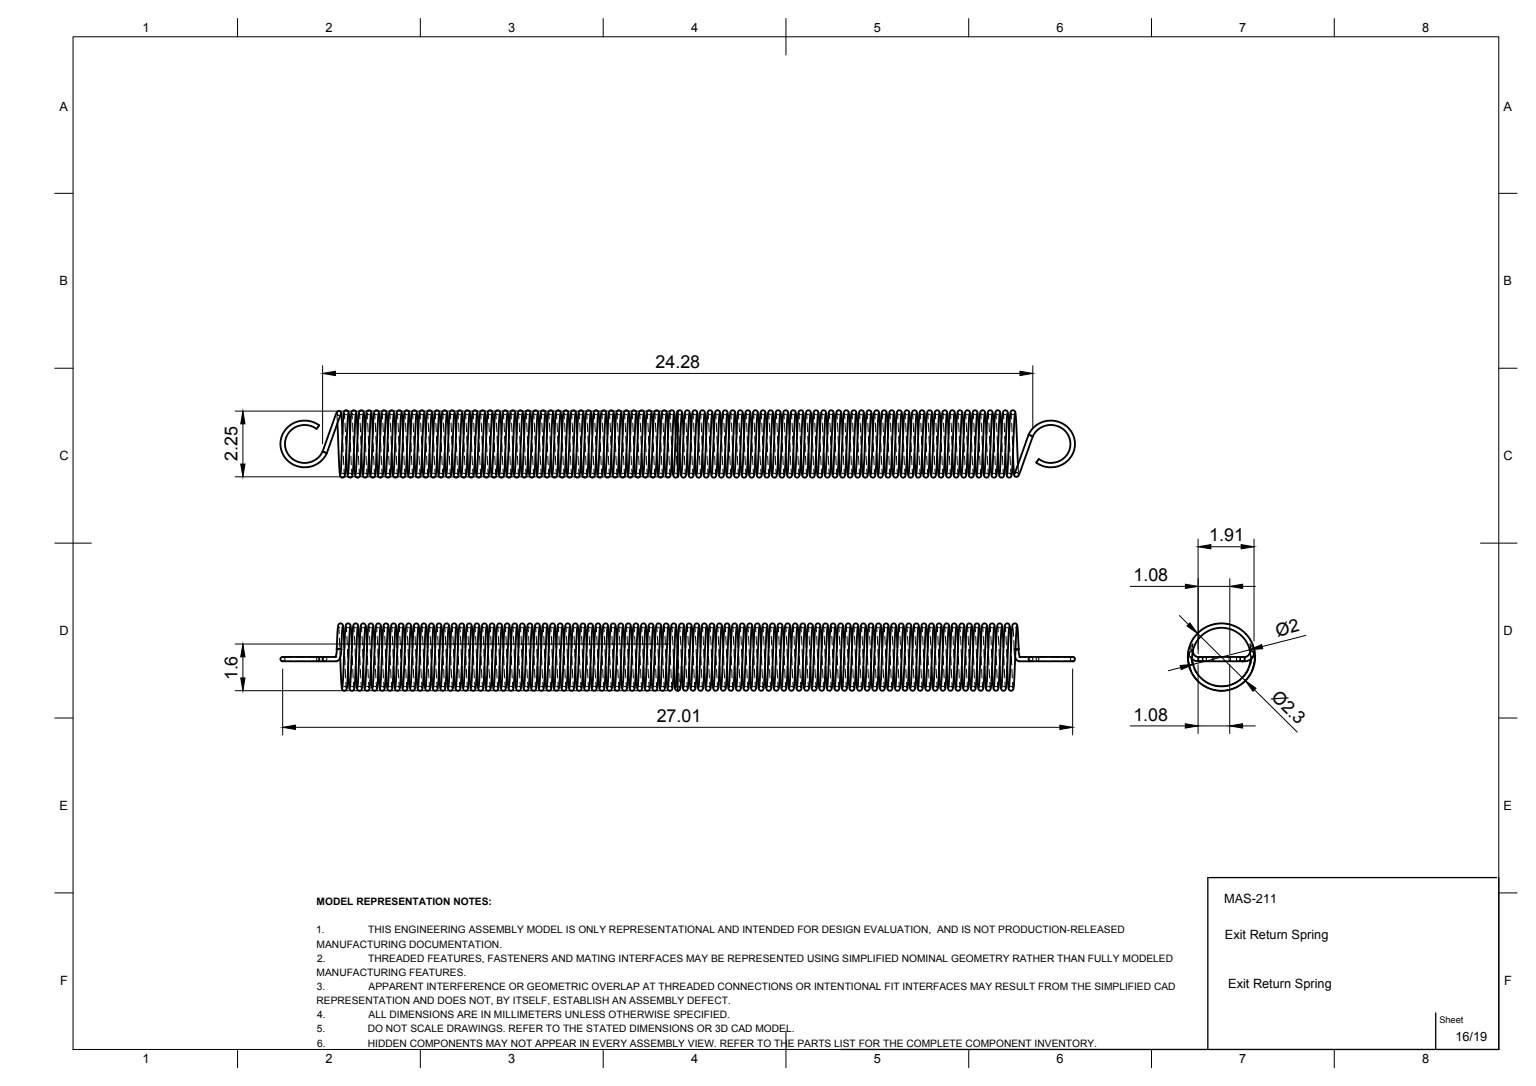
ISO-10303-21;
HEADER;
FILE_DESCRIPTION(
 (''),
 '2;1');
FILE_NAME ( 'Exit Return Spring.step', '2026-10-05T20:07:59+06:00', ( '' ), ( '' ), 'STEP AP214', 'Unspecified', '' );
FILE_SCHEMA (('AUTOMOTIVE_DESIGN { 1 0 10303 214 3 1 1 }'));
ENDSEC;
DATA;
#10=MECHANICAL_DESIGN_GEOMETRIC_PRESENTATION_REPRESENTATION('',(#334),#196741);
#27=(
BOUNDED_CURVE()
B_SPLINE_CURVE(3,(#173354,#173355,#173356,#173357,#173358,#173359,#173360,
#173361,#173362,#173363,#173364,#173365,#173366,#173367,#173368,#173369,
#173370,#173371,#173372,#173373,#173374,#173375,#173376,#173377,#173378,
#173379,#173380,#173381,#173382,#173383,#173384,#173385,#173386,#173387,
#173388,#173389,#173390,#173391,#173392,#173393,#173394,#173395,#173396,
#173397,#173398,#173399,#173400,#173401,#173402,#173403,#173404,#173405,
#173406,#173407,#173408,#173409,#173410,#173411,#173412,#173413,#173414,
#173415,#173416,#173417,#173418,#173419,#173420,#173421,#173422,#173423,
#173424,#173425,#173426,#173427,#173428,#173429,#173430,#173431,#173432,
#173433,#173434,#173435,#173436,#173437,#173438,#173439,#173440,#173441,
#173442,#173443,#173444,#173445,#173446,#173447,#173448,#173449,#173450,
#173451,#173452,#173453,#173454,#173455,#173456,#173457,#173458,#173459,
#173460,#173461,#173462,#173463,#173464,#173465,#173466,#173467,#173468,
#173469,#173470,#173471,#173472,#173473,#173474,#173475,#173476,#173477,
#173478,#173479,#173480,#173481,#173482,#173483,#173484,#173485,#173486,
#173487,#173488,#173489,#173490,#173491,#173492,#173493,#173494,#173495,
#173496,#173497,#173498,#173499,#173500,#173501,#173502,#173503,#173504,
#173505,#173506,#173507,#173508,#173509,#173510,#173511,#173512,#173513,
#173514,#173515,#173516,#173517,#173518,#173519,#173520,#173521,#173522,
#173523,#173524,#173525,#173526,#173527,#173528,#173529,#173530,#173531,
#173532,#173533,#173534,#173535,#173536,#173537,#173538,#173539,#173540,
#173541,#173542,#173543,#173544,#173545,#173546,#173547,#173548,#173549,
#173550,#173551,#173552,#173553,#173554,#173555,#173556,#173557,#173558,
#173559,#173560,#173561,#173562,#173563,#173564,#173565,#173566,#173567,
#173568,#173569,#173570,#173571,#173572,#173573,#173574,#173575,#173576,
#173577,#173578,#173579,#173580,#173581,#173582,#173583,#173584,#173585,
#173586,#173587,#173588,#173589,#173590,#173591,#173592,#173593,#173594,
#173595,#173596,#173597,#173598,#173599,#173600,#173601,#173602,#173603,
#173604,#173605,#173606,#173607,#173608,#173609,#173610,#173611,#173612,
#173613,#173614,#173615,#173616,#173617,#173618,#173619,#173620,#173621,
#173622,#173623,#173624,#173625,#173626,#173627,#173628,#173629,#173630,
#173631,#173632,#173633,#173634,#173635,#173636,#173637,#173638,#173639,
#173640,#173641,#173642,#173643,#173644,#173645,#173646,#173647,#173648,
#173649,#173650,#173651,#173652,#173653,#173654,#173655,#173656,#173657,
#173658,#173659,#173660,#173661,#173662,#173663,#173664,#173665,#173666,
#173667,#173668,#173669,#173670,#173671,#173672,#173673,#173674,#173675,
#173676,#173677,#173678,#173679,#173680,#173681,#173682,#173683,#173684,
#173685,#173686,#173687,#173688,#173689,#173690,#173691,#173692,#173693,
#173694,#173695,#173696,#173697,#173698,#173699,#173700,#173701,#173702,
#173703,#173704,#173705,#173706,#173707,#173708,#173709,#173710,#173711,
#173712,#173713,#173714,#173715,#173716,#173717,#173718,#173719,#173720,
#173721,#173722,#173723,#173724,#173725,#173726,#173727,#173728,#173729,
#173730,#173731,#173732,#173733,#173734,#173735,#173736,#173737,#173738,
#173739,#173740,#173741,#173742,#173743,#173744,#173745,#173746,#173747,
#173748,#173749,#173750,#173751,#173752,#173753,#173754,#173755,#173756,
#173757,#173758,#173759,#173760,#173761,#173762,#173763,#173764,#173765,
#173766,#173767,#173768,#173769,#173770,#173771,#173772,#173773,#173774,
#173775,#173776,#173777,#173778,#173779,#173780,#173781,#173782,#173783,
#173784,#173785,#173786,#173787,#173788,#173789,#173790,#173791,#173792,
#173793,#173794,#173795,#173796,#173797,#173798,#173799,#173800,#173801,
#173802,#173803,#173804,#173805,#173806,#173807,#173808,#173809,#173810,
#173811,#173812,#173813,#173814,#173815,#173816,#173817,#173818,#173819,
#173820,#173821,#173822,#173823,#173824,#173825,#173826,#173827,#173828,
#173829,#173830,#173831,#173832,#173833,#173834,#173835,#173836,#173837,
#173838,#173839,#173840,#173841,#173842,#173843,#173844,#173845,#173846,
#173847,#173848,#173849,#173850,#173851,#173852,#173853,#173854,#173855,
#173856,#173857,#173858,#173859,#173860,#173861,#173862,#173863,#173864,
#173865,#173866,#173867,#173868,#173869,#173870,#173871,#173872,#173873,
#173874,#173875,#173876,#173877,#173878,#173879,#173880,#173881,#173882,
#173883,#173884,#173885,#173886,#173887,#173888,#173889,#173890,#173891,
#173892,#173893,#173894,#173895,#173896,#173897,#173898,#173899,#173900,
#173901,#173902,#173903,#173904,#173905,#173906,#173907,#173908,#173909,
#173910,#173911,#173912,#173913,#173914,#173915,#173916,#173917,#173918,
#173919,#173920,#173921,#173922,#173923,#173924,#173925,#173926,#173927,
#173928,#173929,#173930,#173931,#173932,#173933,#173934,#173935,#173936,
#173937,#173938,#173939,#173940,#173941,#173942,#173943,#173944,#173945,
#173946,#173947,#173948,#173949,#173950,#173951,#173952,#173953,#173954,
#173955,#173956,#173957,#173958,#173959,#173960,#173961,#173962,#173963,
#173964,#173965,#173966,#173967,#173968,#173969,#173970,#173971,#173972,
#173973,#173974,#173975,#173976,#173977,#173978,#173979,#173980,#173981,
#173982,#173983,#173984,#173985,#173986,#173987,#173988,#173989,#173990,
#173991,#173992,#173993,#173994,#173995,#173996,#173997,#173998,#173999,
#174000,#174001,#174002,#174003,#174004,#174005,#174006,#174007,#174008,
#174009,#174010,#174011,#174012,#174013,#174014,#174015,#174016,#174017,
#174018,#174019,#174020,#174021,#174022,#174023,#174024,#174025,#174026,
#174027,#174028,#174029,#174030,#174031,#174032,#174033,#174034,#174035,
#174036,#174037,#174038,#174039,#174040,#174041,#174042,#174043,#174044,
#174045,#174046,#174047,#174048,#174049,#174050,#174051,#174052,#174053,
#174054,#174055,#174056,#174057,#174058,#174059,#174060,#174061,#174062,
#174063,#174064,#174065,#174066,#174067,#174068,#174069,#174070,#174071,
#174072,#174073,#174074,#174075,#174076,#174077,#174078,#174079,#174080,
#174081,#174082,#174083,#174084,#174085,#174086,#174087,#174088,#174089,
#174090,#174091,#174092,#174093,#174094,#174095,#174096,#174097,#174098,
#174099,#174100,#174101,#174102,#174103,#174104,#174105,#174106,#174107,
#174108,#174109,#174110,#174111,#174112,#174113,#174114,#174115,#174116,
#174117,#174118,#174119,#174120,#174121,#174122,#174123,#174124,#174125,
#174126,#174127,#174128,#174129,#174130,#174131,#174132,#174133,#174134,
#174135,#174136,#174137,#174138,#174139,#174140,#174141,#174142,#174143,
#174144,#174145,#174146,#174147,#174148,#174149,#174150,#174151,#174152,
#174153,#174154,#174155,#174156,#174157,#174158,#174159,#174160,#174161,
#174162,#174163,#174164,#174165,#174166,#174167,#174168,#174169,#174170,
#174171,#174172,#174173,#174174,#174175,#174176,#174177,#174178,#174179,
#174180,#174181,#174182,#174183,#174184,#174185,#174186,#174187,#174188,
#174189,#174190,#174191,#174192,#174193,#174194,#174195,#174196,#174197,
#174198,#174199,#174200,#174201,#174202,#174203,#174204,#174205,#174206,
#174207,#174208,#174209,#174210,#174211,#174212,#174213,#174214,#174215,
#174216,#174217,#174218,#174219,#174220,#174221,#174222,#174223,#174224,
#174225,#174226,#174227,#174228,#174229,#174230,#174231,#174232,#174233,
#174234,#174235,#174236,#174237,#174238,#174239,#174240,#174241,#174242,
#174243,#174244,#174245,#174246,#174247,#174248,#174249,#174250,#174251,
#174252,#174253,#174254,#174255,#174256,#174257,#174258,#174259,#174260,
#174261,#174262,#174263,#174264,#174265,#174266,#174267,#174268,#174269,
#174270,#174271,#174272,#174273,#174274,#174275,#174276,#174277,#174278,
#174279,#174280,#174281,#174282,#174283,#174284,#174285,#174286,#174287,
#174288,#174289,#174290,#174291,#174292,#174293,#174294,#174295,#174296,
#174297,#174298,#174299,#174300,#174301,#174302,#174303,#174304,#174305,
#174306,#174307,#174308,#174309,#174310,#174311,#174312,#174313,#174314,
#174315,#174316,#174317,#174318,#174319,#174320,#174321,#174322,#174323,
#174324,#174325,#174326,#174327,#174328,#174329,#174330,#174331,#174332,
#174333,#174334,#174335,#174336,#174337,#174338,#174339,#174340,#174341,
#174342,#174343,#174344,#174345,#174346,#174347,#174348,#174349,#174350,
#174351,#174352,#174353,#174354,#174355,#174356,#174357,#174358,#174359,
#174360,#174361,#174362,#174363,#174364,#174365,#174366,#174367,#174368,
#174369,#174370,#174371,#174372,#174373,#174374,#174375,#174376,#174377,
#174378,#174379,#174380,#174381,#174382,#174383,#174384,#174385,#174386,
#174387,#174388,#174389,#174390,#174391,#174392,#174393,#174394,#174395,
#174396,#174397,#174398,#174399,#174400,#174401,#174402,#174403,#174404,
#174405,#174406,#174407,#174408,#174409,#174410,#174411),.UNSPECIFIED.,
 .F.,.F.)
B_SPLINE_CURVE_WITH_KNOTS((4,1,1,1,1,1,1,1,1,1,1,1,1,1,1,1,1,1,1,1,1,1,
1,1,1,1,1,1,1,1,1,1,1,1,1,1,1,1,1,1,1,1,1,1,1,1,1,1,1,1,1,1,1,1,1,1,1,1,
1,1,1,1,1,1,1,1,1,1,1,1,1,1,1,1,1,1,1,1,1,1,1,1,1,1,1,1,1,1,1,1,1,1,1,1,
1,1,1,1,1,1,1,1,1,1,1,1,1,1,1,1,1,1,1,1,1,1,1,1,1,1,1,1,1,1,1,1,1,1,1,1,
1,1,1,1,1,1,1,1,1,1,1,1,1,1,1,1,1,1,1,1,1,1,1,1,1,1,1,1,1,1,1,1,1,1,1,1,
1,1,1,1,1,1,1,1,1,1,1,1,1,1,1,1,1,1,1,1,1,1,1,1,1,1,1,1,1,1,1,1,1,1,1,1,
1,1,1,1,1,1,1,1,1,1,1,1,1,1,1,1,1,1,1,1,1,1,1,1,1,1,1,1,1,1,1,1,1,1,1,1,
1,1,1,1,1,1,1,1,1,1,1,1,1,1,1,1,1,1,1,1,1,1,1,1,1,1,1,1,1,1,1,1,1,1,1,1,
1,1,1,1,1,1,1,1,1,1,1,1,1,1,1,1,1,1,1,1,1,1,1,1,1,1,1,1,1,1,1,1,1,1,1,1,
1,1,1,1,1,1,1,1,1,1,1,1,1,1,1,1,1,1,1,1,1,1,1,1,1,1,1,1,1,1,1,1,1,1,1,1,
1,1,1,1,1,1,1,1,1,1,1,1,1,1,1,1,1,1,1,1,1,1,1,1,1,1,1,1,1,1,1,1,1,1,1,1,
1,1,1,1,1,1,1,1,1,1,1,1,1,1,1,1,1,1,1,1,1,1,1,1,1,1,1,1,1,1,1,1,1,1,1,1,
1,1,1,1,1,1,1,1,1,1,1,1,1,1,1,1,1,1,1,1,1,1,1,1,1,1,1,1,1,1,1,1,1,1,1,1,
1,1,1,1,1,1,1,1,1,1,1,1,1,1,1,1,1,1,1,1,1,1,1,1,1,1,1,1,1,1,1,1,1,1,1,1,
1,1,1,1,1,1,1,1,1,1,1,1,1,1,1,1,1,1,1,1,1,1,1,1,1,1,1,1,1,1,1,1,1,1,1,1,
1,1,1,1,1,1,1,1,1,1,1,1,1,1,1,1,1,1,1,1,1,1,1,1,1,1,1,1,1,1,1,1,1,1,1,1,
1,1,1,1,1,1,1,1,1,1,1,1,1,1,1,1,1,1,1,1,1,1,1,1,1,1,1,1,1,1,1,1,1,1,1,1,
1,1,1,1,1,1,1,1,1,1,1,1,1,1,1,1,1,1,1,1,1,1,1,1,1,1,1,1,1,1,1,1,1,1,1,1,
1,1,1,1,1,1,1,1,1,1,1,1,1,1,1,1,1,1,1,1,1,1,1,1,1,1,1,1,1,1,1,1,1,1,1,1,
1,1,1,1,1,1,1,1,1,1,1,1,1,1,1,1,1,1,1,1,1,1,1,1,1,1,1,1,1,1,1,1,1,1,1,1,
1,1,1,1,1,1,1,1,1,1,1,1,1,1,1,1,1,1,1,1,1,1,1,1,1,1,1,1,1,1,1,1,1,1,1,1,
1,1,1,1,1,1,1,1,1,1,1,1,1,1,1,1,1,1,1,1,1,1,1,1,1,1,1,1,1,1,1,1,1,1,1,1,
1,1,1,1,1,1,1,1,1,1,1,1,1,1,1,1,1,1,1,1,1,1,1,1,1,1,1,1,1,1,1,1,1,1,1,1,
1,1,1,1,1,1,1,1,1,1,1,1,1,1,1,1,1,1,1,1,1,1,1,1,1,1,1,1,1,1,1,1,1,1,1,1,
1,1,1,1,1,1,1,1,1,1,1,1,1,1,1,1,1,1,1,1,1,1,1,1,1,1,1,1,1,1,1,1,1,1,1,1,
1,1,1,1,1,1,1,1,1,1,1,1,1,1,1,1,1,1,1,1,1,1,1,1,1,1,1,1,1,1,1,1,1,1,1,1,
1,1,1,1,1,1,1,1,1,1,1,1,1,1,1,1,1,1,1,1,1,1,1,1,1,1,1,1,1,1,1,1,1,1,1,1,
1,1,1,1,1,1,1,1,1,1,1,1,1,1,1,1,1,1,1,1,1,1,1,1,1,1,1,1,1,1,1,1,1,1,1,1,
1,1,1,1,1,1,1,1,1,1,1,1,1,1,1,1,1,1,1,1,1,1,1,1,1,1,1,1,1,1,1,1,1,1,1,1,
1,1,1,1,1,1,1,1,1,1,1,1,1,1,1,1,1,1,1,1,1,1,1,1,1,4),(0.,0.01797683372391,
0.286633051710584,0.555289278308216,0.823945516665782,1.09260176953922,
1.36125803873948,1.62991432588463,1.89857063164012,2.16722695661301,2.43588330050525,
2.70453966304674,2.9731960431531,3.24185243981471,3.51050885133453,3.77916527610465,
4.04782171198515,4.31647815691489,4.58513460847725,4.85379106430677,5.12244752187208,
5.39110397865606,5.65976043217153,5.92841687990537,6.19707331956994,6.46572974881596,
6.73438616570634,7.00304256821933,7.2716989549161,7.5403553242696,7.809011675483,
8.07766800769526,8.34632432089157,8.61498061505147,8.8836368910788,9.15229314997201,
9.4209493936865,9.68960562442157,9.95826184531348,10.226918059948,10.4955742727586,
10.7642304884925,11.0328867113173,11.3015429448574,11.5701991918227,11.8388554546081,
12.1075117346518,12.3761680332469,12.6448243507434,12.9134806874637,13.1821370428496,
13.450793416388,13.7194498067883,13.9881062128412,14.2567626326955,14.5254190645885,
14.7940755062772,15.0627319555912,15.3313884100611,15.6000448672586,15.8687013246492,
16.1373577797,16.4060142299691,16.6746706729765,16.9433271065265,17.2119835283531,
17.4806399366567,17.7492963295502,18.0179527057767,18.286609063996,18.555265403637,
18.8239217240786,19.0925780255742,19.3612343083975,19.6298905737625,19.898546823017,
20.1672030584666,20.4358592827168,20.7045154992928,20.973171712245,21.2418279262962,
21.5104841459723,21.7791403749736,22.0477966165324,22.316452872948,22.585109146262,
22.8537654375589,23.1224217478187,23.3910780770929,23.6597344254327,23.9283907920352,
24.197047176159,24.4657035763222,24.7343599911301,25.0030164185931,25.2716728568073,
25.5403293034427,25.8089857562333,26.0776422126729,26.3462986702843,26.6149551265448,
26.8836115789212,27.1522680250308,27.4209244624423,27.6895808890659,27.9582373027346,
28.2268937018004,28.4955500845261,28.7642064498512,29.0328627966379,29.3015191245544,
29.5701754332357,29.838831723217,30.1074879950829,30.3761442503694,30.6448004907916,
30.9134567190168,31.1821129380756,31.450769151893,31.7194253649682,31.9880815819663,
32.2567378070174,32.5253940433706,32.7940502938785,33.0627065604467,33.3313628447765,
33.6000191476151,33.8686754696427,34.1373318106287,34.405988170366,34.6746445478242,
34.9433009420458,35.2119573513747,35.480613774244,35.7492702085419,36.0179266522368,
36.2865831029275,36.5552395582669,36.8238960157264,37.0925524727952,37.3612089269773,
37.6298653757534,37.8985218168153,38.1671782477952,38.4358346667239,38.7044910715485,
38.9731474607866,39.2418038328672,39.5104601869391,39.7791165220837,40.0477728382212,
40.3164291352602,40.5850854140292,40.8537416754418,41.1223979213679,41.3910541539077,
41.6597103761025,41.9283665914244,42.1970228042084,42.4656790192,42.7343352406829,
43.0029914723808,43.2716477171096,43.540303977354,43.8089602546436,44.0776165503516,
44.3462728649052,44.614929198697,44.883585551232,45.1522419220568,45.4208983099307,
45.6895547136931,45.9582111315299,46.2268675617156,46.4955240020317,46.7641804503338,
47.0328369041642,47.3014933611089,47.5701498186329,47.8388062742058,48.107462725373,
48.3761191696448,48.6447756048012,48.9134320285537,49.1820884390673,49.4507448344197,
49.7194012133072,49.9880575743413,50.2567139168934,50.5253702402807,50.7940265446884,
51.0626828303152,51.3313390982961,51.5999953498901,51.8686515873141,52.1373078130706,
52.4059640305862,52.6746202437936,52.9432764573682,53.211932675918,53.480588903259,
53.7492451427202,54.0179013967021,54.2865576673334,54.5552139557853,54.823870263115,
55.0925265894471,55.3611829348992,55.6298392987282,55.8984956802486,56.1671520780245,
56.4358084907065,56.7044649163381,56.9731213530494,57.2417777985307,57.5104342505384,
57.7790907065743,58.0477471641719,58.3164036208043,58.5850600739368,58.8537165211707,
59.1223729600609,59.39102938849,59.6596858042645,59.9283422056975,60.1969985910129,
60.4656549590995,60.7343113087676,61.0029676396243,61.2716239512389,61.540280244075,
61.808936518638,62.0775927763821,62.3462490189291,62.6149052488546,62.8835614690812,
63.1522176834332,63.4208738963055,63.6895301124163,63.9581863359981,64.2268425704115,
64.4954988186027,64.7641550825741,65.0328113641112,65.3014676640435,65.5701239831253,
65.8387803211949,66.1074366781083,66.3760930528907,66.6447494446373,66.9134058517341,
67.1820622726558,67.4507187053199,67.7193751477252,67.988031597487,68.256688052277,
68.5253445095709,68.7940009668648,69.0626574216546,69.3313138714164,69.5999703138218,
69.8686267464858,70.1372831674076,70.4059395745042,70.6745959662509,70.9432523410334,
71.2119086979469,71.4805650360164,71.7492213550982,72.0178776550306,72.2865339365675,
72.5551902005389,72.8238464487301,73.0925026831433,73.3611589067251,73.6298151228357,
73.8984713357081,74.1671275500599,74.4357837702864,74.7044400002118,74.9730962427587,
75.2417525005027,75.5104087750655,75.7790650679015,76.047721379516,76.3163777103726,
76.5850340600405,76.853690428127,77.1223468134422,77.391003214875,77.6596596306495,
77.9283160590784,78.1969724979684,78.4656289452021,78.7342853983344,79.0029418549666,
79.2715983125641,79.5402547685998,79.8089112206075,80.0775676660886,80.3462241027997,
80.6148805284312,80.8835369411131,81.1521933388889,81.4208497204091,81.689506084238,
81.9581624296899,82.2268187560219,82.4954750633515,82.7641313518033,83.0327876224345,
83.3014438764161,83.5701001158772,83.838756343218,84.1074125617677,84.3760687753422,
84.6447249885494,84.913381206065,85.1820374318212,85.4506936692451,85.719349920839,
85.9880061888197,86.2566624744465,86.5253187788541,86.7939751022413,87.0626314447932,
87.3312878058273,87.5999441847146,87.8686005800667,88.1372569905802,88.4059134143327,
88.6745698494889,88.9432262937606,89.2118827449277,89.4805392005005,89.7491956580243,
90.0178521149689,90.2865085687992,90.5551650171012,90.8238214574172,91.0924778876028,
91.3611343054394,91.6297907092016,91.8984470970753,92.1671034679,92.4357598204347,
92.7044161542264,92.9730724687798,93.2417287644878,93.5103850417773,93.7790413020216,
94.0476975467502,94.3163537784479,94.5850099999307,94.8536662149221,95.1223224277061,
95.390978643028,95.6596348652226,95.9282910977624,96.1969473436883,96.4656036051009,
96.7342598838697,97.0029161809086,97.2715724970461,97.5402288321905,97.8088851862623,
98.0775415583427,98.3461979475807,98.6148543524051,98.8835107713336,99.1521672023136,
99.4208236433754,99.6894800921513,99.9581365463333,100.226793003402,100.495449460861,
100.7641059162,101.032762366891,101.301418810586,101.570075244884,101.838731667753,
102.107388077082,102.376044471303,102.644700848761,102.913357208498,103.182013549484,
103.450669871511,103.71932617435,103.98798245868,104.256638725248,104.525294975755,
104.793951212108,105.062607437159,105.331263654157,105.599919867233,105.86857608105,
106.137232300108,106.405888528334,106.674544768756,106.943201024042,107.211857295908,
107.480513585889,107.74916989457,108.017826222487,108.286482569273,108.555138934598,
108.823795317324,109.09245171639,109.361108130058,109.629764556682,109.898420994093,
110.167077440202,110.435733892579,110.704390348839,110.97304680645,111.24170326289,
111.51035971568,111.779016162316,112.04767260053,112.316329027993,112.5849854428,
112.853641842963,113.122298227087,113.39095459369,113.659610942029,113.928267271303,
114.196923581563,114.46557987286,114.734236146174,115.002892402589,115.271548644148,
115.540204873149,115.808861092825,116.077517306876,116.346173519828,116.614829736404,
116.883485960654,117.152142196103,117.420798445358,117.689454710722,117.958110993546,
118.226767295041,118.495423615483,118.764079955123,119.032736313343,119.301392689569,
119.570049082462,119.838705490766,120.107361912592,120.376018346142,120.644674789149,
120.913331239418,121.181987694469,121.45064415186,121.719300609057,121.987957063527,
122.256613512841,122.525269954529,122.793926386422,123.062582806276,123.331239212329,
123.599895602729,123.868551976268,124.137208331653,124.405864668374,124.67452098587,
124.943177284465,125.211833564508,125.480489827294,125.749146074259,126.017802307799,
126.286458530624,126.555114746357,126.823770959168,127.092427173802,127.361083394694,
127.629739625429,127.898395869143,128.167052128037,128.435708404064,128.704364698224,
128.97302101142,129.241677343633,129.510333694846,129.7789900642,130.047646450897,
130.31630285341,130.5849592703,130.853615699547,131.122272139211,131.390928586945,
131.659585040461,131.928241497245,132.19689795481,132.46555441064,132.734210862202,
133.002867307132,133.271523743013,133.540180167783,133.808836579303,134.077492975965,
134.346149356071,134.614805718613,134.883462062505,135.152118387478,135.420774693234,
135.689430980379,135.958087249579,136.226743502453,136.49539974081,136.76405596741,
137.032712185392,137.301368398783,137.570024612174,137.838680830155,138.107337056755,
138.375993295112,138.644649547986,138.913305817186,139.181962104332,139.450618410087,
139.71927473506,139.987931078952,140.256587441494,140.525243821601,140.793900218262,
141.062556629782,141.331213054552,141.599869490433,141.868525935363,142.137182386925,
142.405838842755,142.67449530032,142.943151757104,143.21180821062,143.480464658354,
143.749121098019,144.017777527265,144.286433944155,144.555090346668,144.823746733365,
145.092403102719,145.361059453932,145.629715786145,145.898372099341,146.167028393501,
146.435684669529,146.704340928422,146.972997172137,147.241653402872,147.510309623764,
147.778965838398,148.047622051209,148.316278266943,148.584934489768,148.853590723308,
149.122246970274,149.390903233059,149.659559513103,149.928215811698,150.196872129195,
150.465528465915,150.734184821301,151.00284119484,151.27149758524,151.540153991293,
151.808810411148,152.077466843041,152.34612328473,152.614779734044,152.883436188514,
153.152092645711,153.420749103102,153.689405558153,153.958062008422,154.22671845143,
154.49537488498,154.764031306806,155.03268771511,155.301344108004,155.57000048423,
155.838656842449,156.107313182091,156.375969502532,156.644625804028,156.913282086851,
157.181938352216,157.450594601471,157.719250836921,157.987907061171,158.256563277747,
158.525219490699,158.793875704751,159.062531924427,159.331188153428,159.599844394987,
159.868500651403,160.137156924717,160.405813216014,160.674469526274,160.943125855548,
161.211782203888,161.480438570491,161.749094954615,162.017751354778,162.286407769586,
162.555064197049,162.823720635263,163.092377081899,163.361033534689,163.629689991129,
163.898346448741,164.167002905001,164.435659357378,164.704315803488,164.972972240899,
165.241628667523,165.510285081192,165.778941480257,166.047597862983,166.316254228308,
166.584910575095,166.853566903012,167.122223211693,167.390879501675,167.659535773541,
167.928192028827,168.19684826925,168.465504497475,168.734160716534,169.002816930351,
169.271473143427,169.540129360425,169.808785585476,170.077441821829,170.346098072337,
170.614754338905,170.883410623235,171.152066926074,171.420723248102,171.689379589088,
171.958035948825,172.226692326284,172.495348720505,172.764005129834,173.032661552704,
173.301317987002,173.569974430697,173.838630881388,174.107287336727,174.375943794187,
174.644600251255,174.913256705437,175.181913154214,175.450569595276,175.719226026256,
175.987882445184,176.256538850009,176.525195239247,176.793851611328,177.0625079654,
177.331164300545,177.599820616682,177.868476913721,178.137133192491,178.405789453903,
178.674445699829,178.943101932369,179.211758154564,179.480414369886,179.74907058267,
180.017726797662,180.286383019145,180.555039250843,180.823695495572,181.092351755816,
181.361008033106,181.629664328814,181.898320643368,182.16697697716,182.435633329695,
182.70428970052,182.972946088394,183.241602492156,183.510258909993,183.778915340179,
184.047571780495,184.316228228797,184.584884682628,184.853541139572,185.122197597096,
185.39085405267,185.659510503837,185.928166948109,186.196823383265,186.465479807018,
186.734136217531,187.002792612884,187.271448991771,187.540105352806,187.808761695358,
188.077418018745,188.346074323153,188.61473060878,188.883386876761,189.152043128355,
189.420699365779,189.689355591536,189.958011809051,190.226668022259,190.495324235834,
190.763980454383,191.032636681725,191.301292921186,191.569949175168,191.838605445799,
192.107261734251,192.375918041581,192.644574367913,192.913230713365,193.181887077194,
193.450543458715,193.719199856491,193.987856269173,194.256512694805,194.525169131516,
194.793825576997,195.062482029005,195.331138485041,195.599794942639,195.868451399271,
196.137107852404,196.405764299638,196.674420738528,196.943077166957,197.211733582732,
197.480389984165,197.749046369481,198.017702737567,198.286359087236,198.555015418092,
198.823671729707,199.092328022543,199.360984297106,199.62964055485,199.898296797397,
200.166953027323,200.43560924755,200.704265461902,200.972921674774,201.241577890885,
201.510234114467,201.77889034888,202.047546597072,202.316202861043,202.584859142581,
202.853515442513,203.122171761595,203.390828099665,203.659484456579,203.928140831361,
204.196797223108,204.465453630205,204.734110051127,205.002766483791,205.271422926197,
205.540079375959,205.808735830749,206.077392288043,206.346048745337,206.614705200127,
206.883361649889,207.152018092295,207.420674524959,207.689330945881,207.957987352978,
208.226643744725,208.495300119508,208.763956476421,209.032612814491,209.301269133573,
209.569925433505,209.838581715043,210.107237979014,210.375894227206,210.644550461619,
210.913206685201,211.181862901312,211.450519114184,211.719175328536,211.987831548763,
212.256487778689,212.525144021236,212.79380027898,213.062456553543,213.331112846379,
213.599769157994,213.868425488851,214.137081838519,214.405738206606,214.674394591921,
214.943050993354,215.211707409129,215.480363837558,215.749020276448,216.017676723682,
216.286333176815,216.554989633447,216.823646091045,217.092302547081,217.360958999089,
217.62961544457,217.898271881281,218.166928306913,218.435584719595,218.704241117371,
218.972897498892,219.241553862721,219.510210208173,219.778866534505,220.047522841835,
220.316179130287,220.584835400918,220.8534916549,221.122147894361,221.390804121702,
221.659460340252,221.928116553827,222.196772767034,222.46542898455,222.734085210306,
223.00274144773,223.271397699324,223.540053967305,223.808710252932,224.07736655734,
224.346022880728,224.61467922328,224.883335584314,225.151991963201,225.420648358554,
225.689304769068,225.95796119282,226.226617627977,226.495274072249,226.763930523416,
227.032586978989,227.301243436513,227.569899893458,227.838556347288,228.10721279559,
228.375869235907,228.644525666093,228.913182083929,229.181838487692,229.450494875566,
229.719151246391,229.987807598926,230.256463932718,230.525120247271,230.79377654298,
231.062432820269,231.331089080514,231.599745325243,231.868401556941,232.137057778424,
232.405713993415,232.674370206199,232.943026421521,233.211682643716,233.480338876256,
233.748995122182,234.017651383595,234.286307662364,234.554963959403,234.823620275541,
235.092276610685,235.360932964757,235.629589336838,235.898245726076,236.166902130901,
236.43555854983,236.70421498081,236.972871421872,237.241527870648,237.51018432483,
237.778840781899,238.047497239359,238.316153694698,238.584810145389,238.853466589084,
239.122123023382,239.390779446251,239.65943585558,239.928092249802,240.19674862726,
240.465404986998,240.734061327984,241.002717650011,241.27137395285,241.54003023718,
241.808686503748,242.077342754256,242.345998990609,242.614655215661,242.883311432659,
243.151967645734,243.420623859552,243.68928007861,243.957936306836,244.226592547258,
244.495248802545,244.763905074411,245.032561364392,245.301217673074,245.56987400099,
245.838530347777,246.107186713102,246.375843095828,246.644499494894,246.913155908563,
247.181812335186,247.450468772598,247.719125218708,247.987781671084,248.256438127345,
248.525094584956,248.793751041396,249.062407494187,249.331063940822,249.599720379036,
249.8683768065,250.137033221308,250.405689621471,250.674346005595,250.943002372197,
251.211658720537,251.480315049812,251.748971360071,252.017627651368,252.286283924683,
252.554940181098,252.823596422657,253.092252651658,253.360908871335,253.629565085386,
253.898221298338,254.166877514914,254.435533739165,254.704189974614,254.972846223869,
255.241502489234,255.510158772057,255.778815073553,256.047471393995,256.316127733635,
256.584784091854,256.85344046808,257.122096860973,257.390753269276,257.659409691102,
257.928066124652,258.196722567659,258.465379017928,258.734035472978,259.002691930368,
259.271348387566,259.540004842035,259.808661291349,260.077317733037,260.345974164929,
260.614630584783,260.883286990836,261.151943381235,261.420599754774,261.689256110159,
261.957912446879,262.226568764375,262.49522506297,262.763881343014,263.032537605798,
263.301193852763,263.569850086303,263.838506309127,264.107162524861,264.375818737671,
264.644474952305,264.913131173196,265.181787403931,265.450443647645,265.719099906538,
265.987756182565,266.256412476724,266.52506878992,266.793725122132,267.062381473345,
267.331037842698,267.599694229394,267.868350631907,268.137007048797,268.405663478042,
268.674319917706,268.94297636544,269.211632818955,269.480289275739,269.748945733304,
270.017602189133,270.286258640695,270.554915085624,270.823571521504,271.092227946274,
271.360884357793,271.629540754454,271.89819713456,272.166853497101,272.435509840993,
272.704166165965,272.97282247172,273.241478758865,273.510135028065,273.778791280938,
274.047447519295,274.316103745894,274.584759963875,274.853416177266,275.122072390656,
275.390728608637,275.659384835237,275.928041073593,276.196697326466,276.465353595666,
276.734009882811,277.002666188566,277.271322513539,277.53997885743,277.808635219972,
278.077291600077,278.345947996739,278.614604408258,278.883260833028,279.151917268908,
279.420573713837,279.689230165399,279.957886621228,280.226543078793,280.495199535576,
280.763855989092,281.032512436825,281.301168876489,281.569825305735,281.838481722625,
282.107138125138,282.375794511834,282.644450881187,282.9131072324,283.140531716307),
 .UNSPECIFIED.)
CURVE()
GEOMETRIC_REPRESENTATION_ITEM()
RATIONAL_B_SPLINE_CURVE((1.,1.,1.,1.,1.,1.,1.,1.,1.,1.,1.,1.,1.,1.,1.,1.,
1.,1.,1.,1.,1.,1.,1.,1.,1.,1.,1.,1.,1.,1.,1.,1.,1.,1.,1.,1.,1.,1.,1.,1.,
1.,1.,1.,1.,1.,1.,1.,1.,1.,1.,1.,1.,1.,1.,1.,1.,1.,1.,1.,1.,1.,1.,1.,1.,
1.,1.,1.,1.,1.,1.,1.,1.,1.,1.,1.,1.,1.,1.,1.,1.,1.,1.,1.,1.,1.,1.,1.,1.,
1.,1.,1.,1.,1.,1.,1.,1.,1.,1.,1.,1.,1.,1.,1.,1.,1.,1.,1.,1.,1.,1.,1.,1.,
1.,1.,1.,1.,1.,1.,1.,1.,1.,1.,1.,1.,1.,1.,1.,1.,1.,1.,1.,1.,1.,1.,1.,1.,
1.,1.,1.,1.,1.,1.,1.,1.,1.,1.,1.,1.,1.,1.,1.,1.,1.,1.,1.,1.,1.,1.,1.,1.,
1.,1.,1.,1.,1.,1.,1.,1.,1.,1.,1.,1.,1.,1.,1.,1.,1.,1.,1.,1.,1.,1.,1.,1.,
1.,1.,1.,1.,1.,1.,1.,1.,1.,1.,1.,1.,1.,1.,1.,1.,1.,1.,1.,1.,1.,1.,1.,1.,
1.,1.,1.,1.,1.,1.,1.,1.,1.,1.,1.,1.,1.,1.,1.,1.,1.,1.,1.,1.,1.,1.,1.,1.,
1.,1.,1.,1.,1.,1.,1.,1.,1.,1.,1.,1.,1.,1.,1.,1.,1.,1.,1.,1.,1.,1.,1.,1.,
1.,1.,1.,1.,1.,1.,1.,1.,1.,1.,1.,1.,1.,1.,1.,1.,1.,1.,1.,1.,1.,1.,1.,1.,
1.,1.,1.,1.,1.,1.,1.,1.,1.,1.,1.,1.,1.,1.,1.,1.,1.,1.,1.,1.,1.,1.,1.,1.,
1.,1.,1.,1.,1.,1.,1.,1.,1.,1.,1.,1.,1.,1.,1.,1.,1.,1.,1.,1.,1.,1.,1.,1.,
1.,1.,1.,1.,1.,1.,1.,1.,1.,1.,1.,1.,1.,1.,1.,1.,1.,1.,1.,1.,1.,1.,1.,1.,
1.,1.,1.,1.,1.,1.,1.,1.,1.,1.,1.,1.,1.,1.,1.,1.,1.,1.,1.,1.,1.,1.,1.,1.,
1.,1.,1.,1.,1.,1.,1.,1.,1.,1.,1.,1.,1.,1.,1.,1.,1.,1.,1.,1.,1.,1.,1.,1.,
1.,1.,1.,1.,1.,1.,1.,1.,1.,1.,1.,1.,1.,1.,1.,1.,1.,1.,1.,1.,1.,1.,1.,1.,
1.,1.,1.,1.,1.,1.,1.,1.,1.,1.,1.,1.,1.,1.,1.,1.,1.,1.,1.,1.,1.,1.,1.,1.,
1.,1.,1.,1.,1.,1.,1.,1.,1.,1.,1.,1.,1.,1.,1.,1.,1.,1.,1.,1.,1.,1.,1.,1.,
1.,1.,1.,1.,1.,1.,1.,1.,1.,1.,1.,1.,1.,1.,1.,1.,1.,1.,1.,1.,1.,1.,1.,1.,
1.,1.,1.,1.,1.,1.,1.,1.,1.,1.,1.,1.,1.,1.,1.,1.,1.,1.,1.,1.,1.,1.,1.,1.,
1.,1.,1.,1.,1.,1.,1.,1.,1.,1.,1.,1.,1.,1.,1.,1.,1.,1.,1.,1.,1.,1.,1.,1.,
1.,1.,1.,1.,1.,1.,1.,1.,1.,1.,1.,1.,1.,1.,1.,1.,1.,1.,1.,1.,1.,1.,1.,1.,
1.,1.,1.,1.,1.,1.,1.,1.,1.,1.,1.,1.,1.,1.,1.,1.,1.,1.,1.,1.,1.,1.,1.,1.,
1.,1.,1.,1.,1.,1.,1.,1.,1.,1.,1.,1.,1.,1.,1.,1.,1.,1.,1.,1.,1.,1.,1.,1.,
1.,1.,1.,1.,1.,1.,1.,1.,1.,1.,1.,1.,1.,1.,1.,1.,1.,1.,1.,1.,1.,1.,1.,1.,
1.,1.,1.,1.,1.,1.,1.,1.,1.,1.,1.,1.,1.,1.,1.,1.,1.,1.,1.,1.,1.,1.,1.,1.,
1.,1.,1.,1.,1.,1.,1.,1.,1.,1.,1.,1.,1.,1.,1.,1.,1.,1.,1.,1.,1.,1.,1.,1.,
1.,1.,1.,1.,1.,1.,1.,1.,1.,1.,1.,1.,1.,1.,1.,1.,1.,1.,1.,1.,1.,1.,1.,1.,
1.,1.,1.,1.,1.,1.,1.,1.,1.,1.,1.,1.,1.,1.,1.,1.,1.,1.,1.,1.,1.,1.,1.,1.,
1.,1.,1.,1.,1.,1.,1.,1.,1.,1.,1.,1.,1.,1.,1.,1.,1.,1.,1.,1.,1.,1.,1.,1.,
1.,1.,1.,1.,1.,1.,1.,1.,1.,1.,1.,1.,1.,1.,1.,1.,1.,1.,1.,1.,1.,1.,1.,1.,
1.,1.,1.,1.,1.,1.,1.,1.,1.,1.,1.,1.,1.,1.,1.,1.,1.,1.,1.,1.,1.,1.,1.,1.,
1.,1.,1.,1.,1.,1.,1.,1.,1.,1.,1.,1.,1.,1.,1.,1.,1.,1.,1.,1.,1.,1.,1.,1.,
1.,1.,1.,1.,1.,1.,1.,1.,1.,1.,1.,1.,1.,1.,1.,1.,1.,1.,1.,1.,1.,1.,1.,1.,
1.,1.,1.,1.,1.,1.,1.,1.,1.,1.,1.,1.,1.,1.,1.,1.,1.,1.,1.,1.,1.,1.,1.,1.,
1.,1.,1.,1.,1.,1.,1.,1.,1.,1.,1.,1.,1.,1.,1.,1.,1.,1.,1.,1.,1.,1.,1.,1.,
1.,1.,1.,1.,1.,1.,1.,1.,1.,1.,1.,1.,1.,1.,1.,1.,1.,1.,1.,1.,1.,1.,1.,1.,
1.,1.,1.,1.,1.,1.,1.,1.,1.,1.,1.,1.,1.,1.,1.,1.,1.,1.,1.,1.,1.,1.,1.,1.,
1.,1.,1.,1.,1.,1.,1.,1.,1.,1.,1.,1.,1.,1.,1.,1.,1.,1.,1.,1.,1.,1.,1.,1.,
1.,1.,1.,1.,1.,1.,1.,1.,1.,1.,1.,1.,1.,1.,1.,1.,1.,1.,1.,1.,1.,1.,1.,1.,
1.,1.,1.,1.,1.,1.,1.,1.,1.,1.,1.,1.,1.,1.,1.,1.,1.,1.,1.,1.,1.,1.,1.,1.,
1.,1.,1.,1.,1.,1.,1.,1.,1.,1.,1.,1.,1.,1.,1.,1.,1.,1.,1.,1.,1.,1.,1.,1.,
1.,1.,1.,1.,1.,1.,1.,1.,1.,1.))
REPRESENTATION_ITEM('')
) ;
#28=(
BOUNDED_CURVE()
B_SPLINE_CURVE(3,(#174481,#174482,#174483,#174484,#174485,#174486,#174487),
 .UNSPECIFIED.,.F.,.F.)
B_SPLINE_CURVE_WITH_KNOTS((4,1,1,1,4),(0.,0.0911446219616379,0.182289243923276,
0.273433865884915,0.364578487846551),.UNSPECIFIED.)
CURVE()
GEOMETRIC_REPRESENTATION_ITEM()
RATIONAL_B_SPLINE_CURVE((1.,1.,1.,1.,1.,1.,1.))
REPRESENTATION_ITEM('')
) ;
#29=(
BOUNDED_CURVE()
B_SPLINE_CURVE(3,(#174703,#174704,#174705,#174706,#174707,#174708,#174709,
#174710,#174711,#174712,#174713,#174714,#174715,#174716,#174717,#174718,
#174719,#174720,#174721),.UNSPECIFIED.,.F.,.F.)
B_SPLINE_CURVE_WITH_KNOTS((4,1,1,1,1,1,1,1,1,1,1,1,1,1,1,1,4),(0.,0.226732296973331,
0.464902013928651,0.70307173088397,0.9298040278573,1.15653632483063,1.39470604178595,
1.63287575874127,1.8596080557146,2.08634035268793,2.32451006964325,2.56267978659857,
2.7894120835719,3.01614438054523,3.25431409750055,3.49248381445586,3.7192161114292),
 .UNSPECIFIED.)
CURVE()
GEOMETRIC_REPRESENTATION_ITEM()
RATIONAL_B_SPLINE_CURVE((1.,1.,1.,1.,1.,1.,1.,1.,1.,1.,1.,1.,1.,1.,1.,1.,
1.,1.,1.))
REPRESENTATION_ITEM('')
) ;
#30=(
BOUNDED_CURVE()
B_SPLINE_CURVE(3,(#193341,#193342,#193343,#193344,#193345,#193346,#193347,
#193348,#193349,#193350,#193351,#193352,#193353,#193354,#193355,#193356,
#193357,#193358,#193359,#193360,#193361,#193362,#193363,#193364,#193365,
#193366,#193367,#193368,#193369,#193370,#193371,#193372,#193373,#193374,
#193375,#193376,#193377,#193378,#193379,#193380,#193381,#193382,#193383,
#193384,#193385,#193386,#193387,#193388,#193389,#193390,#193391,#193392,
#193393,#193394,#193395,#193396,#193397,#193398,#193399,#193400,#193401,
#193402,#193403,#193404,#193405,#193406,#193407,#193408,#193409,#193410,
#193411,#193412,#193413,#193414,#193415,#193416,#193417,#193418,#193419,
#193420,#193421,#193422,#193423,#193424,#193425,#193426,#193427,#193428,
#193429,#193430,#193431,#193432,#193433,#193434,#193435,#193436,#193437,
#193438,#193439,#193440,#193441,#193442,#193443,#193444,#193445,#193446,
#193447,#193448,#193449,#193450,#193451,#193452,#193453,#193454,#193455,
#193456,#193457,#193458,#193459,#193460,#193461,#193462,#193463,#193464,
#193465,#193466,#193467,#193468,#193469,#193470,#193471,#193472,#193473,
#193474,#193475,#193476,#193477,#193478,#193479,#193480,#193481,#193482,
#193483,#193484,#193485,#193486,#193487,#193488,#193489,#193490,#193491,
#193492,#193493,#193494,#193495,#193496,#193497,#193498,#193499,#193500,
#193501,#193502,#193503,#193504,#193505,#193506,#193507,#193508,#193509,
#193510,#193511,#193512,#193513,#193514,#193515,#193516,#193517,#193518,
#193519,#193520,#193521,#193522,#193523,#193524,#193525,#193526,#193527,
#193528,#193529,#193530,#193531,#193532,#193533,#193534,#193535,#193536,
#193537,#193538,#193539,#193540,#193541,#193542,#193543,#193544,#193545,
#193546,#193547,#193548,#193549,#193550,#193551,#193552,#193553,#193554,
#193555,#193556,#193557,#193558,#193559,#193560,#193561,#193562,#193563,
#193564,#193565,#193566,#193567,#193568,#193569,#193570,#193571,#193572,
#193573,#193574,#193575,#193576,#193577,#193578,#193579,#193580,#193581,
#193582,#193583,#193584,#193585,#193586,#193587,#193588,#193589,#193590,
#193591,#193592,#193593,#193594,#193595,#193596,#193597,#193598,#193599,
#193600,#193601,#193602,#193603,#193604,#193605,#193606,#193607,#193608,
#193609,#193610,#193611,#193612,#193613,#193614,#193615,#193616,#193617,
#193618,#193619,#193620,#193621,#193622,#193623,#193624,#193625,#193626,
#193627,#193628,#193629,#193630,#193631,#193632,#193633,#193634,#193635,
#193636,#193637,#193638,#193639,#193640,#193641,#193642,#193643,#193644,
#193645,#193646,#193647,#193648,#193649,#193650,#193651,#193652,#193653,
#193654,#193655,#193656,#193657,#193658,#193659,#193660,#193661,#193662,
#193663,#193664,#193665,#193666,#193667,#193668,#193669,#193670,#193671,
#193672,#193673,#193674,#193675,#193676,#193677,#193678,#193679,#193680,
#193681,#193682,#193683,#193684,#193685,#193686,#193687,#193688,#193689,
#193690,#193691,#193692,#193693,#193694,#193695,#193696,#193697,#193698,
#193699,#193700,#193701,#193702,#193703,#193704,#193705,#193706,#193707,
#193708,#193709,#193710,#193711,#193712,#193713,#193714,#193715,#193716,
#193717,#193718,#193719,#193720,#193721,#193722,#193723,#193724,#193725,
#193726,#193727,#193728,#193729,#193730,#193731,#193732,#193733,#193734,
#193735,#193736,#193737,#193738,#193739,#193740,#193741,#193742,#193743,
#193744,#193745,#193746,#193747,#193748,#193749,#193750,#193751,#193752,
#193753,#193754,#193755,#193756,#193757,#193758,#193759,#193760,#193761,
#193762,#193763,#193764,#193765,#193766,#193767,#193768,#193769,#193770,
#193771,#193772,#193773,#193774,#193775,#193776,#193777,#193778,#193779,
#193780,#193781,#193782,#193783,#193784,#193785,#193786,#193787,#193788,
#193789,#193790,#193791,#193792,#193793,#193794,#193795,#193796,#193797,
#193798,#193799,#193800,#193801,#193802,#193803,#193804,#193805,#193806,
#193807,#193808,#193809,#193810,#193811,#193812,#193813,#193814,#193815,
#193816,#193817,#193818,#193819,#193820,#193821,#193822,#193823,#193824,
#193825,#193826,#193827,#193828,#193829,#193830,#193831,#193832,#193833,
#193834,#193835,#193836,#193837,#193838,#193839,#193840,#193841,#193842,
#193843,#193844,#193845,#193846,#193847,#193848,#193849,#193850,#193851,
#193852,#193853,#193854,#193855,#193856,#193857,#193858,#193859,#193860,
#193861,#193862,#193863,#193864,#193865,#193866,#193867,#193868,#193869,
#193870,#193871,#193872,#193873,#193874,#193875,#193876,#193877,#193878,
#193879,#193880,#193881,#193882,#193883,#193884,#193885,#193886,#193887,
#193888,#193889,#193890,#193891,#193892,#193893,#193894,#193895,#193896,
#193897,#193898,#193899,#193900,#193901,#193902,#193903,#193904,#193905,
#193906,#193907,#193908,#193909,#193910,#193911,#193912,#193913,#193914,
#193915,#193916,#193917,#193918,#193919,#193920,#193921,#193922,#193923,
#193924,#193925,#193926,#193927,#193928,#193929,#193930,#193931,#193932,
#193933,#193934,#193935,#193936,#193937,#193938,#193939,#193940,#193941,
#193942,#193943,#193944,#193945,#193946,#193947,#193948,#193949,#193950,
#193951,#193952,#193953,#193954,#193955,#193956,#193957,#193958,#193959,
#193960,#193961,#193962,#193963,#193964,#193965,#193966,#193967,#193968,
#193969,#193970,#193971,#193972,#193973,#193974,#193975,#193976,#193977,
#193978,#193979,#193980,#193981,#193982,#193983,#193984,#193985,#193986,
#193987,#193988,#193989,#193990,#193991,#193992,#193993,#193994,#193995,
#193996,#193997,#193998,#193999,#194000,#194001,#194002,#194003,#194004,
#194005,#194006,#194007,#194008,#194009,#194010,#194011,#194012,#194013,
#194014,#194015,#194016,#194017,#194018,#194019,#194020,#194021,#194022,
#194023,#194024,#194025,#194026,#194027,#194028,#194029,#194030,#194031,
#194032,#194033,#194034,#194035,#194036,#194037,#194038,#194039,#194040,
#194041,#194042,#194043,#194044,#194045,#194046,#194047,#194048,#194049,
#194050,#194051,#194052,#194053,#194054,#194055,#194056,#194057,#194058,
#194059,#194060,#194061,#194062,#194063,#194064,#194065,#194066,#194067,
#194068,#194069,#194070,#194071,#194072,#194073,#194074,#194075,#194076,
#194077,#194078,#194079,#194080,#194081,#194082,#194083,#194084,#194085,
#194086,#194087,#194088,#194089,#194090,#194091,#194092,#194093,#194094,
#194095,#194096,#194097,#194098,#194099,#194100,#194101,#194102,#194103,
#194104,#194105,#194106,#194107,#194108,#194109,#194110,#194111,#194112,
#194113,#194114,#194115,#194116,#194117,#194118,#194119,#194120,#194121,
#194122,#194123,#194124,#194125,#194126,#194127,#194128,#194129,#194130,
#194131,#194132,#194133,#194134,#194135,#194136,#194137,#194138,#194139,
#194140,#194141,#194142,#194143,#194144,#194145,#194146,#194147,#194148,
#194149,#194150,#194151,#194152,#194153,#194154,#194155,#194156,#194157,
#194158,#194159,#194160,#194161,#194162,#194163,#194164,#194165,#194166,
#194167,#194168,#194169,#194170,#194171,#194172,#194173,#194174,#194175,
#194176,#194177,#194178,#194179,#194180,#194181,#194182,#194183,#194184,
#194185,#194186,#194187,#194188,#194189,#194190,#194191,#194192,#194193,
#194194,#194195,#194196,#194197,#194198,#194199,#194200,#194201,#194202,
#194203,#194204,#194205,#194206,#194207,#194208,#194209,#194210,#194211,
#194212,#194213,#194214,#194215,#194216,#194217,#194218,#194219,#194220,
#194221,#194222,#194223,#194224,#194225,#194226,#194227,#194228,#194229,
#194230,#194231,#194232,#194233,#194234,#194235,#194236,#194237,#194238,
#194239,#194240,#194241,#194242,#194243,#194244,#194245,#194246,#194247,
#194248,#194249,#194250,#194251,#194252,#194253,#194254,#194255,#194256,
#194257,#194258,#194259,#194260,#194261,#194262,#194263,#194264,#194265,
#194266,#194267,#194268,#194269,#194270,#194271,#194272,#194273,#194274,
#194275,#194276,#194277,#194278,#194279,#194280,#194281,#194282,#194283,
#194284,#194285,#194286,#194287,#194288,#194289,#194290,#194291,#194292,
#194293,#194294,#194295,#194296,#194297,#194298,#194299,#194300,#194301,
#194302,#194303,#194304,#194305,#194306,#194307,#194308,#194309,#194310,
#194311,#194312,#194313,#194314,#194315,#194316,#194317,#194318,#194319,
#194320,#194321,#194322,#194323,#194324,#194325,#194326,#194327,#194328,
#194329,#194330,#194331,#194332,#194333,#194334,#194335,#194336,#194337,
#194338,#194339,#194340,#194341,#194342,#194343,#194344,#194345,#194346,
#194347,#194348,#194349,#194350,#194351,#194352,#194353,#194354,#194355,
#194356,#194357,#194358,#194359,#194360,#194361,#194362,#194363,#194364,
#194365,#194366,#194367,#194368,#194369,#194370,#194371,#194372,#194373,
#194374,#194375,#194376,#194377,#194378,#194379,#194380,#194381,#194382,
#194383,#194384,#194385,#194386,#194387,#194388,#194389,#194390,#194391,
#194392,#194393,#194394,#194395,#194396,#194397,#194398),.UNSPECIFIED.,
 .F.,.F.)
B_SPLINE_CURVE_WITH_KNOTS((4,1,1,1,1,1,1,1,1,1,1,1,1,1,1,1,1,1,1,1,1,1,
1,1,1,1,1,1,1,1,1,1,1,1,1,1,1,1,1,1,1,1,1,1,1,1,1,1,1,1,1,1,1,1,1,1,1,1,
1,1,1,1,1,1,1,1,1,1,1,1,1,1,1,1,1,1,1,1,1,1,1,1,1,1,1,1,1,1,1,1,1,1,1,1,
1,1,1,1,1,1,1,1,1,1,1,1,1,1,1,1,1,1,1,1,1,1,1,1,1,1,1,1,1,1,1,1,1,1,1,1,
1,1,1,1,1,1,1,1,1,1,1,1,1,1,1,1,1,1,1,1,1,1,1,1,1,1,1,1,1,1,1,1,1,1,1,1,
1,1,1,1,1,1,1,1,1,1,1,1,1,1,1,1,1,1,1,1,1,1,1,1,1,1,1,1,1,1,1,1,1,1,1,1,
1,1,1,1,1,1,1,1,1,1,1,1,1,1,1,1,1,1,1,1,1,1,1,1,1,1,1,1,1,1,1,1,1,1,1,1,
1,1,1,1,1,1,1,1,1,1,1,1,1,1,1,1,1,1,1,1,1,1,1,1,1,1,1,1,1,1,1,1,1,1,1,1,
1,1,1,1,1,1,1,1,1,1,1,1,1,1,1,1,1,1,1,1,1,1,1,1,1,1,1,1,1,1,1,1,1,1,1,1,
1,1,1,1,1,1,1,1,1,1,1,1,1,1,1,1,1,1,1,1,1,1,1,1,1,1,1,1,1,1,1,1,1,1,1,1,
1,1,1,1,1,1,1,1,1,1,1,1,1,1,1,1,1,1,1,1,1,1,1,1,1,1,1,1,1,1,1,1,1,1,1,1,
1,1,1,1,1,1,1,1,1,1,1,1,1,1,1,1,1,1,1,1,1,1,1,1,1,1,1,1,1,1,1,1,1,1,1,1,
1,1,1,1,1,1,1,1,1,1,1,1,1,1,1,1,1,1,1,1,1,1,1,1,1,1,1,1,1,1,1,1,1,1,1,1,
1,1,1,1,1,1,1,1,1,1,1,1,1,1,1,1,1,1,1,1,1,1,1,1,1,1,1,1,1,1,1,1,1,1,1,1,
1,1,1,1,1,1,1,1,1,1,1,1,1,1,1,1,1,1,1,1,1,1,1,1,1,1,1,1,1,1,1,1,1,1,1,1,
1,1,1,1,1,1,1,1,1,1,1,1,1,1,1,1,1,1,1,1,1,1,1,1,1,1,1,1,1,1,1,1,1,1,1,1,
1,1,1,1,1,1,1,1,1,1,1,1,1,1,1,1,1,1,1,1,1,1,1,1,1,1,1,1,1,1,1,1,1,1,1,1,
1,1,1,1,1,1,1,1,1,1,1,1,1,1,1,1,1,1,1,1,1,1,1,1,1,1,1,1,1,1,1,1,1,1,1,1,
1,1,1,1,1,1,1,1,1,1,1,1,1,1,1,1,1,1,1,1,1,1,1,1,1,1,1,1,1,1,1,1,1,1,1,1,
1,1,1,1,1,1,1,1,1,1,1,1,1,1,1,1,1,1,1,1,1,1,1,1,1,1,1,1,1,1,1,1,1,1,1,1,
1,1,1,1,1,1,1,1,1,1,1,1,1,1,1,1,1,1,1,1,1,1,1,1,1,1,1,1,1,1,1,1,1,1,1,1,
1,1,1,1,1,1,1,1,1,1,1,1,1,1,1,1,1,1,1,1,1,1,1,1,1,1,1,1,1,1,1,1,1,1,1,1,
1,1,1,1,1,1,1,1,1,1,1,1,1,1,1,1,1,1,1,1,1,1,1,1,1,1,1,1,1,1,1,1,1,1,1,1,
1,1,1,1,1,1,1,1,1,1,1,1,1,1,1,1,1,1,1,1,1,1,1,1,1,1,1,1,1,1,1,1,1,1,1,1,
1,1,1,1,1,1,1,1,1,1,1,1,1,1,1,1,1,1,1,1,1,1,1,1,1,1,1,1,1,1,1,1,1,1,1,1,
1,1,1,1,1,1,1,1,1,1,1,1,1,1,1,1,1,1,1,1,1,1,1,1,1,1,1,1,1,1,1,1,1,1,1,1,
1,1,1,1,1,1,1,1,1,1,1,1,1,1,1,1,1,1,1,1,1,1,1,1,1,1,1,1,1,1,1,1,1,1,1,1,
1,1,1,1,1,1,1,1,1,1,1,1,1,1,1,1,1,1,1,1,1,1,1,1,1,1,1,1,1,1,1,1,1,1,1,1,
1,1,1,1,1,1,1,1,1,1,1,1,1,1,1,1,1,1,1,1,1,1,1,1,1,1,1,1,1,1,1,1,1,1,1,1,
1,1,1,1,1,1,1,1,1,1,1,1,1,1,1,1,1,1,1,1,1,1,1,1,1,4),(0.,0.01797683372391,
0.286633051710584,0.555289278308216,0.823945516665782,1.09260176953922,
1.36125803873948,1.62991432588463,1.89857063164012,2.16722695661301,2.43588330050525,
2.70453966304674,2.9731960431531,3.24185243981471,3.51050885133453,3.77916527610465,
4.04782171198515,4.31647815691489,4.58513460847725,4.85379106430677,5.12244752187208,
5.39110397865606,5.65976043217153,5.92841687990537,6.19707331956994,6.46572974881596,
6.73438616570634,7.00304256821933,7.2716989549161,7.5403553242696,7.809011675483,
8.07766800769526,8.34632432089157,8.61498061505147,8.8836368910788,9.15229314997201,
9.4209493936865,9.68960562442157,9.95826184531348,10.226918059948,10.4955742727586,
10.7642304884925,11.0328867113173,11.3015429448574,11.5701991918227,11.8388554546081,
12.1075117346518,12.3761680332469,12.6448243507434,12.9134806874637,13.1821370428496,
13.450793416388,13.7194498067883,13.9881062128412,14.2567626326955,14.5254190645885,
14.7940755062772,15.0627319555912,15.3313884100611,15.6000448672586,15.8687013246492,
16.1373577797,16.4060142299691,16.6746706729765,16.9433271065265,17.2119835283531,
17.4806399366567,17.7492963295502,18.0179527057767,18.286609063996,18.555265403637,
18.8239217240786,19.0925780255742,19.3612343083975,19.6298905737625,19.898546823017,
20.1672030584666,20.4358592827168,20.7045154992928,20.973171712245,21.2418279262962,
21.5104841459723,21.7791403749736,22.0477966165324,22.316452872948,22.585109146262,
22.8537654375589,23.1224217478187,23.3910780770929,23.6597344254327,23.9283907920352,
24.197047176159,24.4657035763222,24.7343599911301,25.0030164185931,25.2716728568073,
25.5403293034427,25.8089857562333,26.0776422126729,26.3462986702843,26.6149551265448,
26.8836115789212,27.1522680250308,27.4209244624423,27.6895808890659,27.9582373027346,
28.2268937018004,28.4955500845261,28.7642064498512,29.0328627966379,29.3015191245544,
29.5701754332357,29.838831723217,30.1074879950829,30.3761442503694,30.6448004907916,
30.9134567190168,31.1821129380756,31.450769151893,31.7194253649682,31.9880815819663,
32.2567378070174,32.5253940433706,32.7940502938785,33.0627065604467,33.3313628447765,
33.6000191476151,33.8686754696427,34.1373318106287,34.405988170366,34.6746445478242,
34.9433009420458,35.2119573513747,35.480613774244,35.7492702085419,36.0179266522368,
36.2865831029275,36.5552395582669,36.8238960157264,37.0925524727952,37.3612089269773,
37.6298653757534,37.8985218168153,38.1671782477952,38.4358346667239,38.7044910715485,
38.9731474607866,39.2418038328672,39.5104601869391,39.7791165220837,40.0477728382212,
40.3164291352602,40.5850854140292,40.8537416754418,41.1223979213679,41.3910541539077,
41.6597103761025,41.9283665914244,42.1970228042084,42.4656790192,42.7343352406829,
43.0029914723808,43.2716477171096,43.540303977354,43.8089602546436,44.0776165503516,
44.3462728649052,44.614929198697,44.883585551232,45.1522419220568,45.4208983099307,
45.6895547136931,45.9582111315299,46.2268675617156,46.4955240020317,46.7641804503338,
47.0328369041642,47.3014933611089,47.5701498186329,47.8388062742058,48.107462725373,
48.3761191696448,48.6447756048012,48.9134320285537,49.1820884390673,49.4507448344197,
49.7194012133072,49.9880575743413,50.2567139168934,50.5253702402807,50.7940265446884,
51.0626828303152,51.3313390982961,51.5999953498901,51.8686515873141,52.1373078130706,
52.4059640305862,52.6746202437936,52.9432764573682,53.211932675918,53.480588903259,
53.7492451427202,54.0179013967021,54.2865576673334,54.5552139557853,54.823870263115,
55.0925265894471,55.3611829348992,55.6298392987282,55.8984956802486,56.1671520780245,
56.4358084907065,56.7044649163381,56.9731213530494,57.2417777985307,57.5104342505384,
57.7790907065743,58.0477471641719,58.3164036208043,58.5850600739368,58.8537165211707,
59.1223729600609,59.39102938849,59.6596858042645,59.9283422056975,60.1969985910129,
60.4656549590995,60.7343113087676,61.0029676396243,61.2716239512389,61.540280244075,
61.808936518638,62.0775927763821,62.3462490189291,62.6149052488546,62.8835614690812,
63.1522176834332,63.4208738963055,63.6895301124163,63.9581863359981,64.2268425704115,
64.4954988186027,64.7641550825741,65.0328113641112,65.3014676640435,65.5701239831253,
65.8387803211949,66.1074366781083,66.3760930528907,66.6447494446373,66.9134058517341,
67.1820622726558,67.4507187053199,67.7193751477252,67.988031597487,68.256688052277,
68.5253445095709,68.7940009668648,69.0626574216546,69.3313138714164,69.5999703138218,
69.8686267464858,70.1372831674076,70.4059395745042,70.6745959662509,70.9432523410334,
71.2119086979469,71.4805650360164,71.7492213550982,72.0178776550306,72.2865339365675,
72.5551902005389,72.8238464487301,73.0925026831433,73.3611589067251,73.6298151228357,
73.8984713357081,74.1671275500599,74.4357837702864,74.7044400002118,74.9730962427587,
75.2417525005027,75.5104087750655,75.7790650679015,76.047721379516,76.3163777103726,
76.5850340600405,76.853690428127,77.1223468134422,77.391003214875,77.6596596306495,
77.9283160590784,78.1969724979684,78.4656289452021,78.7342853983344,79.0029418549666,
79.2715983125641,79.5402547685998,79.8089112206075,80.0775676660886,80.3462241027997,
80.6148805284312,80.8835369411131,81.1521933388889,81.4208497204091,81.689506084238,
81.9581624296899,82.2268187560219,82.4954750633515,82.7641313518033,83.0327876224345,
83.3014438764161,83.5701001158772,83.838756343218,84.1074125617677,84.3760687753422,
84.6447249885494,84.913381206065,85.1820374318212,85.4506936692451,85.719349920839,
85.9880061888197,86.2566624744465,86.5253187788541,86.7939751022413,87.0626314447932,
87.3312878058273,87.5999441847146,87.8686005800667,88.1372569905802,88.4059134143327,
88.6745698494889,88.9432262937606,89.2118827449277,89.4805392005005,89.7491956580243,
90.0178521149689,90.2865085687992,90.5551650171012,90.8238214574172,91.0924778876028,
91.3611343054394,91.6297907092016,91.8984470970753,92.1671034679,92.4357598204347,
92.7044161542264,92.9730724687798,93.2417287644878,93.5103850417773,93.7790413020216,
94.0476975467502,94.3163537784479,94.5850099999307,94.8536662149221,95.1223224277061,
95.390978643028,95.6596348652226,95.9282910977624,96.1969473436883,96.4656036051009,
96.7342598838697,97.0029161809086,97.2715724970461,97.5402288321905,97.8088851862623,
98.0775415583427,98.3461979475807,98.6148543524051,98.8835107713336,99.1521672023136,
99.4208236433754,99.6894800921513,99.9581365463333,100.226793003402,100.495449460861,
100.7641059162,101.032762366891,101.301418810586,101.570075244884,101.838731667753,
102.107388077082,102.376044471303,102.644700848761,102.913357208498,103.182013549484,
103.450669871511,103.71932617435,103.98798245868,104.256638725248,104.525294975755,
104.793951212108,105.062607437159,105.331263654157,105.599919867233,105.86857608105,
106.137232300108,106.405888528334,106.674544768756,106.943201024042,107.211857295908,
107.480513585889,107.74916989457,108.017826222487,108.286482569273,108.555138934598,
108.823795317324,109.09245171639,109.361108130058,109.629764556682,109.898420994093,
110.167077440202,110.435733892579,110.704390348839,110.97304680645,111.24170326289,
111.51035971568,111.779016162316,112.04767260053,112.316329027993,112.5849854428,
112.853641842963,113.122298227087,113.39095459369,113.659610942029,113.928267271303,
114.196923581563,114.46557987286,114.734236146174,115.002892402589,115.271548644148,
115.540204873149,115.808861092825,116.077517306876,116.346173519828,116.614829736404,
116.883485960654,117.152142196103,117.420798445358,117.689454710722,117.958110993546,
118.226767295041,118.495423615483,118.764079955123,119.032736313343,119.301392689569,
119.570049082462,119.838705490766,120.107361912592,120.376018346142,120.644674789149,
120.913331239418,121.181987694469,121.45064415186,121.719300609057,121.987957063527,
122.256613512841,122.525269954529,122.793926386422,123.062582806276,123.331239212329,
123.599895602729,123.868551976268,124.137208331653,124.405864668374,124.67452098587,
124.943177284465,125.211833564508,125.480489827294,125.749146074259,126.017802307799,
126.286458530624,126.555114746357,126.823770959168,127.092427173802,127.361083394694,
127.629739625429,127.898395869143,128.167052128037,128.435708404064,128.704364698224,
128.97302101142,129.241677343633,129.510333694846,129.7789900642,130.047646450897,
130.31630285341,130.5849592703,130.853615699547,131.122272139211,131.390928586945,
131.659585040461,131.928241497245,132.19689795481,132.46555441064,132.734210862202,
133.002867307132,133.271523743013,133.540180167783,133.808836579303,134.077492975965,
134.346149356071,134.614805718613,134.883462062505,135.152118387478,135.420774693234,
135.689430980379,135.958087249579,136.226743502453,136.49539974081,136.76405596741,
137.032712185392,137.301368398783,137.570024612174,137.838680830155,138.107337056755,
138.375993295112,138.644649547986,138.913305817186,139.181962104332,139.450618410087,
139.71927473506,139.987931078952,140.256587441494,140.525243821601,140.793900218262,
141.062556629782,141.331213054552,141.599869490433,141.868525935363,142.137182386925,
142.405838842755,142.67449530032,142.943151757104,143.21180821062,143.480464658354,
143.749121098019,144.017777527265,144.286433944155,144.555090346668,144.823746733365,
145.092403102719,145.361059453932,145.629715786145,145.898372099341,146.167028393501,
146.435684669529,146.704340928422,146.972997172137,147.241653402872,147.510309623764,
147.778965838398,148.047622051209,148.316278266943,148.584934489768,148.853590723308,
149.122246970274,149.390903233059,149.659559513103,149.928215811698,150.196872129195,
150.465528465915,150.734184821301,151.00284119484,151.27149758524,151.540153991293,
151.808810411148,152.077466843041,152.34612328473,152.614779734044,152.883436188514,
153.152092645711,153.420749103102,153.689405558153,153.958062008422,154.22671845143,
154.49537488498,154.764031306806,155.03268771511,155.301344108004,155.57000048423,
155.838656842449,156.107313182091,156.375969502532,156.644625804028,156.913282086851,
157.181938352216,157.450594601471,157.719250836921,157.987907061171,158.256563277747,
158.525219490699,158.793875704751,159.062531924427,159.331188153428,159.599844394987,
159.868500651403,160.137156924717,160.405813216014,160.674469526274,160.943125855548,
161.211782203888,161.480438570491,161.749094954615,162.017751354778,162.286407769586,
162.555064197049,162.823720635263,163.092377081899,163.361033534689,163.629689991129,
163.898346448741,164.167002905001,164.435659357378,164.704315803488,164.972972240899,
165.241628667523,165.510285081192,165.778941480257,166.047597862983,166.316254228308,
166.584910575095,166.853566903012,167.122223211693,167.390879501675,167.659535773541,
167.928192028827,168.19684826925,168.465504497475,168.734160716534,169.002816930351,
169.271473143427,169.540129360425,169.808785585476,170.077441821829,170.346098072337,
170.614754338905,170.883410623235,171.152066926074,171.420723248102,171.689379589088,
171.958035948825,172.226692326284,172.495348720505,172.764005129834,173.032661552704,
173.301317987002,173.569974430697,173.838630881388,174.107287336727,174.375943794187,
174.644600251255,174.913256705437,175.181913154214,175.450569595276,175.719226026256,
175.987882445184,176.256538850009,176.525195239247,176.793851611328,177.0625079654,
177.331164300545,177.599820616682,177.868476913721,178.137133192491,178.405789453903,
178.674445699829,178.943101932369,179.211758154564,179.480414369886,179.74907058267,
180.017726797662,180.286383019145,180.555039250843,180.823695495572,181.092351755816,
181.361008033106,181.629664328814,181.898320643368,182.16697697716,182.435633329695,
182.70428970052,182.972946088394,183.241602492156,183.510258909993,183.778915340179,
184.047571780495,184.316228228797,184.584884682628,184.853541139572,185.122197597096,
185.39085405267,185.659510503837,185.928166948109,186.196823383265,186.465479807018,
186.734136217531,187.002792612884,187.271448991771,187.540105352806,187.808761695358,
188.077418018745,188.346074323153,188.61473060878,188.883386876761,189.152043128355,
189.420699365779,189.689355591536,189.958011809051,190.226668022259,190.495324235834,
190.763980454383,191.032636681725,191.301292921186,191.569949175168,191.838605445799,
192.107261734251,192.375918041581,192.644574367913,192.913230713365,193.181887077194,
193.450543458715,193.719199856491,193.987856269173,194.256512694805,194.525169131516,
194.793825576997,195.062482029005,195.331138485041,195.599794942639,195.868451399271,
196.137107852404,196.405764299638,196.674420738528,196.943077166957,197.211733582732,
197.480389984165,197.749046369481,198.017702737567,198.286359087236,198.555015418092,
198.823671729707,199.092328022543,199.360984297106,199.62964055485,199.898296797397,
200.166953027323,200.43560924755,200.704265461902,200.972921674774,201.241577890885,
201.510234114467,201.77889034888,202.047546597072,202.316202861043,202.584859142581,
202.853515442513,203.122171761595,203.390828099665,203.659484456579,203.928140831361,
204.196797223108,204.465453630205,204.734110051127,205.002766483791,205.271422926197,
205.540079375959,205.808735830749,206.077392288043,206.346048745337,206.614705200127,
206.883361649889,207.152018092295,207.420674524959,207.689330945881,207.957987352978,
208.226643744725,208.495300119508,208.763956476421,209.032612814491,209.301269133573,
209.569925433505,209.838581715043,210.107237979014,210.375894227206,210.644550461619,
210.913206685201,211.181862901312,211.450519114184,211.719175328536,211.987831548763,
212.256487778689,212.525144021236,212.79380027898,213.062456553543,213.331112846379,
213.599769157994,213.868425488851,214.137081838519,214.405738206606,214.674394591921,
214.943050993354,215.211707409129,215.480363837558,215.749020276448,216.017676723682,
216.286333176815,216.554989633447,216.823646091045,217.092302547081,217.360958999089,
217.62961544457,217.898271881281,218.166928306913,218.435584719595,218.704241117371,
218.972897498892,219.241553862721,219.510210208173,219.778866534505,220.047522841835,
220.316179130287,220.584835400918,220.8534916549,221.122147894361,221.390804121702,
221.659460340252,221.928116553827,222.196772767034,222.46542898455,222.734085210306,
223.00274144773,223.271397699324,223.540053967305,223.808710252932,224.07736655734,
224.346022880728,224.61467922328,224.883335584314,225.151991963201,225.420648358554,
225.689304769068,225.95796119282,226.226617627977,226.495274072249,226.763930523416,
227.032586978989,227.301243436513,227.569899893458,227.838556347288,228.10721279559,
228.375869235907,228.644525666093,228.913182083929,229.181838487692,229.450494875566,
229.719151246391,229.987807598926,230.256463932718,230.525120247271,230.79377654298,
231.062432820269,231.331089080514,231.599745325243,231.868401556941,232.137057778424,
232.405713993415,232.674370206199,232.943026421521,233.211682643716,233.480338876256,
233.748995122182,234.017651383595,234.286307662364,234.554963959403,234.823620275541,
235.092276610685,235.360932964757,235.629589336838,235.898245726076,236.166902130901,
236.43555854983,236.70421498081,236.972871421872,237.241527870648,237.51018432483,
237.778840781899,238.047497239359,238.316153694698,238.584810145389,238.853466589084,
239.122123023382,239.390779446251,239.65943585558,239.928092249802,240.19674862726,
240.465404986998,240.734061327984,241.002717650011,241.27137395285,241.54003023718,
241.808686503748,242.077342754256,242.345998990609,242.614655215661,242.883311432659,
243.151967645734,243.420623859552,243.68928007861,243.957936306836,244.226592547258,
244.495248802545,244.763905074411,245.032561364392,245.301217673074,245.56987400099,
245.838530347777,246.107186713102,246.375843095828,246.644499494894,246.913155908563,
247.181812335186,247.450468772598,247.719125218708,247.987781671084,248.256438127345,
248.525094584956,248.793751041396,249.062407494187,249.331063940822,249.599720379036,
249.8683768065,250.137033221308,250.405689621471,250.674346005595,250.943002372197,
251.211658720537,251.480315049812,251.748971360071,252.017627651368,252.286283924683,
252.554940181098,252.823596422657,253.092252651658,253.360908871335,253.629565085386,
253.898221298338,254.166877514914,254.435533739165,254.704189974614,254.972846223869,
255.241502489234,255.510158772057,255.778815073553,256.047471393995,256.316127733635,
256.584784091854,256.85344046808,257.122096860973,257.390753269276,257.659409691102,
257.928066124652,258.196722567659,258.465379017928,258.734035472978,259.002691930368,
259.271348387566,259.540004842035,259.808661291349,260.077317733037,260.345974164929,
260.614630584783,260.883286990836,261.151943381235,261.420599754774,261.689256110159,
261.957912446879,262.226568764375,262.49522506297,262.763881343014,263.032537605798,
263.301193852763,263.569850086303,263.838506309127,264.107162524861,264.375818737671,
264.644474952305,264.913131173196,265.181787403931,265.450443647645,265.719099906538,
265.987756182565,266.256412476724,266.52506878992,266.793725122132,267.062381473345,
267.331037842698,267.599694229394,267.868350631907,268.137007048797,268.405663478042,
268.674319917706,268.94297636544,269.211632818955,269.480289275739,269.748945733304,
270.017602189133,270.286258640695,270.554915085624,270.823571521504,271.092227946274,
271.360884357793,271.629540754454,271.89819713456,272.166853497101,272.435509840993,
272.704166165965,272.97282247172,273.241478758865,273.510135028065,273.778791280938,
274.047447519295,274.316103745894,274.584759963875,274.853416177266,275.122072390656,
275.390728608637,275.659384835237,275.928041073593,276.196697326466,276.465353595666,
276.734009882811,277.002666188566,277.271322513539,277.53997885743,277.808635219972,
278.077291600077,278.345947996739,278.614604408258,278.883260833028,279.151917268908,
279.420573713837,279.689230165399,279.957886621228,280.226543078793,280.495199535576,
280.763855989092,281.032512436825,281.301168876489,281.569825305735,281.838481722625,
282.107138125138,282.375794511834,282.644450881187,282.9131072324,283.140531716307),
 .UNSPECIFIED.)
CURVE()
GEOMETRIC_REPRESENTATION_ITEM()
RATIONAL_B_SPLINE_CURVE((1.,1.,1.,1.,1.,1.,1.,1.,1.,1.,1.,1.,1.,1.,1.,1.,
1.,1.,1.,1.,1.,1.,1.,1.,1.,1.,1.,1.,1.,1.,1.,1.,1.,1.,1.,1.,1.,1.,1.,1.,
1.,1.,1.,1.,1.,1.,1.,1.,1.,1.,1.,1.,1.,1.,1.,1.,1.,1.,1.,1.,1.,1.,1.,1.,
1.,1.,1.,1.,1.,1.,1.,1.,1.,1.,1.,1.,1.,1.,1.,1.,1.,1.,1.,1.,1.,1.,1.,1.,
1.,1.,1.,1.,1.,1.,1.,1.,1.,1.,1.,1.,1.,1.,1.,1.,1.,1.,1.,1.,1.,1.,1.,1.,
1.,1.,1.,1.,1.,1.,1.,1.,1.,1.,1.,1.,1.,1.,1.,1.,1.,1.,1.,1.,1.,1.,1.,1.,
1.,1.,1.,1.,1.,1.,1.,1.,1.,1.,1.,1.,1.,1.,1.,1.,1.,1.,1.,1.,1.,1.,1.,1.,
1.,1.,1.,1.,1.,1.,1.,1.,1.,1.,1.,1.,1.,1.,1.,1.,1.,1.,1.,1.,1.,1.,1.,1.,
1.,1.,1.,1.,1.,1.,1.,1.,1.,1.,1.,1.,1.,1.,1.,1.,1.,1.,1.,1.,1.,1.,1.,1.,
1.,1.,1.,1.,1.,1.,1.,1.,1.,1.,1.,1.,1.,1.,1.,1.,1.,1.,1.,1.,1.,1.,1.,1.,
1.,1.,1.,1.,1.,1.,1.,1.,1.,1.,1.,1.,1.,1.,1.,1.,1.,1.,1.,1.,1.,1.,1.,1.,
1.,1.,1.,1.,1.,1.,1.,1.,1.,1.,1.,1.,1.,1.,1.,1.,1.,1.,1.,1.,1.,1.,1.,1.,
1.,1.,1.,1.,1.,1.,1.,1.,1.,1.,1.,1.,1.,1.,1.,1.,1.,1.,1.,1.,1.,1.,1.,1.,
1.,1.,1.,1.,1.,1.,1.,1.,1.,1.,1.,1.,1.,1.,1.,1.,1.,1.,1.,1.,1.,1.,1.,1.,
1.,1.,1.,1.,1.,1.,1.,1.,1.,1.,1.,1.,1.,1.,1.,1.,1.,1.,1.,1.,1.,1.,1.,1.,
1.,1.,1.,1.,1.,1.,1.,1.,1.,1.,1.,1.,1.,1.,1.,1.,1.,1.,1.,1.,1.,1.,1.,1.,
1.,1.,1.,1.,1.,1.,1.,1.,1.,1.,1.,1.,1.,1.,1.,1.,1.,1.,1.,1.,1.,1.,1.,1.,
1.,1.,1.,1.,1.,1.,1.,1.,1.,1.,1.,1.,1.,1.,1.,1.,1.,1.,1.,1.,1.,1.,1.,1.,
1.,1.,1.,1.,1.,1.,1.,1.,1.,1.,1.,1.,1.,1.,1.,1.,1.,1.,1.,1.,1.,1.,1.,1.,
1.,1.,1.,1.,1.,1.,1.,1.,1.,1.,1.,1.,1.,1.,1.,1.,1.,1.,1.,1.,1.,1.,1.,1.,
1.,1.,1.,1.,1.,1.,1.,1.,1.,1.,1.,1.,1.,1.,1.,1.,1.,1.,1.,1.,1.,1.,1.,1.,
1.,1.,1.,1.,1.,1.,1.,1.,1.,1.,1.,1.,1.,1.,1.,1.,1.,1.,1.,1.,1.,1.,1.,1.,
1.,1.,1.,1.,1.,1.,1.,1.,1.,1.,1.,1.,1.,1.,1.,1.,1.,1.,1.,1.,1.,1.,1.,1.,
1.,1.,1.,1.,1.,1.,1.,1.,1.,1.,1.,1.,1.,1.,1.,1.,1.,1.,1.,1.,1.,1.,1.,1.,
1.,1.,1.,1.,1.,1.,1.,1.,1.,1.,1.,1.,1.,1.,1.,1.,1.,1.,1.,1.,1.,1.,1.,1.,
1.,1.,1.,1.,1.,1.,1.,1.,1.,1.,1.,1.,1.,1.,1.,1.,1.,1.,1.,1.,1.,1.,1.,1.,
1.,1.,1.,1.,1.,1.,1.,1.,1.,1.,1.,1.,1.,1.,1.,1.,1.,1.,1.,1.,1.,1.,1.,1.,
1.,1.,1.,1.,1.,1.,1.,1.,1.,1.,1.,1.,1.,1.,1.,1.,1.,1.,1.,1.,1.,1.,1.,1.,
1.,1.,1.,1.,1.,1.,1.,1.,1.,1.,1.,1.,1.,1.,1.,1.,1.,1.,1.,1.,1.,1.,1.,1.,
1.,1.,1.,1.,1.,1.,1.,1.,1.,1.,1.,1.,1.,1.,1.,1.,1.,1.,1.,1.,1.,1.,1.,1.,
1.,1.,1.,1.,1.,1.,1.,1.,1.,1.,1.,1.,1.,1.,1.,1.,1.,1.,1.,1.,1.,1.,1.,1.,
1.,1.,1.,1.,1.,1.,1.,1.,1.,1.,1.,1.,1.,1.,1.,1.,1.,1.,1.,1.,1.,1.,1.,1.,
1.,1.,1.,1.,1.,1.,1.,1.,1.,1.,1.,1.,1.,1.,1.,1.,1.,1.,1.,1.,1.,1.,1.,1.,
1.,1.,1.,1.,1.,1.,1.,1.,1.,1.,1.,1.,1.,1.,1.,1.,1.,1.,1.,1.,1.,1.,1.,1.,
1.,1.,1.,1.,1.,1.,1.,1.,1.,1.,1.,1.,1.,1.,1.,1.,1.,1.,1.,1.,1.,1.,1.,1.,
1.,1.,1.,1.,1.,1.,1.,1.,1.,1.,1.,1.,1.,1.,1.,1.,1.,1.,1.,1.,1.,1.,1.,1.,
1.,1.,1.,1.,1.,1.,1.,1.,1.,1.,1.,1.,1.,1.,1.,1.,1.,1.,1.,1.,1.,1.,1.,1.,
1.,1.,1.,1.,1.,1.,1.,1.,1.,1.,1.,1.,1.,1.,1.,1.,1.,1.,1.,1.,1.,1.,1.,1.,
1.,1.,1.,1.,1.,1.,1.,1.,1.,1.,1.,1.,1.,1.,1.,1.,1.,1.,1.,1.,1.,1.,1.,1.,
1.,1.,1.,1.,1.,1.,1.,1.,1.,1.,1.,1.,1.,1.,1.,1.,1.,1.,1.,1.,1.,1.,1.,1.,
1.,1.,1.,1.,1.,1.,1.,1.,1.,1.,1.,1.,1.,1.,1.,1.,1.,1.,1.,1.,1.,1.,1.,1.,
1.,1.,1.,1.,1.,1.,1.,1.,1.,1.,1.,1.,1.,1.,1.,1.,1.,1.,1.,1.,1.,1.,1.,1.,
1.,1.,1.,1.,1.,1.,1.,1.,1.,1.,1.,1.,1.,1.,1.,1.,1.,1.,1.,1.,1.,1.,1.,1.,
1.,1.,1.,1.,1.,1.,1.,1.,1.,1.,1.,1.,1.,1.,1.,1.,1.,1.,1.,1.,1.,1.,1.,1.,
1.,1.,1.,1.,1.,1.,1.,1.,1.,1.))
REPRESENTATION_ITEM('')
) ;
#31=(
BOUNDED_CURVE()
B_SPLINE_CURVE(3,(#194468,#194469,#194470,#194471,#194472,#194473,#194474),
 .UNSPECIFIED.,.F.,.F.)
B_SPLINE_CURVE_WITH_KNOTS((4,1,1,1,4),(0.,0.0911446219616379,0.182289243923276,
0.273433865884915,0.364578487846551),.UNSPECIFIED.)
CURVE()
GEOMETRIC_REPRESENTATION_ITEM()
RATIONAL_B_SPLINE_CURVE((1.,1.,1.,1.,1.,1.,1.))
REPRESENTATION_ITEM('')
) ;
#32=(
BOUNDED_CURVE()
B_SPLINE_CURVE(3,(#194690,#194691,#194692,#194693,#194694,#194695,#194696,
#194697,#194698,#194699,#194700,#194701,#194702,#194703,#194704,#194705,
#194706,#194707,#194708),.UNSPECIFIED.,.F.,.F.)
B_SPLINE_CURVE_WITH_KNOTS((4,1,1,1,1,1,1,1,1,1,1,1,1,1,1,1,4),(0.,0.226732296973331,
0.464902013928651,0.70307173088397,0.9298040278573,1.15653632483063,1.39470604178595,
1.63287575874127,1.8596080557146,2.08634035268793,2.32451006964325,2.56267978659857,
2.7894120835719,3.01614438054523,3.25431409750055,3.49248381445586,3.7192161114292),
 .UNSPECIFIED.)
CURVE()
GEOMETRIC_REPRESENTATION_ITEM()
RATIONAL_B_SPLINE_CURVE((1.,1.,1.,1.,1.,1.,1.,1.,1.,1.,1.,1.,1.,1.,1.,1.,
1.,1.,1.))
REPRESENTATION_ITEM('')
) ;
#61=(
BOUNDED_SURFACE()
B_SPLINE_SURFACE(3,2,((#154736,#154737,#154738,#154739,#154740,#154741,
#154742,#154743,#154744),(#154745,#154746,#154747,#154748,#154749,#154750,
#154751,#154752,#154753),(#154754,#154755,#154756,#154757,#154758,#154759,
#154760,#154761,#154762),(#154763,#154764,#154765,#154766,#154767,#154768,
#154769,#154770,#154771),(#154772,#154773,#154774,#154775,#154776,#154777,
#154778,#154779,#154780),(#154781,#154782,#154783,#154784,#154785,#154786,
#154787,#154788,#154789),(#154790,#154791,#154792,#154793,#154794,#154795,
#154796,#154797,#154798),(#154799,#154800,#154801,#154802,#154803,#154804,
#154805,#154806,#154807),(#154808,#154809,#154810,#154811,#154812,#154813,
#154814,#154815,#154816),(#154817,#154818,#154819,#154820,#154821,#154822,
#154823,#154824,#154825),(#154826,#154827,#154828,#154829,#154830,#154831,
#154832,#154833,#154834),(#154835,#154836,#154837,#154838,#154839,#154840,
#154841,#154842,#154843),(#154844,#154845,#154846,#154847,#154848,#154849,
#154850,#154851,#154852),(#154853,#154854,#154855,#154856,#154857,#154858,
#154859,#154860,#154861),(#154862,#154863,#154864,#154865,#154866,#154867,
#154868,#154869,#154870),(#154871,#154872,#154873,#154874,#154875,#154876,
#154877,#154878,#154879),(#154880,#154881,#154882,#154883,#154884,#154885,
#154886,#154887,#154888),(#154889,#154890,#154891,#154892,#154893,#154894,
#154895,#154896,#154897),(#154898,#154899,#154900,#154901,#154902,#154903,
#154904,#154905,#154906),(#154907,#154908,#154909,#154910,#154911,#154912,
#154913,#154914,#154915),(#154916,#154917,#154918,#154919,#154920,#154921,
#154922,#154923,#154924),(#154925,#154926,#154927,#154928,#154929,#154930,
#154931,#154932,#154933),(#154934,#154935,#154936,#154937,#154938,#154939,
#154940,#154941,#154942),(#154943,#154944,#154945,#154946,#154947,#154948,
#154949,#154950,#154951),(#154952,#154953,#154954,#154955,#154956,#154957,
#154958,#154959,#154960),(#154961,#154962,#154963,#154964,#154965,#154966,
#154967,#154968,#154969),(#154970,#154971,#154972,#154973,#154974,#154975,
#154976,#154977,#154978),(#154979,#154980,#154981,#154982,#154983,#154984,
#154985,#154986,#154987),(#154988,#154989,#154990,#154991,#154992,#154993,
#154994,#154995,#154996),(#154997,#154998,#154999,#155000,#155001,#155002,
#155003,#155004,#155005),(#155006,#155007,#155008,#155009,#155010,#155011,
#155012,#155013,#155014),(#155015,#155016,#155017,#155018,#155019,#155020,
#155021,#155022,#155023),(#155024,#155025,#155026,#155027,#155028,#155029,
#155030,#155031,#155032),(#155033,#155034,#155035,#155036,#155037,#155038,
#155039,#155040,#155041),(#155042,#155043,#155044,#155045,#155046,#155047,
#155048,#155049,#155050),(#155051,#155052,#155053,#155054,#155055,#155056,
#155057,#155058,#155059),(#155060,#155061,#155062,#155063,#155064,#155065,
#155066,#155067,#155068),(#155069,#155070,#155071,#155072,#155073,#155074,
#155075,#155076,#155077),(#155078,#155079,#155080,#155081,#155082,#155083,
#155084,#155085,#155086),(#155087,#155088,#155089,#155090,#155091,#155092,
#155093,#155094,#155095),(#155096,#155097,#155098,#155099,#155100,#155101,
#155102,#155103,#155104),(#155105,#155106,#155107,#155108,#155109,#155110,
#155111,#155112,#155113),(#155114,#155115,#155116,#155117,#155118,#155119,
#155120,#155121,#155122),(#155123,#155124,#155125,#155126,#155127,#155128,
#155129,#155130,#155131),(#155132,#155133,#155134,#155135,#155136,#155137,
#155138,#155139,#155140),(#155141,#155142,#155143,#155144,#155145,#155146,
#155147,#155148,#155149),(#155150,#155151,#155152,#155153,#155154,#155155,
#155156,#155157,#155158),(#155159,#155160,#155161,#155162,#155163,#155164,
#155165,#155166,#155167),(#155168,#155169,#155170,#155171,#155172,#155173,
#155174,#155175,#155176),(#155177,#155178,#155179,#155180,#155181,#155182,
#155183,#155184,#155185),(#155186,#155187,#155188,#155189,#155190,#155191,
#155192,#155193,#155194),(#155195,#155196,#155197,#155198,#155199,#155200,
#155201,#155202,#155203),(#155204,#155205,#155206,#155207,#155208,#155209,
#155210,#155211,#155212),(#155213,#155214,#155215,#155216,#155217,#155218,
#155219,#155220,#155221),(#155222,#155223,#155224,#155225,#155226,#155227,
#155228,#155229,#155230),(#155231,#155232,#155233,#155234,#155235,#155236,
#155237,#155238,#155239),(#155240,#155241,#155242,#155243,#155244,#155245,
#155246,#155247,#155248),(#155249,#155250,#155251,#155252,#155253,#155254,
#155255,#155256,#155257),(#155258,#155259,#155260,#155261,#155262,#155263,
#155264,#155265,#155266),(#155267,#155268,#155269,#155270,#155271,#155272,
#155273,#155274,#155275),(#155276,#155277,#155278,#155279,#155280,#155281,
#155282,#155283,#155284),(#155285,#155286,#155287,#155288,#155289,#155290,
#155291,#155292,#155293),(#155294,#155295,#155296,#155297,#155298,#155299,
#155300,#155301,#155302),(#155303,#155304,#155305,#155306,#155307,#155308,
#155309,#155310,#155311),(#155312,#155313,#155314,#155315,#155316,#155317,
#155318,#155319,#155320),(#155321,#155322,#155323,#155324,#155325,#155326,
#155327,#155328,#155329),(#155330,#155331,#155332,#155333,#155334,#155335,
#155336,#155337,#155338),(#155339,#155340,#155341,#155342,#155343,#155344,
#155345,#155346,#155347),(#155348,#155349,#155350,#155351,#155352,#155353,
#155354,#155355,#155356),(#155357,#155358,#155359,#155360,#155361,#155362,
#155363,#155364,#155365),(#155366,#155367,#155368,#155369,#155370,#155371,
#155372,#155373,#155374),(#155375,#155376,#155377,#155378,#155379,#155380,
#155381,#155382,#155383),(#155384,#155385,#155386,#155387,#155388,#155389,
#155390,#155391,#155392),(#155393,#155394,#155395,#155396,#155397,#155398,
#155399,#155400,#155401),(#155402,#155403,#155404,#155405,#155406,#155407,
#155408,#155409,#155410),(#155411,#155412,#155413,#155414,#155415,#155416,
#155417,#155418,#155419),(#155420,#155421,#155422,#155423,#155424,#155425,
#155426,#155427,#155428),(#155429,#155430,#155431,#155432,#155433,#155434,
#155435,#155436,#155437),(#155438,#155439,#155440,#155441,#155442,#155443,
#155444,#155445,#155446),(#155447,#155448,#155449,#155450,#155451,#155452,
#155453,#155454,#155455),(#155456,#155457,#155458,#155459,#155460,#155461,
#155462,#155463,#155464),(#155465,#155466,#155467,#155468,#155469,#155470,
#155471,#155472,#155473),(#155474,#155475,#155476,#155477,#155478,#155479,
#155480,#155481,#155482),(#155483,#155484,#155485,#155486,#155487,#155488,
#155489,#155490,#155491),(#155492,#155493,#155494,#155495,#155496,#155497,
#155498,#155499,#155500),(#155501,#155502,#155503,#155504,#155505,#155506,
#155507,#155508,#155509),(#155510,#155511,#155512,#155513,#155514,#155515,
#155516,#155517,#155518),(#155519,#155520,#155521,#155522,#155523,#155524,
#155525,#155526,#155527),(#155528,#155529,#155530,#155531,#155532,#155533,
#155534,#155535,#155536),(#155537,#155538,#155539,#155540,#155541,#155542,
#155543,#155544,#155545),(#155546,#155547,#155548,#155549,#155550,#155551,
#155552,#155553,#155554),(#155555,#155556,#155557,#155558,#155559,#155560,
#155561,#155562,#155563),(#155564,#155565,#155566,#155567,#155568,#155569,
#155570,#155571,#155572),(#155573,#155574,#155575,#155576,#155577,#155578,
#155579,#155580,#155581),(#155582,#155583,#155584,#155585,#155586,#155587,
#155588,#155589,#155590),(#155591,#155592,#155593,#155594,#155595,#155596,
#155597,#155598,#155599),(#155600,#155601,#155602,#155603,#155604,#155605,
#155606,#155607,#155608),(#155609,#155610,#155611,#155612,#155613,#155614,
#155615,#155616,#155617),(#155618,#155619,#155620,#155621,#155622,#155623,
#155624,#155625,#155626),(#155627,#155628,#155629,#155630,#155631,#155632,
#155633,#155634,#155635),(#155636,#155637,#155638,#155639,#155640,#155641,
#155642,#155643,#155644),(#155645,#155646,#155647,#155648,#155649,#155650,
#155651,#155652,#155653),(#155654,#155655,#155656,#155657,#155658,#155659,
#155660,#155661,#155662),(#155663,#155664,#155665,#155666,#155667,#155668,
#155669,#155670,#155671),(#155672,#155673,#155674,#155675,#155676,#155677,
#155678,#155679,#155680),(#155681,#155682,#155683,#155684,#155685,#155686,
#155687,#155688,#155689),(#155690,#155691,#155692,#155693,#155694,#155695,
#155696,#155697,#155698),(#155699,#155700,#155701,#155702,#155703,#155704,
#155705,#155706,#155707),(#155708,#155709,#155710,#155711,#155712,#155713,
#155714,#155715,#155716),(#155717,#155718,#155719,#155720,#155721,#155722,
#155723,#155724,#155725),(#155726,#155727,#155728,#155729,#155730,#155731,
#155732,#155733,#155734),(#155735,#155736,#155737,#155738,#155739,#155740,
#155741,#155742,#155743),(#155744,#155745,#155746,#155747,#155748,#155749,
#155750,#155751,#155752),(#155753,#155754,#155755,#155756,#155757,#155758,
#155759,#155760,#155761),(#155762,#155763,#155764,#155765,#155766,#155767,
#155768,#155769,#155770),(#155771,#155772,#155773,#155774,#155775,#155776,
#155777,#155778,#155779),(#155780,#155781,#155782,#155783,#155784,#155785,
#155786,#155787,#155788),(#155789,#155790,#155791,#155792,#155793,#155794,
#155795,#155796,#155797),(#155798,#155799,#155800,#155801,#155802,#155803,
#155804,#155805,#155806),(#155807,#155808,#155809,#155810,#155811,#155812,
#155813,#155814,#155815),(#155816,#155817,#155818,#155819,#155820,#155821,
#155822,#155823,#155824),(#155825,#155826,#155827,#155828,#155829,#155830,
#155831,#155832,#155833),(#155834,#155835,#155836,#155837,#155838,#155839,
#155840,#155841,#155842),(#155843,#155844,#155845,#155846,#155847,#155848,
#155849,#155850,#155851),(#155852,#155853,#155854,#155855,#155856,#155857,
#155858,#155859,#155860),(#155861,#155862,#155863,#155864,#155865,#155866,
#155867,#155868,#155869),(#155870,#155871,#155872,#155873,#155874,#155875,
#155876,#155877,#155878),(#155879,#155880,#155881,#155882,#155883,#155884,
#155885,#155886,#155887),(#155888,#155889,#155890,#155891,#155892,#155893,
#155894,#155895,#155896),(#155897,#155898,#155899,#155900,#155901,#155902,
#155903,#155904,#155905),(#155906,#155907,#155908,#155909,#155910,#155911,
#155912,#155913,#155914),(#155915,#155916,#155917,#155918,#155919,#155920,
#155921,#155922,#155923),(#155924,#155925,#155926,#155927,#155928,#155929,
#155930,#155931,#155932),(#155933,#155934,#155935,#155936,#155937,#155938,
#155939,#155940,#155941),(#155942,#155943,#155944,#155945,#155946,#155947,
#155948,#155949,#155950),(#155951,#155952,#155953,#155954,#155955,#155956,
#155957,#155958,#155959),(#155960,#155961,#155962,#155963,#155964,#155965,
#155966,#155967,#155968),(#155969,#155970,#155971,#155972,#155973,#155974,
#155975,#155976,#155977),(#155978,#155979,#155980,#155981,#155982,#155983,
#155984,#155985,#155986),(#155987,#155988,#155989,#155990,#155991,#155992,
#155993,#155994,#155995),(#155996,#155997,#155998,#155999,#156000,#156001,
#156002,#156003,#156004),(#156005,#156006,#156007,#156008,#156009,#156010,
#156011,#156012,#156013),(#156014,#156015,#156016,#156017,#156018,#156019,
#156020,#156021,#156022),(#156023,#156024,#156025,#156026,#156027,#156028,
#156029,#156030,#156031),(#156032,#156033,#156034,#156035,#156036,#156037,
#156038,#156039,#156040),(#156041,#156042,#156043,#156044,#156045,#156046,
#156047,#156048,#156049),(#156050,#156051,#156052,#156053,#156054,#156055,
#156056,#156057,#156058),(#156059,#156060,#156061,#156062,#156063,#156064,
#156065,#156066,#156067),(#156068,#156069,#156070,#156071,#156072,#156073,
#156074,#156075,#156076),(#156077,#156078,#156079,#156080,#156081,#156082,
#156083,#156084,#156085),(#156086,#156087,#156088,#156089,#156090,#156091,
#156092,#156093,#156094),(#156095,#156096,#156097,#156098,#156099,#156100,
#156101,#156102,#156103),(#156104,#156105,#156106,#156107,#156108,#156109,
#156110,#156111,#156112),(#156113,#156114,#156115,#156116,#156117,#156118,
#156119,#156120,#156121),(#156122,#156123,#156124,#156125,#156126,#156127,
#156128,#156129,#156130),(#156131,#156132,#156133,#156134,#156135,#156136,
#156137,#156138,#156139),(#156140,#156141,#156142,#156143,#156144,#156145,
#156146,#156147,#156148),(#156149,#156150,#156151,#156152,#156153,#156154,
#156155,#156156,#156157),(#156158,#156159,#156160,#156161,#156162,#156163,
#156164,#156165,#156166),(#156167,#156168,#156169,#156170,#156171,#156172,
#156173,#156174,#156175),(#156176,#156177,#156178,#156179,#156180,#156181,
#156182,#156183,#156184),(#156185,#156186,#156187,#156188,#156189,#156190,
#156191,#156192,#156193),(#156194,#156195,#156196,#156197,#156198,#156199,
#156200,#156201,#156202),(#156203,#156204,#156205,#156206,#156207,#156208,
#156209,#156210,#156211),(#156212,#156213,#156214,#156215,#156216,#156217,
#156218,#156219,#156220),(#156221,#156222,#156223,#156224,#156225,#156226,
#156227,#156228,#156229),(#156230,#156231,#156232,#156233,#156234,#156235,
#156236,#156237,#156238),(#156239,#156240,#156241,#156242,#156243,#156244,
#156245,#156246,#156247),(#156248,#156249,#156250,#156251,#156252,#156253,
#156254,#156255,#156256),(#156257,#156258,#156259,#156260,#156261,#156262,
#156263,#156264,#156265),(#156266,#156267,#156268,#156269,#156270,#156271,
#156272,#156273,#156274),(#156275,#156276,#156277,#156278,#156279,#156280,
#156281,#156282,#156283),(#156284,#156285,#156286,#156287,#156288,#156289,
#156290,#156291,#156292),(#156293,#156294,#156295,#156296,#156297,#156298,
#156299,#156300,#156301),(#156302,#156303,#156304,#156305,#156306,#156307,
#156308,#156309,#156310),(#156311,#156312,#156313,#156314,#156315,#156316,
#156317,#156318,#156319),(#156320,#156321,#156322,#156323,#156324,#156325,
#156326,#156327,#156328),(#156329,#156330,#156331,#156332,#156333,#156334,
#156335,#156336,#156337),(#156338,#156339,#156340,#156341,#156342,#156343,
#156344,#156345,#156346),(#156347,#156348,#156349,#156350,#156351,#156352,
#156353,#156354,#156355),(#156356,#156357,#156358,#156359,#156360,#156361,
#156362,#156363,#156364),(#156365,#156366,#156367,#156368,#156369,#156370,
#156371,#156372,#156373),(#156374,#156375,#156376,#156377,#156378,#156379,
#156380,#156381,#156382),(#156383,#156384,#156385,#156386,#156387,#156388,
#156389,#156390,#156391),(#156392,#156393,#156394,#156395,#156396,#156397,
#156398,#156399,#156400),(#156401,#156402,#156403,#156404,#156405,#156406,
#156407,#156408,#156409),(#156410,#156411,#156412,#156413,#156414,#156415,
#156416,#156417,#156418),(#156419,#156420,#156421,#156422,#156423,#156424,
#156425,#156426,#156427),(#156428,#156429,#156430,#156431,#156432,#156433,
#156434,#156435,#156436),(#156437,#156438,#156439,#156440,#156441,#156442,
#156443,#156444,#156445),(#156446,#156447,#156448,#156449,#156450,#156451,
#156452,#156453,#156454),(#156455,#156456,#156457,#156458,#156459,#156460,
#156461,#156462,#156463),(#156464,#156465,#156466,#156467,#156468,#156469,
#156470,#156471,#156472),(#156473,#156474,#156475,#156476,#156477,#156478,
#156479,#156480,#156481),(#156482,#156483,#156484,#156485,#156486,#156487,
#156488,#156489,#156490),(#156491,#156492,#156493,#156494,#156495,#156496,
#156497,#156498,#156499),(#156500,#156501,#156502,#156503,#156504,#156505,
#156506,#156507,#156508),(#156509,#156510,#156511,#156512,#156513,#156514,
#156515,#156516,#156517),(#156518,#156519,#156520,#156521,#156522,#156523,
#156524,#156525,#156526),(#156527,#156528,#156529,#156530,#156531,#156532,
#156533,#156534,#156535),(#156536,#156537,#156538,#156539,#156540,#156541,
#156542,#156543,#156544),(#156545,#156546,#156547,#156548,#156549,#156550,
#156551,#156552,#156553),(#156554,#156555,#156556,#156557,#156558,#156559,
#156560,#156561,#156562),(#156563,#156564,#156565,#156566,#156567,#156568,
#156569,#156570,#156571),(#156572,#156573,#156574,#156575,#156576,#156577,
#156578,#156579,#156580),(#156581,#156582,#156583,#156584,#156585,#156586,
#156587,#156588,#156589),(#156590,#156591,#156592,#156593,#156594,#156595,
#156596,#156597,#156598),(#156599,#156600,#156601,#156602,#156603,#156604,
#156605,#156606,#156607),(#156608,#156609,#156610,#156611,#156612,#156613,
#156614,#156615,#156616),(#156617,#156618,#156619,#156620,#156621,#156622,
#156623,#156624,#156625),(#156626,#156627,#156628,#156629,#156630,#156631,
#156632,#156633,#156634),(#156635,#156636,#156637,#156638,#156639,#156640,
#156641,#156642,#156643),(#156644,#156645,#156646,#156647,#156648,#156649,
#156650,#156651,#156652),(#156653,#156654,#156655,#156656,#156657,#156658,
#156659,#156660,#156661),(#156662,#156663,#156664,#156665,#156666,#156667,
#156668,#156669,#156670),(#156671,#156672,#156673,#156674,#156675,#156676,
#156677,#156678,#156679),(#156680,#156681,#156682,#156683,#156684,#156685,
#156686,#156687,#156688),(#156689,#156690,#156691,#156692,#156693,#156694,
#156695,#156696,#156697),(#156698,#156699,#156700,#156701,#156702,#156703,
#156704,#156705,#156706),(#156707,#156708,#156709,#156710,#156711,#156712,
#156713,#156714,#156715),(#156716,#156717,#156718,#156719,#156720,#156721,
#156722,#156723,#156724),(#156725,#156726,#156727,#156728,#156729,#156730,
#156731,#156732,#156733),(#156734,#156735,#156736,#156737,#156738,#156739,
#156740,#156741,#156742),(#156743,#156744,#156745,#156746,#156747,#156748,
#156749,#156750,#156751),(#156752,#156753,#156754,#156755,#156756,#156757,
#156758,#156759,#156760),(#156761,#156762,#156763,#156764,#156765,#156766,
#156767,#156768,#156769),(#156770,#156771,#156772,#156773,#156774,#156775,
#156776,#156777,#156778),(#156779,#156780,#156781,#156782,#156783,#156784,
#156785,#156786,#156787),(#156788,#156789,#156790,#156791,#156792,#156793,
#156794,#156795,#156796),(#156797,#156798,#156799,#156800,#156801,#156802,
#156803,#156804,#156805),(#156806,#156807,#156808,#156809,#156810,#156811,
#156812,#156813,#156814),(#156815,#156816,#156817,#156818,#156819,#156820,
#156821,#156822,#156823),(#156824,#156825,#156826,#156827,#156828,#156829,
#156830,#156831,#156832),(#156833,#156834,#156835,#156836,#156837,#156838,
#156839,#156840,#156841),(#156842,#156843,#156844,#156845,#156846,#156847,
#156848,#156849,#156850),(#156851,#156852,#156853,#156854,#156855,#156856,
#156857,#156858,#156859),(#156860,#156861,#156862,#156863,#156864,#156865,
#156866,#156867,#156868),(#156869,#156870,#156871,#156872,#156873,#156874,
#156875,#156876,#156877),(#156878,#156879,#156880,#156881,#156882,#156883,
#156884,#156885,#156886),(#156887,#156888,#156889,#156890,#156891,#156892,
#156893,#156894,#156895),(#156896,#156897,#156898,#156899,#156900,#156901,
#156902,#156903,#156904),(#156905,#156906,#156907,#156908,#156909,#156910,
#156911,#156912,#156913),(#156914,#156915,#156916,#156917,#156918,#156919,
#156920,#156921,#156922),(#156923,#156924,#156925,#156926,#156927,#156928,
#156929,#156930,#156931),(#156932,#156933,#156934,#156935,#156936,#156937,
#156938,#156939,#156940),(#156941,#156942,#156943,#156944,#156945,#156946,
#156947,#156948,#156949),(#156950,#156951,#156952,#156953,#156954,#156955,
#156956,#156957,#156958),(#156959,#156960,#156961,#156962,#156963,#156964,
#156965,#156966,#156967),(#156968,#156969,#156970,#156971,#156972,#156973,
#156974,#156975,#156976),(#156977,#156978,#156979,#156980,#156981,#156982,
#156983,#156984,#156985),(#156986,#156987,#156988,#156989,#156990,#156991,
#156992,#156993,#156994),(#156995,#156996,#156997,#156998,#156999,#157000,
#157001,#157002,#157003),(#157004,#157005,#157006,#157007,#157008,#157009,
#157010,#157011,#157012),(#157013,#157014,#157015,#157016,#157017,#157018,
#157019,#157020,#157021),(#157022,#157023,#157024,#157025,#157026,#157027,
#157028,#157029,#157030),(#157031,#157032,#157033,#157034,#157035,#157036,
#157037,#157038,#157039),(#157040,#157041,#157042,#157043,#157044,#157045,
#157046,#157047,#157048),(#157049,#157050,#157051,#157052,#157053,#157054,
#157055,#157056,#157057),(#157058,#157059,#157060,#157061,#157062,#157063,
#157064,#157065,#157066),(#157067,#157068,#157069,#157070,#157071,#157072,
#157073,#157074,#157075),(#157076,#157077,#157078,#157079,#157080,#157081,
#157082,#157083,#157084),(#157085,#157086,#157087,#157088,#157089,#157090,
#157091,#157092,#157093),(#157094,#157095,#157096,#157097,#157098,#157099,
#157100,#157101,#157102),(#157103,#157104,#157105,#157106,#157107,#157108,
#157109,#157110,#157111),(#157112,#157113,#157114,#157115,#157116,#157117,
#157118,#157119,#157120),(#157121,#157122,#157123,#157124,#157125,#157126,
#157127,#157128,#157129),(#157130,#157131,#157132,#157133,#157134,#157135,
#157136,#157137,#157138),(#157139,#157140,#157141,#157142,#157143,#157144,
#157145,#157146,#157147),(#157148,#157149,#157150,#157151,#157152,#157153,
#157154,#157155,#157156),(#157157,#157158,#157159,#157160,#157161,#157162,
#157163,#157164,#157165),(#157166,#157167,#157168,#157169,#157170,#157171,
#157172,#157173,#157174),(#157175,#157176,#157177,#157178,#157179,#157180,
#157181,#157182,#157183),(#157184,#157185,#157186,#157187,#157188,#157189,
#157190,#157191,#157192),(#157193,#157194,#157195,#157196,#157197,#157198,
#157199,#157200,#157201),(#157202,#157203,#157204,#157205,#157206,#157207,
#157208,#157209,#157210),(#157211,#157212,#157213,#157214,#157215,#157216,
#157217,#157218,#157219),(#157220,#157221,#157222,#157223,#157224,#157225,
#157226,#157227,#157228),(#157229,#157230,#157231,#157232,#157233,#157234,
#157235,#157236,#157237),(#157238,#157239,#157240,#157241,#157242,#157243,
#157244,#157245,#157246),(#157247,#157248,#157249,#157250,#157251,#157252,
#157253,#157254,#157255),(#157256,#157257,#157258,#157259,#157260,#157261,
#157262,#157263,#157264),(#157265,#157266,#157267,#157268,#157269,#157270,
#157271,#157272,#157273),(#157274,#157275,#157276,#157277,#157278,#157279,
#157280,#157281,#157282),(#157283,#157284,#157285,#157286,#157287,#157288,
#157289,#157290,#157291),(#157292,#157293,#157294,#157295,#157296,#157297,
#157298,#157299,#157300),(#157301,#157302,#157303,#157304,#157305,#157306,
#157307,#157308,#157309),(#157310,#157311,#157312,#157313,#157314,#157315,
#157316,#157317,#157318),(#157319,#157320,#157321,#157322,#157323,#157324,
#157325,#157326,#157327),(#157328,#157329,#157330,#157331,#157332,#157333,
#157334,#157335,#157336),(#157337,#157338,#157339,#157340,#157341,#157342,
#157343,#157344,#157345),(#157346,#157347,#157348,#157349,#157350,#157351,
#157352,#157353,#157354),(#157355,#157356,#157357,#157358,#157359,#157360,
#157361,#157362,#157363),(#157364,#157365,#157366,#157367,#157368,#157369,
#157370,#157371,#157372),(#157373,#157374,#157375,#157376,#157377,#157378,
#157379,#157380,#157381),(#157382,#157383,#157384,#157385,#157386,#157387,
#157388,#157389,#157390),(#157391,#157392,#157393,#157394,#157395,#157396,
#157397,#157398,#157399),(#157400,#157401,#157402,#157403,#157404,#157405,
#157406,#157407,#157408),(#157409,#157410,#157411,#157412,#157413,#157414,
#157415,#157416,#157417),(#157418,#157419,#157420,#157421,#157422,#157423,
#157424,#157425,#157426),(#157427,#157428,#157429,#157430,#157431,#157432,
#157433,#157434,#157435),(#157436,#157437,#157438,#157439,#157440,#157441,
#157442,#157443,#157444),(#157445,#157446,#157447,#157448,#157449,#157450,
#157451,#157452,#157453),(#157454,#157455,#157456,#157457,#157458,#157459,
#157460,#157461,#157462),(#157463,#157464,#157465,#157466,#157467,#157468,
#157469,#157470,#157471),(#157472,#157473,#157474,#157475,#157476,#157477,
#157478,#157479,#157480),(#157481,#157482,#157483,#157484,#157485,#157486,
#157487,#157488,#157489),(#157490,#157491,#157492,#157493,#157494,#157495,
#157496,#157497,#157498),(#157499,#157500,#157501,#157502,#157503,#157504,
#157505,#157506,#157507),(#157508,#157509,#157510,#157511,#157512,#157513,
#157514,#157515,#157516),(#157517,#157518,#157519,#157520,#157521,#157522,
#157523,#157524,#157525),(#157526,#157527,#157528,#157529,#157530,#157531,
#157532,#157533,#157534),(#157535,#157536,#157537,#157538,#157539,#157540,
#157541,#157542,#157543),(#157544,#157545,#157546,#157547,#157548,#157549,
#157550,#157551,#157552),(#157553,#157554,#157555,#157556,#157557,#157558,
#157559,#157560,#157561),(#157562,#157563,#157564,#157565,#157566,#157567,
#157568,#157569,#157570),(#157571,#157572,#157573,#157574,#157575,#157576,
#157577,#157578,#157579),(#157580,#157581,#157582,#157583,#157584,#157585,
#157586,#157587,#157588),(#157589,#157590,#157591,#157592,#157593,#157594,
#157595,#157596,#157597),(#157598,#157599,#157600,#157601,#157602,#157603,
#157604,#157605,#157606),(#157607,#157608,#157609,#157610,#157611,#157612,
#157613,#157614,#157615),(#157616,#157617,#157618,#157619,#157620,#157621,
#157622,#157623,#157624),(#157625,#157626,#157627,#157628,#157629,#157630,
#157631,#157632,#157633),(#157634,#157635,#157636,#157637,#157638,#157639,
#157640,#157641,#157642),(#157643,#157644,#157645,#157646,#157647,#157648,
#157649,#157650,#157651),(#157652,#157653,#157654,#157655,#157656,#157657,
#157658,#157659,#157660),(#157661,#157662,#157663,#157664,#157665,#157666,
#157667,#157668,#157669),(#157670,#157671,#157672,#157673,#157674,#157675,
#157676,#157677,#157678),(#157679,#157680,#157681,#157682,#157683,#157684,
#157685,#157686,#157687),(#157688,#157689,#157690,#157691,#157692,#157693,
#157694,#157695,#157696),(#157697,#157698,#157699,#157700,#157701,#157702,
#157703,#157704,#157705),(#157706,#157707,#157708,#157709,#157710,#157711,
#157712,#157713,#157714),(#157715,#157716,#157717,#157718,#157719,#157720,
#157721,#157722,#157723),(#157724,#157725,#157726,#157727,#157728,#157729,
#157730,#157731,#157732),(#157733,#157734,#157735,#157736,#157737,#157738,
#157739,#157740,#157741),(#157742,#157743,#157744,#157745,#157746,#157747,
#157748,#157749,#157750),(#157751,#157752,#157753,#157754,#157755,#157756,
#157757,#157758,#157759),(#157760,#157761,#157762,#157763,#157764,#157765,
#157766,#157767,#157768),(#157769,#157770,#157771,#157772,#157773,#157774,
#157775,#157776,#157777),(#157778,#157779,#157780,#157781,#157782,#157783,
#157784,#157785,#157786),(#157787,#157788,#157789,#157790,#157791,#157792,
#157793,#157794,#157795),(#157796,#157797,#157798,#157799,#157800,#157801,
#157802,#157803,#157804),(#157805,#157806,#157807,#157808,#157809,#157810,
#157811,#157812,#157813),(#157814,#157815,#157816,#157817,#157818,#157819,
#157820,#157821,#157822),(#157823,#157824,#157825,#157826,#157827,#157828,
#157829,#157830,#157831),(#157832,#157833,#157834,#157835,#157836,#157837,
#157838,#157839,#157840),(#157841,#157842,#157843,#157844,#157845,#157846,
#157847,#157848,#157849),(#157850,#157851,#157852,#157853,#157854,#157855,
#157856,#157857,#157858),(#157859,#157860,#157861,#157862,#157863,#157864,
#157865,#157866,#157867),(#157868,#157869,#157870,#157871,#157872,#157873,
#157874,#157875,#157876),(#157877,#157878,#157879,#157880,#157881,#157882,
#157883,#157884,#157885),(#157886,#157887,#157888,#157889,#157890,#157891,
#157892,#157893,#157894),(#157895,#157896,#157897,#157898,#157899,#157900,
#157901,#157902,#157903),(#157904,#157905,#157906,#157907,#157908,#157909,
#157910,#157911,#157912),(#157913,#157914,#157915,#157916,#157917,#157918,
#157919,#157920,#157921),(#157922,#157923,#157924,#157925,#157926,#157927,
#157928,#157929,#157930),(#157931,#157932,#157933,#157934,#157935,#157936,
#157937,#157938,#157939),(#157940,#157941,#157942,#157943,#157944,#157945,
#157946,#157947,#157948),(#157949,#157950,#157951,#157952,#157953,#157954,
#157955,#157956,#157957),(#157958,#157959,#157960,#157961,#157962,#157963,
#157964,#157965,#157966),(#157967,#157968,#157969,#157970,#157971,#157972,
#157973,#157974,#157975),(#157976,#157977,#157978,#157979,#157980,#157981,
#157982,#157983,#157984),(#157985,#157986,#157987,#157988,#157989,#157990,
#157991,#157992,#157993),(#157994,#157995,#157996,#157997,#157998,#157999,
#158000,#158001,#158002),(#158003,#158004,#158005,#158006,#158007,#158008,
#158009,#158010,#158011),(#158012,#158013,#158014,#158015,#158016,#158017,
#158018,#158019,#158020),(#158021,#158022,#158023,#158024,#158025,#158026,
#158027,#158028,#158029),(#158030,#158031,#158032,#158033,#158034,#158035,
#158036,#158037,#158038),(#158039,#158040,#158041,#158042,#158043,#158044,
#158045,#158046,#158047),(#158048,#158049,#158050,#158051,#158052,#158053,
#158054,#158055,#158056),(#158057,#158058,#158059,#158060,#158061,#158062,
#158063,#158064,#158065),(#158066,#158067,#158068,#158069,#158070,#158071,
#158072,#158073,#158074),(#158075,#158076,#158077,#158078,#158079,#158080,
#158081,#158082,#158083),(#158084,#158085,#158086,#158087,#158088,#158089,
#158090,#158091,#158092),(#158093,#158094,#158095,#158096,#158097,#158098,
#158099,#158100,#158101),(#158102,#158103,#158104,#158105,#158106,#158107,
#158108,#158109,#158110),(#158111,#158112,#158113,#158114,#158115,#158116,
#158117,#158118,#158119),(#158120,#158121,#158122,#158123,#158124,#158125,
#158126,#158127,#158128),(#158129,#158130,#158131,#158132,#158133,#158134,
#158135,#158136,#158137),(#158138,#158139,#158140,#158141,#158142,#158143,
#158144,#158145,#158146),(#158147,#158148,#158149,#158150,#158151,#158152,
#158153,#158154,#158155),(#158156,#158157,#158158,#158159,#158160,#158161,
#158162,#158163,#158164),(#158165,#158166,#158167,#158168,#158169,#158170,
#158171,#158172,#158173),(#158174,#158175,#158176,#158177,#158178,#158179,
#158180,#158181,#158182),(#158183,#158184,#158185,#158186,#158187,#158188,
#158189,#158190,#158191),(#158192,#158193,#158194,#158195,#158196,#158197,
#158198,#158199,#158200),(#158201,#158202,#158203,#158204,#158205,#158206,
#158207,#158208,#158209),(#158210,#158211,#158212,#158213,#158214,#158215,
#158216,#158217,#158218),(#158219,#158220,#158221,#158222,#158223,#158224,
#158225,#158226,#158227),(#158228,#158229,#158230,#158231,#158232,#158233,
#158234,#158235,#158236),(#158237,#158238,#158239,#158240,#158241,#158242,
#158243,#158244,#158245),(#158246,#158247,#158248,#158249,#158250,#158251,
#158252,#158253,#158254),(#158255,#158256,#158257,#158258,#158259,#158260,
#158261,#158262,#158263),(#158264,#158265,#158266,#158267,#158268,#158269,
#158270,#158271,#158272),(#158273,#158274,#158275,#158276,#158277,#158278,
#158279,#158280,#158281),(#158282,#158283,#158284,#158285,#158286,#158287,
#158288,#158289,#158290),(#158291,#158292,#158293,#158294,#158295,#158296,
#158297,#158298,#158299),(#158300,#158301,#158302,#158303,#158304,#158305,
#158306,#158307,#158308),(#158309,#158310,#158311,#158312,#158313,#158314,
#158315,#158316,#158317),(#158318,#158319,#158320,#158321,#158322,#158323,
#158324,#158325,#158326),(#158327,#158328,#158329,#158330,#158331,#158332,
#158333,#158334,#158335),(#158336,#158337,#158338,#158339,#158340,#158341,
#158342,#158343,#158344),(#158345,#158346,#158347,#158348,#158349,#158350,
#158351,#158352,#158353),(#158354,#158355,#158356,#158357,#158358,#158359,
#158360,#158361,#158362),(#158363,#158364,#158365,#158366,#158367,#158368,
#158369,#158370,#158371),(#158372,#158373,#158374,#158375,#158376,#158377,
#158378,#158379,#158380),(#158381,#158382,#158383,#158384,#158385,#158386,
#158387,#158388,#158389),(#158390,#158391,#158392,#158393,#158394,#158395,
#158396,#158397,#158398),(#158399,#158400,#158401,#158402,#158403,#158404,
#158405,#158406,#158407),(#158408,#158409,#158410,#158411,#158412,#158413,
#158414,#158415,#158416),(#158417,#158418,#158419,#158420,#158421,#158422,
#158423,#158424,#158425),(#158426,#158427,#158428,#158429,#158430,#158431,
#158432,#158433,#158434),(#158435,#158436,#158437,#158438,#158439,#158440,
#158441,#158442,#158443),(#158444,#158445,#158446,#158447,#158448,#158449,
#158450,#158451,#158452),(#158453,#158454,#158455,#158456,#158457,#158458,
#158459,#158460,#158461),(#158462,#158463,#158464,#158465,#158466,#158467,
#158468,#158469,#158470),(#158471,#158472,#158473,#158474,#158475,#158476,
#158477,#158478,#158479),(#158480,#158481,#158482,#158483,#158484,#158485,
#158486,#158487,#158488),(#158489,#158490,#158491,#158492,#158493,#158494,
#158495,#158496,#158497),(#158498,#158499,#158500,#158501,#158502,#158503,
#158504,#158505,#158506),(#158507,#158508,#158509,#158510,#158511,#158512,
#158513,#158514,#158515),(#158516,#158517,#158518,#158519,#158520,#158521,
#158522,#158523,#158524),(#158525,#158526,#158527,#158528,#158529,#158530,
#158531,#158532,#158533),(#158534,#158535,#158536,#158537,#158538,#158539,
#158540,#158541,#158542),(#158543,#158544,#158545,#158546,#158547,#158548,
#158549,#158550,#158551),(#158552,#158553,#158554,#158555,#158556,#158557,
#158558,#158559,#158560),(#158561,#158562,#158563,#158564,#158565,#158566,
#158567,#158568,#158569),(#158570,#158571,#158572,#158573,#158574,#158575,
#158576,#158577,#158578),(#158579,#158580,#158581,#158582,#158583,#158584,
#158585,#158586,#158587),(#158588,#158589,#158590,#158591,#158592,#158593,
#158594,#158595,#158596),(#158597,#158598,#158599,#158600,#158601,#158602,
#158603,#158604,#158605),(#158606,#158607,#158608,#158609,#158610,#158611,
#158612,#158613,#158614),(#158615,#158616,#158617,#158618,#158619,#158620,
#158621,#158622,#158623),(#158624,#158625,#158626,#158627,#158628,#158629,
#158630,#158631,#158632),(#158633,#158634,#158635,#158636,#158637,#158638,
#158639,#158640,#158641),(#158642,#158643,#158644,#158645,#158646,#158647,
#158648,#158649,#158650),(#158651,#158652,#158653,#158654,#158655,#158656,
#158657,#158658,#158659),(#158660,#158661,#158662,#158663,#158664,#158665,
#158666,#158667,#158668),(#158669,#158670,#158671,#158672,#158673,#158674,
#158675,#158676,#158677),(#158678,#158679,#158680,#158681,#158682,#158683,
#158684,#158685,#158686),(#158687,#158688,#158689,#158690,#158691,#158692,
#158693,#158694,#158695),(#158696,#158697,#158698,#158699,#158700,#158701,
#158702,#158703,#158704),(#158705,#158706,#158707,#158708,#158709,#158710,
#158711,#158712,#158713),(#158714,#158715,#158716,#158717,#158718,#158719,
#158720,#158721,#158722),(#158723,#158724,#158725,#158726,#158727,#158728,
#158729,#158730,#158731),(#158732,#158733,#158734,#158735,#158736,#158737,
#158738,#158739,#158740),(#158741,#158742,#158743,#158744,#158745,#158746,
#158747,#158748,#158749),(#158750,#158751,#158752,#158753,#158754,#158755,
#158756,#158757,#158758),(#158759,#158760,#158761,#158762,#158763,#158764,
#158765,#158766,#158767),(#158768,#158769,#158770,#158771,#158772,#158773,
#158774,#158775,#158776),(#158777,#158778,#158779,#158780,#158781,#158782,
#158783,#158784,#158785),(#158786,#158787,#158788,#158789,#158790,#158791,
#158792,#158793,#158794),(#158795,#158796,#158797,#158798,#158799,#158800,
#158801,#158802,#158803),(#158804,#158805,#158806,#158807,#158808,#158809,
#158810,#158811,#158812),(#158813,#158814,#158815,#158816,#158817,#158818,
#158819,#158820,#158821),(#158822,#158823,#158824,#158825,#158826,#158827,
#158828,#158829,#158830),(#158831,#158832,#158833,#158834,#158835,#158836,
#158837,#158838,#158839),(#158840,#158841,#158842,#158843,#158844,#158845,
#158846,#158847,#158848),(#158849,#158850,#158851,#158852,#158853,#158854,
#158855,#158856,#158857),(#158858,#158859,#158860,#158861,#158862,#158863,
#158864,#158865,#158866),(#158867,#158868,#158869,#158870,#158871,#158872,
#158873,#158874,#158875),(#158876,#158877,#158878,#158879,#158880,#158881,
#158882,#158883,#158884),(#158885,#158886,#158887,#158888,#158889,#158890,
#158891,#158892,#158893),(#158894,#158895,#158896,#158897,#158898,#158899,
#158900,#158901,#158902),(#158903,#158904,#158905,#158906,#158907,#158908,
#158909,#158910,#158911),(#158912,#158913,#158914,#158915,#158916,#158917,
#158918,#158919,#158920),(#158921,#158922,#158923,#158924,#158925,#158926,
#158927,#158928,#158929),(#158930,#158931,#158932,#158933,#158934,#158935,
#158936,#158937,#158938),(#158939,#158940,#158941,#158942,#158943,#158944,
#158945,#158946,#158947),(#158948,#158949,#158950,#158951,#158952,#158953,
#158954,#158955,#158956),(#158957,#158958,#158959,#158960,#158961,#158962,
#158963,#158964,#158965),(#158966,#158967,#158968,#158969,#158970,#158971,
#158972,#158973,#158974),(#158975,#158976,#158977,#158978,#158979,#158980,
#158981,#158982,#158983),(#158984,#158985,#158986,#158987,#158988,#158989,
#158990,#158991,#158992),(#158993,#158994,#158995,#158996,#158997,#158998,
#158999,#159000,#159001),(#159002,#159003,#159004,#159005,#159006,#159007,
#159008,#159009,#159010),(#159011,#159012,#159013,#159014,#159015,#159016,
#159017,#159018,#159019),(#159020,#159021,#159022,#159023,#159024,#159025,
#159026,#159027,#159028),(#159029,#159030,#159031,#159032,#159033,#159034,
#159035,#159036,#159037),(#159038,#159039,#159040,#159041,#159042,#159043,
#159044,#159045,#159046),(#159047,#159048,#159049,#159050,#159051,#159052,
#159053,#159054,#159055),(#159056,#159057,#159058,#159059,#159060,#159061,
#159062,#159063,#159064),(#159065,#159066,#159067,#159068,#159069,#159070,
#159071,#159072,#159073),(#159074,#159075,#159076,#159077,#159078,#159079,
#159080,#159081,#159082),(#159083,#159084,#159085,#159086,#159087,#159088,
#159089,#159090,#159091),(#159092,#159093,#159094,#159095,#159096,#159097,
#159098,#159099,#159100),(#159101,#159102,#159103,#159104,#159105,#159106,
#159107,#159108,#159109),(#159110,#159111,#159112,#159113,#159114,#159115,
#159116,#159117,#159118),(#159119,#159120,#159121,#159122,#159123,#159124,
#159125,#159126,#159127),(#159128,#159129,#159130,#159131,#159132,#159133,
#159134,#159135,#159136),(#159137,#159138,#159139,#159140,#159141,#159142,
#159143,#159144,#159145),(#159146,#159147,#159148,#159149,#159150,#159151,
#159152,#159153,#159154),(#159155,#159156,#159157,#159158,#159159,#159160,
#159161,#159162,#159163),(#159164,#159165,#159166,#159167,#159168,#159169,
#159170,#159171,#159172),(#159173,#159174,#159175,#159176,#159177,#159178,
#159179,#159180,#159181),(#159182,#159183,#159184,#159185,#159186,#159187,
#159188,#159189,#159190),(#159191,#159192,#159193,#159194,#159195,#159196,
#159197,#159198,#159199),(#159200,#159201,#159202,#159203,#159204,#159205,
#159206,#159207,#159208),(#159209,#159210,#159211,#159212,#159213,#159214,
#159215,#159216,#159217),(#159218,#159219,#159220,#159221,#159222,#159223,
#159224,#159225,#159226),(#159227,#159228,#159229,#159230,#159231,#159232,
#159233,#159234,#159235),(#159236,#159237,#159238,#159239,#159240,#159241,
#159242,#159243,#159244),(#159245,#159246,#159247,#159248,#159249,#159250,
#159251,#159252,#159253),(#159254,#159255,#159256,#159257,#159258,#159259,
#159260,#159261,#159262),(#159263,#159264,#159265,#159266,#159267,#159268,
#159269,#159270,#159271),(#159272,#159273,#159274,#159275,#159276,#159277,
#159278,#159279,#159280),(#159281,#159282,#159283,#159284,#159285,#159286,
#159287,#159288,#159289),(#159290,#159291,#159292,#159293,#159294,#159295,
#159296,#159297,#159298),(#159299,#159300,#159301,#159302,#159303,#159304,
#159305,#159306,#159307),(#159308,#159309,#159310,#159311,#159312,#159313,
#159314,#159315,#159316),(#159317,#159318,#159319,#159320,#159321,#159322,
#159323,#159324,#159325),(#159326,#159327,#159328,#159329,#159330,#159331,
#159332,#159333,#159334),(#159335,#159336,#159337,#159338,#159339,#159340,
#159341,#159342,#159343),(#159344,#159345,#159346,#159347,#159348,#159349,
#159350,#159351,#159352),(#159353,#159354,#159355,#159356,#159357,#159358,
#159359,#159360,#159361),(#159362,#159363,#159364,#159365,#159366,#159367,
#159368,#159369,#159370),(#159371,#159372,#159373,#159374,#159375,#159376,
#159377,#159378,#159379),(#159380,#159381,#159382,#159383,#159384,#159385,
#159386,#159387,#159388),(#159389,#159390,#159391,#159392,#159393,#159394,
#159395,#159396,#159397),(#159398,#159399,#159400,#159401,#159402,#159403,
#159404,#159405,#159406),(#159407,#159408,#159409,#159410,#159411,#159412,
#159413,#159414,#159415),(#159416,#159417,#159418,#159419,#159420,#159421,
#159422,#159423,#159424),(#159425,#159426,#159427,#159428,#159429,#159430,
#159431,#159432,#159433),(#159434,#159435,#159436,#159437,#159438,#159439,
#159440,#159441,#159442),(#159443,#159444,#159445,#159446,#159447,#159448,
#159449,#159450,#159451),(#159452,#159453,#159454,#159455,#159456,#159457,
#159458,#159459,#159460),(#159461,#159462,#159463,#159464,#159465,#159466,
#159467,#159468,#159469),(#159470,#159471,#159472,#159473,#159474,#159475,
#159476,#159477,#159478),(#159479,#159480,#159481,#159482,#159483,#159484,
#159485,#159486,#159487),(#159488,#159489,#159490,#159491,#159492,#159493,
#159494,#159495,#159496),(#159497,#159498,#159499,#159500,#159501,#159502,
#159503,#159504,#159505),(#159506,#159507,#159508,#159509,#159510,#159511,
#159512,#159513,#159514),(#159515,#159516,#159517,#159518,#159519,#159520,
#159521,#159522,#159523),(#159524,#159525,#159526,#159527,#159528,#159529,
#159530,#159531,#159532),(#159533,#159534,#159535,#159536,#159537,#159538,
#159539,#159540,#159541),(#159542,#159543,#159544,#159545,#159546,#159547,
#159548,#159549,#159550),(#159551,#159552,#159553,#159554,#159555,#159556,
#159557,#159558,#159559),(#159560,#159561,#159562,#159563,#159564,#159565,
#159566,#159567,#159568),(#159569,#159570,#159571,#159572,#159573,#159574,
#159575,#159576,#159577),(#159578,#159579,#159580,#159581,#159582,#159583,
#159584,#159585,#159586),(#159587,#159588,#159589,#159590,#159591,#159592,
#159593,#159594,#159595),(#159596,#159597,#159598,#159599,#159600,#159601,
#159602,#159603,#159604),(#159605,#159606,#159607,#159608,#159609,#159610,
#159611,#159612,#159613),(#159614,#159615,#159616,#159617,#159618,#159619,
#159620,#159621,#159622),(#159623,#159624,#159625,#159626,#159627,#159628,
#159629,#159630,#159631),(#159632,#159633,#159634,#159635,#159636,#159637,
#159638,#159639,#159640),(#159641,#159642,#159643,#159644,#159645,#159646,
#159647,#159648,#159649),(#159650,#159651,#159652,#159653,#159654,#159655,
#159656,#159657,#159658),(#159659,#159660,#159661,#159662,#159663,#159664,
#159665,#159666,#159667),(#159668,#159669,#159670,#159671,#159672,#159673,
#159674,#159675,#159676),(#159677,#159678,#159679,#159680,#159681,#159682,
#159683,#159684,#159685),(#159686,#159687,#159688,#159689,#159690,#159691,
#159692,#159693,#159694),(#159695,#159696,#159697,#159698,#159699,#159700,
#159701,#159702,#159703),(#159704,#159705,#159706,#159707,#159708,#159709,
#159710,#159711,#159712),(#159713,#159714,#159715,#159716,#159717,#159718,
#159719,#159720,#159721),(#159722,#159723,#159724,#159725,#159726,#159727,
#159728,#159729,#159730),(#159731,#159732,#159733,#159734,#159735,#159736,
#159737,#159738,#159739),(#159740,#159741,#159742,#159743,#159744,#159745,
#159746,#159747,#159748),(#159749,#159750,#159751,#159752,#159753,#159754,
#159755,#159756,#159757),(#159758,#159759,#159760,#159761,#159762,#159763,
#159764,#159765,#159766),(#159767,#159768,#159769,#159770,#159771,#159772,
#159773,#159774,#159775),(#159776,#159777,#159778,#159779,#159780,#159781,
#159782,#159783,#159784),(#159785,#159786,#159787,#159788,#159789,#159790,
#159791,#159792,#159793),(#159794,#159795,#159796,#159797,#159798,#159799,
#159800,#159801,#159802),(#159803,#159804,#159805,#159806,#159807,#159808,
#159809,#159810,#159811),(#159812,#159813,#159814,#159815,#159816,#159817,
#159818,#159819,#159820),(#159821,#159822,#159823,#159824,#159825,#159826,
#159827,#159828,#159829),(#159830,#159831,#159832,#159833,#159834,#159835,
#159836,#159837,#159838),(#159839,#159840,#159841,#159842,#159843,#159844,
#159845,#159846,#159847),(#159848,#159849,#159850,#159851,#159852,#159853,
#159854,#159855,#159856),(#159857,#159858,#159859,#159860,#159861,#159862,
#159863,#159864,#159865),(#159866,#159867,#159868,#159869,#159870,#159871,
#159872,#159873,#159874),(#159875,#159876,#159877,#159878,#159879,#159880,
#159881,#159882,#159883),(#159884,#159885,#159886,#159887,#159888,#159889,
#159890,#159891,#159892),(#159893,#159894,#159895,#159896,#159897,#159898,
#159899,#159900,#159901),(#159902,#159903,#159904,#159905,#159906,#159907,
#159908,#159909,#159910),(#159911,#159912,#159913,#159914,#159915,#159916,
#159917,#159918,#159919),(#159920,#159921,#159922,#159923,#159924,#159925,
#159926,#159927,#159928),(#159929,#159930,#159931,#159932,#159933,#159934,
#159935,#159936,#159937),(#159938,#159939,#159940,#159941,#159942,#159943,
#159944,#159945,#159946),(#159947,#159948,#159949,#159950,#159951,#159952,
#159953,#159954,#159955),(#159956,#159957,#159958,#159959,#159960,#159961,
#159962,#159963,#159964),(#159965,#159966,#159967,#159968,#159969,#159970,
#159971,#159972,#159973),(#159974,#159975,#159976,#159977,#159978,#159979,
#159980,#159981,#159982),(#159983,#159984,#159985,#159986,#159987,#159988,
#159989,#159990,#159991),(#159992,#159993,#159994,#159995,#159996,#159997,
#159998,#159999,#160000),(#160001,#160002,#160003,#160004,#160005,#160006,
#160007,#160008,#160009),(#160010,#160011,#160012,#160013,#160014,#160015,
#160016,#160017,#160018),(#160019,#160020,#160021,#160022,#160023,#160024,
#160025,#160026,#160027),(#160028,#160029,#160030,#160031,#160032,#160033,
#160034,#160035,#160036),(#160037,#160038,#160039,#160040,#160041,#160042,
#160043,#160044,#160045),(#160046,#160047,#160048,#160049,#160050,#160051,
#160052,#160053,#160054),(#160055,#160056,#160057,#160058,#160059,#160060,
#160061,#160062,#160063),(#160064,#160065,#160066,#160067,#160068,#160069,
#160070,#160071,#160072),(#160073,#160074,#160075,#160076,#160077,#160078,
#160079,#160080,#160081),(#160082,#160083,#160084,#160085,#160086,#160087,
#160088,#160089,#160090),(#160091,#160092,#160093,#160094,#160095,#160096,
#160097,#160098,#160099),(#160100,#160101,#160102,#160103,#160104,#160105,
#160106,#160107,#160108),(#160109,#160110,#160111,#160112,#160113,#160114,
#160115,#160116,#160117),(#160118,#160119,#160120,#160121,#160122,#160123,
#160124,#160125,#160126),(#160127,#160128,#160129,#160130,#160131,#160132,
#160133,#160134,#160135),(#160136,#160137,#160138,#160139,#160140,#160141,
#160142,#160143,#160144),(#160145,#160146,#160147,#160148,#160149,#160150,
#160151,#160152,#160153),(#160154,#160155,#160156,#160157,#160158,#160159,
#160160,#160161,#160162),(#160163,#160164,#160165,#160166,#160167,#160168,
#160169,#160170,#160171),(#160172,#160173,#160174,#160175,#160176,#160177,
#160178,#160179,#160180),(#160181,#160182,#160183,#160184,#160185,#160186,
#160187,#160188,#160189),(#160190,#160191,#160192,#160193,#160194,#160195,
#160196,#160197,#160198),(#160199,#160200,#160201,#160202,#160203,#160204,
#160205,#160206,#160207),(#160208,#160209,#160210,#160211,#160212,#160213,
#160214,#160215,#160216),(#160217,#160218,#160219,#160220,#160221,#160222,
#160223,#160224,#160225),(#160226,#160227,#160228,#160229,#160230,#160231,
#160232,#160233,#160234),(#160235,#160236,#160237,#160238,#160239,#160240,
#160241,#160242,#160243),(#160244,#160245,#160246,#160247,#160248,#160249,
#160250,#160251,#160252),(#160253,#160254,#160255,#160256,#160257,#160258,
#160259,#160260,#160261),(#160262,#160263,#160264,#160265,#160266,#160267,
#160268,#160269,#160270),(#160271,#160272,#160273,#160274,#160275,#160276,
#160277,#160278,#160279),(#160280,#160281,#160282,#160283,#160284,#160285,
#160286,#160287,#160288),(#160289,#160290,#160291,#160292,#160293,#160294,
#160295,#160296,#160297),(#160298,#160299,#160300,#160301,#160302,#160303,
#160304,#160305,#160306),(#160307,#160308,#160309,#160310,#160311,#160312,
#160313,#160314,#160315),(#160316,#160317,#160318,#160319,#160320,#160321,
#160322,#160323,#160324),(#160325,#160326,#160327,#160328,#160329,#160330,
#160331,#160332,#160333),(#160334,#160335,#160336,#160337,#160338,#160339,
#160340,#160341,#160342),(#160343,#160344,#160345,#160346,#160347,#160348,
#160349,#160350,#160351),(#160352,#160353,#160354,#160355,#160356,#160357,
#160358,#160359,#160360),(#160361,#160362,#160363,#160364,#160365,#160366,
#160367,#160368,#160369),(#160370,#160371,#160372,#160373,#160374,#160375,
#160376,#160377,#160378),(#160379,#160380,#160381,#160382,#160383,#160384,
#160385,#160386,#160387),(#160388,#160389,#160390,#160391,#160392,#160393,
#160394,#160395,#160396),(#160397,#160398,#160399,#160400,#160401,#160402,
#160403,#160404,#160405),(#160406,#160407,#160408,#160409,#160410,#160411,
#160412,#160413,#160414),(#160415,#160416,#160417,#160418,#160419,#160420,
#160421,#160422,#160423),(#160424,#160425,#160426,#160427,#160428,#160429,
#160430,#160431,#160432),(#160433,#160434,#160435,#160436,#160437,#160438,
#160439,#160440,#160441),(#160442,#160443,#160444,#160445,#160446,#160447,
#160448,#160449,#160450),(#160451,#160452,#160453,#160454,#160455,#160456,
#160457,#160458,#160459),(#160460,#160461,#160462,#160463,#160464,#160465,
#160466,#160467,#160468),(#160469,#160470,#160471,#160472,#160473,#160474,
#160475,#160476,#160477),(#160478,#160479,#160480,#160481,#160482,#160483,
#160484,#160485,#160486),(#160487,#160488,#160489,#160490,#160491,#160492,
#160493,#160494,#160495),(#160496,#160497,#160498,#160499,#160500,#160501,
#160502,#160503,#160504),(#160505,#160506,#160507,#160508,#160509,#160510,
#160511,#160512,#160513),(#160514,#160515,#160516,#160517,#160518,#160519,
#160520,#160521,#160522),(#160523,#160524,#160525,#160526,#160527,#160528,
#160529,#160530,#160531),(#160532,#160533,#160534,#160535,#160536,#160537,
#160538,#160539,#160540),(#160541,#160542,#160543,#160544,#160545,#160546,
#160547,#160548,#160549),(#160550,#160551,#160552,#160553,#160554,#160555,
#160556,#160557,#160558),(#160559,#160560,#160561,#160562,#160563,#160564,
#160565,#160566,#160567),(#160568,#160569,#160570,#160571,#160572,#160573,
#160574,#160575,#160576),(#160577,#160578,#160579,#160580,#160581,#160582,
#160583,#160584,#160585),(#160586,#160587,#160588,#160589,#160590,#160591,
#160592,#160593,#160594),(#160595,#160596,#160597,#160598,#160599,#160600,
#160601,#160602,#160603),(#160604,#160605,#160606,#160607,#160608,#160609,
#160610,#160611,#160612),(#160613,#160614,#160615,#160616,#160617,#160618,
#160619,#160620,#160621),(#160622,#160623,#160624,#160625,#160626,#160627,
#160628,#160629,#160630),(#160631,#160632,#160633,#160634,#160635,#160636,
#160637,#160638,#160639),(#160640,#160641,#160642,#160643,#160644,#160645,
#160646,#160647,#160648),(#160649,#160650,#160651,#160652,#160653,#160654,
#160655,#160656,#160657),(#160658,#160659,#160660,#160661,#160662,#160663,
#160664,#160665,#160666),(#160667,#160668,#160669,#160670,#160671,#160672,
#160673,#160674,#160675),(#160676,#160677,#160678,#160679,#160680,#160681,
#160682,#160683,#160684),(#160685,#160686,#160687,#160688,#160689,#160690,
#160691,#160692,#160693),(#160694,#160695,#160696,#160697,#160698,#160699,
#160700,#160701,#160702),(#160703,#160704,#160705,#160706,#160707,#160708,
#160709,#160710,#160711),(#160712,#160713,#160714,#160715,#160716,#160717,
#160718,#160719,#160720),(#160721,#160722,#160723,#160724,#160725,#160726,
#160727,#160728,#160729),(#160730,#160731,#160732,#160733,#160734,#160735,
#160736,#160737,#160738),(#160739,#160740,#160741,#160742,#160743,#160744,
#160745,#160746,#160747),(#160748,#160749,#160750,#160751,#160752,#160753,
#160754,#160755,#160756),(#160757,#160758,#160759,#160760,#160761,#160762,
#160763,#160764,#160765),(#160766,#160767,#160768,#160769,#160770,#160771,
#160772,#160773,#160774),(#160775,#160776,#160777,#160778,#160779,#160780,
#160781,#160782,#160783),(#160784,#160785,#160786,#160787,#160788,#160789,
#160790,#160791,#160792),(#160793,#160794,#160795,#160796,#160797,#160798,
#160799,#160800,#160801),(#160802,#160803,#160804,#160805,#160806,#160807,
#160808,#160809,#160810),(#160811,#160812,#160813,#160814,#160815,#160816,
#160817,#160818,#160819),(#160820,#160821,#160822,#160823,#160824,#160825,
#160826,#160827,#160828),(#160829,#160830,#160831,#160832,#160833,#160834,
#160835,#160836,#160837),(#160838,#160839,#160840,#160841,#160842,#160843,
#160844,#160845,#160846),(#160847,#160848,#160849,#160850,#160851,#160852,
#160853,#160854,#160855),(#160856,#160857,#160858,#160859,#160860,#160861,
#160862,#160863,#160864),(#160865,#160866,#160867,#160868,#160869,#160870,
#160871,#160872,#160873),(#160874,#160875,#160876,#160877,#160878,#160879,
#160880,#160881,#160882),(#160883,#160884,#160885,#160886,#160887,#160888,
#160889,#160890,#160891),(#160892,#160893,#160894,#160895,#160896,#160897,
#160898,#160899,#160900),(#160901,#160902,#160903,#160904,#160905,#160906,
#160907,#160908,#160909),(#160910,#160911,#160912,#160913,#160914,#160915,
#160916,#160917,#160918),(#160919,#160920,#160921,#160922,#160923,#160924,
#160925,#160926,#160927),(#160928,#160929,#160930,#160931,#160932,#160933,
#160934,#160935,#160936),(#160937,#160938,#160939,#160940,#160941,#160942,
#160943,#160944,#160945),(#160946,#160947,#160948,#160949,#160950,#160951,
#160952,#160953,#160954),(#160955,#160956,#160957,#160958,#160959,#160960,
#160961,#160962,#160963),(#160964,#160965,#160966,#160967,#160968,#160969,
#160970,#160971,#160972),(#160973,#160974,#160975,#160976,#160977,#160978,
#160979,#160980,#160981),(#160982,#160983,#160984,#160985,#160986,#160987,
#160988,#160989,#160990),(#160991,#160992,#160993,#160994,#160995,#160996,
#160997,#160998,#160999),(#161000,#161001,#161002,#161003,#161004,#161005,
#161006,#161007,#161008),(#161009,#161010,#161011,#161012,#161013,#161014,
#161015,#161016,#161017),(#161018,#161019,#161020,#161021,#161022,#161023,
#161024,#161025,#161026),(#161027,#161028,#161029,#161030,#161031,#161032,
#161033,#161034,#161035),(#161036,#161037,#161038,#161039,#161040,#161041,
#161042,#161043,#161044),(#161045,#161046,#161047,#161048,#161049,#161050,
#161051,#161052,#161053),(#161054,#161055,#161056,#161057,#161058,#161059,
#161060,#161061,#161062),(#161063,#161064,#161065,#161066,#161067,#161068,
#161069,#161070,#161071),(#161072,#161073,#161074,#161075,#161076,#161077,
#161078,#161079,#161080),(#161081,#161082,#161083,#161084,#161085,#161086,
#161087,#161088,#161089),(#161090,#161091,#161092,#161093,#161094,#161095,
#161096,#161097,#161098),(#161099,#161100,#161101,#161102,#161103,#161104,
#161105,#161106,#161107),(#161108,#161109,#161110,#161111,#161112,#161113,
#161114,#161115,#161116),(#161117,#161118,#161119,#161120,#161121,#161122,
#161123,#161124,#161125),(#161126,#161127,#161128,#161129,#161130,#161131,
#161132,#161133,#161134),(#161135,#161136,#161137,#161138,#161139,#161140,
#161141,#161142,#161143),(#161144,#161145,#161146,#161147,#161148,#161149,
#161150,#161151,#161152),(#161153,#161154,#161155,#161156,#161157,#161158,
#161159,#161160,#161161),(#161162,#161163,#161164,#161165,#161166,#161167,
#161168,#161169,#161170),(#161171,#161172,#161173,#161174,#161175,#161176,
#161177,#161178,#161179),(#161180,#161181,#161182,#161183,#161184,#161185,
#161186,#161187,#161188),(#161189,#161190,#161191,#161192,#161193,#161194,
#161195,#161196,#161197),(#161198,#161199,#161200,#161201,#161202,#161203,
#161204,#161205,#161206),(#161207,#161208,#161209,#161210,#161211,#161212,
#161213,#161214,#161215),(#161216,#161217,#161218,#161219,#161220,#161221,
#161222,#161223,#161224),(#161225,#161226,#161227,#161228,#161229,#161230,
#161231,#161232,#161233),(#161234,#161235,#161236,#161237,#161238,#161239,
#161240,#161241,#161242),(#161243,#161244,#161245,#161246,#161247,#161248,
#161249,#161250,#161251),(#161252,#161253,#161254,#161255,#161256,#161257,
#161258,#161259,#161260),(#161261,#161262,#161263,#161264,#161265,#161266,
#161267,#161268,#161269),(#161270,#161271,#161272,#161273,#161274,#161275,
#161276,#161277,#161278),(#161279,#161280,#161281,#161282,#161283,#161284,
#161285,#161286,#161287),(#161288,#161289,#161290,#161291,#161292,#161293,
#161294,#161295,#161296),(#161297,#161298,#161299,#161300,#161301,#161302,
#161303,#161304,#161305),(#161306,#161307,#161308,#161309,#161310,#161311,
#161312,#161313,#161314),(#161315,#161316,#161317,#161318,#161319,#161320,
#161321,#161322,#161323),(#161324,#161325,#161326,#161327,#161328,#161329,
#161330,#161331,#161332),(#161333,#161334,#161335,#161336,#161337,#161338,
#161339,#161340,#161341),(#161342,#161343,#161344,#161345,#161346,#161347,
#161348,#161349,#161350),(#161351,#161352,#161353,#161354,#161355,#161356,
#161357,#161358,#161359),(#161360,#161361,#161362,#161363,#161364,#161365,
#161366,#161367,#161368),(#161369,#161370,#161371,#161372,#161373,#161374,
#161375,#161376,#161377),(#161378,#161379,#161380,#161381,#161382,#161383,
#161384,#161385,#161386),(#161387,#161388,#161389,#161390,#161391,#161392,
#161393,#161394,#161395),(#161396,#161397,#161398,#161399,#161400,#161401,
#161402,#161403,#161404),(#161405,#161406,#161407,#161408,#161409,#161410,
#161411,#161412,#161413),(#161414,#161415,#161416,#161417,#161418,#161419,
#161420,#161421,#161422),(#161423,#161424,#161425,#161426,#161427,#161428,
#161429,#161430,#161431),(#161432,#161433,#161434,#161435,#161436,#161437,
#161438,#161439,#161440),(#161441,#161442,#161443,#161444,#161445,#161446,
#161447,#161448,#161449),(#161450,#161451,#161452,#161453,#161454,#161455,
#161456,#161457,#161458),(#161459,#161460,#161461,#161462,#161463,#161464,
#161465,#161466,#161467),(#161468,#161469,#161470,#161471,#161472,#161473,
#161474,#161475,#161476),(#161477,#161478,#161479,#161480,#161481,#161482,
#161483,#161484,#161485),(#161486,#161487,#161488,#161489,#161490,#161491,
#161492,#161493,#161494),(#161495,#161496,#161497,#161498,#161499,#161500,
#161501,#161502,#161503),(#161504,#161505,#161506,#161507,#161508,#161509,
#161510,#161511,#161512),(#161513,#161514,#161515,#161516,#161517,#161518,
#161519,#161520,#161521),(#161522,#161523,#161524,#161525,#161526,#161527,
#161528,#161529,#161530),(#161531,#161532,#161533,#161534,#161535,#161536,
#161537,#161538,#161539),(#161540,#161541,#161542,#161543,#161544,#161545,
#161546,#161547,#161548),(#161549,#161550,#161551,#161552,#161553,#161554,
#161555,#161556,#161557),(#161558,#161559,#161560,#161561,#161562,#161563,
#161564,#161565,#161566),(#161567,#161568,#161569,#161570,#161571,#161572,
#161573,#161574,#161575),(#161576,#161577,#161578,#161579,#161580,#161581,
#161582,#161583,#161584),(#161585,#161586,#161587,#161588,#161589,#161590,
#161591,#161592,#161593),(#161594,#161595,#161596,#161597,#161598,#161599,
#161600,#161601,#161602),(#161603,#161604,#161605,#161606,#161607,#161608,
#161609,#161610,#161611),(#161612,#161613,#161614,#161615,#161616,#161617,
#161618,#161619,#161620),(#161621,#161622,#161623,#161624,#161625,#161626,
#161627,#161628,#161629),(#161630,#161631,#161632,#161633,#161634,#161635,
#161636,#161637,#161638),(#161639,#161640,#161641,#161642,#161643,#161644,
#161645,#161646,#161647),(#161648,#161649,#161650,#161651,#161652,#161653,
#161654,#161655,#161656),(#161657,#161658,#161659,#161660,#161661,#161662,
#161663,#161664,#161665),(#161666,#161667,#161668,#161669,#161670,#161671,
#161672,#161673,#161674),(#161675,#161676,#161677,#161678,#161679,#161680,
#161681,#161682,#161683),(#161684,#161685,#161686,#161687,#161688,#161689,
#161690,#161691,#161692),(#161693,#161694,#161695,#161696,#161697,#161698,
#161699,#161700,#161701),(#161702,#161703,#161704,#161705,#161706,#161707,
#161708,#161709,#161710),(#161711,#161712,#161713,#161714,#161715,#161716,
#161717,#161718,#161719),(#161720,#161721,#161722,#161723,#161724,#161725,
#161726,#161727,#161728),(#161729,#161730,#161731,#161732,#161733,#161734,
#161735,#161736,#161737),(#161738,#161739,#161740,#161741,#161742,#161743,
#161744,#161745,#161746),(#161747,#161748,#161749,#161750,#161751,#161752,
#161753,#161754,#161755),(#161756,#161757,#161758,#161759,#161760,#161761,
#161762,#161763,#161764),(#161765,#161766,#161767,#161768,#161769,#161770,
#161771,#161772,#161773),(#161774,#161775,#161776,#161777,#161778,#161779,
#161780,#161781,#161782),(#161783,#161784,#161785,#161786,#161787,#161788,
#161789,#161790,#161791),(#161792,#161793,#161794,#161795,#161796,#161797,
#161798,#161799,#161800),(#161801,#161802,#161803,#161804,#161805,#161806,
#161807,#161808,#161809),(#161810,#161811,#161812,#161813,#161814,#161815,
#161816,#161817,#161818),(#161819,#161820,#161821,#161822,#161823,#161824,
#161825,#161826,#161827),(#161828,#161829,#161830,#161831,#161832,#161833,
#161834,#161835,#161836),(#161837,#161838,#161839,#161840,#161841,#161842,
#161843,#161844,#161845),(#161846,#161847,#161848,#161849,#161850,#161851,
#161852,#161853,#161854),(#161855,#161856,#161857,#161858,#161859,#161860,
#161861,#161862,#161863),(#161864,#161865,#161866,#161867,#161868,#161869,
#161870,#161871,#161872),(#161873,#161874,#161875,#161876,#161877,#161878,
#161879,#161880,#161881),(#161882,#161883,#161884,#161885,#161886,#161887,
#161888,#161889,#161890),(#161891,#161892,#161893,#161894,#161895,#161896,
#161897,#161898,#161899),(#161900,#161901,#161902,#161903,#161904,#161905,
#161906,#161907,#161908),(#161909,#161910,#161911,#161912,#161913,#161914,
#161915,#161916,#161917),(#161918,#161919,#161920,#161921,#161922,#161923,
#161924,#161925,#161926),(#161927,#161928,#161929,#161930,#161931,#161932,
#161933,#161934,#161935),(#161936,#161937,#161938,#161939,#161940,#161941,
#161942,#161943,#161944),(#161945,#161946,#161947,#161948,#161949,#161950,
#161951,#161952,#161953),(#161954,#161955,#161956,#161957,#161958,#161959,
#161960,#161961,#161962),(#161963,#161964,#161965,#161966,#161967,#161968,
#161969,#161970,#161971),(#161972,#161973,#161974,#161975,#161976,#161977,
#161978,#161979,#161980),(#161981,#161982,#161983,#161984,#161985,#161986,
#161987,#161988,#161989),(#161990,#161991,#161992,#161993,#161994,#161995,
#161996,#161997,#161998),(#161999,#162000,#162001,#162002,#162003,#162004,
#162005,#162006,#162007),(#162008,#162009,#162010,#162011,#162012,#162013,
#162014,#162015,#162016),(#162017,#162018,#162019,#162020,#162021,#162022,
#162023,#162024,#162025),(#162026,#162027,#162028,#162029,#162030,#162031,
#162032,#162033,#162034),(#162035,#162036,#162037,#162038,#162039,#162040,
#162041,#162042,#162043),(#162044,#162045,#162046,#162047,#162048,#162049,
#162050,#162051,#162052),(#162053,#162054,#162055,#162056,#162057,#162058,
#162059,#162060,#162061),(#162062,#162063,#162064,#162065,#162066,#162067,
#162068,#162069,#162070),(#162071,#162072,#162073,#162074,#162075,#162076,
#162077,#162078,#162079),(#162080,#162081,#162082,#162083,#162084,#162085,
#162086,#162087,#162088),(#162089,#162090,#162091,#162092,#162093,#162094,
#162095,#162096,#162097),(#162098,#162099,#162100,#162101,#162102,#162103,
#162104,#162105,#162106),(#162107,#162108,#162109,#162110,#162111,#162112,
#162113,#162114,#162115),(#162116,#162117,#162118,#162119,#162120,#162121,
#162122,#162123,#162124),(#162125,#162126,#162127,#162128,#162129,#162130,
#162131,#162132,#162133),(#162134,#162135,#162136,#162137,#162138,#162139,
#162140,#162141,#162142),(#162143,#162144,#162145,#162146,#162147,#162148,
#162149,#162150,#162151),(#162152,#162153,#162154,#162155,#162156,#162157,
#162158,#162159,#162160),(#162161,#162162,#162163,#162164,#162165,#162166,
#162167,#162168,#162169),(#162170,#162171,#162172,#162173,#162174,#162175,
#162176,#162177,#162178),(#162179,#162180,#162181,#162182,#162183,#162184,
#162185,#162186,#162187),(#162188,#162189,#162190,#162191,#162192,#162193,
#162194,#162195,#162196),(#162197,#162198,#162199,#162200,#162201,#162202,
#162203,#162204,#162205),(#162206,#162207,#162208,#162209,#162210,#162211,
#162212,#162213,#162214),(#162215,#162216,#162217,#162218,#162219,#162220,
#162221,#162222,#162223),(#162224,#162225,#162226,#162227,#162228,#162229,
#162230,#162231,#162232),(#162233,#162234,#162235,#162236,#162237,#162238,
#162239,#162240,#162241),(#162242,#162243,#162244,#162245,#162246,#162247,
#162248,#162249,#162250),(#162251,#162252,#162253,#162254,#162255,#162256,
#162257,#162258,#162259),(#162260,#162261,#162262,#162263,#162264,#162265,
#162266,#162267,#162268),(#162269,#162270,#162271,#162272,#162273,#162274,
#162275,#162276,#162277),(#162278,#162279,#162280,#162281,#162282,#162283,
#162284,#162285,#162286),(#162287,#162288,#162289,#162290,#162291,#162292,
#162293,#162294,#162295),(#162296,#162297,#162298,#162299,#162300,#162301,
#162302,#162303,#162304),(#162305,#162306,#162307,#162308,#162309,#162310,
#162311,#162312,#162313),(#162314,#162315,#162316,#162317,#162318,#162319,
#162320,#162321,#162322),(#162323,#162324,#162325,#162326,#162327,#162328,
#162329,#162330,#162331),(#162332,#162333,#162334,#162335,#162336,#162337,
#162338,#162339,#162340),(#162341,#162342,#162343,#162344,#162345,#162346,
#162347,#162348,#162349),(#162350,#162351,#162352,#162353,#162354,#162355,
#162356,#162357,#162358),(#162359,#162360,#162361,#162362,#162363,#162364,
#162365,#162366,#162367),(#162368,#162369,#162370,#162371,#162372,#162373,
#162374,#162375,#162376),(#162377,#162378,#162379,#162380,#162381,#162382,
#162383,#162384,#162385),(#162386,#162387,#162388,#162389,#162390,#162391,
#162392,#162393,#162394),(#162395,#162396,#162397,#162398,#162399,#162400,
#162401,#162402,#162403),(#162404,#162405,#162406,#162407,#162408,#162409,
#162410,#162411,#162412),(#162413,#162414,#162415,#162416,#162417,#162418,
#162419,#162420,#162421),(#162422,#162423,#162424,#162425,#162426,#162427,
#162428,#162429,#162430),(#162431,#162432,#162433,#162434,#162435,#162436,
#162437,#162438,#162439),(#162440,#162441,#162442,#162443,#162444,#162445,
#162446,#162447,#162448),(#162449,#162450,#162451,#162452,#162453,#162454,
#162455,#162456,#162457),(#162458,#162459,#162460,#162461,#162462,#162463,
#162464,#162465,#162466),(#162467,#162468,#162469,#162470,#162471,#162472,
#162473,#162474,#162475),(#162476,#162477,#162478,#162479,#162480,#162481,
#162482,#162483,#162484),(#162485,#162486,#162487,#162488,#162489,#162490,
#162491,#162492,#162493),(#162494,#162495,#162496,#162497,#162498,#162499,
#162500,#162501,#162502),(#162503,#162504,#162505,#162506,#162507,#162508,
#162509,#162510,#162511),(#162512,#162513,#162514,#162515,#162516,#162517,
#162518,#162519,#162520),(#162521,#162522,#162523,#162524,#162525,#162526,
#162527,#162528,#162529),(#162530,#162531,#162532,#162533,#162534,#162535,
#162536,#162537,#162538),(#162539,#162540,#162541,#162542,#162543,#162544,
#162545,#162546,#162547),(#162548,#162549,#162550,#162551,#162552,#162553,
#162554,#162555,#162556),(#162557,#162558,#162559,#162560,#162561,#162562,
#162563,#162564,#162565),(#162566,#162567,#162568,#162569,#162570,#162571,
#162572,#162573,#162574),(#162575,#162576,#162577,#162578,#162579,#162580,
#162581,#162582,#162583),(#162584,#162585,#162586,#162587,#162588,#162589,
#162590,#162591,#162592),(#162593,#162594,#162595,#162596,#162597,#162598,
#162599,#162600,#162601),(#162602,#162603,#162604,#162605,#162606,#162607,
#162608,#162609,#162610),(#162611,#162612,#162613,#162614,#162615,#162616,
#162617,#162618,#162619),(#162620,#162621,#162622,#162623,#162624,#162625,
#162626,#162627,#162628),(#162629,#162630,#162631,#162632,#162633,#162634,
#162635,#162636,#162637),(#162638,#162639,#162640,#162641,#162642,#162643,
#162644,#162645,#162646),(#162647,#162648,#162649,#162650,#162651,#162652,
#162653,#162654,#162655),(#162656,#162657,#162658,#162659,#162660,#162661,
#162662,#162663,#162664),(#162665,#162666,#162667,#162668,#162669,#162670,
#162671,#162672,#162673),(#162674,#162675,#162676,#162677,#162678,#162679,
#162680,#162681,#162682),(#162683,#162684,#162685,#162686,#162687,#162688,
#162689,#162690,#162691),(#162692,#162693,#162694,#162695,#162696,#162697,
#162698,#162699,#162700),(#162701,#162702,#162703,#162704,#162705,#162706,
#162707,#162708,#162709),(#162710,#162711,#162712,#162713,#162714,#162715,
#162716,#162717,#162718),(#162719,#162720,#162721,#162722,#162723,#162724,
#162725,#162726,#162727),(#162728,#162729,#162730,#162731,#162732,#162733,
#162734,#162735,#162736),(#162737,#162738,#162739,#162740,#162741,#162742,
#162743,#162744,#162745),(#162746,#162747,#162748,#162749,#162750,#162751,
#162752,#162753,#162754),(#162755,#162756,#162757,#162758,#162759,#162760,
#162761,#162762,#162763),(#162764,#162765,#162766,#162767,#162768,#162769,
#162770,#162771,#162772),(#162773,#162774,#162775,#162776,#162777,#162778,
#162779,#162780,#162781),(#162782,#162783,#162784,#162785,#162786,#162787,
#162788,#162789,#162790),(#162791,#162792,#162793,#162794,#162795,#162796,
#162797,#162798,#162799),(#162800,#162801,#162802,#162803,#162804,#162805,
#162806,#162807,#162808),(#162809,#162810,#162811,#162812,#162813,#162814,
#162815,#162816,#162817),(#162818,#162819,#162820,#162821,#162822,#162823,
#162824,#162825,#162826),(#162827,#162828,#162829,#162830,#162831,#162832,
#162833,#162834,#162835),(#162836,#162837,#162838,#162839,#162840,#162841,
#162842,#162843,#162844),(#162845,#162846,#162847,#162848,#162849,#162850,
#162851,#162852,#162853),(#162854,#162855,#162856,#162857,#162858,#162859,
#162860,#162861,#162862),(#162863,#162864,#162865,#162866,#162867,#162868,
#162869,#162870,#162871),(#162872,#162873,#162874,#162875,#162876,#162877,
#162878,#162879,#162880),(#162881,#162882,#162883,#162884,#162885,#162886,
#162887,#162888,#162889),(#162890,#162891,#162892,#162893,#162894,#162895,
#162896,#162897,#162898),(#162899,#162900,#162901,#162902,#162903,#162904,
#162905,#162906,#162907),(#162908,#162909,#162910,#162911,#162912,#162913,
#162914,#162915,#162916),(#162917,#162918,#162919,#162920,#162921,#162922,
#162923,#162924,#162925),(#162926,#162927,#162928,#162929,#162930,#162931,
#162932,#162933,#162934),(#162935,#162936,#162937,#162938,#162939,#162940,
#162941,#162942,#162943),(#162944,#162945,#162946,#162947,#162948,#162949,
#162950,#162951,#162952),(#162953,#162954,#162955,#162956,#162957,#162958,
#162959,#162960,#162961),(#162962,#162963,#162964,#162965,#162966,#162967,
#162968,#162969,#162970),(#162971,#162972,#162973,#162974,#162975,#162976,
#162977,#162978,#162979),(#162980,#162981,#162982,#162983,#162984,#162985,
#162986,#162987,#162988),(#162989,#162990,#162991,#162992,#162993,#162994,
#162995,#162996,#162997),(#162998,#162999,#163000,#163001,#163002,#163003,
#163004,#163005,#163006),(#163007,#163008,#163009,#163010,#163011,#163012,
#163013,#163014,#163015),(#163016,#163017,#163018,#163019,#163020,#163021,
#163022,#163023,#163024),(#163025,#163026,#163027,#163028,#163029,#163030,
#163031,#163032,#163033),(#163034,#163035,#163036,#163037,#163038,#163039,
#163040,#163041,#163042),(#163043,#163044,#163045,#163046,#163047,#163048,
#163049,#163050,#163051),(#163052,#163053,#163054,#163055,#163056,#163057,
#163058,#163059,#163060),(#163061,#163062,#163063,#163064,#163065,#163066,
#163067,#163068,#163069),(#163070,#163071,#163072,#163073,#163074,#163075,
#163076,#163077,#163078),(#163079,#163080,#163081,#163082,#163083,#163084,
#163085,#163086,#163087),(#163088,#163089,#163090,#163091,#163092,#163093,
#163094,#163095,#163096),(#163097,#163098,#163099,#163100,#163101,#163102,
#163103,#163104,#163105),(#163106,#163107,#163108,#163109,#163110,#163111,
#163112,#163113,#163114),(#163115,#163116,#163117,#163118,#163119,#163120,
#163121,#163122,#163123),(#163124,#163125,#163126,#163127,#163128,#163129,
#163130,#163131,#163132),(#163133,#163134,#163135,#163136,#163137,#163138,
#163139,#163140,#163141),(#163142,#163143,#163144,#163145,#163146,#163147,
#163148,#163149,#163150),(#163151,#163152,#163153,#163154,#163155,#163156,
#163157,#163158,#163159),(#163160,#163161,#163162,#163163,#163164,#163165,
#163166,#163167,#163168),(#163169,#163170,#163171,#163172,#163173,#163174,
#163175,#163176,#163177),(#163178,#163179,#163180,#163181,#163182,#163183,
#163184,#163185,#163186),(#163187,#163188,#163189,#163190,#163191,#163192,
#163193,#163194,#163195),(#163196,#163197,#163198,#163199,#163200,#163201,
#163202,#163203,#163204),(#163205,#163206,#163207,#163208,#163209,#163210,
#163211,#163212,#163213),(#163214,#163215,#163216,#163217,#163218,#163219,
#163220,#163221,#163222),(#163223,#163224,#163225,#163226,#163227,#163228,
#163229,#163230,#163231),(#163232,#163233,#163234,#163235,#163236,#163237,
#163238,#163239,#163240),(#163241,#163242,#163243,#163244,#163245,#163246,
#163247,#163248,#163249),(#163250,#163251,#163252,#163253,#163254,#163255,
#163256,#163257,#163258),(#163259,#163260,#163261,#163262,#163263,#163264,
#163265,#163266,#163267),(#163268,#163269,#163270,#163271,#163272,#163273,
#163274,#163275,#163276),(#163277,#163278,#163279,#163280,#163281,#163282,
#163283,#163284,#163285),(#163286,#163287,#163288,#163289,#163290,#163291,
#163292,#163293,#163294),(#163295,#163296,#163297,#163298,#163299,#163300,
#163301,#163302,#163303),(#163304,#163305,#163306,#163307,#163308,#163309,
#163310,#163311,#163312),(#163313,#163314,#163315,#163316,#163317,#163318,
#163319,#163320,#163321),(#163322,#163323,#163324,#163325,#163326,#163327,
#163328,#163329,#163330),(#163331,#163332,#163333,#163334,#163335,#163336,
#163337,#163338,#163339),(#163340,#163341,#163342,#163343,#163344,#163345,
#163346,#163347,#163348),(#163349,#163350,#163351,#163352,#163353,#163354,
#163355,#163356,#163357),(#163358,#163359,#163360,#163361,#163362,#163363,
#163364,#163365,#163366),(#163367,#163368,#163369,#163370,#163371,#163372,
#163373,#163374,#163375),(#163376,#163377,#163378,#163379,#163380,#163381,
#163382,#163383,#163384),(#163385,#163386,#163387,#163388,#163389,#163390,
#163391,#163392,#163393),(#163394,#163395,#163396,#163397,#163398,#163399,
#163400,#163401,#163402),(#163403,#163404,#163405,#163406,#163407,#163408,
#163409,#163410,#163411),(#163412,#163413,#163414,#163415,#163416,#163417,
#163418,#163419,#163420),(#163421,#163422,#163423,#163424,#163425,#163426,
#163427,#163428,#163429),(#163430,#163431,#163432,#163433,#163434,#163435,
#163436,#163437,#163438),(#163439,#163440,#163441,#163442,#163443,#163444,
#163445,#163446,#163447),(#163448,#163449,#163450,#163451,#163452,#163453,
#163454,#163455,#163456),(#163457,#163458,#163459,#163460,#163461,#163462,
#163463,#163464,#163465),(#163466,#163467,#163468,#163469,#163470,#163471,
#163472,#163473,#163474),(#163475,#163476,#163477,#163478,#163479,#163480,
#163481,#163482,#163483),(#163484,#163485,#163486,#163487,#163488,#163489,
#163490,#163491,#163492),(#163493,#163494,#163495,#163496,#163497,#163498,
#163499,#163500,#163501),(#163502,#163503,#163504,#163505,#163506,#163507,
#163508,#163509,#163510),(#163511,#163512,#163513,#163514,#163515,#163516,
#163517,#163518,#163519),(#163520,#163521,#163522,#163523,#163524,#163525,
#163526,#163527,#163528),(#163529,#163530,#163531,#163532,#163533,#163534,
#163535,#163536,#163537),(#163538,#163539,#163540,#163541,#163542,#163543,
#163544,#163545,#163546),(#163547,#163548,#163549,#163550,#163551,#163552,
#163553,#163554,#163555),(#163556,#163557,#163558,#163559,#163560,#163561,
#163562,#163563,#163564),(#163565,#163566,#163567,#163568,#163569,#163570,
#163571,#163572,#163573),(#163574,#163575,#163576,#163577,#163578,#163579,
#163580,#163581,#163582),(#163583,#163584,#163585,#163586,#163587,#163588,
#163589,#163590,#163591),(#163592,#163593,#163594,#163595,#163596,#163597,
#163598,#163599,#163600),(#163601,#163602,#163603,#163604,#163605,#163606,
#163607,#163608,#163609),(#163610,#163611,#163612,#163613,#163614,#163615,
#163616,#163617,#163618),(#163619,#163620,#163621,#163622,#163623,#163624,
#163625,#163626,#163627),(#163628,#163629,#163630,#163631,#163632,#163633,
#163634,#163635,#163636),(#163637,#163638,#163639,#163640,#163641,#163642,
#163643,#163644,#163645),(#163646,#163647,#163648,#163649,#163650,#163651,
#163652,#163653,#163654),(#163655,#163656,#163657,#163658,#163659,#163660,
#163661,#163662,#163663),(#163664,#163665,#163666,#163667,#163668,#163669,
#163670,#163671,#163672),(#163673,#163674,#163675,#163676,#163677,#163678,
#163679,#163680,#163681),(#163682,#163683,#163684,#163685,#163686,#163687,
#163688,#163689,#163690),(#163691,#163692,#163693,#163694,#163695,#163696,
#163697,#163698,#163699),(#163700,#163701,#163702,#163703,#163704,#163705,
#163706,#163707,#163708),(#163709,#163710,#163711,#163712,#163713,#163714,
#163715,#163716,#163717),(#163718,#163719,#163720,#163721,#163722,#163723,
#163724,#163725,#163726),(#163727,#163728,#163729,#163730,#163731,#163732,
#163733,#163734,#163735),(#163736,#163737,#163738,#163739,#163740,#163741,
#163742,#163743,#163744),(#163745,#163746,#163747,#163748,#163749,#163750,
#163751,#163752,#163753),(#163754,#163755,#163756,#163757,#163758,#163759,
#163760,#163761,#163762),(#163763,#163764,#163765,#163766,#163767,#163768,
#163769,#163770,#163771),(#163772,#163773,#163774,#163775,#163776,#163777,
#163778,#163779,#163780),(#163781,#163782,#163783,#163784,#163785,#163786,
#163787,#163788,#163789),(#163790,#163791,#163792,#163793,#163794,#163795,
#163796,#163797,#163798),(#163799,#163800,#163801,#163802,#163803,#163804,
#163805,#163806,#163807),(#163808,#163809,#163810,#163811,#163812,#163813,
#163814,#163815,#163816),(#163817,#163818,#163819,#163820,#163821,#163822,
#163823,#163824,#163825),(#163826,#163827,#163828,#163829,#163830,#163831,
#163832,#163833,#163834),(#163835,#163836,#163837,#163838,#163839,#163840,
#163841,#163842,#163843),(#163844,#163845,#163846,#163847,#163848,#163849,
#163850,#163851,#163852),(#163853,#163854,#163855,#163856,#163857,#163858,
#163859,#163860,#163861),(#163862,#163863,#163864,#163865,#163866,#163867,
#163868,#163869,#163870),(#163871,#163872,#163873,#163874,#163875,#163876,
#163877,#163878,#163879),(#163880,#163881,#163882,#163883,#163884,#163885,
#163886,#163887,#163888),(#163889,#163890,#163891,#163892,#163893,#163894,
#163895,#163896,#163897),(#163898,#163899,#163900,#163901,#163902,#163903,
#163904,#163905,#163906),(#163907,#163908,#163909,#163910,#163911,#163912,
#163913,#163914,#163915),(#163916,#163917,#163918,#163919,#163920,#163921,
#163922,#163923,#163924),(#163925,#163926,#163927,#163928,#163929,#163930,
#163931,#163932,#163933),(#163934,#163935,#163936,#163937,#163938,#163939,
#163940,#163941,#163942),(#163943,#163944,#163945,#163946,#163947,#163948,
#163949,#163950,#163951),(#163952,#163953,#163954,#163955,#163956,#163957,
#163958,#163959,#163960),(#163961,#163962,#163963,#163964,#163965,#163966,
#163967,#163968,#163969),(#163970,#163971,#163972,#163973,#163974,#163975,
#163976,#163977,#163978),(#163979,#163980,#163981,#163982,#163983,#163984,
#163985,#163986,#163987),(#163988,#163989,#163990,#163991,#163992,#163993,
#163994,#163995,#163996),(#163997,#163998,#163999,#164000,#164001,#164002,
#164003,#164004,#164005),(#164006,#164007,#164008,#164009,#164010,#164011,
#164012,#164013,#164014),(#164015,#164016,#164017,#164018,#164019,#164020,
#164021,#164022,#164023),(#164024,#164025,#164026,#164027,#164028,#164029,
#164030,#164031,#164032),(#164033,#164034,#164035,#164036,#164037,#164038,
#164039,#164040,#164041),(#164042,#164043,#164044,#164045,#164046,#164047,
#164048,#164049,#164050),(#164051,#164052,#164053,#164054,#164055,#164056,
#164057,#164058,#164059),(#164060,#164061,#164062,#164063,#164064,#164065,
#164066,#164067,#164068),(#164069,#164070,#164071,#164072,#164073,#164074,
#164075,#164076,#164077),(#164078,#164079,#164080,#164081,#164082,#164083,
#164084,#164085,#164086),(#164087,#164088,#164089,#164090,#164091,#164092,
#164093,#164094,#164095),(#164096,#164097,#164098,#164099,#164100,#164101,
#164102,#164103,#164104),(#164105,#164106,#164107,#164108,#164109,#164110,
#164111,#164112,#164113),(#164114,#164115,#164116,#164117,#164118,#164119,
#164120,#164121,#164122),(#164123,#164124,#164125,#164126,#164127,#164128,
#164129,#164130,#164131),(#164132,#164133,#164134,#164135,#164136,#164137,
#164138,#164139,#164140),(#164141,#164142,#164143,#164144,#164145,#164146,
#164147,#164148,#164149),(#164150,#164151,#164152,#164153,#164154,#164155,
#164156,#164157,#164158),(#164159,#164160,#164161,#164162,#164163,#164164,
#164165,#164166,#164167),(#164168,#164169,#164170,#164171,#164172,#164173,
#164174,#164175,#164176),(#164177,#164178,#164179,#164180,#164181,#164182,
#164183,#164184,#164185),(#164186,#164187,#164188,#164189,#164190,#164191,
#164192,#164193,#164194),(#164195,#164196,#164197,#164198,#164199,#164200,
#164201,#164202,#164203),(#164204,#164205,#164206,#164207,#164208,#164209,
#164210,#164211,#164212),(#164213,#164214,#164215,#164216,#164217,#164218,
#164219,#164220,#164221),(#164222,#164223,#164224,#164225,#164226,#164227,
#164228,#164229,#164230),(#164231,#164232,#164233,#164234,#164235,#164236,
#164237,#164238,#164239),(#164240,#164241,#164242,#164243,#164244,#164245,
#164246,#164247,#164248),(#164249,#164250,#164251,#164252,#164253,#164254,
#164255,#164256,#164257),(#164258,#164259,#164260,#164261,#164262,#164263,
#164264,#164265,#164266),(#164267,#164268,#164269,#164270,#164271,#164272,
#164273,#164274,#164275),(#164276,#164277,#164278,#164279,#164280,#164281,
#164282,#164283,#164284),(#164285,#164286,#164287,#164288,#164289,#164290,
#164291,#164292,#164293),(#164294,#164295,#164296,#164297,#164298,#164299,
#164300,#164301,#164302),(#164303,#164304,#164305,#164306,#164307,#164308,
#164309,#164310,#164311),(#164312,#164313,#164314,#164315,#164316,#164317,
#164318,#164319,#164320),(#164321,#164322,#164323,#164324,#164325,#164326,
#164327,#164328,#164329),(#164330,#164331,#164332,#164333,#164334,#164335,
#164336,#164337,#164338),(#164339,#164340,#164341,#164342,#164343,#164344,
#164345,#164346,#164347),(#164348,#164349,#164350,#164351,#164352,#164353,
#164354,#164355,#164356),(#164357,#164358,#164359,#164360,#164361,#164362,
#164363,#164364,#164365),(#164366,#164367,#164368,#164369,#164370,#164371,
#164372,#164373,#164374),(#164375,#164376,#164377,#164378,#164379,#164380,
#164381,#164382,#164383),(#164384,#164385,#164386,#164387,#164388,#164389,
#164390,#164391,#164392),(#164393,#164394,#164395,#164396,#164397,#164398,
#164399,#164400,#164401),(#164402,#164403,#164404,#164405,#164406,#164407,
#164408,#164409,#164410),(#164411,#164412,#164413,#164414,#164415,#164416,
#164417,#164418,#164419),(#164420,#164421,#164422,#164423,#164424,#164425,
#164426,#164427,#164428),(#164429,#164430,#164431,#164432,#164433,#164434,
#164435,#164436,#164437),(#164438,#164439,#164440,#164441,#164442,#164443,
#164444,#164445,#164446),(#164447,#164448,#164449,#164450,#164451,#164452,
#164453,#164454,#164455),(#164456,#164457,#164458,#164459,#164460,#164461,
#164462,#164463,#164464),(#164465,#164466,#164467,#164468,#164469,#164470,
#164471,#164472,#164473),(#164474,#164475,#164476,#164477,#164478,#164479,
#164480,#164481,#164482),(#164483,#164484,#164485,#164486,#164487,#164488,
#164489,#164490,#164491),(#164492,#164493,#164494,#164495,#164496,#164497,
#164498,#164499,#164500),(#164501,#164502,#164503,#164504,#164505,#164506,
#164507,#164508,#164509),(#164510,#164511,#164512,#164513,#164514,#164515,
#164516,#164517,#164518),(#164519,#164520,#164521,#164522,#164523,#164524,
#164525,#164526,#164527),(#164528,#164529,#164530,#164531,#164532,#164533,
#164534,#164535,#164536),(#164537,#164538,#164539,#164540,#164541,#164542,
#164543,#164544,#164545),(#164546,#164547,#164548,#164549,#164550,#164551,
#164552,#164553,#164554),(#164555,#164556,#164557,#164558,#164559,#164560,
#164561,#164562,#164563),(#164564,#164565,#164566,#164567,#164568,#164569,
#164570,#164571,#164572),(#164573,#164574,#164575,#164576,#164577,#164578,
#164579,#164580,#164581),(#164582,#164583,#164584,#164585,#164586,#164587,
#164588,#164589,#164590),(#164591,#164592,#164593,#164594,#164595,#164596,
#164597,#164598,#164599),(#164600,#164601,#164602,#164603,#164604,#164605,
#164606,#164607,#164608),(#164609,#164610,#164611,#164612,#164613,#164614,
#164615,#164616,#164617),(#164618,#164619,#164620,#164621,#164622,#164623,
#164624,#164625,#164626),(#164627,#164628,#164629,#164630,#164631,#164632,
#164633,#164634,#164635),(#164636,#164637,#164638,#164639,#164640,#164641,
#164642,#164643,#164644),(#164645,#164646,#164647,#164648,#164649,#164650,
#164651,#164652,#164653),(#164654,#164655,#164656,#164657,#164658,#164659,
#164660,#164661,#164662),(#164663,#164664,#164665,#164666,#164667,#164668,
#164669,#164670,#164671),(#164672,#164673,#164674,#164675,#164676,#164677,
#164678,#164679,#164680),(#164681,#164682,#164683,#164684,#164685,#164686,
#164687,#164688,#164689),(#164690,#164691,#164692,#164693,#164694,#164695,
#164696,#164697,#164698),(#164699,#164700,#164701,#164702,#164703,#164704,
#164705,#164706,#164707),(#164708,#164709,#164710,#164711,#164712,#164713,
#164714,#164715,#164716),(#164717,#164718,#164719,#164720,#164721,#164722,
#164723,#164724,#164725),(#164726,#164727,#164728,#164729,#164730,#164731,
#164732,#164733,#164734),(#164735,#164736,#164737,#164738,#164739,#164740,
#164741,#164742,#164743),(#164744,#164745,#164746,#164747,#164748,#164749,
#164750,#164751,#164752),(#164753,#164754,#164755,#164756,#164757,#164758,
#164759,#164760,#164761),(#164762,#164763,#164764,#164765,#164766,#164767,
#164768,#164769,#164770),(#164771,#164772,#164773,#164774,#164775,#164776,
#164777,#164778,#164779),(#164780,#164781,#164782,#164783,#164784,#164785,
#164786,#164787,#164788),(#164789,#164790,#164791,#164792,#164793,#164794,
#164795,#164796,#164797),(#164798,#164799,#164800,#164801,#164802,#164803,
#164804,#164805,#164806),(#164807,#164808,#164809,#164810,#164811,#164812,
#164813,#164814,#164815),(#164816,#164817,#164818,#164819,#164820,#164821,
#164822,#164823,#164824),(#164825,#164826,#164827,#164828,#164829,#164830,
#164831,#164832,#164833),(#164834,#164835,#164836,#164837,#164838,#164839,
#164840,#164841,#164842),(#164843,#164844,#164845,#164846,#164847,#164848,
#164849,#164850,#164851),(#164852,#164853,#164854,#164855,#164856,#164857,
#164858,#164859,#164860),(#164861,#164862,#164863,#164864,#164865,#164866,
#164867,#164868,#164869),(#164870,#164871,#164872,#164873,#164874,#164875,
#164876,#164877,#164878),(#164879,#164880,#164881,#164882,#164883,#164884,
#164885,#164886,#164887),(#164888,#164889,#164890,#164891,#164892,#164893,
#164894,#164895,#164896),(#164897,#164898,#164899,#164900,#164901,#164902,
#164903,#164904,#164905),(#164906,#164907,#164908,#164909,#164910,#164911,
#164912,#164913,#164914),(#164915,#164916,#164917,#164918,#164919,#164920,
#164921,#164922,#164923),(#164924,#164925,#164926,#164927,#164928,#164929,
#164930,#164931,#164932),(#164933,#164934,#164935,#164936,#164937,#164938,
#164939,#164940,#164941),(#164942,#164943,#164944,#164945,#164946,#164947,
#164948,#164949,#164950),(#164951,#164952,#164953,#164954,#164955,#164956,
#164957,#164958,#164959),(#164960,#164961,#164962,#164963,#164964,#164965,
#164966,#164967,#164968),(#164969,#164970,#164971,#164972,#164973,#164974,
#164975,#164976,#164977),(#164978,#164979,#164980,#164981,#164982,#164983,
#164984,#164985,#164986),(#164987,#164988,#164989,#164990,#164991,#164992,
#164993,#164994,#164995),(#164996,#164997,#164998,#164999,#165000,#165001,
#165002,#165003,#165004),(#165005,#165006,#165007,#165008,#165009,#165010,
#165011,#165012,#165013),(#165014,#165015,#165016,#165017,#165018,#165019,
#165020,#165021,#165022),(#165023,#165024,#165025,#165026,#165027,#165028,
#165029,#165030,#165031),(#165032,#165033,#165034,#165035,#165036,#165037,
#165038,#165039,#165040),(#165041,#165042,#165043,#165044,#165045,#165046,
#165047,#165048,#165049),(#165050,#165051,#165052,#165053,#165054,#165055,
#165056,#165057,#165058),(#165059,#165060,#165061,#165062,#165063,#165064,
#165065,#165066,#165067),(#165068,#165069,#165070,#165071,#165072,#165073,
#165074,#165075,#165076),(#165077,#165078,#165079,#165080,#165081,#165082,
#165083,#165084,#165085),(#165086,#165087,#165088,#165089,#165090,#165091,
#165092,#165093,#165094),(#165095,#165096,#165097,#165098,#165099,#165100,
#165101,#165102,#165103),(#165104,#165105,#165106,#165107,#165108,#165109,
#165110,#165111,#165112),(#165113,#165114,#165115,#165116,#165117,#165118,
#165119,#165120,#165121),(#165122,#165123,#165124,#165125,#165126,#165127,
#165128,#165129,#165130),(#165131,#165132,#165133,#165134,#165135,#165136,
#165137,#165138,#165139),(#165140,#165141,#165142,#165143,#165144,#165145,
#165146,#165147,#165148),(#165149,#165150,#165151,#165152,#165153,#165154,
#165155,#165156,#165157),(#165158,#165159,#165160,#165161,#165162,#165163,
#165164,#165165,#165166),(#165167,#165168,#165169,#165170,#165171,#165172,
#165173,#165174,#165175),(#165176,#165177,#165178,#165179,#165180,#165181,
#165182,#165183,#165184),(#165185,#165186,#165187,#165188,#165189,#165190,
#165191,#165192,#165193),(#165194,#165195,#165196,#165197,#165198,#165199,
#165200,#165201,#165202),(#165203,#165204,#165205,#165206,#165207,#165208,
#165209,#165210,#165211),(#165212,#165213,#165214,#165215,#165216,#165217,
#165218,#165219,#165220),(#165221,#165222,#165223,#165224,#165225,#165226,
#165227,#165228,#165229),(#165230,#165231,#165232,#165233,#165234,#165235,
#165236,#165237,#165238),(#165239,#165240,#165241,#165242,#165243,#165244,
#165245,#165246,#165247),(#165248,#165249,#165250,#165251,#165252,#165253,
#165254,#165255,#165256),(#165257,#165258,#165259,#165260,#165261,#165262,
#165263,#165264,#165265),(#165266,#165267,#165268,#165269,#165270,#165271,
#165272,#165273,#165274),(#165275,#165276,#165277,#165278,#165279,#165280,
#165281,#165282,#165283),(#165284,#165285,#165286,#165287,#165288,#165289,
#165290,#165291,#165292),(#165293,#165294,#165295,#165296,#165297,#165298,
#165299,#165300,#165301),(#165302,#165303,#165304,#165305,#165306,#165307,
#165308,#165309,#165310),(#165311,#165312,#165313,#165314,#165315,#165316,
#165317,#165318,#165319),(#165320,#165321,#165322,#165323,#165324,#165325,
#165326,#165327,#165328),(#165329,#165330,#165331,#165332,#165333,#165334,
#165335,#165336,#165337),(#165338,#165339,#165340,#165341,#165342,#165343,
#165344,#165345,#165346),(#165347,#165348,#165349,#165350,#165351,#165352,
#165353,#165354,#165355),(#165356,#165357,#165358,#165359,#165360,#165361,
#165362,#165363,#165364),(#165365,#165366,#165367,#165368,#165369,#165370,
#165371,#165372,#165373),(#165374,#165375,#165376,#165377,#165378,#165379,
#165380,#165381,#165382),(#165383,#165384,#165385,#165386,#165387,#165388,
#165389,#165390,#165391),(#165392,#165393,#165394,#165395,#165396,#165397,
#165398,#165399,#165400),(#165401,#165402,#165403,#165404,#165405,#165406,
#165407,#165408,#165409),(#165410,#165411,#165412,#165413,#165414,#165415,
#165416,#165417,#165418),(#165419,#165420,#165421,#165422,#165423,#165424,
#165425,#165426,#165427),(#165428,#165429,#165430,#165431,#165432,#165433,
#165434,#165435,#165436),(#165437,#165438,#165439,#165440,#165441,#165442,
#165443,#165444,#165445),(#165446,#165447,#165448,#165449,#165450,#165451,
#165452,#165453,#165454),(#165455,#165456,#165457,#165458,#165459,#165460,
#165461,#165462,#165463),(#165464,#165465,#165466,#165467,#165468,#165469,
#165470,#165471,#165472),(#165473,#165474,#165475,#165476,#165477,#165478,
#165479,#165480,#165481),(#165482,#165483,#165484,#165485,#165486,#165487,
#165488,#165489,#165490),(#165491,#165492,#165493,#165494,#165495,#165496,
#165497,#165498,#165499),(#165500,#165501,#165502,#165503,#165504,#165505,
#165506,#165507,#165508),(#165509,#165510,#165511,#165512,#165513,#165514,
#165515,#165516,#165517),(#165518,#165519,#165520,#165521,#165522,#165523,
#165524,#165525,#165526),(#165527,#165528,#165529,#165530,#165531,#165532,
#165533,#165534,#165535),(#165536,#165537,#165538,#165539,#165540,#165541,
#165542,#165543,#165544),(#165545,#165546,#165547,#165548,#165549,#165550,
#165551,#165552,#165553),(#165554,#165555,#165556,#165557,#165558,#165559,
#165560,#165561,#165562),(#165563,#165564,#165565,#165566,#165567,#165568,
#165569,#165570,#165571),(#165572,#165573,#165574,#165575,#165576,#165577,
#165578,#165579,#165580),(#165581,#165582,#165583,#165584,#165585,#165586,
#165587,#165588,#165589),(#165590,#165591,#165592,#165593,#165594,#165595,
#165596,#165597,#165598),(#165599,#165600,#165601,#165602,#165603,#165604,
#165605,#165606,#165607),(#165608,#165609,#165610,#165611,#165612,#165613,
#165614,#165615,#165616),(#165617,#165618,#165619,#165620,#165621,#165622,
#165623,#165624,#165625),(#165626,#165627,#165628,#165629,#165630,#165631,
#165632,#165633,#165634),(#165635,#165636,#165637,#165638,#165639,#165640,
#165641,#165642,#165643),(#165644,#165645,#165646,#165647,#165648,#165649,
#165650,#165651,#165652),(#165653,#165654,#165655,#165656,#165657,#165658,
#165659,#165660,#165661),(#165662,#165663,#165664,#165665,#165666,#165667,
#165668,#165669,#165670),(#165671,#165672,#165673,#165674,#165675,#165676,
#165677,#165678,#165679),(#165680,#165681,#165682,#165683,#165684,#165685,
#165686,#165687,#165688),(#165689,#165690,#165691,#165692,#165693,#165694,
#165695,#165696,#165697),(#165698,#165699,#165700,#165701,#165702,#165703,
#165704,#165705,#165706),(#165707,#165708,#165709,#165710,#165711,#165712,
#165713,#165714,#165715),(#165716,#165717,#165718,#165719,#165720,#165721,
#165722,#165723,#165724),(#165725,#165726,#165727,#165728,#165729,#165730,
#165731,#165732,#165733),(#165734,#165735,#165736,#165737,#165738,#165739,
#165740,#165741,#165742),(#165743,#165744,#165745,#165746,#165747,#165748,
#165749,#165750,#165751),(#165752,#165753,#165754,#165755,#165756,#165757,
#165758,#165759,#165760),(#165761,#165762,#165763,#165764,#165765,#165766,
#165767,#165768,#165769),(#165770,#165771,#165772,#165773,#165774,#165775,
#165776,#165777,#165778),(#165779,#165780,#165781,#165782,#165783,#165784,
#165785,#165786,#165787),(#165788,#165789,#165790,#165791,#165792,#165793,
#165794,#165795,#165796),(#165797,#165798,#165799,#165800,#165801,#165802,
#165803,#165804,#165805),(#165806,#165807,#165808,#165809,#165810,#165811,
#165812,#165813,#165814),(#165815,#165816,#165817,#165818,#165819,#165820,
#165821,#165822,#165823),(#165824,#165825,#165826,#165827,#165828,#165829,
#165830,#165831,#165832),(#165833,#165834,#165835,#165836,#165837,#165838,
#165839,#165840,#165841),(#165842,#165843,#165844,#165845,#165846,#165847,
#165848,#165849,#165850),(#165851,#165852,#165853,#165854,#165855,#165856,
#165857,#165858,#165859),(#165860,#165861,#165862,#165863,#165864,#165865,
#165866,#165867,#165868),(#165869,#165870,#165871,#165872,#165873,#165874,
#165875,#165876,#165877),(#165878,#165879,#165880,#165881,#165882,#165883,
#165884,#165885,#165886),(#165887,#165888,#165889,#165890,#165891,#165892,
#165893,#165894,#165895),(#165896,#165897,#165898,#165899,#165900,#165901,
#165902,#165903,#165904),(#165905,#165906,#165907,#165908,#165909,#165910,
#165911,#165912,#165913),(#165914,#165915,#165916,#165917,#165918,#165919,
#165920,#165921,#165922),(#165923,#165924,#165925,#165926,#165927,#165928,
#165929,#165930,#165931),(#165932,#165933,#165934,#165935,#165936,#165937,
#165938,#165939,#165940),(#165941,#165942,#165943,#165944,#165945,#165946,
#165947,#165948,#165949),(#165950,#165951,#165952,#165953,#165954,#165955,
#165956,#165957,#165958),(#165959,#165960,#165961,#165962,#165963,#165964,
#165965,#165966,#165967),(#165968,#165969,#165970,#165971,#165972,#165973,
#165974,#165975,#165976),(#165977,#165978,#165979,#165980,#165981,#165982,
#165983,#165984,#165985),(#165986,#165987,#165988,#165989,#165990,#165991,
#165992,#165993,#165994),(#165995,#165996,#165997,#165998,#165999,#166000,
#166001,#166002,#166003),(#166004,#166005,#166006,#166007,#166008,#166009,
#166010,#166011,#166012),(#166013,#166014,#166015,#166016,#166017,#166018,
#166019,#166020,#166021),(#166022,#166023,#166024,#166025,#166026,#166027,
#166028,#166029,#166030),(#166031,#166032,#166033,#166034,#166035,#166036,
#166037,#166038,#166039),(#166040,#166041,#166042,#166043,#166044,#166045,
#166046,#166047,#166048),(#166049,#166050,#166051,#166052,#166053,#166054,
#166055,#166056,#166057),(#166058,#166059,#166060,#166061,#166062,#166063,
#166064,#166065,#166066),(#166067,#166068,#166069,#166070,#166071,#166072,
#166073,#166074,#166075),(#166076,#166077,#166078,#166079,#166080,#166081,
#166082,#166083,#166084),(#166085,#166086,#166087,#166088,#166089,#166090,
#166091,#166092,#166093),(#166094,#166095,#166096,#166097,#166098,#166099,
#166100,#166101,#166102),(#166103,#166104,#166105,#166106,#166107,#166108,
#166109,#166110,#166111),(#166112,#166113,#166114,#166115,#166116,#166117,
#166118,#166119,#166120),(#166121,#166122,#166123,#166124,#166125,#166126,
#166127,#166128,#166129),(#166130,#166131,#166132,#166133,#166134,#166135,
#166136,#166137,#166138),(#166139,#166140,#166141,#166142,#166143,#166144,
#166145,#166146,#166147),(#166148,#166149,#166150,#166151,#166152,#166153,
#166154,#166155,#166156),(#166157,#166158,#166159,#166160,#166161,#166162,
#166163,#166164,#166165),(#166166,#166167,#166168,#166169,#166170,#166171,
#166172,#166173,#166174),(#166175,#166176,#166177,#166178,#166179,#166180,
#166181,#166182,#166183),(#166184,#166185,#166186,#166187,#166188,#166189,
#166190,#166191,#166192),(#166193,#166194,#166195,#166196,#166197,#166198,
#166199,#166200,#166201),(#166202,#166203,#166204,#166205,#166206,#166207,
#166208,#166209,#166210),(#166211,#166212,#166213,#166214,#166215,#166216,
#166217,#166218,#166219),(#166220,#166221,#166222,#166223,#166224,#166225,
#166226,#166227,#166228),(#166229,#166230,#166231,#166232,#166233,#166234,
#166235,#166236,#166237),(#166238,#166239,#166240,#166241,#166242,#166243,
#166244,#166245,#166246),(#166247,#166248,#166249,#166250,#166251,#166252,
#166253,#166254,#166255),(#166256,#166257,#166258,#166259,#166260,#166261,
#166262,#166263,#166264),(#166265,#166266,#166267,#166268,#166269,#166270,
#166271,#166272,#166273),(#166274,#166275,#166276,#166277,#166278,#166279,
#166280,#166281,#166282),(#166283,#166284,#166285,#166286,#166287,#166288,
#166289,#166290,#166291),(#166292,#166293,#166294,#166295,#166296,#166297,
#166298,#166299,#166300),(#166301,#166302,#166303,#166304,#166305,#166306,
#166307,#166308,#166309),(#166310,#166311,#166312,#166313,#166314,#166315,
#166316,#166317,#166318),(#166319,#166320,#166321,#166322,#166323,#166324,
#166325,#166326,#166327),(#166328,#166329,#166330,#166331,#166332,#166333,
#166334,#166335,#166336),(#166337,#166338,#166339,#166340,#166341,#166342,
#166343,#166344,#166345),(#166346,#166347,#166348,#166349,#166350,#166351,
#166352,#166353,#166354),(#166355,#166356,#166357,#166358,#166359,#166360,
#166361,#166362,#166363),(#166364,#166365,#166366,#166367,#166368,#166369,
#166370,#166371,#166372),(#166373,#166374,#166375,#166376,#166377,#166378,
#166379,#166380,#166381),(#166382,#166383,#166384,#166385,#166386,#166387,
#166388,#166389,#166390),(#166391,#166392,#166393,#166394,#166395,#166396,
#166397,#166398,#166399),(#166400,#166401,#166402,#166403,#166404,#166405,
#166406,#166407,#166408),(#166409,#166410,#166411,#166412,#166413,#166414,
#166415,#166416,#166417),(#166418,#166419,#166420,#166421,#166422,#166423,
#166424,#166425,#166426),(#166427,#166428,#166429,#166430,#166431,#166432,
#166433,#166434,#166435),(#166436,#166437,#166438,#166439,#166440,#166441,
#166442,#166443,#166444),(#166445,#166446,#166447,#166448,#166449,#166450,
#166451,#166452,#166453),(#166454,#166455,#166456,#166457,#166458,#166459,
#166460,#166461,#166462),(#166463,#166464,#166465,#166466,#166467,#166468,
#166469,#166470,#166471),(#166472,#166473,#166474,#166475,#166476,#166477,
#166478,#166479,#166480),(#166481,#166482,#166483,#166484,#166485,#166486,
#166487,#166488,#166489),(#166490,#166491,#166492,#166493,#166494,#166495,
#166496,#166497,#166498),(#166499,#166500,#166501,#166502,#166503,#166504,
#166505,#166506,#166507),(#166508,#166509,#166510,#166511,#166512,#166513,
#166514,#166515,#166516),(#166517,#166518,#166519,#166520,#166521,#166522,
#166523,#166524,#166525),(#166526,#166527,#166528,#166529,#166530,#166531,
#166532,#166533,#166534),(#166535,#166536,#166537,#166538,#166539,#166540,
#166541,#166542,#166543),(#166544,#166545,#166546,#166547,#166548,#166549,
#166550,#166551,#166552),(#166553,#166554,#166555,#166556,#166557,#166558,
#166559,#166560,#166561),(#166562,#166563,#166564,#166565,#166566,#166567,
#166568,#166569,#166570),(#166571,#166572,#166573,#166574,#166575,#166576,
#166577,#166578,#166579),(#166580,#166581,#166582,#166583,#166584,#166585,
#166586,#166587,#166588),(#166589,#166590,#166591,#166592,#166593,#166594,
#166595,#166596,#166597),(#166598,#166599,#166600,#166601,#166602,#166603,
#166604,#166605,#166606),(#166607,#166608,#166609,#166610,#166611,#166612,
#166613,#166614,#166615),(#166616,#166617,#166618,#166619,#166620,#166621,
#166622,#166623,#166624),(#166625,#166626,#166627,#166628,#166629,#166630,
#166631,#166632,#166633),(#166634,#166635,#166636,#166637,#166638,#166639,
#166640,#166641,#166642),(#166643,#166644,#166645,#166646,#166647,#166648,
#166649,#166650,#166651),(#166652,#166653,#166654,#166655,#166656,#166657,
#166658,#166659,#166660),(#166661,#166662,#166663,#166664,#166665,#166666,
#166667,#166668,#166669),(#166670,#166671,#166672,#166673,#166674,#166675,
#166676,#166677,#166678),(#166679,#166680,#166681,#166682,#166683,#166684,
#166685,#166686,#166687),(#166688,#166689,#166690,#166691,#166692,#166693,
#166694,#166695,#166696),(#166697,#166698,#166699,#166700,#166701,#166702,
#166703,#166704,#166705),(#166706,#166707,#166708,#166709,#166710,#166711,
#166712,#166713,#166714),(#166715,#166716,#166717,#166718,#166719,#166720,
#166721,#166722,#166723),(#166724,#166725,#166726,#166727,#166728,#166729,
#166730,#166731,#166732),(#166733,#166734,#166735,#166736,#166737,#166738,
#166739,#166740,#166741),(#166742,#166743,#166744,#166745,#166746,#166747,
#166748,#166749,#166750),(#166751,#166752,#166753,#166754,#166755,#166756,
#166757,#166758,#166759),(#166760,#166761,#166762,#166763,#166764,#166765,
#166766,#166767,#166768),(#166769,#166770,#166771,#166772,#166773,#166774,
#166775,#166776,#166777),(#166778,#166779,#166780,#166781,#166782,#166783,
#166784,#166785,#166786),(#166787,#166788,#166789,#166790,#166791,#166792,
#166793,#166794,#166795),(#166796,#166797,#166798,#166799,#166800,#166801,
#166802,#166803,#166804),(#166805,#166806,#166807,#166808,#166809,#166810,
#166811,#166812,#166813),(#166814,#166815,#166816,#166817,#166818,#166819,
#166820,#166821,#166822),(#166823,#166824,#166825,#166826,#166827,#166828,
#166829,#166830,#166831),(#166832,#166833,#166834,#166835,#166836,#166837,
#166838,#166839,#166840),(#166841,#166842,#166843,#166844,#166845,#166846,
#166847,#166848,#166849),(#166850,#166851,#166852,#166853,#166854,#166855,
#166856,#166857,#166858),(#166859,#166860,#166861,#166862,#166863,#166864,
#166865,#166866,#166867),(#166868,#166869,#166870,#166871,#166872,#166873,
#166874,#166875,#166876),(#166877,#166878,#166879,#166880,#166881,#166882,
#166883,#166884,#166885),(#166886,#166887,#166888,#166889,#166890,#166891,
#166892,#166893,#166894),(#166895,#166896,#166897,#166898,#166899,#166900,
#166901,#166902,#166903),(#166904,#166905,#166906,#166907,#166908,#166909,
#166910,#166911,#166912),(#166913,#166914,#166915,#166916,#166917,#166918,
#166919,#166920,#166921),(#166922,#166923,#166924,#166925,#166926,#166927,
#166928,#166929,#166930),(#166931,#166932,#166933,#166934,#166935,#166936,
#166937,#166938,#166939),(#166940,#166941,#166942,#166943,#166944,#166945,
#166946,#166947,#166948),(#166949,#166950,#166951,#166952,#166953,#166954,
#166955,#166956,#166957),(#166958,#166959,#166960,#166961,#166962,#166963,
#166964,#166965,#166966),(#166967,#166968,#166969,#166970,#166971,#166972,
#166973,#166974,#166975),(#166976,#166977,#166978,#166979,#166980,#166981,
#166982,#166983,#166984),(#166985,#166986,#166987,#166988,#166989,#166990,
#166991,#166992,#166993),(#166994,#166995,#166996,#166997,#166998,#166999,
#167000,#167001,#167002),(#167003,#167004,#167005,#167006,#167007,#167008,
#167009,#167010,#167011),(#167012,#167013,#167014,#167015,#167016,#167017,
#167018,#167019,#167020),(#167021,#167022,#167023,#167024,#167025,#167026,
#167027,#167028,#167029),(#167030,#167031,#167032,#167033,#167034,#167035,
#167036,#167037,#167038),(#167039,#167040,#167041,#167042,#167043,#167044,
#167045,#167046,#167047),(#167048,#167049,#167050,#167051,#167052,#167053,
#167054,#167055,#167056),(#167057,#167058,#167059,#167060,#167061,#167062,
#167063,#167064,#167065),(#167066,#167067,#167068,#167069,#167070,#167071,
#167072,#167073,#167074),(#167075,#167076,#167077,#167078,#167079,#167080,
#167081,#167082,#167083),(#167084,#167085,#167086,#167087,#167088,#167089,
#167090,#167091,#167092),(#167093,#167094,#167095,#167096,#167097,#167098,
#167099,#167100,#167101),(#167102,#167103,#167104,#167105,#167106,#167107,
#167108,#167109,#167110),(#167111,#167112,#167113,#167114,#167115,#167116,
#167117,#167118,#167119),(#167120,#167121,#167122,#167123,#167124,#167125,
#167126,#167127,#167128),(#167129,#167130,#167131,#167132,#167133,#167134,
#167135,#167136,#167137),(#167138,#167139,#167140,#167141,#167142,#167143,
#167144,#167145,#167146),(#167147,#167148,#167149,#167150,#167151,#167152,
#167153,#167154,#167155),(#167156,#167157,#167158,#167159,#167160,#167161,
#167162,#167163,#167164),(#167165,#167166,#167167,#167168,#167169,#167170,
#167171,#167172,#167173),(#167174,#167175,#167176,#167177,#167178,#167179,
#167180,#167181,#167182),(#167183,#167184,#167185,#167186,#167187,#167188,
#167189,#167190,#167191),(#167192,#167193,#167194,#167195,#167196,#167197,
#167198,#167199,#167200),(#167201,#167202,#167203,#167204,#167205,#167206,
#167207,#167208,#167209),(#167210,#167211,#167212,#167213,#167214,#167215,
#167216,#167217,#167218),(#167219,#167220,#167221,#167222,#167223,#167224,
#167225,#167226,#167227),(#167228,#167229,#167230,#167231,#167232,#167233,
#167234,#167235,#167236),(#167237,#167238,#167239,#167240,#167241,#167242,
#167243,#167244,#167245),(#167246,#167247,#167248,#167249,#167250,#167251,
#167252,#167253,#167254),(#167255,#167256,#167257,#167258,#167259,#167260,
#167261,#167262,#167263),(#167264,#167265,#167266,#167267,#167268,#167269,
#167270,#167271,#167272),(#167273,#167274,#167275,#167276,#167277,#167278,
#167279,#167280,#167281),(#167282,#167283,#167284,#167285,#167286,#167287,
#167288,#167289,#167290),(#167291,#167292,#167293,#167294,#167295,#167296,
#167297,#167298,#167299),(#167300,#167301,#167302,#167303,#167304,#167305,
#167306,#167307,#167308),(#167309,#167310,#167311,#167312,#167313,#167314,
#167315,#167316,#167317),(#167318,#167319,#167320,#167321,#167322,#167323,
#167324,#167325,#167326),(#167327,#167328,#167329,#167330,#167331,#167332,
#167333,#167334,#167335),(#167336,#167337,#167338,#167339,#167340,#167341,
#167342,#167343,#167344),(#167345,#167346,#167347,#167348,#167349,#167350,
#167351,#167352,#167353),(#167354,#167355,#167356,#167357,#167358,#167359,
#167360,#167361,#167362),(#167363,#167364,#167365,#167366,#167367,#167368,
#167369,#167370,#167371),(#167372,#167373,#167374,#167375,#167376,#167377,
#167378,#167379,#167380),(#167381,#167382,#167383,#167384,#167385,#167386,
#167387,#167388,#167389),(#167390,#167391,#167392,#167393,#167394,#167395,
#167396,#167397,#167398),(#167399,#167400,#167401,#167402,#167403,#167404,
#167405,#167406,#167407),(#167408,#167409,#167410,#167411,#167412,#167413,
#167414,#167415,#167416),(#167417,#167418,#167419,#167420,#167421,#167422,
#167423,#167424,#167425),(#167426,#167427,#167428,#167429,#167430,#167431,
#167432,#167433,#167434),(#167435,#167436,#167437,#167438,#167439,#167440,
#167441,#167442,#167443),(#167444,#167445,#167446,#167447,#167448,#167449,
#167450,#167451,#167452),(#167453,#167454,#167455,#167456,#167457,#167458,
#167459,#167460,#167461),(#167462,#167463,#167464,#167465,#167466,#167467,
#167468,#167469,#167470),(#167471,#167472,#167473,#167474,#167475,#167476,
#167477,#167478,#167479),(#167480,#167481,#167482,#167483,#167484,#167485,
#167486,#167487,#167488),(#167489,#167490,#167491,#167492,#167493,#167494,
#167495,#167496,#167497),(#167498,#167499,#167500,#167501,#167502,#167503,
#167504,#167505,#167506),(#167507,#167508,#167509,#167510,#167511,#167512,
#167513,#167514,#167515),(#167516,#167517,#167518,#167519,#167520,#167521,
#167522,#167523,#167524),(#167525,#167526,#167527,#167528,#167529,#167530,
#167531,#167532,#167533),(#167534,#167535,#167536,#167537,#167538,#167539,
#167540,#167541,#167542),(#167543,#167544,#167545,#167546,#167547,#167548,
#167549,#167550,#167551),(#167552,#167553,#167554,#167555,#167556,#167557,
#167558,#167559,#167560),(#167561,#167562,#167563,#167564,#167565,#167566,
#167567,#167568,#167569),(#167570,#167571,#167572,#167573,#167574,#167575,
#167576,#167577,#167578),(#167579,#167580,#167581,#167582,#167583,#167584,
#167585,#167586,#167587),(#167588,#167589,#167590,#167591,#167592,#167593,
#167594,#167595,#167596),(#167597,#167598,#167599,#167600,#167601,#167602,
#167603,#167604,#167605),(#167606,#167607,#167608,#167609,#167610,#167611,
#167612,#167613,#167614),(#167615,#167616,#167617,#167618,#167619,#167620,
#167621,#167622,#167623),(#167624,#167625,#167626,#167627,#167628,#167629,
#167630,#167631,#167632),(#167633,#167634,#167635,#167636,#167637,#167638,
#167639,#167640,#167641),(#167642,#167643,#167644,#167645,#167646,#167647,
#167648,#167649,#167650),(#167651,#167652,#167653,#167654,#167655,#167656,
#167657,#167658,#167659),(#167660,#167661,#167662,#167663,#167664,#167665,
#167666,#167667,#167668),(#167669,#167670,#167671,#167672,#167673,#167674,
#167675,#167676,#167677),(#167678,#167679,#167680,#167681,#167682,#167683,
#167684,#167685,#167686),(#167687,#167688,#167689,#167690,#167691,#167692,
#167693,#167694,#167695),(#167696,#167697,#167698,#167699,#167700,#167701,
#167702,#167703,#167704),(#167705,#167706,#167707,#167708,#167709,#167710,
#167711,#167712,#167713),(#167714,#167715,#167716,#167717,#167718,#167719,
#167720,#167721,#167722),(#167723,#167724,#167725,#167726,#167727,#167728,
#167729,#167730,#167731),(#167732,#167733,#167734,#167735,#167736,#167737,
#167738,#167739,#167740),(#167741,#167742,#167743,#167744,#167745,#167746,
#167747,#167748,#167749),(#167750,#167751,#167752,#167753,#167754,#167755,
#167756,#167757,#167758),(#167759,#167760,#167761,#167762,#167763,#167764,
#167765,#167766,#167767),(#167768,#167769,#167770,#167771,#167772,#167773,
#167774,#167775,#167776),(#167777,#167778,#167779,#167780,#167781,#167782,
#167783,#167784,#167785),(#167786,#167787,#167788,#167789,#167790,#167791,
#167792,#167793,#167794),(#167795,#167796,#167797,#167798,#167799,#167800,
#167801,#167802,#167803),(#167804,#167805,#167806,#167807,#167808,#167809,
#167810,#167811,#167812),(#167813,#167814,#167815,#167816,#167817,#167818,
#167819,#167820,#167821),(#167822,#167823,#167824,#167825,#167826,#167827,
#167828,#167829,#167830),(#167831,#167832,#167833,#167834,#167835,#167836,
#167837,#167838,#167839),(#167840,#167841,#167842,#167843,#167844,#167845,
#167846,#167847,#167848),(#167849,#167850,#167851,#167852,#167853,#167854,
#167855,#167856,#167857),(#167858,#167859,#167860,#167861,#167862,#167863,
#167864,#167865,#167866),(#167867,#167868,#167869,#167870,#167871,#167872,
#167873,#167874,#167875),(#167876,#167877,#167878,#167879,#167880,#167881,
#167882,#167883,#167884),(#167885,#167886,#167887,#167888,#167889,#167890,
#167891,#167892,#167893),(#167894,#167895,#167896,#167897,#167898,#167899,
#167900,#167901,#167902),(#167903,#167904,#167905,#167906,#167907,#167908,
#167909,#167910,#167911),(#167912,#167913,#167914,#167915,#167916,#167917,
#167918,#167919,#167920),(#167921,#167922,#167923,#167924,#167925,#167926,
#167927,#167928,#167929),(#167930,#167931,#167932,#167933,#167934,#167935,
#167936,#167937,#167938),(#167939,#167940,#167941,#167942,#167943,#167944,
#167945,#167946,#167947),(#167948,#167949,#167950,#167951,#167952,#167953,
#167954,#167955,#167956),(#167957,#167958,#167959,#167960,#167961,#167962,
#167963,#167964,#167965),(#167966,#167967,#167968,#167969,#167970,#167971,
#167972,#167973,#167974),(#167975,#167976,#167977,#167978,#167979,#167980,
#167981,#167982,#167983),(#167984,#167985,#167986,#167987,#167988,#167989,
#167990,#167991,#167992),(#167993,#167994,#167995,#167996,#167997,#167998,
#167999,#168000,#168001),(#168002,#168003,#168004,#168005,#168006,#168007,
#168008,#168009,#168010),(#168011,#168012,#168013,#168014,#168015,#168016,
#168017,#168018,#168019),(#168020,#168021,#168022,#168023,#168024,#168025,
#168026,#168027,#168028),(#168029,#168030,#168031,#168032,#168033,#168034,
#168035,#168036,#168037),(#168038,#168039,#168040,#168041,#168042,#168043,
#168044,#168045,#168046),(#168047,#168048,#168049,#168050,#168051,#168052,
#168053,#168054,#168055),(#168056,#168057,#168058,#168059,#168060,#168061,
#168062,#168063,#168064),(#168065,#168066,#168067,#168068,#168069,#168070,
#168071,#168072,#168073),(#168074,#168075,#168076,#168077,#168078,#168079,
#168080,#168081,#168082),(#168083,#168084,#168085,#168086,#168087,#168088,
#168089,#168090,#168091),(#168092,#168093,#168094,#168095,#168096,#168097,
#168098,#168099,#168100),(#168101,#168102,#168103,#168104,#168105,#168106,
#168107,#168108,#168109),(#168110,#168111,#168112,#168113,#168114,#168115,
#168116,#168117,#168118),(#168119,#168120,#168121,#168122,#168123,#168124,
#168125,#168126,#168127),(#168128,#168129,#168130,#168131,#168132,#168133,
#168134,#168135,#168136),(#168137,#168138,#168139,#168140,#168141,#168142,
#168143,#168144,#168145),(#168146,#168147,#168148,#168149,#168150,#168151,
#168152,#168153,#168154),(#168155,#168156,#168157,#168158,#168159,#168160,
#168161,#168162,#168163),(#168164,#168165,#168166,#168167,#168168,#168169,
#168170,#168171,#168172),(#168173,#168174,#168175,#168176,#168177,#168178,
#168179,#168180,#168181),(#168182,#168183,#168184,#168185,#168186,#168187,
#168188,#168189,#168190),(#168191,#168192,#168193,#168194,#168195,#168196,
#168197,#168198,#168199),(#168200,#168201,#168202,#168203,#168204,#168205,
#168206,#168207,#168208),(#168209,#168210,#168211,#168212,#168213,#168214,
#168215,#168216,#168217),(#168218,#168219,#168220,#168221,#168222,#168223,
#168224,#168225,#168226),(#168227,#168228,#168229,#168230,#168231,#168232,
#168233,#168234,#168235),(#168236,#168237,#168238,#168239,#168240,#168241,
#168242,#168243,#168244),(#168245,#168246,#168247,#168248,#168249,#168250,
#168251,#168252,#168253),(#168254,#168255,#168256,#168257,#168258,#168259,
#168260,#168261,#168262),(#168263,#168264,#168265,#168266,#168267,#168268,
#168269,#168270,#168271),(#168272,#168273,#168274,#168275,#168276,#168277,
#168278,#168279,#168280),(#168281,#168282,#168283,#168284,#168285,#168286,
#168287,#168288,#168289),(#168290,#168291,#168292,#168293,#168294,#168295,
#168296,#168297,#168298),(#168299,#168300,#168301,#168302,#168303,#168304,
#168305,#168306,#168307),(#168308,#168309,#168310,#168311,#168312,#168313,
#168314,#168315,#168316),(#168317,#168318,#168319,#168320,#168321,#168322,
#168323,#168324,#168325),(#168326,#168327,#168328,#168329,#168330,#168331,
#168332,#168333,#168334),(#168335,#168336,#168337,#168338,#168339,#168340,
#168341,#168342,#168343),(#168344,#168345,#168346,#168347,#168348,#168349,
#168350,#168351,#168352),(#168353,#168354,#168355,#168356,#168357,#168358,
#168359,#168360,#168361),(#168362,#168363,#168364,#168365,#168366,#168367,
#168368,#168369,#168370),(#168371,#168372,#168373,#168374,#168375,#168376,
#168377,#168378,#168379),(#168380,#168381,#168382,#168383,#168384,#168385,
#168386,#168387,#168388),(#168389,#168390,#168391,#168392,#168393,#168394,
#168395,#168396,#168397),(#168398,#168399,#168400,#168401,#168402,#168403,
#168404,#168405,#168406),(#168407,#168408,#168409,#168410,#168411,#168412,
#168413,#168414,#168415),(#168416,#168417,#168418,#168419,#168420,#168421,
#168422,#168423,#168424),(#168425,#168426,#168427,#168428,#168429,#168430,
#168431,#168432,#168433),(#168434,#168435,#168436,#168437,#168438,#168439,
#168440,#168441,#168442),(#168443,#168444,#168445,#168446,#168447,#168448,
#168449,#168450,#168451),(#168452,#168453,#168454,#168455,#168456,#168457,
#168458,#168459,#168460),(#168461,#168462,#168463,#168464,#168465,#168466,
#168467,#168468,#168469),(#168470,#168471,#168472,#168473,#168474,#168475,
#168476,#168477,#168478),(#168479,#168480,#168481,#168482,#168483,#168484,
#168485,#168486,#168487),(#168488,#168489,#168490,#168491,#168492,#168493,
#168494,#168495,#168496),(#168497,#168498,#168499,#168500,#168501,#168502,
#168503,#168504,#168505),(#168506,#168507,#168508,#168509,#168510,#168511,
#168512,#168513,#168514),(#168515,#168516,#168517,#168518,#168519,#168520,
#168521,#168522,#168523),(#168524,#168525,#168526,#168527,#168528,#168529,
#168530,#168531,#168532),(#168533,#168534,#168535,#168536,#168537,#168538,
#168539,#168540,#168541),(#168542,#168543,#168544,#168545,#168546,#168547,
#168548,#168549,#168550),(#168551,#168552,#168553,#168554,#168555,#168556,
#168557,#168558,#168559),(#168560,#168561,#168562,#168563,#168564,#168565,
#168566,#168567,#168568),(#168569,#168570,#168571,#168572,#168573,#168574,
#168575,#168576,#168577),(#168578,#168579,#168580,#168581,#168582,#168583,
#168584,#168585,#168586),(#168587,#168588,#168589,#168590,#168591,#168592,
#168593,#168594,#168595),(#168596,#168597,#168598,#168599,#168600,#168601,
#168602,#168603,#168604),(#168605,#168606,#168607,#168608,#168609,#168610,
#168611,#168612,#168613),(#168614,#168615,#168616,#168617,#168618,#168619,
#168620,#168621,#168622),(#168623,#168624,#168625,#168626,#168627,#168628,
#168629,#168630,#168631),(#168632,#168633,#168634,#168635,#168636,#168637,
#168638,#168639,#168640),(#168641,#168642,#168643,#168644,#168645,#168646,
#168647,#168648,#168649),(#168650,#168651,#168652,#168653,#168654,#168655,
#168656,#168657,#168658),(#168659,#168660,#168661,#168662,#168663,#168664,
#168665,#168666,#168667),(#168668,#168669,#168670,#168671,#168672,#168673,
#168674,#168675,#168676),(#168677,#168678,#168679,#168680,#168681,#168682,
#168683,#168684,#168685),(#168686,#168687,#168688,#168689,#168690,#168691,
#168692,#168693,#168694),(#168695,#168696,#168697,#168698,#168699,#168700,
#168701,#168702,#168703),(#168704,#168705,#168706,#168707,#168708,#168709,
#168710,#168711,#168712),(#168713,#168714,#168715,#168716,#168717,#168718,
#168719,#168720,#168721),(#168722,#168723,#168724,#168725,#168726,#168727,
#168728,#168729,#168730),(#168731,#168732,#168733,#168734,#168735,#168736,
#168737,#168738,#168739),(#168740,#168741,#168742,#168743,#168744,#168745,
#168746,#168747,#168748),(#168749,#168750,#168751,#168752,#168753,#168754,
#168755,#168756,#168757),(#168758,#168759,#168760,#168761,#168762,#168763,
#168764,#168765,#168766),(#168767,#168768,#168769,#168770,#168771,#168772,
#168773,#168774,#168775),(#168776,#168777,#168778,#168779,#168780,#168781,
#168782,#168783,#168784),(#168785,#168786,#168787,#168788,#168789,#168790,
#168791,#168792,#168793),(#168794,#168795,#168796,#168797,#168798,#168799,
#168800,#168801,#168802),(#168803,#168804,#168805,#168806,#168807,#168808,
#168809,#168810,#168811),(#168812,#168813,#168814,#168815,#168816,#168817,
#168818,#168819,#168820),(#168821,#168822,#168823,#168824,#168825,#168826,
#168827,#168828,#168829),(#168830,#168831,#168832,#168833,#168834,#168835,
#168836,#168837,#168838),(#168839,#168840,#168841,#168842,#168843,#168844,
#168845,#168846,#168847),(#168848,#168849,#168850,#168851,#168852,#168853,
#168854,#168855,#168856),(#168857,#168858,#168859,#168860,#168861,#168862,
#168863,#168864,#168865),(#168866,#168867,#168868,#168869,#168870,#168871,
#168872,#168873,#168874),(#168875,#168876,#168877,#168878,#168879,#168880,
#168881,#168882,#168883),(#168884,#168885,#168886,#168887,#168888,#168889,
#168890,#168891,#168892),(#168893,#168894,#168895,#168896,#168897,#168898,
#168899,#168900,#168901),(#168902,#168903,#168904,#168905,#168906,#168907,
#168908,#168909,#168910),(#168911,#168912,#168913,#168914,#168915,#168916,
#168917,#168918,#168919),(#168920,#168921,#168922,#168923,#168924,#168925,
#168926,#168927,#168928),(#168929,#168930,#168931,#168932,#168933,#168934,
#168935,#168936,#168937),(#168938,#168939,#168940,#168941,#168942,#168943,
#168944,#168945,#168946),(#168947,#168948,#168949,#168950,#168951,#168952,
#168953,#168954,#168955),(#168956,#168957,#168958,#168959,#168960,#168961,
#168962,#168963,#168964),(#168965,#168966,#168967,#168968,#168969,#168970,
#168971,#168972,#168973),(#168974,#168975,#168976,#168977,#168978,#168979,
#168980,#168981,#168982),(#168983,#168984,#168985,#168986,#168987,#168988,
#168989,#168990,#168991),(#168992,#168993,#168994,#168995,#168996,#168997,
#168998,#168999,#169000),(#169001,#169002,#169003,#169004,#169005,#169006,
#169007,#169008,#169009),(#169010,#169011,#169012,#169013,#169014,#169015,
#169016,#169017,#169018),(#169019,#169020,#169021,#169022,#169023,#169024,
#169025,#169026,#169027),(#169028,#169029,#169030,#169031,#169032,#169033,
#169034,#169035,#169036),(#169037,#169038,#169039,#169040,#169041,#169042,
#169043,#169044,#169045),(#169046,#169047,#169048,#169049,#169050,#169051,
#169052,#169053,#169054),(#169055,#169056,#169057,#169058,#169059,#169060,
#169061,#169062,#169063),(#169064,#169065,#169066,#169067,#169068,#169069,
#169070,#169071,#169072),(#169073,#169074,#169075,#169076,#169077,#169078,
#169079,#169080,#169081),(#169082,#169083,#169084,#169085,#169086,#169087,
#169088,#169089,#169090),(#169091,#169092,#169093,#169094,#169095,#169096,
#169097,#169098,#169099),(#169100,#169101,#169102,#169103,#169104,#169105,
#169106,#169107,#169108),(#169109,#169110,#169111,#169112,#169113,#169114,
#169115,#169116,#169117),(#169118,#169119,#169120,#169121,#169122,#169123,
#169124,#169125,#169126),(#169127,#169128,#169129,#169130,#169131,#169132,
#169133,#169134,#169135),(#169136,#169137,#169138,#169139,#169140,#169141,
#169142,#169143,#169144),(#169145,#169146,#169147,#169148,#169149,#169150,
#169151,#169152,#169153),(#169154,#169155,#169156,#169157,#169158,#169159,
#169160,#169161,#169162),(#169163,#169164,#169165,#169166,#169167,#169168,
#169169,#169170,#169171),(#169172,#169173,#169174,#169175,#169176,#169177,
#169178,#169179,#169180),(#169181,#169182,#169183,#169184,#169185,#169186,
#169187,#169188,#169189),(#169190,#169191,#169192,#169193,#169194,#169195,
#169196,#169197,#169198),(#169199,#169200,#169201,#169202,#169203,#169204,
#169205,#169206,#169207),(#169208,#169209,#169210,#169211,#169212,#169213,
#169214,#169215,#169216),(#169217,#169218,#169219,#169220,#169221,#169222,
#169223,#169224,#169225),(#169226,#169227,#169228,#169229,#169230,#169231,
#169232,#169233,#169234),(#169235,#169236,#169237,#169238,#169239,#169240,
#169241,#169242,#169243),(#169244,#169245,#169246,#169247,#169248,#169249,
#169250,#169251,#169252),(#169253,#169254,#169255,#169256,#169257,#169258,
#169259,#169260,#169261),(#169262,#169263,#169264,#169265,#169266,#169267,
#169268,#169269,#169270),(#169271,#169272,#169273,#169274,#169275,#169276,
#169277,#169278,#169279),(#169280,#169281,#169282,#169283,#169284,#169285,
#169286,#169287,#169288),(#169289,#169290,#169291,#169292,#169293,#169294,
#169295,#169296,#169297),(#169298,#169299,#169300,#169301,#169302,#169303,
#169304,#169305,#169306),(#169307,#169308,#169309,#169310,#169311,#169312,
#169313,#169314,#169315),(#169316,#169317,#169318,#169319,#169320,#169321,
#169322,#169323,#169324),(#169325,#169326,#169327,#169328,#169329,#169330,
#169331,#169332,#169333),(#169334,#169335,#169336,#169337,#169338,#169339,
#169340,#169341,#169342),(#169343,#169344,#169345,#169346,#169347,#169348,
#169349,#169350,#169351),(#169352,#169353,#169354,#169355,#169356,#169357,
#169358,#169359,#169360),(#169361,#169362,#169363,#169364,#169365,#169366,
#169367,#169368,#169369),(#169370,#169371,#169372,#169373,#169374,#169375,
#169376,#169377,#169378),(#169379,#169380,#169381,#169382,#169383,#169384,
#169385,#169386,#169387),(#169388,#169389,#169390,#169391,#169392,#169393,
#169394,#169395,#169396),(#169397,#169398,#169399,#169400,#169401,#169402,
#169403,#169404,#169405),(#169406,#169407,#169408,#169409,#169410,#169411,
#169412,#169413,#169414),(#169415,#169416,#169417,#169418,#169419,#169420,
#169421,#169422,#169423),(#169424,#169425,#169426,#169427,#169428,#169429,
#169430,#169431,#169432),(#169433,#169434,#169435,#169436,#169437,#169438,
#169439,#169440,#169441),(#169442,#169443,#169444,#169445,#169446,#169447,
#169448,#169449,#169450),(#169451,#169452,#169453,#169454,#169455,#169456,
#169457,#169458,#169459),(#169460,#169461,#169462,#169463,#169464,#169465,
#169466,#169467,#169468),(#169469,#169470,#169471,#169472,#169473,#169474,
#169475,#169476,#169477),(#169478,#169479,#169480,#169481,#169482,#169483,
#169484,#169485,#169486),(#169487,#169488,#169489,#169490,#169491,#169492,
#169493,#169494,#169495),(#169496,#169497,#169498,#169499,#169500,#169501,
#169502,#169503,#169504),(#169505,#169506,#169507,#169508,#169509,#169510,
#169511,#169512,#169513),(#169514,#169515,#169516,#169517,#169518,#169519,
#169520,#169521,#169522),(#169523,#169524,#169525,#169526,#169527,#169528,
#169529,#169530,#169531),(#169532,#169533,#169534,#169535,#169536,#169537,
#169538,#169539,#169540),(#169541,#169542,#169543,#169544,#169545,#169546,
#169547,#169548,#169549),(#169550,#169551,#169552,#169553,#169554,#169555,
#169556,#169557,#169558),(#169559,#169560,#169561,#169562,#169563,#169564,
#169565,#169566,#169567),(#169568,#169569,#169570,#169571,#169572,#169573,
#169574,#169575,#169576),(#169577,#169578,#169579,#169580,#169581,#169582,
#169583,#169584,#169585),(#169586,#169587,#169588,#169589,#169590,#169591,
#169592,#169593,#169594),(#169595,#169596,#169597,#169598,#169599,#169600,
#169601,#169602,#169603),(#169604,#169605,#169606,#169607,#169608,#169609,
#169610,#169611,#169612),(#169613,#169614,#169615,#169616,#169617,#169618,
#169619,#169620,#169621),(#169622,#169623,#169624,#169625,#169626,#169627,
#169628,#169629,#169630),(#169631,#169632,#169633,#169634,#169635,#169636,
#169637,#169638,#169639),(#169640,#169641,#169642,#169643,#169644,#169645,
#169646,#169647,#169648),(#169649,#169650,#169651,#169652,#169653,#169654,
#169655,#169656,#169657),(#169658,#169659,#169660,#169661,#169662,#169663,
#169664,#169665,#169666),(#169667,#169668,#169669,#169670,#169671,#169672,
#169673,#169674,#169675),(#169676,#169677,#169678,#169679,#169680,#169681,
#169682,#169683,#169684),(#169685,#169686,#169687,#169688,#169689,#169690,
#169691,#169692,#169693),(#169694,#169695,#169696,#169697,#169698,#169699,
#169700,#169701,#169702),(#169703,#169704,#169705,#169706,#169707,#169708,
#169709,#169710,#169711),(#169712,#169713,#169714,#169715,#169716,#169717,
#169718,#169719,#169720),(#169721,#169722,#169723,#169724,#169725,#169726,
#169727,#169728,#169729),(#169730,#169731,#169732,#169733,#169734,#169735,
#169736,#169737,#169738),(#169739,#169740,#169741,#169742,#169743,#169744,
#169745,#169746,#169747),(#169748,#169749,#169750,#169751,#169752,#169753,
#169754,#169755,#169756),(#169757,#169758,#169759,#169760,#169761,#169762,
#169763,#169764,#169765),(#169766,#169767,#169768,#169769,#169770,#169771,
#169772,#169773,#169774),(#169775,#169776,#169777,#169778,#169779,#169780,
#169781,#169782,#169783),(#169784,#169785,#169786,#169787,#169788,#169789,
#169790,#169791,#169792),(#169793,#169794,#169795,#169796,#169797,#169798,
#169799,#169800,#169801),(#169802,#169803,#169804,#169805,#169806,#169807,
#169808,#169809,#169810),(#169811,#169812,#169813,#169814,#169815,#169816,
#169817,#169818,#169819),(#169820,#169821,#169822,#169823,#169824,#169825,
#169826,#169827,#169828),(#169829,#169830,#169831,#169832,#169833,#169834,
#169835,#169836,#169837),(#169838,#169839,#169840,#169841,#169842,#169843,
#169844,#169845,#169846),(#169847,#169848,#169849,#169850,#169851,#169852,
#169853,#169854,#169855),(#169856,#169857,#169858,#169859,#169860,#169861,
#169862,#169863,#169864),(#169865,#169866,#169867,#169868,#169869,#169870,
#169871,#169872,#169873),(#169874,#169875,#169876,#169877,#169878,#169879,
#169880,#169881,#169882),(#169883,#169884,#169885,#169886,#169887,#169888,
#169889,#169890,#169891),(#169892,#169893,#169894,#169895,#169896,#169897,
#169898,#169899,#169900),(#169901,#169902,#169903,#169904,#169905,#169906,
#169907,#169908,#169909),(#169910,#169911,#169912,#169913,#169914,#169915,
#169916,#169917,#169918),(#169919,#169920,#169921,#169922,#169923,#169924,
#169925,#169926,#169927),(#169928,#169929,#169930,#169931,#169932,#169933,
#169934,#169935,#169936),(#169937,#169938,#169939,#169940,#169941,#169942,
#169943,#169944,#169945),(#169946,#169947,#169948,#169949,#169950,#169951,
#169952,#169953,#169954),(#169955,#169956,#169957,#169958,#169959,#169960,
#169961,#169962,#169963),(#169964,#169965,#169966,#169967,#169968,#169969,
#169970,#169971,#169972),(#169973,#169974,#169975,#169976,#169977,#169978,
#169979,#169980,#169981),(#169982,#169983,#169984,#169985,#169986,#169987,
#169988,#169989,#169990),(#169991,#169992,#169993,#169994,#169995,#169996,
#169997,#169998,#169999),(#170000,#170001,#170002,#170003,#170004,#170005,
#170006,#170007,#170008),(#170009,#170010,#170011,#170012,#170013,#170014,
#170015,#170016,#170017),(#170018,#170019,#170020,#170021,#170022,#170023,
#170024,#170025,#170026),(#170027,#170028,#170029,#170030,#170031,#170032,
#170033,#170034,#170035),(#170036,#170037,#170038,#170039,#170040,#170041,
#170042,#170043,#170044),(#170045,#170046,#170047,#170048,#170049,#170050,
#170051,#170052,#170053),(#170054,#170055,#170056,#170057,#170058,#170059,
#170060,#170061,#170062),(#170063,#170064,#170065,#170066,#170067,#170068,
#170069,#170070,#170071),(#170072,#170073,#170074,#170075,#170076,#170077,
#170078,#170079,#170080),(#170081,#170082,#170083,#170084,#170085,#170086,
#170087,#170088,#170089),(#170090,#170091,#170092,#170093,#170094,#170095,
#170096,#170097,#170098),(#170099,#170100,#170101,#170102,#170103,#170104,
#170105,#170106,#170107),(#170108,#170109,#170110,#170111,#170112,#170113,
#170114,#170115,#170116),(#170117,#170118,#170119,#170120,#170121,#170122,
#170123,#170124,#170125),(#170126,#170127,#170128,#170129,#170130,#170131,
#170132,#170133,#170134),(#170135,#170136,#170137,#170138,#170139,#170140,
#170141,#170142,#170143),(#170144,#170145,#170146,#170147,#170148,#170149,
#170150,#170151,#170152),(#170153,#170154,#170155,#170156,#170157,#170158,
#170159,#170160,#170161),(#170162,#170163,#170164,#170165,#170166,#170167,
#170168,#170169,#170170),(#170171,#170172,#170173,#170174,#170175,#170176,
#170177,#170178,#170179),(#170180,#170181,#170182,#170183,#170184,#170185,
#170186,#170187,#170188),(#170189,#170190,#170191,#170192,#170193,#170194,
#170195,#170196,#170197),(#170198,#170199,#170200,#170201,#170202,#170203,
#170204,#170205,#170206),(#170207,#170208,#170209,#170210,#170211,#170212,
#170213,#170214,#170215),(#170216,#170217,#170218,#170219,#170220,#170221,
#170222,#170223,#170224),(#170225,#170226,#170227,#170228,#170229,#170230,
#170231,#170232,#170233),(#170234,#170235,#170236,#170237,#170238,#170239,
#170240,#170241,#170242),(#170243,#170244,#170245,#170246,#170247,#170248,
#170249,#170250,#170251),(#170252,#170253,#170254,#170255,#170256,#170257,
#170258,#170259,#170260),(#170261,#170262,#170263,#170264,#170265,#170266,
#170267,#170268,#170269),(#170270,#170271,#170272,#170273,#170274,#170275,
#170276,#170277,#170278),(#170279,#170280,#170281,#170282,#170283,#170284,
#170285,#170286,#170287),(#170288,#170289,#170290,#170291,#170292,#170293,
#170294,#170295,#170296),(#170297,#170298,#170299,#170300,#170301,#170302,
#170303,#170304,#170305),(#170306,#170307,#170308,#170309,#170310,#170311,
#170312,#170313,#170314),(#170315,#170316,#170317,#170318,#170319,#170320,
#170321,#170322,#170323),(#170324,#170325,#170326,#170327,#170328,#170329,
#170330,#170331,#170332),(#170333,#170334,#170335,#170336,#170337,#170338,
#170339,#170340,#170341),(#170342,#170343,#170344,#170345,#170346,#170347,
#170348,#170349,#170350),(#170351,#170352,#170353,#170354,#170355,#170356,
#170357,#170358,#170359),(#170360,#170361,#170362,#170363,#170364,#170365,
#170366,#170367,#170368),(#170369,#170370,#170371,#170372,#170373,#170374,
#170375,#170376,#170377),(#170378,#170379,#170380,#170381,#170382,#170383,
#170384,#170385,#170386),(#170387,#170388,#170389,#170390,#170391,#170392,
#170393,#170394,#170395),(#170396,#170397,#170398,#170399,#170400,#170401,
#170402,#170403,#170404),(#170405,#170406,#170407,#170408,#170409,#170410,
#170411,#170412,#170413),(#170414,#170415,#170416,#170417,#170418,#170419,
#170420,#170421,#170422),(#170423,#170424,#170425,#170426,#170427,#170428,
#170429,#170430,#170431),(#170432,#170433,#170434,#170435,#170436,#170437,
#170438,#170439,#170440),(#170441,#170442,#170443,#170444,#170445,#170446,
#170447,#170448,#170449),(#170450,#170451,#170452,#170453,#170454,#170455,
#170456,#170457,#170458),(#170459,#170460,#170461,#170462,#170463,#170464,
#170465,#170466,#170467),(#170468,#170469,#170470,#170471,#170472,#170473,
#170474,#170475,#170476),(#170477,#170478,#170479,#170480,#170481,#170482,
#170483,#170484,#170485),(#170486,#170487,#170488,#170489,#170490,#170491,
#170492,#170493,#170494),(#170495,#170496,#170497,#170498,#170499,#170500,
#170501,#170502,#170503),(#170504,#170505,#170506,#170507,#170508,#170509,
#170510,#170511,#170512),(#170513,#170514,#170515,#170516,#170517,#170518,
#170519,#170520,#170521),(#170522,#170523,#170524,#170525,#170526,#170527,
#170528,#170529,#170530),(#170531,#170532,#170533,#170534,#170535,#170536,
#170537,#170538,#170539),(#170540,#170541,#170542,#170543,#170544,#170545,
#170546,#170547,#170548),(#170549,#170550,#170551,#170552,#170553,#170554,
#170555,#170556,#170557),(#170558,#170559,#170560,#170561,#170562,#170563,
#170564,#170565,#170566),(#170567,#170568,#170569,#170570,#170571,#170572,
#170573,#170574,#170575),(#170576,#170577,#170578,#170579,#170580,#170581,
#170582,#170583,#170584),(#170585,#170586,#170587,#170588,#170589,#170590,
#170591,#170592,#170593),(#170594,#170595,#170596,#170597,#170598,#170599,
#170600,#170601,#170602),(#170603,#170604,#170605,#170606,#170607,#170608,
#170609,#170610,#170611),(#170612,#170613,#170614,#170615,#170616,#170617,
#170618,#170619,#170620),(#170621,#170622,#170623,#170624,#170625,#170626,
#170627,#170628,#170629),(#170630,#170631,#170632,#170633,#170634,#170635,
#170636,#170637,#170638),(#170639,#170640,#170641,#170642,#170643,#170644,
#170645,#170646,#170647),(#170648,#170649,#170650,#170651,#170652,#170653,
#170654,#170655,#170656),(#170657,#170658,#170659,#170660,#170661,#170662,
#170663,#170664,#170665),(#170666,#170667,#170668,#170669,#170670,#170671,
#170672,#170673,#170674),(#170675,#170676,#170677,#170678,#170679,#170680,
#170681,#170682,#170683),(#170684,#170685,#170686,#170687,#170688,#170689,
#170690,#170691,#170692),(#170693,#170694,#170695,#170696,#170697,#170698,
#170699,#170700,#170701),(#170702,#170703,#170704,#170705,#170706,#170707,
#170708,#170709,#170710),(#170711,#170712,#170713,#170714,#170715,#170716,
#170717,#170718,#170719),(#170720,#170721,#170722,#170723,#170724,#170725,
#170726,#170727,#170728),(#170729,#170730,#170731,#170732,#170733,#170734,
#170735,#170736,#170737),(#170738,#170739,#170740,#170741,#170742,#170743,
#170744,#170745,#170746),(#170747,#170748,#170749,#170750,#170751,#170752,
#170753,#170754,#170755),(#170756,#170757,#170758,#170759,#170760,#170761,
#170762,#170763,#170764),(#170765,#170766,#170767,#170768,#170769,#170770,
#170771,#170772,#170773),(#170774,#170775,#170776,#170777,#170778,#170779,
#170780,#170781,#170782),(#170783,#170784,#170785,#170786,#170787,#170788,
#170789,#170790,#170791),(#170792,#170793,#170794,#170795,#170796,#170797,
#170798,#170799,#170800),(#170801,#170802,#170803,#170804,#170805,#170806,
#170807,#170808,#170809),(#170810,#170811,#170812,#170813,#170814,#170815,
#170816,#170817,#170818),(#170819,#170820,#170821,#170822,#170823,#170824,
#170825,#170826,#170827),(#170828,#170829,#170830,#170831,#170832,#170833,
#170834,#170835,#170836),(#170837,#170838,#170839,#170840,#170841,#170842,
#170843,#170844,#170845),(#170846,#170847,#170848,#170849,#170850,#170851,
#170852,#170853,#170854),(#170855,#170856,#170857,#170858,#170859,#170860,
#170861,#170862,#170863),(#170864,#170865,#170866,#170867,#170868,#170869,
#170870,#170871,#170872),(#170873,#170874,#170875,#170876,#170877,#170878,
#170879,#170880,#170881),(#170882,#170883,#170884,#170885,#170886,#170887,
#170888,#170889,#170890),(#170891,#170892,#170893,#170894,#170895,#170896,
#170897,#170898,#170899),(#170900,#170901,#170902,#170903,#170904,#170905,
#170906,#170907,#170908),(#170909,#170910,#170911,#170912,#170913,#170914,
#170915,#170916,#170917),(#170918,#170919,#170920,#170921,#170922,#170923,
#170924,#170925,#170926),(#170927,#170928,#170929,#170930,#170931,#170932,
#170933,#170934,#170935),(#170936,#170937,#170938,#170939,#170940,#170941,
#170942,#170943,#170944),(#170945,#170946,#170947,#170948,#170949,#170950,
#170951,#170952,#170953),(#170954,#170955,#170956,#170957,#170958,#170959,
#170960,#170961,#170962),(#170963,#170964,#170965,#170966,#170967,#170968,
#170969,#170970,#170971),(#170972,#170973,#170974,#170975,#170976,#170977,
#170978,#170979,#170980),(#170981,#170982,#170983,#170984,#170985,#170986,
#170987,#170988,#170989),(#170990,#170991,#170992,#170993,#170994,#170995,
#170996,#170997,#170998),(#170999,#171000,#171001,#171002,#171003,#171004,
#171005,#171006,#171007),(#171008,#171009,#171010,#171011,#171012,#171013,
#171014,#171015,#171016),(#171017,#171018,#171019,#171020,#171021,#171022,
#171023,#171024,#171025),(#171026,#171027,#171028,#171029,#171030,#171031,
#171032,#171033,#171034),(#171035,#171036,#171037,#171038,#171039,#171040,
#171041,#171042,#171043),(#171044,#171045,#171046,#171047,#171048,#171049,
#171050,#171051,#171052),(#171053,#171054,#171055,#171056,#171057,#171058,
#171059,#171060,#171061),(#171062,#171063,#171064,#171065,#171066,#171067,
#171068,#171069,#171070),(#171071,#171072,#171073,#171074,#171075,#171076,
#171077,#171078,#171079),(#171080,#171081,#171082,#171083,#171084,#171085,
#171086,#171087,#171088),(#171089,#171090,#171091,#171092,#171093,#171094,
#171095,#171096,#171097),(#171098,#171099,#171100,#171101,#171102,#171103,
#171104,#171105,#171106),(#171107,#171108,#171109,#171110,#171111,#171112,
#171113,#171114,#171115),(#171116,#171117,#171118,#171119,#171120,#171121,
#171122,#171123,#171124),(#171125,#171126,#171127,#171128,#171129,#171130,
#171131,#171132,#171133),(#171134,#171135,#171136,#171137,#171138,#171139,
#171140,#171141,#171142),(#171143,#171144,#171145,#171146,#171147,#171148,
#171149,#171150,#171151),(#171152,#171153,#171154,#171155,#171156,#171157,
#171158,#171159,#171160),(#171161,#171162,#171163,#171164,#171165,#171166,
#171167,#171168,#171169),(#171170,#171171,#171172,#171173,#171174,#171175,
#171176,#171177,#171178),(#171179,#171180,#171181,#171182,#171183,#171184,
#171185,#171186,#171187),(#171188,#171189,#171190,#171191,#171192,#171193,
#171194,#171195,#171196),(#171197,#171198,#171199,#171200,#171201,#171202,
#171203,#171204,#171205),(#171206,#171207,#171208,#171209,#171210,#171211,
#171212,#171213,#171214),(#171215,#171216,#171217,#171218,#171219,#171220,
#171221,#171222,#171223),(#171224,#171225,#171226,#171227,#171228,#171229,
#171230,#171231,#171232),(#171233,#171234,#171235,#171236,#171237,#171238,
#171239,#171240,#171241),(#171242,#171243,#171244,#171245,#171246,#171247,
#171248,#171249,#171250),(#171251,#171252,#171253,#171254,#171255,#171256,
#171257,#171258,#171259),(#171260,#171261,#171262,#171263,#171264,#171265,
#171266,#171267,#171268),(#171269,#171270,#171271,#171272,#171273,#171274,
#171275,#171276,#171277),(#171278,#171279,#171280,#171281,#171282,#171283,
#171284,#171285,#171286),(#171287,#171288,#171289,#171290,#171291,#171292,
#171293,#171294,#171295),(#171296,#171297,#171298,#171299,#171300,#171301,
#171302,#171303,#171304),(#171305,#171306,#171307,#171308,#171309,#171310,
#171311,#171312,#171313),(#171314,#171315,#171316,#171317,#171318,#171319,
#171320,#171321,#171322),(#171323,#171324,#171325,#171326,#171327,#171328,
#171329,#171330,#171331),(#171332,#171333,#171334,#171335,#171336,#171337,
#171338,#171339,#171340),(#171341,#171342,#171343,#171344,#171345,#171346,
#171347,#171348,#171349),(#171350,#171351,#171352,#171353,#171354,#171355,
#171356,#171357,#171358),(#171359,#171360,#171361,#171362,#171363,#171364,
#171365,#171366,#171367),(#171368,#171369,#171370,#171371,#171372,#171373,
#171374,#171375,#171376),(#171377,#171378,#171379,#171380,#171381,#171382,
#171383,#171384,#171385),(#171386,#171387,#171388,#171389,#171390,#171391,
#171392,#171393,#171394),(#171395,#171396,#171397,#171398,#171399,#171400,
#171401,#171402,#171403),(#171404,#171405,#171406,#171407,#171408,#171409,
#171410,#171411,#171412),(#171413,#171414,#171415,#171416,#171417,#171418,
#171419,#171420,#171421),(#171422,#171423,#171424,#171425,#171426,#171427,
#171428,#171429,#171430),(#171431,#171432,#171433,#171434,#171435,#171436,
#171437,#171438,#171439),(#171440,#171441,#171442,#171443,#171444,#171445,
#171446,#171447,#171448),(#171449,#171450,#171451,#171452,#171453,#171454,
#171455,#171456,#171457),(#171458,#171459,#171460,#171461,#171462,#171463,
#171464,#171465,#171466),(#171467,#171468,#171469,#171470,#171471,#171472,
#171473,#171474,#171475),(#171476,#171477,#171478,#171479,#171480,#171481,
#171482,#171483,#171484),(#171485,#171486,#171487,#171488,#171489,#171490,
#171491,#171492,#171493),(#171494,#171495,#171496,#171497,#171498,#171499,
#171500,#171501,#171502),(#171503,#171504,#171505,#171506,#171507,#171508,
#171509,#171510,#171511),(#171512,#171513,#171514,#171515,#171516,#171517,
#171518,#171519,#171520),(#171521,#171522,#171523,#171524,#171525,#171526,
#171527,#171528,#171529),(#171530,#171531,#171532,#171533,#171534,#171535,
#171536,#171537,#171538),(#171539,#171540,#171541,#171542,#171543,#171544,
#171545,#171546,#171547),(#171548,#171549,#171550,#171551,#171552,#171553,
#171554,#171555,#171556),(#171557,#171558,#171559,#171560,#171561,#171562,
#171563,#171564,#171565),(#171566,#171567,#171568,#171569,#171570,#171571,
#171572,#171573,#171574),(#171575,#171576,#171577,#171578,#171579,#171580,
#171581,#171582,#171583),(#171584,#171585,#171586,#171587,#171588,#171589,
#171590,#171591,#171592),(#171593,#171594,#171595,#171596,#171597,#171598,
#171599,#171600,#171601),(#171602,#171603,#171604,#171605,#171606,#171607,
#171608,#171609,#171610),(#171611,#171612,#171613,#171614,#171615,#171616,
#171617,#171618,#171619),(#171620,#171621,#171622,#171623,#171624,#171625,
#171626,#171627,#171628),(#171629,#171630,#171631,#171632,#171633,#171634,
#171635,#171636,#171637),(#171638,#171639,#171640,#171641,#171642,#171643,
#171644,#171645,#171646),(#171647,#171648,#171649,#171650,#171651,#171652,
#171653,#171654,#171655),(#171656,#171657,#171658,#171659,#171660,#171661,
#171662,#171663,#171664),(#171665,#171666,#171667,#171668,#171669,#171670,
#171671,#171672,#171673),(#171674,#171675,#171676,#171677,#171678,#171679,
#171680,#171681,#171682),(#171683,#171684,#171685,#171686,#171687,#171688,
#171689,#171690,#171691),(#171692,#171693,#171694,#171695,#171696,#171697,
#171698,#171699,#171700),(#171701,#171702,#171703,#171704,#171705,#171706,
#171707,#171708,#171709),(#171710,#171711,#171712,#171713,#171714,#171715,
#171716,#171717,#171718),(#171719,#171720,#171721,#171722,#171723,#171724,
#171725,#171726,#171727),(#171728,#171729,#171730,#171731,#171732,#171733,
#171734,#171735,#171736),(#171737,#171738,#171739,#171740,#171741,#171742,
#171743,#171744,#171745),(#171746,#171747,#171748,#171749,#171750,#171751,
#171752,#171753,#171754),(#171755,#171756,#171757,#171758,#171759,#171760,
#171761,#171762,#171763),(#171764,#171765,#171766,#171767,#171768,#171769,
#171770,#171771,#171772),(#171773,#171774,#171775,#171776,#171777,#171778,
#171779,#171780,#171781),(#171782,#171783,#171784,#171785,#171786,#171787,
#171788,#171789,#171790),(#171791,#171792,#171793,#171794,#171795,#171796,
#171797,#171798,#171799),(#171800,#171801,#171802,#171803,#171804,#171805,
#171806,#171807,#171808),(#171809,#171810,#171811,#171812,#171813,#171814,
#171815,#171816,#171817),(#171818,#171819,#171820,#171821,#171822,#171823,
#171824,#171825,#171826),(#171827,#171828,#171829,#171830,#171831,#171832,
#171833,#171834,#171835),(#171836,#171837,#171838,#171839,#171840,#171841,
#171842,#171843,#171844),(#171845,#171846,#171847,#171848,#171849,#171850,
#171851,#171852,#171853),(#171854,#171855,#171856,#171857,#171858,#171859,
#171860,#171861,#171862),(#171863,#171864,#171865,#171866,#171867,#171868,
#171869,#171870,#171871),(#171872,#171873,#171874,#171875,#171876,#171877,
#171878,#171879,#171880),(#171881,#171882,#171883,#171884,#171885,#171886,
#171887,#171888,#171889),(#171890,#171891,#171892,#171893,#171894,#171895,
#171896,#171897,#171898),(#171899,#171900,#171901,#171902,#171903,#171904,
#171905,#171906,#171907),(#171908,#171909,#171910,#171911,#171912,#171913,
#171914,#171915,#171916),(#171917,#171918,#171919,#171920,#171921,#171922,
#171923,#171924,#171925),(#171926,#171927,#171928,#171929,#171930,#171931,
#171932,#171933,#171934),(#171935,#171936,#171937,#171938,#171939,#171940,
#171941,#171942,#171943),(#171944,#171945,#171946,#171947,#171948,#171949,
#171950,#171951,#171952),(#171953,#171954,#171955,#171956,#171957,#171958,
#171959,#171960,#171961),(#171962,#171963,#171964,#171965,#171966,#171967,
#171968,#171969,#171970),(#171971,#171972,#171973,#171974,#171975,#171976,
#171977,#171978,#171979),(#171980,#171981,#171982,#171983,#171984,#171985,
#171986,#171987,#171988),(#171989,#171990,#171991,#171992,#171993,#171994,
#171995,#171996,#171997),(#171998,#171999,#172000,#172001,#172002,#172003,
#172004,#172005,#172006),(#172007,#172008,#172009,#172010,#172011,#172012,
#172013,#172014,#172015),(#172016,#172017,#172018,#172019,#172020,#172021,
#172022,#172023,#172024),(#172025,#172026,#172027,#172028,#172029,#172030,
#172031,#172032,#172033),(#172034,#172035,#172036,#172037,#172038,#172039,
#172040,#172041,#172042),(#172043,#172044,#172045,#172046,#172047,#172048,
#172049,#172050,#172051),(#172052,#172053,#172054,#172055,#172056,#172057,
#172058,#172059,#172060),(#172061,#172062,#172063,#172064,#172065,#172066,
#172067,#172068,#172069),(#172070,#172071,#172072,#172073,#172074,#172075,
#172076,#172077,#172078),(#172079,#172080,#172081,#172082,#172083,#172084,
#172085,#172086,#172087),(#172088,#172089,#172090,#172091,#172092,#172093,
#172094,#172095,#172096),(#172097,#172098,#172099,#172100,#172101,#172102,
#172103,#172104,#172105),(#172106,#172107,#172108,#172109,#172110,#172111,
#172112,#172113,#172114),(#172115,#172116,#172117,#172118,#172119,#172120,
#172121,#172122,#172123),(#172124,#172125,#172126,#172127,#172128,#172129,
#172130,#172131,#172132),(#172133,#172134,#172135,#172136,#172137,#172138,
#172139,#172140,#172141),(#172142,#172143,#172144,#172145,#172146,#172147,
#172148,#172149,#172150),(#172151,#172152,#172153,#172154,#172155,#172156,
#172157,#172158,#172159),(#172160,#172161,#172162,#172163,#172164,#172165,
#172166,#172167,#172168),(#172169,#172170,#172171,#172172,#172173,#172174,
#172175,#172176,#172177),(#172178,#172179,#172180,#172181,#172182,#172183,
#172184,#172185,#172186),(#172187,#172188,#172189,#172190,#172191,#172192,
#172193,#172194,#172195),(#172196,#172197,#172198,#172199,#172200,#172201,
#172202,#172203,#172204),(#172205,#172206,#172207,#172208,#172209,#172210,
#172211,#172212,#172213),(#172214,#172215,#172216,#172217,#172218,#172219,
#172220,#172221,#172222),(#172223,#172224,#172225,#172226,#172227,#172228,
#172229,#172230,#172231),(#172232,#172233,#172234,#172235,#172236,#172237,
#172238,#172239,#172240),(#172241,#172242,#172243,#172244,#172245,#172246,
#172247,#172248,#172249),(#172250,#172251,#172252,#172253,#172254,#172255,
#172256,#172257,#172258),(#172259,#172260,#172261,#172262,#172263,#172264,
#172265,#172266,#172267),(#172268,#172269,#172270,#172271,#172272,#172273,
#172274,#172275,#172276),(#172277,#172278,#172279,#172280,#172281,#172282,
#172283,#172284,#172285),(#172286,#172287,#172288,#172289,#172290,#172291,
#172292,#172293,#172294),(#172295,#172296,#172297,#172298,#172299,#172300,
#172301,#172302,#172303),(#172304,#172305,#172306,#172307,#172308,#172309,
#172310,#172311,#172312),(#172313,#172314,#172315,#172316,#172317,#172318,
#172319,#172320,#172321),(#172322,#172323,#172324,#172325,#172326,#172327,
#172328,#172329,#172330),(#172331,#172332,#172333,#172334,#172335,#172336,
#172337,#172338,#172339),(#172340,#172341,#172342,#172343,#172344,#172345,
#172346,#172347,#172348),(#172349,#172350,#172351,#172352,#172353,#172354,
#172355,#172356,#172357),(#172358,#172359,#172360,#172361,#172362,#172363,
#172364,#172365,#172366),(#172367,#172368,#172369,#172370,#172371,#172372,
#172373,#172374,#172375),(#172376,#172377,#172378,#172379,#172380,#172381,
#172382,#172383,#172384),(#172385,#172386,#172387,#172388,#172389,#172390,
#172391,#172392,#172393),(#172394,#172395,#172396,#172397,#172398,#172399,
#172400,#172401,#172402),(#172403,#172404,#172405,#172406,#172407,#172408,
#172409,#172410,#172411),(#172412,#172413,#172414,#172415,#172416,#172417,
#172418,#172419,#172420),(#172421,#172422,#172423,#172424,#172425,#172426,
#172427,#172428,#172429),(#172430,#172431,#172432,#172433,#172434,#172435,
#172436,#172437,#172438),(#172439,#172440,#172441,#172442,#172443,#172444,
#172445,#172446,#172447),(#172448,#172449,#172450,#172451,#172452,#172453,
#172454,#172455,#172456),(#172457,#172458,#172459,#172460,#172461,#172462,
#172463,#172464,#172465),(#172466,#172467,#172468,#172469,#172470,#172471,
#172472,#172473,#172474),(#172475,#172476,#172477,#172478,#172479,#172480,
#172481,#172482,#172483),(#172484,#172485,#172486,#172487,#172488,#172489,
#172490,#172491,#172492),(#172493,#172494,#172495,#172496,#172497,#172498,
#172499,#172500,#172501),(#172502,#172503,#172504,#172505,#172506,#172507,
#172508,#172509,#172510),(#172511,#172512,#172513,#172514,#172515,#172516,
#172517,#172518,#172519),(#172520,#172521,#172522,#172523,#172524,#172525,
#172526,#172527,#172528),(#172529,#172530,#172531,#172532,#172533,#172534,
#172535,#172536,#172537),(#172538,#172539,#172540,#172541,#172542,#172543,
#172544,#172545,#172546),(#172547,#172548,#172549,#172550,#172551,#172552,
#172553,#172554,#172555),(#172556,#172557,#172558,#172559,#172560,#172561,
#172562,#172563,#172564),(#172565,#172566,#172567,#172568,#172569,#172570,
#172571,#172572,#172573),(#172574,#172575,#172576,#172577,#172578,#172579,
#172580,#172581,#172582),(#172583,#172584,#172585,#172586,#172587,#172588,
#172589,#172590,#172591),(#172592,#172593,#172594,#172595,#172596,#172597,
#172598,#172599,#172600),(#172601,#172602,#172603,#172604,#172605,#172606,
#172607,#172608,#172609),(#172610,#172611,#172612,#172613,#172614,#172615,
#172616,#172617,#172618),(#172619,#172620,#172621,#172622,#172623,#172624,
#172625,#172626,#172627),(#172628,#172629,#172630,#172631,#172632,#172633,
#172634,#172635,#172636),(#172637,#172638,#172639,#172640,#172641,#172642,
#172643,#172644,#172645),(#172646,#172647,#172648,#172649,#172650,#172651,
#172652,#172653,#172654),(#172655,#172656,#172657,#172658,#172659,#172660,
#172661,#172662,#172663),(#172664,#172665,#172666,#172667,#172668,#172669,
#172670,#172671,#172672),(#172673,#172674,#172675,#172676,#172677,#172678,
#172679,#172680,#172681),(#172682,#172683,#172684,#172685,#172686,#172687,
#172688,#172689,#172690),(#172691,#172692,#172693,#172694,#172695,#172696,
#172697,#172698,#172699),(#172700,#172701,#172702,#172703,#172704,#172705,
#172706,#172707,#172708),(#172709,#172710,#172711,#172712,#172713,#172714,
#172715,#172716,#172717),(#172718,#172719,#172720,#172721,#172722,#172723,
#172724,#172725,#172726),(#172727,#172728,#172729,#172730,#172731,#172732,
#172733,#172734,#172735),(#172736,#172737,#172738,#172739,#172740,#172741,
#172742,#172743,#172744),(#172745,#172746,#172747,#172748,#172749,#172750,
#172751,#172752,#172753),(#172754,#172755,#172756,#172757,#172758,#172759,
#172760,#172761,#172762),(#172763,#172764,#172765,#172766,#172767,#172768,
#172769,#172770,#172771),(#172772,#172773,#172774,#172775,#172776,#172777,
#172778,#172779,#172780),(#172781,#172782,#172783,#172784,#172785,#172786,
#172787,#172788,#172789),(#172790,#172791,#172792,#172793,#172794,#172795,
#172796,#172797,#172798),(#172799,#172800,#172801,#172802,#172803,#172804,
#172805,#172806,#172807),(#172808,#172809,#172810,#172811,#172812,#172813,
#172814,#172815,#172816),(#172817,#172818,#172819,#172820,#172821,#172822,
#172823,#172824,#172825),(#172826,#172827,#172828,#172829,#172830,#172831,
#172832,#172833,#172834),(#172835,#172836,#172837,#172838,#172839,#172840,
#172841,#172842,#172843),(#172844,#172845,#172846,#172847,#172848,#172849,
#172850,#172851,#172852),(#172853,#172854,#172855,#172856,#172857,#172858,
#172859,#172860,#172861),(#172862,#172863,#172864,#172865,#172866,#172867,
#172868,#172869,#172870),(#172871,#172872,#172873,#172874,#172875,#172876,
#172877,#172878,#172879),(#172880,#172881,#172882,#172883,#172884,#172885,
#172886,#172887,#172888),(#172889,#172890,#172891,#172892,#172893,#172894,
#172895,#172896,#172897),(#172898,#172899,#172900,#172901,#172902,#172903,
#172904,#172905,#172906),(#172907,#172908,#172909,#172910,#172911,#172912,
#172913,#172914,#172915),(#172916,#172917,#172918,#172919,#172920,#172921,
#172922,#172923,#172924),(#172925,#172926,#172927,#172928,#172929,#172930,
#172931,#172932,#172933),(#172934,#172935,#172936,#172937,#172938,#172939,
#172940,#172941,#172942),(#172943,#172944,#172945,#172946,#172947,#172948,
#172949,#172950,#172951),(#172952,#172953,#172954,#172955,#172956,#172957,
#172958,#172959,#172960),(#172961,#172962,#172963,#172964,#172965,#172966,
#172967,#172968,#172969),(#172970,#172971,#172972,#172973,#172974,#172975,
#172976,#172977,#172978),(#172979,#172980,#172981,#172982,#172983,#172984,
#172985,#172986,#172987),(#172988,#172989,#172990,#172991,#172992,#172993,
#172994,#172995,#172996),(#172997,#172998,#172999,#173000,#173001,#173002,
#173003,#173004,#173005),(#173006,#173007,#173008,#173009,#173010,#173011,
#173012,#173013,#173014),(#173015,#173016,#173017,#173018,#173019,#173020,
#173021,#173022,#173023),(#173024,#173025,#173026,#173027,#173028,#173029,
#173030,#173031,#173032),(#173033,#173034,#173035,#173036,#173037,#173038,
#173039,#173040,#173041),(#173042,#173043,#173044,#173045,#173046,#173047,
#173048,#173049,#173050),(#173051,#173052,#173053,#173054,#173055,#173056,
#173057,#173058,#173059),(#173060,#173061,#173062,#173063,#173064,#173065,
#173066,#173067,#173068),(#173069,#173070,#173071,#173072,#173073,#173074,
#173075,#173076,#173077),(#173078,#173079,#173080,#173081,#173082,#173083,
#173084,#173085,#173086),(#173087,#173088,#173089,#173090,#173091,#173092,
#173093,#173094,#173095),(#173096,#173097,#173098,#173099,#173100,#173101,
#173102,#173103,#173104),(#173105,#173106,#173107,#173108,#173109,#173110,
#173111,#173112,#173113),(#173114,#173115,#173116,#173117,#173118,#173119,
#173120,#173121,#173122),(#173123,#173124,#173125,#173126,#173127,#173128,
#173129,#173130,#173131),(#173132,#173133,#173134,#173135,#173136,#173137,
#173138,#173139,#173140),(#173141,#173142,#173143,#173144,#173145,#173146,
#173147,#173148,#173149),(#173150,#173151,#173152,#173153,#173154,#173155,
#173156,#173157,#173158),(#173159,#173160,#173161,#173162,#173163,#173164,
#173165,#173166,#173167),(#173168,#173169,#173170,#173171,#173172,#173173,
#173174,#173175,#173176),(#173177,#173178,#173179,#173180,#173181,#173182,
#173183,#173184,#173185),(#173186,#173187,#173188,#173189,#173190,#173191,
#173192,#173193,#173194)),.UNSPECIFIED.,.F.,.T.,.F.)
B_SPLINE_SURFACE_WITH_KNOTS((4,1,1,1,1,1,1,1,1,1,1,1,1,1,1,1,1,1,1,1,1,
1,1,1,1,1,1,1,1,1,1,1,1,1,1,1,1,1,1,1,1,1,1,1,1,1,1,1,1,1,1,1,1,1,1,1,1,
1,1,1,1,1,1,1,1,1,1,1,1,1,1,1,1,1,1,1,1,1,1,1,1,1,1,1,1,1,1,1,1,1,1,1,1,
1,1,1,1,1,1,1,1,1,1,1,1,1,1,1,1,1,1,1,1,1,1,1,1,1,1,1,1,1,1,1,1,1,1,1,1,
1,1,1,1,1,1,1,1,1,1,1,1,1,1,1,1,1,1,1,1,1,1,1,1,1,1,1,1,1,1,1,1,1,1,1,1,
1,1,1,1,1,1,1,1,1,1,1,1,1,1,1,1,1,1,1,1,1,1,1,1,1,1,1,1,1,1,1,1,1,1,1,1,
1,1,1,1,1,1,1,1,1,1,1,1,1,1,1,1,1,1,1,1,1,1,1,1,1,1,1,1,1,1,1,1,1,1,1,1,
1,1,1,1,1,1,1,1,1,1,1,1,1,1,1,1,1,1,1,1,1,1,1,1,1,1,1,1,1,1,1,1,1,1,1,1,
1,1,1,1,1,1,1,1,1,1,1,1,1,1,1,1,1,1,1,1,1,1,1,1,1,1,1,1,1,1,1,1,1,1,1,1,
1,1,1,1,1,1,1,1,1,1,1,1,1,1,1,1,1,1,1,1,1,1,1,1,1,1,1,1,1,1,1,1,1,1,1,1,
1,1,1,1,1,1,1,1,1,1,1,1,1,1,1,1,1,1,1,1,1,1,1,1,1,1,1,1,1,1,1,1,1,1,1,1,
1,1,1,1,1,1,1,1,1,1,1,1,1,1,1,1,1,1,1,1,1,1,1,1,1,1,1,1,1,1,1,1,1,1,1,1,
1,1,1,1,1,1,1,1,1,1,1,1,1,1,1,1,1,1,1,1,1,1,1,1,1,1,1,1,1,1,1,1,1,1,1,1,
1,1,1,1,1,1,1,1,1,1,1,1,1,1,1,1,1,1,1,1,1,1,1,1,1,1,1,1,1,1,1,1,1,1,1,1,
1,1,1,1,1,1,1,1,1,1,1,1,1,1,1,1,1,1,1,1,1,1,1,1,1,1,1,1,1,1,1,1,1,1,1,1,
1,1,1,1,1,1,1,1,1,1,1,1,1,1,1,1,1,1,1,1,1,1,1,1,1,1,1,1,1,1,1,1,1,1,1,1,
1,1,1,1,1,1,1,1,1,1,1,1,1,1,1,1,1,1,1,1,1,1,1,1,1,1,1,1,1,1,1,1,1,1,1,1,
1,1,1,1,1,1,1,1,1,1,1,1,1,1,1,1,1,1,1,1,1,1,1,1,1,1,1,1,1,1,1,1,1,1,1,1,
1,1,1,1,1,1,1,1,1,1,1,1,1,1,1,1,1,1,1,1,1,1,1,1,1,1,1,1,1,1,1,1,1,1,1,1,
1,1,1,1,1,1,1,1,1,1,1,1,1,1,1,1,1,1,1,1,1,1,1,1,1,1,1,1,1,1,1,1,1,1,1,1,
1,1,1,1,1,1,1,1,1,1,1,1,1,1,1,1,1,1,1,1,1,1,1,1,1,1,1,1,1,1,1,1,1,1,1,1,
1,1,1,1,1,1,1,1,1,1,1,1,1,1,1,1,1,1,1,1,1,1,1,1,1,1,1,1,1,1,1,1,1,1,1,1,
1,1,1,1,1,1,1,1,1,1,1,1,1,1,1,1,1,1,1,1,1,1,1,1,1,1,1,1,1,1,1,1,1,1,1,1,
1,1,1,1,1,1,1,1,1,1,1,1,1,1,1,1,1,1,1,1,1,1,1,1,1,1,1,1,1,1,1,1,1,1,1,1,
1,1,1,1,1,1,1,1,1,1,1,1,1,1,1,1,1,1,1,1,1,1,1,1,1,1,1,1,1,1,1,1,1,1,1,1,
1,1,1,1,1,1,1,1,1,1,1,1,1,1,1,1,1,1,1,1,1,1,1,1,1,1,1,1,1,1,1,1,1,1,1,1,
1,1,1,1,1,1,1,1,1,1,1,1,1,1,1,1,1,1,1,1,1,1,1,1,1,1,1,1,1,1,1,1,1,1,1,1,
1,1,1,1,1,1,1,1,1,1,1,1,1,1,1,1,1,1,1,1,1,1,1,1,1,1,1,1,1,1,1,1,1,1,1,1,
1,1,1,1,1,1,1,1,1,1,1,1,1,1,1,1,1,1,1,1,1,1,1,1,1,1,1,1,1,1,1,1,1,1,1,1,
1,1,1,1,1,1,1,1,1,1,1,1,1,1,1,1,1,1,1,1,1,1,1,1,1,1,1,1,1,1,1,1,1,1,1,1,
1,1,1,1,1,1,1,1,1,1,1,1,1,1,1,1,1,1,1,1,1,1,1,1,1,1,1,1,1,1,1,1,1,1,1,1,
1,1,1,1,1,1,1,1,1,1,1,1,1,1,1,1,1,1,1,1,1,1,1,1,1,1,1,1,1,1,1,1,1,1,1,1,
1,1,1,1,1,1,1,1,1,1,1,1,1,1,1,1,1,1,1,1,1,1,1,1,1,1,1,1,1,1,1,1,1,1,1,1,
1,1,1,1,1,1,1,1,1,1,1,1,1,1,1,1,1,1,1,1,1,1,1,1,1,1,1,1,1,1,1,1,1,1,1,1,
1,1,1,1,1,1,1,1,1,1,1,1,1,1,1,1,1,1,1,1,1,1,1,1,1,1,1,1,1,1,1,1,1,1,1,1,
1,1,1,1,1,1,1,1,1,1,1,1,1,1,1,1,1,1,1,1,1,1,1,1,1,1,1,1,1,1,1,1,1,1,1,1,
1,1,1,1,1,1,1,1,1,1,1,1,1,1,1,1,1,1,1,1,1,1,1,1,1,1,1,1,1,1,1,1,1,1,1,1,
1,1,1,1,1,1,1,1,1,1,1,1,1,1,1,1,1,1,1,1,1,1,1,1,1,1,1,1,1,1,1,1,1,1,1,1,
1,1,1,1,1,1,1,1,1,1,1,1,1,1,1,1,1,1,1,1,1,1,1,1,1,1,1,1,1,1,1,1,1,1,1,1,
1,1,1,1,1,1,1,1,1,1,1,1,1,1,1,1,1,1,1,1,1,1,1,1,1,1,1,1,1,1,1,1,1,1,1,1,
1,1,1,1,1,1,1,1,1,1,1,1,1,1,1,1,1,1,1,1,1,1,1,1,1,1,1,1,1,1,1,1,1,1,1,1,
1,1,1,1,1,1,1,1,1,1,1,1,1,1,1,1,1,1,1,1,1,1,1,1,1,1,1,1,1,1,1,1,1,1,1,1,
1,1,1,1,1,1,1,1,1,1,1,1,1,1,1,1,1,1,1,1,1,1,1,1,1,1,1,1,1,1,1,1,1,1,1,1,
1,1,1,1,1,1,1,1,1,1,1,1,1,1,1,1,1,1,1,1,1,1,1,1,1,1,1,1,1,1,1,1,1,1,1,1,
1,1,1,1,1,1,1,1,1,1,1,1,1,1,1,1,1,1,1,1,1,1,1,1,1,1,1,1,1,1,1,1,1,1,1,1,
1,1,1,1,1,1,1,1,1,1,1,1,1,1,1,1,1,1,1,1,1,1,1,1,1,1,1,1,1,1,1,1,1,1,1,1,
1,1,1,1,1,1,1,1,1,1,1,1,1,1,1,1,1,1,1,1,1,1,1,1,1,1,1,1,1,1,1,1,1,1,1,1,
1,1,1,1,1,1,1,1,1,1,1,1,1,1,1,1,1,1,1,1,1,1,1,1,1,1,1,1,1,1,1,1,1,1,1,1,
1,1,1,1,1,1,1,1,1,1,1,1,1,1,1,1,1,1,1,1,1,1,1,1,1,1,1,1,1,1,1,1,1,1,1,1,
1,1,1,1,1,1,1,1,1,1,1,1,1,1,1,1,1,1,1,1,1,1,1,1,1,1,1,1,1,1,1,1,1,1,1,1,
1,1,1,1,1,1,1,1,1,1,1,1,1,1,1,1,1,1,1,1,1,1,1,1,1,1,1,1,1,1,1,1,1,1,1,1,
1,1,1,1,1,1,1,1,1,1,1,1,1,1,1,1,1,1,1,1,1,1,1,1,1,1,1,1,1,1,1,1,1,1,1,1,
1,1,1,1,1,1,1,1,1,1,1,1,1,1,1,1,1,1,1,1,1,1,1,1,1,1,1,1,1,1,1,1,1,1,1,1,
1,1,1,1,1,1,1,1,1,1,1,1,1,1,1,1,1,1,1,1,1,1,1,1,1,1,1,1,1,1,1,1,1,1,1,1,
1,1,1,1,1,1,1,1,1,1,1,1,1,1,1,1,1,1,1,1,1,1,1,1,1,1,1,1,1,1,1,1,1,1,1,1,
1,1,1,1,1,1,1,1,1,1,1,1,1,1,1,1,1,1,1,1,1,1,1,1,1,1,1,1,1,1,1,1,1,1,1,1,
1,1,1,1,1,1,1,1,1,1,1,1,1,1,1,1,1,1,1,1,1,1,1,1,1,1,1,1,1,1,1,1,1,1,1,1,
1,1,1,1,1,1,1,1,1,1,1,4),(3,2,2,2,3),(0.,0.01797683372391,0.286633051710584,
0.555289278308216,0.823945516665782,1.09260176953922,1.36125803873948,1.62991432588463,
1.89857063164012,2.16722695661301,2.43588330050525,2.70453966304674,2.9731960431531,
3.24185243981471,3.51050885133453,3.77916527610465,4.04782171198515,4.31647815691489,
4.58513460847725,4.85379106430677,5.12244752187208,5.39110397865606,5.65976043217153,
5.92841687990537,6.19707331956994,6.46572974881596,6.73438616570634,7.00304256821933,
7.2716989549161,7.5403553242696,7.809011675483,8.07766800769526,8.34632432089157,
8.61498061505147,8.8836368910788,9.15229314997201,9.4209493936865,9.68960562442157,
9.95826184531348,10.226918059948,10.4955742727586,10.7642304884925,11.0328867113173,
11.3015429448574,11.5701991918227,11.8388554546081,12.1075117346518,12.3761680332469,
12.6448243507434,12.9134806874637,13.1821370428496,13.450793416388,13.7194498067883,
13.9881062128412,14.2567626326955,14.5254190645885,14.7940755062772,15.0627319555912,
15.3313884100611,15.6000448672586,15.8687013246492,16.1373577797,16.4060142299691,
16.6746706729765,16.9433271065265,17.2119835283531,17.4806399366567,17.7492963295502,
18.0179527057767,18.286609063996,18.555265403637,18.8239217240786,19.0925780255742,
19.3612343083975,19.6298905737625,19.898546823017,20.1672030584666,20.4358592827168,
20.7045154992928,20.973171712245,21.2418279262962,21.5104841459723,21.7791403749736,
22.0477966165324,22.316452872948,22.585109146262,22.8537654375589,23.1224217478187,
23.3910780770929,23.6597344254327,23.9283907920352,24.197047176159,24.4657035763222,
24.7343599911301,25.0030164185931,25.2716728568073,25.5403293034427,25.8089857562333,
26.0776422126729,26.3462986702843,26.6149551265448,26.8836115789212,27.1522680250308,
27.4209244624423,27.6895808890659,27.9582373027346,28.2268937018004,28.4955500845261,
28.7642064498512,29.0328627966379,29.3015191245544,29.5701754332357,29.838831723217,
30.1074879950829,30.3761442503694,30.6448004907916,30.9134567190168,31.1821129380756,
31.450769151893,31.7194253649682,31.9880815819663,32.2567378070174,32.5253940433706,
32.7940502938785,33.0627065604467,33.3313628447765,33.6000191476151,33.8686754696427,
34.1373318106287,34.405988170366,34.6746445478242,34.9433009420458,35.2119573513747,
35.480613774244,35.7492702085419,36.0179266522368,36.2865831029275,36.5552395582669,
36.8238960157264,37.0925524727952,37.3612089269773,37.6298653757534,37.8985218168153,
38.1671782477952,38.4358346667239,38.7044910715485,38.9731474607866,39.2418038328672,
39.5104601869391,39.7791165220837,40.0477728382212,40.3164291352602,40.5850854140292,
40.8537416754418,41.1223979213679,41.3910541539077,41.6597103761025,41.9283665914244,
42.1970228042084,42.4656790192,42.7343352406829,43.0029914723808,43.2716477171096,
43.540303977354,43.8089602546436,44.0776165503516,44.3462728649052,44.614929198697,
44.883585551232,45.1522419220568,45.4208983099307,45.6895547136931,45.9582111315299,
46.2268675617156,46.4955240020317,46.7641804503338,47.0328369041642,47.3014933611089,
47.5701498186329,47.8388062742058,48.107462725373,48.3761191696448,48.6447756048012,
48.9134320285537,49.1820884390673,49.4507448344197,49.7194012133072,49.9880575743413,
50.2567139168934,50.5253702402807,50.7940265446884,51.0626828303152,51.3313390982961,
51.5999953498901,51.8686515873141,52.1373078130706,52.4059640305862,52.6746202437936,
52.9432764573682,53.211932675918,53.480588903259,53.7492451427202,54.0179013967021,
54.2865576673334,54.5552139557853,54.823870263115,55.0925265894471,55.3611829348992,
55.6298392987282,55.8984956802486,56.1671520780245,56.4358084907065,56.7044649163381,
56.9731213530494,57.2417777985307,57.5104342505384,57.7790907065743,58.0477471641719,
58.3164036208043,58.5850600739368,58.8537165211707,59.1223729600609,59.39102938849,
59.6596858042645,59.9283422056975,60.1969985910129,60.4656549590995,60.7343113087676,
61.0029676396243,61.2716239512389,61.540280244075,61.808936518638,62.0775927763821,
62.3462490189291,62.6149052488546,62.8835614690812,63.1522176834332,63.4208738963055,
63.6895301124163,63.9581863359981,64.2268425704115,64.4954988186027,64.7641550825741,
65.0328113641112,65.3014676640435,65.5701239831253,65.8387803211949,66.1074366781083,
66.3760930528907,66.6447494446373,66.9134058517341,67.1820622726558,67.4507187053199,
67.7193751477252,67.988031597487,68.256688052277,68.5253445095709,68.7940009668648,
69.0626574216546,69.3313138714164,69.5999703138218,69.8686267464858,70.1372831674076,
70.4059395745042,70.6745959662509,70.9432523410334,71.2119086979469,71.4805650360164,
71.7492213550982,72.0178776550306,72.2865339365675,72.5551902005389,72.8238464487301,
73.0925026831433,73.3611589067251,73.6298151228357,73.8984713357081,74.1671275500599,
74.4357837702864,74.7044400002118,74.9730962427587,75.2417525005027,75.5104087750655,
75.7790650679015,76.047721379516,76.3163777103726,76.5850340600405,76.853690428127,
77.1223468134422,77.391003214875,77.6596596306495,77.9283160590784,78.1969724979684,
78.4656289452021,78.7342853983344,79.0029418549666,79.2715983125641,79.5402547685998,
79.8089112206075,80.0775676660886,80.3462241027997,80.6148805284312,80.8835369411131,
81.1521933388889,81.4208497204091,81.689506084238,81.9581624296899,82.2268187560219,
82.4954750633515,82.7641313518033,83.0327876224345,83.3014438764161,83.5701001158772,
83.838756343218,84.1074125617677,84.3760687753422,84.6447249885494,84.913381206065,
85.1820374318212,85.4506936692451,85.719349920839,85.9880061888197,86.2566624744465,
86.5253187788541,86.7939751022413,87.0626314447932,87.3312878058273,87.5999441847146,
87.8686005800667,88.1372569905802,88.4059134143327,88.6745698494889,88.9432262937606,
89.2118827449277,89.4805392005005,89.7491956580243,90.0178521149689,90.2865085687992,
90.5551650171012,90.8238214574172,91.0924778876028,91.3611343054394,91.6297907092016,
91.8984470970753,92.1671034679,92.4357598204347,92.7044161542264,92.9730724687798,
93.2417287644878,93.5103850417773,93.7790413020216,94.0476975467502,94.3163537784479,
94.5850099999307,94.8536662149221,95.1223224277061,95.390978643028,95.6596348652226,
95.9282910977624,96.1969473436883,96.4656036051009,96.7342598838697,97.0029161809086,
97.2715724970461,97.5402288321905,97.8088851862623,98.0775415583427,98.3461979475807,
98.6148543524051,98.8835107713336,99.1521672023136,99.4208236433754,99.6894800921513,
99.9581365463333,100.226793003402,100.495449460861,100.7641059162,101.032762366891,
101.301418810586,101.570075244884,101.838731667753,102.107388077082,102.376044471303,
102.644700848761,102.913357208498,103.182013549484,103.450669871511,103.71932617435,
103.98798245868,104.256638725248,104.525294975755,104.793951212108,105.062607437159,
105.331263654157,105.599919867233,105.86857608105,106.137232300108,106.405888528334,
106.674544768756,106.943201024042,107.211857295908,107.480513585889,107.74916989457,
108.017826222487,108.286482569273,108.555138934598,108.823795317324,109.09245171639,
109.361108130058,109.629764556682,109.898420994093,110.167077440202,110.435733892579,
110.704390348839,110.97304680645,111.24170326289,111.51035971568,111.779016162316,
112.04767260053,112.316329027993,112.5849854428,112.853641842963,113.122298227087,
113.39095459369,113.659610942029,113.928267271303,114.196923581563,114.46557987286,
114.734236146174,115.002892402589,115.271548644148,115.540204873149,115.808861092825,
116.077517306876,116.346173519828,116.614829736404,116.883485960654,117.152142196103,
117.420798445358,117.689454710722,117.958110993546,118.226767295041,118.495423615483,
118.764079955123,119.032736313343,119.301392689569,119.570049082462,119.838705490766,
120.107361912592,120.376018346142,120.644674789149,120.913331239418,121.181987694469,
121.45064415186,121.719300609057,121.987957063527,122.256613512841,122.525269954529,
122.793926386422,123.062582806276,123.331239212329,123.599895602729,123.868551976268,
124.137208331653,124.405864668374,124.67452098587,124.943177284465,125.211833564508,
125.480489827294,125.749146074259,126.017802307799,126.286458530624,126.555114746357,
126.823770959168,127.092427173802,127.361083394694,127.629739625429,127.898395869143,
128.167052128037,128.435708404064,128.704364698224,128.97302101142,129.241677343633,
129.510333694846,129.7789900642,130.047646450897,130.31630285341,130.5849592703,
130.853615699547,131.122272139211,131.390928586945,131.659585040461,131.928241497245,
132.19689795481,132.46555441064,132.734210862202,133.002867307132,133.271523743013,
133.540180167783,133.808836579303,134.077492975965,134.346149356071,134.614805718613,
134.883462062505,135.152118387478,135.420774693234,135.689430980379,135.958087249579,
136.226743502453,136.49539974081,136.76405596741,137.032712185392,137.301368398783,
137.570024612174,137.838680830155,138.107337056755,138.375993295112,138.644649547986,
138.913305817186,139.181962104332,139.450618410087,139.71927473506,139.987931078952,
140.256587441494,140.525243821601,140.793900218262,141.062556629782,141.331213054552,
141.599869490433,141.868525935363,142.137182386925,142.405838842755,142.67449530032,
142.943151757104,143.21180821062,143.480464658354,143.749121098019,144.017777527265,
144.286433944155,144.555090346668,144.823746733365,145.092403102719,145.361059453932,
145.629715786145,145.898372099341,146.167028393501,146.435684669529,146.704340928422,
146.972997172137,147.241653402872,147.510309623764,147.778965838398,148.047622051209,
148.316278266943,148.584934489768,148.853590723308,149.122246970274,149.390903233059,
149.659559513103,149.928215811698,150.196872129195,150.465528465915,150.734184821301,
151.00284119484,151.27149758524,151.540153991293,151.808810411148,152.077466843041,
152.34612328473,152.614779734044,152.883436188514,153.152092645711,153.420749103102,
153.689405558153,153.958062008422,154.22671845143,154.49537488498,154.764031306806,
155.03268771511,155.301344108004,155.57000048423,155.838656842449,156.107313182091,
156.375969502532,156.644625804028,156.913282086851,157.181938352216,157.450594601471,
157.719250836921,157.987907061171,158.256563277747,158.525219490699,158.793875704751,
159.062531924427,159.331188153428,159.599844394987,159.868500651403,160.137156924717,
160.405813216014,160.674469526274,160.943125855548,161.211782203888,161.480438570491,
161.749094954615,162.017751354778,162.286407769586,162.555064197049,162.823720635263,
163.092377081899,163.361033534689,163.629689991129,163.898346448741,164.167002905001,
164.435659357378,164.704315803488,164.972972240899,165.241628667523,165.510285081192,
165.778941480257,166.047597862983,166.316254228308,166.584910575095,166.853566903012,
167.122223211693,167.390879501675,167.659535773541,167.928192028827,168.19684826925,
168.465504497475,168.734160716534,169.002816930351,169.271473143427,169.540129360425,
169.808785585476,170.077441821829,170.346098072337,170.614754338905,170.883410623235,
171.152066926074,171.420723248102,171.689379589088,171.958035948825,172.226692326284,
172.495348720505,172.764005129834,173.032661552704,173.301317987002,173.569974430697,
173.838630881388,174.107287336727,174.375943794187,174.644600251255,174.913256705437,
175.181913154214,175.450569595276,175.719226026256,175.987882445184,176.256538850009,
176.525195239247,176.793851611328,177.0625079654,177.331164300545,177.599820616682,
177.868476913721,178.137133192491,178.405789453903,178.674445699829,178.943101932369,
179.211758154564,179.480414369886,179.74907058267,180.017726797662,180.286383019145,
180.555039250843,180.823695495572,181.092351755816,181.361008033106,181.629664328814,
181.898320643368,182.16697697716,182.435633329695,182.70428970052,182.972946088394,
183.241602492156,183.510258909993,183.778915340179,184.047571780495,184.316228228797,
184.584884682628,184.853541139572,185.122197597096,185.39085405267,185.659510503837,
185.928166948109,186.196823383265,186.465479807018,186.734136217531,187.002792612884,
187.271448991771,187.540105352806,187.808761695358,188.077418018745,188.346074323153,
188.61473060878,188.883386876761,189.152043128355,189.420699365779,189.689355591536,
189.958011809051,190.226668022259,190.495324235834,190.763980454383,191.032636681725,
191.301292921186,191.569949175168,191.838605445799,192.107261734251,192.375918041581,
192.644574367913,192.913230713365,193.181887077194,193.450543458715,193.719199856491,
193.987856269173,194.256512694805,194.525169131516,194.793825576997,195.062482029005,
195.331138485041,195.599794942639,195.868451399271,196.137107852404,196.405764299638,
196.674420738528,196.943077166957,197.211733582732,197.480389984165,197.749046369481,
198.017702737567,198.286359087236,198.555015418092,198.823671729707,199.092328022543,
199.360984297106,199.62964055485,199.898296797397,200.166953027323,200.43560924755,
200.704265461902,200.972921674774,201.241577890885,201.510234114467,201.77889034888,
202.047546597072,202.316202861043,202.584859142581,202.853515442513,203.122171761595,
203.390828099665,203.659484456579,203.928140831361,204.196797223108,204.465453630205,
204.734110051127,205.002766483791,205.271422926197,205.540079375959,205.808735830749,
206.077392288043,206.346048745337,206.614705200127,206.883361649889,207.152018092295,
207.420674524959,207.689330945881,207.957987352978,208.226643744725,208.495300119508,
208.763956476421,209.032612814491,209.301269133573,209.569925433505,209.838581715043,
210.107237979014,210.375894227206,210.644550461619,210.913206685201,211.181862901312,
211.450519114184,211.719175328536,211.987831548763,212.256487778689,212.525144021236,
212.79380027898,213.062456553543,213.331112846379,213.599769157994,213.868425488851,
214.137081838519,214.405738206606,214.674394591921,214.943050993354,215.211707409129,
215.480363837558,215.749020276448,216.017676723682,216.286333176815,216.554989633447,
216.823646091045,217.092302547081,217.360958999089,217.62961544457,217.898271881281,
218.166928306913,218.435584719595,218.704241117371,218.972897498892,219.241553862721,
219.510210208173,219.778866534505,220.047522841835,220.316179130287,220.584835400918,
220.8534916549,221.122147894361,221.390804121702,221.659460340252,221.928116553827,
222.196772767034,222.46542898455,222.734085210306,223.00274144773,223.271397699324,
223.540053967305,223.808710252932,224.07736655734,224.346022880728,224.61467922328,
224.883335584314,225.151991963201,225.420648358554,225.689304769068,225.95796119282,
226.226617627977,226.495274072249,226.763930523416,227.032586978989,227.301243436513,
227.569899893458,227.838556347288,228.10721279559,228.375869235907,228.644525666093,
228.913182083929,229.181838487692,229.450494875566,229.719151246391,229.987807598926,
230.256463932718,230.525120247271,230.79377654298,231.062432820269,231.331089080514,
231.599745325243,231.868401556941,232.137057778424,232.405713993415,232.674370206199,
232.943026421521,233.211682643716,233.480338876256,233.748995122182,234.017651383595,
234.286307662364,234.554963959403,234.823620275541,235.092276610685,235.360932964757,
235.629589336838,235.898245726076,236.166902130901,236.43555854983,236.70421498081,
236.972871421872,237.241527870648,237.51018432483,237.778840781899,238.047497239359,
238.316153694698,238.584810145389,238.853466589084,239.122123023382,239.390779446251,
239.65943585558,239.928092249802,240.19674862726,240.465404986998,240.734061327984,
241.002717650011,241.27137395285,241.54003023718,241.808686503748,242.077342754256,
242.345998990609,242.614655215661,242.883311432659,243.151967645734,243.420623859552,
243.68928007861,243.957936306836,244.226592547258,244.495248802545,244.763905074411,
245.032561364392,245.301217673074,245.56987400099,245.838530347777,246.107186713102,
246.375843095828,246.644499494894,246.913155908563,247.181812335186,247.450468772598,
247.719125218708,247.987781671084,248.256438127345,248.525094584956,248.793751041396,
249.062407494187,249.331063940822,249.599720379036,249.8683768065,250.137033221308,
250.405689621471,250.674346005595,250.943002372197,251.211658720537,251.480315049812,
251.748971360071,252.017627651368,252.286283924683,252.554940181098,252.823596422657,
253.092252651658,253.360908871335,253.629565085386,253.898221298338,254.166877514914,
254.435533739165,254.704189974614,254.972846223869,255.241502489234,255.510158772057,
255.778815073553,256.047471393995,256.316127733635,256.584784091854,256.85344046808,
257.122096860973,257.390753269276,257.659409691102,257.928066124652,258.196722567659,
258.465379017928,258.734035472978,259.002691930368,259.271348387566,259.540004842035,
259.808661291349,260.077317733037,260.345974164929,260.614630584783,260.883286990836,
261.151943381235,261.420599754774,261.689256110159,261.957912446879,262.226568764375,
262.49522506297,262.763881343014,263.032537605798,263.301193852763,263.569850086303,
263.838506309127,264.107162524861,264.375818737671,264.644474952305,264.913131173196,
265.181787403931,265.450443647645,265.719099906538,265.987756182565,266.256412476724,
266.52506878992,266.793725122132,267.062381473345,267.331037842698,267.599694229394,
267.868350631907,268.137007048797,268.405663478042,268.674319917706,268.94297636544,
269.211632818955,269.480289275739,269.748945733304,270.017602189133,270.286258640695,
270.554915085624,270.823571521504,271.092227946274,271.360884357793,271.629540754454,
271.89819713456,272.166853497101,272.435509840993,272.704166165965,272.97282247172,
273.241478758865,273.510135028065,273.778791280938,274.047447519295,274.316103745894,
274.584759963875,274.853416177266,275.122072390656,275.390728608637,275.659384835237,
275.928041073593,276.196697326466,276.465353595666,276.734009882811,277.002666188566,
277.271322513539,277.53997885743,277.808635219972,278.077291600077,278.345947996739,
278.614604408258,278.883260833028,279.151917268908,279.420573713837,279.689230165399,
279.957886621228,280.226543078793,280.495199535576,280.763855989092,281.032512436825,
281.301168876489,281.569825305735,281.838481722625,282.107138125138,282.375794511834,
282.644450881187,282.9131072324,283.181763564612,283.450419877808,283.719076171967,
283.987732447994,284.256388706887,284.525044950601,284.793701181336,285.062357402228,
285.331013616862,285.599669829672,285.868326045405,286.136982268229,286.405638501769,
286.674294748734,286.942951011519,287.211607291562,287.480263590157,287.748919907653,
288.017576244373,288.286232599758,288.554888973296,288.823545363696,289.092201769749,
289.360858189603,289.629514621495,289.898171063183,290.166827512497,290.435483966966,
290.704140424163,290.972796881554,291.241453336604,291.510109786873,291.77876622988,
292.047422663429,292.316079085255,292.584735493559,292.853391886452,293.122048262678,
293.390704620897,293.659360960537,293.928017280978,294.196673582474,294.465329865297,
294.733986130661,295.002642379915,295.271298615364,295.539954839614,295.808611056189,
296.077267269141,296.345923483192,296.614579702867,296.883235931868,297.151892173427,
297.420548429842,297.689204703155,297.957860994452,298.226517304711,298.495173633985,
298.763829982324,299.032486348927,299.30114273305,299.569799133212,299.83845554802,
300.107111975482,300.375768413696,300.644424860331,300.913081313121,301.181737769561,
301.450394227172,301.719050683432,301.987707135808,302.256363581917,302.525020019328,
302.793676445951,303.062332859619,303.330989258684,303.59964564141,303.868302006734,
304.136958353521,304.405614681437,304.674270990118,304.942927280098,305.211583551964,
305.48023980725,305.748896047671,306.017552275896,306.286208494954,306.554864708772,
306.823520921846,307.092177138844,307.360833363895,307.629489600247,307.898145850755,
308.166802117323,308.435458401652,308.70411470449,308.972771026517,309.241427367503,
309.51008372724,309.778740104698,310.047396498919,310.316052908247,310.584709331116,
310.853365765414,311.122022209108,311.390678659798,311.659335115137,311.927991572596,
312.196648029665,312.465304483846,312.733960932622,313.002617373684,313.271273804663,
313.539930223591,313.808586628416,314.077243017653,314.345899389733,314.614555743805,
314.883212078949,315.151868395086,315.420524692125,315.689180970894,315.957837232306,
316.226493478231,316.495149710771,316.763805932965,317.032462148286,317.30111836107,
317.569774576061,317.838430797543,318.107087029241,318.375743273969,318.644399534213,
318.913055811502,319.18171210721,319.450368421763,319.719024755555,319.987681108089,
320.256337478914,320.524993866787,320.793650270549,321.062306688385,321.33096311857,
321.599619558886,321.868276007188,322.136932461018,322.405588917962,322.674245375486,
322.942901831059,323.211558282225,323.480214726497,323.748871161653,324.017527585405,
324.286183995918,324.55484039127,324.823496770157,325.09215313119,325.360809473742,
325.629465797129,325.898122101536,326.166778387163,326.435434655143,326.704090906737,
326.97274714416,327.241403369916,327.510059587432,327.778715800638,328.047372014213,
328.316028232762,328.584684460102,328.853340699563,329.121996953545,329.390653224175,
329.659309512627,329.927965819956,330.196622146288,330.46527849174,330.733934855568,
331.002591237088,331.271247634863,331.539904047545,331.808560473176,332.077216909887,
332.345873355368,332.614529807375,332.883186263411,333.151842721008,333.42049917764,
333.689155630772,333.957812078005,334.226468516895,334.495124945324,334.763781361098,
335.03243776253,335.301094147845,335.569750515931,335.838406865599,336.107063196455,
336.375719508069,336.644375800905,336.913032075468,337.181688333211,337.450344575758,
337.719000805683,337.987657025909,338.256313240261,338.524969453133,338.793625669243,
339.062281892824,339.330938127237,339.599594375428,339.868250639399,340.136906920936,
340.405563220868,340.674219539949,340.942875878019,341.211532234932,341.480188609714,
341.74884500146,342.017501408557,342.286157829478,342.554814262142,342.823470704547,
343.092127154308,343.360783609098,343.629440066391,343.898096523685,344.166752978475,
344.435409428236,344.704065870641,344.972722303305,345.241378724226,345.510035131323,
345.778691523069,346.047347897851,346.316004254764,346.584660592834,346.853316911915,
347.121973211847,347.390629493384,347.659285757355,347.927942005546,348.196598239959,
348.46525446354,348.733910679651,349.002566892523,349.271223106874,349.5398793271,
349.808535557025,350.077191799572,350.345848057315,350.614504331878,350.883160624714,
351.151816936328,351.420473267184,351.689129616852,351.957785984938,352.226442370253,
352.495098771685,352.76375518746,353.032411615888,353.301068054778,353.569724502012,
353.838380955144,354.107037411776,354.375693869373,354.644350325408,354.913006777416,
355.181663222896,355.450319659607,355.718976085238,355.98763249792,356.256288895695,
356.524945277215,356.793601641044,357.062257986496,357.330914312827,357.599570620156,
357.868226908608,358.136883179239,358.40553943322,358.674195672681,358.942851900021,
359.211508118571,359.480164332145,359.748820545352,360.017476762867,360.286132988623,
360.554789226047,360.82344547764,361.09210174562,361.360758031247,361.629414335654,
361.898070659041,362.166727001593,362.435383362626,362.704039741513,362.972696136865,
363.241352547378,363.510008971131,363.778665406287,364.047321850558,364.315978301725,
364.584634757297,364.853291214821,365.121947671765,365.390604125595,365.659260573897,
365.927917014213,366.196573444398,366.465229862234,366.733886265996,367.002542653869,
367.271199024694,367.539855377228,367.808511711019,368.077168025573,368.34582432128,
368.614480598569,368.883136858813,369.151793103542,369.420449335239,369.689105556722,
369.957761771713,370.226417984496,370.495074199818,370.763730422012,371.032386654551,
371.301042900477,371.569699161889,371.838355440658,372.107011737697,372.375668053834,
372.644324388978,372.912980743049,373.18163711513,373.450293504367,373.718949909191,
373.98760632812,374.256262759099,374.524919200161,374.793575648936,375.062232103118,
375.330888560186,375.599545017646,375.868201472985,376.136857923675,376.40551436737,
376.674170801667,376.942827224536,377.211483633864,377.480140028085,377.748796405543,
378.01745276528,378.286109106266,378.554765428293,378.823421731131,379.092078015461,
379.360734282028,379.629390532536,379.898046768888,380.166702993939,380.435359210937,
380.704015424011,380.972671637828,381.241327856887,381.509984085112,381.778640325533,
382.047296580819,382.315952852685,382.584609142666,382.853265451347,383.121921779263,
383.390578126049,383.659234491374,383.927890874099,384.196547273165,384.465203686833,
384.733860113456,385.002516550867,385.271172996977,385.539829449352,385.808485905613,
386.077142363224,386.345798819663,386.614455272453,386.883111719088,387.151768157302,
387.420424584764,387.689080999572,387.957737399735,388.226393783858,388.49505015046,
388.7637064988,389.032362828074,389.301019138333,389.56967542963,389.838331702943,
390.106987959358,390.375644200917,390.644300429918,390.912956649593,391.181612863644,
391.450269076596,391.718925293171,391.987581517421,392.25623775287,392.524894002124,
392.793550267489,393.062206550312,393.330862851807,393.599519172248,393.868175511888,
394.136831870107,394.405488246334,394.674144639227,394.94280104753,395.211457469356,
395.480113902905,395.748770345913,396.017426796181,396.286083251232,396.554739708622,
396.823396165819,397.092052620289,397.360709069602,397.629365511291,397.898021943183,
398.166678363037,398.43533476909,398.703991159489,398.972647533028,399.241303888413,
399.509960225133,399.778616542629,400.047272841224,400.315929121267,400.584585384052,
400.853241631017,401.121897864557,401.390554087381,401.659210303115,401.927866515925,
402.196522730559,402.465178951451,402.733835182185,403.002491425899,403.271147684792,
403.539803960819,403.808460254978,404.077116568174,404.345772900386,404.614429251599,
404.883085620952,405.151742007649,405.420398410161,405.689054827051,405.957711256297,
406.226367695961,406.495024143695,406.76368059721,407.032337053993,407.300993511558,
407.569649967387,407.838306418949,408.106962863879,408.375619299759,408.644275724528,
408.912932136048,409.181588532709,409.450244912815,409.718901275356,409.987557619248,
410.25621394422,410.524870249975,410.79352653712,411.06218280632,411.330839059193,
411.599495297549,411.868151524149,412.13680774213,412.40546395552,412.674120168911,
412.942776386892,413.211432613491,413.480088851848,413.748745104721,414.017401373921,
414.286057661065,414.55471396682,414.823370291793,415.092026635685,415.360682998226,
415.629339378332,415.897995774993,416.166652186512,416.435308611282,416.703965047162,
416.972621492092,417.241277943654,417.509934399483,417.778590857048,418.047247313831,
418.315903767346,418.58456021508,418.853216654744,419.121873083989,419.390529500879,
419.659185903392,419.927842290088,420.196498659441,420.465155010654,420.733811342866,
421.002467656062,421.271123950222,421.539780226249,421.808436485141,422.077092728855,
422.34574895959,422.614405180482,422.883061395116,423.151717607926,423.42037382366,
423.689030046484,423.957686280024,424.226342526988,424.494998789773,424.763655069817,
425.032311368411,425.300967685907,425.569624022627,425.838280378013,426.106936751551,
426.375593141951,426.644249548003,426.912905967857,427.18156239975,427.450218841438,
427.718875290752,427.987531745221,428.256188202418,428.524844659809,428.793501114859,
429.062157565128,429.330814008135,429.599470441684,429.868126863511,430.136783271814,
430.405439664707,430.674096040933,430.942752399152,431.211408738792,431.480065059233,
431.748721360729,432.017377643552,432.286033908916,432.554690158171,432.823346393619,
433.092002617869,433.360658834445,433.629315047397,433.897971261447,434.166627481123,
434.435283710124,434.703939951682,434.972596208097,435.241252481411,435.509908772707,
435.778565082967,436.047221412241,436.31587776058,436.584534127182,436.853190511305,
437.121846911468,437.390503326275,437.659159753738,437.927816191952,438.196472638587,
438.465129091377,438.733785547816,439.002442005427,439.271098461688,439.539754914064,
439.808411360173,440.077067797584,440.345724224207,440.614380637875,440.883037036941,
441.151693419666,441.420349784991,441.689006131777,441.957662459693,442.226318768374,
442.494975058355,442.763631330221,443.032287585506,443.300943825928,443.569600054153,
443.838256273211,444.106912487028,444.375568700103,444.644224917101,444.912881142151,
445.181537378504,445.450193629011,445.718849895579,445.987506179909,446.256162482747,
446.524818804774,446.79347514576,447.062131505496,447.330787882954,447.599444277176,
447.868100686504,448.136757109373,448.40541354367,448.674069987365,448.942726438055,
449.211382893394,449.480039350853,449.748695807921,450.017352262103,450.286008710879,
450.55466515194,450.82332158292,451.091978001848,451.360634406672,451.62929079591,
451.89794716799,452.166603522061,452.435259857205,452.703916173343,452.972572470381,
453.24122874915,453.509885010562,453.778541256488,454.047197489028,454.315853711222,
454.584509926543,454.853166139327,455.121822354318,455.3904785758,455.659134807498,
455.927791052226,456.19644731247,456.465103589759,456.733759885467,457.00241620002,
457.271072533811,457.539728886346,457.80838525717,458.077041645044,458.345698048806,
458.614354466642,458.883010896827,459.151667337143,459.420323785445,459.688980239275,
459.957636696219,460.226293153743,460.494949609316,460.763606060482,461.032262504754,
461.300918939909,461.569575363662,461.838231774175,462.106888169527,462.375544548414,
462.644200909447,462.912857251999,463.181513575386,463.450169879794,463.71882616542,
463.987482433401,464.256138684994,464.524794922418,464.793451148174,465.062107365689,
465.330763578896,465.59941979247,465.86807601102,466.13673223836,466.405388477821,
466.674044731802,466.942701002433,467.211357290885,467.480013598214,467.748669924546,
468.017326269997,468.285982633826,468.554639015346,468.823295413121,469.091951825803,
469.360608251434,469.629264688145,469.897921133626,470.166577585633,470.435234041669,
470.703890499266,470.972546955898,471.24120340903,471.509859856263,471.778516295153,
472.047172723582,472.315829139356,472.584485540789,472.853141926103,473.12179829419,
473.390454643857,473.659110974714,473.927767286328,474.196423579164,474.465079853726,
474.73373611147,475.002392354016,475.271048583941,475.539704804167,475.808361018519,
476.077017231391,476.345673447501,476.614329671083,476.882985905496,477.151642153686,
477.420298417658,477.688954699194,477.957610999126,478.226267318208,478.494923656277,
478.76358001319,479.032236387973,479.300892779719,479.569549186815,479.838205607737,
480.106862040401,480.375518482806,480.644174932567,480.912831387357,481.18148784465,
481.450144301944,481.718800756733,481.987457206495,482.2561136489,482.524770081563,
482.793426502485,483.062082909582,483.330739301328,483.59939567611,483.868052033023,
484.136708371092,484.405364690174,484.674020990106,484.942677271643,485.211333535614,
485.479989783805,485.748646018218,486.017302241799,486.28595845791,486.554614670781,
486.823270885133,487.091927105359,487.360583335284,487.629239577831,487.897895835574,
488.166552110137,488.435208402973,488.703864714587,488.972521045443,489.241177395111,
489.509833763197,489.778490148512,490.047146549945,490.315802965719,490.584459394147,
490.853115833037,491.12177228027,491.390428733402,491.659085190034,491.927741647632,
492.196398103667,492.465054555674,492.733711001155,493.002367437866,493.271023863497,
493.539680276179,493.808336673954,494.076993055474,494.345649419303,494.614305764754,
494.882962091086,495.151618398416,495.420274686867,495.688930957498,495.95758721148,
496.22624345094,496.494899678281,496.76355589683,497.032212110404,497.300868323611,
497.569524541126,497.838180766882,498.106837004306,498.3754932559,498.64414952388,
498.912805809507,499.181462113914,499.450118437301,499.718774779852,499.987431140886,
500.256087519773,500.524743915125,500.793400325638,501.06205674939,501.330713184546,
501.599369628818,501.868026079984,502.136682535557,502.40533899308,502.673995450025,
502.942651903855,503.211308352156,503.479964792472,503.748621222657,504.017277640494,
504.285934044256,504.554590432129,504.823246802954,505.091903155488,505.360559489279,
505.629215803832,505.89787209954,506.166528376829,506.435184637073,506.703840881801,
506.972497113499,507.241153334981,507.509809549972,507.778465762756,508.047121978078,
508.315778200272,508.584434432811,508.853090678737,509.121746940149,509.390403218918,
509.659059515956,509.927715832093,510.196372167238,510.465028521309,510.733684893389,
511.002341282627,511.270997687451,511.53965410638,511.808310537359,512.076966978421,
512.345623427198,512.614279881382,512.882936338452,513.151592795914,513.420249251254,
513.688905701946,513.957562145643,514.226218579942,514.494875002812,514.763531412143,
515.032187806366,515.300844183826,515.569500543564,515.838156884552,516.106813206581,
516.375469509421,516.644125793752,516.912782060321,517.181438310831,517.450094547186,
517.718750772238,517.987406989238,518.256063202315,518.524719416134,518.793375635194,
519.062031863421,519.330688103845,519.599344359133,519.868000631,520.136656920983,
520.405313229665,520.673969557583,520.942625904371,521.211282269698,521.479938652425,
521.748595051492,522.017251465163,522.285907891788,522.554564329201,522.823220775312,
523.091877227689,523.360533683951,523.629190141564,523.897846598005,524.166503050797,
524.435159497434,524.70381593565,524.972472363114,525.241128777924,525.509785178088,
525.778441562214,526.047097928818,526.315754277159,526.584410606435,526.853066916696,
527.121723207994,527.390379481309,527.659035737726,527.927691979287,528.19634820829,
528.465004427967,528.73366064202,529.002316854973,529.270973071551,529.539629295803,
529.808285531254,530.07694178051,530.345598045876,530.614254328701,530.882910630198,
531.151566950641,531.420223290284,531.688879648504,531.957536024733,532.226192417628,
532.494848825933,532.76350524776,533.032161681312,533.30081812432,533.569474574591,
533.838131029643,534.106787487035,534.375443944235,534.644100398706,534.912756848021,
535.181413289711,535.450069721605,535.718726141461,535.987382547516,536.256038937917,
536.524695311458,536.793351666845,537.062008003567,537.330664321065,537.599320619661,
537.867976899706,538.136633162493,538.40528940946,538.673945643001,538.942601865828,
539.211258081563,539.479914294375,539.748570509011,540.017226729904,540.285882960641,
540.554539204357,540.823195463252,541.09185173928,541.360508033441,541.629164346639,
541.897820678853,542.166477030068,542.435133399423,542.703789786121,542.972446188636,
543.241102605527,543.509759034775,543.778415474441,544.047071922176,544.315728375693,
544.584384832479,544.853041290046,545.121697745877,545.390354197441,545.659010642372,
545.927667078254,546.196323503025,546.464979914547,546.733636311202,547.002292691334,
547.270949053789,547.539605397955,547.808261722147,548.076918029812,548.345574313508,
548.614230583738,548.882886864851,549.151542935882,549.420199787641,549.68885445376,
549.957511414581),(0.,0.117809724509617,0.235619449019234,0.353429173528852,
0.471238898038469),.UNSPECIFIED.)
GEOMETRIC_REPRESENTATION_ITEM()
RATIONAL_B_SPLINE_SURFACE(((1.,0.707106781186548,1.,0.707106781186548,1.,
0.707106781186548,1.,0.707106781186548,1.),(1.,0.707106781186548,1.,0.707106781186548,
1.,0.707106781186548,1.,0.707106781186548,1.),(1.,0.707106781186548,1.,
0.707106781186548,1.,0.707106781186548,1.,0.707106781186548,1.),(1.,0.707106781186547,
1.,0.707106781186547,1.,0.707106781186547,1.,0.707106781186547,1.),(1.,
0.707106781186547,1.,0.707106781186547,1.,0.707106781186547,1.,0.707106781186547,
1.),(1.,0.707106781186548,1.,0.707106781186548,1.,0.707106781186548,1.,
0.707106781186548,1.),(1.,0.707106781186547,1.,0.707106781186547,1.,0.707106781186547,
1.,0.707106781186547,1.),(1.,0.707106781186547,1.,0.707106781186547,1.,
0.707106781186547,1.,0.707106781186547,1.),(1.,0.707106781186547,1.,0.707106781186547,
1.,0.707106781186547,1.,0.707106781186547,1.),(1.,0.707106781186547,1.,
0.707106781186547,1.,0.707106781186547,1.,0.707106781186547,1.),(1.,0.707106781186547,
1.,0.707106781186547,1.,0.707106781186547,1.,0.707106781186547,1.),(1.,
0.707106781186548,1.,0.707106781186548,1.,0.707106781186548,1.,0.707106781186548,
1.),(1.,0.707106781186548,1.,0.707106781186548,1.,0.707106781186548,1.,
0.707106781186548,1.),(1.,0.707106781186548,1.,0.707106781186548,1.,0.707106781186548,
1.,0.707106781186548,1.),(1.,0.707106781186547,1.,0.707106781186547,1.,
0.707106781186547,1.,0.707106781186547,1.),(1.,0.707106781186548,1.,0.707106781186548,
1.,0.707106781186548,1.,0.707106781186548,1.),(1.,0.707106781186547,1.,
0.707106781186547,1.,0.707106781186547,1.,0.707106781186547,1.),(1.,0.707106781186547,
1.,0.707106781186547,1.,0.707106781186547,1.,0.707106781186547,1.),(1.,
0.707106781186548,1.,0.707106781186548,1.,0.707106781186548,1.,0.707106781186548,
1.),(1.,0.707106781186547,1.,0.707106781186547,1.,0.707106781186547,1.,
0.707106781186547,1.),(1.,0.707106781186548,1.,0.707106781186548,1.,0.707106781186548,
1.,0.707106781186548,1.),(1.,0.707106781186547,1.,0.707106781186547,1.,
0.707106781186547,1.,0.707106781186547,1.),(1.,0.707106781186548,1.,0.707106781186548,
1.,0.707106781186548,1.,0.707106781186548,1.),(1.,0.707106781186547,1.,
0.707106781186547,1.,0.707106781186547,1.,0.707106781186547,1.),(1.,0.707106781186548,
1.,0.707106781186548,1.,0.707106781186548,1.,0.707106781186548,1.),(1.,
0.707106781186547,1.,0.707106781186547,1.,0.707106781186547,1.,0.707106781186547,
1.),(1.,0.707106781186547,1.,0.707106781186547,1.,0.707106781186547,1.,
0.707106781186547,1.),(1.,0.707106781186547,1.,0.707106781186547,1.,0.707106781186547,
1.,0.707106781186547,1.),(1.,0.707106781186547,1.,0.707106781186547,1.,
0.707106781186547,1.,0.707106781186547,1.),(1.,0.707106781186547,1.,0.707106781186547,
1.,0.707106781186547,1.,0.707106781186547,1.),(1.,0.707106781186548,1.,
0.707106781186548,1.,0.707106781186548,1.,0.707106781186548,1.),(1.,0.707106781186547,
1.,0.707106781186547,1.,0.707106781186547,1.,0.707106781186547,1.),(1.,
0.707106781186547,1.,0.707106781186547,1.,0.707106781186547,1.,0.707106781186547,
1.),(1.,0.707106781186548,1.,0.707106781186548,1.,0.707106781186548,1.,
0.707106781186548,1.),(1.,0.707106781186547,1.,0.707106781186547,1.,0.707106781186547,
1.,0.707106781186547,1.),(1.,0.707106781186547,1.,0.707106781186547,1.,
0.707106781186547,1.,0.707106781186547,1.),(1.,0.707106781186548,1.,0.707106781186548,
1.,0.707106781186548,1.,0.707106781186548,1.),(1.,0.707106781186547,1.,
0.707106781186547,1.,0.707106781186547,1.,0.707106781186547,1.),(1.,0.707106781186547,
1.,0.707106781186547,1.,0.707106781186547,1.,0.707106781186547,1.),(1.,
0.707106781186548,1.,0.707106781186548,1.,0.707106781186548,1.,0.707106781186548,
1.),(1.,0.707106781186548,1.,0.707106781186548,1.,0.707106781186548,1.,
0.707106781186548,1.),(1.,0.707106781186547,1.,0.707106781186547,1.,0.707106781186547,
1.,0.707106781186547,1.),(1.,0.707106781186548,1.,0.707106781186548,1.,
0.707106781186548,1.,0.707106781186548,1.),(1.,0.707106781186547,1.,0.707106781186547,
1.,0.707106781186547,1.,0.707106781186547,1.),(1.,0.707106781186547,1.,
0.707106781186547,1.,0.707106781186547,1.,0.707106781186547,1.),(1.,0.707106781186547,
1.,0.707106781186547,1.,0.707106781186547,1.,0.707106781186547,1.),(1.,
0.707106781186548,1.,0.707106781186548,1.,0.707106781186548,1.,0.707106781186548,
1.),(1.,0.707106781186548,1.,0.707106781186548,1.,0.707106781186548,1.,
0.707106781186548,1.),(1.,0.707106781186547,1.,0.707106781186547,1.,0.707106781186547,
1.,0.707106781186547,1.),(1.,0.707106781186547,1.,0.707106781186547,1.,
0.707106781186547,1.,0.707106781186547,1.),(1.,0.707106781186548,1.,0.707106781186548,
1.,0.707106781186548,1.,0.707106781186548,1.),(1.,0.707106781186547,1.,
0.707106781186547,1.,0.707106781186547,1.,0.707106781186547,1.),(1.,0.707106781186548,
1.,0.707106781186548,1.,0.707106781186548,1.,0.707106781186548,1.),(1.,
0.707106781186547,1.,0.707106781186547,1.,0.707106781186547,1.,0.707106781186547,
1.),(1.,0.707106781186547,1.,0.707106781186547,1.,0.707106781186547,1.,
0.707106781186547,1.),(1.,0.707106781186547,1.,0.707106781186547,1.,0.707106781186547,
1.,0.707106781186547,1.),(1.,0.707106781186547,1.,0.707106781186547,1.,
0.707106781186547,1.,0.707106781186547,1.),(1.,0.707106781186547,1.,0.707106781186547,
1.,0.707106781186547,1.,0.707106781186547,1.),(1.,0.707106781186548,1.,
0.707106781186548,1.,0.707106781186548,1.,0.707106781186548,1.),(1.,0.707106781186547,
1.,0.707106781186547,1.,0.707106781186547,1.,0.707106781186547,1.),(1.,
0.707106781186548,1.,0.707106781186548,1.,0.707106781186548,1.,0.707106781186548,
1.),(1.,0.707106781186547,1.,0.707106781186547,1.,0.707106781186547,1.,
0.707106781186547,1.),(1.,0.707106781186548,1.,0.707106781186548,1.,0.707106781186548,
1.,0.707106781186548,1.),(1.,0.707106781186547,1.,0.707106781186547,1.,
0.707106781186547,1.,0.707106781186547,1.),(1.,0.707106781186548,1.,0.707106781186548,
1.,0.707106781186548,1.,0.707106781186548,1.),(1.,0.707106781186547,1.,
0.707106781186547,1.,0.707106781186547,1.,0.707106781186547,1.),(1.,0.707106781186547,
1.,0.707106781186547,1.,0.707106781186547,1.,0.707106781186547,1.),(1.,
0.707106781186548,1.,0.707106781186548,1.,0.707106781186548,1.,0.707106781186548,
1.),(1.,0.707106781186547,1.,0.707106781186547,1.,0.707106781186547,1.,
0.707106781186547,1.),(1.,0.707106781186547,1.,0.707106781186547,1.,0.707106781186547,
1.,0.707106781186547,1.),(1.,0.707106781186548,1.,0.707106781186548,1.,
0.707106781186548,1.,0.707106781186548,1.),(1.,0.707106781186547,1.,0.707106781186547,
1.,0.707106781186547,1.,0.707106781186547,1.),(1.,0.707106781186548,1.,
0.707106781186548,1.,0.707106781186548,1.,0.707106781186548,1.),(1.,0.707106781186547,
1.,0.707106781186547,1.,0.707106781186547,1.,0.707106781186547,1.),(1.,
0.707106781186548,1.,0.707106781186548,1.,0.707106781186548,1.,0.707106781186548,
1.),(1.,0.707106781186548,1.,0.707106781186548,1.,0.707106781186548,1.,
0.707106781186548,1.),(1.,0.707106781186547,1.,0.707106781186547,1.,0.707106781186547,
1.,0.707106781186547,1.),(1.,0.707106781186548,1.,0.707106781186548,1.,
0.707106781186548,1.,0.707106781186548,1.),(1.,0.707106781186547,1.,0.707106781186547,
1.,0.707106781186547,1.,0.707106781186547,1.),(1.,0.707106781186547,1.,
0.707106781186547,1.,0.707106781186547,1.,0.707106781186547,1.),(1.,0.707106781186548,
1.,0.707106781186548,1.,0.707106781186548,1.,0.707106781186548,1.),(1.,
0.707106781186547,1.,0.707106781186547,1.,0.707106781186547,1.,0.707106781186547,
1.),(1.,0.707106781186547,1.,0.707106781186547,1.,0.707106781186547,1.,
0.707106781186547,1.),(1.,0.707106781186547,1.,0.707106781186547,1.,0.707106781186547,
1.,0.707106781186547,1.),(1.,0.707106781186548,1.,0.707106781186548,1.,
0.707106781186548,1.,0.707106781186548,1.),(1.,0.707106781186547,1.,0.707106781186547,
1.,0.707106781186547,1.,0.707106781186547,1.),(1.,0.707106781186547,1.,
0.707106781186547,1.,0.707106781186547,1.,0.707106781186547,1.),(1.,0.707106781186547,
1.,0.707106781186547,1.,0.707106781186547,1.,0.707106781186547,1.),(1.,
0.707106781186547,1.,0.707106781186547,1.,0.707106781186547,1.,0.707106781186547,
1.),(1.,0.707106781186547,1.,0.707106781186547,1.,0.707106781186547,1.,
0.707106781186547,1.),(1.,0.707106781186547,1.,0.707106781186547,1.,0.707106781186547,
1.,0.707106781186547,1.),(1.,0.707106781186548,1.,0.707106781186548,1.,
0.707106781186548,1.,0.707106781186548,1.),(1.,0.707106781186548,1.,0.707106781186548,
1.,0.707106781186548,1.,0.707106781186548,1.),(1.,0.707106781186547,1.,
0.707106781186547,1.,0.707106781186547,1.,0.707106781186547,1.),(1.,0.707106781186548,
1.,0.707106781186548,1.,0.707106781186548,1.,0.707106781186548,1.),(1.,
0.707106781186547,1.,0.707106781186547,1.,0.707106781186547,1.,0.707106781186547,
1.),(1.,0.707106781186548,1.,0.707106781186548,1.,0.707106781186548,1.,
0.707106781186548,1.),(1.,0.707106781186548,1.,0.707106781186548,1.,0.707106781186548,
1.,0.707106781186548,1.),(1.,0.707106781186547,1.,0.707106781186547,1.,
0.707106781186547,1.,0.707106781186547,1.),(1.,0.707106781186548,1.,0.707106781186548,
1.,0.707106781186548,1.,0.707106781186548,1.),(1.,0.707106781186548,1.,
0.707106781186548,1.,0.707106781186548,1.,0.707106781186548,1.),(1.,0.707106781186548,
1.,0.707106781186548,1.,0.707106781186548,1.,0.707106781186548,1.),(1.,
0.707106781186547,1.,0.707106781186547,1.,0.707106781186547,1.,0.707106781186547,
1.),(1.,0.707106781186548,1.,0.707106781186548,1.,0.707106781186548,1.,
0.707106781186548,1.),(1.,0.707106781186547,1.,0.707106781186547,1.,0.707106781186547,
1.,0.707106781186547,1.),(1.,0.707106781186548,1.,0.707106781186548,1.,
0.707106781186548,1.,0.707106781186548,1.),(1.,0.707106781186548,1.,0.707106781186548,
1.,0.707106781186548,1.,0.707106781186548,1.),(1.,0.707106781186548,1.,
0.707106781186548,1.,0.707106781186548,1.,0.707106781186548,1.),(1.,0.707106781186547,
1.,0.707106781186547,1.,0.707106781186547,1.,0.707106781186547,1.),(1.,
0.707106781186547,1.,0.707106781186547,1.,0.707106781186547,1.,0.707106781186547,
1.),(1.,0.707106781186547,1.,0.707106781186547,1.,0.707106781186547,1.,
0.707106781186547,1.),(1.,0.707106781186548,1.,0.707106781186548,1.,0.707106781186548,
1.,0.707106781186548,1.),(1.,0.707106781186548,1.,0.707106781186548,1.,
0.707106781186548,1.,0.707106781186548,1.),(1.,0.707106781186548,1.,0.707106781186548,
1.,0.707106781186548,1.,0.707106781186548,1.),(1.,0.707106781186547,1.,
0.707106781186547,1.,0.707106781186547,1.,0.707106781186547,1.),(1.,0.707106781186547,
1.,0.707106781186547,1.,0.707106781186547,1.,0.707106781186547,1.),(1.,
0.707106781186547,1.,0.707106781186547,1.,0.707106781186547,1.,0.707106781186547,
1.),(1.,0.707106781186548,1.,0.707106781186548,1.,0.707106781186548,1.,
0.707106781186548,1.),(1.,0.707106781186548,1.,0.707106781186548,1.,0.707106781186548,
1.,0.707106781186548,1.),(1.,0.707106781186547,1.,0.707106781186547,1.,
0.707106781186547,1.,0.707106781186547,1.),(1.,0.707106781186547,1.,0.707106781186547,
1.,0.707106781186547,1.,0.707106781186547,1.),(1.,0.707106781186548,1.,
0.707106781186548,1.,0.707106781186548,1.,0.707106781186548,1.),(1.,0.707106781186547,
1.,0.707106781186547,1.,0.707106781186547,1.,0.707106781186547,1.),(1.,
0.707106781186547,1.,0.707106781186547,1.,0.707106781186547,1.,0.707106781186547,
1.),(1.,0.707106781186547,1.,0.707106781186547,1.,0.707106781186547,1.,
0.707106781186547,1.),(1.,0.707106781186547,1.,0.707106781186547,1.,0.707106781186547,
1.,0.707106781186547,1.),(1.,0.707106781186548,1.,0.707106781186548,1.,
0.707106781186548,1.,0.707106781186548,1.),(1.,0.707106781186547,1.,0.707106781186547,
1.,0.707106781186547,1.,0.707106781186547,1.),(1.,0.707106781186548,1.,
0.707106781186548,1.,0.707106781186548,1.,0.707106781186548,1.),(1.,0.707106781186547,
1.,0.707106781186547,1.,0.707106781186547,1.,0.707106781186547,1.),(1.,
0.707106781186547,1.,0.707106781186547,1.,0.707106781186547,1.,0.707106781186547,
1.),(1.,0.707106781186547,1.,0.707106781186547,1.,0.707106781186547,1.,
0.707106781186547,1.),(1.,0.707106781186548,1.,0.707106781186548,1.,0.707106781186548,
1.,0.707106781186548,1.),(1.,0.707106781186548,1.,0.707106781186548,1.,
0.707106781186548,1.,0.707106781186548,1.),(1.,0.707106781186547,1.,0.707106781186547,
1.,0.707106781186547,1.,0.707106781186547,1.),(1.,0.707106781186548,1.,
0.707106781186548,1.,0.707106781186548,1.,0.707106781186548,1.),(1.,0.707106781186548,
1.,0.707106781186548,1.,0.707106781186548,1.,0.707106781186548,1.),(1.,
0.707106781186547,1.,0.707106781186547,1.,0.707106781186547,1.,0.707106781186547,
1.),(1.,0.707106781186548,1.,0.707106781186548,1.,0.707106781186548,1.,
0.707106781186548,1.),(1.,0.707106781186547,1.,0.707106781186547,1.,0.707106781186547,
1.,0.707106781186547,1.),(1.,0.707106781186548,1.,0.707106781186548,1.,
0.707106781186548,1.,0.707106781186548,1.),(1.,0.707106781186547,1.,0.707106781186547,
1.,0.707106781186547,1.,0.707106781186547,1.),(1.,0.707106781186548,1.,
0.707106781186548,1.,0.707106781186548,1.,0.707106781186548,1.),(1.,0.707106781186547,
1.,0.707106781186547,1.,0.707106781186547,1.,0.707106781186547,1.),(1.,
0.707106781186547,1.,0.707106781186547,1.,0.707106781186547,1.,0.707106781186547,
1.),(1.,0.707106781186548,1.,0.707106781186548,1.,0.707106781186548,1.,
0.707106781186548,1.),(1.,0.707106781186547,1.,0.707106781186547,1.,0.707106781186547,
1.,0.707106781186547,1.),(1.,0.707106781186547,1.,0.707106781186547,1.,
0.707106781186547,1.,0.707106781186547,1.),(1.,0.707106781186548,1.,0.707106781186548,
1.,0.707106781186548,1.,0.707106781186548,1.),(1.,0.707106781186547,1.,
0.707106781186547,1.,0.707106781186547,1.,0.707106781186547,1.),(1.,0.707106781186547,
1.,0.707106781186547,1.,0.707106781186547,1.,0.707106781186547,1.),(1.,
0.707106781186548,1.,0.707106781186548,1.,0.707106781186548,1.,0.707106781186548,
1.),(1.,0.707106781186547,1.,0.707106781186547,1.,0.707106781186547,1.,
0.707106781186547,1.),(1.,0.707106781186548,1.,0.707106781186548,1.,0.707106781186548,
1.,0.707106781186548,1.),(1.,0.707106781186547,1.,0.707106781186547,1.,
0.707106781186547,1.,0.707106781186547,1.),(1.,0.707106781186547,1.,0.707106781186547,
1.,0.707106781186547,1.,0.707106781186547,1.),(1.,0.707106781186548,1.,
0.707106781186548,1.,0.707106781186548,1.,0.707106781186548,1.),(1.,0.707106781186548,
1.,0.707106781186548,1.,0.707106781186548,1.,0.707106781186548,1.),(1.,
0.707106781186547,1.,0.707106781186547,1.,0.707106781186547,1.,0.707106781186547,
1.),(1.,0.707106781186548,1.,0.707106781186548,1.,0.707106781186548,1.,
0.707106781186548,1.),(1.,0.707106781186547,1.,0.707106781186547,1.,0.707106781186547,
1.,0.707106781186547,1.),(1.,0.707106781186548,1.,0.707106781186548,1.,
0.707106781186548,1.,0.707106781186548,1.),(1.,0.707106781186547,1.,0.707106781186547,
1.,0.707106781186547,1.,0.707106781186547,1.),(1.,0.707106781186548,1.,
0.707106781186548,1.,0.707106781186548,1.,0.707106781186548,1.),(1.,0.707106781186547,
1.,0.707106781186547,1.,0.707106781186547,1.,0.707106781186547,1.),(1.,
0.707106781186548,1.,0.707106781186548,1.,0.707106781186548,1.,0.707106781186548,
1.),(1.,0.707106781186547,1.,0.707106781186547,1.,0.707106781186547,1.,
0.707106781186547,1.),(1.,0.707106781186548,1.,0.707106781186548,1.,0.707106781186548,
1.,0.707106781186548,1.),(1.,0.707106781186547,1.,0.707106781186547,1.,
0.707106781186547,1.,0.707106781186547,1.),(1.,0.707106781186548,1.,0.707106781186548,
1.,0.707106781186548,1.,0.707106781186548,1.),(1.,0.707106781186547,1.,
0.707106781186547,1.,0.707106781186547,1.,0.707106781186547,1.),(1.,0.707106781186548,
1.,0.707106781186548,1.,0.707106781186548,1.,0.707106781186548,1.),(1.,
0.707106781186547,1.,0.707106781186547,1.,0.707106781186547,1.,0.707106781186547,
1.),(1.,0.707106781186547,1.,0.707106781186547,1.,0.707106781186547,1.,
0.707106781186547,1.),(1.,0.707106781186548,1.,0.707106781186548,1.,0.707106781186548,
1.,0.707106781186548,1.),(1.,0.707106781186547,1.,0.707106781186547,1.,
0.707106781186547,1.,0.707106781186547,1.),(1.,0.707106781186548,1.,0.707106781186548,
1.,0.707106781186548,1.,0.707106781186548,1.),(1.,0.707106781186547,1.,
0.707106781186547,1.,0.707106781186547,1.,0.707106781186547,1.),(1.,0.707106781186548,
1.,0.707106781186548,1.,0.707106781186548,1.,0.707106781186548,1.),(1.,
0.707106781186547,1.,0.707106781186547,1.,0.707106781186547,1.,0.707106781186547,
1.),(1.,0.707106781186548,1.,0.707106781186548,1.,0.707106781186548,1.,
0.707106781186548,1.),(1.,0.707106781186547,1.,0.707106781186547,1.,0.707106781186547,
1.,0.707106781186547,1.),(1.,0.707106781186547,1.,0.707106781186547,1.,
0.707106781186547,1.,0.707106781186547,1.),(1.,0.707106781186548,1.,0.707106781186548,
1.,0.707106781186548,1.,0.707106781186548,1.),(1.,0.707106781186547,1.,
0.707106781186547,1.,0.707106781186547,1.,0.707106781186547,1.),(1.,0.707106781186548,
1.,0.707106781186548,1.,0.707106781186548,1.,0.707106781186548,1.),(1.,
0.707106781186548,1.,0.707106781186548,1.,0.707106781186548,1.,0.707106781186548,
1.),(1.,0.707106781186548,1.,0.707106781186548,1.,0.707106781186548,1.,
0.707106781186548,1.),(1.,0.707106781186547,1.,0.707106781186547,1.,0.707106781186547,
1.,0.707106781186547,1.),(1.,0.707106781186547,1.,0.707106781186547,1.,
0.707106781186547,1.,0.707106781186547,1.),(1.,0.707106781186547,1.,0.707106781186547,
1.,0.707106781186547,1.,0.707106781186547,1.),(1.,0.707106781186547,1.,
0.707106781186547,1.,0.707106781186547,1.,0.707106781186547,1.),(1.,0.707106781186548,
1.,0.707106781186548,1.,0.707106781186548,1.,0.707106781186548,1.),(1.,
0.707106781186547,1.,0.707106781186547,1.,0.707106781186547,1.,0.707106781186547,
1.),(1.,0.707106781186548,1.,0.707106781186548,1.,0.707106781186548,1.,
0.707106781186548,1.),(1.,0.707106781186548,1.,0.707106781186548,1.,0.707106781186548,
1.,0.707106781186548,1.),(1.,0.707106781186547,1.,0.707106781186547,1.,
0.707106781186547,1.,0.707106781186547,1.),(1.,0.707106781186547,1.,0.707106781186547,
1.,0.707106781186547,1.,0.707106781186547,1.),(1.,0.707106781186548,1.,
0.707106781186548,1.,0.707106781186548,1.,0.707106781186548,1.),(1.,0.707106781186548,
1.,0.707106781186548,1.,0.707106781186548,1.,0.707106781186548,1.),(1.,
0.707106781186547,1.,0.707106781186547,1.,0.707106781186547,1.,0.707106781186547,
1.),(1.,0.707106781186547,1.,0.707106781186547,1.,0.707106781186547,1.,
0.707106781186547,1.),(1.,0.707106781186548,1.,0.707106781186548,1.,0.707106781186548,
1.,0.707106781186548,1.),(1.,0.707106781186547,1.,0.707106781186547,1.,
0.707106781186547,1.,0.707106781186547,1.),(1.,0.707106781186548,1.,0.707106781186548,
1.,0.707106781186548,1.,0.707106781186548,1.),(1.,0.707106781186547,1.,
0.707106781186547,1.,0.707106781186547,1.,0.707106781186547,1.),(1.,0.707106781186547,
1.,0.707106781186547,1.,0.707106781186547,1.,0.707106781186547,1.),(1.,
0.707106781186547,1.,0.707106781186547,1.,0.707106781186547,1.,0.707106781186547,
1.),(1.,0.707106781186547,1.,0.707106781186547,1.,0.707106781186547,1.,
0.707106781186547,1.),(1.,0.707106781186547,1.,0.707106781186547,1.,0.707106781186547,
1.,0.707106781186547,1.),(1.,0.707106781186547,1.,0.707106781186547,1.,
0.707106781186547,1.,0.707106781186547,1.),(1.,0.707106781186547,1.,0.707106781186547,
1.,0.707106781186547,1.,0.707106781186547,1.),(1.,0.707106781186548,1.,
0.707106781186548,1.,0.707106781186548,1.,0.707106781186548,1.),(1.,0.707106781186547,
1.,0.707106781186547,1.,0.707106781186547,1.,0.707106781186547,1.),(1.,
0.707106781186548,1.,0.707106781186548,1.,0.707106781186548,1.,0.707106781186548,
1.),(1.,0.707106781186547,1.,0.707106781186547,1.,0.707106781186547,1.,
0.707106781186547,1.),(1.,0.707106781186548,1.,0.707106781186548,1.,0.707106781186548,
1.,0.707106781186548,1.),(1.,0.707106781186548,1.,0.707106781186548,1.,
0.707106781186548,1.,0.707106781186548,1.),(1.,0.707106781186547,1.,0.707106781186547,
1.,0.707106781186547,1.,0.707106781186547,1.),(1.,0.707106781186548,1.,
0.707106781186548,1.,0.707106781186548,1.,0.707106781186548,1.),(1.,0.707106781186548,
1.,0.707106781186548,1.,0.707106781186548,1.,0.707106781186548,1.),(1.,
0.707106781186548,1.,0.707106781186548,1.,0.707106781186548,1.,0.707106781186548,
1.),(1.,0.707106781186548,1.,0.707106781186548,1.,0.707106781186548,1.,
0.707106781186548,1.),(1.,0.707106781186547,1.,0.707106781186547,1.,0.707106781186547,
1.,0.707106781186547,1.),(1.,0.707106781186548,1.,0.707106781186548,1.,
0.707106781186548,1.,0.707106781186548,1.),(1.,0.707106781186547,1.,0.707106781186547,
1.,0.707106781186547,1.,0.707106781186547,1.),(1.,0.707106781186548,1.,
0.707106781186548,1.,0.707106781186548,1.,0.707106781186548,1.),(1.,0.707106781186547,
1.,0.707106781186547,1.,0.707106781186547,1.,0.707106781186547,1.),(1.,
0.707106781186547,1.,0.707106781186547,1.,0.707106781186547,1.,0.707106781186547,
1.),(1.,0.707106781186548,1.,0.707106781186548,1.,0.707106781186548,1.,
0.707106781186548,1.),(1.,0.707106781186548,1.,0.707106781186548,1.,0.707106781186548,
1.,0.707106781186548,1.),(1.,0.707106781186547,1.,0.707106781186547,1.,
0.707106781186547,1.,0.707106781186547,1.),(1.,0.707106781186547,1.,0.707106781186547,
1.,0.707106781186547,1.,0.707106781186547,1.),(1.,0.707106781186547,1.,
0.707106781186547,1.,0.707106781186547,1.,0.707106781186547,1.),(1.,0.707106781186547,
1.,0.707106781186547,1.,0.707106781186547,1.,0.707106781186547,1.),(1.,
0.707106781186547,1.,0.707106781186547,1.,0.707106781186547,1.,0.707106781186547,
1.),(1.,0.707106781186548,1.,0.707106781186548,1.,0.707106781186548,1.,
0.707106781186548,1.),(1.,0.707106781186548,1.,0.707106781186548,1.,0.707106781186548,
1.,0.707106781186548,1.),(1.,0.707106781186547,1.,0.707106781186547,1.,
0.707106781186547,1.,0.707106781186547,1.),(1.,0.707106781186547,1.,0.707106781186547,
1.,0.707106781186547,1.,0.707106781186547,1.),(1.,0.707106781186548,1.,
0.707106781186548,1.,0.707106781186548,1.,0.707106781186548,1.),(1.,0.707106781186548,
1.,0.707106781186548,1.,0.707106781186548,1.,0.707106781186548,1.),(1.,
0.707106781186547,1.,0.707106781186547,1.,0.707106781186547,1.,0.707106781186547,
1.),(1.,0.707106781186548,1.,0.707106781186548,1.,0.707106781186548,1.,
0.707106781186548,1.),(1.,0.707106781186547,1.,0.707106781186547,1.,0.707106781186547,
1.,0.707106781186547,1.),(1.,0.707106781186548,1.,0.707106781186548,1.,
0.707106781186548,1.,0.707106781186548,1.),(1.,0.707106781186548,1.,0.707106781186548,
1.,0.707106781186548,1.,0.707106781186548,1.),(1.,0.707106781186547,1.,
0.707106781186547,1.,0.707106781186547,1.,0.707106781186547,1.),(1.,0.707106781186547,
1.,0.707106781186547,1.,0.707106781186547,1.,0.707106781186547,1.),(1.,
0.707106781186548,1.,0.707106781186548,1.,0.707106781186548,1.,0.707106781186548,
1.),(1.,0.707106781186547,1.,0.707106781186547,1.,0.707106781186547,1.,
0.707106781186547,1.),(1.,0.707106781186547,1.,0.707106781186547,1.,0.707106781186547,
1.,0.707106781186547,1.),(1.,0.707106781186548,1.,0.707106781186548,1.,
0.707106781186548,1.,0.707106781186548,1.),(1.,0.707106781186547,1.,0.707106781186547,
1.,0.707106781186547,1.,0.707106781186547,1.),(1.,0.707106781186548,1.,
0.707106781186548,1.,0.707106781186548,1.,0.707106781186548,1.),(1.,0.707106781186547,
1.,0.707106781186547,1.,0.707106781186547,1.,0.707106781186547,1.),(1.,
0.707106781186548,1.,0.707106781186548,1.,0.707106781186548,1.,0.707106781186548,
1.),(1.,0.707106781186547,1.,0.707106781186547,1.,0.707106781186547,1.,
0.707106781186547,1.),(1.,0.707106781186547,1.,0.707106781186547,1.,0.707106781186547,
1.,0.707106781186547,1.),(1.,0.707106781186548,1.,0.707106781186548,1.,
0.707106781186548,1.,0.707106781186548,1.),(1.,0.707106781186548,1.,0.707106781186548,
1.,0.707106781186548,1.,0.707106781186548,1.),(1.,0.707106781186547,1.,
0.707106781186547,1.,0.707106781186547,1.,0.707106781186547,1.),(1.,0.707106781186547,
1.,0.707106781186547,1.,0.707106781186547,1.,0.707106781186547,1.),(1.,
0.707106781186548,1.,0.707106781186548,1.,0.707106781186548,1.,0.707106781186548,
1.),(1.,0.707106781186547,1.,0.707106781186547,1.,0.707106781186547,1.,
0.707106781186547,1.),(1.,0.707106781186547,1.,0.707106781186547,1.,0.707106781186547,
1.,0.707106781186547,1.),(1.,0.707106781186548,1.,0.707106781186548,1.,
0.707106781186548,1.,0.707106781186548,1.),(1.,0.707106781186547,1.,0.707106781186547,
1.,0.707106781186547,1.,0.707106781186547,1.),(1.,0.707106781186548,1.,
0.707106781186548,1.,0.707106781186548,1.,0.707106781186548,1.),(1.,0.707106781186547,
1.,0.707106781186547,1.,0.707106781186547,1.,0.707106781186547,1.),(1.,
0.707106781186548,1.,0.707106781186548,1.,0.707106781186548,1.,0.707106781186548,
1.),(1.,0.707106781186547,1.,0.707106781186547,1.,0.707106781186547,1.,
0.707106781186547,1.),(1.,0.707106781186548,1.,0.707106781186548,1.,0.707106781186548,
1.,0.707106781186548,1.),(1.,0.707106781186547,1.,0.707106781186547,1.,
0.707106781186547,1.,0.707106781186547,1.),(1.,0.707106781186547,1.,0.707106781186547,
1.,0.707106781186547,1.,0.707106781186547,1.),(1.,0.707106781186547,1.,
0.707106781186547,1.,0.707106781186547,1.,0.707106781186547,1.),(1.,0.707106781186547,
1.,0.707106781186547,1.,0.707106781186547,1.,0.707106781186547,1.),(1.,
0.707106781186547,1.,0.707106781186547,1.,0.707106781186547,1.,0.707106781186547,
1.),(1.,0.707106781186547,1.,0.707106781186547,1.,0.707106781186547,1.,
0.707106781186547,1.),(1.,0.707106781186548,1.,0.707106781186548,1.,0.707106781186548,
1.,0.707106781186548,1.),(1.,0.707106781186547,1.,0.707106781186547,1.,
0.707106781186547,1.,0.707106781186547,1.),(1.,0.707106781186548,1.,0.707106781186548,
1.,0.707106781186548,1.,0.707106781186548,1.),(1.,0.707106781186547,1.,
0.707106781186547,1.,0.707106781186547,1.,0.707106781186547,1.),(1.,0.707106781186548,
1.,0.707106781186548,1.,0.707106781186548,1.,0.707106781186548,1.),(1.,
0.707106781186548,1.,0.707106781186548,1.,0.707106781186548,1.,0.707106781186548,
1.),(1.,0.707106781186547,1.,0.707106781186547,1.,0.707106781186547,1.,
0.707106781186547,1.),(1.,0.707106781186548,1.,0.707106781186548,1.,0.707106781186548,
1.,0.707106781186548,1.),(1.,0.707106781186548,1.,0.707106781186548,1.,
0.707106781186548,1.,0.707106781186548,1.),(1.,0.707106781186547,1.,0.707106781186547,
1.,0.707106781186547,1.,0.707106781186547,1.),(1.,0.707106781186548,1.,
0.707106781186548,1.,0.707106781186548,1.,0.707106781186548,1.),(1.,0.707106781186547,
1.,0.707106781186547,1.,0.707106781186547,1.,0.707106781186547,1.),(1.,
0.707106781186547,1.,0.707106781186547,1.,0.707106781186547,1.,0.707106781186547,
1.),(1.,0.707106781186547,1.,0.707106781186547,1.,0.707106781186547,1.,
0.707106781186547,1.),(1.,0.707106781186548,1.,0.707106781186548,1.,0.707106781186548,
1.,0.707106781186548,1.),(1.,0.707106781186547,1.,0.707106781186547,1.,
0.707106781186547,1.,0.707106781186547,1.),(1.,0.707106781186547,1.,0.707106781186547,
1.,0.707106781186547,1.,0.707106781186547,1.),(1.,0.707106781186548,1.,
0.707106781186548,1.,0.707106781186548,1.,0.707106781186548,1.),(1.,0.707106781186547,
1.,0.707106781186547,1.,0.707106781186547,1.,0.707106781186547,1.),(1.,
0.707106781186548,1.,0.707106781186548,1.,0.707106781186548,1.,0.707106781186548,
1.),(1.,0.707106781186547,1.,0.707106781186547,1.,0.707106781186547,1.,
0.707106781186547,1.),(1.,0.707106781186547,1.,0.707106781186547,1.,0.707106781186547,
1.,0.707106781186547,1.),(1.,0.707106781186547,1.,0.707106781186547,1.,
0.707106781186547,1.,0.707106781186547,1.),(1.,0.707106781186548,1.,0.707106781186548,
1.,0.707106781186548,1.,0.707106781186548,1.),(1.,0.707106781186548,1.,
0.707106781186548,1.,0.707106781186548,1.,0.707106781186548,1.),(1.,0.707106781186547,
1.,0.707106781186547,1.,0.707106781186547,1.,0.707106781186547,1.),(1.,
0.707106781186548,1.,0.707106781186548,1.,0.707106781186548,1.,0.707106781186548,
1.),(1.,0.707106781186548,1.,0.707106781186548,1.,0.707106781186548,1.,
0.707106781186548,1.),(1.,0.707106781186547,1.,0.707106781186547,1.,0.707106781186547,
1.,0.707106781186547,1.),(1.,0.707106781186548,1.,0.707106781186548,1.,
0.707106781186548,1.,0.707106781186548,1.),(1.,0.707106781186547,1.,0.707106781186547,
1.,0.707106781186547,1.,0.707106781186547,1.),(1.,0.707106781186548,1.,
0.707106781186548,1.,0.707106781186548,1.,0.707106781186548,1.),(1.,0.707106781186548,
1.,0.707106781186548,1.,0.707106781186548,1.,0.707106781186548,1.),(1.,
0.707106781186547,1.,0.707106781186547,1.,0.707106781186547,1.,0.707106781186547,
1.),(1.,0.707106781186548,1.,0.707106781186548,1.,0.707106781186548,1.,
0.707106781186548,1.),(1.,0.707106781186548,1.,0.707106781186548,1.,0.707106781186548,
1.,0.707106781186548,1.),(1.,0.707106781186548,1.,0.707106781186548,1.,
0.707106781186548,1.,0.707106781186548,1.),(1.,0.707106781186547,1.,0.707106781186547,
1.,0.707106781186547,1.,0.707106781186547,1.),(1.,0.707106781186547,1.,
0.707106781186547,1.,0.707106781186547,1.,0.707106781186547,1.),(1.,0.707106781186548,
1.,0.707106781186548,1.,0.707106781186548,1.,0.707106781186548,1.),(1.,
0.707106781186547,1.,0.707106781186547,1.,0.707106781186547,1.,0.707106781186547,
1.),(1.,0.707106781186548,1.,0.707106781186548,1.,0.707106781186548,1.,
0.707106781186548,1.),(1.,0.707106781186547,1.,0.707106781186547,1.,0.707106781186547,
1.,0.707106781186547,1.),(1.,0.707106781186547,1.,0.707106781186547,1.,
0.707106781186547,1.,0.707106781186547,1.),(1.,0.707106781186548,1.,0.707106781186548,
1.,0.707106781186548,1.,0.707106781186548,1.),(1.,0.707106781186548,1.,
0.707106781186548,1.,0.707106781186548,1.,0.707106781186548,1.),(1.,0.707106781186548,
1.,0.707106781186548,1.,0.707106781186548,1.,0.707106781186548,1.),(1.,
0.707106781186547,1.,0.707106781186547,1.,0.707106781186547,1.,0.707106781186547,
1.),(1.,0.707106781186547,1.,0.707106781186547,1.,0.707106781186547,1.,
0.707106781186547,1.),(1.,0.707106781186548,1.,0.707106781186548,1.,0.707106781186548,
1.,0.707106781186548,1.),(1.,0.707106781186548,1.,0.707106781186548,1.,
0.707106781186548,1.,0.707106781186548,1.),(1.,0.707106781186547,1.,0.707106781186547,
1.,0.707106781186547,1.,0.707106781186547,1.),(1.,0.707106781186547,1.,
0.707106781186547,1.,0.707106781186547,1.,0.707106781186547,1.),(1.,0.707106781186548,
1.,0.707106781186548,1.,0.707106781186548,1.,0.707106781186548,1.),(1.,
0.707106781186547,1.,0.707106781186547,1.,0.707106781186547,1.,0.707106781186547,
1.),(1.,0.707106781186547,1.,0.707106781186547,1.,0.707106781186547,1.,
0.707106781186547,1.),(1.,0.707106781186548,1.,0.707106781186548,1.,0.707106781186548,
1.,0.707106781186548,1.),(1.,0.707106781186548,1.,0.707106781186548,1.,
0.707106781186548,1.,0.707106781186548,1.),(1.,0.707106781186547,1.,0.707106781186547,
1.,0.707106781186547,1.,0.707106781186547,1.),(1.,0.707106781186547,1.,
0.707106781186547,1.,0.707106781186547,1.,0.707106781186547,1.),(1.,0.707106781186547,
1.,0.707106781186547,1.,0.707106781186547,1.,0.707106781186547,1.),(1.,
0.707106781186548,1.,0.707106781186548,1.,0.707106781186548,1.,0.707106781186548,
1.),(1.,0.707106781186547,1.,0.707106781186547,1.,0.707106781186547,1.,
0.707106781186547,1.),(1.,0.707106781186547,1.,0.707106781186547,1.,0.707106781186547,
1.,0.707106781186547,1.),(1.,0.707106781186547,1.,0.707106781186547,1.,
0.707106781186547,1.,0.707106781186547,1.),(1.,0.707106781186548,1.,0.707106781186548,
1.,0.707106781186548,1.,0.707106781186548,1.),(1.,0.707106781186548,1.,
0.707106781186548,1.,0.707106781186548,1.,0.707106781186548,1.),(1.,0.707106781186547,
1.,0.707106781186547,1.,0.707106781186547,1.,0.707106781186547,1.),(1.,
0.707106781186548,1.,0.707106781186548,1.,0.707106781186548,1.,0.707106781186548,
1.),(1.,0.707106781186547,1.,0.707106781186547,1.,0.707106781186547,1.,
0.707106781186547,1.),(1.,0.707106781186548,1.,0.707106781186548,1.,0.707106781186548,
1.,0.707106781186548,1.),(1.,0.707106781186547,1.,0.707106781186547,1.,
0.707106781186547,1.,0.707106781186547,1.),(1.,0.707106781186548,1.,0.707106781186548,
1.,0.707106781186548,1.,0.707106781186548,1.),(1.,0.707106781186548,1.,
0.707106781186548,1.,0.707106781186548,1.,0.707106781186548,1.),(1.,0.707106781186547,
1.,0.707106781186547,1.,0.707106781186547,1.,0.707106781186547,1.),(1.,
0.707106781186547,1.,0.707106781186547,1.,0.707106781186547,1.,0.707106781186547,
1.),(1.,0.707106781186548,1.,0.707106781186548,1.,0.707106781186548,1.,
0.707106781186548,1.),(1.,0.707106781186547,1.,0.707106781186547,1.,0.707106781186547,
1.,0.707106781186547,1.),(1.,0.707106781186547,1.,0.707106781186547,1.,
0.707106781186547,1.,0.707106781186547,1.),(1.,0.707106781186548,1.,0.707106781186548,
1.,0.707106781186548,1.,0.707106781186548,1.),(1.,0.707106781186547,1.,
0.707106781186547,1.,0.707106781186547,1.,0.707106781186547,1.),(1.,0.707106781186548,
1.,0.707106781186548,1.,0.707106781186548,1.,0.707106781186548,1.),(1.,
0.707106781186548,1.,0.707106781186548,1.,0.707106781186548,1.,0.707106781186548,
1.),(1.,0.707106781186547,1.,0.707106781186547,1.,0.707106781186547,1.,
0.707106781186547,1.),(1.,0.707106781186548,1.,0.707106781186548,1.,0.707106781186548,
1.,0.707106781186548,1.),(1.,0.707106781186547,1.,0.707106781186547,1.,
0.707106781186547,1.,0.707106781186547,1.),(1.,0.707106781186547,1.,0.707106781186547,
1.,0.707106781186547,1.,0.707106781186547,1.),(1.,0.707106781186547,1.,
0.707106781186547,1.,0.707106781186547,1.,0.707106781186547,1.),(1.,0.707106781186548,
1.,0.707106781186548,1.,0.707106781186548,1.,0.707106781186548,1.),(1.,
0.707106781186548,1.,0.707106781186548,1.,0.707106781186548,1.,0.707106781186548,
1.),(1.,0.707106781186548,1.,0.707106781186548,1.,0.707106781186548,1.,
0.707106781186548,1.),(1.,0.707106781186547,1.,0.707106781186547,1.,0.707106781186547,
1.,0.707106781186547,1.),(1.,0.707106781186548,1.,0.707106781186548,1.,
0.707106781186548,1.,0.707106781186548,1.),(1.,0.707106781186547,1.,0.707106781186547,
1.,0.707106781186547,1.,0.707106781186547,1.),(1.,0.707106781186548,1.,
0.707106781186548,1.,0.707106781186548,1.,0.707106781186548,1.),(1.,0.707106781186547,
1.,0.707106781186547,1.,0.707106781186547,1.,0.707106781186547,1.),(1.,
0.707106781186547,1.,0.707106781186547,1.,0.707106781186547,1.,0.707106781186547,
1.),(1.,0.707106781186547,1.,0.707106781186547,1.,0.707106781186547,1.,
0.707106781186547,1.),(1.,0.707106781186547,1.,0.707106781186547,1.,0.707106781186547,
1.,0.707106781186547,1.),(1.,0.707106781186548,1.,0.707106781186548,1.,
0.707106781186548,1.,0.707106781186548,1.),(1.,0.707106781186548,1.,0.707106781186548,
1.,0.707106781186548,1.,0.707106781186548,1.),(1.,0.707106781186547,1.,
0.707106781186547,1.,0.707106781186547,1.,0.707106781186547,1.),(1.,0.707106781186547,
1.,0.707106781186547,1.,0.707106781186547,1.,0.707106781186547,1.),(1.,
0.707106781186548,1.,0.707106781186548,1.,0.707106781186548,1.,0.707106781186548,
1.),(1.,0.707106781186547,1.,0.707106781186547,1.,0.707106781186547,1.,
0.707106781186547,1.),(1.,0.707106781186548,1.,0.707106781186548,1.,0.707106781186548,
1.,0.707106781186548,1.),(1.,0.707106781186547,1.,0.707106781186547,1.,
0.707106781186547,1.,0.707106781186547,1.),(1.,0.707106781186548,1.,0.707106781186548,
1.,0.707106781186548,1.,0.707106781186548,1.),(1.,0.707106781186547,1.,
0.707106781186547,1.,0.707106781186547,1.,0.707106781186547,1.),(1.,0.707106781186547,
1.,0.707106781186547,1.,0.707106781186547,1.,0.707106781186547,1.),(1.,
0.707106781186548,1.,0.707106781186548,1.,0.707106781186548,1.,0.707106781186548,
1.),(1.,0.707106781186547,1.,0.707106781186547,1.,0.707106781186547,1.,
0.707106781186547,1.),(1.,0.707106781186548,1.,0.707106781186548,1.,0.707106781186548,
1.,0.707106781186548,1.),(1.,0.707106781186547,1.,0.707106781186547,1.,
0.707106781186547,1.,0.707106781186547,1.),(1.,0.707106781186548,1.,0.707106781186548,
1.,0.707106781186548,1.,0.707106781186548,1.),(1.,0.707106781186548,1.,
0.707106781186548,1.,0.707106781186548,1.,0.707106781186548,1.),(1.,0.707106781186547,
1.,0.707106781186547,1.,0.707106781186547,1.,0.707106781186547,1.),(1.,
0.707106781186548,1.,0.707106781186548,1.,0.707106781186548,1.,0.707106781186548,
1.),(1.,0.707106781186547,1.,0.707106781186547,1.,0.707106781186547,1.,
0.707106781186547,1.),(1.,0.707106781186548,1.,0.707106781186548,1.,0.707106781186548,
1.,0.707106781186548,1.),(1.,0.707106781186548,1.,0.707106781186548,1.,
0.707106781186548,1.,0.707106781186548,1.),(1.,0.707106781186547,1.,0.707106781186547,
1.,0.707106781186547,1.,0.707106781186547,1.),(1.,0.707106781186548,1.,
0.707106781186548,1.,0.707106781186548,1.,0.707106781186548,1.),(1.,0.707106781186547,
1.,0.707106781186547,1.,0.707106781186547,1.,0.707106781186547,1.),(1.,
0.707106781186547,1.,0.707106781186547,1.,0.707106781186547,1.,0.707106781186547,
1.),(1.,0.707106781186548,1.,0.707106781186548,1.,0.707106781186548,1.,
0.707106781186548,1.),(1.,0.707106781186547,1.,0.707106781186547,1.,0.707106781186547,
1.,0.707106781186547,1.),(1.,0.707106781186548,1.,0.707106781186548,1.,
0.707106781186548,1.,0.707106781186548,1.),(1.,0.707106781186547,1.,0.707106781186547,
1.,0.707106781186547,1.,0.707106781186547,1.),(1.,0.707106781186548,1.,
0.707106781186548,1.,0.707106781186548,1.,0.707106781186548,1.),(1.,0.707106781186547,
1.,0.707106781186547,1.,0.707106781186547,1.,0.707106781186547,1.),(1.,
0.707106781186547,1.,0.707106781186547,1.,0.707106781186547,1.,0.707106781186547,
1.),(1.,0.707106781186548,1.,0.707106781186548,1.,0.707106781186548,1.,
0.707106781186548,1.),(1.,0.707106781186548,1.,0.707106781186548,1.,0.707106781186548,
1.,0.707106781186548,1.),(1.,0.707106781186548,1.,0.707106781186548,1.,
0.707106781186548,1.,0.707106781186548,1.),(1.,0.707106781186548,1.,0.707106781186548,
1.,0.707106781186548,1.,0.707106781186548,1.),(1.,0.707106781186547,1.,
0.707106781186547,1.,0.707106781186547,1.,0.707106781186547,1.),(1.,0.707106781186548,
1.,0.707106781186548,1.,0.707106781186548,1.,0.707106781186548,1.),(1.,
0.707106781186548,1.,0.707106781186548,1.,0.707106781186548,1.,0.707106781186548,
1.),(1.,0.707106781186548,1.,0.707106781186548,1.,0.707106781186548,1.,
0.707106781186548,1.),(1.,0.707106781186547,1.,0.707106781186547,1.,0.707106781186547,
1.,0.707106781186547,1.),(1.,0.707106781186548,1.,0.707106781186548,1.,
0.707106781186548,1.,0.707106781186548,1.),(1.,0.707106781186548,1.,0.707106781186548,
1.,0.707106781186548,1.,0.707106781186548,1.),(1.,0.707106781186548,1.,
0.707106781186548,1.,0.707106781186548,1.,0.707106781186548,1.),(1.,0.707106781186547,
1.,0.707106781186547,1.,0.707106781186547,1.,0.707106781186547,1.),(1.,
0.707106781186547,1.,0.707106781186547,1.,0.707106781186547,1.,0.707106781186547,
1.),(1.,0.707106781186548,1.,0.707106781186548,1.,0.707106781186548,1.,
0.707106781186548,1.),(1.,0.707106781186547,1.,0.707106781186547,1.,0.707106781186547,
1.,0.707106781186547,1.),(1.,0.707106781186548,1.,0.707106781186548,1.,
0.707106781186548,1.,0.707106781186548,1.),(1.,0.707106781186547,1.,0.707106781186547,
1.,0.707106781186547,1.,0.707106781186547,1.),(1.,0.707106781186548,1.,
0.707106781186548,1.,0.707106781186548,1.,0.707106781186548,1.),(1.,0.707106781186548,
1.,0.707106781186548,1.,0.707106781186548,1.,0.707106781186548,1.),(1.,
0.707106781186547,1.,0.707106781186547,1.,0.707106781186547,1.,0.707106781186547,
1.),(1.,0.707106781186547,1.,0.707106781186547,1.,0.707106781186547,1.,
0.707106781186547,1.),(1.,0.707106781186548,1.,0.707106781186548,1.,0.707106781186548,
1.,0.707106781186548,1.),(1.,0.707106781186547,1.,0.707106781186547,1.,
0.707106781186547,1.,0.707106781186547,1.),(1.,0.707106781186548,1.,0.707106781186548,
1.,0.707106781186548,1.,0.707106781186548,1.),(1.,0.707106781186547,1.,
0.707106781186547,1.,0.707106781186547,1.,0.707106781186547,1.),(1.,0.707106781186548,
1.,0.707106781186548,1.,0.707106781186548,1.,0.707106781186548,1.),(1.,
0.707106781186548,1.,0.707106781186548,1.,0.707106781186548,1.,0.707106781186548,
1.),(1.,0.707106781186547,1.,0.707106781186547,1.,0.707106781186547,1.,
0.707106781186547,1.),(1.,0.707106781186547,1.,0.707106781186547,1.,0.707106781186547,
1.,0.707106781186547,1.),(1.,0.707106781186547,1.,0.707106781186547,1.,
0.707106781186547,1.,0.707106781186547,1.),(1.,0.707106781186548,1.,0.707106781186548,
1.,0.707106781186548,1.,0.707106781186548,1.),(1.,0.707106781186548,1.,
0.707106781186548,1.,0.707106781186548,1.,0.707106781186548,1.),(1.,0.707106781186547,
1.,0.707106781186547,1.,0.707106781186547,1.,0.707106781186547,1.),(1.,
0.707106781186547,1.,0.707106781186547,1.,0.707106781186547,1.,0.707106781186547,
1.),(1.,0.707106781186548,1.,0.707106781186548,1.,0.707106781186548,1.,
0.707106781186548,1.),(1.,0.707106781186548,1.,0.707106781186548,1.,0.707106781186548,
1.,0.707106781186548,1.),(1.,0.707106781186548,1.,0.707106781186548,1.,
0.707106781186548,1.,0.707106781186548,1.),(1.,0.707106781186548,1.,0.707106781186548,
1.,0.707106781186548,1.,0.707106781186548,1.),(1.,0.707106781186547,1.,
0.707106781186547,1.,0.707106781186547,1.,0.707106781186547,1.),(1.,0.707106781186547,
1.,0.707106781186547,1.,0.707106781186547,1.,0.707106781186547,1.),(1.,
0.707106781186548,1.,0.707106781186548,1.,0.707106781186548,1.,0.707106781186548,
1.),(1.,0.707106781186548,1.,0.707106781186548,1.,0.707106781186548,1.,
0.707106781186548,1.),(1.,0.707106781186547,1.,0.707106781186547,1.,0.707106781186547,
1.,0.707106781186547,1.),(1.,0.707106781186548,1.,0.707106781186548,1.,
0.707106781186548,1.,0.707106781186548,1.),(1.,0.707106781186547,1.,0.707106781186547,
1.,0.707106781186547,1.,0.707106781186547,1.),(1.,0.707106781186548,1.,
0.707106781186548,1.,0.707106781186548,1.,0.707106781186548,1.),(1.,0.707106781186547,
1.,0.707106781186547,1.,0.707106781186547,1.,0.707106781186547,1.),(1.,
0.707106781186548,1.,0.707106781186548,1.,0.707106781186548,1.,0.707106781186548,
1.),(1.,0.707106781186547,1.,0.707106781186547,1.,0.707106781186547,1.,
0.707106781186547,1.),(1.,0.707106781186547,1.,0.707106781186547,1.,0.707106781186547,
1.,0.707106781186547,1.),(1.,0.707106781186548,1.,0.707106781186548,1.,
0.707106781186548,1.,0.707106781186548,1.),(1.,0.707106781186547,1.,0.707106781186547,
1.,0.707106781186547,1.,0.707106781186547,1.),(1.,0.707106781186547,1.,
0.707106781186547,1.,0.707106781186547,1.,0.707106781186547,1.),(1.,0.707106781186548,
1.,0.707106781186548,1.,0.707106781186548,1.,0.707106781186548,1.),(1.,
0.707106781186547,1.,0.707106781186547,1.,0.707106781186547,1.,0.707106781186547,
1.),(1.,0.707106781186548,1.,0.707106781186548,1.,0.707106781186548,1.,
0.707106781186548,1.),(1.,0.707106781186547,1.,0.707106781186547,1.,0.707106781186547,
1.,0.707106781186547,1.),(1.,0.707106781186548,1.,0.707106781186548,1.,
0.707106781186548,1.,0.707106781186548,1.),(1.,0.707106781186547,1.,0.707106781186547,
1.,0.707106781186547,1.,0.707106781186547,1.),(1.,0.707106781186548,1.,
0.707106781186548,1.,0.707106781186548,1.,0.707106781186548,1.),(1.,0.707106781186547,
1.,0.707106781186547,1.,0.707106781186547,1.,0.707106781186547,1.),(1.,
0.707106781186548,1.,0.707106781186548,1.,0.707106781186548,1.,0.707106781186548,
1.),(1.,0.707106781186547,1.,0.707106781186547,1.,0.707106781186547,1.,
0.707106781186547,1.),(1.,0.707106781186548,1.,0.707106781186548,1.,0.707106781186548,
1.,0.707106781186548,1.),(1.,0.707106781186547,1.,0.707106781186547,1.,
0.707106781186547,1.,0.707106781186547,1.),(1.,0.707106781186547,1.,0.707106781186547,
1.,0.707106781186547,1.,0.707106781186547,1.),(1.,0.707106781186548,1.,
0.707106781186548,1.,0.707106781186548,1.,0.707106781186548,1.),(1.,0.707106781186548,
1.,0.707106781186548,1.,0.707106781186548,1.,0.707106781186548,1.),(1.,
0.707106781186547,1.,0.707106781186547,1.,0.707106781186547,1.,0.707106781186547,
1.),(1.,0.707106781186547,1.,0.707106781186547,1.,0.707106781186547,1.,
0.707106781186547,1.),(1.,0.707106781186547,1.,0.707106781186547,1.,0.707106781186547,
1.,0.707106781186547,1.),(1.,0.707106781186548,1.,0.707106781186548,1.,
0.707106781186548,1.,0.707106781186548,1.),(1.,0.707106781186547,1.,0.707106781186547,
1.,0.707106781186547,1.,0.707106781186547,1.),(1.,0.707106781186548,1.,
0.707106781186548,1.,0.707106781186548,1.,0.707106781186548,1.),(1.,0.707106781186547,
1.,0.707106781186547,1.,0.707106781186547,1.,0.707106781186547,1.),(1.,
0.707106781186548,1.,0.707106781186548,1.,0.707106781186548,1.,0.707106781186548,
1.),(1.,0.707106781186547,1.,0.707106781186547,1.,0.707106781186547,1.,
0.707106781186547,1.),(1.,0.707106781186548,1.,0.707106781186548,1.,0.707106781186548,
1.,0.707106781186548,1.),(1.,0.707106781186547,1.,0.707106781186547,1.,
0.707106781186547,1.,0.707106781186547,1.),(1.,0.707106781186547,1.,0.707106781186547,
1.,0.707106781186547,1.,0.707106781186547,1.),(1.,0.707106781186547,1.,
0.707106781186547,1.,0.707106781186547,1.,0.707106781186547,1.),(1.,0.707106781186548,
1.,0.707106781186548,1.,0.707106781186548,1.,0.707106781186548,1.),(1.,
0.707106781186547,1.,0.707106781186547,1.,0.707106781186547,1.,0.707106781186547,
1.),(1.,0.707106781186548,1.,0.707106781186548,1.,0.707106781186548,1.,
0.707106781186548,1.),(1.,0.707106781186548,1.,0.707106781186548,1.,0.707106781186548,
1.,0.707106781186548,1.),(1.,0.707106781186547,1.,0.707106781186547,1.,
0.707106781186547,1.,0.707106781186547,1.),(1.,0.707106781186548,1.,0.707106781186548,
1.,0.707106781186548,1.,0.707106781186548,1.),(1.,0.707106781186547,1.,
0.707106781186547,1.,0.707106781186547,1.,0.707106781186547,1.),(1.,0.707106781186547,
1.,0.707106781186547,1.,0.707106781186547,1.,0.707106781186547,1.),(1.,
0.707106781186548,1.,0.707106781186548,1.,0.707106781186548,1.,0.707106781186548,
1.),(1.,0.707106781186547,1.,0.707106781186547,1.,0.707106781186547,1.,
0.707106781186547,1.),(1.,0.707106781186547,1.,0.707106781186547,1.,0.707106781186547,
1.,0.707106781186547,1.),(1.,0.707106781186548,1.,0.707106781186548,1.,
0.707106781186548,1.,0.707106781186548,1.),(1.,0.707106781186547,1.,0.707106781186547,
1.,0.707106781186547,1.,0.707106781186547,1.),(1.,0.707106781186547,1.,
0.707106781186547,1.,0.707106781186547,1.,0.707106781186547,1.),(1.,0.707106781186547,
1.,0.707106781186547,1.,0.707106781186547,1.,0.707106781186547,1.),(1.,
0.707106781186547,1.,0.707106781186547,1.,0.707106781186547,1.,0.707106781186547,
1.),(1.,0.707106781186548,1.,0.707106781186548,1.,0.707106781186548,1.,
0.707106781186548,1.),(1.,0.707106781186547,1.,0.707106781186547,1.,0.707106781186547,
1.,0.707106781186547,1.),(1.,0.707106781186547,1.,0.707106781186547,1.,
0.707106781186547,1.,0.707106781186547,1.),(1.,0.707106781186547,1.,0.707106781186547,
1.,0.707106781186547,1.,0.707106781186547,1.),(1.,0.707106781186548,1.,
0.707106781186548,1.,0.707106781186548,1.,0.707106781186548,1.),(1.,0.707106781186547,
1.,0.707106781186547,1.,0.707106781186547,1.,0.707106781186547,1.),(1.,
0.707106781186547,1.,0.707106781186547,1.,0.707106781186547,1.,0.707106781186547,
1.),(1.,0.707106781186548,1.,0.707106781186548,1.,0.707106781186548,1.,
0.707106781186548,1.),(1.,0.707106781186548,1.,0.707106781186548,1.,0.707106781186548,
1.,0.707106781186548,1.),(1.,0.707106781186547,1.,0.707106781186547,1.,
0.707106781186547,1.,0.707106781186547,1.),(1.,0.707106781186548,1.,0.707106781186548,
1.,0.707106781186548,1.,0.707106781186548,1.),(1.,0.707106781186548,1.,
0.707106781186548,1.,0.707106781186548,1.,0.707106781186548,1.),(1.,0.707106781186547,
1.,0.707106781186547,1.,0.707106781186547,1.,0.707106781186547,1.),(1.,
0.707106781186547,1.,0.707106781186547,1.,0.707106781186547,1.,0.707106781186547,
1.),(1.,0.707106781186548,1.,0.707106781186548,1.,0.707106781186548,1.,
0.707106781186548,1.),(1.,0.707106781186547,1.,0.707106781186547,1.,0.707106781186547,
1.,0.707106781186547,1.),(1.,0.707106781186547,1.,0.707106781186547,1.,
0.707106781186547,1.,0.707106781186547,1.),(1.,0.707106781186548,1.,0.707106781186548,
1.,0.707106781186548,1.,0.707106781186548,1.),(1.,0.707106781186547,1.,
0.707106781186547,1.,0.707106781186547,1.,0.707106781186547,1.),(1.,0.707106781186547,
1.,0.707106781186547,1.,0.707106781186547,1.,0.707106781186547,1.),(1.,
0.707106781186547,1.,0.707106781186547,1.,0.707106781186547,1.,0.707106781186547,
1.),(1.,0.707106781186548,1.,0.707106781186548,1.,0.707106781186548,1.,
0.707106781186548,1.),(1.,0.707106781186547,1.,0.707106781186547,1.,0.707106781186547,
1.,0.707106781186547,1.),(1.,0.707106781186548,1.,0.707106781186548,1.,
0.707106781186548,1.,0.707106781186548,1.),(1.,0.707106781186547,1.,0.707106781186547,
1.,0.707106781186547,1.,0.707106781186547,1.),(1.,0.707106781186548,1.,
0.707106781186548,1.,0.707106781186548,1.,0.707106781186548,1.),(1.,0.707106781186547,
1.,0.707106781186547,1.,0.707106781186547,1.,0.707106781186547,1.),(1.,
0.707106781186548,1.,0.707106781186548,1.,0.707106781186548,1.,0.707106781186548,
1.),(1.,0.707106781186547,1.,0.707106781186547,1.,0.707106781186547,1.,
0.707106781186547,1.),(1.,0.707106781186548,1.,0.707106781186548,1.,0.707106781186548,
1.,0.707106781186548,1.),(1.,0.707106781186547,1.,0.707106781186547,1.,
0.707106781186547,1.,0.707106781186547,1.),(1.,0.707106781186548,1.,0.707106781186548,
1.,0.707106781186548,1.,0.707106781186548,1.),(1.,0.707106781186548,1.,
0.707106781186548,1.,0.707106781186548,1.,0.707106781186548,1.),(1.,0.707106781186547,
1.,0.707106781186547,1.,0.707106781186547,1.,0.707106781186547,1.),(1.,
0.707106781186547,1.,0.707106781186547,1.,0.707106781186547,1.,0.707106781186547,
1.),(1.,0.707106781186548,1.,0.707106781186548,1.,0.707106781186548,1.,
0.707106781186548,1.),(1.,0.707106781186547,1.,0.707106781186547,1.,0.707106781186547,
1.,0.707106781186547,1.),(1.,0.707106781186548,1.,0.707106781186548,1.,
0.707106781186548,1.,0.707106781186548,1.),(1.,0.707106781186547,1.,0.707106781186547,
1.,0.707106781186547,1.,0.707106781186547,1.),(1.,0.707106781186548,1.,
0.707106781186548,1.,0.707106781186548,1.,0.707106781186548,1.),(1.,0.707106781186548,
1.,0.707106781186548,1.,0.707106781186548,1.,0.707106781186548,1.),(1.,
0.707106781186547,1.,0.707106781186547,1.,0.707106781186547,1.,0.707106781186547,
1.),(1.,0.707106781186548,1.,0.707106781186548,1.,0.707106781186548,1.,
0.707106781186548,1.),(1.,0.707106781186547,1.,0.707106781186547,1.,0.707106781186547,
1.,0.707106781186547,1.),(1.,0.707106781186548,1.,0.707106781186548,1.,
0.707106781186548,1.,0.707106781186548,1.),(1.,0.707106781186548,1.,0.707106781186548,
1.,0.707106781186548,1.,0.707106781186548,1.),(1.,0.707106781186547,1.,
0.707106781186547,1.,0.707106781186547,1.,0.707106781186547,1.),(1.,0.707106781186547,
1.,0.707106781186547,1.,0.707106781186547,1.,0.707106781186547,1.),(1.,
0.707106781186548,1.,0.707106781186548,1.,0.707106781186548,1.,0.707106781186548,
1.),(1.,0.707106781186547,1.,0.707106781186547,1.,0.707106781186547,1.,
0.707106781186547,1.),(1.,0.707106781186548,1.,0.707106781186548,1.,0.707106781186548,
1.,0.707106781186548,1.),(1.,0.707106781186547,1.,0.707106781186547,1.,
0.707106781186547,1.,0.707106781186547,1.),(1.,0.707106781186548,1.,0.707106781186548,
1.,0.707106781186548,1.,0.707106781186548,1.),(1.,0.707106781186547,1.,
0.707106781186547,1.,0.707106781186547,1.,0.707106781186547,1.),(1.,0.707106781186548,
1.,0.707106781186548,1.,0.707106781186548,1.,0.707106781186548,1.),(1.,
0.707106781186547,1.,0.707106781186547,1.,0.707106781186547,1.,0.707106781186547,
1.),(1.,0.707106781186547,1.,0.707106781186547,1.,0.707106781186547,1.,
0.707106781186547,1.),(1.,0.707106781186547,1.,0.707106781186547,1.,0.707106781186547,
1.,0.707106781186547,1.),(1.,0.707106781186547,1.,0.707106781186547,1.,
0.707106781186547,1.,0.707106781186547,1.),(1.,0.707106781186547,1.,0.707106781186547,
1.,0.707106781186547,1.,0.707106781186547,1.),(1.,0.707106781186547,1.,
0.707106781186547,1.,0.707106781186547,1.,0.707106781186547,1.),(1.,0.707106781186547,
1.,0.707106781186547,1.,0.707106781186547,1.,0.707106781186547,1.),(1.,
0.707106781186547,1.,0.707106781186547,1.,0.707106781186547,1.,0.707106781186547,
1.),(1.,0.707106781186548,1.,0.707106781186548,1.,0.707106781186548,1.,
0.707106781186548,1.),(1.,0.707106781186547,1.,0.707106781186547,1.,0.707106781186547,
1.,0.707106781186547,1.),(1.,0.707106781186548,1.,0.707106781186548,1.,
0.707106781186548,1.,0.707106781186548,1.),(1.,0.707106781186547,1.,0.707106781186547,
1.,0.707106781186547,1.,0.707106781186547,1.),(1.,0.707106781186547,1.,
0.707106781186547,1.,0.707106781186547,1.,0.707106781186547,1.),(1.,0.707106781186548,
1.,0.707106781186548,1.,0.707106781186548,1.,0.707106781186548,1.),(1.,
0.707106781186547,1.,0.707106781186547,1.,0.707106781186547,1.,0.707106781186547,
1.),(1.,0.707106781186548,1.,0.707106781186548,1.,0.707106781186548,1.,
0.707106781186548,1.),(1.,0.707106781186547,1.,0.707106781186547,1.,0.707106781186547,
1.,0.707106781186547,1.),(1.,0.707106781186547,1.,0.707106781186547,1.,
0.707106781186547,1.,0.707106781186547,1.),(1.,0.707106781186548,1.,0.707106781186548,
1.,0.707106781186548,1.,0.707106781186548,1.),(1.,0.707106781186547,1.,
0.707106781186547,1.,0.707106781186547,1.,0.707106781186547,1.),(1.,0.707106781186548,
1.,0.707106781186548,1.,0.707106781186548,1.,0.707106781186548,1.),(1.,
0.707106781186547,1.,0.707106781186547,1.,0.707106781186547,1.,0.707106781186547,
1.),(1.,0.707106781186548,1.,0.707106781186548,1.,0.707106781186548,1.,
0.707106781186548,1.),(1.,0.707106781186547,1.,0.707106781186547,1.,0.707106781186547,
1.,0.707106781186547,1.),(1.,0.707106781186548,1.,0.707106781186548,1.,
0.707106781186548,1.,0.707106781186548,1.),(1.,0.707106781186547,1.,0.707106781186547,
1.,0.707106781186547,1.,0.707106781186547,1.),(1.,0.707106781186548,1.,
0.707106781186548,1.,0.707106781186548,1.,0.707106781186548,1.),(1.,0.707106781186547,
1.,0.707106781186547,1.,0.707106781186547,1.,0.707106781186547,1.),(1.,
0.707106781186548,1.,0.707106781186548,1.,0.707106781186548,1.,0.707106781186548,
1.),(1.,0.707106781186547,1.,0.707106781186547,1.,0.707106781186547,1.,
0.707106781186547,1.),(1.,0.707106781186548,1.,0.707106781186548,1.,0.707106781186548,
1.,0.707106781186548,1.),(1.,0.707106781186548,1.,0.707106781186548,1.,
0.707106781186548,1.,0.707106781186548,1.),(1.,0.707106781186547,1.,0.707106781186547,
1.,0.707106781186547,1.,0.707106781186547,1.),(1.,0.707106781186548,1.,
0.707106781186548,1.,0.707106781186548,1.,0.707106781186548,1.),(1.,0.707106781186547,
1.,0.707106781186547,1.,0.707106781186547,1.,0.707106781186547,1.),(1.,
0.707106781186547,1.,0.707106781186547,1.,0.707106781186547,1.,0.707106781186547,
1.),(1.,0.707106781186547,1.,0.707106781186547,1.,0.707106781186547,1.,
0.707106781186547,1.),(1.,0.707106781186548,1.,0.707106781186548,1.,0.707106781186548,
1.,0.707106781186548,1.),(1.,0.707106781186547,1.,0.707106781186547,1.,
0.707106781186547,1.,0.707106781186547,1.),(1.,0.707106781186547,1.,0.707106781186547,
1.,0.707106781186547,1.,0.707106781186547,1.),(1.,0.707106781186547,1.,
0.707106781186547,1.,0.707106781186547,1.,0.707106781186547,1.),(1.,0.707106781186548,
1.,0.707106781186548,1.,0.707106781186548,1.,0.707106781186548,1.),(1.,
0.707106781186547,1.,0.707106781186547,1.,0.707106781186547,1.,0.707106781186547,
1.),(1.,0.707106781186547,1.,0.707106781186547,1.,0.707106781186547,1.,
0.707106781186547,1.),(1.,0.707106781186548,1.,0.707106781186548,1.,0.707106781186548,
1.,0.707106781186548,1.),(1.,0.707106781186547,1.,0.707106781186547,1.,
0.707106781186547,1.,0.707106781186547,1.),(1.,0.707106781186547,1.,0.707106781186547,
1.,0.707106781186547,1.,0.707106781186547,1.),(1.,0.707106781186547,1.,
0.707106781186547,1.,0.707106781186547,1.,0.707106781186547,1.),(1.,0.707106781186547,
1.,0.707106781186547,1.,0.707106781186547,1.,0.707106781186547,1.),(1.,
0.707106781186548,1.,0.707106781186548,1.,0.707106781186548,1.,0.707106781186548,
1.),(1.,0.707106781186547,1.,0.707106781186547,1.,0.707106781186547,1.,
0.707106781186547,1.),(1.,0.707106781186547,1.,0.707106781186547,1.,0.707106781186547,
1.,0.707106781186547,1.),(1.,0.707106781186547,1.,0.707106781186547,1.,
0.707106781186547,1.,0.707106781186547,1.),(1.,0.707106781186548,1.,0.707106781186548,
1.,0.707106781186548,1.,0.707106781186548,1.),(1.,0.707106781186548,1.,
0.707106781186548,1.,0.707106781186548,1.,0.707106781186548,1.),(1.,0.707106781186548,
1.,0.707106781186548,1.,0.707106781186548,1.,0.707106781186548,1.),(1.,
0.707106781186548,1.,0.707106781186548,1.,0.707106781186548,1.,0.707106781186548,
1.),(1.,0.707106781186547,1.,0.707106781186547,1.,0.707106781186547,1.,
0.707106781186547,1.),(1.,0.707106781186548,1.,0.707106781186548,1.,0.707106781186548,
1.,0.707106781186548,1.),(1.,0.707106781186547,1.,0.707106781186547,1.,
0.707106781186547,1.,0.707106781186547,1.),(1.,0.707106781186547,1.,0.707106781186547,
1.,0.707106781186547,1.,0.707106781186547,1.),(1.,0.707106781186548,1.,
0.707106781186548,1.,0.707106781186548,1.,0.707106781186548,1.),(1.,0.707106781186547,
1.,0.707106781186547,1.,0.707106781186547,1.,0.707106781186547,1.),(1.,
0.707106781186548,1.,0.707106781186548,1.,0.707106781186548,1.,0.707106781186548,
1.),(1.,0.707106781186547,1.,0.707106781186547,1.,0.707106781186547,1.,
0.707106781186547,1.),(1.,0.707106781186547,1.,0.707106781186547,1.,0.707106781186547,
1.,0.707106781186547,1.),(1.,0.707106781186548,1.,0.707106781186548,1.,
0.707106781186548,1.,0.707106781186548,1.),(1.,0.707106781186547,1.,0.707106781186547,
1.,0.707106781186547,1.,0.707106781186547,1.),(1.,0.707106781186547,1.,
0.707106781186547,1.,0.707106781186547,1.,0.707106781186547,1.),(1.,0.707106781186547,
1.,0.707106781186547,1.,0.707106781186547,1.,0.707106781186547,1.),(1.,
0.707106781186547,1.,0.707106781186547,1.,0.707106781186547,1.,0.707106781186547,
1.),(1.,0.707106781186548,1.,0.707106781186548,1.,0.707106781186548,1.,
0.707106781186548,1.),(1.,0.707106781186548,1.,0.707106781186548,1.,0.707106781186548,
1.,0.707106781186548,1.),(1.,0.707106781186547,1.,0.707106781186547,1.,
0.707106781186547,1.,0.707106781186547,1.),(1.,0.707106781186547,1.,0.707106781186547,
1.,0.707106781186547,1.,0.707106781186547,1.),(1.,0.707106781186548,1.,
0.707106781186548,1.,0.707106781186548,1.,0.707106781186548,1.),(1.,0.707106781186547,
1.,0.707106781186547,1.,0.707106781186547,1.,0.707106781186547,1.),(1.,
0.707106781186548,1.,0.707106781186548,1.,0.707106781186548,1.,0.707106781186548,
1.),(1.,0.707106781186547,1.,0.707106781186547,1.,0.707106781186547,1.,
0.707106781186547,1.),(1.,0.707106781186548,1.,0.707106781186548,1.,0.707106781186548,
1.,0.707106781186548,1.),(1.,0.707106781186548,1.,0.707106781186548,1.,
0.707106781186548,1.,0.707106781186548,1.),(1.,0.707106781186547,1.,0.707106781186547,
1.,0.707106781186547,1.,0.707106781186547,1.),(1.,0.707106781186547,1.,
0.707106781186547,1.,0.707106781186547,1.,0.707106781186547,1.),(1.,0.707106781186548,
1.,0.707106781186548,1.,0.707106781186548,1.,0.707106781186548,1.),(1.,
0.707106781186548,1.,0.707106781186548,1.,0.707106781186548,1.,0.707106781186548,
1.),(1.,0.707106781186547,1.,0.707106781186547,1.,0.707106781186547,1.,
0.707106781186547,1.),(1.,0.707106781186548,1.,0.707106781186548,1.,0.707106781186548,
1.,0.707106781186548,1.),(1.,0.707106781186548,1.,0.707106781186548,1.,
0.707106781186548,1.,0.707106781186548,1.),(1.,0.707106781186547,1.,0.707106781186547,
1.,0.707106781186547,1.,0.707106781186547,1.),(1.,0.707106781186548,1.,
0.707106781186548,1.,0.707106781186548,1.,0.707106781186548,1.),(1.,0.707106781186548,
1.,0.707106781186548,1.,0.707106781186548,1.,0.707106781186548,1.),(1.,
0.707106781186548,1.,0.707106781186548,1.,0.707106781186548,1.,0.707106781186548,
1.),(1.,0.707106781186547,1.,0.707106781186547,1.,0.707106781186547,1.,
0.707106781186547,1.),(1.,0.707106781186548,1.,0.707106781186548,1.,0.707106781186548,
1.,0.707106781186548,1.),(1.,0.707106781186547,1.,0.707106781186547,1.,
0.707106781186547,1.,0.707106781186547,1.),(1.,0.707106781186548,1.,0.707106781186548,
1.,0.707106781186548,1.,0.707106781186548,1.),(1.,0.707106781186547,1.,
0.707106781186547,1.,0.707106781186547,1.,0.707106781186547,1.),(1.,0.707106781186548,
1.,0.707106781186548,1.,0.707106781186548,1.,0.707106781186548,1.),(1.,
0.707106781186547,1.,0.707106781186547,1.,0.707106781186547,1.,0.707106781186547,
1.),(1.,0.707106781186548,1.,0.707106781186548,1.,0.707106781186548,1.,
0.707106781186548,1.),(1.,0.707106781186547,1.,0.707106781186547,1.,0.707106781186547,
1.,0.707106781186547,1.),(1.,0.707106781186548,1.,0.707106781186548,1.,
0.707106781186548,1.,0.707106781186548,1.),(1.,0.707106781186548,1.,0.707106781186548,
1.,0.707106781186548,1.,0.707106781186548,1.),(1.,0.707106781186547,1.,
0.707106781186547,1.,0.707106781186547,1.,0.707106781186547,1.),(1.,0.707106781186547,
1.,0.707106781186547,1.,0.707106781186547,1.,0.707106781186547,1.),(1.,
0.707106781186548,1.,0.707106781186548,1.,0.707106781186548,1.,0.707106781186548,
1.),(1.,0.707106781186547,1.,0.707106781186547,1.,0.707106781186547,1.,
0.707106781186547,1.),(1.,0.707106781186548,1.,0.707106781186548,1.,0.707106781186548,
1.,0.707106781186548,1.),(1.,0.707106781186547,1.,0.707106781186547,1.,
0.707106781186547,1.,0.707106781186547,1.),(1.,0.707106781186548,1.,0.707106781186548,
1.,0.707106781186548,1.,0.707106781186548,1.),(1.,0.707106781186548,1.,
0.707106781186548,1.,0.707106781186548,1.,0.707106781186548,1.),(1.,0.707106781186548,
1.,0.707106781186548,1.,0.707106781186548,1.,0.707106781186548,1.),(1.,
0.707106781186548,1.,0.707106781186548,1.,0.707106781186548,1.,0.707106781186548,
1.),(1.,0.707106781186548,1.,0.707106781186548,1.,0.707106781186548,1.,
0.707106781186548,1.),(1.,0.707106781186547,1.,0.707106781186547,1.,0.707106781186547,
1.,0.707106781186547,1.),(1.,0.707106781186547,1.,0.707106781186547,1.,
0.707106781186547,1.,0.707106781186547,1.),(1.,0.707106781186547,1.,0.707106781186547,
1.,0.707106781186547,1.,0.707106781186547,1.),(1.,0.707106781186547,1.,
0.707106781186547,1.,0.707106781186547,1.,0.707106781186547,1.),(1.,0.707106781186548,
1.,0.707106781186548,1.,0.707106781186548,1.,0.707106781186548,1.),(1.,
0.707106781186547,1.,0.707106781186547,1.,0.707106781186547,1.,0.707106781186547,
1.),(1.,0.707106781186548,1.,0.707106781186548,1.,0.707106781186548,1.,
0.707106781186548,1.),(1.,0.707106781186547,1.,0.707106781186547,1.,0.707106781186547,
1.,0.707106781186547,1.),(1.,0.707106781186547,1.,0.707106781186547,1.,
0.707106781186547,1.,0.707106781186547,1.),(1.,0.707106781186548,1.,0.707106781186548,
1.,0.707106781186548,1.,0.707106781186548,1.),(1.,0.707106781186548,1.,
0.707106781186548,1.,0.707106781186548,1.,0.707106781186548,1.),(1.,0.707106781186547,
1.,0.707106781186547,1.,0.707106781186547,1.,0.707106781186547,1.),(1.,
0.707106781186548,1.,0.707106781186548,1.,0.707106781186548,1.,0.707106781186548,
1.),(1.,0.707106781186547,1.,0.707106781186547,1.,0.707106781186547,1.,
0.707106781186547,1.),(1.,0.707106781186548,1.,0.707106781186548,1.,0.707106781186548,
1.,0.707106781186548,1.),(1.,0.707106781186548,1.,0.707106781186548,1.,
0.707106781186548,1.,0.707106781186548,1.),(1.,0.707106781186547,1.,0.707106781186547,
1.,0.707106781186547,1.,0.707106781186547,1.),(1.,0.707106781186547,1.,
0.707106781186547,1.,0.707106781186547,1.,0.707106781186547,1.),(1.,0.707106781186548,
1.,0.707106781186548,1.,0.707106781186548,1.,0.707106781186548,1.),(1.,
0.707106781186547,1.,0.707106781186547,1.,0.707106781186547,1.,0.707106781186547,
1.),(1.,0.707106781186548,1.,0.707106781186548,1.,0.707106781186548,1.,
0.707106781186548,1.),(1.,0.707106781186547,1.,0.707106781186547,1.,0.707106781186547,
1.,0.707106781186547,1.),(1.,0.707106781186548,1.,0.707106781186548,1.,
0.707106781186548,1.,0.707106781186548,1.),(1.,0.707106781186547,1.,0.707106781186547,
1.,0.707106781186547,1.,0.707106781186547,1.),(1.,0.707106781186548,1.,
0.707106781186548,1.,0.707106781186548,1.,0.707106781186548,1.),(1.,0.707106781186547,
1.,0.707106781186547,1.,0.707106781186547,1.,0.707106781186547,1.),(1.,
0.707106781186548,1.,0.707106781186548,1.,0.707106781186548,1.,0.707106781186548,
1.),(1.,0.707106781186547,1.,0.707106781186547,1.,0.707106781186547,1.,
0.707106781186547,1.),(1.,0.707106781186548,1.,0.707106781186548,1.,0.707106781186548,
1.,0.707106781186548,1.),(1.,0.707106781186547,1.,0.707106781186547,1.,
0.707106781186547,1.,0.707106781186547,1.),(1.,0.707106781186548,1.,0.707106781186548,
1.,0.707106781186548,1.,0.707106781186548,1.),(1.,0.707106781186548,1.,
0.707106781186548,1.,0.707106781186548,1.,0.707106781186548,1.),(1.,0.707106781186547,
1.,0.707106781186547,1.,0.707106781186547,1.,0.707106781186547,1.),(1.,
0.707106781186548,1.,0.707106781186548,1.,0.707106781186548,1.,0.707106781186548,
1.),(1.,0.707106781186547,1.,0.707106781186547,1.,0.707106781186547,1.,
0.707106781186547,1.),(1.,0.707106781186548,1.,0.707106781186548,1.,0.707106781186548,
1.,0.707106781186548,1.),(1.,0.707106781186547,1.,0.707106781186547,1.,
0.707106781186547,1.,0.707106781186547,1.),(1.,0.707106781186548,1.,0.707106781186548,
1.,0.707106781186548,1.,0.707106781186548,1.),(1.,0.707106781186548,1.,
0.707106781186548,1.,0.707106781186548,1.,0.707106781186548,1.),(1.,0.707106781186548,
1.,0.707106781186548,1.,0.707106781186548,1.,0.707106781186548,1.),(1.,
0.707106781186547,1.,0.707106781186547,1.,0.707106781186547,1.,0.707106781186547,
1.),(1.,0.707106781186547,1.,0.707106781186547,1.,0.707106781186547,1.,
0.707106781186547,1.),(1.,0.707106781186548,1.,0.707106781186548,1.,0.707106781186548,
1.,0.707106781186548,1.),(1.,0.707106781186548,1.,0.707106781186548,1.,
0.707106781186548,1.,0.707106781186548,1.),(1.,0.707106781186547,1.,0.707106781186547,
1.,0.707106781186547,1.,0.707106781186547,1.),(1.,0.707106781186547,1.,
0.707106781186547,1.,0.707106781186547,1.,0.707106781186547,1.),(1.,0.707106781186547,
1.,0.707106781186547,1.,0.707106781186547,1.,0.707106781186547,1.),(1.,
0.707106781186548,1.,0.707106781186548,1.,0.707106781186548,1.,0.707106781186548,
1.),(1.,0.707106781186547,1.,0.707106781186547,1.,0.707106781186547,1.,
0.707106781186547,1.),(1.,0.707106781186548,1.,0.707106781186548,1.,0.707106781186548,
1.,0.707106781186548,1.),(1.,0.707106781186547,1.,0.707106781186547,1.,
0.707106781186547,1.,0.707106781186547,1.),(1.,0.707106781186548,1.,0.707106781186548,
1.,0.707106781186548,1.,0.707106781186548,1.),(1.,0.707106781186547,1.,
0.707106781186547,1.,0.707106781186547,1.,0.707106781186547,1.),(1.,0.707106781186547,
1.,0.707106781186547,1.,0.707106781186547,1.,0.707106781186547,1.),(1.,
0.707106781186547,1.,0.707106781186547,1.,0.707106781186547,1.,0.707106781186547,
1.),(1.,0.707106781186548,1.,0.707106781186548,1.,0.707106781186548,1.,
0.707106781186548,1.),(1.,0.707106781186547,1.,0.707106781186547,1.,0.707106781186547,
1.,0.707106781186547,1.),(1.,0.707106781186548,1.,0.707106781186548,1.,
0.707106781186548,1.,0.707106781186548,1.),(1.,0.707106781186547,1.,0.707106781186547,
1.,0.707106781186547,1.,0.707106781186547,1.),(1.,0.707106781186548,1.,
0.707106781186548,1.,0.707106781186548,1.,0.707106781186548,1.),(1.,0.707106781186547,
1.,0.707106781186547,1.,0.707106781186547,1.,0.707106781186547,1.),(1.,
0.707106781186548,1.,0.707106781186548,1.,0.707106781186548,1.,0.707106781186548,
1.),(1.,0.707106781186547,1.,0.707106781186547,1.,0.707106781186547,1.,
0.707106781186547,1.),(1.,0.707106781186547,1.,0.707106781186547,1.,0.707106781186547,
1.,0.707106781186547,1.),(1.,0.707106781186548,1.,0.707106781186548,1.,
0.707106781186548,1.,0.707106781186548,1.),(1.,0.707106781186547,1.,0.707106781186547,
1.,0.707106781186547,1.,0.707106781186547,1.),(1.,0.707106781186547,1.,
0.707106781186547,1.,0.707106781186547,1.,0.707106781186547,1.),(1.,0.707106781186548,
1.,0.707106781186548,1.,0.707106781186548,1.,0.707106781186548,1.),(1.,
0.707106781186547,1.,0.707106781186547,1.,0.707106781186547,1.,0.707106781186547,
1.),(1.,0.707106781186547,1.,0.707106781186547,1.,0.707106781186547,1.,
0.707106781186547,1.),(1.,0.707106781186548,1.,0.707106781186548,1.,0.707106781186548,
1.,0.707106781186548,1.),(1.,0.707106781186547,1.,0.707106781186547,1.,
0.707106781186547,1.,0.707106781186547,1.),(1.,0.707106781186547,1.,0.707106781186547,
1.,0.707106781186547,1.,0.707106781186547,1.),(1.,0.707106781186547,1.,
0.707106781186547,1.,0.707106781186547,1.,0.707106781186547,1.),(1.,0.707106781186548,
1.,0.707106781186548,1.,0.707106781186548,1.,0.707106781186548,1.),(1.,
0.707106781186547,1.,0.707106781186547,1.,0.707106781186547,1.,0.707106781186547,
1.),(1.,0.707106781186548,1.,0.707106781186548,1.,0.707106781186548,1.,
0.707106781186548,1.),(1.,0.707106781186547,1.,0.707106781186547,1.,0.707106781186547,
1.,0.707106781186547,1.),(1.,0.707106781186547,1.,0.707106781186547,1.,
0.707106781186547,1.,0.707106781186547,1.),(1.,0.707106781186547,1.,0.707106781186547,
1.,0.707106781186547,1.,0.707106781186547,1.),(1.,0.707106781186548,1.,
0.707106781186548,1.,0.707106781186548,1.,0.707106781186548,1.),(1.,0.707106781186548,
1.,0.707106781186548,1.,0.707106781186548,1.,0.707106781186548,1.),(1.,
0.707106781186547,1.,0.707106781186547,1.,0.707106781186547,1.,0.707106781186547,
1.),(1.,0.707106781186547,1.,0.707106781186547,1.,0.707106781186547,1.,
0.707106781186547,1.),(1.,0.707106781186548,1.,0.707106781186548,1.,0.707106781186548,
1.,0.707106781186548,1.),(1.,0.707106781186548,1.,0.707106781186548,1.,
0.707106781186548,1.,0.707106781186548,1.),(1.,0.707106781186548,1.,0.707106781186548,
1.,0.707106781186548,1.,0.707106781186548,1.),(1.,0.707106781186547,1.,
0.707106781186547,1.,0.707106781186547,1.,0.707106781186547,1.),(1.,0.707106781186548,
1.,0.707106781186548,1.,0.707106781186548,1.,0.707106781186548,1.),(1.,
0.707106781186547,1.,0.707106781186547,1.,0.707106781186547,1.,0.707106781186547,
1.),(1.,0.707106781186548,1.,0.707106781186548,1.,0.707106781186548,1.,
0.707106781186548,1.),(1.,0.707106781186547,1.,0.707106781186547,1.,0.707106781186547,
1.,0.707106781186547,1.),(1.,0.707106781186548,1.,0.707106781186548,1.,
0.707106781186548,1.,0.707106781186548,1.),(1.,0.707106781186547,1.,0.707106781186547,
1.,0.707106781186547,1.,0.707106781186547,1.),(1.,0.707106781186547,1.,
0.707106781186547,1.,0.707106781186547,1.,0.707106781186547,1.),(1.,0.707106781186547,
1.,0.707106781186547,1.,0.707106781186547,1.,0.707106781186547,1.),(1.,
0.707106781186547,1.,0.707106781186547,1.,0.707106781186547,1.,0.707106781186547,
1.),(1.,0.707106781186548,1.,0.707106781186548,1.,0.707106781186548,1.,
0.707106781186548,1.),(1.,0.707106781186547,1.,0.707106781186547,1.,0.707106781186547,
1.,0.707106781186547,1.),(1.,0.707106781186548,1.,0.707106781186548,1.,
0.707106781186548,1.,0.707106781186548,1.),(1.,0.707106781186548,1.,0.707106781186548,
1.,0.707106781186548,1.,0.707106781186548,1.),(1.,0.707106781186547,1.,
0.707106781186547,1.,0.707106781186547,1.,0.707106781186547,1.),(1.,0.707106781186548,
1.,0.707106781186548,1.,0.707106781186548,1.,0.707106781186548,1.),(1.,
0.707106781186547,1.,0.707106781186547,1.,0.707106781186547,1.,0.707106781186547,
1.),(1.,0.707106781186547,1.,0.707106781186547,1.,0.707106781186547,1.,
0.707106781186547,1.),(1.,0.707106781186547,1.,0.707106781186547,1.,0.707106781186547,
1.,0.707106781186547,1.),(1.,0.707106781186547,1.,0.707106781186547,1.,
0.707106781186547,1.,0.707106781186547,1.),(1.,0.707106781186548,1.,0.707106781186548,
1.,0.707106781186548,1.,0.707106781186548,1.),(1.,0.707106781186547,1.,
0.707106781186547,1.,0.707106781186547,1.,0.707106781186547,1.),(1.,0.707106781186548,
1.,0.707106781186548,1.,0.707106781186548,1.,0.707106781186548,1.),(1.,
0.707106781186547,1.,0.707106781186547,1.,0.707106781186547,1.,0.707106781186547,
1.),(1.,0.707106781186548,1.,0.707106781186548,1.,0.707106781186548,1.,
0.707106781186548,1.),(1.,0.707106781186548,1.,0.707106781186548,1.,0.707106781186548,
1.,0.707106781186548,1.),(1.,0.707106781186547,1.,0.707106781186547,1.,
0.707106781186547,1.,0.707106781186547,1.),(1.,0.707106781186548,1.,0.707106781186548,
1.,0.707106781186548,1.,0.707106781186548,1.),(1.,0.707106781186547,1.,
0.707106781186547,1.,0.707106781186547,1.,0.707106781186547,1.),(1.,0.707106781186547,
1.,0.707106781186547,1.,0.707106781186547,1.,0.707106781186547,1.),(1.,
0.707106781186547,1.,0.707106781186547,1.,0.707106781186547,1.,0.707106781186547,
1.),(1.,0.707106781186547,1.,0.707106781186547,1.,0.707106781186547,1.,
0.707106781186547,1.),(1.,0.707106781186548,1.,0.707106781186548,1.,0.707106781186548,
1.,0.707106781186548,1.),(1.,0.707106781186547,1.,0.707106781186547,1.,
0.707106781186547,1.,0.707106781186547,1.),(1.,0.707106781186548,1.,0.707106781186548,
1.,0.707106781186548,1.,0.707106781186548,1.),(1.,0.707106781186548,1.,
0.707106781186548,1.,0.707106781186548,1.,0.707106781186548,1.),(1.,0.707106781186547,
1.,0.707106781186547,1.,0.707106781186547,1.,0.707106781186547,1.),(1.,
0.707106781186548,1.,0.707106781186548,1.,0.707106781186548,1.,0.707106781186548,
1.),(1.,0.707106781186547,1.,0.707106781186547,1.,0.707106781186547,1.,
0.707106781186547,1.),(1.,0.707106781186548,1.,0.707106781186548,1.,0.707106781186548,
1.,0.707106781186548,1.),(1.,0.707106781186547,1.,0.707106781186547,1.,
0.707106781186547,1.,0.707106781186547,1.),(1.,0.707106781186547,1.,0.707106781186547,
1.,0.707106781186547,1.,0.707106781186547,1.),(1.,0.707106781186548,1.,
0.707106781186548,1.,0.707106781186548,1.,0.707106781186548,1.),(1.,0.707106781186547,
1.,0.707106781186547,1.,0.707106781186547,1.,0.707106781186547,1.),(1.,
0.707106781186548,1.,0.707106781186548,1.,0.707106781186548,1.,0.707106781186548,
1.),(1.,0.707106781186548,1.,0.707106781186548,1.,0.707106781186548,1.,
0.707106781186548,1.),(1.,0.707106781186547,1.,0.707106781186547,1.,0.707106781186547,
1.,0.707106781186547,1.),(1.,0.707106781186547,1.,0.707106781186547,1.,
0.707106781186547,1.,0.707106781186547,1.),(1.,0.707106781186548,1.,0.707106781186548,
1.,0.707106781186548,1.,0.707106781186548,1.),(1.,0.707106781186548,1.,
0.707106781186548,1.,0.707106781186548,1.,0.707106781186548,1.),(1.,0.707106781186547,
1.,0.707106781186547,1.,0.707106781186547,1.,0.707106781186547,1.),(1.,
0.707106781186547,1.,0.707106781186547,1.,0.707106781186547,1.,0.707106781186547,
1.),(1.,0.707106781186548,1.,0.707106781186548,1.,0.707106781186548,1.,
0.707106781186548,1.),(1.,0.707106781186547,1.,0.707106781186547,1.,0.707106781186547,
1.,0.707106781186547,1.),(1.,0.707106781186547,1.,0.707106781186547,1.,
0.707106781186547,1.,0.707106781186547,1.),(1.,0.707106781186548,1.,0.707106781186548,
1.,0.707106781186548,1.,0.707106781186548,1.),(1.,0.707106781186547,1.,
0.707106781186547,1.,0.707106781186547,1.,0.707106781186547,1.),(1.,0.707106781186547,
1.,0.707106781186547,1.,0.707106781186547,1.,0.707106781186547,1.),(1.,
0.707106781186548,1.,0.707106781186548,1.,0.707106781186548,1.,0.707106781186548,
1.),(1.,0.707106781186547,1.,0.707106781186547,1.,0.707106781186547,1.,
0.707106781186547,1.),(1.,0.707106781186548,1.,0.707106781186548,1.,0.707106781186548,
1.,0.707106781186548,1.),(1.,0.707106781186547,1.,0.707106781186547,1.,
0.707106781186547,1.,0.707106781186547,1.),(1.,0.707106781186547,1.,0.707106781186547,
1.,0.707106781186547,1.,0.707106781186547,1.),(1.,0.707106781186548,1.,
0.707106781186548,1.,0.707106781186548,1.,0.707106781186548,1.),(1.,0.707106781186547,
1.,0.707106781186547,1.,0.707106781186547,1.,0.707106781186547,1.),(1.,
0.707106781186548,1.,0.707106781186548,1.,0.707106781186548,1.,0.707106781186548,
1.),(1.,0.707106781186547,1.,0.707106781186547,1.,0.707106781186547,1.,
0.707106781186547,1.),(1.,0.707106781186548,1.,0.707106781186548,1.,0.707106781186548,
1.,0.707106781186548,1.),(1.,0.707106781186547,1.,0.707106781186547,1.,
0.707106781186547,1.,0.707106781186547,1.),(1.,0.707106781186547,1.,0.707106781186547,
1.,0.707106781186547,1.,0.707106781186547,1.),(1.,0.707106781186547,1.,
0.707106781186547,1.,0.707106781186547,1.,0.707106781186547,1.),(1.,0.707106781186548,
1.,0.707106781186548,1.,0.707106781186548,1.,0.707106781186548,1.),(1.,
0.707106781186547,1.,0.707106781186547,1.,0.707106781186547,1.,0.707106781186547,
1.),(1.,0.707106781186548,1.,0.707106781186548,1.,0.707106781186548,1.,
0.707106781186548,1.),(1.,0.707106781186547,1.,0.707106781186547,1.,0.707106781186547,
1.,0.707106781186547,1.),(1.,0.707106781186548,1.,0.707106781186548,1.,
0.707106781186548,1.,0.707106781186548,1.),(1.,0.707106781186548,1.,0.707106781186548,
1.,0.707106781186548,1.,0.707106781186548,1.),(1.,0.707106781186548,1.,
0.707106781186548,1.,0.707106781186548,1.,0.707106781186548,1.),(1.,0.707106781186548,
1.,0.707106781186548,1.,0.707106781186548,1.,0.707106781186548,1.),(1.,
0.707106781186547,1.,0.707106781186547,1.,0.707106781186547,1.,0.707106781186547,
1.),(1.,0.707106781186547,1.,0.707106781186547,1.,0.707106781186547,1.,
0.707106781186547,1.),(1.,0.707106781186547,1.,0.707106781186547,1.,0.707106781186547,
1.,0.707106781186547,1.),(1.,0.707106781186548,1.,0.707106781186548,1.,
0.707106781186548,1.,0.707106781186548,1.),(1.,0.707106781186547,1.,0.707106781186547,
1.,0.707106781186547,1.,0.707106781186547,1.),(1.,0.707106781186548,1.,
0.707106781186548,1.,0.707106781186548,1.,0.707106781186548,1.),(1.,0.707106781186547,
1.,0.707106781186547,1.,0.707106781186547,1.,0.707106781186547,1.),(1.,
0.707106781186547,1.,0.707106781186547,1.,0.707106781186547,1.,0.707106781186547,
1.),(1.,0.707106781186548,1.,0.707106781186548,1.,0.707106781186548,1.,
0.707106781186548,1.),(1.,0.707106781186547,1.,0.707106781186547,1.,0.707106781186547,
1.,0.707106781186547,1.),(1.,0.707106781186547,1.,0.707106781186547,1.,
0.707106781186547,1.,0.707106781186547,1.),(1.,0.707106781186548,1.,0.707106781186548,
1.,0.707106781186548,1.,0.707106781186548,1.),(1.,0.707106781186547,1.,
0.707106781186547,1.,0.707106781186547,1.,0.707106781186547,1.),(1.,0.707106781186547,
1.,0.707106781186547,1.,0.707106781186547,1.,0.707106781186547,1.),(1.,
0.707106781186548,1.,0.707106781186548,1.,0.707106781186548,1.,0.707106781186548,
1.),(1.,0.707106781186548,1.,0.707106781186548,1.,0.707106781186548,1.,
0.707106781186548,1.),(1.,0.707106781186547,1.,0.707106781186547,1.,0.707106781186547,
1.,0.707106781186547,1.),(1.,0.707106781186548,1.,0.707106781186548,1.,
0.707106781186548,1.,0.707106781186548,1.),(1.,0.707106781186547,1.,0.707106781186547,
1.,0.707106781186547,1.,0.707106781186547,1.),(1.,0.707106781186547,1.,
0.707106781186547,1.,0.707106781186547,1.,0.707106781186547,1.),(1.,0.707106781186548,
1.,0.707106781186548,1.,0.707106781186548,1.,0.707106781186548,1.),(1.,
0.707106781186547,1.,0.707106781186547,1.,0.707106781186547,1.,0.707106781186547,
1.),(1.,0.707106781186548,1.,0.707106781186548,1.,0.707106781186548,1.,
0.707106781186548,1.),(1.,0.707106781186547,1.,0.707106781186547,1.,0.707106781186547,
1.,0.707106781186547,1.),(1.,0.707106781186548,1.,0.707106781186548,1.,
0.707106781186548,1.,0.707106781186548,1.),(1.,0.707106781186547,1.,0.707106781186547,
1.,0.707106781186547,1.,0.707106781186547,1.),(1.,0.707106781186547,1.,
0.707106781186547,1.,0.707106781186547,1.,0.707106781186547,1.),(1.,0.707106781186547,
1.,0.707106781186547,1.,0.707106781186547,1.,0.707106781186547,1.),(1.,
0.707106781186548,1.,0.707106781186548,1.,0.707106781186548,1.,0.707106781186548,
1.),(1.,0.707106781186547,1.,0.707106781186547,1.,0.707106781186547,1.,
0.707106781186547,1.),(1.,0.707106781186548,1.,0.707106781186548,1.,0.707106781186548,
1.,0.707106781186548,1.),(1.,0.707106781186547,1.,0.707106781186547,1.,
0.707106781186547,1.,0.707106781186547,1.),(1.,0.707106781186548,1.,0.707106781186548,
1.,0.707106781186548,1.,0.707106781186548,1.),(1.,0.707106781186547,1.,
0.707106781186547,1.,0.707106781186547,1.,0.707106781186547,1.),(1.,0.707106781186547,
1.,0.707106781186547,1.,0.707106781186547,1.,0.707106781186547,1.),(1.,
0.707106781186548,1.,0.707106781186548,1.,0.707106781186548,1.,0.707106781186548,
1.),(1.,0.707106781186548,1.,0.707106781186548,1.,0.707106781186548,1.,
0.707106781186548,1.),(1.,0.707106781186548,1.,0.707106781186548,1.,0.707106781186548,
1.,0.707106781186548,1.),(1.,0.707106781186547,1.,0.707106781186547,1.,
0.707106781186547,1.,0.707106781186547,1.),(1.,0.707106781186548,1.,0.707106781186548,
1.,0.707106781186548,1.,0.707106781186548,1.),(1.,0.707106781186547,1.,
0.707106781186547,1.,0.707106781186547,1.,0.707106781186547,1.),(1.,0.707106781186548,
1.,0.707106781186548,1.,0.707106781186548,1.,0.707106781186548,1.),(1.,
0.707106781186547,1.,0.707106781186547,1.,0.707106781186547,1.,0.707106781186547,
1.),(1.,0.707106781186548,1.,0.707106781186548,1.,0.707106781186548,1.,
0.707106781186548,1.),(1.,0.707106781186547,1.,0.707106781186547,1.,0.707106781186547,
1.,0.707106781186547,1.),(1.,0.707106781186548,1.,0.707106781186548,1.,
0.707106781186548,1.,0.707106781186548,1.),(1.,0.707106781186548,1.,0.707106781186548,
1.,0.707106781186548,1.,0.707106781186548,1.),(1.,0.707106781186547,1.,
0.707106781186547,1.,0.707106781186547,1.,0.707106781186547,1.),(1.,0.707106781186547,
1.,0.707106781186547,1.,0.707106781186547,1.,0.707106781186547,1.),(1.,
0.707106781186547,1.,0.707106781186547,1.,0.707106781186547,1.,0.707106781186547,
1.),(1.,0.707106781186548,1.,0.707106781186548,1.,0.707106781186548,1.,
0.707106781186548,1.),(1.,0.707106781186547,1.,0.707106781186547,1.,0.707106781186547,
1.,0.707106781186547,1.),(1.,0.707106781186547,1.,0.707106781186547,1.,
0.707106781186547,1.,0.707106781186547,1.),(1.,0.707106781186548,1.,0.707106781186548,
1.,0.707106781186548,1.,0.707106781186548,1.),(1.,0.707106781186547,1.,
0.707106781186547,1.,0.707106781186547,1.,0.707106781186547,1.),(1.,0.707106781186547,
1.,0.707106781186547,1.,0.707106781186547,1.,0.707106781186547,1.),(1.,
0.707106781186548,1.,0.707106781186548,1.,0.707106781186548,1.,0.707106781186548,
1.),(1.,0.707106781186547,1.,0.707106781186547,1.,0.707106781186547,1.,
0.707106781186547,1.),(1.,0.707106781186548,1.,0.707106781186548,1.,0.707106781186548,
1.,0.707106781186548,1.),(1.,0.707106781186548,1.,0.707106781186548,1.,
0.707106781186548,1.,0.707106781186548,1.),(1.,0.707106781186548,1.,0.707106781186548,
1.,0.707106781186548,1.,0.707106781186548,1.),(1.,0.707106781186547,1.,
0.707106781186547,1.,0.707106781186547,1.,0.707106781186547,1.),(1.,0.707106781186548,
1.,0.707106781186548,1.,0.707106781186548,1.,0.707106781186548,1.),(1.,
0.707106781186547,1.,0.707106781186547,1.,0.707106781186547,1.,0.707106781186547,
1.),(1.,0.707106781186548,1.,0.707106781186548,1.,0.707106781186548,1.,
0.707106781186548,1.),(1.,0.707106781186547,1.,0.707106781186547,1.,0.707106781186547,
1.,0.707106781186547,1.),(1.,0.707106781186548,1.,0.707106781186548,1.,
0.707106781186548,1.,0.707106781186548,1.),(1.,0.707106781186547,1.,0.707106781186547,
1.,0.707106781186547,1.,0.707106781186547,1.),(1.,0.707106781186548,1.,
0.707106781186548,1.,0.707106781186548,1.,0.707106781186548,1.),(1.,0.707106781186547,
1.,0.707106781186547,1.,0.707106781186547,1.,0.707106781186547,1.),(1.,
0.707106781186548,1.,0.707106781186548,1.,0.707106781186548,1.,0.707106781186548,
1.),(1.,0.707106781186547,1.,0.707106781186547,1.,0.707106781186547,1.,
0.707106781186547,1.),(1.,0.707106781186548,1.,0.707106781186548,1.,0.707106781186548,
1.,0.707106781186548,1.),(1.,0.707106781186548,1.,0.707106781186548,1.,
0.707106781186548,1.,0.707106781186548,1.),(1.,0.707106781186547,1.,0.707106781186547,
1.,0.707106781186547,1.,0.707106781186547,1.),(1.,0.707106781186548,1.,
0.707106781186548,1.,0.707106781186548,1.,0.707106781186548,1.),(1.,0.707106781186547,
1.,0.707106781186547,1.,0.707106781186547,1.,0.707106781186547,1.),(1.,
0.707106781186548,1.,0.707106781186548,1.,0.707106781186548,1.,0.707106781186548,
1.),(1.,0.707106781186548,1.,0.707106781186548,1.,0.707106781186548,1.,
0.707106781186548,1.),(1.,0.707106781186547,1.,0.707106781186547,1.,0.707106781186547,
1.,0.707106781186547,1.),(1.,0.707106781186547,1.,0.707106781186547,1.,
0.707106781186547,1.,0.707106781186547,1.),(1.,0.707106781186548,1.,0.707106781186548,
1.,0.707106781186548,1.,0.707106781186548,1.),(1.,0.707106781186547,1.,
0.707106781186547,1.,0.707106781186547,1.,0.707106781186547,1.),(1.,0.707106781186547,
1.,0.707106781186547,1.,0.707106781186547,1.,0.707106781186547,1.),(1.,
0.707106781186548,1.,0.707106781186548,1.,0.707106781186548,1.,0.707106781186548,
1.),(1.,0.707106781186547,1.,0.707106781186547,1.,0.707106781186547,1.,
0.707106781186547,1.),(1.,0.707106781186548,1.,0.707106781186548,1.,0.707106781186548,
1.,0.707106781186548,1.),(1.,0.707106781186548,1.,0.707106781186548,1.,
0.707106781186548,1.,0.707106781186548,1.),(1.,0.707106781186547,1.,0.707106781186547,
1.,0.707106781186547,1.,0.707106781186547,1.),(1.,0.707106781186548,1.,
0.707106781186548,1.,0.707106781186548,1.,0.707106781186548,1.),(1.,0.707106781186548,
1.,0.707106781186548,1.,0.707106781186548,1.,0.707106781186548,1.),(1.,
0.707106781186548,1.,0.707106781186548,1.,0.707106781186548,1.,0.707106781186548,
1.),(1.,0.707106781186548,1.,0.707106781186548,1.,0.707106781186548,1.,
0.707106781186548,1.),(1.,0.707106781186548,1.,0.707106781186548,1.,0.707106781186548,
1.,0.707106781186548,1.),(1.,0.707106781186547,1.,0.707106781186547,1.,
0.707106781186547,1.,0.707106781186547,1.),(1.,0.707106781186548,1.,0.707106781186548,
1.,0.707106781186548,1.,0.707106781186548,1.),(1.,0.707106781186548,1.,
0.707106781186548,1.,0.707106781186548,1.,0.707106781186548,1.),(1.,0.707106781186548,
1.,0.707106781186548,1.,0.707106781186548,1.,0.707106781186548,1.),(1.,
0.707106781186547,1.,0.707106781186547,1.,0.707106781186547,1.,0.707106781186547,
1.),(1.,0.707106781186548,1.,0.707106781186548,1.,0.707106781186548,1.,
0.707106781186548,1.),(1.,0.707106781186547,1.,0.707106781186547,1.,0.707106781186547,
1.,0.707106781186547,1.),(1.,0.707106781186548,1.,0.707106781186548,1.,
0.707106781186548,1.,0.707106781186548,1.),(1.,0.707106781186547,1.,0.707106781186547,
1.,0.707106781186547,1.,0.707106781186547,1.),(1.,0.707106781186548,1.,
0.707106781186548,1.,0.707106781186548,1.,0.707106781186548,1.),(1.,0.707106781186547,
1.,0.707106781186547,1.,0.707106781186547,1.,0.707106781186547,1.),(1.,
0.707106781186548,1.,0.707106781186548,1.,0.707106781186548,1.,0.707106781186548,
1.),(1.,0.707106781186547,1.,0.707106781186547,1.,0.707106781186547,1.,
0.707106781186547,1.),(1.,0.707106781186548,1.,0.707106781186548,1.,0.707106781186548,
1.,0.707106781186548,1.),(1.,0.707106781186547,1.,0.707106781186547,1.,
0.707106781186547,1.,0.707106781186547,1.),(1.,0.707106781186547,1.,0.707106781186547,
1.,0.707106781186547,1.,0.707106781186547,1.),(1.,0.707106781186548,1.,
0.707106781186548,1.,0.707106781186548,1.,0.707106781186548,1.),(1.,0.707106781186547,
1.,0.707106781186547,1.,0.707106781186547,1.,0.707106781186547,1.),(1.,
0.707106781186547,1.,0.707106781186547,1.,0.707106781186547,1.,0.707106781186547,
1.),(1.,0.707106781186548,1.,0.707106781186548,1.,0.707106781186548,1.,
0.707106781186548,1.),(1.,0.707106781186547,1.,0.707106781186547,1.,0.707106781186547,
1.,0.707106781186547,1.),(1.,0.707106781186548,1.,0.707106781186548,1.,
0.707106781186548,1.,0.707106781186548,1.),(1.,0.707106781186547,1.,0.707106781186547,
1.,0.707106781186547,1.,0.707106781186547,1.),(1.,0.707106781186548,1.,
0.707106781186548,1.,0.707106781186548,1.,0.707106781186548,1.),(1.,0.707106781186547,
1.,0.707106781186547,1.,0.707106781186547,1.,0.707106781186547,1.),(1.,
0.707106781186548,1.,0.707106781186548,1.,0.707106781186548,1.,0.707106781186548,
1.),(1.,0.707106781186547,1.,0.707106781186547,1.,0.707106781186547,1.,
0.707106781186547,1.),(1.,0.707106781186547,1.,0.707106781186547,1.,0.707106781186547,
1.,0.707106781186547,1.),(1.,0.707106781186548,1.,0.707106781186548,1.,
0.707106781186548,1.,0.707106781186548,1.),(1.,0.707106781186547,1.,0.707106781186547,
1.,0.707106781186547,1.,0.707106781186547,1.),(1.,0.707106781186547,1.,
0.707106781186547,1.,0.707106781186547,1.,0.707106781186547,1.),(1.,0.707106781186548,
1.,0.707106781186548,1.,0.707106781186548,1.,0.707106781186548,1.),(1.,
0.707106781186547,1.,0.707106781186547,1.,0.707106781186547,1.,0.707106781186547,
1.),(1.,0.707106781186548,1.,0.707106781186548,1.,0.707106781186548,1.,
0.707106781186548,1.),(1.,0.707106781186547,1.,0.707106781186547,1.,0.707106781186547,
1.,0.707106781186547,1.),(1.,0.707106781186547,1.,0.707106781186547,1.,
0.707106781186547,1.,0.707106781186547,1.),(1.,0.707106781186548,1.,0.707106781186548,
1.,0.707106781186548,1.,0.707106781186548,1.),(1.,0.707106781186548,1.,
0.707106781186548,1.,0.707106781186548,1.,0.707106781186548,1.),(1.,0.707106781186547,
1.,0.707106781186547,1.,0.707106781186547,1.,0.707106781186547,1.),(1.,
0.707106781186548,1.,0.707106781186548,1.,0.707106781186548,1.,0.707106781186548,
1.),(1.,0.707106781186547,1.,0.707106781186547,1.,0.707106781186547,1.,
0.707106781186547,1.),(1.,0.707106781186547,1.,0.707106781186547,1.,0.707106781186547,
1.,0.707106781186547,1.),(1.,0.707106781186547,1.,0.707106781186547,1.,
0.707106781186547,1.,0.707106781186547,1.),(1.,0.707106781186548,1.,0.707106781186548,
1.,0.707106781186548,1.,0.707106781186548,1.),(1.,0.707106781186547,1.,
0.707106781186547,1.,0.707106781186547,1.,0.707106781186547,1.),(1.,0.707106781186547,
1.,0.707106781186547,1.,0.707106781186547,1.,0.707106781186547,1.),(1.,
0.707106781186548,1.,0.707106781186548,1.,0.707106781186548,1.,0.707106781186548,
1.),(1.,0.707106781186547,1.,0.707106781186547,1.,0.707106781186547,1.,
0.707106781186547,1.),(1.,0.707106781186547,1.,0.707106781186547,1.,0.707106781186547,
1.,0.707106781186547,1.),(1.,0.707106781186547,1.,0.707106781186547,1.,
0.707106781186547,1.,0.707106781186547,1.),(1.,0.707106781186548,1.,0.707106781186548,
1.,0.707106781186548,1.,0.707106781186548,1.),(1.,0.707106781186548,1.,
0.707106781186548,1.,0.707106781186548,1.,0.707106781186548,1.),(1.,0.707106781186547,
1.,0.707106781186547,1.,0.707106781186547,1.,0.707106781186547,1.),(1.,
0.707106781186548,1.,0.707106781186548,1.,0.707106781186548,1.,0.707106781186548,
1.),(1.,0.707106781186547,1.,0.707106781186547,1.,0.707106781186547,1.,
0.707106781186547,1.),(1.,0.707106781186548,1.,0.707106781186548,1.,0.707106781186548,
1.,0.707106781186548,1.),(1.,0.707106781186547,1.,0.707106781186547,1.,
0.707106781186547,1.,0.707106781186547,1.),(1.,0.707106781186547,1.,0.707106781186547,
1.,0.707106781186547,1.,0.707106781186547,1.),(1.,0.707106781186548,1.,
0.707106781186548,1.,0.707106781186548,1.,0.707106781186548,1.),(1.,0.707106781186547,
1.,0.707106781186547,1.,0.707106781186547,1.,0.707106781186547,1.),(1.,
0.707106781186548,1.,0.707106781186548,1.,0.707106781186548,1.,0.707106781186548,
1.),(1.,0.707106781186547,1.,0.707106781186547,1.,0.707106781186547,1.,
0.707106781186547,1.),(1.,0.707106781186547,1.,0.707106781186547,1.,0.707106781186547,
1.,0.707106781186547,1.),(1.,0.707106781186547,1.,0.707106781186547,1.,
0.707106781186547,1.,0.707106781186547,1.),(1.,0.707106781186547,1.,0.707106781186547,
1.,0.707106781186547,1.,0.707106781186547,1.),(1.,0.707106781186548,1.,
0.707106781186548,1.,0.707106781186548,1.,0.707106781186548,1.),(1.,0.707106781186547,
1.,0.707106781186547,1.,0.707106781186547,1.,0.707106781186547,1.),(1.,
0.707106781186547,1.,0.707106781186547,1.,0.707106781186547,1.,0.707106781186547,
1.),(1.,0.707106781186547,1.,0.707106781186547,1.,0.707106781186547,1.,
0.707106781186547,1.),(1.,0.707106781186547,1.,0.707106781186547,1.,0.707106781186547,
1.,0.707106781186547,1.),(1.,0.707106781186547,1.,0.707106781186547,1.,
0.707106781186547,1.,0.707106781186547,1.),(1.,0.707106781186548,1.,0.707106781186548,
1.,0.707106781186548,1.,0.707106781186548,1.),(1.,0.707106781186547,1.,
0.707106781186547,1.,0.707106781186547,1.,0.707106781186547,1.),(1.,0.707106781186547,
1.,0.707106781186547,1.,0.707106781186547,1.,0.707106781186547,1.),(1.,
0.707106781186547,1.,0.707106781186547,1.,0.707106781186547,1.,0.707106781186547,
1.),(1.,0.707106781186547,1.,0.707106781186547,1.,0.707106781186547,1.,
0.707106781186547,1.),(1.,0.707106781186548,1.,0.707106781186548,1.,0.707106781186548,
1.,0.707106781186548,1.),(1.,0.707106781186547,1.,0.707106781186547,1.,
0.707106781186547,1.,0.707106781186547,1.),(1.,0.707106781186548,1.,0.707106781186548,
1.,0.707106781186548,1.,0.707106781186548,1.),(1.,0.707106781186547,1.,
0.707106781186547,1.,0.707106781186547,1.,0.707106781186547,1.),(1.,0.707106781186547,
1.,0.707106781186547,1.,0.707106781186547,1.,0.707106781186547,1.),(1.,
0.707106781186548,1.,0.707106781186548,1.,0.707106781186548,1.,0.707106781186548,
1.),(1.,0.707106781186547,1.,0.707106781186547,1.,0.707106781186547,1.,
0.707106781186547,1.),(1.,0.707106781186548,1.,0.707106781186548,1.,0.707106781186548,
1.,0.707106781186548,1.),(1.,0.707106781186547,1.,0.707106781186547,1.,
0.707106781186547,1.,0.707106781186547,1.),(1.,0.707106781186547,1.,0.707106781186547,
1.,0.707106781186547,1.,0.707106781186547,1.),(1.,0.707106781186548,1.,
0.707106781186548,1.,0.707106781186548,1.,0.707106781186548,1.),(1.,0.707106781186547,
1.,0.707106781186547,1.,0.707106781186547,1.,0.707106781186547,1.),(1.,
0.707106781186547,1.,0.707106781186547,1.,0.707106781186547,1.,0.707106781186547,
1.),(1.,0.707106781186548,1.,0.707106781186548,1.,0.707106781186548,1.,
0.707106781186548,1.),(1.,0.707106781186547,1.,0.707106781186547,1.,0.707106781186547,
1.,0.707106781186547,1.),(1.,0.707106781186547,1.,0.707106781186547,1.,
0.707106781186547,1.,0.707106781186547,1.),(1.,0.707106781186547,1.,0.707106781186547,
1.,0.707106781186547,1.,0.707106781186547,1.),(1.,0.707106781186547,1.,
0.707106781186547,1.,0.707106781186547,1.,0.707106781186547,1.),(1.,0.707106781186548,
1.,0.707106781186548,1.,0.707106781186548,1.,0.707106781186548,1.),(1.,
0.707106781186547,1.,0.707106781186547,1.,0.707106781186547,1.,0.707106781186547,
1.),(1.,0.707106781186548,1.,0.707106781186548,1.,0.707106781186548,1.,
0.707106781186548,1.),(1.,0.707106781186548,1.,0.707106781186548,1.,0.707106781186548,
1.,0.707106781186548,1.),(1.,0.707106781186547,1.,0.707106781186547,1.,
0.707106781186547,1.,0.707106781186547,1.),(1.,0.707106781186548,1.,0.707106781186548,
1.,0.707106781186548,1.,0.707106781186548,1.),(1.,0.707106781186548,1.,
0.707106781186548,1.,0.707106781186548,1.,0.707106781186548,1.),(1.,0.707106781186547,
1.,0.707106781186547,1.,0.707106781186547,1.,0.707106781186547,1.),(1.,
0.707106781186547,1.,0.707106781186547,1.,0.707106781186547,1.,0.707106781186547,
1.),(1.,0.707106781186548,1.,0.707106781186548,1.,0.707106781186548,1.,
0.707106781186548,1.),(1.,0.707106781186547,1.,0.707106781186547,1.,0.707106781186547,
1.,0.707106781186547,1.),(1.,0.707106781186547,1.,0.707106781186547,1.,
0.707106781186547,1.,0.707106781186547,1.),(1.,0.707106781186547,1.,0.707106781186547,
1.,0.707106781186547,1.,0.707106781186547,1.),(1.,0.707106781186548,1.,
0.707106781186548,1.,0.707106781186548,1.,0.707106781186548,1.),(1.,0.707106781186547,
1.,0.707106781186547,1.,0.707106781186547,1.,0.707106781186547,1.),(1.,
0.707106781186547,1.,0.707106781186547,1.,0.707106781186547,1.,0.707106781186547,
1.),(1.,0.707106781186548,1.,0.707106781186548,1.,0.707106781186548,1.,
0.707106781186548,1.),(1.,0.707106781186547,1.,0.707106781186547,1.,0.707106781186547,
1.,0.707106781186547,1.),(1.,0.707106781186548,1.,0.707106781186548,1.,
0.707106781186548,1.,0.707106781186548,1.),(1.,0.707106781186547,1.,0.707106781186547,
1.,0.707106781186547,1.,0.707106781186547,1.),(1.,0.707106781186548,1.,
0.707106781186548,1.,0.707106781186548,1.,0.707106781186548,1.),(1.,0.707106781186547,
1.,0.707106781186547,1.,0.707106781186547,1.,0.707106781186547,1.),(1.,
0.707106781186547,1.,0.707106781186547,1.,0.707106781186547,1.,0.707106781186547,
1.),(1.,0.707106781186548,1.,0.707106781186548,1.,0.707106781186548,1.,
0.707106781186548,1.),(1.,0.707106781186547,1.,0.707106781186547,1.,0.707106781186547,
1.,0.707106781186547,1.),(1.,0.707106781186548,1.,0.707106781186548,1.,
0.707106781186548,1.,0.707106781186548,1.),(1.,0.707106781186547,1.,0.707106781186547,
1.,0.707106781186547,1.,0.707106781186547,1.),(1.,0.707106781186548,1.,
0.707106781186548,1.,0.707106781186548,1.,0.707106781186548,1.),(1.,0.707106781186547,
1.,0.707106781186547,1.,0.707106781186547,1.,0.707106781186547,1.),(1.,
0.707106781186548,1.,0.707106781186548,1.,0.707106781186548,1.,0.707106781186548,
1.),(1.,0.707106781186547,1.,0.707106781186547,1.,0.707106781186547,1.,
0.707106781186547,1.),(1.,0.707106781186548,1.,0.707106781186548,1.,0.707106781186548,
1.,0.707106781186548,1.),(1.,0.707106781186547,1.,0.707106781186547,1.,
0.707106781186547,1.,0.707106781186547,1.),(1.,0.707106781186547,1.,0.707106781186547,
1.,0.707106781186547,1.,0.707106781186547,1.),(1.,0.707106781186547,1.,
0.707106781186547,1.,0.707106781186547,1.,0.707106781186547,1.),(1.,0.707106781186547,
1.,0.707106781186547,1.,0.707106781186547,1.,0.707106781186547,1.),(1.,
0.707106781186548,1.,0.707106781186548,1.,0.707106781186548,1.,0.707106781186548,
1.),(1.,0.707106781186548,1.,0.707106781186548,1.,0.707106781186548,1.,
0.707106781186548,1.),(1.,0.707106781186547,1.,0.707106781186547,1.,0.707106781186547,
1.,0.707106781186547,1.),(1.,0.707106781186548,1.,0.707106781186548,1.,
0.707106781186548,1.,0.707106781186548,1.),(1.,0.707106781186548,1.,0.707106781186548,
1.,0.707106781186548,1.,0.707106781186548,1.),(1.,0.707106781186547,1.,
0.707106781186547,1.,0.707106781186547,1.,0.707106781186547,1.),(1.,0.707106781186548,
1.,0.707106781186548,1.,0.707106781186548,1.,0.707106781186548,1.),(1.,
0.707106781186547,1.,0.707106781186547,1.,0.707106781186547,1.,0.707106781186547,
1.),(1.,0.707106781186547,1.,0.707106781186547,1.,0.707106781186547,1.,
0.707106781186547,1.),(1.,0.707106781186548,1.,0.707106781186548,1.,0.707106781186548,
1.,0.707106781186548,1.),(1.,0.707106781186547,1.,0.707106781186547,1.,
0.707106781186547,1.,0.707106781186547,1.),(1.,0.707106781186547,1.,0.707106781186547,
1.,0.707106781186547,1.,0.707106781186547,1.),(1.,0.707106781186547,1.,
0.707106781186547,1.,0.707106781186547,1.,0.707106781186547,1.),(1.,0.707106781186547,
1.,0.707106781186547,1.,0.707106781186547,1.,0.707106781186547,1.),(1.,
0.707106781186548,1.,0.707106781186548,1.,0.707106781186548,1.,0.707106781186548,
1.),(1.,0.707106781186547,1.,0.707106781186547,1.,0.707106781186547,1.,
0.707106781186547,1.),(1.,0.707106781186547,1.,0.707106781186547,1.,0.707106781186547,
1.,0.707106781186547,1.),(1.,0.707106781186547,1.,0.707106781186547,1.,
0.707106781186547,1.,0.707106781186547,1.),(1.,0.707106781186548,1.,0.707106781186548,
1.,0.707106781186548,1.,0.707106781186548,1.),(1.,0.707106781186547,1.,
0.707106781186547,1.,0.707106781186547,1.,0.707106781186547,1.),(1.,0.707106781186547,
1.,0.707106781186547,1.,0.707106781186547,1.,0.707106781186547,1.),(1.,
0.707106781186548,1.,0.707106781186548,1.,0.707106781186548,1.,0.707106781186548,
1.),(1.,0.707106781186547,1.,0.707106781186547,1.,0.707106781186547,1.,
0.707106781186547,1.),(1.,0.707106781186548,1.,0.707106781186548,1.,0.707106781186548,
1.,0.707106781186548,1.),(1.,0.707106781186548,1.,0.707106781186548,1.,
0.707106781186548,1.,0.707106781186548,1.),(1.,0.707106781186547,1.,0.707106781186547,
1.,0.707106781186547,1.,0.707106781186547,1.),(1.,0.707106781186548,1.,
0.707106781186548,1.,0.707106781186548,1.,0.707106781186548,1.),(1.,0.707106781186547,
1.,0.707106781186547,1.,0.707106781186547,1.,0.707106781186547,1.),(1.,
0.707106781186548,1.,0.707106781186548,1.,0.707106781186548,1.,0.707106781186548,
1.),(1.,0.707106781186547,1.,0.707106781186547,1.,0.707106781186547,1.,
0.707106781186547,1.),(1.,0.707106781186548,1.,0.707106781186548,1.,0.707106781186548,
1.,0.707106781186548,1.),(1.,0.707106781186547,1.,0.707106781186547,1.,
0.707106781186547,1.,0.707106781186547,1.),(1.,0.707106781186547,1.,0.707106781186547,
1.,0.707106781186547,1.,0.707106781186547,1.),(1.,0.707106781186548,1.,
0.707106781186548,1.,0.707106781186548,1.,0.707106781186548,1.),(1.,0.707106781186547,
1.,0.707106781186547,1.,0.707106781186547,1.,0.707106781186547,1.),(1.,
0.707106781186548,1.,0.707106781186548,1.,0.707106781186548,1.,0.707106781186548,
1.),(1.,0.707106781186548,1.,0.707106781186548,1.,0.707106781186548,1.,
0.707106781186548,1.),(1.,0.707106781186547,1.,0.707106781186547,1.,0.707106781186547,
1.,0.707106781186547,1.),(1.,0.707106781186547,1.,0.707106781186547,1.,
0.707106781186547,1.,0.707106781186547,1.),(1.,0.707106781186548,1.,0.707106781186548,
1.,0.707106781186548,1.,0.707106781186548,1.),(1.,0.707106781186547,1.,
0.707106781186547,1.,0.707106781186547,1.,0.707106781186547,1.),(1.,0.707106781186548,
1.,0.707106781186548,1.,0.707106781186548,1.,0.707106781186548,1.),(1.,
0.707106781186547,1.,0.707106781186547,1.,0.707106781186547,1.,0.707106781186547,
1.),(1.,0.707106781186548,1.,0.707106781186548,1.,0.707106781186548,1.,
0.707106781186548,1.),(1.,0.707106781186547,1.,0.707106781186547,1.,0.707106781186547,
1.,0.707106781186547,1.),(1.,0.707106781186547,1.,0.707106781186547,1.,
0.707106781186547,1.,0.707106781186547,1.),(1.,0.707106781186548,1.,0.707106781186548,
1.,0.707106781186548,1.,0.707106781186548,1.),(1.,0.707106781186548,1.,
0.707106781186548,1.,0.707106781186548,1.,0.707106781186548,1.),(1.,0.707106781186547,
1.,0.707106781186547,1.,0.707106781186547,1.,0.707106781186547,1.),(1.,
0.707106781186548,1.,0.707106781186548,1.,0.707106781186548,1.,0.707106781186548,
1.),(1.,0.707106781186548,1.,0.707106781186548,1.,0.707106781186548,1.,
0.707106781186548,1.),(1.,0.707106781186547,1.,0.707106781186547,1.,0.707106781186547,
1.,0.707106781186547,1.),(1.,0.707106781186548,1.,0.707106781186548,1.,
0.707106781186548,1.,0.707106781186548,1.),(1.,0.707106781186548,1.,0.707106781186548,
1.,0.707106781186548,1.,0.707106781186548,1.),(1.,0.707106781186547,1.,
0.707106781186547,1.,0.707106781186547,1.,0.707106781186547,1.),(1.,0.707106781186548,
1.,0.707106781186548,1.,0.707106781186548,1.,0.707106781186548,1.),(1.,
0.707106781186547,1.,0.707106781186547,1.,0.707106781186547,1.,0.707106781186547,
1.),(1.,0.707106781186548,1.,0.707106781186548,1.,0.707106781186548,1.,
0.707106781186548,1.),(1.,0.707106781186547,1.,0.707106781186547,1.,0.707106781186547,
1.,0.707106781186547,1.),(1.,0.707106781186548,1.,0.707106781186548,1.,
0.707106781186548,1.,0.707106781186548,1.),(1.,0.707106781186547,1.,0.707106781186547,
1.,0.707106781186547,1.,0.707106781186547,1.),(1.,0.707106781186548,1.,
0.707106781186548,1.,0.707106781186548,1.,0.707106781186548,1.),(1.,0.707106781186547,
1.,0.707106781186547,1.,0.707106781186547,1.,0.707106781186547,1.),(1.,
0.707106781186547,1.,0.707106781186547,1.,0.707106781186547,1.,0.707106781186547,
1.),(1.,0.707106781186548,1.,0.707106781186548,1.,0.707106781186548,1.,
0.707106781186548,1.),(1.,0.707106781186547,1.,0.707106781186547,1.,0.707106781186547,
1.,0.707106781186547,1.),(1.,0.707106781186547,1.,0.707106781186547,1.,
0.707106781186547,1.,0.707106781186547,1.),(1.,0.707106781186548,1.,0.707106781186548,
1.,0.707106781186548,1.,0.707106781186548,1.),(1.,0.707106781186547,1.,
0.707106781186547,1.,0.707106781186547,1.,0.707106781186547,1.),(1.,0.707106781186548,
1.,0.707106781186548,1.,0.707106781186548,1.,0.707106781186548,1.),(1.,
0.707106781186548,1.,0.707106781186548,1.,0.707106781186548,1.,0.707106781186548,
1.),(1.,0.707106781186547,1.,0.707106781186547,1.,0.707106781186547,1.,
0.707106781186547,1.),(1.,0.707106781186547,1.,0.707106781186547,1.,0.707106781186547,
1.,0.707106781186547,1.),(1.,0.707106781186547,1.,0.707106781186547,1.,
0.707106781186547,1.,0.707106781186547,1.),(1.,0.707106781186548,1.,0.707106781186548,
1.,0.707106781186548,1.,0.707106781186548,1.),(1.,0.707106781186547,1.,
0.707106781186547,1.,0.707106781186547,1.,0.707106781186547,1.),(1.,0.707106781186548,
1.,0.707106781186548,1.,0.707106781186548,1.,0.707106781186548,1.),(1.,
0.707106781186548,1.,0.707106781186548,1.,0.707106781186548,1.,0.707106781186548,
1.),(1.,0.707106781186547,1.,0.707106781186547,1.,0.707106781186547,1.,
0.707106781186547,1.),(1.,0.707106781186548,1.,0.707106781186548,1.,0.707106781186548,
1.,0.707106781186548,1.),(1.,0.707106781186547,1.,0.707106781186547,1.,
0.707106781186547,1.,0.707106781186547,1.),(1.,0.707106781186548,1.,0.707106781186548,
1.,0.707106781186548,1.,0.707106781186548,1.),(1.,0.707106781186547,1.,
0.707106781186547,1.,0.707106781186547,1.,0.707106781186547,1.),(1.,0.707106781186548,
1.,0.707106781186548,1.,0.707106781186548,1.,0.707106781186548,1.),(1.,
0.707106781186547,1.,0.707106781186547,1.,0.707106781186547,1.,0.707106781186547,
1.),(1.,0.707106781186547,1.,0.707106781186547,1.,0.707106781186547,1.,
0.707106781186547,1.),(1.,0.707106781186548,1.,0.707106781186548,1.,0.707106781186548,
1.,0.707106781186548,1.),(1.,0.707106781186548,1.,0.707106781186548,1.,
0.707106781186548,1.,0.707106781186548,1.),(1.,0.707106781186548,1.,0.707106781186548,
1.,0.707106781186548,1.,0.707106781186548,1.),(1.,0.707106781186547,1.,
0.707106781186547,1.,0.707106781186547,1.,0.707106781186547,1.),(1.,0.707106781186548,
1.,0.707106781186548,1.,0.707106781186548,1.,0.707106781186548,1.),(1.,
0.707106781186548,1.,0.707106781186548,1.,0.707106781186548,1.,0.707106781186548,
1.),(1.,0.707106781186547,1.,0.707106781186547,1.,0.707106781186547,1.,
0.707106781186547,1.),(1.,0.707106781186548,1.,0.707106781186548,1.,0.707106781186548,
1.,0.707106781186548,1.),(1.,0.707106781186547,1.,0.707106781186547,1.,
0.707106781186547,1.,0.707106781186547,1.),(1.,0.707106781186548,1.,0.707106781186548,
1.,0.707106781186548,1.,0.707106781186548,1.),(1.,0.707106781186548,1.,
0.707106781186548,1.,0.707106781186548,1.,0.707106781186548,1.),(1.,0.707106781186548,
1.,0.707106781186548,1.,0.707106781186548,1.,0.707106781186548,1.),(1.,
0.707106781186548,1.,0.707106781186548,1.,0.707106781186548,1.,0.707106781186548,
1.),(1.,0.707106781186548,1.,0.707106781186548,1.,0.707106781186548,1.,
0.707106781186548,1.),(1.,0.707106781186548,1.,0.707106781186548,1.,0.707106781186548,
1.,0.707106781186548,1.),(1.,0.707106781186547,1.,0.707106781186547,1.,
0.707106781186547,1.,0.707106781186547,1.),(1.,0.707106781186547,1.,0.707106781186547,
1.,0.707106781186547,1.,0.707106781186547,1.),(1.,0.707106781186548,1.,
0.707106781186548,1.,0.707106781186548,1.,0.707106781186548,1.),(1.,0.707106781186547,
1.,0.707106781186547,1.,0.707106781186547,1.,0.707106781186547,1.),(1.,
0.707106781186547,1.,0.707106781186547,1.,0.707106781186547,1.,0.707106781186547,
1.),(1.,0.707106781186548,1.,0.707106781186548,1.,0.707106781186548,1.,
0.707106781186548,1.),(1.,0.707106781186547,1.,0.707106781186547,1.,0.707106781186547,
1.,0.707106781186547,1.),(1.,0.707106781186547,1.,0.707106781186547,1.,
0.707106781186547,1.,0.707106781186547,1.),(1.,0.707106781186548,1.,0.707106781186548,
1.,0.707106781186548,1.,0.707106781186548,1.),(1.,0.707106781186547,1.,
0.707106781186547,1.,0.707106781186547,1.,0.707106781186547,1.),(1.,0.707106781186548,
1.,0.707106781186548,1.,0.707106781186548,1.,0.707106781186548,1.),(1.,
0.707106781186547,1.,0.707106781186547,1.,0.707106781186547,1.,0.707106781186547,
1.),(1.,0.707106781186548,1.,0.707106781186548,1.,0.707106781186548,1.,
0.707106781186548,1.),(1.,0.707106781186547,1.,0.707106781186547,1.,0.707106781186547,
1.,0.707106781186547,1.),(1.,0.707106781186547,1.,0.707106781186547,1.,
0.707106781186547,1.,0.707106781186547,1.),(1.,0.707106781186547,1.,0.707106781186547,
1.,0.707106781186547,1.,0.707106781186547,1.),(1.,0.707106781186548,1.,
0.707106781186548,1.,0.707106781186548,1.,0.707106781186548,1.),(1.,0.707106781186547,
1.,0.707106781186547,1.,0.707106781186547,1.,0.707106781186547,1.),(1.,
0.707106781186547,1.,0.707106781186547,1.,0.707106781186547,1.,0.707106781186547,
1.),(1.,0.707106781186548,1.,0.707106781186548,1.,0.707106781186548,1.,
0.707106781186548,1.),(1.,0.707106781186547,1.,0.707106781186547,1.,0.707106781186547,
1.,0.707106781186547,1.),(1.,0.707106781186548,1.,0.707106781186548,1.,
0.707106781186548,1.,0.707106781186548,1.),(1.,0.707106781186547,1.,0.707106781186547,
1.,0.707106781186547,1.,0.707106781186547,1.),(1.,0.707106781186548,1.,
0.707106781186548,1.,0.707106781186548,1.,0.707106781186548,1.),(1.,0.707106781186547,
1.,0.707106781186547,1.,0.707106781186547,1.,0.707106781186547,1.),(1.,
0.707106781186547,1.,0.707106781186547,1.,0.707106781186547,1.,0.707106781186547,
1.),(1.,0.707106781186547,1.,0.707106781186547,1.,0.707106781186547,1.,
0.707106781186547,1.),(1.,0.707106781186547,1.,0.707106781186547,1.,0.707106781186547,
1.,0.707106781186547,1.),(1.,0.707106781186548,1.,0.707106781186548,1.,
0.707106781186548,1.,0.707106781186548,1.),(1.,0.707106781186547,1.,0.707106781186547,
1.,0.707106781186547,1.,0.707106781186547,1.),(1.,0.707106781186547,1.,
0.707106781186547,1.,0.707106781186547,1.,0.707106781186547,1.),(1.,0.707106781186548,
1.,0.707106781186548,1.,0.707106781186548,1.,0.707106781186548,1.),(1.,
0.707106781186548,1.,0.707106781186548,1.,0.707106781186548,1.,0.707106781186548,
1.),(1.,0.707106781186547,1.,0.707106781186547,1.,0.707106781186547,1.,
0.707106781186547,1.),(1.,0.707106781186548,1.,0.707106781186548,1.,0.707106781186548,
1.,0.707106781186548,1.),(1.,0.707106781186547,1.,0.707106781186547,1.,
0.707106781186547,1.,0.707106781186547,1.),(1.,0.707106781186548,1.,0.707106781186548,
1.,0.707106781186548,1.,0.707106781186548,1.),(1.,0.707106781186547,1.,
0.707106781186547,1.,0.707106781186547,1.,0.707106781186547,1.),(1.,0.707106781186547,
1.,0.707106781186547,1.,0.707106781186547,1.,0.707106781186547,1.),(1.,
0.707106781186548,1.,0.707106781186548,1.,0.707106781186548,1.,0.707106781186548,
1.),(1.,0.707106781186547,1.,0.707106781186547,1.,0.707106781186547,1.,
0.707106781186547,1.),(1.,0.707106781186548,1.,0.707106781186548,1.,0.707106781186548,
1.,0.707106781186548,1.),(1.,0.707106781186547,1.,0.707106781186547,1.,
0.707106781186547,1.,0.707106781186547,1.),(1.,0.707106781186548,1.,0.707106781186548,
1.,0.707106781186548,1.,0.707106781186548,1.),(1.,0.707106781186547,1.,
0.707106781186547,1.,0.707106781186547,1.,0.707106781186547,1.),(1.,0.707106781186548,
1.,0.707106781186548,1.,0.707106781186548,1.,0.707106781186548,1.),(1.,
0.707106781186548,1.,0.707106781186548,1.,0.707106781186548,1.,0.707106781186548,
1.),(1.,0.707106781186547,1.,0.707106781186547,1.,0.707106781186547,1.,
0.707106781186547,1.),(1.,0.707106781186548,1.,0.707106781186548,1.,0.707106781186548,
1.,0.707106781186548,1.),(1.,0.707106781186547,1.,0.707106781186547,1.,
0.707106781186547,1.,0.707106781186547,1.),(1.,0.707106781186547,1.,0.707106781186547,
1.,0.707106781186547,1.,0.707106781186547,1.),(1.,0.707106781186548,1.,
0.707106781186548,1.,0.707106781186548,1.,0.707106781186548,1.),(1.,0.707106781186547,
1.,0.707106781186547,1.,0.707106781186547,1.,0.707106781186547,1.),(1.,
0.707106781186547,1.,0.707106781186547,1.,0.707106781186547,1.,0.707106781186547,
1.),(1.,0.707106781186548,1.,0.707106781186548,1.,0.707106781186548,1.,
0.707106781186548,1.),(1.,0.707106781186548,1.,0.707106781186548,1.,0.707106781186548,
1.,0.707106781186548,1.),(1.,0.707106781186548,1.,0.707106781186548,1.,
0.707106781186548,1.,0.707106781186548,1.),(1.,0.707106781186547,1.,0.707106781186547,
1.,0.707106781186547,1.,0.707106781186547,1.),(1.,0.707106781186548,1.,
0.707106781186548,1.,0.707106781186548,1.,0.707106781186548,1.),(1.,0.707106781186547,
1.,0.707106781186547,1.,0.707106781186547,1.,0.707106781186547,1.),(1.,
0.707106781186547,1.,0.707106781186547,1.,0.707106781186547,1.,0.707106781186547,
1.),(1.,0.707106781186547,1.,0.707106781186547,1.,0.707106781186547,1.,
0.707106781186547,1.),(1.,0.707106781186548,1.,0.707106781186548,1.,0.707106781186548,
1.,0.707106781186548,1.),(1.,0.707106781186547,1.,0.707106781186547,1.,
0.707106781186547,1.,0.707106781186547,1.),(1.,0.707106781186548,1.,0.707106781186548,
1.,0.707106781186548,1.,0.707106781186548,1.),(1.,0.707106781186548,1.,
0.707106781186548,1.,0.707106781186548,1.,0.707106781186548,1.),(1.,0.707106781186548,
1.,0.707106781186548,1.,0.707106781186548,1.,0.707106781186548,1.),(1.,
0.707106781186547,1.,0.707106781186547,1.,0.707106781186547,1.,0.707106781186547,
1.),(1.,0.707106781186547,1.,0.707106781186547,1.,0.707106781186547,1.,
0.707106781186547,1.),(1.,0.707106781186547,1.,0.707106781186547,1.,0.707106781186547,
1.,0.707106781186547,1.),(1.,0.707106781186547,1.,0.707106781186547,1.,
0.707106781186547,1.,0.707106781186547,1.),(1.,0.707106781186548,1.,0.707106781186548,
1.,0.707106781186548,1.,0.707106781186548,1.),(1.,0.707106781186547,1.,
0.707106781186547,1.,0.707106781186547,1.,0.707106781186547,1.),(1.,0.707106781186547,
1.,0.707106781186547,1.,0.707106781186547,1.,0.707106781186547,1.),(1.,
0.707106781186548,1.,0.707106781186548,1.,0.707106781186548,1.,0.707106781186548,
1.),(1.,0.707106781186547,1.,0.707106781186547,1.,0.707106781186547,1.,
0.707106781186547,1.),(1.,0.707106781186548,1.,0.707106781186548,1.,0.707106781186548,
1.,0.707106781186548,1.),(1.,0.707106781186547,1.,0.707106781186547,1.,
0.707106781186547,1.,0.707106781186547,1.),(1.,0.707106781186547,1.,0.707106781186547,
1.,0.707106781186547,1.,0.707106781186547,1.),(1.,0.707106781186548,1.,
0.707106781186548,1.,0.707106781186548,1.,0.707106781186548,1.),(1.,0.707106781186547,
1.,0.707106781186547,1.,0.707106781186547,1.,0.707106781186547,1.),(1.,
0.707106781186548,1.,0.707106781186548,1.,0.707106781186548,1.,0.707106781186548,
1.),(1.,0.707106781186547,1.,0.707106781186547,1.,0.707106781186547,1.,
0.707106781186547,1.),(1.,0.707106781186548,1.,0.707106781186548,1.,0.707106781186548,
1.,0.707106781186548,1.),(1.,0.707106781186547,1.,0.707106781186547,1.,
0.707106781186547,1.,0.707106781186547,1.),(1.,0.707106781186547,1.,0.707106781186547,
1.,0.707106781186547,1.,0.707106781186547,1.),(1.,0.707106781186547,1.,
0.707106781186547,1.,0.707106781186547,1.,0.707106781186547,1.),(1.,0.707106781186547,
1.,0.707106781186547,1.,0.707106781186547,1.,0.707106781186547,1.),(1.,
0.707106781186547,1.,0.707106781186547,1.,0.707106781186547,1.,0.707106781186547,
1.),(1.,0.707106781186547,1.,0.707106781186547,1.,0.707106781186547,1.,
0.707106781186547,1.),(1.,0.707106781186548,1.,0.707106781186548,1.,0.707106781186548,
1.,0.707106781186548,1.),(1.,0.707106781186547,1.,0.707106781186547,1.,
0.707106781186547,1.,0.707106781186547,1.),(1.,0.707106781186547,1.,0.707106781186547,
1.,0.707106781186547,1.,0.707106781186547,1.),(1.,0.707106781186548,1.,
0.707106781186548,1.,0.707106781186548,1.,0.707106781186548,1.),(1.,0.707106781186548,
1.,0.707106781186548,1.,0.707106781186548,1.,0.707106781186548,1.),(1.,
0.707106781186547,1.,0.707106781186547,1.,0.707106781186547,1.,0.707106781186547,
1.),(1.,0.707106781186548,1.,0.707106781186548,1.,0.707106781186548,1.,
0.707106781186548,1.),(1.,0.707106781186548,1.,0.707106781186548,1.,0.707106781186548,
1.,0.707106781186548,1.),(1.,0.707106781186547,1.,0.707106781186547,1.,
0.707106781186547,1.,0.707106781186547,1.),(1.,0.707106781186547,1.,0.707106781186547,
1.,0.707106781186547,1.,0.707106781186547,1.),(1.,0.707106781186548,1.,
0.707106781186548,1.,0.707106781186548,1.,0.707106781186548,1.),(1.,0.707106781186547,
1.,0.707106781186547,1.,0.707106781186547,1.,0.707106781186547,1.),(1.,
0.707106781186547,1.,0.707106781186547,1.,0.707106781186547,1.,0.707106781186547,
1.),(1.,0.707106781186548,1.,0.707106781186548,1.,0.707106781186548,1.,
0.707106781186548,1.),(1.,0.707106781186547,1.,0.707106781186547,1.,0.707106781186547,
1.,0.707106781186547,1.),(1.,0.707106781186548,1.,0.707106781186548,1.,
0.707106781186548,1.,0.707106781186548,1.),(1.,0.707106781186548,1.,0.707106781186548,
1.,0.707106781186548,1.,0.707106781186548,1.),(1.,0.707106781186548,1.,
0.707106781186548,1.,0.707106781186548,1.,0.707106781186548,1.),(1.,0.707106781186547,
1.,0.707106781186547,1.,0.707106781186547,1.,0.707106781186547,1.),(1.,
0.707106781186547,1.,0.707106781186547,1.,0.707106781186547,1.,0.707106781186547,
1.),(1.,0.707106781186547,1.,0.707106781186547,1.,0.707106781186547,1.,
0.707106781186547,1.),(1.,0.707106781186547,1.,0.707106781186547,1.,0.707106781186547,
1.,0.707106781186547,1.),(1.,0.707106781186548,1.,0.707106781186548,1.,
0.707106781186548,1.,0.707106781186548,1.),(1.,0.707106781186548,1.,0.707106781186548,
1.,0.707106781186548,1.,0.707106781186548,1.),(1.,0.707106781186548,1.,
0.707106781186548,1.,0.707106781186548,1.,0.707106781186548,1.),(1.,0.707106781186547,
1.,0.707106781186547,1.,0.707106781186547,1.,0.707106781186547,1.),(1.,
0.707106781186548,1.,0.707106781186548,1.,0.707106781186548,1.,0.707106781186548,
1.),(1.,0.707106781186547,1.,0.707106781186547,1.,0.707106781186547,1.,
0.707106781186547,1.),(1.,0.707106781186548,1.,0.707106781186548,1.,0.707106781186548,
1.,0.707106781186548,1.),(1.,0.707106781186548,1.,0.707106781186548,1.,
0.707106781186548,1.,0.707106781186548,1.),(1.,0.707106781186547,1.,0.707106781186547,
1.,0.707106781186547,1.,0.707106781186547,1.),(1.,0.707106781186548,1.,
0.707106781186548,1.,0.707106781186548,1.,0.707106781186548,1.),(1.,0.707106781186547,
1.,0.707106781186547,1.,0.707106781186547,1.,0.707106781186547,1.),(1.,
0.707106781186548,1.,0.707106781186548,1.,0.707106781186548,1.,0.707106781186548,
1.),(1.,0.707106781186548,1.,0.707106781186548,1.,0.707106781186548,1.,
0.707106781186548,1.),(1.,0.707106781186547,1.,0.707106781186547,1.,0.707106781186547,
1.,0.707106781186547,1.),(1.,0.707106781186547,1.,0.707106781186547,1.,
0.707106781186547,1.,0.707106781186547,1.),(1.,0.707106781186548,1.,0.707106781186548,
1.,0.707106781186548,1.,0.707106781186548,1.),(1.,0.707106781186547,1.,
0.707106781186547,1.,0.707106781186547,1.,0.707106781186547,1.),(1.,0.707106781186548,
1.,0.707106781186548,1.,0.707106781186548,1.,0.707106781186548,1.),(1.,
0.707106781186547,1.,0.707106781186547,1.,0.707106781186547,1.,0.707106781186547,
1.),(1.,0.707106781186548,1.,0.707106781186548,1.,0.707106781186548,1.,
0.707106781186548,1.),(1.,0.707106781186548,1.,0.707106781186548,1.,0.707106781186548,
1.,0.707106781186548,1.),(1.,0.707106781186548,1.,0.707106781186548,1.,
0.707106781186548,1.,0.707106781186548,1.),(1.,0.707106781186547,1.,0.707106781186547,
1.,0.707106781186547,1.,0.707106781186547,1.),(1.,0.707106781186548,1.,
0.707106781186548,1.,0.707106781186548,1.,0.707106781186548,1.),(1.,0.707106781186547,
1.,0.707106781186547,1.,0.707106781186547,1.,0.707106781186547,1.),(1.,
0.707106781186547,1.,0.707106781186547,1.,0.707106781186547,1.,0.707106781186547,
1.),(1.,0.707106781186547,1.,0.707106781186547,1.,0.707106781186547,1.,
0.707106781186547,1.),(1.,0.707106781186547,1.,0.707106781186547,1.,0.707106781186547,
1.,0.707106781186547,1.),(1.,0.707106781186548,1.,0.707106781186548,1.,
0.707106781186548,1.,0.707106781186548,1.),(1.,0.707106781186548,1.,0.707106781186548,
1.,0.707106781186548,1.,0.707106781186548,1.),(1.,0.707106781186547,1.,
0.707106781186547,1.,0.707106781186547,1.,0.707106781186547,1.),(1.,0.707106781186547,
1.,0.707106781186547,1.,0.707106781186547,1.,0.707106781186547,1.),(1.,
0.707106781186547,1.,0.707106781186547,1.,0.707106781186547,1.,0.707106781186547,
1.),(1.,0.707106781186548,1.,0.707106781186548,1.,0.707106781186548,1.,
0.707106781186548,1.),(1.,0.707106781186547,1.,0.707106781186547,1.,0.707106781186547,
1.,0.707106781186547,1.),(1.,0.707106781186547,1.,0.707106781186547,1.,
0.707106781186547,1.,0.707106781186547,1.),(1.,0.707106781186548,1.,0.707106781186548,
1.,0.707106781186548,1.,0.707106781186548,1.),(1.,0.707106781186547,1.,
0.707106781186547,1.,0.707106781186547,1.,0.707106781186547,1.),(1.,0.707106781186548,
1.,0.707106781186548,1.,0.707106781186548,1.,0.707106781186548,1.),(1.,
0.707106781186548,1.,0.707106781186548,1.,0.707106781186548,1.,0.707106781186548,
1.),(1.,0.707106781186548,1.,0.707106781186548,1.,0.707106781186548,1.,
0.707106781186548,1.),(1.,0.707106781186547,1.,0.707106781186547,1.,0.707106781186547,
1.,0.707106781186547,1.),(1.,0.707106781186547,1.,0.707106781186547,1.,
0.707106781186547,1.,0.707106781186547,1.),(1.,0.707106781186547,1.,0.707106781186547,
1.,0.707106781186547,1.,0.707106781186547,1.),(1.,0.707106781186547,1.,
0.707106781186547,1.,0.707106781186547,1.,0.707106781186547,1.),(1.,0.707106781186548,
1.,0.707106781186548,1.,0.707106781186548,1.,0.707106781186548,1.),(1.,
0.707106781186548,1.,0.707106781186548,1.,0.707106781186548,1.,0.707106781186548,
1.),(1.,0.707106781186547,1.,0.707106781186547,1.,0.707106781186547,1.,
0.707106781186547,1.),(1.,0.707106781186548,1.,0.707106781186548,1.,0.707106781186548,
1.,0.707106781186548,1.),(1.,0.707106781186547,1.,0.707106781186547,1.,
0.707106781186547,1.,0.707106781186547,1.),(1.,0.707106781186548,1.,0.707106781186548,
1.,0.707106781186548,1.,0.707106781186548,1.),(1.,0.707106781186548,1.,
0.707106781186548,1.,0.707106781186548,1.,0.707106781186548,1.),(1.,0.707106781186547,
1.,0.707106781186547,1.,0.707106781186547,1.,0.707106781186547,1.),(1.,
0.707106781186548,1.,0.707106781186548,1.,0.707106781186548,1.,0.707106781186548,
1.),(1.,0.707106781186547,1.,0.707106781186547,1.,0.707106781186547,1.,
0.707106781186547,1.),(1.,0.707106781186548,1.,0.707106781186548,1.,0.707106781186548,
1.,0.707106781186548,1.),(1.,0.707106781186547,1.,0.707106781186547,1.,
0.707106781186547,1.,0.707106781186547,1.),(1.,0.707106781186547,1.,0.707106781186547,
1.,0.707106781186547,1.,0.707106781186547,1.),(1.,0.707106781186547,1.,
0.707106781186547,1.,0.707106781186547,1.,0.707106781186547,1.),(1.,0.707106781186548,
1.,0.707106781186548,1.,0.707106781186548,1.,0.707106781186548,1.),(1.,
0.707106781186547,1.,0.707106781186547,1.,0.707106781186547,1.,0.707106781186547,
1.),(1.,0.707106781186548,1.,0.707106781186548,1.,0.707106781186548,1.,
0.707106781186548,1.),(1.,0.707106781186547,1.,0.707106781186547,1.,0.707106781186547,
1.,0.707106781186547,1.),(1.,0.707106781186548,1.,0.707106781186548,1.,
0.707106781186548,1.,0.707106781186548,1.),(1.,0.707106781186547,1.,0.707106781186547,
1.,0.707106781186547,1.,0.707106781186547,1.),(1.,0.707106781186548,1.,
0.707106781186548,1.,0.707106781186548,1.,0.707106781186548,1.),(1.,0.707106781186547,
1.,0.707106781186547,1.,0.707106781186547,1.,0.707106781186547,1.),(1.,
0.707106781186548,1.,0.707106781186548,1.,0.707106781186548,1.,0.707106781186548,
1.),(1.,0.707106781186547,1.,0.707106781186547,1.,0.707106781186547,1.,
0.707106781186547,1.),(1.,0.707106781186547,1.,0.707106781186547,1.,0.707106781186547,
1.,0.707106781186547,1.),(1.,0.707106781186548,1.,0.707106781186548,1.,
0.707106781186548,1.,0.707106781186548,1.),(1.,0.707106781186547,1.,0.707106781186547,
1.,0.707106781186547,1.,0.707106781186547,1.),(1.,0.707106781186548,1.,
0.707106781186548,1.,0.707106781186548,1.,0.707106781186548,1.),(1.,0.707106781186547,
1.,0.707106781186547,1.,0.707106781186547,1.,0.707106781186547,1.),(1.,
0.707106781186547,1.,0.707106781186547,1.,0.707106781186547,1.,0.707106781186547,
1.),(1.,0.707106781186548,1.,0.707106781186548,1.,0.707106781186548,1.,
0.707106781186548,1.),(1.,0.707106781186548,1.,0.707106781186548,1.,0.707106781186548,
1.,0.707106781186548,1.),(1.,0.707106781186547,1.,0.707106781186547,1.,
0.707106781186547,1.,0.707106781186547,1.),(1.,0.707106781186548,1.,0.707106781186548,
1.,0.707106781186548,1.,0.707106781186548,1.),(1.,0.707106781186548,1.,
0.707106781186548,1.,0.707106781186548,1.,0.707106781186548,1.),(1.,0.707106781186547,
1.,0.707106781186547,1.,0.707106781186547,1.,0.707106781186547,1.),(1.,
0.707106781186548,1.,0.707106781186548,1.,0.707106781186548,1.,0.707106781186548,
1.),(1.,0.707106781186547,1.,0.707106781186547,1.,0.707106781186547,1.,
0.707106781186547,1.),(1.,0.707106781186548,1.,0.707106781186548,1.,0.707106781186548,
1.,0.707106781186548,1.),(1.,0.707106781186547,1.,0.707106781186547,1.,
0.707106781186547,1.,0.707106781186547,1.),(1.,0.707106781186547,1.,0.707106781186547,
1.,0.707106781186547,1.,0.707106781186547,1.),(1.,0.707106781186547,1.,
0.707106781186547,1.,0.707106781186547,1.,0.707106781186547,1.),(1.,0.707106781186548,
1.,0.707106781186548,1.,0.707106781186548,1.,0.707106781186548,1.),(1.,
0.707106781186547,1.,0.707106781186547,1.,0.707106781186547,1.,0.707106781186547,
1.),(1.,0.707106781186547,1.,0.707106781186547,1.,0.707106781186547,1.,
0.707106781186547,1.),(1.,0.707106781186548,1.,0.707106781186548,1.,0.707106781186548,
1.,0.707106781186548,1.),(1.,0.707106781186547,1.,0.707106781186547,1.,
0.707106781186547,1.,0.707106781186547,1.),(1.,0.707106781186548,1.,0.707106781186548,
1.,0.707106781186548,1.,0.707106781186548,1.),(1.,0.707106781186547,1.,
0.707106781186547,1.,0.707106781186547,1.,0.707106781186547,1.),(1.,0.707106781186548,
1.,0.707106781186548,1.,0.707106781186548,1.,0.707106781186548,1.),(1.,
0.707106781186548,1.,0.707106781186548,1.,0.707106781186548,1.,0.707106781186548,
1.),(1.,0.707106781186547,1.,0.707106781186547,1.,0.707106781186547,1.,
0.707106781186547,1.),(1.,0.707106781186548,1.,0.707106781186548,1.,0.707106781186548,
1.,0.707106781186548,1.),(1.,0.707106781186547,1.,0.707106781186547,1.,
0.707106781186547,1.,0.707106781186547,1.),(1.,0.707106781186548,1.,0.707106781186548,
1.,0.707106781186548,1.,0.707106781186548,1.),(1.,0.707106781186548,1.,
0.707106781186548,1.,0.707106781186548,1.,0.707106781186548,1.),(1.,0.707106781186548,
1.,0.707106781186548,1.,0.707106781186548,1.,0.707106781186548,1.),(1.,
0.707106781186548,1.,0.707106781186548,1.,0.707106781186548,1.,0.707106781186548,
1.),(1.,0.707106781186547,1.,0.707106781186547,1.,0.707106781186547,1.,
0.707106781186547,1.),(1.,0.707106781186547,1.,0.707106781186547,1.,0.707106781186547,
1.,0.707106781186547,1.),(1.,0.707106781186548,1.,0.707106781186548,1.,
0.707106781186548,1.,0.707106781186548,1.),(1.,0.707106781186547,1.,0.707106781186547,
1.,0.707106781186547,1.,0.707106781186547,1.),(1.,0.707106781186547,1.,
0.707106781186547,1.,0.707106781186547,1.,0.707106781186547,1.),(1.,0.707106781186548,
1.,0.707106781186548,1.,0.707106781186548,1.,0.707106781186548,1.),(1.,
0.707106781186548,1.,0.707106781186548,1.,0.707106781186548,1.,0.707106781186548,
1.),(1.,0.707106781186547,1.,0.707106781186547,1.,0.707106781186547,1.,
0.707106781186547,1.),(1.,0.707106781186547,1.,0.707106781186547,1.,0.707106781186547,
1.,0.707106781186547,1.),(1.,0.707106781186548,1.,0.707106781186548,1.,
0.707106781186548,1.,0.707106781186548,1.),(1.,0.707106781186547,1.,0.707106781186547,
1.,0.707106781186547,1.,0.707106781186547,1.),(1.,0.707106781186547,1.,
0.707106781186547,1.,0.707106781186547,1.,0.707106781186547,1.),(1.,0.707106781186548,
1.,0.707106781186548,1.,0.707106781186548,1.,0.707106781186548,1.),(1.,
0.707106781186547,1.,0.707106781186547,1.,0.707106781186547,1.,0.707106781186547,
1.),(1.,0.707106781186548,1.,0.707106781186548,1.,0.707106781186548,1.,
0.707106781186548,1.),(1.,0.707106781186547,1.,0.707106781186547,1.,0.707106781186547,
1.,0.707106781186547,1.),(1.,0.707106781186548,1.,0.707106781186548,1.,
0.707106781186548,1.,0.707106781186548,1.),(1.,0.707106781186547,1.,0.707106781186547,
1.,0.707106781186547,1.,0.707106781186547,1.),(1.,0.707106781186547,1.,
0.707106781186547,1.,0.707106781186547,1.,0.707106781186547,1.),(1.,0.707106781186547,
1.,0.707106781186547,1.,0.707106781186547,1.,0.707106781186547,1.),(1.,
0.707106781186548,1.,0.707106781186548,1.,0.707106781186548,1.,0.707106781186548,
1.),(1.,0.707106781186547,1.,0.707106781186547,1.,0.707106781186547,1.,
0.707106781186547,1.),(1.,0.707106781186547,1.,0.707106781186547,1.,0.707106781186547,
1.,0.707106781186547,1.),(1.,0.707106781186548,1.,0.707106781186548,1.,
0.707106781186548,1.,0.707106781186548,1.),(1.,0.707106781186547,1.,0.707106781186547,
1.,0.707106781186547,1.,0.707106781186547,1.),(1.,0.707106781186548,1.,
0.707106781186548,1.,0.707106781186548,1.,0.707106781186548,1.),(1.,0.707106781186548,
1.,0.707106781186548,1.,0.707106781186548,1.,0.707106781186548,1.),(1.,
0.707106781186548,1.,0.707106781186548,1.,0.707106781186548,1.,0.707106781186548,
1.),(1.,0.707106781186547,1.,0.707106781186547,1.,0.707106781186547,1.,
0.707106781186547,1.),(1.,0.707106781186547,1.,0.707106781186547,1.,0.707106781186547,
1.,0.707106781186547,1.),(1.,0.707106781186547,1.,0.707106781186547,1.,
0.707106781186547,1.,0.707106781186547,1.),(1.,0.707106781186548,1.,0.707106781186548,
1.,0.707106781186548,1.,0.707106781186548,1.),(1.,0.707106781186548,1.,
0.707106781186548,1.,0.707106781186548,1.,0.707106781186548,1.),(1.,0.707106781186547,
1.,0.707106781186547,1.,0.707106781186547,1.,0.707106781186547,1.),(1.,
0.707106781186547,1.,0.707106781186547,1.,0.707106781186547,1.,0.707106781186547,
1.),(1.,0.707106781186547,1.,0.707106781186547,1.,0.707106781186547,1.,
0.707106781186547,1.),(1.,0.707106781186547,1.,0.707106781186547,1.,0.707106781186547,
1.,0.707106781186547,1.),(1.,0.707106781186548,1.,0.707106781186548,1.,
0.707106781186548,1.,0.707106781186548,1.),(1.,0.707106781186548,1.,0.707106781186548,
1.,0.707106781186548,1.,0.707106781186548,1.),(1.,0.707106781186547,1.,
0.707106781186547,1.,0.707106781186547,1.,0.707106781186547,1.),(1.,0.707106781186547,
1.,0.707106781186547,1.,0.707106781186547,1.,0.707106781186547,1.),(1.,
0.707106781186547,1.,0.707106781186547,1.,0.707106781186547,1.,0.707106781186547,
1.),(1.,0.707106781186548,1.,0.707106781186548,1.,0.707106781186548,1.,
0.707106781186548,1.),(1.,0.707106781186548,1.,0.707106781186548,1.,0.707106781186548,
1.,0.707106781186548,1.),(1.,0.707106781186547,1.,0.707106781186547,1.,
0.707106781186547,1.,0.707106781186547,1.),(1.,0.707106781186548,1.,0.707106781186548,
1.,0.707106781186548,1.,0.707106781186548,1.),(1.,0.707106781186547,1.,
0.707106781186547,1.,0.707106781186547,1.,0.707106781186547,1.),(1.,0.707106781186548,
1.,0.707106781186548,1.,0.707106781186548,1.,0.707106781186548,1.),(1.,
0.707106781186547,1.,0.707106781186547,1.,0.707106781186547,1.,0.707106781186547,
1.),(1.,0.707106781186548,1.,0.707106781186548,1.,0.707106781186548,1.,
0.707106781186548,1.),(1.,0.707106781186548,1.,0.707106781186548,1.,0.707106781186548,
1.,0.707106781186548,1.),(1.,0.707106781186547,1.,0.707106781186547,1.,
0.707106781186547,1.,0.707106781186547,1.),(1.,0.707106781186548,1.,0.707106781186548,
1.,0.707106781186548,1.,0.707106781186548,1.),(1.,0.707106781186548,1.,
0.707106781186548,1.,0.707106781186548,1.,0.707106781186548,1.),(1.,0.707106781186548,
1.,0.707106781186548,1.,0.707106781186548,1.,0.707106781186548,1.),(1.,
0.707106781186547,1.,0.707106781186547,1.,0.707106781186547,1.,0.707106781186547,
1.),(1.,0.707106781186547,1.,0.707106781186547,1.,0.707106781186547,1.,
0.707106781186547,1.),(1.,0.707106781186547,1.,0.707106781186547,1.,0.707106781186547,
1.,0.707106781186547,1.),(1.,0.707106781186548,1.,0.707106781186548,1.,
0.707106781186548,1.,0.707106781186548,1.),(1.,0.707106781186548,1.,0.707106781186548,
1.,0.707106781186548,1.,0.707106781186548,1.),(1.,0.707106781186548,1.,
0.707106781186548,1.,0.707106781186548,1.,0.707106781186548,1.),(1.,0.707106781186547,
1.,0.707106781186547,1.,0.707106781186547,1.,0.707106781186547,1.),(1.,
0.707106781186547,1.,0.707106781186547,1.,0.707106781186547,1.,0.707106781186547,
1.),(1.,0.707106781186548,1.,0.707106781186548,1.,0.707106781186548,1.,
0.707106781186548,1.),(1.,0.707106781186548,1.,0.707106781186548,1.,0.707106781186548,
1.,0.707106781186548,1.),(1.,0.707106781186547,1.,0.707106781186547,1.,
0.707106781186547,1.,0.707106781186547,1.),(1.,0.707106781186548,1.,0.707106781186548,
1.,0.707106781186548,1.,0.707106781186548,1.),(1.,0.707106781186547,1.,
0.707106781186547,1.,0.707106781186547,1.,0.707106781186547,1.),(1.,0.707106781186547,
1.,0.707106781186547,1.,0.707106781186547,1.,0.707106781186547,1.),(1.,
0.707106781186548,1.,0.707106781186548,1.,0.707106781186548,1.,0.707106781186548,
1.),(1.,0.707106781186547,1.,0.707106781186547,1.,0.707106781186547,1.,
0.707106781186547,1.),(1.,0.707106781186548,1.,0.707106781186548,1.,0.707106781186548,
1.,0.707106781186548,1.),(1.,0.707106781186547,1.,0.707106781186547,1.,
0.707106781186547,1.,0.707106781186547,1.),(1.,0.707106781186547,1.,0.707106781186547,
1.,0.707106781186547,1.,0.707106781186547,1.),(1.,0.707106781186548,1.,
0.707106781186548,1.,0.707106781186548,1.,0.707106781186548,1.),(1.,0.707106781186547,
1.,0.707106781186547,1.,0.707106781186547,1.,0.707106781186547,1.),(1.,
0.707106781186548,1.,0.707106781186548,1.,0.707106781186548,1.,0.707106781186548,
1.),(1.,0.707106781186548,1.,0.707106781186548,1.,0.707106781186548,1.,
0.707106781186548,1.),(1.,0.707106781186547,1.,0.707106781186547,1.,0.707106781186547,
1.,0.707106781186547,1.),(1.,0.707106781186547,1.,0.707106781186547,1.,
0.707106781186547,1.,0.707106781186547,1.),(1.,0.707106781186548,1.,0.707106781186548,
1.,0.707106781186548,1.,0.707106781186548,1.),(1.,0.707106781186547,1.,
0.707106781186547,1.,0.707106781186547,1.,0.707106781186547,1.),(1.,0.707106781186548,
1.,0.707106781186548,1.,0.707106781186548,1.,0.707106781186548,1.),(1.,
0.707106781186547,1.,0.707106781186547,1.,0.707106781186547,1.,0.707106781186547,
1.),(1.,0.707106781186547,1.,0.707106781186547,1.,0.707106781186547,1.,
0.707106781186547,1.),(1.,0.707106781186548,1.,0.707106781186548,1.,0.707106781186548,
1.,0.707106781186548,1.),(1.,0.707106781186547,1.,0.707106781186547,1.,
0.707106781186547,1.,0.707106781186547,1.),(1.,0.707106781186548,1.,0.707106781186548,
1.,0.707106781186548,1.,0.707106781186548,1.),(1.,0.707106781186547,1.,
0.707106781186547,1.,0.707106781186547,1.,0.707106781186547,1.),(1.,0.707106781186548,
1.,0.707106781186548,1.,0.707106781186548,1.,0.707106781186548,1.),(1.,
0.707106781186547,1.,0.707106781186547,1.,0.707106781186547,1.,0.707106781186547,
1.),(1.,0.707106781186547,1.,0.707106781186547,1.,0.707106781186547,1.,
0.707106781186547,1.),(1.,0.707106781186548,1.,0.707106781186548,1.,0.707106781186548,
1.,0.707106781186548,1.),(1.,0.707106781186547,1.,0.707106781186547,1.,
0.707106781186547,1.,0.707106781186547,1.),(1.,0.707106781186547,1.,0.707106781186547,
1.,0.707106781186547,1.,0.707106781186547,1.),(1.,0.707106781186547,1.,
0.707106781186547,1.,0.707106781186547,1.,0.707106781186547,1.),(1.,0.707106781186547,
1.,0.707106781186547,1.,0.707106781186547,1.,0.707106781186547,1.),(1.,
0.707106781186547,1.,0.707106781186547,1.,0.707106781186547,1.,0.707106781186547,
1.),(1.,0.707106781186547,1.,0.707106781186547,1.,0.707106781186547,1.,
0.707106781186547,1.),(1.,0.707106781186548,1.,0.707106781186548,1.,0.707106781186548,
1.,0.707106781186548,1.),(1.,0.707106781186547,1.,0.707106781186547,1.,
0.707106781186547,1.,0.707106781186547,1.),(1.,0.707106781186548,1.,0.707106781186548,
1.,0.707106781186548,1.,0.707106781186548,1.),(1.,0.707106781186548,1.,
0.707106781186548,1.,0.707106781186548,1.,0.707106781186548,1.),(1.,0.707106781186548,
1.,0.707106781186548,1.,0.707106781186548,1.,0.707106781186548,1.),(1.,
0.707106781186547,1.,0.707106781186547,1.,0.707106781186547,1.,0.707106781186547,
1.),(1.,0.707106781186547,1.,0.707106781186547,1.,0.707106781186547,1.,
0.707106781186547,1.),(1.,0.707106781186547,1.,0.707106781186547,1.,0.707106781186547,
1.,0.707106781186547,1.),(1.,0.707106781186548,1.,0.707106781186548,1.,
0.707106781186548,1.,0.707106781186548,1.),(1.,0.707106781186547,1.,0.707106781186547,
1.,0.707106781186547,1.,0.707106781186547,1.),(1.,0.707106781186548,1.,
0.707106781186548,1.,0.707106781186548,1.,0.707106781186548,1.),(1.,0.707106781186547,
1.,0.707106781186547,1.,0.707106781186547,1.,0.707106781186547,1.),(1.,
0.707106781186547,1.,0.707106781186547,1.,0.707106781186547,1.,0.707106781186547,
1.),(1.,0.707106781186548,1.,0.707106781186548,1.,0.707106781186548,1.,
0.707106781186548,1.),(1.,0.707106781186547,1.,0.707106781186547,1.,0.707106781186547,
1.,0.707106781186547,1.),(1.,0.707106781186547,1.,0.707106781186547,1.,
0.707106781186547,1.,0.707106781186547,1.),(1.,0.707106781186547,1.,0.707106781186547,
1.,0.707106781186547,1.,0.707106781186547,1.),(1.,0.707106781186547,1.,
0.707106781186547,1.,0.707106781186547,1.,0.707106781186547,1.),(1.,0.707106781186547,
1.,0.707106781186547,1.,0.707106781186547,1.,0.707106781186547,1.),(1.,
0.707106781186548,1.,0.707106781186548,1.,0.707106781186548,1.,0.707106781186548,
1.),(1.,0.707106781186547,1.,0.707106781186547,1.,0.707106781186547,1.,
0.707106781186547,1.),(1.,0.707106781186548,1.,0.707106781186548,1.,0.707106781186548,
1.,0.707106781186548,1.),(1.,0.707106781186547,1.,0.707106781186547,1.,
0.707106781186547,1.,0.707106781186547,1.),(1.,0.707106781186547,1.,0.707106781186547,
1.,0.707106781186547,1.,0.707106781186547,1.),(1.,0.707106781186548,1.,
0.707106781186548,1.,0.707106781186548,1.,0.707106781186548,1.),(1.,0.707106781186548,
1.,0.707106781186548,1.,0.707106781186548,1.,0.707106781186548,1.),(1.,
0.707106781186547,1.,0.707106781186547,1.,0.707106781186547,1.,0.707106781186547,
1.),(1.,0.707106781186547,1.,0.707106781186547,1.,0.707106781186547,1.,
0.707106781186547,1.),(1.,0.707106781186547,1.,0.707106781186547,1.,0.707106781186547,
1.,0.707106781186547,1.),(1.,0.707106781186548,1.,0.707106781186548,1.,
0.707106781186548,1.,0.707106781186548,1.),(1.,0.707106781186547,1.,0.707106781186547,
1.,0.707106781186547,1.,0.707106781186547,1.),(1.,0.707106781186547,1.,
0.707106781186547,1.,0.707106781186547,1.,0.707106781186547,1.),(1.,0.707106781186548,
1.,0.707106781186548,1.,0.707106781186548,1.,0.707106781186548,1.),(1.,
0.707106781186548,1.,0.707106781186548,1.,0.707106781186548,1.,0.707106781186548,
1.),(1.,0.707106781186547,1.,0.707106781186547,1.,0.707106781186547,1.,
0.707106781186547,1.),(1.,0.707106781186548,1.,0.707106781186548,1.,0.707106781186548,
1.,0.707106781186548,1.),(1.,0.707106781186547,1.,0.707106781186547,1.,
0.707106781186547,1.,0.707106781186547,1.),(1.,0.707106781186548,1.,0.707106781186548,
1.,0.707106781186548,1.,0.707106781186548,1.),(1.,0.707106781186548,1.,
0.707106781186548,1.,0.707106781186548,1.,0.707106781186548,1.),(1.,0.707106781186547,
1.,0.707106781186547,1.,0.707106781186547,1.,0.707106781186547,1.),(1.,
0.707106781186547,1.,0.707106781186547,1.,0.707106781186547,1.,0.707106781186547,
1.),(1.,0.707106781186547,1.,0.707106781186547,1.,0.707106781186547,1.,
0.707106781186547,1.),(1.,0.707106781186548,1.,0.707106781186548,1.,0.707106781186548,
1.,0.707106781186548,1.),(1.,0.707106781186548,1.,0.707106781186548,1.,
0.707106781186548,1.,0.707106781186548,1.),(1.,0.707106781186547,1.,0.707106781186547,
1.,0.707106781186547,1.,0.707106781186547,1.),(1.,0.707106781186548,1.,
0.707106781186548,1.,0.707106781186548,1.,0.707106781186548,1.),(1.,0.707106781186547,
1.,0.707106781186547,1.,0.707106781186547,1.,0.707106781186547,1.),(1.,
0.707106781186548,1.,0.707106781186548,1.,0.707106781186548,1.,0.707106781186548,
1.),(1.,0.707106781186548,1.,0.707106781186548,1.,0.707106781186548,1.,
0.707106781186548,1.),(1.,0.707106781186547,1.,0.707106781186547,1.,0.707106781186547,
1.,0.707106781186547,1.),(1.,0.707106781186548,1.,0.707106781186548,1.,
0.707106781186548,1.,0.707106781186548,1.),(1.,0.707106781186547,1.,0.707106781186547,
1.,0.707106781186547,1.,0.707106781186547,1.),(1.,0.707106781186547,1.,
0.707106781186547,1.,0.707106781186547,1.,0.707106781186547,1.),(1.,0.707106781186547,
1.,0.707106781186547,1.,0.707106781186547,1.,0.707106781186547,1.),(1.,
0.707106781186548,1.,0.707106781186548,1.,0.707106781186548,1.,0.707106781186548,
1.),(1.,0.707106781186547,1.,0.707106781186547,1.,0.707106781186547,1.,
0.707106781186547,1.),(1.,0.707106781186548,1.,0.707106781186548,1.,0.707106781186548,
1.,0.707106781186548,1.),(1.,0.707106781186547,1.,0.707106781186547,1.,
0.707106781186547,1.,0.707106781186547,1.),(1.,0.707106781186548,1.,0.707106781186548,
1.,0.707106781186548,1.,0.707106781186548,1.),(1.,0.707106781186547,1.,
0.707106781186547,1.,0.707106781186547,1.,0.707106781186547,1.),(1.,0.707106781186547,
1.,0.707106781186547,1.,0.707106781186547,1.,0.707106781186547,1.),(1.,
0.707106781186547,1.,0.707106781186547,1.,0.707106781186547,1.,0.707106781186547,
1.),(1.,0.707106781186547,1.,0.707106781186547,1.,0.707106781186547,1.,
0.707106781186547,1.),(1.,0.707106781186547,1.,0.707106781186547,1.,0.707106781186547,
1.,0.707106781186547,1.),(1.,0.707106781186548,1.,0.707106781186548,1.,
0.707106781186548,1.,0.707106781186548,1.),(1.,0.707106781186547,1.,0.707106781186547,
1.,0.707106781186547,1.,0.707106781186547,1.),(1.,0.707106781186548,1.,
0.707106781186548,1.,0.707106781186548,1.,0.707106781186548,1.),(1.,0.707106781186547,
1.,0.707106781186547,1.,0.707106781186547,1.,0.707106781186547,1.),(1.,
0.707106781186548,1.,0.707106781186548,1.,0.707106781186548,1.,0.707106781186548,
1.),(1.,0.707106781186547,1.,0.707106781186547,1.,0.707106781186547,1.,
0.707106781186547,1.),(1.,0.707106781186548,1.,0.707106781186548,1.,0.707106781186548,
1.,0.707106781186548,1.),(1.,0.707106781186547,1.,0.707106781186547,1.,
0.707106781186547,1.,0.707106781186547,1.),(1.,0.707106781186547,1.,0.707106781186547,
1.,0.707106781186547,1.,0.707106781186547,1.),(1.,0.707106781186547,1.,
0.707106781186547,1.,0.707106781186547,1.,0.707106781186547,1.),(1.,0.707106781186547,
1.,0.707106781186547,1.,0.707106781186547,1.,0.707106781186547,1.),(1.,
0.707106781186547,1.,0.707106781186547,1.,0.707106781186547,1.,0.707106781186547,
1.),(1.,0.707106781186548,1.,0.707106781186548,1.,0.707106781186548,1.,
0.707106781186548,1.),(1.,0.707106781186548,1.,0.707106781186548,1.,0.707106781186548,
1.,0.707106781186548,1.),(1.,0.707106781186548,1.,0.707106781186548,1.,
0.707106781186548,1.,0.707106781186548,1.),(1.,0.707106781186547,1.,0.707106781186547,
1.,0.707106781186547,1.,0.707106781186547,1.),(1.,0.707106781186548,1.,
0.707106781186548,1.,0.707106781186548,1.,0.707106781186548,1.),(1.,0.707106781186547,
1.,0.707106781186547,1.,0.707106781186547,1.,0.707106781186547,1.),(1.,
0.707106781186548,1.,0.707106781186548,1.,0.707106781186548,1.,0.707106781186548,
1.),(1.,0.707106781186547,1.,0.707106781186547,1.,0.707106781186547,1.,
0.707106781186547,1.),(1.,0.707106781186547,1.,0.707106781186547,1.,0.707106781186547,
1.,0.707106781186547,1.),(1.,0.707106781186548,1.,0.707106781186548,1.,
0.707106781186548,1.,0.707106781186548,1.),(1.,0.707106781186547,1.,0.707106781186547,
1.,0.707106781186547,1.,0.707106781186547,1.),(1.,0.707106781186548,1.,
0.707106781186548,1.,0.707106781186548,1.,0.707106781186548,1.),(1.,0.707106781186547,
1.,0.707106781186547,1.,0.707106781186547,1.,0.707106781186547,1.),(1.,
0.707106781186547,1.,0.707106781186547,1.,0.707106781186547,1.,0.707106781186547,
1.),(1.,0.707106781186547,1.,0.707106781186547,1.,0.707106781186547,1.,
0.707106781186547,1.),(1.,0.707106781186548,1.,0.707106781186548,1.,0.707106781186548,
1.,0.707106781186548,1.),(1.,0.707106781186548,1.,0.707106781186548,1.,
0.707106781186548,1.,0.707106781186548,1.),(1.,0.707106781186547,1.,0.707106781186547,
1.,0.707106781186547,1.,0.707106781186547,1.),(1.,0.707106781186548,1.,
0.707106781186548,1.,0.707106781186548,1.,0.707106781186548,1.),(1.,0.707106781186547,
1.,0.707106781186547,1.,0.707106781186547,1.,0.707106781186547,1.),(1.,
0.707106781186548,1.,0.707106781186548,1.,0.707106781186548,1.,0.707106781186548,
1.),(1.,0.707106781186548,1.,0.707106781186548,1.,0.707106781186548,1.,
0.707106781186548,1.),(1.,0.707106781186547,1.,0.707106781186547,1.,0.707106781186547,
1.,0.707106781186547,1.),(1.,0.707106781186548,1.,0.707106781186548,1.,
0.707106781186548,1.,0.707106781186548,1.),(1.,0.707106781186547,1.,0.707106781186547,
1.,0.707106781186547,1.,0.707106781186547,1.),(1.,0.707106781186548,1.,
0.707106781186548,1.,0.707106781186548,1.,0.707106781186548,1.),(1.,0.707106781186548,
1.,0.707106781186548,1.,0.707106781186548,1.,0.707106781186548,1.),(1.,
0.707106781186547,1.,0.707106781186547,1.,0.707106781186547,1.,0.707106781186547,
1.),(1.,0.707106781186547,1.,0.707106781186547,1.,0.707106781186547,1.,
0.707106781186547,1.),(1.,0.707106781186547,1.,0.707106781186547,1.,0.707106781186547,
1.,0.707106781186547,1.),(1.,0.707106781186547,1.,0.707106781186547,1.,
0.707106781186547,1.,0.707106781186547,1.),(1.,0.707106781186547,1.,0.707106781186547,
1.,0.707106781186547,1.,0.707106781186547,1.),(1.,0.707106781186547,1.,
0.707106781186547,1.,0.707106781186547,1.,0.707106781186547,1.),(1.,0.707106781186548,
1.,0.707106781186548,1.,0.707106781186548,1.,0.707106781186548,1.),(1.,
0.707106781186548,1.,0.707106781186548,1.,0.707106781186548,1.,0.707106781186548,
1.),(1.,0.707106781186547,1.,0.707106781186547,1.,0.707106781186547,1.,
0.707106781186547,1.),(1.,0.707106781186548,1.,0.707106781186548,1.,0.707106781186548,
1.,0.707106781186548,1.),(1.,0.707106781186547,1.,0.707106781186547,1.,
0.707106781186547,1.,0.707106781186547,1.),(1.,0.707106781186547,1.,0.707106781186547,
1.,0.707106781186547,1.,0.707106781186547,1.),(1.,0.707106781186548,1.,
0.707106781186548,1.,0.707106781186548,1.,0.707106781186548,1.),(1.,0.707106781186547,
1.,0.707106781186547,1.,0.707106781186547,1.,0.707106781186547,1.),(1.,
0.707106781186547,1.,0.707106781186547,1.,0.707106781186547,1.,0.707106781186547,
1.),(1.,0.707106781186548,1.,0.707106781186548,1.,0.707106781186548,1.,
0.707106781186548,1.),(1.,0.707106781186547,1.,0.707106781186547,1.,0.707106781186547,
1.,0.707106781186547,1.),(1.,0.707106781186547,1.,0.707106781186547,1.,
0.707106781186547,1.,0.707106781186547,1.),(1.,0.707106781186547,1.,0.707106781186547,
1.,0.707106781186547,1.,0.707106781186547,1.),(1.,0.707106781186548,1.,
0.707106781186548,1.,0.707106781186548,1.,0.707106781186548,1.),(1.,0.707106781186547,
1.,0.707106781186547,1.,0.707106781186547,1.,0.707106781186547,1.),(1.,
0.707106781186547,1.,0.707106781186547,1.,0.707106781186547,1.,0.707106781186547,
1.),(1.,0.707106781186548,1.,0.707106781186548,1.,0.707106781186548,1.,
0.707106781186548,1.),(1.,0.707106781186547,1.,0.707106781186547,1.,0.707106781186547,
1.,0.707106781186547,1.),(1.,0.707106781186548,1.,0.707106781186548,1.,
0.707106781186548,1.,0.707106781186548,1.),(1.,0.707106781186548,1.,0.707106781186548,
1.,0.707106781186548,1.,0.707106781186548,1.),(1.,0.707106781186547,1.,
0.707106781186547,1.,0.707106781186547,1.,0.707106781186547,1.),(1.,0.707106781186547,
1.,0.707106781186547,1.,0.707106781186547,1.,0.707106781186547,1.),(1.,
0.707106781186547,1.,0.707106781186547,1.,0.707106781186547,1.,0.707106781186547,
1.),(1.,0.707106781186548,1.,0.707106781186548,1.,0.707106781186548,1.,
0.707106781186548,1.),(1.,0.707106781186547,1.,0.707106781186547,1.,0.707106781186547,
1.,0.707106781186547,1.),(1.,0.707106781186547,1.,0.707106781186547,1.,
0.707106781186547,1.,0.707106781186547,1.),(1.,0.707106781186548,1.,0.707106781186548,
1.,0.707106781186548,1.,0.707106781186548,1.),(1.,0.707106781186548,1.,
0.707106781186548,1.,0.707106781186548,1.,0.707106781186548,1.),(1.,0.707106781186548,
1.,0.707106781186548,1.,0.707106781186548,1.,0.707106781186548,1.),(1.,
0.707106781186548,1.,0.707106781186548,1.,0.707106781186548,1.,0.707106781186548,
1.),(1.,0.707106781186547,1.,0.707106781186547,1.,0.707106781186547,1.,
0.707106781186547,1.),(1.,0.707106781186548,1.,0.707106781186548,1.,0.707106781186548,
1.,0.707106781186548,1.),(1.,0.707106781186548,1.,0.707106781186548,1.,
0.707106781186548,1.,0.707106781186548,1.),(1.,0.707106781186547,1.,0.707106781186547,
1.,0.707106781186547,1.,0.707106781186547,1.),(1.,0.707106781186547,1.,
0.707106781186547,1.,0.707106781186547,1.,0.707106781186547,1.),(1.,0.707106781186548,
1.,0.707106781186548,1.,0.707106781186548,1.,0.707106781186548,1.),(1.,
0.707106781186547,1.,0.707106781186547,1.,0.707106781186547,1.,0.707106781186547,
1.),(1.,0.707106781186548,1.,0.707106781186548,1.,0.707106781186548,1.,
0.707106781186548,1.),(1.,0.707106781186547,1.,0.707106781186547,1.,0.707106781186547,
1.,0.707106781186547,1.),(1.,0.707106781186547,1.,0.707106781186547,1.,
0.707106781186547,1.,0.707106781186547,1.),(1.,0.707106781186548,1.,0.707106781186548,
1.,0.707106781186548,1.,0.707106781186548,1.),(1.,0.707106781186547,1.,
0.707106781186547,1.,0.707106781186547,1.,0.707106781186547,1.),(1.,0.707106781186547,
1.,0.707106781186547,1.,0.707106781186547,1.,0.707106781186547,1.),(1.,
0.707106781186548,1.,0.707106781186548,1.,0.707106781186548,1.,0.707106781186548,
1.),(1.,0.707106781186547,1.,0.707106781186547,1.,0.707106781186547,1.,
0.707106781186547,1.),(1.,0.707106781186548,1.,0.707106781186548,1.,0.707106781186548,
1.,0.707106781186548,1.),(1.,0.707106781186547,1.,0.707106781186547,1.,
0.707106781186547,1.,0.707106781186547,1.),(1.,0.707106781186548,1.,0.707106781186548,
1.,0.707106781186548,1.,0.707106781186548,1.),(1.,0.707106781186547,1.,
0.707106781186547,1.,0.707106781186547,1.,0.707106781186547,1.),(1.,0.707106781186548,
1.,0.707106781186548,1.,0.707106781186548,1.,0.707106781186548,1.),(1.,
0.707106781186547,1.,0.707106781186547,1.,0.707106781186547,1.,0.707106781186547,
1.),(1.,0.707106781186548,1.,0.707106781186548,1.,0.707106781186548,1.,
0.707106781186548,1.),(1.,0.707106781186547,1.,0.707106781186547,1.,0.707106781186547,
1.,0.707106781186547,1.),(1.,0.707106781186548,1.,0.707106781186548,1.,
0.707106781186548,1.,0.707106781186548,1.),(1.,0.707106781186548,1.,0.707106781186548,
1.,0.707106781186548,1.,0.707106781186548,1.),(1.,0.707106781186547,1.,
0.707106781186547,1.,0.707106781186547,1.,0.707106781186547,1.),(1.,0.707106781186547,
1.,0.707106781186547,1.,0.707106781186547,1.,0.707106781186547,1.),(1.,
0.707106781186548,1.,0.707106781186548,1.,0.707106781186548,1.,0.707106781186548,
1.),(1.,0.707106781186548,1.,0.707106781186548,1.,0.707106781186548,1.,
0.707106781186548,1.),(1.,0.707106781186547,1.,0.707106781186547,1.,0.707106781186547,
1.,0.707106781186547,1.),(1.,0.707106781186547,1.,0.707106781186547,1.,
0.707106781186547,1.,0.707106781186547,1.),(1.,0.707106781186547,1.,0.707106781186547,
1.,0.707106781186547,1.,0.707106781186547,1.),(1.,0.707106781186547,1.,
0.707106781186547,1.,0.707106781186547,1.,0.707106781186547,1.),(1.,0.707106781186547,
1.,0.707106781186547,1.,0.707106781186547,1.,0.707106781186547,1.),(1.,
0.707106781186548,1.,0.707106781186548,1.,0.707106781186548,1.,0.707106781186548,
1.),(1.,0.707106781186547,1.,0.707106781186547,1.,0.707106781186547,1.,
0.707106781186547,1.),(1.,0.707106781186547,1.,0.707106781186547,1.,0.707106781186547,
1.,0.707106781186547,1.),(1.,0.707106781186548,1.,0.707106781186548,1.,
0.707106781186548,1.,0.707106781186548,1.),(1.,0.707106781186547,1.,0.707106781186547,
1.,0.707106781186547,1.,0.707106781186547,1.),(1.,0.707106781186548,1.,
0.707106781186548,1.,0.707106781186548,1.,0.707106781186548,1.),(1.,0.707106781186548,
1.,0.707106781186548,1.,0.707106781186548,1.,0.707106781186548,1.),(1.,
0.707106781186547,1.,0.707106781186547,1.,0.707106781186547,1.,0.707106781186547,
1.),(1.,0.707106781186548,1.,0.707106781186548,1.,0.707106781186548,1.,
0.707106781186548,1.),(1.,0.707106781186547,1.,0.707106781186547,1.,0.707106781186547,
1.,0.707106781186547,1.),(1.,0.707106781186548,1.,0.707106781186548,1.,
0.707106781186548,1.,0.707106781186548,1.),(1.,0.707106781186547,1.,0.707106781186547,
1.,0.707106781186547,1.,0.707106781186547,1.),(1.,0.707106781186548,1.,
0.707106781186548,1.,0.707106781186548,1.,0.707106781186548,1.),(1.,0.707106781186547,
1.,0.707106781186547,1.,0.707106781186547,1.,0.707106781186547,1.),(1.,
0.707106781186547,1.,0.707106781186547,1.,0.707106781186547,1.,0.707106781186547,
1.),(1.,0.707106781186547,1.,0.707106781186547,1.,0.707106781186547,1.,
0.707106781186547,1.),(1.,0.707106781186547,1.,0.707106781186547,1.,0.707106781186547,
1.,0.707106781186547,1.),(1.,0.707106781186547,1.,0.707106781186547,1.,
0.707106781186547,1.,0.707106781186547,1.),(1.,0.707106781186547,1.,0.707106781186547,
1.,0.707106781186547,1.,0.707106781186547,1.),(1.,0.707106781186548,1.,
0.707106781186548,1.,0.707106781186548,1.,0.707106781186548,1.),(1.,0.707106781186547,
1.,0.707106781186547,1.,0.707106781186547,1.,0.707106781186547,1.),(1.,
0.707106781186548,1.,0.707106781186548,1.,0.707106781186548,1.,0.707106781186548,
1.),(1.,0.707106781186547,1.,0.707106781186547,1.,0.707106781186547,1.,
0.707106781186547,1.),(1.,0.707106781186547,1.,0.707106781186547,1.,0.707106781186547,
1.,0.707106781186547,1.),(1.,0.707106781186547,1.,0.707106781186547,1.,
0.707106781186547,1.,0.707106781186547,1.),(1.,0.707106781186548,1.,0.707106781186548,
1.,0.707106781186548,1.,0.707106781186548,1.),(1.,0.707106781186547,1.,
0.707106781186547,1.,0.707106781186547,1.,0.707106781186547,1.),(1.,0.707106781186548,
1.,0.707106781186548,1.,0.707106781186548,1.,0.707106781186548,1.),(1.,
0.707106781186548,1.,0.707106781186548,1.,0.707106781186548,1.,0.707106781186548,
1.),(1.,0.707106781186547,1.,0.707106781186547,1.,0.707106781186547,1.,
0.707106781186547,1.),(1.,0.707106781186547,1.,0.707106781186547,1.,0.707106781186547,
1.,0.707106781186547,1.),(1.,0.707106781186548,1.,0.707106781186548,1.,
0.707106781186548,1.,0.707106781186548,1.),(1.,0.707106781186547,1.,0.707106781186547,
1.,0.707106781186547,1.,0.707106781186547,1.),(1.,0.707106781186548,1.,
0.707106781186548,1.,0.707106781186548,1.,0.707106781186548,1.),(1.,0.707106781186547,
1.,0.707106781186547,1.,0.707106781186547,1.,0.707106781186547,1.),(1.,
0.707106781186548,1.,0.707106781186548,1.,0.707106781186548,1.,0.707106781186548,
1.),(1.,0.707106781186547,1.,0.707106781186547,1.,0.707106781186547,1.,
0.707106781186547,1.),(1.,0.707106781186548,1.,0.707106781186548,1.,0.707106781186548,
1.,0.707106781186548,1.),(1.,0.707106781186547,1.,0.707106781186547,1.,
0.707106781186547,1.,0.707106781186547,1.),(1.,0.707106781186547,1.,0.707106781186547,
1.,0.707106781186547,1.,0.707106781186547,1.),(1.,0.707106781186548,1.,
0.707106781186548,1.,0.707106781186548,1.,0.707106781186548,1.),(1.,0.707106781186547,
1.,0.707106781186547,1.,0.707106781186547,1.,0.707106781186547,1.),(1.,
0.707106781186548,1.,0.707106781186548,1.,0.707106781186548,1.,0.707106781186548,
1.),(1.,0.707106781186547,1.,0.707106781186547,1.,0.707106781186547,1.,
0.707106781186547,1.),(1.,0.707106781186548,1.,0.707106781186548,1.,0.707106781186548,
1.,0.707106781186548,1.),(1.,0.707106781186548,1.,0.707106781186548,1.,
0.707106781186548,1.,0.707106781186548,1.),(1.,0.707106781186548,1.,0.707106781186548,
1.,0.707106781186548,1.,0.707106781186548,1.),(1.,0.707106781186548,1.,
0.707106781186548,1.,0.707106781186548,1.,0.707106781186548,1.),(1.,0.707106781186547,
1.,0.707106781186547,1.,0.707106781186547,1.,0.707106781186547,1.),(1.,
0.707106781186548,1.,0.707106781186548,1.,0.707106781186548,1.,0.707106781186548,
1.),(1.,0.707106781186548,1.,0.707106781186548,1.,0.707106781186548,1.,
0.707106781186548,1.),(1.,0.707106781186548,1.,0.707106781186548,1.,0.707106781186548,
1.,0.707106781186548,1.),(1.,0.707106781186547,1.,0.707106781186547,1.,
0.707106781186547,1.,0.707106781186547,1.),(1.,0.707106781186548,1.,0.707106781186548,
1.,0.707106781186548,1.,0.707106781186548,1.),(1.,0.707106781186548,1.,
0.707106781186548,1.,0.707106781186548,1.,0.707106781186548,1.),(1.,0.707106781186547,
1.,0.707106781186547,1.,0.707106781186547,1.,0.707106781186547,1.),(1.,
0.707106781186548,1.,0.707106781186548,1.,0.707106781186548,1.,0.707106781186548,
1.),(1.,0.707106781186547,1.,0.707106781186547,1.,0.707106781186547,1.,
0.707106781186547,1.),(1.,0.707106781186548,1.,0.707106781186548,1.,0.707106781186548,
1.,0.707106781186548,1.),(1.,0.707106781186547,1.,0.707106781186547,1.,
0.707106781186547,1.,0.707106781186547,1.),(1.,0.707106781186547,1.,0.707106781186547,
1.,0.707106781186547,1.,0.707106781186547,1.),(1.,0.707106781186547,1.,
0.707106781186547,1.,0.707106781186547,1.,0.707106781186547,1.),(1.,0.707106781186548,
1.,0.707106781186548,1.,0.707106781186548,1.,0.707106781186548,1.),(1.,
0.707106781186548,1.,0.707106781186548,1.,0.707106781186548,1.,0.707106781186548,
1.),(1.,0.707106781186547,1.,0.707106781186547,1.,0.707106781186547,1.,
0.707106781186547,1.),(1.,0.707106781186548,1.,0.707106781186548,1.,0.707106781186548,
1.,0.707106781186548,1.),(1.,0.707106781186547,1.,0.707106781186547,1.,
0.707106781186547,1.,0.707106781186547,1.),(1.,0.707106781186548,1.,0.707106781186548,
1.,0.707106781186548,1.,0.707106781186548,1.),(1.,0.707106781186547,1.,
0.707106781186547,1.,0.707106781186547,1.,0.707106781186547,1.),(1.,0.707106781186548,
1.,0.707106781186548,1.,0.707106781186548,1.,0.707106781186548,1.),(1.,
0.707106781186548,1.,0.707106781186548,1.,0.707106781186548,1.,0.707106781186548,
1.),(1.,0.707106781186547,1.,0.707106781186547,1.,0.707106781186547,1.,
0.707106781186547,1.),(1.,0.707106781186548,1.,0.707106781186548,1.,0.707106781186548,
1.,0.707106781186548,1.),(1.,0.707106781186547,1.,0.707106781186547,1.,
0.707106781186547,1.,0.707106781186547,1.),(1.,0.707106781186547,1.,0.707106781186547,
1.,0.707106781186547,1.,0.707106781186547,1.),(1.,0.707106781186548,1.,
0.707106781186548,1.,0.707106781186548,1.,0.707106781186548,1.),(1.,0.707106781186547,
1.,0.707106781186547,1.,0.707106781186547,1.,0.707106781186547,1.),(1.,
0.707106781186547,1.,0.707106781186547,1.,0.707106781186547,1.,0.707106781186547,
1.),(1.,0.707106781186547,1.,0.707106781186547,1.,0.707106781186547,1.,
0.707106781186547,1.),(1.,0.707106781186548,1.,0.707106781186548,1.,0.707106781186548,
1.,0.707106781186548,1.),(1.,0.707106781186547,1.,0.707106781186547,1.,
0.707106781186547,1.,0.707106781186547,1.),(1.,0.707106781186548,1.,0.707106781186548,
1.,0.707106781186548,1.,0.707106781186548,1.),(1.,0.707106781186548,1.,
0.707106781186548,1.,0.707106781186548,1.,0.707106781186548,1.),(1.,0.707106781186547,
1.,0.707106781186547,1.,0.707106781186547,1.,0.707106781186547,1.),(1.,
0.707106781186548,1.,0.707106781186548,1.,0.707106781186548,1.,0.707106781186548,
1.),(1.,0.707106781186547,1.,0.707106781186547,1.,0.707106781186547,1.,
0.707106781186547,1.),(1.,0.707106781186548,1.,0.707106781186548,1.,0.707106781186548,
1.,0.707106781186548,1.),(1.,0.707106781186548,1.,0.707106781186548,1.,
0.707106781186548,1.,0.707106781186548,1.),(1.,0.707106781186548,1.,0.707106781186548,
1.,0.707106781186548,1.,0.707106781186548,1.),(1.,0.707106781186548,1.,
0.707106781186548,1.,0.707106781186548,1.,0.707106781186548,1.),(1.,0.707106781186547,
1.,0.707106781186547,1.,0.707106781186547,1.,0.707106781186547,1.),(1.,
0.707106781186548,1.,0.707106781186548,1.,0.707106781186548,1.,0.707106781186548,
1.),(1.,0.707106781186547,1.,0.707106781186547,1.,0.707106781186547,1.,
0.707106781186547,1.),(1.,0.707106781186548,1.,0.707106781186548,1.,0.707106781186548,
1.,0.707106781186548,1.),(1.,0.707106781186547,1.,0.707106781186547,1.,
0.707106781186547,1.,0.707106781186547,1.),(1.,0.707106781186548,1.,0.707106781186548,
1.,0.707106781186548,1.,0.707106781186548,1.),(1.,0.707106781186547,1.,
0.707106781186547,1.,0.707106781186547,1.,0.707106781186547,1.),(1.,0.707106781186547,
1.,0.707106781186547,1.,0.707106781186547,1.,0.707106781186547,1.),(1.,
0.707106781186547,1.,0.707106781186547,1.,0.707106781186547,1.,0.707106781186547,
1.),(1.,0.707106781186547,1.,0.707106781186547,1.,0.707106781186547,1.,
0.707106781186547,1.),(1.,0.707106781186548,1.,0.707106781186548,1.,0.707106781186548,
1.,0.707106781186548,1.),(1.,0.707106781186547,1.,0.707106781186547,1.,
0.707106781186547,1.,0.707106781186547,1.),(1.,0.707106781186548,1.,0.707106781186548,
1.,0.707106781186548,1.,0.707106781186548,1.),(1.,0.707106781186547,1.,
0.707106781186547,1.,0.707106781186547,1.,0.707106781186547,1.),(1.,0.707106781186547,
1.,0.707106781186547,1.,0.707106781186547,1.,0.707106781186547,1.),(1.,
0.707106781186548,1.,0.707106781186548,1.,0.707106781186548,1.,0.707106781186548,
1.),(1.,0.707106781186547,1.,0.707106781186547,1.,0.707106781186547,1.,
0.707106781186547,1.),(1.,0.707106781186548,1.,0.707106781186548,1.,0.707106781186548,
1.,0.707106781186548,1.),(1.,0.707106781186547,1.,0.707106781186547,1.,
0.707106781186547,1.,0.707106781186547,1.),(1.,0.707106781186548,1.,0.707106781186548,
1.,0.707106781186548,1.,0.707106781186548,1.),(1.,0.707106781186547,1.,
0.707106781186547,1.,0.707106781186547,1.,0.707106781186547,1.),(1.,0.707106781186548,
1.,0.707106781186548,1.,0.707106781186548,1.,0.707106781186548,1.),(1.,
0.707106781186548,1.,0.707106781186548,1.,0.707106781186548,1.,0.707106781186548,
1.),(1.,0.707106781186548,1.,0.707106781186548,1.,0.707106781186548,1.,
0.707106781186548,1.),(1.,0.707106781186548,1.,0.707106781186548,1.,0.707106781186548,
1.,0.707106781186548,1.),(1.,0.707106781186547,1.,0.707106781186547,1.,
0.707106781186547,1.,0.707106781186547,1.),(1.,0.707106781186548,1.,0.707106781186548,
1.,0.707106781186548,1.,0.707106781186548,1.),(1.,0.707106781186548,1.,
0.707106781186548,1.,0.707106781186548,1.,0.707106781186548,1.),(1.,0.707106781186547,
1.,0.707106781186547,1.,0.707106781186547,1.,0.707106781186547,1.),(1.,
0.707106781186548,1.,0.707106781186548,1.,0.707106781186548,1.,0.707106781186548,
1.),(1.,0.707106781186547,1.,0.707106781186547,1.,0.707106781186547,1.,
0.707106781186547,1.),(1.,0.707106781186548,1.,0.707106781186548,1.,0.707106781186548,
1.,0.707106781186548,1.),(1.,0.707106781186547,1.,0.707106781186547,1.,
0.707106781186547,1.,0.707106781186547,1.),(1.,0.707106781186548,1.,0.707106781186548,
1.,0.707106781186548,1.,0.707106781186548,1.),(1.,0.707106781186547,1.,
0.707106781186547,1.,0.707106781186547,1.,0.707106781186547,1.),(1.,0.707106781186547,
1.,0.707106781186547,1.,0.707106781186547,1.,0.707106781186547,1.),(1.,
0.707106781186548,1.,0.707106781186548,1.,0.707106781186548,1.,0.707106781186548,
1.),(1.,0.707106781186547,1.,0.707106781186547,1.,0.707106781186547,1.,
0.707106781186547,1.),(1.,0.707106781186548,1.,0.707106781186548,1.,0.707106781186548,
1.,0.707106781186548,1.),(1.,0.707106781186547,1.,0.707106781186547,1.,
0.707106781186547,1.,0.707106781186547,1.),(1.,0.707106781186547,1.,0.707106781186547,
1.,0.707106781186547,1.,0.707106781186547,1.),(1.,0.707106781186548,1.,
0.707106781186548,1.,0.707106781186548,1.,0.707106781186548,1.),(1.,0.707106781186547,
1.,0.707106781186547,1.,0.707106781186547,1.,0.707106781186547,1.),(1.,
0.707106781186548,1.,0.707106781186548,1.,0.707106781186548,1.,0.707106781186548,
1.),(1.,0.707106781186547,1.,0.707106781186547,1.,0.707106781186547,1.,
0.707106781186547,1.),(1.,0.707106781186547,1.,0.707106781186547,1.,0.707106781186547,
1.,0.707106781186547,1.),(1.,0.707106781186548,1.,0.707106781186548,1.,
0.707106781186548,1.,0.707106781186548,1.),(1.,0.707106781186548,1.,0.707106781186548,
1.,0.707106781186548,1.,0.707106781186548,1.),(1.,0.707106781186548,1.,
0.707106781186548,1.,0.707106781186548,1.,0.707106781186548,1.),(1.,0.707106781186548,
1.,0.707106781186548,1.,0.707106781186548,1.,0.707106781186548,1.),(1.,
0.707106781186548,1.,0.707106781186548,1.,0.707106781186548,1.,0.707106781186548,
1.),(1.,0.707106781186548,1.,0.707106781186548,1.,0.707106781186548,1.,
0.707106781186548,1.),(1.,0.707106781186548,1.,0.707106781186548,1.,0.707106781186548,
1.,0.707106781186548,1.),(1.,0.707106781186548,1.,0.707106781186548,1.,
0.707106781186548,1.,0.707106781186548,1.),(1.,0.707106781186548,1.,0.707106781186548,
1.,0.707106781186548,1.,0.707106781186548,1.),(1.,0.707106781186547,1.,
0.707106781186547,1.,0.707106781186547,1.,0.707106781186547,1.),(1.,0.707106781186548,
1.,0.707106781186548,1.,0.707106781186548,1.,0.707106781186548,1.),(1.,
0.707106781186547,1.,0.707106781186547,1.,0.707106781186547,1.,0.707106781186547,
1.),(1.,0.707106781186547,1.,0.707106781186547,1.,0.707106781186547,1.,
0.707106781186547,1.),(1.,0.707106781186548,1.,0.707106781186548,1.,0.707106781186548,
1.,0.707106781186548,1.),(1.,0.707106781186547,1.,0.707106781186547,1.,
0.707106781186547,1.,0.707106781186547,1.),(1.,0.707106781186548,1.,0.707106781186548,
1.,0.707106781186548,1.,0.707106781186548,1.),(1.,0.707106781186548,1.,
0.707106781186548,1.,0.707106781186548,1.,0.707106781186548,1.),(1.,0.707106781186547,
1.,0.707106781186547,1.,0.707106781186547,1.,0.707106781186547,1.),(1.,
0.707106781186547,1.,0.707106781186547,1.,0.707106781186547,1.,0.707106781186547,
1.),(1.,0.707106781186548,1.,0.707106781186548,1.,0.707106781186548,1.,
0.707106781186548,1.),(1.,0.707106781186548,1.,0.707106781186548,1.,0.707106781186548,
1.,0.707106781186548,1.),(1.,0.707106781186547,1.,0.707106781186547,1.,
0.707106781186547,1.,0.707106781186547,1.),(1.,0.707106781186547,1.,0.707106781186547,
1.,0.707106781186547,1.,0.707106781186547,1.),(1.,0.707106781186547,1.,
0.707106781186547,1.,0.707106781186547,1.,0.707106781186547,1.),(1.,0.707106781186547,
1.,0.707106781186547,1.,0.707106781186547,1.,0.707106781186547,1.),(1.,
0.707106781186547,1.,0.707106781186547,1.,0.707106781186547,1.,0.707106781186547,
1.),(1.,0.707106781186548,1.,0.707106781186548,1.,0.707106781186548,1.,
0.707106781186548,1.),(1.,0.707106781186547,1.,0.707106781186547,1.,0.707106781186547,
1.,0.707106781186547,1.),(1.,0.707106781186548,1.,0.707106781186548,1.,
0.707106781186548,1.,0.707106781186548,1.),(1.,0.707106781186548,1.,0.707106781186548,
1.,0.707106781186548,1.,0.707106781186548,1.),(1.,0.707106781186548,1.,
0.707106781186548,1.,0.707106781186548,1.,0.707106781186548,1.),(1.,0.707106781186547,
1.,0.707106781186547,1.,0.707106781186547,1.,0.707106781186547,1.),(1.,
0.707106781186548,1.,0.707106781186548,1.,0.707106781186548,1.,0.707106781186548,
1.),(1.,0.707106781186547,1.,0.707106781186547,1.,0.707106781186547,1.,
0.707106781186547,1.),(1.,0.707106781186548,1.,0.707106781186548,1.,0.707106781186548,
1.,0.707106781186548,1.),(1.,0.707106781186547,1.,0.707106781186547,1.,
0.707106781186547,1.,0.707106781186547,1.),(1.,0.707106781186548,1.,0.707106781186548,
1.,0.707106781186548,1.,0.707106781186548,1.),(1.,0.707106781186547,1.,
0.707106781186547,1.,0.707106781186547,1.,0.707106781186547,1.),(1.,0.707106781186548,
1.,0.707106781186548,1.,0.707106781186548,1.,0.707106781186548,1.),(1.,
0.707106781186548,1.,0.707106781186548,1.,0.707106781186548,1.,0.707106781186548,
1.),(1.,0.707106781186547,1.,0.707106781186547,1.,0.707106781186547,1.,
0.707106781186547,1.),(1.,0.707106781186547,1.,0.707106781186547,1.,0.707106781186547,
1.,0.707106781186547,1.),(1.,0.707106781186548,1.,0.707106781186548,1.,
0.707106781186548,1.,0.707106781186548,1.),(1.,0.707106781186548,1.,0.707106781186548,
1.,0.707106781186548,1.,0.707106781186548,1.),(1.,0.707106781186548,1.,
0.707106781186548,1.,0.707106781186548,1.,0.707106781186548,1.),(1.,0.707106781186547,
1.,0.707106781186547,1.,0.707106781186547,1.,0.707106781186547,1.),(1.,
0.707106781186547,1.,0.707106781186547,1.,0.707106781186547,1.,0.707106781186547,
1.),(1.,0.707106781186548,1.,0.707106781186548,1.,0.707106781186548,1.,
0.707106781186548,1.),(1.,0.707106781186547,1.,0.707106781186547,1.,0.707106781186547,
1.,0.707106781186547,1.),(1.,0.707106781186547,1.,0.707106781186547,1.,
0.707106781186547,1.,0.707106781186547,1.),(1.,0.707106781186548,1.,0.707106781186548,
1.,0.707106781186548,1.,0.707106781186548,1.),(1.,0.707106781186547,1.,
0.707106781186547,1.,0.707106781186547,1.,0.707106781186547,1.),(1.,0.707106781186548,
1.,0.707106781186548,1.,0.707106781186548,1.,0.707106781186548,1.),(1.,
0.707106781186547,1.,0.707106781186547,1.,0.707106781186547,1.,0.707106781186547,
1.),(1.,0.707106781186547,1.,0.707106781186547,1.,0.707106781186547,1.,
0.707106781186547,1.),(1.,0.707106781186548,1.,0.707106781186548,1.,0.707106781186548,
1.,0.707106781186548,1.),(1.,0.707106781186548,1.,0.707106781186548,1.,
0.707106781186548,1.,0.707106781186548,1.),(1.,0.707106781186548,1.,0.707106781186548,
1.,0.707106781186548,1.,0.707106781186548,1.),(1.,0.707106781186547,1.,
0.707106781186547,1.,0.707106781186547,1.,0.707106781186547,1.),(1.,0.707106781186547,
1.,0.707106781186547,1.,0.707106781186547,1.,0.707106781186547,1.),(1.,
0.707106781186548,1.,0.707106781186548,1.,0.707106781186548,1.,0.707106781186548,
1.),(1.,0.707106781186547,1.,0.707106781186547,1.,0.707106781186547,1.,
0.707106781186547,1.),(1.,0.707106781186548,1.,0.707106781186548,1.,0.707106781186548,
1.,0.707106781186548,1.),(1.,0.707106781186547,1.,0.707106781186547,1.,
0.707106781186547,1.,0.707106781186547,1.),(1.,0.707106781186548,1.,0.707106781186548,
1.,0.707106781186548,1.,0.707106781186548,1.),(1.,0.707106781186547,1.,
0.707106781186547,1.,0.707106781186547,1.,0.707106781186547,1.),(1.,0.707106781186548,
1.,0.707106781186548,1.,0.707106781186548,1.,0.707106781186548,1.),(1.,
0.707106781186548,1.,0.707106781186548,1.,0.707106781186548,1.,0.707106781186548,
1.),(1.,0.707106781186547,1.,0.707106781186547,1.,0.707106781186547,1.,
0.707106781186547,1.),(1.,0.707106781186548,1.,0.707106781186548,1.,0.707106781186548,
1.,0.707106781186548,1.),(1.,0.707106781186547,1.,0.707106781186547,1.,
0.707106781186547,1.,0.707106781186547,1.),(1.,0.707106781186548,1.,0.707106781186548,
1.,0.707106781186548,1.,0.707106781186548,1.),(1.,0.707106781186547,1.,
0.707106781186547,1.,0.707106781186547,1.,0.707106781186547,1.),(1.,0.707106781186547,
1.,0.707106781186547,1.,0.707106781186547,1.,0.707106781186547,1.),(1.,
0.707106781186547,1.,0.707106781186547,1.,0.707106781186547,1.,0.707106781186547,
1.),(1.,0.707106781186548,1.,0.707106781186548,1.,0.707106781186548,1.,
0.707106781186548,1.),(1.,0.707106781186547,1.,0.707106781186547,1.,0.707106781186547,
1.,0.707106781186547,1.),(1.,0.707106781186548,1.,0.707106781186548,1.,
0.707106781186548,1.,0.707106781186548,1.),(1.,0.707106781186547,1.,0.707106781186547,
1.,0.707106781186547,1.,0.707106781186547,1.),(1.,0.707106781186547,1.,
0.707106781186547,1.,0.707106781186547,1.,0.707106781186547,1.),(1.,0.707106781186547,
1.,0.707106781186547,1.,0.707106781186547,1.,0.707106781186547,1.),(1.,
0.707106781186548,1.,0.707106781186548,1.,0.707106781186548,1.,0.707106781186548,
1.),(1.,0.707106781186547,1.,0.707106781186547,1.,0.707106781186547,1.,
0.707106781186547,1.),(1.,0.707106781186547,1.,0.707106781186547,1.,0.707106781186547,
1.,0.707106781186547,1.),(1.,0.707106781186548,1.,0.707106781186548,1.,
0.707106781186548,1.,0.707106781186548,1.),(1.,0.707106781186548,1.,0.707106781186548,
1.,0.707106781186548,1.,0.707106781186548,1.),(1.,0.707106781186547,1.,
0.707106781186547,1.,0.707106781186547,1.,0.707106781186547,1.),(1.,0.707106781186548,
1.,0.707106781186548,1.,0.707106781186548,1.,0.707106781186548,1.),(1.,
0.707106781186547,1.,0.707106781186547,1.,0.707106781186547,1.,0.707106781186547,
1.),(1.,0.707106781186548,1.,0.707106781186548,1.,0.707106781186548,1.,
0.707106781186548,1.),(1.,0.707106781186548,1.,0.707106781186548,1.,0.707106781186548,
1.,0.707106781186548,1.),(1.,0.707106781186547,1.,0.707106781186547,1.,
0.707106781186547,1.,0.707106781186547,1.),(1.,0.707106781186548,1.,0.707106781186548,
1.,0.707106781186548,1.,0.707106781186548,1.),(1.,0.707106781186547,1.,
0.707106781186547,1.,0.707106781186547,1.,0.707106781186547,1.),(1.,0.707106781186547,
1.,0.707106781186547,1.,0.707106781186547,1.,0.707106781186547,1.),(1.,
0.707106781186548,1.,0.707106781186548,1.,0.707106781186548,1.,0.707106781186548,
1.),(1.,0.707106781186547,1.,0.707106781186547,1.,0.707106781186547,1.,
0.707106781186547,1.),(1.,0.707106781186547,1.,0.707106781186547,1.,0.707106781186547,
1.,0.707106781186547,1.),(1.,0.707106781186547,1.,0.707106781186547,1.,
0.707106781186547,1.,0.707106781186547,1.),(1.,0.707106781186548,1.,0.707106781186548,
1.,0.707106781186548,1.,0.707106781186548,1.),(1.,0.707106781186547,1.,
0.707106781186547,1.,0.707106781186547,1.,0.707106781186547,1.),(1.,0.707106781186548,
1.,0.707106781186548,1.,0.707106781186548,1.,0.707106781186548,1.),(1.,
0.707106781186547,1.,0.707106781186547,1.,0.707106781186547,1.,0.707106781186547,
1.),(1.,0.707106781186548,1.,0.707106781186548,1.,0.707106781186548,1.,
0.707106781186548,1.),(1.,0.707106781186548,1.,0.707106781186548,1.,0.707106781186548,
1.,0.707106781186548,1.),(1.,0.707106781186548,1.,0.707106781186548,1.,
0.707106781186548,1.,0.707106781186548,1.),(1.,0.707106781186547,1.,0.707106781186547,
1.,0.707106781186547,1.,0.707106781186547,1.),(1.,0.707106781186548,1.,
0.707106781186548,1.,0.707106781186548,1.,0.707106781186548,1.),(1.,0.707106781186548,
1.,0.707106781186548,1.,0.707106781186548,1.,0.707106781186548,1.),(1.,
0.707106781186548,1.,0.707106781186548,1.,0.707106781186548,1.,0.707106781186548,
1.),(1.,0.707106781186547,1.,0.707106781186547,1.,0.707106781186547,1.,
0.707106781186547,1.),(1.,0.707106781186548,1.,0.707106781186548,1.,0.707106781186548,
1.,0.707106781186548,1.),(1.,0.707106781186547,1.,0.707106781186547,1.,
0.707106781186547,1.,0.707106781186547,1.),(1.,0.707106781186547,1.,0.707106781186547,
1.,0.707106781186547,1.,0.707106781186547,1.),(1.,0.707106781186548,1.,
0.707106781186548,1.,0.707106781186548,1.,0.707106781186548,1.),(1.,0.707106781186547,
1.,0.707106781186547,1.,0.707106781186547,1.,0.707106781186547,1.),(1.,
0.707106781186547,1.,0.707106781186547,1.,0.707106781186547,1.,0.707106781186547,
1.),(1.,0.707106781186548,1.,0.707106781186548,1.,0.707106781186548,1.,
0.707106781186548,1.),(1.,0.707106781186548,1.,0.707106781186548,1.,0.707106781186548,
1.,0.707106781186548,1.),(1.,0.707106781186547,1.,0.707106781186547,1.,
0.707106781186547,1.,0.707106781186547,1.),(1.,0.707106781186548,1.,0.707106781186548,
1.,0.707106781186548,1.,0.707106781186548,1.),(1.,0.707106781186547,1.,
0.707106781186547,1.,0.707106781186547,1.,0.707106781186547,1.),(1.,0.707106781186548,
1.,0.707106781186548,1.,0.707106781186548,1.,0.707106781186548,1.),(1.,
0.707106781186548,1.,0.707106781186548,1.,0.707106781186548,1.,0.707106781186548,
1.),(1.,0.707106781186547,1.,0.707106781186547,1.,0.707106781186547,1.,
0.707106781186547,1.),(1.,0.707106781186548,1.,0.707106781186548,1.,0.707106781186548,
1.,0.707106781186548,1.),(1.,0.707106781186547,1.,0.707106781186547,1.,
0.707106781186547,1.,0.707106781186547,1.),(1.,0.707106781186548,1.,0.707106781186548,
1.,0.707106781186548,1.,0.707106781186548,1.),(1.,0.707106781186547,1.,
0.707106781186547,1.,0.707106781186547,1.,0.707106781186547,1.),(1.,0.707106781186548,
1.,0.707106781186548,1.,0.707106781186548,1.,0.707106781186548,1.),(1.,
0.707106781186547,1.,0.707106781186547,1.,0.707106781186547,1.,0.707106781186547,
1.),(1.,0.707106781186548,1.,0.707106781186548,1.,0.707106781186548,1.,
0.707106781186548,1.),(1.,0.707106781186548,1.,0.707106781186548,1.,0.707106781186548,
1.,0.707106781186548,1.),(1.,0.707106781186548,1.,0.707106781186548,1.,
0.707106781186548,1.,0.707106781186548,1.),(1.,0.707106781186547,1.,0.707106781186547,
1.,0.707106781186547,1.,0.707106781186547,1.),(1.,0.707106781186548,1.,
0.707106781186548,1.,0.707106781186548,1.,0.707106781186548,1.),(1.,0.707106781186548,
1.,0.707106781186548,1.,0.707106781186548,1.,0.707106781186548,1.),(1.,
0.707106781186547,1.,0.707106781186547,1.,0.707106781186547,1.,0.707106781186547,
1.),(1.,0.707106781186547,1.,0.707106781186547,1.,0.707106781186547,1.,
0.707106781186547,1.),(1.,0.707106781186548,1.,0.707106781186548,1.,0.707106781186548,
1.,0.707106781186548,1.),(1.,0.707106781186547,1.,0.707106781186547,1.,
0.707106781186547,1.,0.707106781186547,1.),(1.,0.707106781186548,1.,0.707106781186548,
1.,0.707106781186548,1.,0.707106781186548,1.),(1.,0.707106781186548,1.,
0.707106781186548,1.,0.707106781186548,1.,0.707106781186548,1.),(1.,0.707106781186547,
1.,0.707106781186547,1.,0.707106781186547,1.,0.707106781186547,1.),(1.,
0.707106781186548,1.,0.707106781186548,1.,0.707106781186548,1.,0.707106781186548,
1.),(1.,0.707106781186548,1.,0.707106781186548,1.,0.707106781186548,1.,
0.707106781186548,1.),(1.,0.707106781186547,1.,0.707106781186547,1.,0.707106781186547,
1.,0.707106781186547,1.),(1.,0.707106781186548,1.,0.707106781186548,1.,
0.707106781186548,1.,0.707106781186548,1.),(1.,0.707106781186548,1.,0.707106781186548,
1.,0.707106781186548,1.,0.707106781186548,1.),(1.,0.707106781186547,1.,
0.707106781186547,1.,0.707106781186547,1.,0.707106781186547,1.),(1.,0.707106781186547,
1.,0.707106781186547,1.,0.707106781186547,1.,0.707106781186547,1.),(1.,
0.707106781186548,1.,0.707106781186548,1.,0.707106781186548,1.,0.707106781186548,
1.),(1.,0.707106781186547,1.,0.707106781186547,1.,0.707106781186547,1.,
0.707106781186547,1.),(1.,0.707106781186548,1.,0.707106781186548,1.,0.707106781186548,
1.,0.707106781186548,1.),(1.,0.707106781186547,1.,0.707106781186547,1.,
0.707106781186547,1.,0.707106781186547,1.),(1.,0.707106781186548,1.,0.707106781186548,
1.,0.707106781186548,1.,0.707106781186548,1.),(1.,0.707106781186547,1.,
0.707106781186547,1.,0.707106781186547,1.,0.707106781186547,1.),(1.,0.707106781186548,
1.,0.707106781186548,1.,0.707106781186548,1.,0.707106781186548,1.),(1.,
0.707106781186548,1.,0.707106781186548,1.,0.707106781186548,1.,0.707106781186548,
1.),(1.,0.707106781186548,1.,0.707106781186548,1.,0.707106781186548,1.,
0.707106781186548,1.),(1.,0.707106781186547,1.,0.707106781186547,1.,0.707106781186547,
1.,0.707106781186547,1.),(1.,0.707106781186548,1.,0.707106781186548,1.,
0.707106781186548,1.,0.707106781186548,1.),(1.,0.707106781186547,1.,0.707106781186547,
1.,0.707106781186547,1.,0.707106781186547,1.),(1.,0.707106781186548,1.,
0.707106781186548,1.,0.707106781186548,1.,0.707106781186548,1.),(1.,0.707106781186547,
1.,0.707106781186547,1.,0.707106781186547,1.,0.707106781186547,1.),(1.,
0.707106781186548,1.,0.707106781186548,1.,0.707106781186548,1.,0.707106781186548,
1.),(1.,0.707106781186547,1.,0.707106781186547,1.,0.707106781186547,1.,
0.707106781186547,1.),(1.,0.707106781186548,1.,0.707106781186548,1.,0.707106781186548,
1.,0.707106781186548,1.),(1.,0.707106781186547,1.,0.707106781186547,1.,
0.707106781186547,1.,0.707106781186547,1.),(1.,0.707106781186548,1.,0.707106781186548,
1.,0.707106781186548,1.,0.707106781186548,1.),(1.,0.707106781186547,1.,
0.707106781186547,1.,0.707106781186547,1.,0.707106781186547,1.),(1.,0.707106781186548,
1.,0.707106781186548,1.,0.707106781186548,1.,0.707106781186548,1.),(1.,
0.707106781186547,1.,0.707106781186547,1.,0.707106781186547,1.,0.707106781186547,
1.),(1.,0.707106781186547,1.,0.707106781186547,1.,0.707106781186547,1.,
0.707106781186547,1.),(1.,0.707106781186547,1.,0.707106781186547,1.,0.707106781186547,
1.,0.707106781186547,1.),(1.,0.707106781186548,1.,0.707106781186548,1.,
0.707106781186548,1.,0.707106781186548,1.),(1.,0.707106781186547,1.,0.707106781186547,
1.,0.707106781186547,1.,0.707106781186547,1.),(1.,0.707106781186548,1.,
0.707106781186548,1.,0.707106781186548,1.,0.707106781186548,1.),(1.,0.707106781186547,
1.,0.707106781186547,1.,0.707106781186547,1.,0.707106781186547,1.),(1.,
0.707106781186548,1.,0.707106781186548,1.,0.707106781186548,1.,0.707106781186548,
1.),(1.,0.707106781186547,1.,0.707106781186547,1.,0.707106781186547,1.,
0.707106781186547,1.),(1.,0.707106781186548,1.,0.707106781186548,1.,0.707106781186548,
1.,0.707106781186548,1.),(1.,0.707106781186547,1.,0.707106781186547,1.,
0.707106781186547,1.,0.707106781186547,1.),(1.,0.707106781186548,1.,0.707106781186548,
1.,0.707106781186548,1.,0.707106781186548,1.),(1.,0.707106781186548,1.,
0.707106781186548,1.,0.707106781186548,1.,0.707106781186548,1.),(1.,0.707106781186548,
1.,0.707106781186548,1.,0.707106781186548,1.,0.707106781186548,1.),(1.,
0.707106781186547,1.,0.707106781186547,1.,0.707106781186547,1.,0.707106781186547,
1.),(1.,0.707106781186548,1.,0.707106781186548,1.,0.707106781186548,1.,
0.707106781186548,1.),(1.,0.707106781186547,1.,0.707106781186547,1.,0.707106781186547,
1.,0.707106781186547,1.),(1.,0.707106781186548,1.,0.707106781186548,1.,
0.707106781186548,1.,0.707106781186548,1.),(1.,0.707106781186548,1.,0.707106781186548,
1.,0.707106781186548,1.,0.707106781186548,1.),(1.,0.707106781186547,1.,
0.707106781186547,1.,0.707106781186547,1.,0.707106781186547,1.),(1.,0.707106781186548,
1.,0.707106781186548,1.,0.707106781186548,1.,0.707106781186548,1.),(1.,
0.707106781186547,1.,0.707106781186547,1.,0.707106781186547,1.,0.707106781186547,
1.),(1.,0.707106781186548,1.,0.707106781186548,1.,0.707106781186548,1.,
0.707106781186548,1.),(1.,0.707106781186547,1.,0.707106781186547,1.,0.707106781186547,
1.,0.707106781186547,1.),(1.,0.707106781186548,1.,0.707106781186548,1.,
0.707106781186548,1.,0.707106781186548,1.),(1.,0.707106781186547,1.,0.707106781186547,
1.,0.707106781186547,1.,0.707106781186547,1.),(1.,0.707106781186548,1.,
0.707106781186548,1.,0.707106781186548,1.,0.707106781186548,1.),(1.,0.707106781186547,
1.,0.707106781186547,1.,0.707106781186547,1.,0.707106781186547,1.),(1.,
0.707106781186547,1.,0.707106781186547,1.,0.707106781186547,1.,0.707106781186547,
1.),(1.,0.707106781186547,1.,0.707106781186547,1.,0.707106781186547,1.,
0.707106781186547,1.),(1.,0.707106781186548,1.,0.707106781186548,1.,0.707106781186548,
1.,0.707106781186548,1.),(1.,0.707106781186547,1.,0.707106781186547,1.,
0.707106781186547,1.,0.707106781186547,1.),(1.,0.707106781186547,1.,0.707106781186547,
1.,0.707106781186547,1.,0.707106781186547,1.),(1.,0.707106781186548,1.,
0.707106781186548,1.,0.707106781186548,1.,0.707106781186548,1.),(1.,0.707106781186547,
1.,0.707106781186547,1.,0.707106781186547,1.,0.707106781186547,1.),(1.,
0.707106781186548,1.,0.707106781186548,1.,0.707106781186548,1.,0.707106781186548,
1.),(1.,0.707106781186547,1.,0.707106781186547,1.,0.707106781186547,1.,
0.707106781186547,1.),(1.,0.707106781186547,1.,0.707106781186547,1.,0.707106781186547,
1.,0.707106781186547,1.),(1.,0.707106781186548,1.,0.707106781186548,1.,
0.707106781186548,1.,0.707106781186548,1.),(1.,0.707106781186547,1.,0.707106781186547,
1.,0.707106781186547,1.,0.707106781186547,1.),(1.,0.707106781186548,1.,
0.707106781186548,1.,0.707106781186548,1.,0.707106781186548,1.),(1.,0.707106781186547,
1.,0.707106781186547,1.,0.707106781186547,1.,0.707106781186547,1.),(1.,
0.707106781186548,1.,0.707106781186548,1.,0.707106781186548,1.,0.707106781186548,
1.),(1.,0.707106781186548,1.,0.707106781186548,1.,0.707106781186548,1.,
0.707106781186548,1.),(1.,0.707106781186548,1.,0.707106781186548,1.,0.707106781186548,
1.,0.707106781186548,1.),(1.,0.707106781186547,1.,0.707106781186547,1.,
0.707106781186547,1.,0.707106781186547,1.),(1.,0.707106781186547,1.,0.707106781186547,
1.,0.707106781186547,1.,0.707106781186547,1.),(1.,0.707106781186548,1.,
0.707106781186548,1.,0.707106781186548,1.,0.707106781186548,1.),(1.,0.707106781186548,
1.,0.707106781186548,1.,0.707106781186548,1.,0.707106781186548,1.),(1.,
0.707106781186547,1.,0.707106781186547,1.,0.707106781186547,1.,0.707106781186547,
1.),(1.,0.707106781186548,1.,0.707106781186548,1.,0.707106781186548,1.,
0.707106781186548,1.),(1.,0.707106781186547,1.,0.707106781186547,1.,0.707106781186547,
1.,0.707106781186547,1.),(1.,0.707106781186547,1.,0.707106781186547,1.,
0.707106781186547,1.,0.707106781186547,1.),(1.,0.707106781186547,1.,0.707106781186547,
1.,0.707106781186547,1.,0.707106781186547,1.),(1.,0.707106781186548,1.,
0.707106781186548,1.,0.707106781186548,1.,0.707106781186548,1.),(1.,0.707106781186547,
1.,0.707106781186547,1.,0.707106781186547,1.,0.707106781186547,1.),(1.,
0.707106781186548,1.,0.707106781186548,1.,0.707106781186548,1.,0.707106781186548,
1.),(1.,0.707106781186547,1.,0.707106781186547,1.,0.707106781186547,1.,
0.707106781186547,1.),(1.,0.707106781186548,1.,0.707106781186548,1.,0.707106781186548,
1.,0.707106781186548,1.),(1.,0.707106781186548,1.,0.707106781186548,1.,
0.707106781186548,1.,0.707106781186548,1.),(1.,0.707106781186548,1.,0.707106781186548,
1.,0.707106781186548,1.,0.707106781186548,1.),(1.,0.707106781186547,1.,
0.707106781186547,1.,0.707106781186547,1.,0.707106781186547,1.),(1.,0.707106781186547,
1.,0.707106781186547,1.,0.707106781186547,1.,0.707106781186547,1.),(1.,
0.707106781186547,1.,0.707106781186547,1.,0.707106781186547,1.,0.707106781186547,
1.),(1.,0.707106781186547,1.,0.707106781186547,1.,0.707106781186547,1.,
0.707106781186547,1.),(1.,0.707106781186547,1.,0.707106781186547,1.,0.707106781186547,
1.,0.707106781186547,1.),(1.,0.707106781186547,1.,0.707106781186547,1.,
0.707106781186547,1.,0.707106781186547,1.),(1.,0.707106781186548,1.,0.707106781186548,
1.,0.707106781186548,1.,0.707106781186548,1.),(1.,0.707106781186547,1.,
0.707106781186547,1.,0.707106781186547,1.,0.707106781186547,1.),(1.,0.707106781186548,
1.,0.707106781186548,1.,0.707106781186548,1.,0.707106781186548,1.),(1.,
0.707106781186547,1.,0.707106781186547,1.,0.707106781186547,1.,0.707106781186547,
1.),(1.,0.707106781186548,1.,0.707106781186548,1.,0.707106781186548,1.,
0.707106781186548,1.),(1.,0.707106781186547,1.,0.707106781186547,1.,0.707106781186547,
1.,0.707106781186547,1.),(1.,0.707106781186547,1.,0.707106781186547,1.,
0.707106781186547,1.,0.707106781186547,1.),(1.,0.707106781186548,1.,0.707106781186548,
1.,0.707106781186548,1.,0.707106781186548,1.),(1.,0.707106781186547,1.,
0.707106781186547,1.,0.707106781186547,1.,0.707106781186547,1.),(1.,0.707106781186547,
1.,0.707106781186547,1.,0.707106781186547,1.,0.707106781186547,1.),(1.,
0.707106781186548,1.,0.707106781186548,1.,0.707106781186548,1.,0.707106781186548,
1.),(1.,0.707106781186548,1.,0.707106781186548,1.,0.707106781186548,1.,
0.707106781186548,1.),(1.,0.707106781186547,1.,0.707106781186547,1.,0.707106781186547,
1.,0.707106781186547,1.),(1.,0.707106781186547,1.,0.707106781186547,1.,
0.707106781186547,1.,0.707106781186547,1.),(1.,0.707106781186547,1.,0.707106781186547,
1.,0.707106781186547,1.,0.707106781186547,1.),(1.,0.707106781186548,1.,
0.707106781186548,1.,0.707106781186548,1.,0.707106781186548,1.),(1.,0.707106781186547,
1.,0.707106781186547,1.,0.707106781186547,1.,0.707106781186547,1.),(1.,
0.707106781186547,1.,0.707106781186547,1.,0.707106781186547,1.,0.707106781186547,
1.),(1.,0.707106781186548,1.,0.707106781186548,1.,0.707106781186548,1.,
0.707106781186548,1.),(1.,0.707106781186548,1.,0.707106781186548,1.,0.707106781186548,
1.,0.707106781186548,1.)))
REPRESENTATION_ITEM('')
SURFACE()
) ;
#62=(
BOUNDED_SURFACE()
B_SPLINE_SURFACE(2,3,((#174417,#174418,#174419,#174420,#174421,#174422,
#174423),(#174424,#174425,#174426,#174427,#174428,#174429,#174430),(#174431,
#174432,#174433,#174434,#174435,#174436,#174437),(#174438,#174439,#174440,
#174441,#174442,#174443,#174444),(#174445,#174446,#174447,#174448,#174449,
#174450,#174451),(#174452,#174453,#174454,#174455,#174456,#174457,#174458),
(#174459,#174460,#174461,#174462,#174463,#174464,#174465),(#174466,#174467,
#174468,#174469,#174470,#174471,#174472),(#174473,#174474,#174475,#174476,
#174477,#174478,#174479)),.UNSPECIFIED.,.T.,.F.,.F.)
B_SPLINE_SURFACE_WITH_KNOTS((3,2,2,2,3),(4,1,1,1,4),(0.,0.117809724509617,
0.235619449019234,0.353429173528852,0.471238898038469),(0.,0.0911446219616379,
0.182289243923276,0.273433865884915,0.364578487846551),.UNSPECIFIED.)
GEOMETRIC_REPRESENTATION_ITEM()
RATIONAL_B_SPLINE_SURFACE(((1.,1.,1.,1.,1.,1.,1.),(0.707106781186548,0.707106781186548,
0.707106781186547,0.707106781186548,0.707106781186547,0.707106781186548,
0.707106781186548),(1.,1.,1.,1.,1.,1.,1.),(0.707106781186548,0.707106781186548,
0.707106781186547,0.707106781186548,0.707106781186547,0.707106781186548,
0.707106781186548),(1.,1.,1.,1.,1.,1.,1.),(0.707106781186548,0.707106781186548,
0.707106781186547,0.707106781186548,0.707106781186547,0.707106781186548,
0.707106781186548),(1.,1.,1.,1.,1.,1.,1.),(0.707106781186548,0.707106781186548,
0.707106781186547,0.707106781186548,0.707106781186547,0.707106781186548,
0.707106781186548),(1.,1.,1.,1.,1.,1.,1.)))
REPRESENTATION_ITEM('')
SURFACE()
) ;
#63=(
BOUNDED_SURFACE()
B_SPLINE_SURFACE(2,3,((#174489,#174490,#174491,#174492),(#174493,#174494,
#174495,#174496),(#174497,#174498,#174499,#174500),(#174501,#174502,#174503,
#174504),(#174505,#174506,#174507,#174508),(#174509,#174510,#174511,#174512),
(#174513,#174514,#174515,#174516),(#174517,#174518,#174519,#174520),(#174521,
#174522,#174523,#174524)),.UNSPECIFIED.,.T.,.F.,.F.)
B_SPLINE_SURFACE_WITH_KNOTS((3,2,2,2,3),(4,4),(0.,0.117809724509617,0.235619449019234,
0.353429173528852,0.471238898038469),(0.,1.1454147408364),.UNSPECIFIED.)
GEOMETRIC_REPRESENTATION_ITEM()
RATIONAL_B_SPLINE_SURFACE(((1.,1.,1.,1.),(0.707106781186548,0.707106781186548,
0.707106781186547,0.707106781186548),(1.,1.,1.,1.),(0.707106781186548,0.707106781186548,
0.707106781186547,0.707106781186548),(1.,1.,1.,1.),(0.707106781186548,0.707106781186548,
0.707106781186547,0.707106781186548),(1.,1.,1.,1.),(0.707106781186548,0.707106781186548,
0.707106781186547,0.707106781186548),(1.,1.,1.,1.)))
REPRESENTATION_ITEM('')
SURFACE()
) ;
#64=(
BOUNDED_SURFACE()
B_SPLINE_SURFACE(2,3,((#174532,#174533,#174534,#174535,#174536,#174537,
#174538,#174539,#174540,#174541,#174542,#174543,#174544,#174545,#174546,
#174547,#174548,#174549,#174550),(#174551,#174552,#174553,#174554,#174555,
#174556,#174557,#174558,#174559,#174560,#174561,#174562,#174563,#174564,
#174565,#174566,#174567,#174568,#174569),(#174570,#174571,#174572,#174573,
#174574,#174575,#174576,#174577,#174578,#174579,#174580,#174581,#174582,
#174583,#174584,#174585,#174586,#174587,#174588),(#174589,#174590,#174591,
#174592,#174593,#174594,#174595,#174596,#174597,#174598,#174599,#174600,
#174601,#174602,#174603,#174604,#174605,#174606,#174607),(#174608,#174609,
#174610,#174611,#174612,#174613,#174614,#174615,#174616,#174617,#174618,
#174619,#174620,#174621,#174622,#174623,#174624,#174625,#174626),(#174627,
#174628,#174629,#174630,#174631,#174632,#174633,#174634,#174635,#174636,
#174637,#174638,#174639,#174640,#174641,#174642,#174643,#174644,#174645),
(#174646,#174647,#174648,#174649,#174650,#174651,#174652,#174653,#174654,
#174655,#174656,#174657,#174658,#174659,#174660,#174661,#174662,#174663,
#174664),(#174665,#174666,#174667,#174668,#174669,#174670,#174671,#174672,
#174673,#174674,#174675,#174676,#174677,#174678,#174679,#174680,#174681,
#174682,#174683),(#174684,#174685,#174686,#174687,#174688,#174689,#174690,
#174691,#174692,#174693,#174694,#174695,#174696,#174697,#174698,#174699,
#174700,#174701,#174702)),.UNSPECIFIED.,.T.,.F.,.F.)
B_SPLINE_SURFACE_WITH_KNOTS((3,2,2,2,3),(4,1,1,1,1,1,1,1,1,1,1,1,1,1,1,
1,4),(0.,0.117809724509617,0.235619449019234,0.353429173528852,0.471238898038469),
(0.,0.226732296973331,0.464902013928651,0.70307173088397,0.9298040278573,
1.15653632483063,1.39470604178595,1.63287575874127,1.8596080557146,2.08634035268793,
2.32451006964325,2.56267978659857,2.7894120835719,3.01614438054523,3.25431409750055,
3.49248381445586,3.7192161114292),.UNSPECIFIED.)
GEOMETRIC_REPRESENTATION_ITEM()
RATIONAL_B_SPLINE_SURFACE(((1.,1.,1.,1.,1.,1.,1.,1.,1.,1.,1.,1.,1.,1.,1.,
1.,1.,1.,1.),(0.707106781186548,0.707106781186547,0.707106781186548,0.707106781186547,
0.707106781186548,0.707106781186547,0.707106781186548,0.707106781186547,
0.707106781186547,0.707106781186547,0.707106781186548,0.707106781186547,
0.707106781186547,0.707106781186547,0.707106781186547,0.707106781186547,
0.707106781186548,0.707106781186547,0.707106781186548),(1.,1.,1.,1.,1.,
1.,1.,1.,1.,1.,1.,1.,1.,1.,1.,1.,1.,1.,1.),(0.707106781186548,0.707106781186547,
0.707106781186548,0.707106781186547,0.707106781186548,0.707106781186547,
0.707106781186548,0.707106781186547,0.707106781186547,0.707106781186547,
0.707106781186548,0.707106781186547,0.707106781186547,0.707106781186547,
0.707106781186547,0.707106781186547,0.707106781186548,0.707106781186547,
0.707106781186548),(1.,1.,1.,1.,1.,1.,1.,1.,1.,1.,1.,1.,1.,1.,1.,1.,1.,
1.,1.),(0.707106781186548,0.707106781186547,0.707106781186548,0.707106781186547,
0.707106781186548,0.707106781186547,0.707106781186548,0.707106781186547,
0.707106781186547,0.707106781186547,0.707106781186548,0.707106781186547,
0.707106781186547,0.707106781186547,0.707106781186547,0.707106781186547,
0.707106781186548,0.707106781186547,0.707106781186548),(1.,1.,1.,1.,1.,
1.,1.,1.,1.,1.,1.,1.,1.,1.,1.,1.,1.,1.,1.),(0.707106781186548,0.707106781186547,
0.707106781186548,0.707106781186547,0.707106781186548,0.707106781186547,
0.707106781186548,0.707106781186547,0.707106781186547,0.707106781186547,
0.707106781186548,0.707106781186547,0.707106781186547,0.707106781186547,
0.707106781186547,0.707106781186547,0.707106781186548,0.707106781186547,
0.707106781186548),(1.,1.,1.,1.,1.,1.,1.,1.,1.,1.,1.,1.,1.,1.,1.,1.,1.,
1.,1.)))
REPRESENTATION_ITEM('')
SURFACE()
) ;
#65=(
BOUNDED_SURFACE()
B_SPLINE_SURFACE(3,2,((#174725,#174726,#174727,#174728,#174729,#174730,
#174731,#174732,#174733),(#174734,#174735,#174736,#174737,#174738,#174739,
#174740,#174741,#174742),(#174743,#174744,#174745,#174746,#174747,#174748,
#174749,#174750,#174751),(#174752,#174753,#174754,#174755,#174756,#174757,
#174758,#174759,#174760),(#174761,#174762,#174763,#174764,#174765,#174766,
#174767,#174768,#174769),(#174770,#174771,#174772,#174773,#174774,#174775,
#174776,#174777,#174778),(#174779,#174780,#174781,#174782,#174783,#174784,
#174785,#174786,#174787),(#174788,#174789,#174790,#174791,#174792,#174793,
#174794,#174795,#174796),(#174797,#174798,#174799,#174800,#174801,#174802,
#174803,#174804,#174805),(#174806,#174807,#174808,#174809,#174810,#174811,
#174812,#174813,#174814),(#174815,#174816,#174817,#174818,#174819,#174820,
#174821,#174822,#174823),(#174824,#174825,#174826,#174827,#174828,#174829,
#174830,#174831,#174832),(#174833,#174834,#174835,#174836,#174837,#174838,
#174839,#174840,#174841),(#174842,#174843,#174844,#174845,#174846,#174847,
#174848,#174849,#174850),(#174851,#174852,#174853,#174854,#174855,#174856,
#174857,#174858,#174859),(#174860,#174861,#174862,#174863,#174864,#174865,
#174866,#174867,#174868),(#174869,#174870,#174871,#174872,#174873,#174874,
#174875,#174876,#174877),(#174878,#174879,#174880,#174881,#174882,#174883,
#174884,#174885,#174886),(#174887,#174888,#174889,#174890,#174891,#174892,
#174893,#174894,#174895),(#174896,#174897,#174898,#174899,#174900,#174901,
#174902,#174903,#174904),(#174905,#174906,#174907,#174908,#174909,#174910,
#174911,#174912,#174913),(#174914,#174915,#174916,#174917,#174918,#174919,
#174920,#174921,#174922),(#174923,#174924,#174925,#174926,#174927,#174928,
#174929,#174930,#174931),(#174932,#174933,#174934,#174935,#174936,#174937,
#174938,#174939,#174940),(#174941,#174942,#174943,#174944,#174945,#174946,
#174947,#174948,#174949),(#174950,#174951,#174952,#174953,#174954,#174955,
#174956,#174957,#174958),(#174959,#174960,#174961,#174962,#174963,#174964,
#174965,#174966,#174967),(#174968,#174969,#174970,#174971,#174972,#174973,
#174974,#174975,#174976),(#174977,#174978,#174979,#174980,#174981,#174982,
#174983,#174984,#174985),(#174986,#174987,#174988,#174989,#174990,#174991,
#174992,#174993,#174994),(#174995,#174996,#174997,#174998,#174999,#175000,
#175001,#175002,#175003),(#175004,#175005,#175006,#175007,#175008,#175009,
#175010,#175011,#175012),(#175013,#175014,#175015,#175016,#175017,#175018,
#175019,#175020,#175021),(#175022,#175023,#175024,#175025,#175026,#175027,
#175028,#175029,#175030),(#175031,#175032,#175033,#175034,#175035,#175036,
#175037,#175038,#175039),(#175040,#175041,#175042,#175043,#175044,#175045,
#175046,#175047,#175048),(#175049,#175050,#175051,#175052,#175053,#175054,
#175055,#175056,#175057),(#175058,#175059,#175060,#175061,#175062,#175063,
#175064,#175065,#175066),(#175067,#175068,#175069,#175070,#175071,#175072,
#175073,#175074,#175075),(#175076,#175077,#175078,#175079,#175080,#175081,
#175082,#175083,#175084),(#175085,#175086,#175087,#175088,#175089,#175090,
#175091,#175092,#175093),(#175094,#175095,#175096,#175097,#175098,#175099,
#175100,#175101,#175102),(#175103,#175104,#175105,#175106,#175107,#175108,
#175109,#175110,#175111),(#175112,#175113,#175114,#175115,#175116,#175117,
#175118,#175119,#175120),(#175121,#175122,#175123,#175124,#175125,#175126,
#175127,#175128,#175129),(#175130,#175131,#175132,#175133,#175134,#175135,
#175136,#175137,#175138),(#175139,#175140,#175141,#175142,#175143,#175144,
#175145,#175146,#175147),(#175148,#175149,#175150,#175151,#175152,#175153,
#175154,#175155,#175156),(#175157,#175158,#175159,#175160,#175161,#175162,
#175163,#175164,#175165),(#175166,#175167,#175168,#175169,#175170,#175171,
#175172,#175173,#175174),(#175175,#175176,#175177,#175178,#175179,#175180,
#175181,#175182,#175183),(#175184,#175185,#175186,#175187,#175188,#175189,
#175190,#175191,#175192),(#175193,#175194,#175195,#175196,#175197,#175198,
#175199,#175200,#175201),(#175202,#175203,#175204,#175205,#175206,#175207,
#175208,#175209,#175210),(#175211,#175212,#175213,#175214,#175215,#175216,
#175217,#175218,#175219),(#175220,#175221,#175222,#175223,#175224,#175225,
#175226,#175227,#175228),(#175229,#175230,#175231,#175232,#175233,#175234,
#175235,#175236,#175237),(#175238,#175239,#175240,#175241,#175242,#175243,
#175244,#175245,#175246),(#175247,#175248,#175249,#175250,#175251,#175252,
#175253,#175254,#175255),(#175256,#175257,#175258,#175259,#175260,#175261,
#175262,#175263,#175264),(#175265,#175266,#175267,#175268,#175269,#175270,
#175271,#175272,#175273),(#175274,#175275,#175276,#175277,#175278,#175279,
#175280,#175281,#175282),(#175283,#175284,#175285,#175286,#175287,#175288,
#175289,#175290,#175291),(#175292,#175293,#175294,#175295,#175296,#175297,
#175298,#175299,#175300),(#175301,#175302,#175303,#175304,#175305,#175306,
#175307,#175308,#175309),(#175310,#175311,#175312,#175313,#175314,#175315,
#175316,#175317,#175318),(#175319,#175320,#175321,#175322,#175323,#175324,
#175325,#175326,#175327),(#175328,#175329,#175330,#175331,#175332,#175333,
#175334,#175335,#175336),(#175337,#175338,#175339,#175340,#175341,#175342,
#175343,#175344,#175345),(#175346,#175347,#175348,#175349,#175350,#175351,
#175352,#175353,#175354),(#175355,#175356,#175357,#175358,#175359,#175360,
#175361,#175362,#175363),(#175364,#175365,#175366,#175367,#175368,#175369,
#175370,#175371,#175372),(#175373,#175374,#175375,#175376,#175377,#175378,
#175379,#175380,#175381),(#175382,#175383,#175384,#175385,#175386,#175387,
#175388,#175389,#175390),(#175391,#175392,#175393,#175394,#175395,#175396,
#175397,#175398,#175399),(#175400,#175401,#175402,#175403,#175404,#175405,
#175406,#175407,#175408),(#175409,#175410,#175411,#175412,#175413,#175414,
#175415,#175416,#175417),(#175418,#175419,#175420,#175421,#175422,#175423,
#175424,#175425,#175426),(#175427,#175428,#175429,#175430,#175431,#175432,
#175433,#175434,#175435),(#175436,#175437,#175438,#175439,#175440,#175441,
#175442,#175443,#175444),(#175445,#175446,#175447,#175448,#175449,#175450,
#175451,#175452,#175453),(#175454,#175455,#175456,#175457,#175458,#175459,
#175460,#175461,#175462),(#175463,#175464,#175465,#175466,#175467,#175468,
#175469,#175470,#175471),(#175472,#175473,#175474,#175475,#175476,#175477,
#175478,#175479,#175480),(#175481,#175482,#175483,#175484,#175485,#175486,
#175487,#175488,#175489),(#175490,#175491,#175492,#175493,#175494,#175495,
#175496,#175497,#175498),(#175499,#175500,#175501,#175502,#175503,#175504,
#175505,#175506,#175507),(#175508,#175509,#175510,#175511,#175512,#175513,
#175514,#175515,#175516),(#175517,#175518,#175519,#175520,#175521,#175522,
#175523,#175524,#175525),(#175526,#175527,#175528,#175529,#175530,#175531,
#175532,#175533,#175534),(#175535,#175536,#175537,#175538,#175539,#175540,
#175541,#175542,#175543),(#175544,#175545,#175546,#175547,#175548,#175549,
#175550,#175551,#175552),(#175553,#175554,#175555,#175556,#175557,#175558,
#175559,#175560,#175561),(#175562,#175563,#175564,#175565,#175566,#175567,
#175568,#175569,#175570),(#175571,#175572,#175573,#175574,#175575,#175576,
#175577,#175578,#175579),(#175580,#175581,#175582,#175583,#175584,#175585,
#175586,#175587,#175588),(#175589,#175590,#175591,#175592,#175593,#175594,
#175595,#175596,#175597),(#175598,#175599,#175600,#175601,#175602,#175603,
#175604,#175605,#175606),(#175607,#175608,#175609,#175610,#175611,#175612,
#175613,#175614,#175615),(#175616,#175617,#175618,#175619,#175620,#175621,
#175622,#175623,#175624),(#175625,#175626,#175627,#175628,#175629,#175630,
#175631,#175632,#175633),(#175634,#175635,#175636,#175637,#175638,#175639,
#175640,#175641,#175642),(#175643,#175644,#175645,#175646,#175647,#175648,
#175649,#175650,#175651),(#175652,#175653,#175654,#175655,#175656,#175657,
#175658,#175659,#175660),(#175661,#175662,#175663,#175664,#175665,#175666,
#175667,#175668,#175669),(#175670,#175671,#175672,#175673,#175674,#175675,
#175676,#175677,#175678),(#175679,#175680,#175681,#175682,#175683,#175684,
#175685,#175686,#175687),(#175688,#175689,#175690,#175691,#175692,#175693,
#175694,#175695,#175696),(#175697,#175698,#175699,#175700,#175701,#175702,
#175703,#175704,#175705),(#175706,#175707,#175708,#175709,#175710,#175711,
#175712,#175713,#175714),(#175715,#175716,#175717,#175718,#175719,#175720,
#175721,#175722,#175723),(#175724,#175725,#175726,#175727,#175728,#175729,
#175730,#175731,#175732),(#175733,#175734,#175735,#175736,#175737,#175738,
#175739,#175740,#175741),(#175742,#175743,#175744,#175745,#175746,#175747,
#175748,#175749,#175750),(#175751,#175752,#175753,#175754,#175755,#175756,
#175757,#175758,#175759),(#175760,#175761,#175762,#175763,#175764,#175765,
#175766,#175767,#175768),(#175769,#175770,#175771,#175772,#175773,#175774,
#175775,#175776,#175777),(#175778,#175779,#175780,#175781,#175782,#175783,
#175784,#175785,#175786),(#175787,#175788,#175789,#175790,#175791,#175792,
#175793,#175794,#175795),(#175796,#175797,#175798,#175799,#175800,#175801,
#175802,#175803,#175804),(#175805,#175806,#175807,#175808,#175809,#175810,
#175811,#175812,#175813),(#175814,#175815,#175816,#175817,#175818,#175819,
#175820,#175821,#175822),(#175823,#175824,#175825,#175826,#175827,#175828,
#175829,#175830,#175831),(#175832,#175833,#175834,#175835,#175836,#175837,
#175838,#175839,#175840),(#175841,#175842,#175843,#175844,#175845,#175846,
#175847,#175848,#175849),(#175850,#175851,#175852,#175853,#175854,#175855,
#175856,#175857,#175858),(#175859,#175860,#175861,#175862,#175863,#175864,
#175865,#175866,#175867),(#175868,#175869,#175870,#175871,#175872,#175873,
#175874,#175875,#175876),(#175877,#175878,#175879,#175880,#175881,#175882,
#175883,#175884,#175885),(#175886,#175887,#175888,#175889,#175890,#175891,
#175892,#175893,#175894),(#175895,#175896,#175897,#175898,#175899,#175900,
#175901,#175902,#175903),(#175904,#175905,#175906,#175907,#175908,#175909,
#175910,#175911,#175912),(#175913,#175914,#175915,#175916,#175917,#175918,
#175919,#175920,#175921),(#175922,#175923,#175924,#175925,#175926,#175927,
#175928,#175929,#175930),(#175931,#175932,#175933,#175934,#175935,#175936,
#175937,#175938,#175939),(#175940,#175941,#175942,#175943,#175944,#175945,
#175946,#175947,#175948),(#175949,#175950,#175951,#175952,#175953,#175954,
#175955,#175956,#175957),(#175958,#175959,#175960,#175961,#175962,#175963,
#175964,#175965,#175966),(#175967,#175968,#175969,#175970,#175971,#175972,
#175973,#175974,#175975),(#175976,#175977,#175978,#175979,#175980,#175981,
#175982,#175983,#175984),(#175985,#175986,#175987,#175988,#175989,#175990,
#175991,#175992,#175993),(#175994,#175995,#175996,#175997,#175998,#175999,
#176000,#176001,#176002),(#176003,#176004,#176005,#176006,#176007,#176008,
#176009,#176010,#176011),(#176012,#176013,#176014,#176015,#176016,#176017,
#176018,#176019,#176020),(#176021,#176022,#176023,#176024,#176025,#176026,
#176027,#176028,#176029),(#176030,#176031,#176032,#176033,#176034,#176035,
#176036,#176037,#176038),(#176039,#176040,#176041,#176042,#176043,#176044,
#176045,#176046,#176047),(#176048,#176049,#176050,#176051,#176052,#176053,
#176054,#176055,#176056),(#176057,#176058,#176059,#176060,#176061,#176062,
#176063,#176064,#176065),(#176066,#176067,#176068,#176069,#176070,#176071,
#176072,#176073,#176074),(#176075,#176076,#176077,#176078,#176079,#176080,
#176081,#176082,#176083),(#176084,#176085,#176086,#176087,#176088,#176089,
#176090,#176091,#176092),(#176093,#176094,#176095,#176096,#176097,#176098,
#176099,#176100,#176101),(#176102,#176103,#176104,#176105,#176106,#176107,
#176108,#176109,#176110),(#176111,#176112,#176113,#176114,#176115,#176116,
#176117,#176118,#176119),(#176120,#176121,#176122,#176123,#176124,#176125,
#176126,#176127,#176128),(#176129,#176130,#176131,#176132,#176133,#176134,
#176135,#176136,#176137),(#176138,#176139,#176140,#176141,#176142,#176143,
#176144,#176145,#176146),(#176147,#176148,#176149,#176150,#176151,#176152,
#176153,#176154,#176155),(#176156,#176157,#176158,#176159,#176160,#176161,
#176162,#176163,#176164),(#176165,#176166,#176167,#176168,#176169,#176170,
#176171,#176172,#176173),(#176174,#176175,#176176,#176177,#176178,#176179,
#176180,#176181,#176182),(#176183,#176184,#176185,#176186,#176187,#176188,
#176189,#176190,#176191),(#176192,#176193,#176194,#176195,#176196,#176197,
#176198,#176199,#176200),(#176201,#176202,#176203,#176204,#176205,#176206,
#176207,#176208,#176209),(#176210,#176211,#176212,#176213,#176214,#176215,
#176216,#176217,#176218),(#176219,#176220,#176221,#176222,#176223,#176224,
#176225,#176226,#176227),(#176228,#176229,#176230,#176231,#176232,#176233,
#176234,#176235,#176236),(#176237,#176238,#176239,#176240,#176241,#176242,
#176243,#176244,#176245),(#176246,#176247,#176248,#176249,#176250,#176251,
#176252,#176253,#176254),(#176255,#176256,#176257,#176258,#176259,#176260,
#176261,#176262,#176263),(#176264,#176265,#176266,#176267,#176268,#176269,
#176270,#176271,#176272),(#176273,#176274,#176275,#176276,#176277,#176278,
#176279,#176280,#176281),(#176282,#176283,#176284,#176285,#176286,#176287,
#176288,#176289,#176290),(#176291,#176292,#176293,#176294,#176295,#176296,
#176297,#176298,#176299),(#176300,#176301,#176302,#176303,#176304,#176305,
#176306,#176307,#176308),(#176309,#176310,#176311,#176312,#176313,#176314,
#176315,#176316,#176317),(#176318,#176319,#176320,#176321,#176322,#176323,
#176324,#176325,#176326),(#176327,#176328,#176329,#176330,#176331,#176332,
#176333,#176334,#176335),(#176336,#176337,#176338,#176339,#176340,#176341,
#176342,#176343,#176344),(#176345,#176346,#176347,#176348,#176349,#176350,
#176351,#176352,#176353),(#176354,#176355,#176356,#176357,#176358,#176359,
#176360,#176361,#176362),(#176363,#176364,#176365,#176366,#176367,#176368,
#176369,#176370,#176371),(#176372,#176373,#176374,#176375,#176376,#176377,
#176378,#176379,#176380),(#176381,#176382,#176383,#176384,#176385,#176386,
#176387,#176388,#176389),(#176390,#176391,#176392,#176393,#176394,#176395,
#176396,#176397,#176398),(#176399,#176400,#176401,#176402,#176403,#176404,
#176405,#176406,#176407),(#176408,#176409,#176410,#176411,#176412,#176413,
#176414,#176415,#176416),(#176417,#176418,#176419,#176420,#176421,#176422,
#176423,#176424,#176425),(#176426,#176427,#176428,#176429,#176430,#176431,
#176432,#176433,#176434),(#176435,#176436,#176437,#176438,#176439,#176440,
#176441,#176442,#176443),(#176444,#176445,#176446,#176447,#176448,#176449,
#176450,#176451,#176452),(#176453,#176454,#176455,#176456,#176457,#176458,
#176459,#176460,#176461),(#176462,#176463,#176464,#176465,#176466,#176467,
#176468,#176469,#176470),(#176471,#176472,#176473,#176474,#176475,#176476,
#176477,#176478,#176479),(#176480,#176481,#176482,#176483,#176484,#176485,
#176486,#176487,#176488),(#176489,#176490,#176491,#176492,#176493,#176494,
#176495,#176496,#176497),(#176498,#176499,#176500,#176501,#176502,#176503,
#176504,#176505,#176506),(#176507,#176508,#176509,#176510,#176511,#176512,
#176513,#176514,#176515),(#176516,#176517,#176518,#176519,#176520,#176521,
#176522,#176523,#176524),(#176525,#176526,#176527,#176528,#176529,#176530,
#176531,#176532,#176533),(#176534,#176535,#176536,#176537,#176538,#176539,
#176540,#176541,#176542),(#176543,#176544,#176545,#176546,#176547,#176548,
#176549,#176550,#176551),(#176552,#176553,#176554,#176555,#176556,#176557,
#176558,#176559,#176560),(#176561,#176562,#176563,#176564,#176565,#176566,
#176567,#176568,#176569),(#176570,#176571,#176572,#176573,#176574,#176575,
#176576,#176577,#176578),(#176579,#176580,#176581,#176582,#176583,#176584,
#176585,#176586,#176587),(#176588,#176589,#176590,#176591,#176592,#176593,
#176594,#176595,#176596),(#176597,#176598,#176599,#176600,#176601,#176602,
#176603,#176604,#176605),(#176606,#176607,#176608,#176609,#176610,#176611,
#176612,#176613,#176614),(#176615,#176616,#176617,#176618,#176619,#176620,
#176621,#176622,#176623),(#176624,#176625,#176626,#176627,#176628,#176629,
#176630,#176631,#176632),(#176633,#176634,#176635,#176636,#176637,#176638,
#176639,#176640,#176641),(#176642,#176643,#176644,#176645,#176646,#176647,
#176648,#176649,#176650),(#176651,#176652,#176653,#176654,#176655,#176656,
#176657,#176658,#176659),(#176660,#176661,#176662,#176663,#176664,#176665,
#176666,#176667,#176668),(#176669,#176670,#176671,#176672,#176673,#176674,
#176675,#176676,#176677),(#176678,#176679,#176680,#176681,#176682,#176683,
#176684,#176685,#176686),(#176687,#176688,#176689,#176690,#176691,#176692,
#176693,#176694,#176695),(#176696,#176697,#176698,#176699,#176700,#176701,
#176702,#176703,#176704),(#176705,#176706,#176707,#176708,#176709,#176710,
#176711,#176712,#176713),(#176714,#176715,#176716,#176717,#176718,#176719,
#176720,#176721,#176722),(#176723,#176724,#176725,#176726,#176727,#176728,
#176729,#176730,#176731),(#176732,#176733,#176734,#176735,#176736,#176737,
#176738,#176739,#176740),(#176741,#176742,#176743,#176744,#176745,#176746,
#176747,#176748,#176749),(#176750,#176751,#176752,#176753,#176754,#176755,
#176756,#176757,#176758),(#176759,#176760,#176761,#176762,#176763,#176764,
#176765,#176766,#176767),(#176768,#176769,#176770,#176771,#176772,#176773,
#176774,#176775,#176776),(#176777,#176778,#176779,#176780,#176781,#176782,
#176783,#176784,#176785),(#176786,#176787,#176788,#176789,#176790,#176791,
#176792,#176793,#176794),(#176795,#176796,#176797,#176798,#176799,#176800,
#176801,#176802,#176803),(#176804,#176805,#176806,#176807,#176808,#176809,
#176810,#176811,#176812),(#176813,#176814,#176815,#176816,#176817,#176818,
#176819,#176820,#176821),(#176822,#176823,#176824,#176825,#176826,#176827,
#176828,#176829,#176830),(#176831,#176832,#176833,#176834,#176835,#176836,
#176837,#176838,#176839),(#176840,#176841,#176842,#176843,#176844,#176845,
#176846,#176847,#176848),(#176849,#176850,#176851,#176852,#176853,#176854,
#176855,#176856,#176857),(#176858,#176859,#176860,#176861,#176862,#176863,
#176864,#176865,#176866),(#176867,#176868,#176869,#176870,#176871,#176872,
#176873,#176874,#176875),(#176876,#176877,#176878,#176879,#176880,#176881,
#176882,#176883,#176884),(#176885,#176886,#176887,#176888,#176889,#176890,
#176891,#176892,#176893),(#176894,#176895,#176896,#176897,#176898,#176899,
#176900,#176901,#176902),(#176903,#176904,#176905,#176906,#176907,#176908,
#176909,#176910,#176911),(#176912,#176913,#176914,#176915,#176916,#176917,
#176918,#176919,#176920),(#176921,#176922,#176923,#176924,#176925,#176926,
#176927,#176928,#176929),(#176930,#176931,#176932,#176933,#176934,#176935,
#176936,#176937,#176938),(#176939,#176940,#176941,#176942,#176943,#176944,
#176945,#176946,#176947),(#176948,#176949,#176950,#176951,#176952,#176953,
#176954,#176955,#176956),(#176957,#176958,#176959,#176960,#176961,#176962,
#176963,#176964,#176965),(#176966,#176967,#176968,#176969,#176970,#176971,
#176972,#176973,#176974),(#176975,#176976,#176977,#176978,#176979,#176980,
#176981,#176982,#176983),(#176984,#176985,#176986,#176987,#176988,#176989,
#176990,#176991,#176992),(#176993,#176994,#176995,#176996,#176997,#176998,
#176999,#177000,#177001),(#177002,#177003,#177004,#177005,#177006,#177007,
#177008,#177009,#177010),(#177011,#177012,#177013,#177014,#177015,#177016,
#177017,#177018,#177019),(#177020,#177021,#177022,#177023,#177024,#177025,
#177026,#177027,#177028),(#177029,#177030,#177031,#177032,#177033,#177034,
#177035,#177036,#177037),(#177038,#177039,#177040,#177041,#177042,#177043,
#177044,#177045,#177046),(#177047,#177048,#177049,#177050,#177051,#177052,
#177053,#177054,#177055),(#177056,#177057,#177058,#177059,#177060,#177061,
#177062,#177063,#177064),(#177065,#177066,#177067,#177068,#177069,#177070,
#177071,#177072,#177073),(#177074,#177075,#177076,#177077,#177078,#177079,
#177080,#177081,#177082),(#177083,#177084,#177085,#177086,#177087,#177088,
#177089,#177090,#177091),(#177092,#177093,#177094,#177095,#177096,#177097,
#177098,#177099,#177100),(#177101,#177102,#177103,#177104,#177105,#177106,
#177107,#177108,#177109),(#177110,#177111,#177112,#177113,#177114,#177115,
#177116,#177117,#177118),(#177119,#177120,#177121,#177122,#177123,#177124,
#177125,#177126,#177127),(#177128,#177129,#177130,#177131,#177132,#177133,
#177134,#177135,#177136),(#177137,#177138,#177139,#177140,#177141,#177142,
#177143,#177144,#177145),(#177146,#177147,#177148,#177149,#177150,#177151,
#177152,#177153,#177154),(#177155,#177156,#177157,#177158,#177159,#177160,
#177161,#177162,#177163),(#177164,#177165,#177166,#177167,#177168,#177169,
#177170,#177171,#177172),(#177173,#177174,#177175,#177176,#177177,#177178,
#177179,#177180,#177181),(#177182,#177183,#177184,#177185,#177186,#177187,
#177188,#177189,#177190),(#177191,#177192,#177193,#177194,#177195,#177196,
#177197,#177198,#177199),(#177200,#177201,#177202,#177203,#177204,#177205,
#177206,#177207,#177208),(#177209,#177210,#177211,#177212,#177213,#177214,
#177215,#177216,#177217),(#177218,#177219,#177220,#177221,#177222,#177223,
#177224,#177225,#177226),(#177227,#177228,#177229,#177230,#177231,#177232,
#177233,#177234,#177235),(#177236,#177237,#177238,#177239,#177240,#177241,
#177242,#177243,#177244),(#177245,#177246,#177247,#177248,#177249,#177250,
#177251,#177252,#177253),(#177254,#177255,#177256,#177257,#177258,#177259,
#177260,#177261,#177262),(#177263,#177264,#177265,#177266,#177267,#177268,
#177269,#177270,#177271),(#177272,#177273,#177274,#177275,#177276,#177277,
#177278,#177279,#177280),(#177281,#177282,#177283,#177284,#177285,#177286,
#177287,#177288,#177289),(#177290,#177291,#177292,#177293,#177294,#177295,
#177296,#177297,#177298),(#177299,#177300,#177301,#177302,#177303,#177304,
#177305,#177306,#177307),(#177308,#177309,#177310,#177311,#177312,#177313,
#177314,#177315,#177316),(#177317,#177318,#177319,#177320,#177321,#177322,
#177323,#177324,#177325),(#177326,#177327,#177328,#177329,#177330,#177331,
#177332,#177333,#177334),(#177335,#177336,#177337,#177338,#177339,#177340,
#177341,#177342,#177343),(#177344,#177345,#177346,#177347,#177348,#177349,
#177350,#177351,#177352),(#177353,#177354,#177355,#177356,#177357,#177358,
#177359,#177360,#177361),(#177362,#177363,#177364,#177365,#177366,#177367,
#177368,#177369,#177370),(#177371,#177372,#177373,#177374,#177375,#177376,
#177377,#177378,#177379),(#177380,#177381,#177382,#177383,#177384,#177385,
#177386,#177387,#177388),(#177389,#177390,#177391,#177392,#177393,#177394,
#177395,#177396,#177397),(#177398,#177399,#177400,#177401,#177402,#177403,
#177404,#177405,#177406),(#177407,#177408,#177409,#177410,#177411,#177412,
#177413,#177414,#177415),(#177416,#177417,#177418,#177419,#177420,#177421,
#177422,#177423,#177424),(#177425,#177426,#177427,#177428,#177429,#177430,
#177431,#177432,#177433),(#177434,#177435,#177436,#177437,#177438,#177439,
#177440,#177441,#177442),(#177443,#177444,#177445,#177446,#177447,#177448,
#177449,#177450,#177451),(#177452,#177453,#177454,#177455,#177456,#177457,
#177458,#177459,#177460),(#177461,#177462,#177463,#177464,#177465,#177466,
#177467,#177468,#177469),(#177470,#177471,#177472,#177473,#177474,#177475,
#177476,#177477,#177478),(#177479,#177480,#177481,#177482,#177483,#177484,
#177485,#177486,#177487),(#177488,#177489,#177490,#177491,#177492,#177493,
#177494,#177495,#177496),(#177497,#177498,#177499,#177500,#177501,#177502,
#177503,#177504,#177505),(#177506,#177507,#177508,#177509,#177510,#177511,
#177512,#177513,#177514),(#177515,#177516,#177517,#177518,#177519,#177520,
#177521,#177522,#177523),(#177524,#177525,#177526,#177527,#177528,#177529,
#177530,#177531,#177532),(#177533,#177534,#177535,#177536,#177537,#177538,
#177539,#177540,#177541),(#177542,#177543,#177544,#177545,#177546,#177547,
#177548,#177549,#177550),(#177551,#177552,#177553,#177554,#177555,#177556,
#177557,#177558,#177559),(#177560,#177561,#177562,#177563,#177564,#177565,
#177566,#177567,#177568),(#177569,#177570,#177571,#177572,#177573,#177574,
#177575,#177576,#177577),(#177578,#177579,#177580,#177581,#177582,#177583,
#177584,#177585,#177586),(#177587,#177588,#177589,#177590,#177591,#177592,
#177593,#177594,#177595),(#177596,#177597,#177598,#177599,#177600,#177601,
#177602,#177603,#177604),(#177605,#177606,#177607,#177608,#177609,#177610,
#177611,#177612,#177613),(#177614,#177615,#177616,#177617,#177618,#177619,
#177620,#177621,#177622),(#177623,#177624,#177625,#177626,#177627,#177628,
#177629,#177630,#177631),(#177632,#177633,#177634,#177635,#177636,#177637,
#177638,#177639,#177640),(#177641,#177642,#177643,#177644,#177645,#177646,
#177647,#177648,#177649),(#177650,#177651,#177652,#177653,#177654,#177655,
#177656,#177657,#177658),(#177659,#177660,#177661,#177662,#177663,#177664,
#177665,#177666,#177667),(#177668,#177669,#177670,#177671,#177672,#177673,
#177674,#177675,#177676),(#177677,#177678,#177679,#177680,#177681,#177682,
#177683,#177684,#177685),(#177686,#177687,#177688,#177689,#177690,#177691,
#177692,#177693,#177694),(#177695,#177696,#177697,#177698,#177699,#177700,
#177701,#177702,#177703),(#177704,#177705,#177706,#177707,#177708,#177709,
#177710,#177711,#177712),(#177713,#177714,#177715,#177716,#177717,#177718,
#177719,#177720,#177721),(#177722,#177723,#177724,#177725,#177726,#177727,
#177728,#177729,#177730),(#177731,#177732,#177733,#177734,#177735,#177736,
#177737,#177738,#177739),(#177740,#177741,#177742,#177743,#177744,#177745,
#177746,#177747,#177748),(#177749,#177750,#177751,#177752,#177753,#177754,
#177755,#177756,#177757),(#177758,#177759,#177760,#177761,#177762,#177763,
#177764,#177765,#177766),(#177767,#177768,#177769,#177770,#177771,#177772,
#177773,#177774,#177775),(#177776,#177777,#177778,#177779,#177780,#177781,
#177782,#177783,#177784),(#177785,#177786,#177787,#177788,#177789,#177790,
#177791,#177792,#177793),(#177794,#177795,#177796,#177797,#177798,#177799,
#177800,#177801,#177802),(#177803,#177804,#177805,#177806,#177807,#177808,
#177809,#177810,#177811),(#177812,#177813,#177814,#177815,#177816,#177817,
#177818,#177819,#177820),(#177821,#177822,#177823,#177824,#177825,#177826,
#177827,#177828,#177829),(#177830,#177831,#177832,#177833,#177834,#177835,
#177836,#177837,#177838),(#177839,#177840,#177841,#177842,#177843,#177844,
#177845,#177846,#177847),(#177848,#177849,#177850,#177851,#177852,#177853,
#177854,#177855,#177856),(#177857,#177858,#177859,#177860,#177861,#177862,
#177863,#177864,#177865),(#177866,#177867,#177868,#177869,#177870,#177871,
#177872,#177873,#177874),(#177875,#177876,#177877,#177878,#177879,#177880,
#177881,#177882,#177883),(#177884,#177885,#177886,#177887,#177888,#177889,
#177890,#177891,#177892),(#177893,#177894,#177895,#177896,#177897,#177898,
#177899,#177900,#177901),(#177902,#177903,#177904,#177905,#177906,#177907,
#177908,#177909,#177910),(#177911,#177912,#177913,#177914,#177915,#177916,
#177917,#177918,#177919),(#177920,#177921,#177922,#177923,#177924,#177925,
#177926,#177927,#177928),(#177929,#177930,#177931,#177932,#177933,#177934,
#177935,#177936,#177937),(#177938,#177939,#177940,#177941,#177942,#177943,
#177944,#177945,#177946),(#177947,#177948,#177949,#177950,#177951,#177952,
#177953,#177954,#177955),(#177956,#177957,#177958,#177959,#177960,#177961,
#177962,#177963,#177964),(#177965,#177966,#177967,#177968,#177969,#177970,
#177971,#177972,#177973),(#177974,#177975,#177976,#177977,#177978,#177979,
#177980,#177981,#177982),(#177983,#177984,#177985,#177986,#177987,#177988,
#177989,#177990,#177991),(#177992,#177993,#177994,#177995,#177996,#177997,
#177998,#177999,#178000),(#178001,#178002,#178003,#178004,#178005,#178006,
#178007,#178008,#178009),(#178010,#178011,#178012,#178013,#178014,#178015,
#178016,#178017,#178018),(#178019,#178020,#178021,#178022,#178023,#178024,
#178025,#178026,#178027),(#178028,#178029,#178030,#178031,#178032,#178033,
#178034,#178035,#178036),(#178037,#178038,#178039,#178040,#178041,#178042,
#178043,#178044,#178045),(#178046,#178047,#178048,#178049,#178050,#178051,
#178052,#178053,#178054),(#178055,#178056,#178057,#178058,#178059,#178060,
#178061,#178062,#178063),(#178064,#178065,#178066,#178067,#178068,#178069,
#178070,#178071,#178072),(#178073,#178074,#178075,#178076,#178077,#178078,
#178079,#178080,#178081),(#178082,#178083,#178084,#178085,#178086,#178087,
#178088,#178089,#178090),(#178091,#178092,#178093,#178094,#178095,#178096,
#178097,#178098,#178099),(#178100,#178101,#178102,#178103,#178104,#178105,
#178106,#178107,#178108),(#178109,#178110,#178111,#178112,#178113,#178114,
#178115,#178116,#178117),(#178118,#178119,#178120,#178121,#178122,#178123,
#178124,#178125,#178126),(#178127,#178128,#178129,#178130,#178131,#178132,
#178133,#178134,#178135),(#178136,#178137,#178138,#178139,#178140,#178141,
#178142,#178143,#178144),(#178145,#178146,#178147,#178148,#178149,#178150,
#178151,#178152,#178153),(#178154,#178155,#178156,#178157,#178158,#178159,
#178160,#178161,#178162),(#178163,#178164,#178165,#178166,#178167,#178168,
#178169,#178170,#178171),(#178172,#178173,#178174,#178175,#178176,#178177,
#178178,#178179,#178180),(#178181,#178182,#178183,#178184,#178185,#178186,
#178187,#178188,#178189),(#178190,#178191,#178192,#178193,#178194,#178195,
#178196,#178197,#178198),(#178199,#178200,#178201,#178202,#178203,#178204,
#178205,#178206,#178207),(#178208,#178209,#178210,#178211,#178212,#178213,
#178214,#178215,#178216),(#178217,#178218,#178219,#178220,#178221,#178222,
#178223,#178224,#178225),(#178226,#178227,#178228,#178229,#178230,#178231,
#178232,#178233,#178234),(#178235,#178236,#178237,#178238,#178239,#178240,
#178241,#178242,#178243),(#178244,#178245,#178246,#178247,#178248,#178249,
#178250,#178251,#178252),(#178253,#178254,#178255,#178256,#178257,#178258,
#178259,#178260,#178261),(#178262,#178263,#178264,#178265,#178266,#178267,
#178268,#178269,#178270),(#178271,#178272,#178273,#178274,#178275,#178276,
#178277,#178278,#178279),(#178280,#178281,#178282,#178283,#178284,#178285,
#178286,#178287,#178288),(#178289,#178290,#178291,#178292,#178293,#178294,
#178295,#178296,#178297),(#178298,#178299,#178300,#178301,#178302,#178303,
#178304,#178305,#178306),(#178307,#178308,#178309,#178310,#178311,#178312,
#178313,#178314,#178315),(#178316,#178317,#178318,#178319,#178320,#178321,
#178322,#178323,#178324),(#178325,#178326,#178327,#178328,#178329,#178330,
#178331,#178332,#178333),(#178334,#178335,#178336,#178337,#178338,#178339,
#178340,#178341,#178342),(#178343,#178344,#178345,#178346,#178347,#178348,
#178349,#178350,#178351),(#178352,#178353,#178354,#178355,#178356,#178357,
#178358,#178359,#178360),(#178361,#178362,#178363,#178364,#178365,#178366,
#178367,#178368,#178369),(#178370,#178371,#178372,#178373,#178374,#178375,
#178376,#178377,#178378),(#178379,#178380,#178381,#178382,#178383,#178384,
#178385,#178386,#178387),(#178388,#178389,#178390,#178391,#178392,#178393,
#178394,#178395,#178396),(#178397,#178398,#178399,#178400,#178401,#178402,
#178403,#178404,#178405),(#178406,#178407,#178408,#178409,#178410,#178411,
#178412,#178413,#178414),(#178415,#178416,#178417,#178418,#178419,#178420,
#178421,#178422,#178423),(#178424,#178425,#178426,#178427,#178428,#178429,
#178430,#178431,#178432),(#178433,#178434,#178435,#178436,#178437,#178438,
#178439,#178440,#178441),(#178442,#178443,#178444,#178445,#178446,#178447,
#178448,#178449,#178450),(#178451,#178452,#178453,#178454,#178455,#178456,
#178457,#178458,#178459),(#178460,#178461,#178462,#178463,#178464,#178465,
#178466,#178467,#178468),(#178469,#178470,#178471,#178472,#178473,#178474,
#178475,#178476,#178477),(#178478,#178479,#178480,#178481,#178482,#178483,
#178484,#178485,#178486),(#178487,#178488,#178489,#178490,#178491,#178492,
#178493,#178494,#178495),(#178496,#178497,#178498,#178499,#178500,#178501,
#178502,#178503,#178504),(#178505,#178506,#178507,#178508,#178509,#178510,
#178511,#178512,#178513),(#178514,#178515,#178516,#178517,#178518,#178519,
#178520,#178521,#178522),(#178523,#178524,#178525,#178526,#178527,#178528,
#178529,#178530,#178531),(#178532,#178533,#178534,#178535,#178536,#178537,
#178538,#178539,#178540),(#178541,#178542,#178543,#178544,#178545,#178546,
#178547,#178548,#178549),(#178550,#178551,#178552,#178553,#178554,#178555,
#178556,#178557,#178558),(#178559,#178560,#178561,#178562,#178563,#178564,
#178565,#178566,#178567),(#178568,#178569,#178570,#178571,#178572,#178573,
#178574,#178575,#178576),(#178577,#178578,#178579,#178580,#178581,#178582,
#178583,#178584,#178585),(#178586,#178587,#178588,#178589,#178590,#178591,
#178592,#178593,#178594),(#178595,#178596,#178597,#178598,#178599,#178600,
#178601,#178602,#178603),(#178604,#178605,#178606,#178607,#178608,#178609,
#178610,#178611,#178612),(#178613,#178614,#178615,#178616,#178617,#178618,
#178619,#178620,#178621),(#178622,#178623,#178624,#178625,#178626,#178627,
#178628,#178629,#178630),(#178631,#178632,#178633,#178634,#178635,#178636,
#178637,#178638,#178639),(#178640,#178641,#178642,#178643,#178644,#178645,
#178646,#178647,#178648),(#178649,#178650,#178651,#178652,#178653,#178654,
#178655,#178656,#178657),(#178658,#178659,#178660,#178661,#178662,#178663,
#178664,#178665,#178666),(#178667,#178668,#178669,#178670,#178671,#178672,
#178673,#178674,#178675),(#178676,#178677,#178678,#178679,#178680,#178681,
#178682,#178683,#178684),(#178685,#178686,#178687,#178688,#178689,#178690,
#178691,#178692,#178693),(#178694,#178695,#178696,#178697,#178698,#178699,
#178700,#178701,#178702),(#178703,#178704,#178705,#178706,#178707,#178708,
#178709,#178710,#178711),(#178712,#178713,#178714,#178715,#178716,#178717,
#178718,#178719,#178720),(#178721,#178722,#178723,#178724,#178725,#178726,
#178727,#178728,#178729),(#178730,#178731,#178732,#178733,#178734,#178735,
#178736,#178737,#178738),(#178739,#178740,#178741,#178742,#178743,#178744,
#178745,#178746,#178747),(#178748,#178749,#178750,#178751,#178752,#178753,
#178754,#178755,#178756),(#178757,#178758,#178759,#178760,#178761,#178762,
#178763,#178764,#178765),(#178766,#178767,#178768,#178769,#178770,#178771,
#178772,#178773,#178774),(#178775,#178776,#178777,#178778,#178779,#178780,
#178781,#178782,#178783),(#178784,#178785,#178786,#178787,#178788,#178789,
#178790,#178791,#178792),(#178793,#178794,#178795,#178796,#178797,#178798,
#178799,#178800,#178801),(#178802,#178803,#178804,#178805,#178806,#178807,
#178808,#178809,#178810),(#178811,#178812,#178813,#178814,#178815,#178816,
#178817,#178818,#178819),(#178820,#178821,#178822,#178823,#178824,#178825,
#178826,#178827,#178828),(#178829,#178830,#178831,#178832,#178833,#178834,
#178835,#178836,#178837),(#178838,#178839,#178840,#178841,#178842,#178843,
#178844,#178845,#178846),(#178847,#178848,#178849,#178850,#178851,#178852,
#178853,#178854,#178855),(#178856,#178857,#178858,#178859,#178860,#178861,
#178862,#178863,#178864),(#178865,#178866,#178867,#178868,#178869,#178870,
#178871,#178872,#178873),(#178874,#178875,#178876,#178877,#178878,#178879,
#178880,#178881,#178882),(#178883,#178884,#178885,#178886,#178887,#178888,
#178889,#178890,#178891),(#178892,#178893,#178894,#178895,#178896,#178897,
#178898,#178899,#178900),(#178901,#178902,#178903,#178904,#178905,#178906,
#178907,#178908,#178909),(#178910,#178911,#178912,#178913,#178914,#178915,
#178916,#178917,#178918),(#178919,#178920,#178921,#178922,#178923,#178924,
#178925,#178926,#178927),(#178928,#178929,#178930,#178931,#178932,#178933,
#178934,#178935,#178936),(#178937,#178938,#178939,#178940,#178941,#178942,
#178943,#178944,#178945),(#178946,#178947,#178948,#178949,#178950,#178951,
#178952,#178953,#178954),(#178955,#178956,#178957,#178958,#178959,#178960,
#178961,#178962,#178963),(#178964,#178965,#178966,#178967,#178968,#178969,
#178970,#178971,#178972),(#178973,#178974,#178975,#178976,#178977,#178978,
#178979,#178980,#178981),(#178982,#178983,#178984,#178985,#178986,#178987,
#178988,#178989,#178990),(#178991,#178992,#178993,#178994,#178995,#178996,
#178997,#178998,#178999),(#179000,#179001,#179002,#179003,#179004,#179005,
#179006,#179007,#179008),(#179009,#179010,#179011,#179012,#179013,#179014,
#179015,#179016,#179017),(#179018,#179019,#179020,#179021,#179022,#179023,
#179024,#179025,#179026),(#179027,#179028,#179029,#179030,#179031,#179032,
#179033,#179034,#179035),(#179036,#179037,#179038,#179039,#179040,#179041,
#179042,#179043,#179044),(#179045,#179046,#179047,#179048,#179049,#179050,
#179051,#179052,#179053),(#179054,#179055,#179056,#179057,#179058,#179059,
#179060,#179061,#179062),(#179063,#179064,#179065,#179066,#179067,#179068,
#179069,#179070,#179071),(#179072,#179073,#179074,#179075,#179076,#179077,
#179078,#179079,#179080),(#179081,#179082,#179083,#179084,#179085,#179086,
#179087,#179088,#179089),(#179090,#179091,#179092,#179093,#179094,#179095,
#179096,#179097,#179098),(#179099,#179100,#179101,#179102,#179103,#179104,
#179105,#179106,#179107),(#179108,#179109,#179110,#179111,#179112,#179113,
#179114,#179115,#179116),(#179117,#179118,#179119,#179120,#179121,#179122,
#179123,#179124,#179125),(#179126,#179127,#179128,#179129,#179130,#179131,
#179132,#179133,#179134),(#179135,#179136,#179137,#179138,#179139,#179140,
#179141,#179142,#179143),(#179144,#179145,#179146,#179147,#179148,#179149,
#179150,#179151,#179152),(#179153,#179154,#179155,#179156,#179157,#179158,
#179159,#179160,#179161),(#179162,#179163,#179164,#179165,#179166,#179167,
#179168,#179169,#179170),(#179171,#179172,#179173,#179174,#179175,#179176,
#179177,#179178,#179179),(#179180,#179181,#179182,#179183,#179184,#179185,
#179186,#179187,#179188),(#179189,#179190,#179191,#179192,#179193,#179194,
#179195,#179196,#179197),(#179198,#179199,#179200,#179201,#179202,#179203,
#179204,#179205,#179206),(#179207,#179208,#179209,#179210,#179211,#179212,
#179213,#179214,#179215),(#179216,#179217,#179218,#179219,#179220,#179221,
#179222,#179223,#179224),(#179225,#179226,#179227,#179228,#179229,#179230,
#179231,#179232,#179233),(#179234,#179235,#179236,#179237,#179238,#179239,
#179240,#179241,#179242),(#179243,#179244,#179245,#179246,#179247,#179248,
#179249,#179250,#179251),(#179252,#179253,#179254,#179255,#179256,#179257,
#179258,#179259,#179260),(#179261,#179262,#179263,#179264,#179265,#179266,
#179267,#179268,#179269),(#179270,#179271,#179272,#179273,#179274,#179275,
#179276,#179277,#179278),(#179279,#179280,#179281,#179282,#179283,#179284,
#179285,#179286,#179287),(#179288,#179289,#179290,#179291,#179292,#179293,
#179294,#179295,#179296),(#179297,#179298,#179299,#179300,#179301,#179302,
#179303,#179304,#179305),(#179306,#179307,#179308,#179309,#179310,#179311,
#179312,#179313,#179314),(#179315,#179316,#179317,#179318,#179319,#179320,
#179321,#179322,#179323),(#179324,#179325,#179326,#179327,#179328,#179329,
#179330,#179331,#179332),(#179333,#179334,#179335,#179336,#179337,#179338,
#179339,#179340,#179341),(#179342,#179343,#179344,#179345,#179346,#179347,
#179348,#179349,#179350),(#179351,#179352,#179353,#179354,#179355,#179356,
#179357,#179358,#179359),(#179360,#179361,#179362,#179363,#179364,#179365,
#179366,#179367,#179368),(#179369,#179370,#179371,#179372,#179373,#179374,
#179375,#179376,#179377),(#179378,#179379,#179380,#179381,#179382,#179383,
#179384,#179385,#179386),(#179387,#179388,#179389,#179390,#179391,#179392,
#179393,#179394,#179395),(#179396,#179397,#179398,#179399,#179400,#179401,
#179402,#179403,#179404),(#179405,#179406,#179407,#179408,#179409,#179410,
#179411,#179412,#179413),(#179414,#179415,#179416,#179417,#179418,#179419,
#179420,#179421,#179422),(#179423,#179424,#179425,#179426,#179427,#179428,
#179429,#179430,#179431),(#179432,#179433,#179434,#179435,#179436,#179437,
#179438,#179439,#179440),(#179441,#179442,#179443,#179444,#179445,#179446,
#179447,#179448,#179449),(#179450,#179451,#179452,#179453,#179454,#179455,
#179456,#179457,#179458),(#179459,#179460,#179461,#179462,#179463,#179464,
#179465,#179466,#179467),(#179468,#179469,#179470,#179471,#179472,#179473,
#179474,#179475,#179476),(#179477,#179478,#179479,#179480,#179481,#179482,
#179483,#179484,#179485),(#179486,#179487,#179488,#179489,#179490,#179491,
#179492,#179493,#179494),(#179495,#179496,#179497,#179498,#179499,#179500,
#179501,#179502,#179503),(#179504,#179505,#179506,#179507,#179508,#179509,
#179510,#179511,#179512),(#179513,#179514,#179515,#179516,#179517,#179518,
#179519,#179520,#179521),(#179522,#179523,#179524,#179525,#179526,#179527,
#179528,#179529,#179530),(#179531,#179532,#179533,#179534,#179535,#179536,
#179537,#179538,#179539),(#179540,#179541,#179542,#179543,#179544,#179545,
#179546,#179547,#179548),(#179549,#179550,#179551,#179552,#179553,#179554,
#179555,#179556,#179557),(#179558,#179559,#179560,#179561,#179562,#179563,
#179564,#179565,#179566),(#179567,#179568,#179569,#179570,#179571,#179572,
#179573,#179574,#179575),(#179576,#179577,#179578,#179579,#179580,#179581,
#179582,#179583,#179584),(#179585,#179586,#179587,#179588,#179589,#179590,
#179591,#179592,#179593),(#179594,#179595,#179596,#179597,#179598,#179599,
#179600,#179601,#179602),(#179603,#179604,#179605,#179606,#179607,#179608,
#179609,#179610,#179611),(#179612,#179613,#179614,#179615,#179616,#179617,
#179618,#179619,#179620),(#179621,#179622,#179623,#179624,#179625,#179626,
#179627,#179628,#179629),(#179630,#179631,#179632,#179633,#179634,#179635,
#179636,#179637,#179638),(#179639,#179640,#179641,#179642,#179643,#179644,
#179645,#179646,#179647),(#179648,#179649,#179650,#179651,#179652,#179653,
#179654,#179655,#179656),(#179657,#179658,#179659,#179660,#179661,#179662,
#179663,#179664,#179665),(#179666,#179667,#179668,#179669,#179670,#179671,
#179672,#179673,#179674),(#179675,#179676,#179677,#179678,#179679,#179680,
#179681,#179682,#179683),(#179684,#179685,#179686,#179687,#179688,#179689,
#179690,#179691,#179692),(#179693,#179694,#179695,#179696,#179697,#179698,
#179699,#179700,#179701),(#179702,#179703,#179704,#179705,#179706,#179707,
#179708,#179709,#179710),(#179711,#179712,#179713,#179714,#179715,#179716,
#179717,#179718,#179719),(#179720,#179721,#179722,#179723,#179724,#179725,
#179726,#179727,#179728),(#179729,#179730,#179731,#179732,#179733,#179734,
#179735,#179736,#179737),(#179738,#179739,#179740,#179741,#179742,#179743,
#179744,#179745,#179746),(#179747,#179748,#179749,#179750,#179751,#179752,
#179753,#179754,#179755),(#179756,#179757,#179758,#179759,#179760,#179761,
#179762,#179763,#179764),(#179765,#179766,#179767,#179768,#179769,#179770,
#179771,#179772,#179773),(#179774,#179775,#179776,#179777,#179778,#179779,
#179780,#179781,#179782),(#179783,#179784,#179785,#179786,#179787,#179788,
#179789,#179790,#179791),(#179792,#179793,#179794,#179795,#179796,#179797,
#179798,#179799,#179800),(#179801,#179802,#179803,#179804,#179805,#179806,
#179807,#179808,#179809),(#179810,#179811,#179812,#179813,#179814,#179815,
#179816,#179817,#179818),(#179819,#179820,#179821,#179822,#179823,#179824,
#179825,#179826,#179827),(#179828,#179829,#179830,#179831,#179832,#179833,
#179834,#179835,#179836),(#179837,#179838,#179839,#179840,#179841,#179842,
#179843,#179844,#179845),(#179846,#179847,#179848,#179849,#179850,#179851,
#179852,#179853,#179854),(#179855,#179856,#179857,#179858,#179859,#179860,
#179861,#179862,#179863),(#179864,#179865,#179866,#179867,#179868,#179869,
#179870,#179871,#179872),(#179873,#179874,#179875,#179876,#179877,#179878,
#179879,#179880,#179881),(#179882,#179883,#179884,#179885,#179886,#179887,
#179888,#179889,#179890),(#179891,#179892,#179893,#179894,#179895,#179896,
#179897,#179898,#179899),(#179900,#179901,#179902,#179903,#179904,#179905,
#179906,#179907,#179908),(#179909,#179910,#179911,#179912,#179913,#179914,
#179915,#179916,#179917),(#179918,#179919,#179920,#179921,#179922,#179923,
#179924,#179925,#179926),(#179927,#179928,#179929,#179930,#179931,#179932,
#179933,#179934,#179935),(#179936,#179937,#179938,#179939,#179940,#179941,
#179942,#179943,#179944),(#179945,#179946,#179947,#179948,#179949,#179950,
#179951,#179952,#179953),(#179954,#179955,#179956,#179957,#179958,#179959,
#179960,#179961,#179962),(#179963,#179964,#179965,#179966,#179967,#179968,
#179969,#179970,#179971),(#179972,#179973,#179974,#179975,#179976,#179977,
#179978,#179979,#179980),(#179981,#179982,#179983,#179984,#179985,#179986,
#179987,#179988,#179989),(#179990,#179991,#179992,#179993,#179994,#179995,
#179996,#179997,#179998),(#179999,#180000,#180001,#180002,#180003,#180004,
#180005,#180006,#180007),(#180008,#180009,#180010,#180011,#180012,#180013,
#180014,#180015,#180016),(#180017,#180018,#180019,#180020,#180021,#180022,
#180023,#180024,#180025),(#180026,#180027,#180028,#180029,#180030,#180031,
#180032,#180033,#180034),(#180035,#180036,#180037,#180038,#180039,#180040,
#180041,#180042,#180043),(#180044,#180045,#180046,#180047,#180048,#180049,
#180050,#180051,#180052),(#180053,#180054,#180055,#180056,#180057,#180058,
#180059,#180060,#180061),(#180062,#180063,#180064,#180065,#180066,#180067,
#180068,#180069,#180070),(#180071,#180072,#180073,#180074,#180075,#180076,
#180077,#180078,#180079),(#180080,#180081,#180082,#180083,#180084,#180085,
#180086,#180087,#180088),(#180089,#180090,#180091,#180092,#180093,#180094,
#180095,#180096,#180097),(#180098,#180099,#180100,#180101,#180102,#180103,
#180104,#180105,#180106),(#180107,#180108,#180109,#180110,#180111,#180112,
#180113,#180114,#180115),(#180116,#180117,#180118,#180119,#180120,#180121,
#180122,#180123,#180124),(#180125,#180126,#180127,#180128,#180129,#180130,
#180131,#180132,#180133),(#180134,#180135,#180136,#180137,#180138,#180139,
#180140,#180141,#180142),(#180143,#180144,#180145,#180146,#180147,#180148,
#180149,#180150,#180151),(#180152,#180153,#180154,#180155,#180156,#180157,
#180158,#180159,#180160),(#180161,#180162,#180163,#180164,#180165,#180166,
#180167,#180168,#180169),(#180170,#180171,#180172,#180173,#180174,#180175,
#180176,#180177,#180178),(#180179,#180180,#180181,#180182,#180183,#180184,
#180185,#180186,#180187),(#180188,#180189,#180190,#180191,#180192,#180193,
#180194,#180195,#180196),(#180197,#180198,#180199,#180200,#180201,#180202,
#180203,#180204,#180205),(#180206,#180207,#180208,#180209,#180210,#180211,
#180212,#180213,#180214),(#180215,#180216,#180217,#180218,#180219,#180220,
#180221,#180222,#180223),(#180224,#180225,#180226,#180227,#180228,#180229,
#180230,#180231,#180232),(#180233,#180234,#180235,#180236,#180237,#180238,
#180239,#180240,#180241),(#180242,#180243,#180244,#180245,#180246,#180247,
#180248,#180249,#180250),(#180251,#180252,#180253,#180254,#180255,#180256,
#180257,#180258,#180259),(#180260,#180261,#180262,#180263,#180264,#180265,
#180266,#180267,#180268),(#180269,#180270,#180271,#180272,#180273,#180274,
#180275,#180276,#180277),(#180278,#180279,#180280,#180281,#180282,#180283,
#180284,#180285,#180286),(#180287,#180288,#180289,#180290,#180291,#180292,
#180293,#180294,#180295),(#180296,#180297,#180298,#180299,#180300,#180301,
#180302,#180303,#180304),(#180305,#180306,#180307,#180308,#180309,#180310,
#180311,#180312,#180313),(#180314,#180315,#180316,#180317,#180318,#180319,
#180320,#180321,#180322),(#180323,#180324,#180325,#180326,#180327,#180328,
#180329,#180330,#180331),(#180332,#180333,#180334,#180335,#180336,#180337,
#180338,#180339,#180340),(#180341,#180342,#180343,#180344,#180345,#180346,
#180347,#180348,#180349),(#180350,#180351,#180352,#180353,#180354,#180355,
#180356,#180357,#180358),(#180359,#180360,#180361,#180362,#180363,#180364,
#180365,#180366,#180367),(#180368,#180369,#180370,#180371,#180372,#180373,
#180374,#180375,#180376),(#180377,#180378,#180379,#180380,#180381,#180382,
#180383,#180384,#180385),(#180386,#180387,#180388,#180389,#180390,#180391,
#180392,#180393,#180394),(#180395,#180396,#180397,#180398,#180399,#180400,
#180401,#180402,#180403),(#180404,#180405,#180406,#180407,#180408,#180409,
#180410,#180411,#180412),(#180413,#180414,#180415,#180416,#180417,#180418,
#180419,#180420,#180421),(#180422,#180423,#180424,#180425,#180426,#180427,
#180428,#180429,#180430),(#180431,#180432,#180433,#180434,#180435,#180436,
#180437,#180438,#180439),(#180440,#180441,#180442,#180443,#180444,#180445,
#180446,#180447,#180448),(#180449,#180450,#180451,#180452,#180453,#180454,
#180455,#180456,#180457),(#180458,#180459,#180460,#180461,#180462,#180463,
#180464,#180465,#180466),(#180467,#180468,#180469,#180470,#180471,#180472,
#180473,#180474,#180475),(#180476,#180477,#180478,#180479,#180480,#180481,
#180482,#180483,#180484),(#180485,#180486,#180487,#180488,#180489,#180490,
#180491,#180492,#180493),(#180494,#180495,#180496,#180497,#180498,#180499,
#180500,#180501,#180502),(#180503,#180504,#180505,#180506,#180507,#180508,
#180509,#180510,#180511),(#180512,#180513,#180514,#180515,#180516,#180517,
#180518,#180519,#180520),(#180521,#180522,#180523,#180524,#180525,#180526,
#180527,#180528,#180529),(#180530,#180531,#180532,#180533,#180534,#180535,
#180536,#180537,#180538),(#180539,#180540,#180541,#180542,#180543,#180544,
#180545,#180546,#180547),(#180548,#180549,#180550,#180551,#180552,#180553,
#180554,#180555,#180556),(#180557,#180558,#180559,#180560,#180561,#180562,
#180563,#180564,#180565),(#180566,#180567,#180568,#180569,#180570,#180571,
#180572,#180573,#180574),(#180575,#180576,#180577,#180578,#180579,#180580,
#180581,#180582,#180583),(#180584,#180585,#180586,#180587,#180588,#180589,
#180590,#180591,#180592),(#180593,#180594,#180595,#180596,#180597,#180598,
#180599,#180600,#180601),(#180602,#180603,#180604,#180605,#180606,#180607,
#180608,#180609,#180610),(#180611,#180612,#180613,#180614,#180615,#180616,
#180617,#180618,#180619),(#180620,#180621,#180622,#180623,#180624,#180625,
#180626,#180627,#180628),(#180629,#180630,#180631,#180632,#180633,#180634,
#180635,#180636,#180637),(#180638,#180639,#180640,#180641,#180642,#180643,
#180644,#180645,#180646),(#180647,#180648,#180649,#180650,#180651,#180652,
#180653,#180654,#180655),(#180656,#180657,#180658,#180659,#180660,#180661,
#180662,#180663,#180664),(#180665,#180666,#180667,#180668,#180669,#180670,
#180671,#180672,#180673),(#180674,#180675,#180676,#180677,#180678,#180679,
#180680,#180681,#180682),(#180683,#180684,#180685,#180686,#180687,#180688,
#180689,#180690,#180691),(#180692,#180693,#180694,#180695,#180696,#180697,
#180698,#180699,#180700),(#180701,#180702,#180703,#180704,#180705,#180706,
#180707,#180708,#180709),(#180710,#180711,#180712,#180713,#180714,#180715,
#180716,#180717,#180718),(#180719,#180720,#180721,#180722,#180723,#180724,
#180725,#180726,#180727),(#180728,#180729,#180730,#180731,#180732,#180733,
#180734,#180735,#180736),(#180737,#180738,#180739,#180740,#180741,#180742,
#180743,#180744,#180745),(#180746,#180747,#180748,#180749,#180750,#180751,
#180752,#180753,#180754),(#180755,#180756,#180757,#180758,#180759,#180760,
#180761,#180762,#180763),(#180764,#180765,#180766,#180767,#180768,#180769,
#180770,#180771,#180772),(#180773,#180774,#180775,#180776,#180777,#180778,
#180779,#180780,#180781),(#180782,#180783,#180784,#180785,#180786,#180787,
#180788,#180789,#180790),(#180791,#180792,#180793,#180794,#180795,#180796,
#180797,#180798,#180799),(#180800,#180801,#180802,#180803,#180804,#180805,
#180806,#180807,#180808),(#180809,#180810,#180811,#180812,#180813,#180814,
#180815,#180816,#180817),(#180818,#180819,#180820,#180821,#180822,#180823,
#180824,#180825,#180826),(#180827,#180828,#180829,#180830,#180831,#180832,
#180833,#180834,#180835),(#180836,#180837,#180838,#180839,#180840,#180841,
#180842,#180843,#180844),(#180845,#180846,#180847,#180848,#180849,#180850,
#180851,#180852,#180853),(#180854,#180855,#180856,#180857,#180858,#180859,
#180860,#180861,#180862),(#180863,#180864,#180865,#180866,#180867,#180868,
#180869,#180870,#180871),(#180872,#180873,#180874,#180875,#180876,#180877,
#180878,#180879,#180880),(#180881,#180882,#180883,#180884,#180885,#180886,
#180887,#180888,#180889),(#180890,#180891,#180892,#180893,#180894,#180895,
#180896,#180897,#180898),(#180899,#180900,#180901,#180902,#180903,#180904,
#180905,#180906,#180907),(#180908,#180909,#180910,#180911,#180912,#180913,
#180914,#180915,#180916),(#180917,#180918,#180919,#180920,#180921,#180922,
#180923,#180924,#180925),(#180926,#180927,#180928,#180929,#180930,#180931,
#180932,#180933,#180934),(#180935,#180936,#180937,#180938,#180939,#180940,
#180941,#180942,#180943),(#180944,#180945,#180946,#180947,#180948,#180949,
#180950,#180951,#180952),(#180953,#180954,#180955,#180956,#180957,#180958,
#180959,#180960,#180961),(#180962,#180963,#180964,#180965,#180966,#180967,
#180968,#180969,#180970),(#180971,#180972,#180973,#180974,#180975,#180976,
#180977,#180978,#180979),(#180980,#180981,#180982,#180983,#180984,#180985,
#180986,#180987,#180988),(#180989,#180990,#180991,#180992,#180993,#180994,
#180995,#180996,#180997),(#180998,#180999,#181000,#181001,#181002,#181003,
#181004,#181005,#181006),(#181007,#181008,#181009,#181010,#181011,#181012,
#181013,#181014,#181015),(#181016,#181017,#181018,#181019,#181020,#181021,
#181022,#181023,#181024),(#181025,#181026,#181027,#181028,#181029,#181030,
#181031,#181032,#181033),(#181034,#181035,#181036,#181037,#181038,#181039,
#181040,#181041,#181042),(#181043,#181044,#181045,#181046,#181047,#181048,
#181049,#181050,#181051),(#181052,#181053,#181054,#181055,#181056,#181057,
#181058,#181059,#181060),(#181061,#181062,#181063,#181064,#181065,#181066,
#181067,#181068,#181069),(#181070,#181071,#181072,#181073,#181074,#181075,
#181076,#181077,#181078),(#181079,#181080,#181081,#181082,#181083,#181084,
#181085,#181086,#181087),(#181088,#181089,#181090,#181091,#181092,#181093,
#181094,#181095,#181096),(#181097,#181098,#181099,#181100,#181101,#181102,
#181103,#181104,#181105),(#181106,#181107,#181108,#181109,#181110,#181111,
#181112,#181113,#181114),(#181115,#181116,#181117,#181118,#181119,#181120,
#181121,#181122,#181123),(#181124,#181125,#181126,#181127,#181128,#181129,
#181130,#181131,#181132),(#181133,#181134,#181135,#181136,#181137,#181138,
#181139,#181140,#181141),(#181142,#181143,#181144,#181145,#181146,#181147,
#181148,#181149,#181150),(#181151,#181152,#181153,#181154,#181155,#181156,
#181157,#181158,#181159),(#181160,#181161,#181162,#181163,#181164,#181165,
#181166,#181167,#181168),(#181169,#181170,#181171,#181172,#181173,#181174,
#181175,#181176,#181177),(#181178,#181179,#181180,#181181,#181182,#181183,
#181184,#181185,#181186),(#181187,#181188,#181189,#181190,#181191,#181192,
#181193,#181194,#181195),(#181196,#181197,#181198,#181199,#181200,#181201,
#181202,#181203,#181204),(#181205,#181206,#181207,#181208,#181209,#181210,
#181211,#181212,#181213),(#181214,#181215,#181216,#181217,#181218,#181219,
#181220,#181221,#181222),(#181223,#181224,#181225,#181226,#181227,#181228,
#181229,#181230,#181231),(#181232,#181233,#181234,#181235,#181236,#181237,
#181238,#181239,#181240),(#181241,#181242,#181243,#181244,#181245,#181246,
#181247,#181248,#181249),(#181250,#181251,#181252,#181253,#181254,#181255,
#181256,#181257,#181258),(#181259,#181260,#181261,#181262,#181263,#181264,
#181265,#181266,#181267),(#181268,#181269,#181270,#181271,#181272,#181273,
#181274,#181275,#181276),(#181277,#181278,#181279,#181280,#181281,#181282,
#181283,#181284,#181285),(#181286,#181287,#181288,#181289,#181290,#181291,
#181292,#181293,#181294),(#181295,#181296,#181297,#181298,#181299,#181300,
#181301,#181302,#181303),(#181304,#181305,#181306,#181307,#181308,#181309,
#181310,#181311,#181312),(#181313,#181314,#181315,#181316,#181317,#181318,
#181319,#181320,#181321),(#181322,#181323,#181324,#181325,#181326,#181327,
#181328,#181329,#181330),(#181331,#181332,#181333,#181334,#181335,#181336,
#181337,#181338,#181339),(#181340,#181341,#181342,#181343,#181344,#181345,
#181346,#181347,#181348),(#181349,#181350,#181351,#181352,#181353,#181354,
#181355,#181356,#181357),(#181358,#181359,#181360,#181361,#181362,#181363,
#181364,#181365,#181366),(#181367,#181368,#181369,#181370,#181371,#181372,
#181373,#181374,#181375),(#181376,#181377,#181378,#181379,#181380,#181381,
#181382,#181383,#181384),(#181385,#181386,#181387,#181388,#181389,#181390,
#181391,#181392,#181393),(#181394,#181395,#181396,#181397,#181398,#181399,
#181400,#181401,#181402),(#181403,#181404,#181405,#181406,#181407,#181408,
#181409,#181410,#181411),(#181412,#181413,#181414,#181415,#181416,#181417,
#181418,#181419,#181420),(#181421,#181422,#181423,#181424,#181425,#181426,
#181427,#181428,#181429),(#181430,#181431,#181432,#181433,#181434,#181435,
#181436,#181437,#181438),(#181439,#181440,#181441,#181442,#181443,#181444,
#181445,#181446,#181447),(#181448,#181449,#181450,#181451,#181452,#181453,
#181454,#181455,#181456),(#181457,#181458,#181459,#181460,#181461,#181462,
#181463,#181464,#181465),(#181466,#181467,#181468,#181469,#181470,#181471,
#181472,#181473,#181474),(#181475,#181476,#181477,#181478,#181479,#181480,
#181481,#181482,#181483),(#181484,#181485,#181486,#181487,#181488,#181489,
#181490,#181491,#181492),(#181493,#181494,#181495,#181496,#181497,#181498,
#181499,#181500,#181501),(#181502,#181503,#181504,#181505,#181506,#181507,
#181508,#181509,#181510),(#181511,#181512,#181513,#181514,#181515,#181516,
#181517,#181518,#181519),(#181520,#181521,#181522,#181523,#181524,#181525,
#181526,#181527,#181528),(#181529,#181530,#181531,#181532,#181533,#181534,
#181535,#181536,#181537),(#181538,#181539,#181540,#181541,#181542,#181543,
#181544,#181545,#181546),(#181547,#181548,#181549,#181550,#181551,#181552,
#181553,#181554,#181555),(#181556,#181557,#181558,#181559,#181560,#181561,
#181562,#181563,#181564),(#181565,#181566,#181567,#181568,#181569,#181570,
#181571,#181572,#181573),(#181574,#181575,#181576,#181577,#181578,#181579,
#181580,#181581,#181582),(#181583,#181584,#181585,#181586,#181587,#181588,
#181589,#181590,#181591),(#181592,#181593,#181594,#181595,#181596,#181597,
#181598,#181599,#181600),(#181601,#181602,#181603,#181604,#181605,#181606,
#181607,#181608,#181609),(#181610,#181611,#181612,#181613,#181614,#181615,
#181616,#181617,#181618),(#181619,#181620,#181621,#181622,#181623,#181624,
#181625,#181626,#181627),(#181628,#181629,#181630,#181631,#181632,#181633,
#181634,#181635,#181636),(#181637,#181638,#181639,#181640,#181641,#181642,
#181643,#181644,#181645),(#181646,#181647,#181648,#181649,#181650,#181651,
#181652,#181653,#181654),(#181655,#181656,#181657,#181658,#181659,#181660,
#181661,#181662,#181663),(#181664,#181665,#181666,#181667,#181668,#181669,
#181670,#181671,#181672),(#181673,#181674,#181675,#181676,#181677,#181678,
#181679,#181680,#181681),(#181682,#181683,#181684,#181685,#181686,#181687,
#181688,#181689,#181690),(#181691,#181692,#181693,#181694,#181695,#181696,
#181697,#181698,#181699),(#181700,#181701,#181702,#181703,#181704,#181705,
#181706,#181707,#181708),(#181709,#181710,#181711,#181712,#181713,#181714,
#181715,#181716,#181717),(#181718,#181719,#181720,#181721,#181722,#181723,
#181724,#181725,#181726),(#181727,#181728,#181729,#181730,#181731,#181732,
#181733,#181734,#181735),(#181736,#181737,#181738,#181739,#181740,#181741,
#181742,#181743,#181744),(#181745,#181746,#181747,#181748,#181749,#181750,
#181751,#181752,#181753),(#181754,#181755,#181756,#181757,#181758,#181759,
#181760,#181761,#181762),(#181763,#181764,#181765,#181766,#181767,#181768,
#181769,#181770,#181771),(#181772,#181773,#181774,#181775,#181776,#181777,
#181778,#181779,#181780),(#181781,#181782,#181783,#181784,#181785,#181786,
#181787,#181788,#181789),(#181790,#181791,#181792,#181793,#181794,#181795,
#181796,#181797,#181798),(#181799,#181800,#181801,#181802,#181803,#181804,
#181805,#181806,#181807),(#181808,#181809,#181810,#181811,#181812,#181813,
#181814,#181815,#181816),(#181817,#181818,#181819,#181820,#181821,#181822,
#181823,#181824,#181825),(#181826,#181827,#181828,#181829,#181830,#181831,
#181832,#181833,#181834),(#181835,#181836,#181837,#181838,#181839,#181840,
#181841,#181842,#181843),(#181844,#181845,#181846,#181847,#181848,#181849,
#181850,#181851,#181852),(#181853,#181854,#181855,#181856,#181857,#181858,
#181859,#181860,#181861),(#181862,#181863,#181864,#181865,#181866,#181867,
#181868,#181869,#181870),(#181871,#181872,#181873,#181874,#181875,#181876,
#181877,#181878,#181879),(#181880,#181881,#181882,#181883,#181884,#181885,
#181886,#181887,#181888),(#181889,#181890,#181891,#181892,#181893,#181894,
#181895,#181896,#181897),(#181898,#181899,#181900,#181901,#181902,#181903,
#181904,#181905,#181906),(#181907,#181908,#181909,#181910,#181911,#181912,
#181913,#181914,#181915),(#181916,#181917,#181918,#181919,#181920,#181921,
#181922,#181923,#181924),(#181925,#181926,#181927,#181928,#181929,#181930,
#181931,#181932,#181933),(#181934,#181935,#181936,#181937,#181938,#181939,
#181940,#181941,#181942),(#181943,#181944,#181945,#181946,#181947,#181948,
#181949,#181950,#181951),(#181952,#181953,#181954,#181955,#181956,#181957,
#181958,#181959,#181960),(#181961,#181962,#181963,#181964,#181965,#181966,
#181967,#181968,#181969),(#181970,#181971,#181972,#181973,#181974,#181975,
#181976,#181977,#181978),(#181979,#181980,#181981,#181982,#181983,#181984,
#181985,#181986,#181987),(#181988,#181989,#181990,#181991,#181992,#181993,
#181994,#181995,#181996),(#181997,#181998,#181999,#182000,#182001,#182002,
#182003,#182004,#182005),(#182006,#182007,#182008,#182009,#182010,#182011,
#182012,#182013,#182014),(#182015,#182016,#182017,#182018,#182019,#182020,
#182021,#182022,#182023),(#182024,#182025,#182026,#182027,#182028,#182029,
#182030,#182031,#182032),(#182033,#182034,#182035,#182036,#182037,#182038,
#182039,#182040,#182041),(#182042,#182043,#182044,#182045,#182046,#182047,
#182048,#182049,#182050),(#182051,#182052,#182053,#182054,#182055,#182056,
#182057,#182058,#182059),(#182060,#182061,#182062,#182063,#182064,#182065,
#182066,#182067,#182068),(#182069,#182070,#182071,#182072,#182073,#182074,
#182075,#182076,#182077),(#182078,#182079,#182080,#182081,#182082,#182083,
#182084,#182085,#182086),(#182087,#182088,#182089,#182090,#182091,#182092,
#182093,#182094,#182095),(#182096,#182097,#182098,#182099,#182100,#182101,
#182102,#182103,#182104),(#182105,#182106,#182107,#182108,#182109,#182110,
#182111,#182112,#182113),(#182114,#182115,#182116,#182117,#182118,#182119,
#182120,#182121,#182122),(#182123,#182124,#182125,#182126,#182127,#182128,
#182129,#182130,#182131),(#182132,#182133,#182134,#182135,#182136,#182137,
#182138,#182139,#182140),(#182141,#182142,#182143,#182144,#182145,#182146,
#182147,#182148,#182149),(#182150,#182151,#182152,#182153,#182154,#182155,
#182156,#182157,#182158),(#182159,#182160,#182161,#182162,#182163,#182164,
#182165,#182166,#182167),(#182168,#182169,#182170,#182171,#182172,#182173,
#182174,#182175,#182176),(#182177,#182178,#182179,#182180,#182181,#182182,
#182183,#182184,#182185),(#182186,#182187,#182188,#182189,#182190,#182191,
#182192,#182193,#182194),(#182195,#182196,#182197,#182198,#182199,#182200,
#182201,#182202,#182203),(#182204,#182205,#182206,#182207,#182208,#182209,
#182210,#182211,#182212),(#182213,#182214,#182215,#182216,#182217,#182218,
#182219,#182220,#182221),(#182222,#182223,#182224,#182225,#182226,#182227,
#182228,#182229,#182230),(#182231,#182232,#182233,#182234,#182235,#182236,
#182237,#182238,#182239),(#182240,#182241,#182242,#182243,#182244,#182245,
#182246,#182247,#182248),(#182249,#182250,#182251,#182252,#182253,#182254,
#182255,#182256,#182257),(#182258,#182259,#182260,#182261,#182262,#182263,
#182264,#182265,#182266),(#182267,#182268,#182269,#182270,#182271,#182272,
#182273,#182274,#182275),(#182276,#182277,#182278,#182279,#182280,#182281,
#182282,#182283,#182284),(#182285,#182286,#182287,#182288,#182289,#182290,
#182291,#182292,#182293),(#182294,#182295,#182296,#182297,#182298,#182299,
#182300,#182301,#182302),(#182303,#182304,#182305,#182306,#182307,#182308,
#182309,#182310,#182311),(#182312,#182313,#182314,#182315,#182316,#182317,
#182318,#182319,#182320),(#182321,#182322,#182323,#182324,#182325,#182326,
#182327,#182328,#182329),(#182330,#182331,#182332,#182333,#182334,#182335,
#182336,#182337,#182338),(#182339,#182340,#182341,#182342,#182343,#182344,
#182345,#182346,#182347),(#182348,#182349,#182350,#182351,#182352,#182353,
#182354,#182355,#182356),(#182357,#182358,#182359,#182360,#182361,#182362,
#182363,#182364,#182365),(#182366,#182367,#182368,#182369,#182370,#182371,
#182372,#182373,#182374),(#182375,#182376,#182377,#182378,#182379,#182380,
#182381,#182382,#182383),(#182384,#182385,#182386,#182387,#182388,#182389,
#182390,#182391,#182392),(#182393,#182394,#182395,#182396,#182397,#182398,
#182399,#182400,#182401),(#182402,#182403,#182404,#182405,#182406,#182407,
#182408,#182409,#182410),(#182411,#182412,#182413,#182414,#182415,#182416,
#182417,#182418,#182419),(#182420,#182421,#182422,#182423,#182424,#182425,
#182426,#182427,#182428),(#182429,#182430,#182431,#182432,#182433,#182434,
#182435,#182436,#182437),(#182438,#182439,#182440,#182441,#182442,#182443,
#182444,#182445,#182446),(#182447,#182448,#182449,#182450,#182451,#182452,
#182453,#182454,#182455),(#182456,#182457,#182458,#182459,#182460,#182461,
#182462,#182463,#182464),(#182465,#182466,#182467,#182468,#182469,#182470,
#182471,#182472,#182473),(#182474,#182475,#182476,#182477,#182478,#182479,
#182480,#182481,#182482),(#182483,#182484,#182485,#182486,#182487,#182488,
#182489,#182490,#182491),(#182492,#182493,#182494,#182495,#182496,#182497,
#182498,#182499,#182500),(#182501,#182502,#182503,#182504,#182505,#182506,
#182507,#182508,#182509),(#182510,#182511,#182512,#182513,#182514,#182515,
#182516,#182517,#182518),(#182519,#182520,#182521,#182522,#182523,#182524,
#182525,#182526,#182527),(#182528,#182529,#182530,#182531,#182532,#182533,
#182534,#182535,#182536),(#182537,#182538,#182539,#182540,#182541,#182542,
#182543,#182544,#182545),(#182546,#182547,#182548,#182549,#182550,#182551,
#182552,#182553,#182554),(#182555,#182556,#182557,#182558,#182559,#182560,
#182561,#182562,#182563),(#182564,#182565,#182566,#182567,#182568,#182569,
#182570,#182571,#182572),(#182573,#182574,#182575,#182576,#182577,#182578,
#182579,#182580,#182581),(#182582,#182583,#182584,#182585,#182586,#182587,
#182588,#182589,#182590),(#182591,#182592,#182593,#182594,#182595,#182596,
#182597,#182598,#182599),(#182600,#182601,#182602,#182603,#182604,#182605,
#182606,#182607,#182608),(#182609,#182610,#182611,#182612,#182613,#182614,
#182615,#182616,#182617),(#182618,#182619,#182620,#182621,#182622,#182623,
#182624,#182625,#182626),(#182627,#182628,#182629,#182630,#182631,#182632,
#182633,#182634,#182635),(#182636,#182637,#182638,#182639,#182640,#182641,
#182642,#182643,#182644),(#182645,#182646,#182647,#182648,#182649,#182650,
#182651,#182652,#182653),(#182654,#182655,#182656,#182657,#182658,#182659,
#182660,#182661,#182662),(#182663,#182664,#182665,#182666,#182667,#182668,
#182669,#182670,#182671),(#182672,#182673,#182674,#182675,#182676,#182677,
#182678,#182679,#182680),(#182681,#182682,#182683,#182684,#182685,#182686,
#182687,#182688,#182689),(#182690,#182691,#182692,#182693,#182694,#182695,
#182696,#182697,#182698),(#182699,#182700,#182701,#182702,#182703,#182704,
#182705,#182706,#182707),(#182708,#182709,#182710,#182711,#182712,#182713,
#182714,#182715,#182716),(#182717,#182718,#182719,#182720,#182721,#182722,
#182723,#182724,#182725),(#182726,#182727,#182728,#182729,#182730,#182731,
#182732,#182733,#182734),(#182735,#182736,#182737,#182738,#182739,#182740,
#182741,#182742,#182743),(#182744,#182745,#182746,#182747,#182748,#182749,
#182750,#182751,#182752),(#182753,#182754,#182755,#182756,#182757,#182758,
#182759,#182760,#182761),(#182762,#182763,#182764,#182765,#182766,#182767,
#182768,#182769,#182770),(#182771,#182772,#182773,#182774,#182775,#182776,
#182777,#182778,#182779),(#182780,#182781,#182782,#182783,#182784,#182785,
#182786,#182787,#182788),(#182789,#182790,#182791,#182792,#182793,#182794,
#182795,#182796,#182797),(#182798,#182799,#182800,#182801,#182802,#182803,
#182804,#182805,#182806),(#182807,#182808,#182809,#182810,#182811,#182812,
#182813,#182814,#182815),(#182816,#182817,#182818,#182819,#182820,#182821,
#182822,#182823,#182824),(#182825,#182826,#182827,#182828,#182829,#182830,
#182831,#182832,#182833),(#182834,#182835,#182836,#182837,#182838,#182839,
#182840,#182841,#182842),(#182843,#182844,#182845,#182846,#182847,#182848,
#182849,#182850,#182851),(#182852,#182853,#182854,#182855,#182856,#182857,
#182858,#182859,#182860),(#182861,#182862,#182863,#182864,#182865,#182866,
#182867,#182868,#182869),(#182870,#182871,#182872,#182873,#182874,#182875,
#182876,#182877,#182878),(#182879,#182880,#182881,#182882,#182883,#182884,
#182885,#182886,#182887),(#182888,#182889,#182890,#182891,#182892,#182893,
#182894,#182895,#182896),(#182897,#182898,#182899,#182900,#182901,#182902,
#182903,#182904,#182905),(#182906,#182907,#182908,#182909,#182910,#182911,
#182912,#182913,#182914),(#182915,#182916,#182917,#182918,#182919,#182920,
#182921,#182922,#182923),(#182924,#182925,#182926,#182927,#182928,#182929,
#182930,#182931,#182932),(#182933,#182934,#182935,#182936,#182937,#182938,
#182939,#182940,#182941),(#182942,#182943,#182944,#182945,#182946,#182947,
#182948,#182949,#182950),(#182951,#182952,#182953,#182954,#182955,#182956,
#182957,#182958,#182959),(#182960,#182961,#182962,#182963,#182964,#182965,
#182966,#182967,#182968),(#182969,#182970,#182971,#182972,#182973,#182974,
#182975,#182976,#182977),(#182978,#182979,#182980,#182981,#182982,#182983,
#182984,#182985,#182986),(#182987,#182988,#182989,#182990,#182991,#182992,
#182993,#182994,#182995),(#182996,#182997,#182998,#182999,#183000,#183001,
#183002,#183003,#183004),(#183005,#183006,#183007,#183008,#183009,#183010,
#183011,#183012,#183013),(#183014,#183015,#183016,#183017,#183018,#183019,
#183020,#183021,#183022),(#183023,#183024,#183025,#183026,#183027,#183028,
#183029,#183030,#183031),(#183032,#183033,#183034,#183035,#183036,#183037,
#183038,#183039,#183040),(#183041,#183042,#183043,#183044,#183045,#183046,
#183047,#183048,#183049),(#183050,#183051,#183052,#183053,#183054,#183055,
#183056,#183057,#183058),(#183059,#183060,#183061,#183062,#183063,#183064,
#183065,#183066,#183067),(#183068,#183069,#183070,#183071,#183072,#183073,
#183074,#183075,#183076),(#183077,#183078,#183079,#183080,#183081,#183082,
#183083,#183084,#183085),(#183086,#183087,#183088,#183089,#183090,#183091,
#183092,#183093,#183094),(#183095,#183096,#183097,#183098,#183099,#183100,
#183101,#183102,#183103),(#183104,#183105,#183106,#183107,#183108,#183109,
#183110,#183111,#183112),(#183113,#183114,#183115,#183116,#183117,#183118,
#183119,#183120,#183121),(#183122,#183123,#183124,#183125,#183126,#183127,
#183128,#183129,#183130),(#183131,#183132,#183133,#183134,#183135,#183136,
#183137,#183138,#183139),(#183140,#183141,#183142,#183143,#183144,#183145,
#183146,#183147,#183148),(#183149,#183150,#183151,#183152,#183153,#183154,
#183155,#183156,#183157),(#183158,#183159,#183160,#183161,#183162,#183163,
#183164,#183165,#183166),(#183167,#183168,#183169,#183170,#183171,#183172,
#183173,#183174,#183175),(#183176,#183177,#183178,#183179,#183180,#183181,
#183182,#183183,#183184),(#183185,#183186,#183187,#183188,#183189,#183190,
#183191,#183192,#183193),(#183194,#183195,#183196,#183197,#183198,#183199,
#183200,#183201,#183202),(#183203,#183204,#183205,#183206,#183207,#183208,
#183209,#183210,#183211),(#183212,#183213,#183214,#183215,#183216,#183217,
#183218,#183219,#183220),(#183221,#183222,#183223,#183224,#183225,#183226,
#183227,#183228,#183229),(#183230,#183231,#183232,#183233,#183234,#183235,
#183236,#183237,#183238),(#183239,#183240,#183241,#183242,#183243,#183244,
#183245,#183246,#183247),(#183248,#183249,#183250,#183251,#183252,#183253,
#183254,#183255,#183256),(#183257,#183258,#183259,#183260,#183261,#183262,
#183263,#183264,#183265),(#183266,#183267,#183268,#183269,#183270,#183271,
#183272,#183273,#183274),(#183275,#183276,#183277,#183278,#183279,#183280,
#183281,#183282,#183283),(#183284,#183285,#183286,#183287,#183288,#183289,
#183290,#183291,#183292),(#183293,#183294,#183295,#183296,#183297,#183298,
#183299,#183300,#183301),(#183302,#183303,#183304,#183305,#183306,#183307,
#183308,#183309,#183310),(#183311,#183312,#183313,#183314,#183315,#183316,
#183317,#183318,#183319),(#183320,#183321,#183322,#183323,#183324,#183325,
#183326,#183327,#183328),(#183329,#183330,#183331,#183332,#183333,#183334,
#183335,#183336,#183337),(#183338,#183339,#183340,#183341,#183342,#183343,
#183344,#183345,#183346),(#183347,#183348,#183349,#183350,#183351,#183352,
#183353,#183354,#183355),(#183356,#183357,#183358,#183359,#183360,#183361,
#183362,#183363,#183364),(#183365,#183366,#183367,#183368,#183369,#183370,
#183371,#183372,#183373),(#183374,#183375,#183376,#183377,#183378,#183379,
#183380,#183381,#183382),(#183383,#183384,#183385,#183386,#183387,#183388,
#183389,#183390,#183391),(#183392,#183393,#183394,#183395,#183396,#183397,
#183398,#183399,#183400),(#183401,#183402,#183403,#183404,#183405,#183406,
#183407,#183408,#183409),(#183410,#183411,#183412,#183413,#183414,#183415,
#183416,#183417,#183418),(#183419,#183420,#183421,#183422,#183423,#183424,
#183425,#183426,#183427),(#183428,#183429,#183430,#183431,#183432,#183433,
#183434,#183435,#183436),(#183437,#183438,#183439,#183440,#183441,#183442,
#183443,#183444,#183445),(#183446,#183447,#183448,#183449,#183450,#183451,
#183452,#183453,#183454),(#183455,#183456,#183457,#183458,#183459,#183460,
#183461,#183462,#183463),(#183464,#183465,#183466,#183467,#183468,#183469,
#183470,#183471,#183472),(#183473,#183474,#183475,#183476,#183477,#183478,
#183479,#183480,#183481),(#183482,#183483,#183484,#183485,#183486,#183487,
#183488,#183489,#183490),(#183491,#183492,#183493,#183494,#183495,#183496,
#183497,#183498,#183499),(#183500,#183501,#183502,#183503,#183504,#183505,
#183506,#183507,#183508),(#183509,#183510,#183511,#183512,#183513,#183514,
#183515,#183516,#183517),(#183518,#183519,#183520,#183521,#183522,#183523,
#183524,#183525,#183526),(#183527,#183528,#183529,#183530,#183531,#183532,
#183533,#183534,#183535),(#183536,#183537,#183538,#183539,#183540,#183541,
#183542,#183543,#183544),(#183545,#183546,#183547,#183548,#183549,#183550,
#183551,#183552,#183553),(#183554,#183555,#183556,#183557,#183558,#183559,
#183560,#183561,#183562),(#183563,#183564,#183565,#183566,#183567,#183568,
#183569,#183570,#183571),(#183572,#183573,#183574,#183575,#183576,#183577,
#183578,#183579,#183580),(#183581,#183582,#183583,#183584,#183585,#183586,
#183587,#183588,#183589),(#183590,#183591,#183592,#183593,#183594,#183595,
#183596,#183597,#183598),(#183599,#183600,#183601,#183602,#183603,#183604,
#183605,#183606,#183607),(#183608,#183609,#183610,#183611,#183612,#183613,
#183614,#183615,#183616),(#183617,#183618,#183619,#183620,#183621,#183622,
#183623,#183624,#183625),(#183626,#183627,#183628,#183629,#183630,#183631,
#183632,#183633,#183634),(#183635,#183636,#183637,#183638,#183639,#183640,
#183641,#183642,#183643),(#183644,#183645,#183646,#183647,#183648,#183649,
#183650,#183651,#183652),(#183653,#183654,#183655,#183656,#183657,#183658,
#183659,#183660,#183661),(#183662,#183663,#183664,#183665,#183666,#183667,
#183668,#183669,#183670),(#183671,#183672,#183673,#183674,#183675,#183676,
#183677,#183678,#183679),(#183680,#183681,#183682,#183683,#183684,#183685,
#183686,#183687,#183688),(#183689,#183690,#183691,#183692,#183693,#183694,
#183695,#183696,#183697),(#183698,#183699,#183700,#183701,#183702,#183703,
#183704,#183705,#183706),(#183707,#183708,#183709,#183710,#183711,#183712,
#183713,#183714,#183715),(#183716,#183717,#183718,#183719,#183720,#183721,
#183722,#183723,#183724),(#183725,#183726,#183727,#183728,#183729,#183730,
#183731,#183732,#183733),(#183734,#183735,#183736,#183737,#183738,#183739,
#183740,#183741,#183742),(#183743,#183744,#183745,#183746,#183747,#183748,
#183749,#183750,#183751),(#183752,#183753,#183754,#183755,#183756,#183757,
#183758,#183759,#183760),(#183761,#183762,#183763,#183764,#183765,#183766,
#183767,#183768,#183769),(#183770,#183771,#183772,#183773,#183774,#183775,
#183776,#183777,#183778),(#183779,#183780,#183781,#183782,#183783,#183784,
#183785,#183786,#183787),(#183788,#183789,#183790,#183791,#183792,#183793,
#183794,#183795,#183796),(#183797,#183798,#183799,#183800,#183801,#183802,
#183803,#183804,#183805),(#183806,#183807,#183808,#183809,#183810,#183811,
#183812,#183813,#183814),(#183815,#183816,#183817,#183818,#183819,#183820,
#183821,#183822,#183823),(#183824,#183825,#183826,#183827,#183828,#183829,
#183830,#183831,#183832),(#183833,#183834,#183835,#183836,#183837,#183838,
#183839,#183840,#183841),(#183842,#183843,#183844,#183845,#183846,#183847,
#183848,#183849,#183850),(#183851,#183852,#183853,#183854,#183855,#183856,
#183857,#183858,#183859),(#183860,#183861,#183862,#183863,#183864,#183865,
#183866,#183867,#183868),(#183869,#183870,#183871,#183872,#183873,#183874,
#183875,#183876,#183877),(#183878,#183879,#183880,#183881,#183882,#183883,
#183884,#183885,#183886),(#183887,#183888,#183889,#183890,#183891,#183892,
#183893,#183894,#183895),(#183896,#183897,#183898,#183899,#183900,#183901,
#183902,#183903,#183904),(#183905,#183906,#183907,#183908,#183909,#183910,
#183911,#183912,#183913),(#183914,#183915,#183916,#183917,#183918,#183919,
#183920,#183921,#183922),(#183923,#183924,#183925,#183926,#183927,#183928,
#183929,#183930,#183931),(#183932,#183933,#183934,#183935,#183936,#183937,
#183938,#183939,#183940),(#183941,#183942,#183943,#183944,#183945,#183946,
#183947,#183948,#183949),(#183950,#183951,#183952,#183953,#183954,#183955,
#183956,#183957,#183958),(#183959,#183960,#183961,#183962,#183963,#183964,
#183965,#183966,#183967),(#183968,#183969,#183970,#183971,#183972,#183973,
#183974,#183975,#183976),(#183977,#183978,#183979,#183980,#183981,#183982,
#183983,#183984,#183985),(#183986,#183987,#183988,#183989,#183990,#183991,
#183992,#183993,#183994),(#183995,#183996,#183997,#183998,#183999,#184000,
#184001,#184002,#184003),(#184004,#184005,#184006,#184007,#184008,#184009,
#184010,#184011,#184012),(#184013,#184014,#184015,#184016,#184017,#184018,
#184019,#184020,#184021),(#184022,#184023,#184024,#184025,#184026,#184027,
#184028,#184029,#184030),(#184031,#184032,#184033,#184034,#184035,#184036,
#184037,#184038,#184039),(#184040,#184041,#184042,#184043,#184044,#184045,
#184046,#184047,#184048),(#184049,#184050,#184051,#184052,#184053,#184054,
#184055,#184056,#184057),(#184058,#184059,#184060,#184061,#184062,#184063,
#184064,#184065,#184066),(#184067,#184068,#184069,#184070,#184071,#184072,
#184073,#184074,#184075),(#184076,#184077,#184078,#184079,#184080,#184081,
#184082,#184083,#184084),(#184085,#184086,#184087,#184088,#184089,#184090,
#184091,#184092,#184093),(#184094,#184095,#184096,#184097,#184098,#184099,
#184100,#184101,#184102),(#184103,#184104,#184105,#184106,#184107,#184108,
#184109,#184110,#184111),(#184112,#184113,#184114,#184115,#184116,#184117,
#184118,#184119,#184120),(#184121,#184122,#184123,#184124,#184125,#184126,
#184127,#184128,#184129),(#184130,#184131,#184132,#184133,#184134,#184135,
#184136,#184137,#184138),(#184139,#184140,#184141,#184142,#184143,#184144,
#184145,#184146,#184147),(#184148,#184149,#184150,#184151,#184152,#184153,
#184154,#184155,#184156),(#184157,#184158,#184159,#184160,#184161,#184162,
#184163,#184164,#184165),(#184166,#184167,#184168,#184169,#184170,#184171,
#184172,#184173,#184174),(#184175,#184176,#184177,#184178,#184179,#184180,
#184181,#184182,#184183),(#184184,#184185,#184186,#184187,#184188,#184189,
#184190,#184191,#184192),(#184193,#184194,#184195,#184196,#184197,#184198,
#184199,#184200,#184201),(#184202,#184203,#184204,#184205,#184206,#184207,
#184208,#184209,#184210),(#184211,#184212,#184213,#184214,#184215,#184216,
#184217,#184218,#184219),(#184220,#184221,#184222,#184223,#184224,#184225,
#184226,#184227,#184228),(#184229,#184230,#184231,#184232,#184233,#184234,
#184235,#184236,#184237),(#184238,#184239,#184240,#184241,#184242,#184243,
#184244,#184245,#184246),(#184247,#184248,#184249,#184250,#184251,#184252,
#184253,#184254,#184255),(#184256,#184257,#184258,#184259,#184260,#184261,
#184262,#184263,#184264),(#184265,#184266,#184267,#184268,#184269,#184270,
#184271,#184272,#184273),(#184274,#184275,#184276,#184277,#184278,#184279,
#184280,#184281,#184282),(#184283,#184284,#184285,#184286,#184287,#184288,
#184289,#184290,#184291),(#184292,#184293,#184294,#184295,#184296,#184297,
#184298,#184299,#184300),(#184301,#184302,#184303,#184304,#184305,#184306,
#184307,#184308,#184309),(#184310,#184311,#184312,#184313,#184314,#184315,
#184316,#184317,#184318),(#184319,#184320,#184321,#184322,#184323,#184324,
#184325,#184326,#184327),(#184328,#184329,#184330,#184331,#184332,#184333,
#184334,#184335,#184336),(#184337,#184338,#184339,#184340,#184341,#184342,
#184343,#184344,#184345),(#184346,#184347,#184348,#184349,#184350,#184351,
#184352,#184353,#184354),(#184355,#184356,#184357,#184358,#184359,#184360,
#184361,#184362,#184363),(#184364,#184365,#184366,#184367,#184368,#184369,
#184370,#184371,#184372),(#184373,#184374,#184375,#184376,#184377,#184378,
#184379,#184380,#184381),(#184382,#184383,#184384,#184385,#184386,#184387,
#184388,#184389,#184390),(#184391,#184392,#184393,#184394,#184395,#184396,
#184397,#184398,#184399),(#184400,#184401,#184402,#184403,#184404,#184405,
#184406,#184407,#184408),(#184409,#184410,#184411,#184412,#184413,#184414,
#184415,#184416,#184417),(#184418,#184419,#184420,#184421,#184422,#184423,
#184424,#184425,#184426),(#184427,#184428,#184429,#184430,#184431,#184432,
#184433,#184434,#184435),(#184436,#184437,#184438,#184439,#184440,#184441,
#184442,#184443,#184444),(#184445,#184446,#184447,#184448,#184449,#184450,
#184451,#184452,#184453),(#184454,#184455,#184456,#184457,#184458,#184459,
#184460,#184461,#184462),(#184463,#184464,#184465,#184466,#184467,#184468,
#184469,#184470,#184471),(#184472,#184473,#184474,#184475,#184476,#184477,
#184478,#184479,#184480),(#184481,#184482,#184483,#184484,#184485,#184486,
#184487,#184488,#184489),(#184490,#184491,#184492,#184493,#184494,#184495,
#184496,#184497,#184498),(#184499,#184500,#184501,#184502,#184503,#184504,
#184505,#184506,#184507),(#184508,#184509,#184510,#184511,#184512,#184513,
#184514,#184515,#184516),(#184517,#184518,#184519,#184520,#184521,#184522,
#184523,#184524,#184525),(#184526,#184527,#184528,#184529,#184530,#184531,
#184532,#184533,#184534),(#184535,#184536,#184537,#184538,#184539,#184540,
#184541,#184542,#184543),(#184544,#184545,#184546,#184547,#184548,#184549,
#184550,#184551,#184552),(#184553,#184554,#184555,#184556,#184557,#184558,
#184559,#184560,#184561),(#184562,#184563,#184564,#184565,#184566,#184567,
#184568,#184569,#184570),(#184571,#184572,#184573,#184574,#184575,#184576,
#184577,#184578,#184579),(#184580,#184581,#184582,#184583,#184584,#184585,
#184586,#184587,#184588),(#184589,#184590,#184591,#184592,#184593,#184594,
#184595,#184596,#184597),(#184598,#184599,#184600,#184601,#184602,#184603,
#184604,#184605,#184606),(#184607,#184608,#184609,#184610,#184611,#184612,
#184613,#184614,#184615),(#184616,#184617,#184618,#184619,#184620,#184621,
#184622,#184623,#184624),(#184625,#184626,#184627,#184628,#184629,#184630,
#184631,#184632,#184633),(#184634,#184635,#184636,#184637,#184638,#184639,
#184640,#184641,#184642),(#184643,#184644,#184645,#184646,#184647,#184648,
#184649,#184650,#184651),(#184652,#184653,#184654,#184655,#184656,#184657,
#184658,#184659,#184660),(#184661,#184662,#184663,#184664,#184665,#184666,
#184667,#184668,#184669),(#184670,#184671,#184672,#184673,#184674,#184675,
#184676,#184677,#184678),(#184679,#184680,#184681,#184682,#184683,#184684,
#184685,#184686,#184687),(#184688,#184689,#184690,#184691,#184692,#184693,
#184694,#184695,#184696),(#184697,#184698,#184699,#184700,#184701,#184702,
#184703,#184704,#184705),(#184706,#184707,#184708,#184709,#184710,#184711,
#184712,#184713,#184714),(#184715,#184716,#184717,#184718,#184719,#184720,
#184721,#184722,#184723),(#184724,#184725,#184726,#184727,#184728,#184729,
#184730,#184731,#184732),(#184733,#184734,#184735,#184736,#184737,#184738,
#184739,#184740,#184741),(#184742,#184743,#184744,#184745,#184746,#184747,
#184748,#184749,#184750),(#184751,#184752,#184753,#184754,#184755,#184756,
#184757,#184758,#184759),(#184760,#184761,#184762,#184763,#184764,#184765,
#184766,#184767,#184768),(#184769,#184770,#184771,#184772,#184773,#184774,
#184775,#184776,#184777),(#184778,#184779,#184780,#184781,#184782,#184783,
#184784,#184785,#184786),(#184787,#184788,#184789,#184790,#184791,#184792,
#184793,#184794,#184795),(#184796,#184797,#184798,#184799,#184800,#184801,
#184802,#184803,#184804),(#184805,#184806,#184807,#184808,#184809,#184810,
#184811,#184812,#184813),(#184814,#184815,#184816,#184817,#184818,#184819,
#184820,#184821,#184822),(#184823,#184824,#184825,#184826,#184827,#184828,
#184829,#184830,#184831),(#184832,#184833,#184834,#184835,#184836,#184837,
#184838,#184839,#184840),(#184841,#184842,#184843,#184844,#184845,#184846,
#184847,#184848,#184849),(#184850,#184851,#184852,#184853,#184854,#184855,
#184856,#184857,#184858),(#184859,#184860,#184861,#184862,#184863,#184864,
#184865,#184866,#184867),(#184868,#184869,#184870,#184871,#184872,#184873,
#184874,#184875,#184876),(#184877,#184878,#184879,#184880,#184881,#184882,
#184883,#184884,#184885),(#184886,#184887,#184888,#184889,#184890,#184891,
#184892,#184893,#184894),(#184895,#184896,#184897,#184898,#184899,#184900,
#184901,#184902,#184903),(#184904,#184905,#184906,#184907,#184908,#184909,
#184910,#184911,#184912),(#184913,#184914,#184915,#184916,#184917,#184918,
#184919,#184920,#184921),(#184922,#184923,#184924,#184925,#184926,#184927,
#184928,#184929,#184930),(#184931,#184932,#184933,#184934,#184935,#184936,
#184937,#184938,#184939),(#184940,#184941,#184942,#184943,#184944,#184945,
#184946,#184947,#184948),(#184949,#184950,#184951,#184952,#184953,#184954,
#184955,#184956,#184957),(#184958,#184959,#184960,#184961,#184962,#184963,
#184964,#184965,#184966),(#184967,#184968,#184969,#184970,#184971,#184972,
#184973,#184974,#184975),(#184976,#184977,#184978,#184979,#184980,#184981,
#184982,#184983,#184984),(#184985,#184986,#184987,#184988,#184989,#184990,
#184991,#184992,#184993),(#184994,#184995,#184996,#184997,#184998,#184999,
#185000,#185001,#185002),(#185003,#185004,#185005,#185006,#185007,#185008,
#185009,#185010,#185011),(#185012,#185013,#185014,#185015,#185016,#185017,
#185018,#185019,#185020),(#185021,#185022,#185023,#185024,#185025,#185026,
#185027,#185028,#185029),(#185030,#185031,#185032,#185033,#185034,#185035,
#185036,#185037,#185038),(#185039,#185040,#185041,#185042,#185043,#185044,
#185045,#185046,#185047),(#185048,#185049,#185050,#185051,#185052,#185053,
#185054,#185055,#185056),(#185057,#185058,#185059,#185060,#185061,#185062,
#185063,#185064,#185065),(#185066,#185067,#185068,#185069,#185070,#185071,
#185072,#185073,#185074),(#185075,#185076,#185077,#185078,#185079,#185080,
#185081,#185082,#185083),(#185084,#185085,#185086,#185087,#185088,#185089,
#185090,#185091,#185092),(#185093,#185094,#185095,#185096,#185097,#185098,
#185099,#185100,#185101),(#185102,#185103,#185104,#185105,#185106,#185107,
#185108,#185109,#185110),(#185111,#185112,#185113,#185114,#185115,#185116,
#185117,#185118,#185119),(#185120,#185121,#185122,#185123,#185124,#185125,
#185126,#185127,#185128),(#185129,#185130,#185131,#185132,#185133,#185134,
#185135,#185136,#185137),(#185138,#185139,#185140,#185141,#185142,#185143,
#185144,#185145,#185146),(#185147,#185148,#185149,#185150,#185151,#185152,
#185153,#185154,#185155),(#185156,#185157,#185158,#185159,#185160,#185161,
#185162,#185163,#185164),(#185165,#185166,#185167,#185168,#185169,#185170,
#185171,#185172,#185173),(#185174,#185175,#185176,#185177,#185178,#185179,
#185180,#185181,#185182),(#185183,#185184,#185185,#185186,#185187,#185188,
#185189,#185190,#185191),(#185192,#185193,#185194,#185195,#185196,#185197,
#185198,#185199,#185200),(#185201,#185202,#185203,#185204,#185205,#185206,
#185207,#185208,#185209),(#185210,#185211,#185212,#185213,#185214,#185215,
#185216,#185217,#185218),(#185219,#185220,#185221,#185222,#185223,#185224,
#185225,#185226,#185227),(#185228,#185229,#185230,#185231,#185232,#185233,
#185234,#185235,#185236),(#185237,#185238,#185239,#185240,#185241,#185242,
#185243,#185244,#185245),(#185246,#185247,#185248,#185249,#185250,#185251,
#185252,#185253,#185254),(#185255,#185256,#185257,#185258,#185259,#185260,
#185261,#185262,#185263),(#185264,#185265,#185266,#185267,#185268,#185269,
#185270,#185271,#185272),(#185273,#185274,#185275,#185276,#185277,#185278,
#185279,#185280,#185281),(#185282,#185283,#185284,#185285,#185286,#185287,
#185288,#185289,#185290),(#185291,#185292,#185293,#185294,#185295,#185296,
#185297,#185298,#185299),(#185300,#185301,#185302,#185303,#185304,#185305,
#185306,#185307,#185308),(#185309,#185310,#185311,#185312,#185313,#185314,
#185315,#185316,#185317),(#185318,#185319,#185320,#185321,#185322,#185323,
#185324,#185325,#185326),(#185327,#185328,#185329,#185330,#185331,#185332,
#185333,#185334,#185335),(#185336,#185337,#185338,#185339,#185340,#185341,
#185342,#185343,#185344),(#185345,#185346,#185347,#185348,#185349,#185350,
#185351,#185352,#185353),(#185354,#185355,#185356,#185357,#185358,#185359,
#185360,#185361,#185362),(#185363,#185364,#185365,#185366,#185367,#185368,
#185369,#185370,#185371),(#185372,#185373,#185374,#185375,#185376,#185377,
#185378,#185379,#185380),(#185381,#185382,#185383,#185384,#185385,#185386,
#185387,#185388,#185389),(#185390,#185391,#185392,#185393,#185394,#185395,
#185396,#185397,#185398),(#185399,#185400,#185401,#185402,#185403,#185404,
#185405,#185406,#185407),(#185408,#185409,#185410,#185411,#185412,#185413,
#185414,#185415,#185416),(#185417,#185418,#185419,#185420,#185421,#185422,
#185423,#185424,#185425),(#185426,#185427,#185428,#185429,#185430,#185431,
#185432,#185433,#185434),(#185435,#185436,#185437,#185438,#185439,#185440,
#185441,#185442,#185443),(#185444,#185445,#185446,#185447,#185448,#185449,
#185450,#185451,#185452),(#185453,#185454,#185455,#185456,#185457,#185458,
#185459,#185460,#185461),(#185462,#185463,#185464,#185465,#185466,#185467,
#185468,#185469,#185470),(#185471,#185472,#185473,#185474,#185475,#185476,
#185477,#185478,#185479),(#185480,#185481,#185482,#185483,#185484,#185485,
#185486,#185487,#185488),(#185489,#185490,#185491,#185492,#185493,#185494,
#185495,#185496,#185497),(#185498,#185499,#185500,#185501,#185502,#185503,
#185504,#185505,#185506),(#185507,#185508,#185509,#185510,#185511,#185512,
#185513,#185514,#185515),(#185516,#185517,#185518,#185519,#185520,#185521,
#185522,#185523,#185524),(#185525,#185526,#185527,#185528,#185529,#185530,
#185531,#185532,#185533),(#185534,#185535,#185536,#185537,#185538,#185539,
#185540,#185541,#185542),(#185543,#185544,#185545,#185546,#185547,#185548,
#185549,#185550,#185551),(#185552,#185553,#185554,#185555,#185556,#185557,
#185558,#185559,#185560),(#185561,#185562,#185563,#185564,#185565,#185566,
#185567,#185568,#185569),(#185570,#185571,#185572,#185573,#185574,#185575,
#185576,#185577,#185578),(#185579,#185580,#185581,#185582,#185583,#185584,
#185585,#185586,#185587),(#185588,#185589,#185590,#185591,#185592,#185593,
#185594,#185595,#185596),(#185597,#185598,#185599,#185600,#185601,#185602,
#185603,#185604,#185605),(#185606,#185607,#185608,#185609,#185610,#185611,
#185612,#185613,#185614),(#185615,#185616,#185617,#185618,#185619,#185620,
#185621,#185622,#185623),(#185624,#185625,#185626,#185627,#185628,#185629,
#185630,#185631,#185632),(#185633,#185634,#185635,#185636,#185637,#185638,
#185639,#185640,#185641),(#185642,#185643,#185644,#185645,#185646,#185647,
#185648,#185649,#185650),(#185651,#185652,#185653,#185654,#185655,#185656,
#185657,#185658,#185659),(#185660,#185661,#185662,#185663,#185664,#185665,
#185666,#185667,#185668),(#185669,#185670,#185671,#185672,#185673,#185674,
#185675,#185676,#185677),(#185678,#185679,#185680,#185681,#185682,#185683,
#185684,#185685,#185686),(#185687,#185688,#185689,#185690,#185691,#185692,
#185693,#185694,#185695),(#185696,#185697,#185698,#185699,#185700,#185701,
#185702,#185703,#185704),(#185705,#185706,#185707,#185708,#185709,#185710,
#185711,#185712,#185713),(#185714,#185715,#185716,#185717,#185718,#185719,
#185720,#185721,#185722),(#185723,#185724,#185725,#185726,#185727,#185728,
#185729,#185730,#185731),(#185732,#185733,#185734,#185735,#185736,#185737,
#185738,#185739,#185740),(#185741,#185742,#185743,#185744,#185745,#185746,
#185747,#185748,#185749),(#185750,#185751,#185752,#185753,#185754,#185755,
#185756,#185757,#185758),(#185759,#185760,#185761,#185762,#185763,#185764,
#185765,#185766,#185767),(#185768,#185769,#185770,#185771,#185772,#185773,
#185774,#185775,#185776),(#185777,#185778,#185779,#185780,#185781,#185782,
#185783,#185784,#185785),(#185786,#185787,#185788,#185789,#185790,#185791,
#185792,#185793,#185794),(#185795,#185796,#185797,#185798,#185799,#185800,
#185801,#185802,#185803),(#185804,#185805,#185806,#185807,#185808,#185809,
#185810,#185811,#185812),(#185813,#185814,#185815,#185816,#185817,#185818,
#185819,#185820,#185821),(#185822,#185823,#185824,#185825,#185826,#185827,
#185828,#185829,#185830),(#185831,#185832,#185833,#185834,#185835,#185836,
#185837,#185838,#185839),(#185840,#185841,#185842,#185843,#185844,#185845,
#185846,#185847,#185848),(#185849,#185850,#185851,#185852,#185853,#185854,
#185855,#185856,#185857),(#185858,#185859,#185860,#185861,#185862,#185863,
#185864,#185865,#185866),(#185867,#185868,#185869,#185870,#185871,#185872,
#185873,#185874,#185875),(#185876,#185877,#185878,#185879,#185880,#185881,
#185882,#185883,#185884),(#185885,#185886,#185887,#185888,#185889,#185890,
#185891,#185892,#185893),(#185894,#185895,#185896,#185897,#185898,#185899,
#185900,#185901,#185902),(#185903,#185904,#185905,#185906,#185907,#185908,
#185909,#185910,#185911),(#185912,#185913,#185914,#185915,#185916,#185917,
#185918,#185919,#185920),(#185921,#185922,#185923,#185924,#185925,#185926,
#185927,#185928,#185929),(#185930,#185931,#185932,#185933,#185934,#185935,
#185936,#185937,#185938),(#185939,#185940,#185941,#185942,#185943,#185944,
#185945,#185946,#185947),(#185948,#185949,#185950,#185951,#185952,#185953,
#185954,#185955,#185956),(#185957,#185958,#185959,#185960,#185961,#185962,
#185963,#185964,#185965),(#185966,#185967,#185968,#185969,#185970,#185971,
#185972,#185973,#185974),(#185975,#185976,#185977,#185978,#185979,#185980,
#185981,#185982,#185983),(#185984,#185985,#185986,#185987,#185988,#185989,
#185990,#185991,#185992),(#185993,#185994,#185995,#185996,#185997,#185998,
#185999,#186000,#186001),(#186002,#186003,#186004,#186005,#186006,#186007,
#186008,#186009,#186010),(#186011,#186012,#186013,#186014,#186015,#186016,
#186017,#186018,#186019),(#186020,#186021,#186022,#186023,#186024,#186025,
#186026,#186027,#186028),(#186029,#186030,#186031,#186032,#186033,#186034,
#186035,#186036,#186037),(#186038,#186039,#186040,#186041,#186042,#186043,
#186044,#186045,#186046),(#186047,#186048,#186049,#186050,#186051,#186052,
#186053,#186054,#186055),(#186056,#186057,#186058,#186059,#186060,#186061,
#186062,#186063,#186064),(#186065,#186066,#186067,#186068,#186069,#186070,
#186071,#186072,#186073),(#186074,#186075,#186076,#186077,#186078,#186079,
#186080,#186081,#186082),(#186083,#186084,#186085,#186086,#186087,#186088,
#186089,#186090,#186091),(#186092,#186093,#186094,#186095,#186096,#186097,
#186098,#186099,#186100),(#186101,#186102,#186103,#186104,#186105,#186106,
#186107,#186108,#186109),(#186110,#186111,#186112,#186113,#186114,#186115,
#186116,#186117,#186118),(#186119,#186120,#186121,#186122,#186123,#186124,
#186125,#186126,#186127),(#186128,#186129,#186130,#186131,#186132,#186133,
#186134,#186135,#186136),(#186137,#186138,#186139,#186140,#186141,#186142,
#186143,#186144,#186145),(#186146,#186147,#186148,#186149,#186150,#186151,
#186152,#186153,#186154),(#186155,#186156,#186157,#186158,#186159,#186160,
#186161,#186162,#186163),(#186164,#186165,#186166,#186167,#186168,#186169,
#186170,#186171,#186172),(#186173,#186174,#186175,#186176,#186177,#186178,
#186179,#186180,#186181),(#186182,#186183,#186184,#186185,#186186,#186187,
#186188,#186189,#186190),(#186191,#186192,#186193,#186194,#186195,#186196,
#186197,#186198,#186199),(#186200,#186201,#186202,#186203,#186204,#186205,
#186206,#186207,#186208),(#186209,#186210,#186211,#186212,#186213,#186214,
#186215,#186216,#186217),(#186218,#186219,#186220,#186221,#186222,#186223,
#186224,#186225,#186226),(#186227,#186228,#186229,#186230,#186231,#186232,
#186233,#186234,#186235),(#186236,#186237,#186238,#186239,#186240,#186241,
#186242,#186243,#186244),(#186245,#186246,#186247,#186248,#186249,#186250,
#186251,#186252,#186253),(#186254,#186255,#186256,#186257,#186258,#186259,
#186260,#186261,#186262),(#186263,#186264,#186265,#186266,#186267,#186268,
#186269,#186270,#186271),(#186272,#186273,#186274,#186275,#186276,#186277,
#186278,#186279,#186280),(#186281,#186282,#186283,#186284,#186285,#186286,
#186287,#186288,#186289),(#186290,#186291,#186292,#186293,#186294,#186295,
#186296,#186297,#186298),(#186299,#186300,#186301,#186302,#186303,#186304,
#186305,#186306,#186307),(#186308,#186309,#186310,#186311,#186312,#186313,
#186314,#186315,#186316),(#186317,#186318,#186319,#186320,#186321,#186322,
#186323,#186324,#186325),(#186326,#186327,#186328,#186329,#186330,#186331,
#186332,#186333,#186334),(#186335,#186336,#186337,#186338,#186339,#186340,
#186341,#186342,#186343),(#186344,#186345,#186346,#186347,#186348,#186349,
#186350,#186351,#186352),(#186353,#186354,#186355,#186356,#186357,#186358,
#186359,#186360,#186361),(#186362,#186363,#186364,#186365,#186366,#186367,
#186368,#186369,#186370),(#186371,#186372,#186373,#186374,#186375,#186376,
#186377,#186378,#186379),(#186380,#186381,#186382,#186383,#186384,#186385,
#186386,#186387,#186388),(#186389,#186390,#186391,#186392,#186393,#186394,
#186395,#186396,#186397),(#186398,#186399,#186400,#186401,#186402,#186403,
#186404,#186405,#186406),(#186407,#186408,#186409,#186410,#186411,#186412,
#186413,#186414,#186415),(#186416,#186417,#186418,#186419,#186420,#186421,
#186422,#186423,#186424),(#186425,#186426,#186427,#186428,#186429,#186430,
#186431,#186432,#186433),(#186434,#186435,#186436,#186437,#186438,#186439,
#186440,#186441,#186442),(#186443,#186444,#186445,#186446,#186447,#186448,
#186449,#186450,#186451),(#186452,#186453,#186454,#186455,#186456,#186457,
#186458,#186459,#186460),(#186461,#186462,#186463,#186464,#186465,#186466,
#186467,#186468,#186469),(#186470,#186471,#186472,#186473,#186474,#186475,
#186476,#186477,#186478),(#186479,#186480,#186481,#186482,#186483,#186484,
#186485,#186486,#186487),(#186488,#186489,#186490,#186491,#186492,#186493,
#186494,#186495,#186496),(#186497,#186498,#186499,#186500,#186501,#186502,
#186503,#186504,#186505),(#186506,#186507,#186508,#186509,#186510,#186511,
#186512,#186513,#186514),(#186515,#186516,#186517,#186518,#186519,#186520,
#186521,#186522,#186523),(#186524,#186525,#186526,#186527,#186528,#186529,
#186530,#186531,#186532),(#186533,#186534,#186535,#186536,#186537,#186538,
#186539,#186540,#186541),(#186542,#186543,#186544,#186545,#186546,#186547,
#186548,#186549,#186550),(#186551,#186552,#186553,#186554,#186555,#186556,
#186557,#186558,#186559),(#186560,#186561,#186562,#186563,#186564,#186565,
#186566,#186567,#186568),(#186569,#186570,#186571,#186572,#186573,#186574,
#186575,#186576,#186577),(#186578,#186579,#186580,#186581,#186582,#186583,
#186584,#186585,#186586),(#186587,#186588,#186589,#186590,#186591,#186592,
#186593,#186594,#186595),(#186596,#186597,#186598,#186599,#186600,#186601,
#186602,#186603,#186604),(#186605,#186606,#186607,#186608,#186609,#186610,
#186611,#186612,#186613),(#186614,#186615,#186616,#186617,#186618,#186619,
#186620,#186621,#186622),(#186623,#186624,#186625,#186626,#186627,#186628,
#186629,#186630,#186631),(#186632,#186633,#186634,#186635,#186636,#186637,
#186638,#186639,#186640),(#186641,#186642,#186643,#186644,#186645,#186646,
#186647,#186648,#186649),(#186650,#186651,#186652,#186653,#186654,#186655,
#186656,#186657,#186658),(#186659,#186660,#186661,#186662,#186663,#186664,
#186665,#186666,#186667),(#186668,#186669,#186670,#186671,#186672,#186673,
#186674,#186675,#186676),(#186677,#186678,#186679,#186680,#186681,#186682,
#186683,#186684,#186685),(#186686,#186687,#186688,#186689,#186690,#186691,
#186692,#186693,#186694),(#186695,#186696,#186697,#186698,#186699,#186700,
#186701,#186702,#186703),(#186704,#186705,#186706,#186707,#186708,#186709,
#186710,#186711,#186712),(#186713,#186714,#186715,#186716,#186717,#186718,
#186719,#186720,#186721),(#186722,#186723,#186724,#186725,#186726,#186727,
#186728,#186729,#186730),(#186731,#186732,#186733,#186734,#186735,#186736,
#186737,#186738,#186739),(#186740,#186741,#186742,#186743,#186744,#186745,
#186746,#186747,#186748),(#186749,#186750,#186751,#186752,#186753,#186754,
#186755,#186756,#186757),(#186758,#186759,#186760,#186761,#186762,#186763,
#186764,#186765,#186766),(#186767,#186768,#186769,#186770,#186771,#186772,
#186773,#186774,#186775),(#186776,#186777,#186778,#186779,#186780,#186781,
#186782,#186783,#186784),(#186785,#186786,#186787,#186788,#186789,#186790,
#186791,#186792,#186793),(#186794,#186795,#186796,#186797,#186798,#186799,
#186800,#186801,#186802),(#186803,#186804,#186805,#186806,#186807,#186808,
#186809,#186810,#186811),(#186812,#186813,#186814,#186815,#186816,#186817,
#186818,#186819,#186820),(#186821,#186822,#186823,#186824,#186825,#186826,
#186827,#186828,#186829),(#186830,#186831,#186832,#186833,#186834,#186835,
#186836,#186837,#186838),(#186839,#186840,#186841,#186842,#186843,#186844,
#186845,#186846,#186847),(#186848,#186849,#186850,#186851,#186852,#186853,
#186854,#186855,#186856),(#186857,#186858,#186859,#186860,#186861,#186862,
#186863,#186864,#186865),(#186866,#186867,#186868,#186869,#186870,#186871,
#186872,#186873,#186874),(#186875,#186876,#186877,#186878,#186879,#186880,
#186881,#186882,#186883),(#186884,#186885,#186886,#186887,#186888,#186889,
#186890,#186891,#186892),(#186893,#186894,#186895,#186896,#186897,#186898,
#186899,#186900,#186901),(#186902,#186903,#186904,#186905,#186906,#186907,
#186908,#186909,#186910),(#186911,#186912,#186913,#186914,#186915,#186916,
#186917,#186918,#186919),(#186920,#186921,#186922,#186923,#186924,#186925,
#186926,#186927,#186928),(#186929,#186930,#186931,#186932,#186933,#186934,
#186935,#186936,#186937),(#186938,#186939,#186940,#186941,#186942,#186943,
#186944,#186945,#186946),(#186947,#186948,#186949,#186950,#186951,#186952,
#186953,#186954,#186955),(#186956,#186957,#186958,#186959,#186960,#186961,
#186962,#186963,#186964),(#186965,#186966,#186967,#186968,#186969,#186970,
#186971,#186972,#186973),(#186974,#186975,#186976,#186977,#186978,#186979,
#186980,#186981,#186982),(#186983,#186984,#186985,#186986,#186987,#186988,
#186989,#186990,#186991),(#186992,#186993,#186994,#186995,#186996,#186997,
#186998,#186999,#187000),(#187001,#187002,#187003,#187004,#187005,#187006,
#187007,#187008,#187009),(#187010,#187011,#187012,#187013,#187014,#187015,
#187016,#187017,#187018),(#187019,#187020,#187021,#187022,#187023,#187024,
#187025,#187026,#187027),(#187028,#187029,#187030,#187031,#187032,#187033,
#187034,#187035,#187036),(#187037,#187038,#187039,#187040,#187041,#187042,
#187043,#187044,#187045),(#187046,#187047,#187048,#187049,#187050,#187051,
#187052,#187053,#187054),(#187055,#187056,#187057,#187058,#187059,#187060,
#187061,#187062,#187063),(#187064,#187065,#187066,#187067,#187068,#187069,
#187070,#187071,#187072),(#187073,#187074,#187075,#187076,#187077,#187078,
#187079,#187080,#187081),(#187082,#187083,#187084,#187085,#187086,#187087,
#187088,#187089,#187090),(#187091,#187092,#187093,#187094,#187095,#187096,
#187097,#187098,#187099),(#187100,#187101,#187102,#187103,#187104,#187105,
#187106,#187107,#187108),(#187109,#187110,#187111,#187112,#187113,#187114,
#187115,#187116,#187117),(#187118,#187119,#187120,#187121,#187122,#187123,
#187124,#187125,#187126),(#187127,#187128,#187129,#187130,#187131,#187132,
#187133,#187134,#187135),(#187136,#187137,#187138,#187139,#187140,#187141,
#187142,#187143,#187144),(#187145,#187146,#187147,#187148,#187149,#187150,
#187151,#187152,#187153),(#187154,#187155,#187156,#187157,#187158,#187159,
#187160,#187161,#187162),(#187163,#187164,#187165,#187166,#187167,#187168,
#187169,#187170,#187171),(#187172,#187173,#187174,#187175,#187176,#187177,
#187178,#187179,#187180),(#187181,#187182,#187183,#187184,#187185,#187186,
#187187,#187188,#187189),(#187190,#187191,#187192,#187193,#187194,#187195,
#187196,#187197,#187198),(#187199,#187200,#187201,#187202,#187203,#187204,
#187205,#187206,#187207),(#187208,#187209,#187210,#187211,#187212,#187213,
#187214,#187215,#187216),(#187217,#187218,#187219,#187220,#187221,#187222,
#187223,#187224,#187225),(#187226,#187227,#187228,#187229,#187230,#187231,
#187232,#187233,#187234),(#187235,#187236,#187237,#187238,#187239,#187240,
#187241,#187242,#187243),(#187244,#187245,#187246,#187247,#187248,#187249,
#187250,#187251,#187252),(#187253,#187254,#187255,#187256,#187257,#187258,
#187259,#187260,#187261),(#187262,#187263,#187264,#187265,#187266,#187267,
#187268,#187269,#187270),(#187271,#187272,#187273,#187274,#187275,#187276,
#187277,#187278,#187279),(#187280,#187281,#187282,#187283,#187284,#187285,
#187286,#187287,#187288),(#187289,#187290,#187291,#187292,#187293,#187294,
#187295,#187296,#187297),(#187298,#187299,#187300,#187301,#187302,#187303,
#187304,#187305,#187306),(#187307,#187308,#187309,#187310,#187311,#187312,
#187313,#187314,#187315),(#187316,#187317,#187318,#187319,#187320,#187321,
#187322,#187323,#187324),(#187325,#187326,#187327,#187328,#187329,#187330,
#187331,#187332,#187333),(#187334,#187335,#187336,#187337,#187338,#187339,
#187340,#187341,#187342),(#187343,#187344,#187345,#187346,#187347,#187348,
#187349,#187350,#187351),(#187352,#187353,#187354,#187355,#187356,#187357,
#187358,#187359,#187360),(#187361,#187362,#187363,#187364,#187365,#187366,
#187367,#187368,#187369),(#187370,#187371,#187372,#187373,#187374,#187375,
#187376,#187377,#187378),(#187379,#187380,#187381,#187382,#187383,#187384,
#187385,#187386,#187387),(#187388,#187389,#187390,#187391,#187392,#187393,
#187394,#187395,#187396),(#187397,#187398,#187399,#187400,#187401,#187402,
#187403,#187404,#187405),(#187406,#187407,#187408,#187409,#187410,#187411,
#187412,#187413,#187414),(#187415,#187416,#187417,#187418,#187419,#187420,
#187421,#187422,#187423),(#187424,#187425,#187426,#187427,#187428,#187429,
#187430,#187431,#187432),(#187433,#187434,#187435,#187436,#187437,#187438,
#187439,#187440,#187441),(#187442,#187443,#187444,#187445,#187446,#187447,
#187448,#187449,#187450),(#187451,#187452,#187453,#187454,#187455,#187456,
#187457,#187458,#187459),(#187460,#187461,#187462,#187463,#187464,#187465,
#187466,#187467,#187468),(#187469,#187470,#187471,#187472,#187473,#187474,
#187475,#187476,#187477),(#187478,#187479,#187480,#187481,#187482,#187483,
#187484,#187485,#187486),(#187487,#187488,#187489,#187490,#187491,#187492,
#187493,#187494,#187495),(#187496,#187497,#187498,#187499,#187500,#187501,
#187502,#187503,#187504),(#187505,#187506,#187507,#187508,#187509,#187510,
#187511,#187512,#187513),(#187514,#187515,#187516,#187517,#187518,#187519,
#187520,#187521,#187522),(#187523,#187524,#187525,#187526,#187527,#187528,
#187529,#187530,#187531),(#187532,#187533,#187534,#187535,#187536,#187537,
#187538,#187539,#187540),(#187541,#187542,#187543,#187544,#187545,#187546,
#187547,#187548,#187549),(#187550,#187551,#187552,#187553,#187554,#187555,
#187556,#187557,#187558),(#187559,#187560,#187561,#187562,#187563,#187564,
#187565,#187566,#187567),(#187568,#187569,#187570,#187571,#187572,#187573,
#187574,#187575,#187576),(#187577,#187578,#187579,#187580,#187581,#187582,
#187583,#187584,#187585),(#187586,#187587,#187588,#187589,#187590,#187591,
#187592,#187593,#187594),(#187595,#187596,#187597,#187598,#187599,#187600,
#187601,#187602,#187603),(#187604,#187605,#187606,#187607,#187608,#187609,
#187610,#187611,#187612),(#187613,#187614,#187615,#187616,#187617,#187618,
#187619,#187620,#187621),(#187622,#187623,#187624,#187625,#187626,#187627,
#187628,#187629,#187630),(#187631,#187632,#187633,#187634,#187635,#187636,
#187637,#187638,#187639),(#187640,#187641,#187642,#187643,#187644,#187645,
#187646,#187647,#187648),(#187649,#187650,#187651,#187652,#187653,#187654,
#187655,#187656,#187657),(#187658,#187659,#187660,#187661,#187662,#187663,
#187664,#187665,#187666),(#187667,#187668,#187669,#187670,#187671,#187672,
#187673,#187674,#187675),(#187676,#187677,#187678,#187679,#187680,#187681,
#187682,#187683,#187684),(#187685,#187686,#187687,#187688,#187689,#187690,
#187691,#187692,#187693),(#187694,#187695,#187696,#187697,#187698,#187699,
#187700,#187701,#187702),(#187703,#187704,#187705,#187706,#187707,#187708,
#187709,#187710,#187711),(#187712,#187713,#187714,#187715,#187716,#187717,
#187718,#187719,#187720),(#187721,#187722,#187723,#187724,#187725,#187726,
#187727,#187728,#187729),(#187730,#187731,#187732,#187733,#187734,#187735,
#187736,#187737,#187738),(#187739,#187740,#187741,#187742,#187743,#187744,
#187745,#187746,#187747),(#187748,#187749,#187750,#187751,#187752,#187753,
#187754,#187755,#187756),(#187757,#187758,#187759,#187760,#187761,#187762,
#187763,#187764,#187765),(#187766,#187767,#187768,#187769,#187770,#187771,
#187772,#187773,#187774),(#187775,#187776,#187777,#187778,#187779,#187780,
#187781,#187782,#187783),(#187784,#187785,#187786,#187787,#187788,#187789,
#187790,#187791,#187792),(#187793,#187794,#187795,#187796,#187797,#187798,
#187799,#187800,#187801),(#187802,#187803,#187804,#187805,#187806,#187807,
#187808,#187809,#187810),(#187811,#187812,#187813,#187814,#187815,#187816,
#187817,#187818,#187819),(#187820,#187821,#187822,#187823,#187824,#187825,
#187826,#187827,#187828),(#187829,#187830,#187831,#187832,#187833,#187834,
#187835,#187836,#187837),(#187838,#187839,#187840,#187841,#187842,#187843,
#187844,#187845,#187846),(#187847,#187848,#187849,#187850,#187851,#187852,
#187853,#187854,#187855),(#187856,#187857,#187858,#187859,#187860,#187861,
#187862,#187863,#187864),(#187865,#187866,#187867,#187868,#187869,#187870,
#187871,#187872,#187873),(#187874,#187875,#187876,#187877,#187878,#187879,
#187880,#187881,#187882),(#187883,#187884,#187885,#187886,#187887,#187888,
#187889,#187890,#187891),(#187892,#187893,#187894,#187895,#187896,#187897,
#187898,#187899,#187900),(#187901,#187902,#187903,#187904,#187905,#187906,
#187907,#187908,#187909),(#187910,#187911,#187912,#187913,#187914,#187915,
#187916,#187917,#187918),(#187919,#187920,#187921,#187922,#187923,#187924,
#187925,#187926,#187927),(#187928,#187929,#187930,#187931,#187932,#187933,
#187934,#187935,#187936),(#187937,#187938,#187939,#187940,#187941,#187942,
#187943,#187944,#187945),(#187946,#187947,#187948,#187949,#187950,#187951,
#187952,#187953,#187954),(#187955,#187956,#187957,#187958,#187959,#187960,
#187961,#187962,#187963),(#187964,#187965,#187966,#187967,#187968,#187969,
#187970,#187971,#187972),(#187973,#187974,#187975,#187976,#187977,#187978,
#187979,#187980,#187981),(#187982,#187983,#187984,#187985,#187986,#187987,
#187988,#187989,#187990),(#187991,#187992,#187993,#187994,#187995,#187996,
#187997,#187998,#187999),(#188000,#188001,#188002,#188003,#188004,#188005,
#188006,#188007,#188008),(#188009,#188010,#188011,#188012,#188013,#188014,
#188015,#188016,#188017),(#188018,#188019,#188020,#188021,#188022,#188023,
#188024,#188025,#188026),(#188027,#188028,#188029,#188030,#188031,#188032,
#188033,#188034,#188035),(#188036,#188037,#188038,#188039,#188040,#188041,
#188042,#188043,#188044),(#188045,#188046,#188047,#188048,#188049,#188050,
#188051,#188052,#188053),(#188054,#188055,#188056,#188057,#188058,#188059,
#188060,#188061,#188062),(#188063,#188064,#188065,#188066,#188067,#188068,
#188069,#188070,#188071),(#188072,#188073,#188074,#188075,#188076,#188077,
#188078,#188079,#188080),(#188081,#188082,#188083,#188084,#188085,#188086,
#188087,#188088,#188089),(#188090,#188091,#188092,#188093,#188094,#188095,
#188096,#188097,#188098),(#188099,#188100,#188101,#188102,#188103,#188104,
#188105,#188106,#188107),(#188108,#188109,#188110,#188111,#188112,#188113,
#188114,#188115,#188116),(#188117,#188118,#188119,#188120,#188121,#188122,
#188123,#188124,#188125),(#188126,#188127,#188128,#188129,#188130,#188131,
#188132,#188133,#188134),(#188135,#188136,#188137,#188138,#188139,#188140,
#188141,#188142,#188143),(#188144,#188145,#188146,#188147,#188148,#188149,
#188150,#188151,#188152),(#188153,#188154,#188155,#188156,#188157,#188158,
#188159,#188160,#188161),(#188162,#188163,#188164,#188165,#188166,#188167,
#188168,#188169,#188170),(#188171,#188172,#188173,#188174,#188175,#188176,
#188177,#188178,#188179),(#188180,#188181,#188182,#188183,#188184,#188185,
#188186,#188187,#188188),(#188189,#188190,#188191,#188192,#188193,#188194,
#188195,#188196,#188197),(#188198,#188199,#188200,#188201,#188202,#188203,
#188204,#188205,#188206),(#188207,#188208,#188209,#188210,#188211,#188212,
#188213,#188214,#188215),(#188216,#188217,#188218,#188219,#188220,#188221,
#188222,#188223,#188224),(#188225,#188226,#188227,#188228,#188229,#188230,
#188231,#188232,#188233),(#188234,#188235,#188236,#188237,#188238,#188239,
#188240,#188241,#188242),(#188243,#188244,#188245,#188246,#188247,#188248,
#188249,#188250,#188251),(#188252,#188253,#188254,#188255,#188256,#188257,
#188258,#188259,#188260),(#188261,#188262,#188263,#188264,#188265,#188266,
#188267,#188268,#188269),(#188270,#188271,#188272,#188273,#188274,#188275,
#188276,#188277,#188278),(#188279,#188280,#188281,#188282,#188283,#188284,
#188285,#188286,#188287),(#188288,#188289,#188290,#188291,#188292,#188293,
#188294,#188295,#188296),(#188297,#188298,#188299,#188300,#188301,#188302,
#188303,#188304,#188305),(#188306,#188307,#188308,#188309,#188310,#188311,
#188312,#188313,#188314),(#188315,#188316,#188317,#188318,#188319,#188320,
#188321,#188322,#188323),(#188324,#188325,#188326,#188327,#188328,#188329,
#188330,#188331,#188332),(#188333,#188334,#188335,#188336,#188337,#188338,
#188339,#188340,#188341),(#188342,#188343,#188344,#188345,#188346,#188347,
#188348,#188349,#188350),(#188351,#188352,#188353,#188354,#188355,#188356,
#188357,#188358,#188359),(#188360,#188361,#188362,#188363,#188364,#188365,
#188366,#188367,#188368),(#188369,#188370,#188371,#188372,#188373,#188374,
#188375,#188376,#188377),(#188378,#188379,#188380,#188381,#188382,#188383,
#188384,#188385,#188386),(#188387,#188388,#188389,#188390,#188391,#188392,
#188393,#188394,#188395),(#188396,#188397,#188398,#188399,#188400,#188401,
#188402,#188403,#188404),(#188405,#188406,#188407,#188408,#188409,#188410,
#188411,#188412,#188413),(#188414,#188415,#188416,#188417,#188418,#188419,
#188420,#188421,#188422),(#188423,#188424,#188425,#188426,#188427,#188428,
#188429,#188430,#188431),(#188432,#188433,#188434,#188435,#188436,#188437,
#188438,#188439,#188440),(#188441,#188442,#188443,#188444,#188445,#188446,
#188447,#188448,#188449),(#188450,#188451,#188452,#188453,#188454,#188455,
#188456,#188457,#188458),(#188459,#188460,#188461,#188462,#188463,#188464,
#188465,#188466,#188467),(#188468,#188469,#188470,#188471,#188472,#188473,
#188474,#188475,#188476),(#188477,#188478,#188479,#188480,#188481,#188482,
#188483,#188484,#188485),(#188486,#188487,#188488,#188489,#188490,#188491,
#188492,#188493,#188494),(#188495,#188496,#188497,#188498,#188499,#188500,
#188501,#188502,#188503),(#188504,#188505,#188506,#188507,#188508,#188509,
#188510,#188511,#188512),(#188513,#188514,#188515,#188516,#188517,#188518,
#188519,#188520,#188521),(#188522,#188523,#188524,#188525,#188526,#188527,
#188528,#188529,#188530),(#188531,#188532,#188533,#188534,#188535,#188536,
#188537,#188538,#188539),(#188540,#188541,#188542,#188543,#188544,#188545,
#188546,#188547,#188548),(#188549,#188550,#188551,#188552,#188553,#188554,
#188555,#188556,#188557),(#188558,#188559,#188560,#188561,#188562,#188563,
#188564,#188565,#188566),(#188567,#188568,#188569,#188570,#188571,#188572,
#188573,#188574,#188575),(#188576,#188577,#188578,#188579,#188580,#188581,
#188582,#188583,#188584),(#188585,#188586,#188587,#188588,#188589,#188590,
#188591,#188592,#188593),(#188594,#188595,#188596,#188597,#188598,#188599,
#188600,#188601,#188602),(#188603,#188604,#188605,#188606,#188607,#188608,
#188609,#188610,#188611),(#188612,#188613,#188614,#188615,#188616,#188617,
#188618,#188619,#188620),(#188621,#188622,#188623,#188624,#188625,#188626,
#188627,#188628,#188629),(#188630,#188631,#188632,#188633,#188634,#188635,
#188636,#188637,#188638),(#188639,#188640,#188641,#188642,#188643,#188644,
#188645,#188646,#188647),(#188648,#188649,#188650,#188651,#188652,#188653,
#188654,#188655,#188656),(#188657,#188658,#188659,#188660,#188661,#188662,
#188663,#188664,#188665),(#188666,#188667,#188668,#188669,#188670,#188671,
#188672,#188673,#188674),(#188675,#188676,#188677,#188678,#188679,#188680,
#188681,#188682,#188683),(#188684,#188685,#188686,#188687,#188688,#188689,
#188690,#188691,#188692),(#188693,#188694,#188695,#188696,#188697,#188698,
#188699,#188700,#188701),(#188702,#188703,#188704,#188705,#188706,#188707,
#188708,#188709,#188710),(#188711,#188712,#188713,#188714,#188715,#188716,
#188717,#188718,#188719),(#188720,#188721,#188722,#188723,#188724,#188725,
#188726,#188727,#188728),(#188729,#188730,#188731,#188732,#188733,#188734,
#188735,#188736,#188737),(#188738,#188739,#188740,#188741,#188742,#188743,
#188744,#188745,#188746),(#188747,#188748,#188749,#188750,#188751,#188752,
#188753,#188754,#188755),(#188756,#188757,#188758,#188759,#188760,#188761,
#188762,#188763,#188764),(#188765,#188766,#188767,#188768,#188769,#188770,
#188771,#188772,#188773),(#188774,#188775,#188776,#188777,#188778,#188779,
#188780,#188781,#188782),(#188783,#188784,#188785,#188786,#188787,#188788,
#188789,#188790,#188791),(#188792,#188793,#188794,#188795,#188796,#188797,
#188798,#188799,#188800),(#188801,#188802,#188803,#188804,#188805,#188806,
#188807,#188808,#188809),(#188810,#188811,#188812,#188813,#188814,#188815,
#188816,#188817,#188818),(#188819,#188820,#188821,#188822,#188823,#188824,
#188825,#188826,#188827),(#188828,#188829,#188830,#188831,#188832,#188833,
#188834,#188835,#188836),(#188837,#188838,#188839,#188840,#188841,#188842,
#188843,#188844,#188845),(#188846,#188847,#188848,#188849,#188850,#188851,
#188852,#188853,#188854),(#188855,#188856,#188857,#188858,#188859,#188860,
#188861,#188862,#188863),(#188864,#188865,#188866,#188867,#188868,#188869,
#188870,#188871,#188872),(#188873,#188874,#188875,#188876,#188877,#188878,
#188879,#188880,#188881),(#188882,#188883,#188884,#188885,#188886,#188887,
#188888,#188889,#188890),(#188891,#188892,#188893,#188894,#188895,#188896,
#188897,#188898,#188899),(#188900,#188901,#188902,#188903,#188904,#188905,
#188906,#188907,#188908),(#188909,#188910,#188911,#188912,#188913,#188914,
#188915,#188916,#188917),(#188918,#188919,#188920,#188921,#188922,#188923,
#188924,#188925,#188926),(#188927,#188928,#188929,#188930,#188931,#188932,
#188933,#188934,#188935),(#188936,#188937,#188938,#188939,#188940,#188941,
#188942,#188943,#188944),(#188945,#188946,#188947,#188948,#188949,#188950,
#188951,#188952,#188953),(#188954,#188955,#188956,#188957,#188958,#188959,
#188960,#188961,#188962),(#188963,#188964,#188965,#188966,#188967,#188968,
#188969,#188970,#188971),(#188972,#188973,#188974,#188975,#188976,#188977,
#188978,#188979,#188980),(#188981,#188982,#188983,#188984,#188985,#188986,
#188987,#188988,#188989),(#188990,#188991,#188992,#188993,#188994,#188995,
#188996,#188997,#188998),(#188999,#189000,#189001,#189002,#189003,#189004,
#189005,#189006,#189007),(#189008,#189009,#189010,#189011,#189012,#189013,
#189014,#189015,#189016),(#189017,#189018,#189019,#189020,#189021,#189022,
#189023,#189024,#189025),(#189026,#189027,#189028,#189029,#189030,#189031,
#189032,#189033,#189034),(#189035,#189036,#189037,#189038,#189039,#189040,
#189041,#189042,#189043),(#189044,#189045,#189046,#189047,#189048,#189049,
#189050,#189051,#189052),(#189053,#189054,#189055,#189056,#189057,#189058,
#189059,#189060,#189061),(#189062,#189063,#189064,#189065,#189066,#189067,
#189068,#189069,#189070),(#189071,#189072,#189073,#189074,#189075,#189076,
#189077,#189078,#189079),(#189080,#189081,#189082,#189083,#189084,#189085,
#189086,#189087,#189088),(#189089,#189090,#189091,#189092,#189093,#189094,
#189095,#189096,#189097),(#189098,#189099,#189100,#189101,#189102,#189103,
#189104,#189105,#189106),(#189107,#189108,#189109,#189110,#189111,#189112,
#189113,#189114,#189115),(#189116,#189117,#189118,#189119,#189120,#189121,
#189122,#189123,#189124),(#189125,#189126,#189127,#189128,#189129,#189130,
#189131,#189132,#189133),(#189134,#189135,#189136,#189137,#189138,#189139,
#189140,#189141,#189142),(#189143,#189144,#189145,#189146,#189147,#189148,
#189149,#189150,#189151),(#189152,#189153,#189154,#189155,#189156,#189157,
#189158,#189159,#189160),(#189161,#189162,#189163,#189164,#189165,#189166,
#189167,#189168,#189169),(#189170,#189171,#189172,#189173,#189174,#189175,
#189176,#189177,#189178),(#189179,#189180,#189181,#189182,#189183,#189184,
#189185,#189186,#189187),(#189188,#189189,#189190,#189191,#189192,#189193,
#189194,#189195,#189196),(#189197,#189198,#189199,#189200,#189201,#189202,
#189203,#189204,#189205),(#189206,#189207,#189208,#189209,#189210,#189211,
#189212,#189213,#189214),(#189215,#189216,#189217,#189218,#189219,#189220,
#189221,#189222,#189223),(#189224,#189225,#189226,#189227,#189228,#189229,
#189230,#189231,#189232),(#189233,#189234,#189235,#189236,#189237,#189238,
#189239,#189240,#189241),(#189242,#189243,#189244,#189245,#189246,#189247,
#189248,#189249,#189250),(#189251,#189252,#189253,#189254,#189255,#189256,
#189257,#189258,#189259),(#189260,#189261,#189262,#189263,#189264,#189265,
#189266,#189267,#189268),(#189269,#189270,#189271,#189272,#189273,#189274,
#189275,#189276,#189277),(#189278,#189279,#189280,#189281,#189282,#189283,
#189284,#189285,#189286),(#189287,#189288,#189289,#189290,#189291,#189292,
#189293,#189294,#189295),(#189296,#189297,#189298,#189299,#189300,#189301,
#189302,#189303,#189304),(#189305,#189306,#189307,#189308,#189309,#189310,
#189311,#189312,#189313),(#189314,#189315,#189316,#189317,#189318,#189319,
#189320,#189321,#189322),(#189323,#189324,#189325,#189326,#189327,#189328,
#189329,#189330,#189331),(#189332,#189333,#189334,#189335,#189336,#189337,
#189338,#189339,#189340),(#189341,#189342,#189343,#189344,#189345,#189346,
#189347,#189348,#189349),(#189350,#189351,#189352,#189353,#189354,#189355,
#189356,#189357,#189358),(#189359,#189360,#189361,#189362,#189363,#189364,
#189365,#189366,#189367),(#189368,#189369,#189370,#189371,#189372,#189373,
#189374,#189375,#189376),(#189377,#189378,#189379,#189380,#189381,#189382,
#189383,#189384,#189385),(#189386,#189387,#189388,#189389,#189390,#189391,
#189392,#189393,#189394),(#189395,#189396,#189397,#189398,#189399,#189400,
#189401,#189402,#189403),(#189404,#189405,#189406,#189407,#189408,#189409,
#189410,#189411,#189412),(#189413,#189414,#189415,#189416,#189417,#189418,
#189419,#189420,#189421),(#189422,#189423,#189424,#189425,#189426,#189427,
#189428,#189429,#189430),(#189431,#189432,#189433,#189434,#189435,#189436,
#189437,#189438,#189439),(#189440,#189441,#189442,#189443,#189444,#189445,
#189446,#189447,#189448),(#189449,#189450,#189451,#189452,#189453,#189454,
#189455,#189456,#189457),(#189458,#189459,#189460,#189461,#189462,#189463,
#189464,#189465,#189466),(#189467,#189468,#189469,#189470,#189471,#189472,
#189473,#189474,#189475),(#189476,#189477,#189478,#189479,#189480,#189481,
#189482,#189483,#189484),(#189485,#189486,#189487,#189488,#189489,#189490,
#189491,#189492,#189493),(#189494,#189495,#189496,#189497,#189498,#189499,
#189500,#189501,#189502),(#189503,#189504,#189505,#189506,#189507,#189508,
#189509,#189510,#189511),(#189512,#189513,#189514,#189515,#189516,#189517,
#189518,#189519,#189520),(#189521,#189522,#189523,#189524,#189525,#189526,
#189527,#189528,#189529),(#189530,#189531,#189532,#189533,#189534,#189535,
#189536,#189537,#189538),(#189539,#189540,#189541,#189542,#189543,#189544,
#189545,#189546,#189547),(#189548,#189549,#189550,#189551,#189552,#189553,
#189554,#189555,#189556),(#189557,#189558,#189559,#189560,#189561,#189562,
#189563,#189564,#189565),(#189566,#189567,#189568,#189569,#189570,#189571,
#189572,#189573,#189574),(#189575,#189576,#189577,#189578,#189579,#189580,
#189581,#189582,#189583),(#189584,#189585,#189586,#189587,#189588,#189589,
#189590,#189591,#189592),(#189593,#189594,#189595,#189596,#189597,#189598,
#189599,#189600,#189601),(#189602,#189603,#189604,#189605,#189606,#189607,
#189608,#189609,#189610),(#189611,#189612,#189613,#189614,#189615,#189616,
#189617,#189618,#189619),(#189620,#189621,#189622,#189623,#189624,#189625,
#189626,#189627,#189628),(#189629,#189630,#189631,#189632,#189633,#189634,
#189635,#189636,#189637),(#189638,#189639,#189640,#189641,#189642,#189643,
#189644,#189645,#189646),(#189647,#189648,#189649,#189650,#189651,#189652,
#189653,#189654,#189655),(#189656,#189657,#189658,#189659,#189660,#189661,
#189662,#189663,#189664),(#189665,#189666,#189667,#189668,#189669,#189670,
#189671,#189672,#189673),(#189674,#189675,#189676,#189677,#189678,#189679,
#189680,#189681,#189682),(#189683,#189684,#189685,#189686,#189687,#189688,
#189689,#189690,#189691),(#189692,#189693,#189694,#189695,#189696,#189697,
#189698,#189699,#189700),(#189701,#189702,#189703,#189704,#189705,#189706,
#189707,#189708,#189709),(#189710,#189711,#189712,#189713,#189714,#189715,
#189716,#189717,#189718),(#189719,#189720,#189721,#189722,#189723,#189724,
#189725,#189726,#189727),(#189728,#189729,#189730,#189731,#189732,#189733,
#189734,#189735,#189736),(#189737,#189738,#189739,#189740,#189741,#189742,
#189743,#189744,#189745),(#189746,#189747,#189748,#189749,#189750,#189751,
#189752,#189753,#189754),(#189755,#189756,#189757,#189758,#189759,#189760,
#189761,#189762,#189763),(#189764,#189765,#189766,#189767,#189768,#189769,
#189770,#189771,#189772),(#189773,#189774,#189775,#189776,#189777,#189778,
#189779,#189780,#189781),(#189782,#189783,#189784,#189785,#189786,#189787,
#189788,#189789,#189790),(#189791,#189792,#189793,#189794,#189795,#189796,
#189797,#189798,#189799),(#189800,#189801,#189802,#189803,#189804,#189805,
#189806,#189807,#189808),(#189809,#189810,#189811,#189812,#189813,#189814,
#189815,#189816,#189817),(#189818,#189819,#189820,#189821,#189822,#189823,
#189824,#189825,#189826),(#189827,#189828,#189829,#189830,#189831,#189832,
#189833,#189834,#189835),(#189836,#189837,#189838,#189839,#189840,#189841,
#189842,#189843,#189844),(#189845,#189846,#189847,#189848,#189849,#189850,
#189851,#189852,#189853),(#189854,#189855,#189856,#189857,#189858,#189859,
#189860,#189861,#189862),(#189863,#189864,#189865,#189866,#189867,#189868,
#189869,#189870,#189871),(#189872,#189873,#189874,#189875,#189876,#189877,
#189878,#189879,#189880),(#189881,#189882,#189883,#189884,#189885,#189886,
#189887,#189888,#189889),(#189890,#189891,#189892,#189893,#189894,#189895,
#189896,#189897,#189898),(#189899,#189900,#189901,#189902,#189903,#189904,
#189905,#189906,#189907),(#189908,#189909,#189910,#189911,#189912,#189913,
#189914,#189915,#189916),(#189917,#189918,#189919,#189920,#189921,#189922,
#189923,#189924,#189925),(#189926,#189927,#189928,#189929,#189930,#189931,
#189932,#189933,#189934),(#189935,#189936,#189937,#189938,#189939,#189940,
#189941,#189942,#189943),(#189944,#189945,#189946,#189947,#189948,#189949,
#189950,#189951,#189952),(#189953,#189954,#189955,#189956,#189957,#189958,
#189959,#189960,#189961),(#189962,#189963,#189964,#189965,#189966,#189967,
#189968,#189969,#189970),(#189971,#189972,#189973,#189974,#189975,#189976,
#189977,#189978,#189979),(#189980,#189981,#189982,#189983,#189984,#189985,
#189986,#189987,#189988),(#189989,#189990,#189991,#189992,#189993,#189994,
#189995,#189996,#189997),(#189998,#189999,#190000,#190001,#190002,#190003,
#190004,#190005,#190006),(#190007,#190008,#190009,#190010,#190011,#190012,
#190013,#190014,#190015),(#190016,#190017,#190018,#190019,#190020,#190021,
#190022,#190023,#190024),(#190025,#190026,#190027,#190028,#190029,#190030,
#190031,#190032,#190033),(#190034,#190035,#190036,#190037,#190038,#190039,
#190040,#190041,#190042),(#190043,#190044,#190045,#190046,#190047,#190048,
#190049,#190050,#190051),(#190052,#190053,#190054,#190055,#190056,#190057,
#190058,#190059,#190060),(#190061,#190062,#190063,#190064,#190065,#190066,
#190067,#190068,#190069),(#190070,#190071,#190072,#190073,#190074,#190075,
#190076,#190077,#190078),(#190079,#190080,#190081,#190082,#190083,#190084,
#190085,#190086,#190087),(#190088,#190089,#190090,#190091,#190092,#190093,
#190094,#190095,#190096),(#190097,#190098,#190099,#190100,#190101,#190102,
#190103,#190104,#190105),(#190106,#190107,#190108,#190109,#190110,#190111,
#190112,#190113,#190114),(#190115,#190116,#190117,#190118,#190119,#190120,
#190121,#190122,#190123),(#190124,#190125,#190126,#190127,#190128,#190129,
#190130,#190131,#190132),(#190133,#190134,#190135,#190136,#190137,#190138,
#190139,#190140,#190141),(#190142,#190143,#190144,#190145,#190146,#190147,
#190148,#190149,#190150),(#190151,#190152,#190153,#190154,#190155,#190156,
#190157,#190158,#190159),(#190160,#190161,#190162,#190163,#190164,#190165,
#190166,#190167,#190168),(#190169,#190170,#190171,#190172,#190173,#190174,
#190175,#190176,#190177),(#190178,#190179,#190180,#190181,#190182,#190183,
#190184,#190185,#190186),(#190187,#190188,#190189,#190190,#190191,#190192,
#190193,#190194,#190195),(#190196,#190197,#190198,#190199,#190200,#190201,
#190202,#190203,#190204),(#190205,#190206,#190207,#190208,#190209,#190210,
#190211,#190212,#190213),(#190214,#190215,#190216,#190217,#190218,#190219,
#190220,#190221,#190222),(#190223,#190224,#190225,#190226,#190227,#190228,
#190229,#190230,#190231),(#190232,#190233,#190234,#190235,#190236,#190237,
#190238,#190239,#190240),(#190241,#190242,#190243,#190244,#190245,#190246,
#190247,#190248,#190249),(#190250,#190251,#190252,#190253,#190254,#190255,
#190256,#190257,#190258),(#190259,#190260,#190261,#190262,#190263,#190264,
#190265,#190266,#190267),(#190268,#190269,#190270,#190271,#190272,#190273,
#190274,#190275,#190276),(#190277,#190278,#190279,#190280,#190281,#190282,
#190283,#190284,#190285),(#190286,#190287,#190288,#190289,#190290,#190291,
#190292,#190293,#190294),(#190295,#190296,#190297,#190298,#190299,#190300,
#190301,#190302,#190303),(#190304,#190305,#190306,#190307,#190308,#190309,
#190310,#190311,#190312),(#190313,#190314,#190315,#190316,#190317,#190318,
#190319,#190320,#190321),(#190322,#190323,#190324,#190325,#190326,#190327,
#190328,#190329,#190330),(#190331,#190332,#190333,#190334,#190335,#190336,
#190337,#190338,#190339),(#190340,#190341,#190342,#190343,#190344,#190345,
#190346,#190347,#190348),(#190349,#190350,#190351,#190352,#190353,#190354,
#190355,#190356,#190357),(#190358,#190359,#190360,#190361,#190362,#190363,
#190364,#190365,#190366),(#190367,#190368,#190369,#190370,#190371,#190372,
#190373,#190374,#190375),(#190376,#190377,#190378,#190379,#190380,#190381,
#190382,#190383,#190384),(#190385,#190386,#190387,#190388,#190389,#190390,
#190391,#190392,#190393),(#190394,#190395,#190396,#190397,#190398,#190399,
#190400,#190401,#190402),(#190403,#190404,#190405,#190406,#190407,#190408,
#190409,#190410,#190411),(#190412,#190413,#190414,#190415,#190416,#190417,
#190418,#190419,#190420),(#190421,#190422,#190423,#190424,#190425,#190426,
#190427,#190428,#190429),(#190430,#190431,#190432,#190433,#190434,#190435,
#190436,#190437,#190438),(#190439,#190440,#190441,#190442,#190443,#190444,
#190445,#190446,#190447),(#190448,#190449,#190450,#190451,#190452,#190453,
#190454,#190455,#190456),(#190457,#190458,#190459,#190460,#190461,#190462,
#190463,#190464,#190465),(#190466,#190467,#190468,#190469,#190470,#190471,
#190472,#190473,#190474),(#190475,#190476,#190477,#190478,#190479,#190480,
#190481,#190482,#190483),(#190484,#190485,#190486,#190487,#190488,#190489,
#190490,#190491,#190492),(#190493,#190494,#190495,#190496,#190497,#190498,
#190499,#190500,#190501),(#190502,#190503,#190504,#190505,#190506,#190507,
#190508,#190509,#190510),(#190511,#190512,#190513,#190514,#190515,#190516,
#190517,#190518,#190519),(#190520,#190521,#190522,#190523,#190524,#190525,
#190526,#190527,#190528),(#190529,#190530,#190531,#190532,#190533,#190534,
#190535,#190536,#190537),(#190538,#190539,#190540,#190541,#190542,#190543,
#190544,#190545,#190546),(#190547,#190548,#190549,#190550,#190551,#190552,
#190553,#190554,#190555),(#190556,#190557,#190558,#190559,#190560,#190561,
#190562,#190563,#190564),(#190565,#190566,#190567,#190568,#190569,#190570,
#190571,#190572,#190573),(#190574,#190575,#190576,#190577,#190578,#190579,
#190580,#190581,#190582),(#190583,#190584,#190585,#190586,#190587,#190588,
#190589,#190590,#190591),(#190592,#190593,#190594,#190595,#190596,#190597,
#190598,#190599,#190600),(#190601,#190602,#190603,#190604,#190605,#190606,
#190607,#190608,#190609),(#190610,#190611,#190612,#190613,#190614,#190615,
#190616,#190617,#190618),(#190619,#190620,#190621,#190622,#190623,#190624,
#190625,#190626,#190627),(#190628,#190629,#190630,#190631,#190632,#190633,
#190634,#190635,#190636),(#190637,#190638,#190639,#190640,#190641,#190642,
#190643,#190644,#190645),(#190646,#190647,#190648,#190649,#190650,#190651,
#190652,#190653,#190654),(#190655,#190656,#190657,#190658,#190659,#190660,
#190661,#190662,#190663),(#190664,#190665,#190666,#190667,#190668,#190669,
#190670,#190671,#190672),(#190673,#190674,#190675,#190676,#190677,#190678,
#190679,#190680,#190681),(#190682,#190683,#190684,#190685,#190686,#190687,
#190688,#190689,#190690),(#190691,#190692,#190693,#190694,#190695,#190696,
#190697,#190698,#190699),(#190700,#190701,#190702,#190703,#190704,#190705,
#190706,#190707,#190708),(#190709,#190710,#190711,#190712,#190713,#190714,
#190715,#190716,#190717),(#190718,#190719,#190720,#190721,#190722,#190723,
#190724,#190725,#190726),(#190727,#190728,#190729,#190730,#190731,#190732,
#190733,#190734,#190735),(#190736,#190737,#190738,#190739,#190740,#190741,
#190742,#190743,#190744),(#190745,#190746,#190747,#190748,#190749,#190750,
#190751,#190752,#190753),(#190754,#190755,#190756,#190757,#190758,#190759,
#190760,#190761,#190762),(#190763,#190764,#190765,#190766,#190767,#190768,
#190769,#190770,#190771),(#190772,#190773,#190774,#190775,#190776,#190777,
#190778,#190779,#190780),(#190781,#190782,#190783,#190784,#190785,#190786,
#190787,#190788,#190789),(#190790,#190791,#190792,#190793,#190794,#190795,
#190796,#190797,#190798),(#190799,#190800,#190801,#190802,#190803,#190804,
#190805,#190806,#190807),(#190808,#190809,#190810,#190811,#190812,#190813,
#190814,#190815,#190816),(#190817,#190818,#190819,#190820,#190821,#190822,
#190823,#190824,#190825),(#190826,#190827,#190828,#190829,#190830,#190831,
#190832,#190833,#190834),(#190835,#190836,#190837,#190838,#190839,#190840,
#190841,#190842,#190843),(#190844,#190845,#190846,#190847,#190848,#190849,
#190850,#190851,#190852),(#190853,#190854,#190855,#190856,#190857,#190858,
#190859,#190860,#190861),(#190862,#190863,#190864,#190865,#190866,#190867,
#190868,#190869,#190870),(#190871,#190872,#190873,#190874,#190875,#190876,
#190877,#190878,#190879),(#190880,#190881,#190882,#190883,#190884,#190885,
#190886,#190887,#190888),(#190889,#190890,#190891,#190892,#190893,#190894,
#190895,#190896,#190897),(#190898,#190899,#190900,#190901,#190902,#190903,
#190904,#190905,#190906),(#190907,#190908,#190909,#190910,#190911,#190912,
#190913,#190914,#190915),(#190916,#190917,#190918,#190919,#190920,#190921,
#190922,#190923,#190924),(#190925,#190926,#190927,#190928,#190929,#190930,
#190931,#190932,#190933),(#190934,#190935,#190936,#190937,#190938,#190939,
#190940,#190941,#190942),(#190943,#190944,#190945,#190946,#190947,#190948,
#190949,#190950,#190951),(#190952,#190953,#190954,#190955,#190956,#190957,
#190958,#190959,#190960),(#190961,#190962,#190963,#190964,#190965,#190966,
#190967,#190968,#190969),(#190970,#190971,#190972,#190973,#190974,#190975,
#190976,#190977,#190978),(#190979,#190980,#190981,#190982,#190983,#190984,
#190985,#190986,#190987),(#190988,#190989,#190990,#190991,#190992,#190993,
#190994,#190995,#190996),(#190997,#190998,#190999,#191000,#191001,#191002,
#191003,#191004,#191005),(#191006,#191007,#191008,#191009,#191010,#191011,
#191012,#191013,#191014),(#191015,#191016,#191017,#191018,#191019,#191020,
#191021,#191022,#191023),(#191024,#191025,#191026,#191027,#191028,#191029,
#191030,#191031,#191032),(#191033,#191034,#191035,#191036,#191037,#191038,
#191039,#191040,#191041),(#191042,#191043,#191044,#191045,#191046,#191047,
#191048,#191049,#191050),(#191051,#191052,#191053,#191054,#191055,#191056,
#191057,#191058,#191059),(#191060,#191061,#191062,#191063,#191064,#191065,
#191066,#191067,#191068),(#191069,#191070,#191071,#191072,#191073,#191074,
#191075,#191076,#191077),(#191078,#191079,#191080,#191081,#191082,#191083,
#191084,#191085,#191086),(#191087,#191088,#191089,#191090,#191091,#191092,
#191093,#191094,#191095),(#191096,#191097,#191098,#191099,#191100,#191101,
#191102,#191103,#191104),(#191105,#191106,#191107,#191108,#191109,#191110,
#191111,#191112,#191113),(#191114,#191115,#191116,#191117,#191118,#191119,
#191120,#191121,#191122),(#191123,#191124,#191125,#191126,#191127,#191128,
#191129,#191130,#191131),(#191132,#191133,#191134,#191135,#191136,#191137,
#191138,#191139,#191140),(#191141,#191142,#191143,#191144,#191145,#191146,
#191147,#191148,#191149),(#191150,#191151,#191152,#191153,#191154,#191155,
#191156,#191157,#191158),(#191159,#191160,#191161,#191162,#191163,#191164,
#191165,#191166,#191167),(#191168,#191169,#191170,#191171,#191172,#191173,
#191174,#191175,#191176),(#191177,#191178,#191179,#191180,#191181,#191182,
#191183,#191184,#191185),(#191186,#191187,#191188,#191189,#191190,#191191,
#191192,#191193,#191194),(#191195,#191196,#191197,#191198,#191199,#191200,
#191201,#191202,#191203),(#191204,#191205,#191206,#191207,#191208,#191209,
#191210,#191211,#191212),(#191213,#191214,#191215,#191216,#191217,#191218,
#191219,#191220,#191221),(#191222,#191223,#191224,#191225,#191226,#191227,
#191228,#191229,#191230),(#191231,#191232,#191233,#191234,#191235,#191236,
#191237,#191238,#191239),(#191240,#191241,#191242,#191243,#191244,#191245,
#191246,#191247,#191248),(#191249,#191250,#191251,#191252,#191253,#191254,
#191255,#191256,#191257),(#191258,#191259,#191260,#191261,#191262,#191263,
#191264,#191265,#191266),(#191267,#191268,#191269,#191270,#191271,#191272,
#191273,#191274,#191275),(#191276,#191277,#191278,#191279,#191280,#191281,
#191282,#191283,#191284),(#191285,#191286,#191287,#191288,#191289,#191290,
#191291,#191292,#191293),(#191294,#191295,#191296,#191297,#191298,#191299,
#191300,#191301,#191302),(#191303,#191304,#191305,#191306,#191307,#191308,
#191309,#191310,#191311),(#191312,#191313,#191314,#191315,#191316,#191317,
#191318,#191319,#191320),(#191321,#191322,#191323,#191324,#191325,#191326,
#191327,#191328,#191329),(#191330,#191331,#191332,#191333,#191334,#191335,
#191336,#191337,#191338),(#191339,#191340,#191341,#191342,#191343,#191344,
#191345,#191346,#191347),(#191348,#191349,#191350,#191351,#191352,#191353,
#191354,#191355,#191356),(#191357,#191358,#191359,#191360,#191361,#191362,
#191363,#191364,#191365),(#191366,#191367,#191368,#191369,#191370,#191371,
#191372,#191373,#191374),(#191375,#191376,#191377,#191378,#191379,#191380,
#191381,#191382,#191383),(#191384,#191385,#191386,#191387,#191388,#191389,
#191390,#191391,#191392),(#191393,#191394,#191395,#191396,#191397,#191398,
#191399,#191400,#191401),(#191402,#191403,#191404,#191405,#191406,#191407,
#191408,#191409,#191410),(#191411,#191412,#191413,#191414,#191415,#191416,
#191417,#191418,#191419),(#191420,#191421,#191422,#191423,#191424,#191425,
#191426,#191427,#191428),(#191429,#191430,#191431,#191432,#191433,#191434,
#191435,#191436,#191437),(#191438,#191439,#191440,#191441,#191442,#191443,
#191444,#191445,#191446),(#191447,#191448,#191449,#191450,#191451,#191452,
#191453,#191454,#191455),(#191456,#191457,#191458,#191459,#191460,#191461,
#191462,#191463,#191464),(#191465,#191466,#191467,#191468,#191469,#191470,
#191471,#191472,#191473),(#191474,#191475,#191476,#191477,#191478,#191479,
#191480,#191481,#191482),(#191483,#191484,#191485,#191486,#191487,#191488,
#191489,#191490,#191491),(#191492,#191493,#191494,#191495,#191496,#191497,
#191498,#191499,#191500),(#191501,#191502,#191503,#191504,#191505,#191506,
#191507,#191508,#191509),(#191510,#191511,#191512,#191513,#191514,#191515,
#191516,#191517,#191518),(#191519,#191520,#191521,#191522,#191523,#191524,
#191525,#191526,#191527),(#191528,#191529,#191530,#191531,#191532,#191533,
#191534,#191535,#191536),(#191537,#191538,#191539,#191540,#191541,#191542,
#191543,#191544,#191545),(#191546,#191547,#191548,#191549,#191550,#191551,
#191552,#191553,#191554),(#191555,#191556,#191557,#191558,#191559,#191560,
#191561,#191562,#191563),(#191564,#191565,#191566,#191567,#191568,#191569,
#191570,#191571,#191572),(#191573,#191574,#191575,#191576,#191577,#191578,
#191579,#191580,#191581),(#191582,#191583,#191584,#191585,#191586,#191587,
#191588,#191589,#191590),(#191591,#191592,#191593,#191594,#191595,#191596,
#191597,#191598,#191599),(#191600,#191601,#191602,#191603,#191604,#191605,
#191606,#191607,#191608),(#191609,#191610,#191611,#191612,#191613,#191614,
#191615,#191616,#191617),(#191618,#191619,#191620,#191621,#191622,#191623,
#191624,#191625,#191626),(#191627,#191628,#191629,#191630,#191631,#191632,
#191633,#191634,#191635),(#191636,#191637,#191638,#191639,#191640,#191641,
#191642,#191643,#191644),(#191645,#191646,#191647,#191648,#191649,#191650,
#191651,#191652,#191653),(#191654,#191655,#191656,#191657,#191658,#191659,
#191660,#191661,#191662),(#191663,#191664,#191665,#191666,#191667,#191668,
#191669,#191670,#191671),(#191672,#191673,#191674,#191675,#191676,#191677,
#191678,#191679,#191680),(#191681,#191682,#191683,#191684,#191685,#191686,
#191687,#191688,#191689),(#191690,#191691,#191692,#191693,#191694,#191695,
#191696,#191697,#191698),(#191699,#191700,#191701,#191702,#191703,#191704,
#191705,#191706,#191707),(#191708,#191709,#191710,#191711,#191712,#191713,
#191714,#191715,#191716),(#191717,#191718,#191719,#191720,#191721,#191722,
#191723,#191724,#191725),(#191726,#191727,#191728,#191729,#191730,#191731,
#191732,#191733,#191734),(#191735,#191736,#191737,#191738,#191739,#191740,
#191741,#191742,#191743),(#191744,#191745,#191746,#191747,#191748,#191749,
#191750,#191751,#191752),(#191753,#191754,#191755,#191756,#191757,#191758,
#191759,#191760,#191761),(#191762,#191763,#191764,#191765,#191766,#191767,
#191768,#191769,#191770),(#191771,#191772,#191773,#191774,#191775,#191776,
#191777,#191778,#191779),(#191780,#191781,#191782,#191783,#191784,#191785,
#191786,#191787,#191788),(#191789,#191790,#191791,#191792,#191793,#191794,
#191795,#191796,#191797),(#191798,#191799,#191800,#191801,#191802,#191803,
#191804,#191805,#191806),(#191807,#191808,#191809,#191810,#191811,#191812,
#191813,#191814,#191815),(#191816,#191817,#191818,#191819,#191820,#191821,
#191822,#191823,#191824),(#191825,#191826,#191827,#191828,#191829,#191830,
#191831,#191832,#191833),(#191834,#191835,#191836,#191837,#191838,#191839,
#191840,#191841,#191842),(#191843,#191844,#191845,#191846,#191847,#191848,
#191849,#191850,#191851),(#191852,#191853,#191854,#191855,#191856,#191857,
#191858,#191859,#191860),(#191861,#191862,#191863,#191864,#191865,#191866,
#191867,#191868,#191869),(#191870,#191871,#191872,#191873,#191874,#191875,
#191876,#191877,#191878),(#191879,#191880,#191881,#191882,#191883,#191884,
#191885,#191886,#191887),(#191888,#191889,#191890,#191891,#191892,#191893,
#191894,#191895,#191896),(#191897,#191898,#191899,#191900,#191901,#191902,
#191903,#191904,#191905),(#191906,#191907,#191908,#191909,#191910,#191911,
#191912,#191913,#191914),(#191915,#191916,#191917,#191918,#191919,#191920,
#191921,#191922,#191923),(#191924,#191925,#191926,#191927,#191928,#191929,
#191930,#191931,#191932),(#191933,#191934,#191935,#191936,#191937,#191938,
#191939,#191940,#191941),(#191942,#191943,#191944,#191945,#191946,#191947,
#191948,#191949,#191950),(#191951,#191952,#191953,#191954,#191955,#191956,
#191957,#191958,#191959),(#191960,#191961,#191962,#191963,#191964,#191965,
#191966,#191967,#191968),(#191969,#191970,#191971,#191972,#191973,#191974,
#191975,#191976,#191977),(#191978,#191979,#191980,#191981,#191982,#191983,
#191984,#191985,#191986),(#191987,#191988,#191989,#191990,#191991,#191992,
#191993,#191994,#191995),(#191996,#191997,#191998,#191999,#192000,#192001,
#192002,#192003,#192004),(#192005,#192006,#192007,#192008,#192009,#192010,
#192011,#192012,#192013),(#192014,#192015,#192016,#192017,#192018,#192019,
#192020,#192021,#192022),(#192023,#192024,#192025,#192026,#192027,#192028,
#192029,#192030,#192031),(#192032,#192033,#192034,#192035,#192036,#192037,
#192038,#192039,#192040),(#192041,#192042,#192043,#192044,#192045,#192046,
#192047,#192048,#192049),(#192050,#192051,#192052,#192053,#192054,#192055,
#192056,#192057,#192058),(#192059,#192060,#192061,#192062,#192063,#192064,
#192065,#192066,#192067),(#192068,#192069,#192070,#192071,#192072,#192073,
#192074,#192075,#192076),(#192077,#192078,#192079,#192080,#192081,#192082,
#192083,#192084,#192085),(#192086,#192087,#192088,#192089,#192090,#192091,
#192092,#192093,#192094),(#192095,#192096,#192097,#192098,#192099,#192100,
#192101,#192102,#192103),(#192104,#192105,#192106,#192107,#192108,#192109,
#192110,#192111,#192112),(#192113,#192114,#192115,#192116,#192117,#192118,
#192119,#192120,#192121),(#192122,#192123,#192124,#192125,#192126,#192127,
#192128,#192129,#192130),(#192131,#192132,#192133,#192134,#192135,#192136,
#192137,#192138,#192139),(#192140,#192141,#192142,#192143,#192144,#192145,
#192146,#192147,#192148),(#192149,#192150,#192151,#192152,#192153,#192154,
#192155,#192156,#192157),(#192158,#192159,#192160,#192161,#192162,#192163,
#192164,#192165,#192166),(#192167,#192168,#192169,#192170,#192171,#192172,
#192173,#192174,#192175),(#192176,#192177,#192178,#192179,#192180,#192181,
#192182,#192183,#192184),(#192185,#192186,#192187,#192188,#192189,#192190,
#192191,#192192,#192193),(#192194,#192195,#192196,#192197,#192198,#192199,
#192200,#192201,#192202),(#192203,#192204,#192205,#192206,#192207,#192208,
#192209,#192210,#192211),(#192212,#192213,#192214,#192215,#192216,#192217,
#192218,#192219,#192220),(#192221,#192222,#192223,#192224,#192225,#192226,
#192227,#192228,#192229),(#192230,#192231,#192232,#192233,#192234,#192235,
#192236,#192237,#192238),(#192239,#192240,#192241,#192242,#192243,#192244,
#192245,#192246,#192247),(#192248,#192249,#192250,#192251,#192252,#192253,
#192254,#192255,#192256),(#192257,#192258,#192259,#192260,#192261,#192262,
#192263,#192264,#192265),(#192266,#192267,#192268,#192269,#192270,#192271,
#192272,#192273,#192274),(#192275,#192276,#192277,#192278,#192279,#192280,
#192281,#192282,#192283),(#192284,#192285,#192286,#192287,#192288,#192289,
#192290,#192291,#192292),(#192293,#192294,#192295,#192296,#192297,#192298,
#192299,#192300,#192301),(#192302,#192303,#192304,#192305,#192306,#192307,
#192308,#192309,#192310),(#192311,#192312,#192313,#192314,#192315,#192316,
#192317,#192318,#192319),(#192320,#192321,#192322,#192323,#192324,#192325,
#192326,#192327,#192328),(#192329,#192330,#192331,#192332,#192333,#192334,
#192335,#192336,#192337),(#192338,#192339,#192340,#192341,#192342,#192343,
#192344,#192345,#192346),(#192347,#192348,#192349,#192350,#192351,#192352,
#192353,#192354,#192355),(#192356,#192357,#192358,#192359,#192360,#192361,
#192362,#192363,#192364),(#192365,#192366,#192367,#192368,#192369,#192370,
#192371,#192372,#192373),(#192374,#192375,#192376,#192377,#192378,#192379,
#192380,#192381,#192382),(#192383,#192384,#192385,#192386,#192387,#192388,
#192389,#192390,#192391),(#192392,#192393,#192394,#192395,#192396,#192397,
#192398,#192399,#192400),(#192401,#192402,#192403,#192404,#192405,#192406,
#192407,#192408,#192409),(#192410,#192411,#192412,#192413,#192414,#192415,
#192416,#192417,#192418),(#192419,#192420,#192421,#192422,#192423,#192424,
#192425,#192426,#192427),(#192428,#192429,#192430,#192431,#192432,#192433,
#192434,#192435,#192436),(#192437,#192438,#192439,#192440,#192441,#192442,
#192443,#192444,#192445),(#192446,#192447,#192448,#192449,#192450,#192451,
#192452,#192453,#192454),(#192455,#192456,#192457,#192458,#192459,#192460,
#192461,#192462,#192463),(#192464,#192465,#192466,#192467,#192468,#192469,
#192470,#192471,#192472),(#192473,#192474,#192475,#192476,#192477,#192478,
#192479,#192480,#192481),(#192482,#192483,#192484,#192485,#192486,#192487,
#192488,#192489,#192490),(#192491,#192492,#192493,#192494,#192495,#192496,
#192497,#192498,#192499),(#192500,#192501,#192502,#192503,#192504,#192505,
#192506,#192507,#192508),(#192509,#192510,#192511,#192512,#192513,#192514,
#192515,#192516,#192517),(#192518,#192519,#192520,#192521,#192522,#192523,
#192524,#192525,#192526),(#192527,#192528,#192529,#192530,#192531,#192532,
#192533,#192534,#192535),(#192536,#192537,#192538,#192539,#192540,#192541,
#192542,#192543,#192544),(#192545,#192546,#192547,#192548,#192549,#192550,
#192551,#192552,#192553),(#192554,#192555,#192556,#192557,#192558,#192559,
#192560,#192561,#192562),(#192563,#192564,#192565,#192566,#192567,#192568,
#192569,#192570,#192571),(#192572,#192573,#192574,#192575,#192576,#192577,
#192578,#192579,#192580),(#192581,#192582,#192583,#192584,#192585,#192586,
#192587,#192588,#192589),(#192590,#192591,#192592,#192593,#192594,#192595,
#192596,#192597,#192598),(#192599,#192600,#192601,#192602,#192603,#192604,
#192605,#192606,#192607),(#192608,#192609,#192610,#192611,#192612,#192613,
#192614,#192615,#192616),(#192617,#192618,#192619,#192620,#192621,#192622,
#192623,#192624,#192625),(#192626,#192627,#192628,#192629,#192630,#192631,
#192632,#192633,#192634),(#192635,#192636,#192637,#192638,#192639,#192640,
#192641,#192642,#192643),(#192644,#192645,#192646,#192647,#192648,#192649,
#192650,#192651,#192652),(#192653,#192654,#192655,#192656,#192657,#192658,
#192659,#192660,#192661),(#192662,#192663,#192664,#192665,#192666,#192667,
#192668,#192669,#192670),(#192671,#192672,#192673,#192674,#192675,#192676,
#192677,#192678,#192679),(#192680,#192681,#192682,#192683,#192684,#192685,
#192686,#192687,#192688),(#192689,#192690,#192691,#192692,#192693,#192694,
#192695,#192696,#192697),(#192698,#192699,#192700,#192701,#192702,#192703,
#192704,#192705,#192706),(#192707,#192708,#192709,#192710,#192711,#192712,
#192713,#192714,#192715),(#192716,#192717,#192718,#192719,#192720,#192721,
#192722,#192723,#192724),(#192725,#192726,#192727,#192728,#192729,#192730,
#192731,#192732,#192733),(#192734,#192735,#192736,#192737,#192738,#192739,
#192740,#192741,#192742),(#192743,#192744,#192745,#192746,#192747,#192748,
#192749,#192750,#192751),(#192752,#192753,#192754,#192755,#192756,#192757,
#192758,#192759,#192760),(#192761,#192762,#192763,#192764,#192765,#192766,
#192767,#192768,#192769),(#192770,#192771,#192772,#192773,#192774,#192775,
#192776,#192777,#192778),(#192779,#192780,#192781,#192782,#192783,#192784,
#192785,#192786,#192787),(#192788,#192789,#192790,#192791,#192792,#192793,
#192794,#192795,#192796),(#192797,#192798,#192799,#192800,#192801,#192802,
#192803,#192804,#192805),(#192806,#192807,#192808,#192809,#192810,#192811,
#192812,#192813,#192814),(#192815,#192816,#192817,#192818,#192819,#192820,
#192821,#192822,#192823),(#192824,#192825,#192826,#192827,#192828,#192829,
#192830,#192831,#192832),(#192833,#192834,#192835,#192836,#192837,#192838,
#192839,#192840,#192841),(#192842,#192843,#192844,#192845,#192846,#192847,
#192848,#192849,#192850),(#192851,#192852,#192853,#192854,#192855,#192856,
#192857,#192858,#192859),(#192860,#192861,#192862,#192863,#192864,#192865,
#192866,#192867,#192868),(#192869,#192870,#192871,#192872,#192873,#192874,
#192875,#192876,#192877),(#192878,#192879,#192880,#192881,#192882,#192883,
#192884,#192885,#192886),(#192887,#192888,#192889,#192890,#192891,#192892,
#192893,#192894,#192895),(#192896,#192897,#192898,#192899,#192900,#192901,
#192902,#192903,#192904),(#192905,#192906,#192907,#192908,#192909,#192910,
#192911,#192912,#192913),(#192914,#192915,#192916,#192917,#192918,#192919,
#192920,#192921,#192922),(#192923,#192924,#192925,#192926,#192927,#192928,
#192929,#192930,#192931),(#192932,#192933,#192934,#192935,#192936,#192937,
#192938,#192939,#192940),(#192941,#192942,#192943,#192944,#192945,#192946,
#192947,#192948,#192949),(#192950,#192951,#192952,#192953,#192954,#192955,
#192956,#192957,#192958),(#192959,#192960,#192961,#192962,#192963,#192964,
#192965,#192966,#192967),(#192968,#192969,#192970,#192971,#192972,#192973,
#192974,#192975,#192976),(#192977,#192978,#192979,#192980,#192981,#192982,
#192983,#192984,#192985),(#192986,#192987,#192988,#192989,#192990,#192991,
#192992,#192993,#192994),(#192995,#192996,#192997,#192998,#192999,#193000,
#193001,#193002,#193003),(#193004,#193005,#193006,#193007,#193008,#193009,
#193010,#193011,#193012),(#193013,#193014,#193015,#193016,#193017,#193018,
#193019,#193020,#193021),(#193022,#193023,#193024,#193025,#193026,#193027,
#193028,#193029,#193030),(#193031,#193032,#193033,#193034,#193035,#193036,
#193037,#193038,#193039),(#193040,#193041,#193042,#193043,#193044,#193045,
#193046,#193047,#193048),(#193049,#193050,#193051,#193052,#193053,#193054,
#193055,#193056,#193057),(#193058,#193059,#193060,#193061,#193062,#193063,
#193064,#193065,#193066),(#193067,#193068,#193069,#193070,#193071,#193072,
#193073,#193074,#193075),(#193076,#193077,#193078,#193079,#193080,#193081,
#193082,#193083,#193084),(#193085,#193086,#193087,#193088,#193089,#193090,
#193091,#193092,#193093),(#193094,#193095,#193096,#193097,#193098,#193099,
#193100,#193101,#193102),(#193103,#193104,#193105,#193106,#193107,#193108,
#193109,#193110,#193111),(#193112,#193113,#193114,#193115,#193116,#193117,
#193118,#193119,#193120),(#193121,#193122,#193123,#193124,#193125,#193126,
#193127,#193128,#193129),(#193130,#193131,#193132,#193133,#193134,#193135,
#193136,#193137,#193138),(#193139,#193140,#193141,#193142,#193143,#193144,
#193145,#193146,#193147),(#193148,#193149,#193150,#193151,#193152,#193153,
#193154,#193155,#193156),(#193157,#193158,#193159,#193160,#193161,#193162,
#193163,#193164,#193165),(#193166,#193167,#193168,#193169,#193170,#193171,
#193172,#193173,#193174),(#193175,#193176,#193177,#193178,#193179,#193180,
#193181,#193182,#193183)),.UNSPECIFIED.,.F.,.T.,.F.)
B_SPLINE_SURFACE_WITH_KNOTS((4,1,1,1,1,1,1,1,1,1,1,1,1,1,1,1,1,1,1,1,1,
1,1,1,1,1,1,1,1,1,1,1,1,1,1,1,1,1,1,1,1,1,1,1,1,1,1,1,1,1,1,1,1,1,1,1,1,
1,1,1,1,1,1,1,1,1,1,1,1,1,1,1,1,1,1,1,1,1,1,1,1,1,1,1,1,1,1,1,1,1,1,1,1,
1,1,1,1,1,1,1,1,1,1,1,1,1,1,1,1,1,1,1,1,1,1,1,1,1,1,1,1,1,1,1,1,1,1,1,1,
1,1,1,1,1,1,1,1,1,1,1,1,1,1,1,1,1,1,1,1,1,1,1,1,1,1,1,1,1,1,1,1,1,1,1,1,
1,1,1,1,1,1,1,1,1,1,1,1,1,1,1,1,1,1,1,1,1,1,1,1,1,1,1,1,1,1,1,1,1,1,1,1,
1,1,1,1,1,1,1,1,1,1,1,1,1,1,1,1,1,1,1,1,1,1,1,1,1,1,1,1,1,1,1,1,1,1,1,1,
1,1,1,1,1,1,1,1,1,1,1,1,1,1,1,1,1,1,1,1,1,1,1,1,1,1,1,1,1,1,1,1,1,1,1,1,
1,1,1,1,1,1,1,1,1,1,1,1,1,1,1,1,1,1,1,1,1,1,1,1,1,1,1,1,1,1,1,1,1,1,1,1,
1,1,1,1,1,1,1,1,1,1,1,1,1,1,1,1,1,1,1,1,1,1,1,1,1,1,1,1,1,1,1,1,1,1,1,1,
1,1,1,1,1,1,1,1,1,1,1,1,1,1,1,1,1,1,1,1,1,1,1,1,1,1,1,1,1,1,1,1,1,1,1,1,
1,1,1,1,1,1,1,1,1,1,1,1,1,1,1,1,1,1,1,1,1,1,1,1,1,1,1,1,1,1,1,1,1,1,1,1,
1,1,1,1,1,1,1,1,1,1,1,1,1,1,1,1,1,1,1,1,1,1,1,1,1,1,1,1,1,1,1,1,1,1,1,1,
1,1,1,1,1,1,1,1,1,1,1,1,1,1,1,1,1,1,1,1,1,1,1,1,1,1,1,1,1,1,1,1,1,1,1,1,
1,1,1,1,1,1,1,1,1,1,1,1,1,1,1,1,1,1,1,1,1,1,1,1,1,1,1,1,1,1,1,1,1,1,1,1,
1,1,1,1,1,1,1,1,1,1,1,1,1,1,1,1,1,1,1,1,1,1,1,1,1,1,1,1,1,1,1,1,1,1,1,1,
1,1,1,1,1,1,1,1,1,1,1,1,1,1,1,1,1,1,1,1,1,1,1,1,1,1,1,1,1,1,1,1,1,1,1,1,
1,1,1,1,1,1,1,1,1,1,1,1,1,1,1,1,1,1,1,1,1,1,1,1,1,1,1,1,1,1,1,1,1,1,1,1,
1,1,1,1,1,1,1,1,1,1,1,1,1,1,1,1,1,1,1,1,1,1,1,1,1,1,1,1,1,1,1,1,1,1,1,1,
1,1,1,1,1,1,1,1,1,1,1,1,1,1,1,1,1,1,1,1,1,1,1,1,1,1,1,1,1,1,1,1,1,1,1,1,
1,1,1,1,1,1,1,1,1,1,1,1,1,1,1,1,1,1,1,1,1,1,1,1,1,1,1,1,1,1,1,1,1,1,1,1,
1,1,1,1,1,1,1,1,1,1,1,1,1,1,1,1,1,1,1,1,1,1,1,1,1,1,1,1,1,1,1,1,1,1,1,1,
1,1,1,1,1,1,1,1,1,1,1,1,1,1,1,1,1,1,1,1,1,1,1,1,1,1,1,1,1,1,1,1,1,1,1,1,
1,1,1,1,1,1,1,1,1,1,1,1,1,1,1,1,1,1,1,1,1,1,1,1,1,1,1,1,1,1,1,1,1,1,1,1,
1,1,1,1,1,1,1,1,1,1,1,1,1,1,1,1,1,1,1,1,1,1,1,1,1,1,1,1,1,1,1,1,1,1,1,1,
1,1,1,1,1,1,1,1,1,1,1,1,1,1,1,1,1,1,1,1,1,1,1,1,1,1,1,1,1,1,1,1,1,1,1,1,
1,1,1,1,1,1,1,1,1,1,1,1,1,1,1,1,1,1,1,1,1,1,1,1,1,1,1,1,1,1,1,1,1,1,1,1,
1,1,1,1,1,1,1,1,1,1,1,1,1,1,1,1,1,1,1,1,1,1,1,1,1,1,1,1,1,1,1,1,1,1,1,1,
1,1,1,1,1,1,1,1,1,1,1,1,1,1,1,1,1,1,1,1,1,1,1,1,1,1,1,1,1,1,1,1,1,1,1,1,
1,1,1,1,1,1,1,1,1,1,1,1,1,1,1,1,1,1,1,1,1,1,1,1,1,1,1,1,1,1,1,1,1,1,1,1,
1,1,1,1,1,1,1,1,1,1,1,1,1,1,1,1,1,1,1,1,1,1,1,1,1,1,1,1,1,1,1,1,1,1,1,1,
1,1,1,1,1,1,1,1,1,1,1,1,1,1,1,1,1,1,1,1,1,1,1,1,1,1,1,1,1,1,1,1,1,1,1,1,
1,1,1,1,1,1,1,1,1,1,1,1,1,1,1,1,1,1,1,1,1,1,1,1,1,1,1,1,1,1,1,1,1,1,1,1,
1,1,1,1,1,1,1,1,1,1,1,1,1,1,1,1,1,1,1,1,1,1,1,1,1,1,1,1,1,1,1,1,1,1,1,1,
1,1,1,1,1,1,1,1,1,1,1,1,1,1,1,1,1,1,1,1,1,1,1,1,1,1,1,1,1,1,1,1,1,1,1,1,
1,1,1,1,1,1,1,1,1,1,1,1,1,1,1,1,1,1,1,1,1,1,1,1,1,1,1,1,1,1,1,1,1,1,1,1,
1,1,1,1,1,1,1,1,1,1,1,1,1,1,1,1,1,1,1,1,1,1,1,1,1,1,1,1,1,1,1,1,1,1,1,1,
1,1,1,1,1,1,1,1,1,1,1,1,1,1,1,1,1,1,1,1,1,1,1,1,1,1,1,1,1,1,1,1,1,1,1,1,
1,1,1,1,1,1,1,1,1,1,1,1,1,1,1,1,1,1,1,1,1,1,1,1,1,1,1,1,1,1,1,1,1,1,1,1,
1,1,1,1,1,1,1,1,1,1,1,1,1,1,1,1,1,1,1,1,1,1,1,1,1,1,1,1,1,1,1,1,1,1,1,1,
1,1,1,1,1,1,1,1,1,1,1,1,1,1,1,1,1,1,1,1,1,1,1,1,1,1,1,1,1,1,1,1,1,1,1,1,
1,1,1,1,1,1,1,1,1,1,1,1,1,1,1,1,1,1,1,1,1,1,1,1,1,1,1,1,1,1,1,1,1,1,1,1,
1,1,1,1,1,1,1,1,1,1,1,1,1,1,1,1,1,1,1,1,1,1,1,1,1,1,1,1,1,1,1,1,1,1,1,1,
1,1,1,1,1,1,1,1,1,1,1,1,1,1,1,1,1,1,1,1,1,1,1,1,1,1,1,1,1,1,1,1,1,1,1,1,
1,1,1,1,1,1,1,1,1,1,1,1,1,1,1,1,1,1,1,1,1,1,1,1,1,1,1,1,1,1,1,1,1,1,1,1,
1,1,1,1,1,1,1,1,1,1,1,1,1,1,1,1,1,1,1,1,1,1,1,1,1,1,1,1,1,1,1,1,1,1,1,1,
1,1,1,1,1,1,1,1,1,1,1,1,1,1,1,1,1,1,1,1,1,1,1,1,1,1,1,1,1,1,1,1,1,1,1,1,
1,1,1,1,1,1,1,1,1,1,1,1,1,1,1,1,1,1,1,1,1,1,1,1,1,1,1,1,1,1,1,1,1,1,1,1,
1,1,1,1,1,1,1,1,1,1,1,1,1,1,1,1,1,1,1,1,1,1,1,1,1,1,1,1,1,1,1,1,1,1,1,1,
1,1,1,1,1,1,1,1,1,1,1,1,1,1,1,1,1,1,1,1,1,1,1,1,1,1,1,1,1,1,1,1,1,1,1,1,
1,1,1,1,1,1,1,1,1,1,1,1,1,1,1,1,1,1,1,1,1,1,1,1,1,1,1,1,1,1,1,1,1,1,1,1,
1,1,1,1,1,1,1,1,1,1,1,1,1,1,1,1,1,1,1,1,1,1,1,1,1,1,1,1,1,1,1,1,1,1,1,1,
1,1,1,1,1,1,1,1,1,1,1,1,1,1,1,1,1,1,1,1,1,1,1,1,1,1,1,1,1,1,1,1,1,1,1,1,
1,1,1,1,1,1,1,1,1,1,1,1,1,1,1,1,1,1,1,1,1,1,1,1,1,1,1,1,1,1,1,1,1,1,1,1,
1,1,1,1,1,1,1,1,1,1,1,1,1,1,1,1,1,1,1,1,1,1,1,1,1,1,1,1,1,1,1,1,1,1,1,1,
1,1,1,1,1,1,1,1,1,1,1,1,1,1,1,1,1,1,1,1,1,1,1,1,1,1,1,1,1,1,1,1,1,1,1,1,
1,1,1,1,1,1,1,1,1,1,1,1,1,1,1,1,1,1,1,1,1,1,1,1,1,1,1,1,1,1,1,1,1,1,1,1,
1,1,1,1,1,1,1,1,1,1,1,4),(3,2,2,2,3),(0.,0.01797683372391,0.286633051710584,
0.555289278308216,0.823945516665782,1.09260176953922,1.36125803873948,1.62991432588463,
1.89857063164012,2.16722695661301,2.43588330050525,2.70453966304674,2.9731960431531,
3.24185243981471,3.51050885133453,3.77916527610465,4.04782171198515,4.31647815691489,
4.58513460847725,4.85379106430677,5.12244752187208,5.39110397865606,5.65976043217153,
5.92841687990537,6.19707331956994,6.46572974881596,6.73438616570634,7.00304256821933,
7.2716989549161,7.5403553242696,7.809011675483,8.07766800769526,8.34632432089157,
8.61498061505147,8.8836368910788,9.15229314997201,9.4209493936865,9.68960562442157,
9.95826184531348,10.226918059948,10.4955742727586,10.7642304884925,11.0328867113173,
11.3015429448574,11.5701991918227,11.8388554546081,12.1075117346518,12.3761680332469,
12.6448243507434,12.9134806874637,13.1821370428496,13.450793416388,13.7194498067883,
13.9881062128412,14.2567626326955,14.5254190645885,14.7940755062772,15.0627319555912,
15.3313884100611,15.6000448672586,15.8687013246492,16.1373577797,16.4060142299691,
16.6746706729765,16.9433271065265,17.2119835283531,17.4806399366567,17.7492963295502,
18.0179527057767,18.286609063996,18.555265403637,18.8239217240786,19.0925780255742,
19.3612343083975,19.6298905737625,19.898546823017,20.1672030584666,20.4358592827168,
20.7045154992928,20.973171712245,21.2418279262962,21.5104841459723,21.7791403749736,
22.0477966165324,22.316452872948,22.585109146262,22.8537654375589,23.1224217478187,
23.3910780770929,23.6597344254327,23.9283907920352,24.197047176159,24.4657035763222,
24.7343599911301,25.0030164185931,25.2716728568073,25.5403293034427,25.8089857562333,
26.0776422126729,26.3462986702843,26.6149551265448,26.8836115789212,27.1522680250308,
27.4209244624423,27.6895808890659,27.9582373027346,28.2268937018004,28.4955500845261,
28.7642064498512,29.0328627966379,29.3015191245544,29.5701754332357,29.838831723217,
30.1074879950829,30.3761442503694,30.6448004907916,30.9134567190168,31.1821129380756,
31.450769151893,31.7194253649682,31.9880815819663,32.2567378070174,32.5253940433706,
32.7940502938785,33.0627065604467,33.3313628447765,33.6000191476151,33.8686754696427,
34.1373318106287,34.405988170366,34.6746445478242,34.9433009420458,35.2119573513747,
35.480613774244,35.7492702085419,36.0179266522368,36.2865831029275,36.5552395582669,
36.8238960157264,37.0925524727952,37.3612089269773,37.6298653757534,37.8985218168153,
38.1671782477952,38.4358346667239,38.7044910715485,38.9731474607866,39.2418038328672,
39.5104601869391,39.7791165220837,40.0477728382212,40.3164291352602,40.5850854140292,
40.8537416754418,41.1223979213679,41.3910541539077,41.6597103761025,41.9283665914244,
42.1970228042084,42.4656790192,42.7343352406829,43.0029914723808,43.2716477171096,
43.540303977354,43.8089602546436,44.0776165503516,44.3462728649052,44.614929198697,
44.883585551232,45.1522419220568,45.4208983099307,45.6895547136931,45.9582111315299,
46.2268675617156,46.4955240020317,46.7641804503338,47.0328369041642,47.3014933611089,
47.5701498186329,47.8388062742058,48.107462725373,48.3761191696448,48.6447756048012,
48.9134320285537,49.1820884390673,49.4507448344197,49.7194012133072,49.9880575743413,
50.2567139168934,50.5253702402807,50.7940265446884,51.0626828303152,51.3313390982961,
51.5999953498901,51.8686515873141,52.1373078130706,52.4059640305862,52.6746202437936,
52.9432764573682,53.211932675918,53.480588903259,53.7492451427202,54.0179013967021,
54.2865576673334,54.5552139557853,54.823870263115,55.0925265894471,55.3611829348992,
55.6298392987282,55.8984956802486,56.1671520780245,56.4358084907065,56.7044649163381,
56.9731213530494,57.2417777985307,57.5104342505384,57.7790907065743,58.0477471641719,
58.3164036208043,58.5850600739368,58.8537165211707,59.1223729600609,59.39102938849,
59.6596858042645,59.9283422056975,60.1969985910129,60.4656549590995,60.7343113087676,
61.0029676396243,61.2716239512389,61.540280244075,61.808936518638,62.0775927763821,
62.3462490189291,62.6149052488546,62.8835614690812,63.1522176834332,63.4208738963055,
63.6895301124163,63.9581863359981,64.2268425704115,64.4954988186027,64.7641550825741,
65.0328113641112,65.3014676640435,65.5701239831253,65.8387803211949,66.1074366781083,
66.3760930528907,66.6447494446373,66.9134058517341,67.1820622726558,67.4507187053199,
67.7193751477252,67.988031597487,68.256688052277,68.5253445095709,68.7940009668648,
69.0626574216546,69.3313138714164,69.5999703138218,69.8686267464858,70.1372831674076,
70.4059395745042,70.6745959662509,70.9432523410334,71.2119086979469,71.4805650360164,
71.7492213550982,72.0178776550306,72.2865339365675,72.5551902005389,72.8238464487301,
73.0925026831433,73.3611589067251,73.6298151228357,73.8984713357081,74.1671275500599,
74.4357837702864,74.7044400002118,74.9730962427587,75.2417525005027,75.5104087750655,
75.7790650679015,76.047721379516,76.3163777103726,76.5850340600405,76.853690428127,
77.1223468134422,77.391003214875,77.6596596306495,77.9283160590784,78.1969724979684,
78.4656289452021,78.7342853983344,79.0029418549666,79.2715983125641,79.5402547685998,
79.8089112206075,80.0775676660886,80.3462241027997,80.6148805284312,80.8835369411131,
81.1521933388889,81.4208497204091,81.689506084238,81.9581624296899,82.2268187560219,
82.4954750633515,82.7641313518033,83.0327876224345,83.3014438764161,83.5701001158772,
83.838756343218,84.1074125617677,84.3760687753422,84.6447249885494,84.913381206065,
85.1820374318212,85.4506936692451,85.719349920839,85.9880061888197,86.2566624744465,
86.5253187788541,86.7939751022413,87.0626314447932,87.3312878058273,87.5999441847146,
87.8686005800667,88.1372569905802,88.4059134143327,88.6745698494889,88.9432262937606,
89.2118827449277,89.4805392005005,89.7491956580243,90.0178521149689,90.2865085687992,
90.5551650171012,90.8238214574172,91.0924778876028,91.3611343054394,91.6297907092016,
91.8984470970753,92.1671034679,92.4357598204347,92.7044161542264,92.9730724687798,
93.2417287644878,93.5103850417773,93.7790413020216,94.0476975467502,94.3163537784479,
94.5850099999307,94.8536662149221,95.1223224277061,95.390978643028,95.6596348652226,
95.9282910977624,96.1969473436883,96.4656036051009,96.7342598838697,97.0029161809086,
97.2715724970461,97.5402288321905,97.8088851862623,98.0775415583427,98.3461979475807,
98.6148543524051,98.8835107713336,99.1521672023136,99.4208236433754,99.6894800921513,
99.9581365463333,100.226793003402,100.495449460861,100.7641059162,101.032762366891,
101.301418810586,101.570075244884,101.838731667753,102.107388077082,102.376044471303,
102.644700848761,102.913357208498,103.182013549484,103.450669871511,103.71932617435,
103.98798245868,104.256638725248,104.525294975755,104.793951212108,105.062607437159,
105.331263654157,105.599919867233,105.86857608105,106.137232300108,106.405888528334,
106.674544768756,106.943201024042,107.211857295908,107.480513585889,107.74916989457,
108.017826222487,108.286482569273,108.555138934598,108.823795317324,109.09245171639,
109.361108130058,109.629764556682,109.898420994093,110.167077440202,110.435733892579,
110.704390348839,110.97304680645,111.24170326289,111.51035971568,111.779016162316,
112.04767260053,112.316329027993,112.5849854428,112.853641842963,113.122298227087,
113.39095459369,113.659610942029,113.928267271303,114.196923581563,114.46557987286,
114.734236146174,115.002892402589,115.271548644148,115.540204873149,115.808861092825,
116.077517306876,116.346173519828,116.614829736404,116.883485960654,117.152142196103,
117.420798445358,117.689454710722,117.958110993546,118.226767295041,118.495423615483,
118.764079955123,119.032736313343,119.301392689569,119.570049082462,119.838705490766,
120.107361912592,120.376018346142,120.644674789149,120.913331239418,121.181987694469,
121.45064415186,121.719300609057,121.987957063527,122.256613512841,122.525269954529,
122.793926386422,123.062582806276,123.331239212329,123.599895602729,123.868551976268,
124.137208331653,124.405864668374,124.67452098587,124.943177284465,125.211833564508,
125.480489827294,125.749146074259,126.017802307799,126.286458530624,126.555114746357,
126.823770959168,127.092427173802,127.361083394694,127.629739625429,127.898395869143,
128.167052128037,128.435708404064,128.704364698224,128.97302101142,129.241677343633,
129.510333694846,129.7789900642,130.047646450897,130.31630285341,130.5849592703,
130.853615699547,131.122272139211,131.390928586945,131.659585040461,131.928241497245,
132.19689795481,132.46555441064,132.734210862202,133.002867307132,133.271523743013,
133.540180167783,133.808836579303,134.077492975965,134.346149356071,134.614805718613,
134.883462062505,135.152118387478,135.420774693234,135.689430980379,135.958087249579,
136.226743502453,136.49539974081,136.76405596741,137.032712185392,137.301368398783,
137.570024612174,137.838680830155,138.107337056755,138.375993295112,138.644649547986,
138.913305817186,139.181962104332,139.450618410087,139.71927473506,139.987931078952,
140.256587441494,140.525243821601,140.793900218262,141.062556629782,141.331213054552,
141.599869490433,141.868525935363,142.137182386925,142.405838842755,142.67449530032,
142.943151757104,143.21180821062,143.480464658354,143.749121098019,144.017777527265,
144.286433944155,144.555090346668,144.823746733365,145.092403102719,145.361059453932,
145.629715786145,145.898372099341,146.167028393501,146.435684669529,146.704340928422,
146.972997172137,147.241653402872,147.510309623764,147.778965838398,148.047622051209,
148.316278266943,148.584934489768,148.853590723308,149.122246970274,149.390903233059,
149.659559513103,149.928215811698,150.196872129195,150.465528465915,150.734184821301,
151.00284119484,151.27149758524,151.540153991293,151.808810411148,152.077466843041,
152.34612328473,152.614779734044,152.883436188514,153.152092645711,153.420749103102,
153.689405558153,153.958062008422,154.22671845143,154.49537488498,154.764031306806,
155.03268771511,155.301344108004,155.57000048423,155.838656842449,156.107313182091,
156.375969502532,156.644625804028,156.913282086851,157.181938352216,157.450594601471,
157.719250836921,157.987907061171,158.256563277747,158.525219490699,158.793875704751,
159.062531924427,159.331188153428,159.599844394987,159.868500651403,160.137156924717,
160.405813216014,160.674469526274,160.943125855548,161.211782203888,161.480438570491,
161.749094954615,162.017751354778,162.286407769586,162.555064197049,162.823720635263,
163.092377081899,163.361033534689,163.629689991129,163.898346448741,164.167002905001,
164.435659357378,164.704315803488,164.972972240899,165.241628667523,165.510285081192,
165.778941480257,166.047597862983,166.316254228308,166.584910575095,166.853566903012,
167.122223211693,167.390879501675,167.659535773541,167.928192028827,168.19684826925,
168.465504497475,168.734160716534,169.002816930351,169.271473143427,169.540129360425,
169.808785585476,170.077441821829,170.346098072337,170.614754338905,170.883410623235,
171.152066926074,171.420723248102,171.689379589088,171.958035948825,172.226692326284,
172.495348720505,172.764005129834,173.032661552704,173.301317987002,173.569974430697,
173.838630881388,174.107287336727,174.375943794187,174.644600251255,174.913256705437,
175.181913154214,175.450569595276,175.719226026256,175.987882445184,176.256538850009,
176.525195239247,176.793851611328,177.0625079654,177.331164300545,177.599820616682,
177.868476913721,178.137133192491,178.405789453903,178.674445699829,178.943101932369,
179.211758154564,179.480414369886,179.74907058267,180.017726797662,180.286383019145,
180.555039250843,180.823695495572,181.092351755816,181.361008033106,181.629664328814,
181.898320643368,182.16697697716,182.435633329695,182.70428970052,182.972946088394,
183.241602492156,183.510258909993,183.778915340179,184.047571780495,184.316228228797,
184.584884682628,184.853541139572,185.122197597096,185.39085405267,185.659510503837,
185.928166948109,186.196823383265,186.465479807018,186.734136217531,187.002792612884,
187.271448991771,187.540105352806,187.808761695358,188.077418018745,188.346074323153,
188.61473060878,188.883386876761,189.152043128355,189.420699365779,189.689355591536,
189.958011809051,190.226668022259,190.495324235834,190.763980454383,191.032636681725,
191.301292921186,191.569949175168,191.838605445799,192.107261734251,192.375918041581,
192.644574367913,192.913230713365,193.181887077194,193.450543458715,193.719199856491,
193.987856269173,194.256512694805,194.525169131516,194.793825576997,195.062482029005,
195.331138485041,195.599794942639,195.868451399271,196.137107852404,196.405764299638,
196.674420738528,196.943077166957,197.211733582732,197.480389984165,197.749046369481,
198.017702737567,198.286359087236,198.555015418092,198.823671729707,199.092328022543,
199.360984297106,199.62964055485,199.898296797397,200.166953027323,200.43560924755,
200.704265461902,200.972921674774,201.241577890885,201.510234114467,201.77889034888,
202.047546597072,202.316202861043,202.584859142581,202.853515442513,203.122171761595,
203.390828099665,203.659484456579,203.928140831361,204.196797223108,204.465453630205,
204.734110051127,205.002766483791,205.271422926197,205.540079375959,205.808735830749,
206.077392288043,206.346048745337,206.614705200127,206.883361649889,207.152018092295,
207.420674524959,207.689330945881,207.957987352978,208.226643744725,208.495300119508,
208.763956476421,209.032612814491,209.301269133573,209.569925433505,209.838581715043,
210.107237979014,210.375894227206,210.644550461619,210.913206685201,211.181862901312,
211.450519114184,211.719175328536,211.987831548763,212.256487778689,212.525144021236,
212.79380027898,213.062456553543,213.331112846379,213.599769157994,213.868425488851,
214.137081838519,214.405738206606,214.674394591921,214.943050993354,215.211707409129,
215.480363837558,215.749020276448,216.017676723682,216.286333176815,216.554989633447,
216.823646091045,217.092302547081,217.360958999089,217.62961544457,217.898271881281,
218.166928306913,218.435584719595,218.704241117371,218.972897498892,219.241553862721,
219.510210208173,219.778866534505,220.047522841835,220.316179130287,220.584835400918,
220.8534916549,221.122147894361,221.390804121702,221.659460340252,221.928116553827,
222.196772767034,222.46542898455,222.734085210306,223.00274144773,223.271397699324,
223.540053967305,223.808710252932,224.07736655734,224.346022880728,224.61467922328,
224.883335584314,225.151991963201,225.420648358554,225.689304769068,225.95796119282,
226.226617627977,226.495274072249,226.763930523416,227.032586978989,227.301243436513,
227.569899893458,227.838556347288,228.10721279559,228.375869235907,228.644525666093,
228.913182083929,229.181838487692,229.450494875566,229.719151246391,229.987807598926,
230.256463932718,230.525120247271,230.79377654298,231.062432820269,231.331089080514,
231.599745325243,231.868401556941,232.137057778424,232.405713993415,232.674370206199,
232.943026421521,233.211682643716,233.480338876256,233.748995122182,234.017651383595,
234.286307662364,234.554963959403,234.823620275541,235.092276610685,235.360932964757,
235.629589336838,235.898245726076,236.166902130901,236.43555854983,236.70421498081,
236.972871421872,237.241527870648,237.51018432483,237.778840781899,238.047497239359,
238.316153694698,238.584810145389,238.853466589084,239.122123023382,239.390779446251,
239.65943585558,239.928092249802,240.19674862726,240.465404986998,240.734061327984,
241.002717650011,241.27137395285,241.54003023718,241.808686503748,242.077342754256,
242.345998990609,242.614655215661,242.883311432659,243.151967645734,243.420623859552,
243.68928007861,243.957936306836,244.226592547258,244.495248802545,244.763905074411,
245.032561364392,245.301217673074,245.56987400099,245.838530347777,246.107186713102,
246.375843095828,246.644499494894,246.913155908563,247.181812335186,247.450468772598,
247.719125218708,247.987781671084,248.256438127345,248.525094584956,248.793751041396,
249.062407494187,249.331063940822,249.599720379036,249.8683768065,250.137033221308,
250.405689621471,250.674346005595,250.943002372197,251.211658720537,251.480315049812,
251.748971360071,252.017627651368,252.286283924683,252.554940181098,252.823596422657,
253.092252651658,253.360908871335,253.629565085386,253.898221298338,254.166877514914,
254.435533739165,254.704189974614,254.972846223869,255.241502489234,255.510158772057,
255.778815073553,256.047471393995,256.316127733635,256.584784091854,256.85344046808,
257.122096860973,257.390753269276,257.659409691102,257.928066124652,258.196722567659,
258.465379017928,258.734035472978,259.002691930368,259.271348387566,259.540004842035,
259.808661291349,260.077317733037,260.345974164929,260.614630584783,260.883286990836,
261.151943381235,261.420599754774,261.689256110159,261.957912446879,262.226568764375,
262.49522506297,262.763881343014,263.032537605798,263.301193852763,263.569850086303,
263.838506309127,264.107162524861,264.375818737671,264.644474952305,264.913131173196,
265.181787403931,265.450443647645,265.719099906538,265.987756182565,266.256412476724,
266.52506878992,266.793725122132,267.062381473345,267.331037842698,267.599694229394,
267.868350631907,268.137007048797,268.405663478042,268.674319917706,268.94297636544,
269.211632818955,269.480289275739,269.748945733304,270.017602189133,270.286258640695,
270.554915085624,270.823571521504,271.092227946274,271.360884357793,271.629540754454,
271.89819713456,272.166853497101,272.435509840993,272.704166165965,272.97282247172,
273.241478758865,273.510135028065,273.778791280938,274.047447519295,274.316103745894,
274.584759963875,274.853416177266,275.122072390656,275.390728608637,275.659384835237,
275.928041073593,276.196697326466,276.465353595666,276.734009882811,277.002666188566,
277.271322513539,277.53997885743,277.808635219972,278.077291600077,278.345947996739,
278.614604408258,278.883260833028,279.151917268908,279.420573713837,279.689230165399,
279.957886621228,280.226543078793,280.495199535576,280.763855989092,281.032512436825,
281.301168876489,281.569825305735,281.838481722625,282.107138125138,282.375794511834,
282.644450881187,282.9131072324,283.181763564612,283.450419877808,283.719076171967,
283.987732447994,284.256388706887,284.525044950601,284.793701181336,285.062357402228,
285.331013616862,285.599669829672,285.868326045405,286.136982268229,286.405638501769,
286.674294748734,286.942951011519,287.211607291562,287.480263590157,287.748919907653,
288.017576244373,288.286232599758,288.554888973296,288.823545363696,289.092201769749,
289.360858189603,289.629514621495,289.898171063183,290.166827512497,290.435483966966,
290.704140424163,290.972796881554,291.241453336604,291.510109786873,291.77876622988,
292.047422663429,292.316079085255,292.584735493559,292.853391886452,293.122048262678,
293.390704620897,293.659360960537,293.928017280978,294.196673582474,294.465329865297,
294.733986130661,295.002642379915,295.271298615364,295.539954839614,295.808611056189,
296.077267269141,296.345923483192,296.614579702867,296.883235931868,297.151892173427,
297.420548429842,297.689204703155,297.957860994452,298.226517304711,298.495173633985,
298.763829982324,299.032486348927,299.30114273305,299.569799133212,299.83845554802,
300.107111975482,300.375768413696,300.644424860331,300.913081313121,301.181737769561,
301.450394227172,301.719050683432,301.987707135808,302.256363581917,302.525020019328,
302.793676445951,303.062332859619,303.330989258684,303.59964564141,303.868302006734,
304.136958353521,304.405614681437,304.674270990118,304.942927280098,305.211583551964,
305.48023980725,305.748896047671,306.017552275896,306.286208494954,306.554864708772,
306.823520921846,307.092177138844,307.360833363895,307.629489600247,307.898145850755,
308.166802117323,308.435458401652,308.70411470449,308.972771026517,309.241427367503,
309.51008372724,309.778740104698,310.047396498919,310.316052908247,310.584709331116,
310.853365765414,311.122022209108,311.390678659798,311.659335115137,311.927991572596,
312.196648029665,312.465304483846,312.733960932622,313.002617373684,313.271273804663,
313.539930223591,313.808586628416,314.077243017653,314.345899389733,314.614555743805,
314.883212078949,315.151868395086,315.420524692125,315.689180970894,315.957837232306,
316.226493478231,316.495149710771,316.763805932965,317.032462148286,317.30111836107,
317.569774576061,317.838430797543,318.107087029241,318.375743273969,318.644399534213,
318.913055811502,319.18171210721,319.450368421763,319.719024755555,319.987681108089,
320.256337478914,320.524993866787,320.793650270549,321.062306688385,321.33096311857,
321.599619558886,321.868276007188,322.136932461018,322.405588917962,322.674245375486,
322.942901831059,323.211558282225,323.480214726497,323.748871161653,324.017527585405,
324.286183995918,324.55484039127,324.823496770157,325.09215313119,325.360809473742,
325.629465797129,325.898122101536,326.166778387163,326.435434655143,326.704090906737,
326.97274714416,327.241403369916,327.510059587432,327.778715800638,328.047372014213,
328.316028232762,328.584684460102,328.853340699563,329.121996953545,329.390653224175,
329.659309512627,329.927965819956,330.196622146288,330.46527849174,330.733934855568,
331.002591237088,331.271247634863,331.539904047545,331.808560473176,332.077216909887,
332.345873355368,332.614529807375,332.883186263411,333.151842721008,333.42049917764,
333.689155630772,333.957812078005,334.226468516895,334.495124945324,334.763781361098,
335.03243776253,335.301094147845,335.569750515931,335.838406865599,336.107063196455,
336.375719508069,336.644375800905,336.913032075468,337.181688333211,337.450344575758,
337.719000805683,337.987657025909,338.256313240261,338.524969453133,338.793625669243,
339.062281892824,339.330938127237,339.599594375428,339.868250639399,340.136906920936,
340.405563220868,340.674219539949,340.942875878019,341.211532234932,341.480188609714,
341.74884500146,342.017501408557,342.286157829478,342.554814262142,342.823470704547,
343.092127154308,343.360783609098,343.629440066391,343.898096523685,344.166752978475,
344.435409428236,344.704065870641,344.972722303305,345.241378724226,345.510035131323,
345.778691523069,346.047347897851,346.316004254764,346.584660592834,346.853316911915,
347.121973211847,347.390629493384,347.659285757355,347.927942005546,348.196598239959,
348.46525446354,348.733910679651,349.002566892523,349.271223106874,349.5398793271,
349.808535557025,350.077191799572,350.345848057315,350.614504331878,350.883160624714,
351.151816936328,351.420473267184,351.689129616852,351.957785984938,352.226442370253,
352.495098771685,352.76375518746,353.032411615888,353.301068054778,353.569724502012,
353.838380955144,354.107037411776,354.375693869373,354.644350325408,354.913006777416,
355.181663222896,355.450319659607,355.718976085238,355.98763249792,356.256288895695,
356.524945277215,356.793601641044,357.062257986496,357.330914312827,357.599570620156,
357.868226908608,358.136883179239,358.40553943322,358.674195672681,358.942851900021,
359.211508118571,359.480164332145,359.748820545352,360.017476762867,360.286132988623,
360.554789226047,360.82344547764,361.09210174562,361.360758031247,361.629414335654,
361.898070659041,362.166727001593,362.435383362626,362.704039741513,362.972696136865,
363.241352547378,363.510008971131,363.778665406287,364.047321850558,364.315978301725,
364.584634757297,364.853291214821,365.121947671765,365.390604125595,365.659260573897,
365.927917014213,366.196573444398,366.465229862234,366.733886265996,367.002542653869,
367.271199024694,367.539855377228,367.808511711019,368.077168025573,368.34582432128,
368.614480598569,368.883136858813,369.151793103542,369.420449335239,369.689105556722,
369.957761771713,370.226417984496,370.495074199818,370.763730422012,371.032386654551,
371.301042900477,371.569699161889,371.838355440658,372.107011737697,372.375668053834,
372.644324388978,372.912980743049,373.18163711513,373.450293504367,373.718949909191,
373.98760632812,374.256262759099,374.524919200161,374.793575648936,375.062232103118,
375.330888560186,375.599545017646,375.868201472985,376.136857923675,376.40551436737,
376.674170801667,376.942827224536,377.211483633864,377.480140028085,377.748796405543,
378.01745276528,378.286109106266,378.554765428293,378.823421731131,379.092078015461,
379.360734282028,379.629390532536,379.898046768888,380.166702993939,380.435359210937,
380.704015424011,380.972671637828,381.241327856887,381.509984085112,381.778640325533,
382.047296580819,382.315952852685,382.584609142666,382.853265451347,383.121921779263,
383.390578126049,383.659234491374,383.927890874099,384.196547273165,384.465203686833,
384.733860113456,385.002516550867,385.271172996977,385.539829449352,385.808485905613,
386.077142363224,386.345798819663,386.614455272453,386.883111719088,387.151768157302,
387.420424584764,387.689080999572,387.957737399735,388.226393783858,388.49505015046,
388.7637064988,389.032362828074,389.301019138333,389.56967542963,389.838331702943,
390.106987959358,390.375644200917,390.644300429918,390.912956649593,391.181612863644,
391.450269076596,391.718925293171,391.987581517421,392.25623775287,392.524894002124,
392.793550267489,393.062206550312,393.330862851807,393.599519172248,393.868175511888,
394.136831870107,394.405488246334,394.674144639227,394.94280104753,395.211457469356,
395.480113902905,395.748770345913,396.017426796181,396.286083251232,396.554739708622,
396.823396165819,397.092052620289,397.360709069602,397.629365511291,397.898021943183,
398.166678363037,398.43533476909,398.703991159489,398.972647533028,399.241303888413,
399.509960225133,399.778616542629,400.047272841224,400.315929121267,400.584585384052,
400.853241631017,401.121897864557,401.390554087381,401.659210303115,401.927866515925,
402.196522730559,402.465178951451,402.733835182185,403.002491425899,403.271147684792,
403.539803960819,403.808460254978,404.077116568174,404.345772900386,404.614429251599,
404.883085620952,405.151742007649,405.420398410161,405.689054827051,405.957711256297,
406.226367695961,406.495024143695,406.76368059721,407.032337053993,407.300993511558,
407.569649967387,407.838306418949,408.106962863879,408.375619299759,408.644275724528,
408.912932136048,409.181588532709,409.450244912815,409.718901275356,409.987557619248,
410.25621394422,410.524870249975,410.79352653712,411.06218280632,411.330839059193,
411.599495297549,411.868151524149,412.13680774213,412.40546395552,412.674120168911,
412.942776386892,413.211432613491,413.480088851848,413.748745104721,414.017401373921,
414.286057661065,414.55471396682,414.823370291793,415.092026635685,415.360682998226,
415.629339378332,415.897995774993,416.166652186512,416.435308611282,416.703965047162,
416.972621492092,417.241277943654,417.509934399483,417.778590857048,418.047247313831,
418.315903767346,418.58456021508,418.853216654744,419.121873083989,419.390529500879,
419.659185903392,419.927842290088,420.196498659441,420.465155010654,420.733811342866,
421.002467656062,421.271123950222,421.539780226249,421.808436485141,422.077092728855,
422.34574895959,422.614405180482,422.883061395116,423.151717607926,423.42037382366,
423.689030046484,423.957686280024,424.226342526988,424.494998789773,424.763655069817,
425.032311368411,425.300967685907,425.569624022627,425.838280378013,426.106936751551,
426.375593141951,426.644249548003,426.912905967857,427.18156239975,427.450218841438,
427.718875290752,427.987531745221,428.256188202418,428.524844659809,428.793501114859,
429.062157565128,429.330814008135,429.599470441684,429.868126863511,430.136783271814,
430.405439664707,430.674096040933,430.942752399152,431.211408738792,431.480065059233,
431.748721360729,432.017377643552,432.286033908916,432.554690158171,432.823346393619,
433.092002617869,433.360658834445,433.629315047397,433.897971261447,434.166627481123,
434.435283710124,434.703939951682,434.972596208097,435.241252481411,435.509908772707,
435.778565082967,436.047221412241,436.31587776058,436.584534127182,436.853190511305,
437.121846911468,437.390503326275,437.659159753738,437.927816191952,438.196472638587,
438.465129091377,438.733785547816,439.002442005427,439.271098461688,439.539754914064,
439.808411360173,440.077067797584,440.345724224207,440.614380637875,440.883037036941,
441.151693419666,441.420349784991,441.689006131777,441.957662459693,442.226318768374,
442.494975058355,442.763631330221,443.032287585506,443.300943825928,443.569600054153,
443.838256273211,444.106912487028,444.375568700103,444.644224917101,444.912881142151,
445.181537378504,445.450193629011,445.718849895579,445.987506179909,446.256162482747,
446.524818804774,446.79347514576,447.062131505496,447.330787882954,447.599444277176,
447.868100686504,448.136757109373,448.40541354367,448.674069987365,448.942726438055,
449.211382893394,449.480039350853,449.748695807921,450.017352262103,450.286008710879,
450.55466515194,450.82332158292,451.091978001848,451.360634406672,451.62929079591,
451.89794716799,452.166603522061,452.435259857205,452.703916173343,452.972572470381,
453.24122874915,453.509885010562,453.778541256488,454.047197489028,454.315853711222,
454.584509926543,454.853166139327,455.121822354318,455.3904785758,455.659134807498,
455.927791052226,456.19644731247,456.465103589759,456.733759885467,457.00241620002,
457.271072533811,457.539728886346,457.80838525717,458.077041645044,458.345698048806,
458.614354466642,458.883010896827,459.151667337143,459.420323785445,459.688980239275,
459.957636696219,460.226293153743,460.494949609316,460.763606060482,461.032262504754,
461.300918939909,461.569575363662,461.838231774175,462.106888169527,462.375544548414,
462.644200909447,462.912857251999,463.181513575386,463.450169879794,463.71882616542,
463.987482433401,464.256138684994,464.524794922418,464.793451148174,465.062107365689,
465.330763578896,465.59941979247,465.86807601102,466.13673223836,466.405388477821,
466.674044731802,466.942701002433,467.211357290885,467.480013598214,467.748669924546,
468.017326269997,468.285982633826,468.554639015346,468.823295413121,469.091951825803,
469.360608251434,469.629264688145,469.897921133626,470.166577585633,470.435234041669,
470.703890499266,470.972546955898,471.24120340903,471.509859856263,471.778516295153,
472.047172723582,472.315829139356,472.584485540789,472.853141926103,473.12179829419,
473.390454643857,473.659110974714,473.927767286328,474.196423579164,474.465079853726,
474.73373611147,475.002392354016,475.271048583941,475.539704804167,475.808361018519,
476.077017231391,476.345673447501,476.614329671083,476.882985905496,477.151642153686,
477.420298417658,477.688954699194,477.957610999126,478.226267318208,478.494923656277,
478.76358001319,479.032236387973,479.300892779719,479.569549186815,479.838205607737,
480.106862040401,480.375518482806,480.644174932567,480.912831387357,481.18148784465,
481.450144301944,481.718800756733,481.987457206495,482.2561136489,482.524770081563,
482.793426502485,483.062082909582,483.330739301328,483.59939567611,483.868052033023,
484.136708371092,484.405364690174,484.674020990106,484.942677271643,485.211333535614,
485.479989783805,485.748646018218,486.017302241799,486.28595845791,486.554614670781,
486.823270885133,487.091927105359,487.360583335284,487.629239577831,487.897895835574,
488.166552110137,488.435208402973,488.703864714587,488.972521045443,489.241177395111,
489.509833763197,489.778490148512,490.047146549945,490.315802965719,490.584459394147,
490.853115833037,491.12177228027,491.390428733402,491.659085190034,491.927741647632,
492.196398103667,492.465054555674,492.733711001155,493.002367437866,493.271023863497,
493.539680276179,493.808336673954,494.076993055474,494.345649419303,494.614305764754,
494.882962091086,495.151618398416,495.420274686867,495.688930957498,495.95758721148,
496.22624345094,496.494899678281,496.76355589683,497.032212110404,497.300868323611,
497.569524541126,497.838180766882,498.106837004306,498.3754932559,498.64414952388,
498.912805809507,499.181462113914,499.450118437301,499.718774779852,499.987431140886,
500.256087519773,500.524743915125,500.793400325638,501.06205674939,501.330713184546,
501.599369628818,501.868026079984,502.136682535557,502.40533899308,502.673995450025,
502.942651903855,503.211308352156,503.479964792472,503.748621222657,504.017277640494,
504.285934044256,504.554590432129,504.823246802954,505.091903155488,505.360559489279,
505.629215803832,505.89787209954,506.166528376829,506.435184637073,506.703840881801,
506.972497113499,507.241153334981,507.509809549972,507.778465762756,508.047121978078,
508.315778200272,508.584434432811,508.853090678737,509.121746940149,509.390403218918,
509.659059515956,509.927715832093,510.196372167238,510.465028521309,510.733684893389,
511.002341282627,511.270997687451,511.53965410638,511.808310537359,512.076966978421,
512.345623427198,512.614279881382,512.882936338452,513.151592795914,513.420249251254,
513.688905701946,513.957562145643,514.226218579942,514.494875002812,514.763531412143,
515.032187806366,515.300844183826,515.569500543564,515.838156884552,516.106813206581,
516.375469509421,516.644125793752,516.912782060321,517.181438310831,517.450094547186,
517.718750772238,517.987406989238,518.256063202315,518.524719416134,518.793375635194,
519.062031863421,519.330688103845,519.599344359133,519.868000631,520.136656920983,
520.405313229665,520.673969557583,520.942625904371,521.211282269698,521.479938652425,
521.748595051492,522.017251465163,522.285907891788,522.554564329201,522.823220775312,
523.091877227689,523.360533683951,523.629190141564,523.897846598005,524.166503050797,
524.435159497434,524.70381593565,524.972472363114,525.241128777924,525.509785178088,
525.778441562214,526.047097928818,526.315754277159,526.584410606435,526.853066916696,
527.121723207994,527.390379481309,527.659035737726,527.927691979287,528.19634820829,
528.465004427967,528.73366064202,529.002316854973,529.270973071551,529.539629295803,
529.808285531254,530.07694178051,530.345598045876,530.614254328701,530.882910630198,
531.151566950641,531.420223290284,531.688879648504,531.957536024733,532.226192417628,
532.494848825933,532.76350524776,533.032161681312,533.30081812432,533.569474574591,
533.838131029643,534.106787487035,534.375443944235,534.644100398706,534.912756848021,
535.181413289711,535.450069721605,535.718726141461,535.987382547516,536.256038937917,
536.524695311458,536.793351666845,537.062008003567,537.330664321065,537.599320619661,
537.867976899706,538.136633162493,538.40528940946,538.673945643001,538.942601865828,
539.211258081563,539.479914294375,539.748570509011,540.017226729904,540.285882960641,
540.554539204357,540.823195463252,541.09185173928,541.360508033441,541.629164346639,
541.897820678853,542.166477030068,542.435133399423,542.703789786121,542.972446188636,
543.241102605527,543.509759034775,543.778415474441,544.047071922176,544.315728375693,
544.584384832479,544.853041290046,545.121697745877,545.390354197441,545.659010642372,
545.927667078254,546.196323503025,546.464979914547,546.733636311202,547.002292691334,
547.270949053789,547.539605397955,547.808261722147,548.076918029812,548.345574313508,
548.614230583738,548.882886864851,549.151542935882,549.420199787641,549.68885445376,
549.957511414581),(0.,0.117809724509617,0.235619449019234,0.353429173528852,
0.471238898038469),.UNSPECIFIED.)
GEOMETRIC_REPRESENTATION_ITEM()
RATIONAL_B_SPLINE_SURFACE(((1.,0.707106781186548,1.,0.707106781186548,1.,
0.707106781186548,1.,0.707106781186548,1.),(1.,0.707106781186548,1.,0.707106781186548,
1.,0.707106781186548,1.,0.707106781186548,1.),(1.,0.707106781186548,1.,
0.707106781186548,1.,0.707106781186548,1.,0.707106781186548,1.),(1.,0.707106781186547,
1.,0.707106781186547,1.,0.707106781186547,1.,0.707106781186547,1.),(1.,
0.707106781186547,1.,0.707106781186547,1.,0.707106781186547,1.,0.707106781186547,
1.),(1.,0.707106781186548,1.,0.707106781186548,1.,0.707106781186548,1.,
0.707106781186548,1.),(1.,0.707106781186547,1.,0.707106781186547,1.,0.707106781186547,
1.,0.707106781186547,1.),(1.,0.707106781186547,1.,0.707106781186547,1.,
0.707106781186547,1.,0.707106781186547,1.),(1.,0.707106781186547,1.,0.707106781186547,
1.,0.707106781186547,1.,0.707106781186547,1.),(1.,0.707106781186547,1.,
0.707106781186547,1.,0.707106781186547,1.,0.707106781186547,1.),(1.,0.707106781186547,
1.,0.707106781186547,1.,0.707106781186547,1.,0.707106781186547,1.),(1.,
0.707106781186548,1.,0.707106781186548,1.,0.707106781186548,1.,0.707106781186548,
1.),(1.,0.707106781186548,1.,0.707106781186548,1.,0.707106781186548,1.,
0.707106781186548,1.),(1.,0.707106781186548,1.,0.707106781186548,1.,0.707106781186548,
1.,0.707106781186548,1.),(1.,0.707106781186547,1.,0.707106781186547,1.,
0.707106781186547,1.,0.707106781186547,1.),(1.,0.707106781186548,1.,0.707106781186548,
1.,0.707106781186548,1.,0.707106781186548,1.),(1.,0.707106781186547,1.,
0.707106781186547,1.,0.707106781186547,1.,0.707106781186547,1.),(1.,0.707106781186547,
1.,0.707106781186547,1.,0.707106781186547,1.,0.707106781186547,1.),(1.,
0.707106781186548,1.,0.707106781186548,1.,0.707106781186548,1.,0.707106781186548,
1.),(1.,0.707106781186547,1.,0.707106781186547,1.,0.707106781186547,1.,
0.707106781186547,1.),(1.,0.707106781186548,1.,0.707106781186548,1.,0.707106781186548,
1.,0.707106781186548,1.),(1.,0.707106781186547,1.,0.707106781186547,1.,
0.707106781186547,1.,0.707106781186547,1.),(1.,0.707106781186548,1.,0.707106781186548,
1.,0.707106781186548,1.,0.707106781186548,1.),(1.,0.707106781186547,1.,
0.707106781186547,1.,0.707106781186547,1.,0.707106781186547,1.),(1.,0.707106781186548,
1.,0.707106781186548,1.,0.707106781186548,1.,0.707106781186548,1.),(1.,
0.707106781186547,1.,0.707106781186547,1.,0.707106781186547,1.,0.707106781186547,
1.),(1.,0.707106781186547,1.,0.707106781186547,1.,0.707106781186547,1.,
0.707106781186547,1.),(1.,0.707106781186547,1.,0.707106781186547,1.,0.707106781186547,
1.,0.707106781186547,1.),(1.,0.707106781186547,1.,0.707106781186547,1.,
0.707106781186547,1.,0.707106781186547,1.),(1.,0.707106781186547,1.,0.707106781186547,
1.,0.707106781186547,1.,0.707106781186547,1.),(1.,0.707106781186548,1.,
0.707106781186548,1.,0.707106781186548,1.,0.707106781186548,1.),(1.,0.707106781186547,
1.,0.707106781186547,1.,0.707106781186547,1.,0.707106781186547,1.),(1.,
0.707106781186547,1.,0.707106781186547,1.,0.707106781186547,1.,0.707106781186547,
1.),(1.,0.707106781186548,1.,0.707106781186548,1.,0.707106781186548,1.,
0.707106781186548,1.),(1.,0.707106781186547,1.,0.707106781186547,1.,0.707106781186547,
1.,0.707106781186547,1.),(1.,0.707106781186547,1.,0.707106781186547,1.,
0.707106781186547,1.,0.707106781186547,1.),(1.,0.707106781186548,1.,0.707106781186548,
1.,0.707106781186548,1.,0.707106781186548,1.),(1.,0.707106781186547,1.,
0.707106781186547,1.,0.707106781186547,1.,0.707106781186547,1.),(1.,0.707106781186547,
1.,0.707106781186547,1.,0.707106781186547,1.,0.707106781186547,1.),(1.,
0.707106781186548,1.,0.707106781186548,1.,0.707106781186548,1.,0.707106781186548,
1.),(1.,0.707106781186548,1.,0.707106781186548,1.,0.707106781186548,1.,
0.707106781186548,1.),(1.,0.707106781186547,1.,0.707106781186547,1.,0.707106781186547,
1.,0.707106781186547,1.),(1.,0.707106781186548,1.,0.707106781186548,1.,
0.707106781186548,1.,0.707106781186548,1.),(1.,0.707106781186547,1.,0.707106781186547,
1.,0.707106781186547,1.,0.707106781186547,1.),(1.,0.707106781186547,1.,
0.707106781186547,1.,0.707106781186547,1.,0.707106781186547,1.),(1.,0.707106781186547,
1.,0.707106781186547,1.,0.707106781186547,1.,0.707106781186547,1.),(1.,
0.707106781186548,1.,0.707106781186548,1.,0.707106781186548,1.,0.707106781186548,
1.),(1.,0.707106781186548,1.,0.707106781186548,1.,0.707106781186548,1.,
0.707106781186548,1.),(1.,0.707106781186547,1.,0.707106781186547,1.,0.707106781186547,
1.,0.707106781186547,1.),(1.,0.707106781186547,1.,0.707106781186547,1.,
0.707106781186547,1.,0.707106781186547,1.),(1.,0.707106781186548,1.,0.707106781186548,
1.,0.707106781186548,1.,0.707106781186548,1.),(1.,0.707106781186547,1.,
0.707106781186547,1.,0.707106781186547,1.,0.707106781186547,1.),(1.,0.707106781186548,
1.,0.707106781186548,1.,0.707106781186548,1.,0.707106781186548,1.),(1.,
0.707106781186547,1.,0.707106781186547,1.,0.707106781186547,1.,0.707106781186547,
1.),(1.,0.707106781186547,1.,0.707106781186547,1.,0.707106781186547,1.,
0.707106781186547,1.),(1.,0.707106781186547,1.,0.707106781186547,1.,0.707106781186547,
1.,0.707106781186547,1.),(1.,0.707106781186547,1.,0.707106781186547,1.,
0.707106781186547,1.,0.707106781186547,1.),(1.,0.707106781186547,1.,0.707106781186547,
1.,0.707106781186547,1.,0.707106781186547,1.),(1.,0.707106781186548,1.,
0.707106781186548,1.,0.707106781186548,1.,0.707106781186548,1.),(1.,0.707106781186547,
1.,0.707106781186547,1.,0.707106781186547,1.,0.707106781186547,1.),(1.,
0.707106781186548,1.,0.707106781186548,1.,0.707106781186548,1.,0.707106781186548,
1.),(1.,0.707106781186547,1.,0.707106781186547,1.,0.707106781186547,1.,
0.707106781186547,1.),(1.,0.707106781186548,1.,0.707106781186548,1.,0.707106781186548,
1.,0.707106781186548,1.),(1.,0.707106781186547,1.,0.707106781186547,1.,
0.707106781186547,1.,0.707106781186547,1.),(1.,0.707106781186548,1.,0.707106781186548,
1.,0.707106781186548,1.,0.707106781186548,1.),(1.,0.707106781186547,1.,
0.707106781186547,1.,0.707106781186547,1.,0.707106781186547,1.),(1.,0.707106781186547,
1.,0.707106781186547,1.,0.707106781186547,1.,0.707106781186547,1.),(1.,
0.707106781186548,1.,0.707106781186548,1.,0.707106781186548,1.,0.707106781186548,
1.),(1.,0.707106781186547,1.,0.707106781186547,1.,0.707106781186547,1.,
0.707106781186547,1.),(1.,0.707106781186547,1.,0.707106781186547,1.,0.707106781186547,
1.,0.707106781186547,1.),(1.,0.707106781186548,1.,0.707106781186548,1.,
0.707106781186548,1.,0.707106781186548,1.),(1.,0.707106781186547,1.,0.707106781186547,
1.,0.707106781186547,1.,0.707106781186547,1.),(1.,0.707106781186548,1.,
0.707106781186548,1.,0.707106781186548,1.,0.707106781186548,1.),(1.,0.707106781186547,
1.,0.707106781186547,1.,0.707106781186547,1.,0.707106781186547,1.),(1.,
0.707106781186548,1.,0.707106781186548,1.,0.707106781186548,1.,0.707106781186548,
1.),(1.,0.707106781186548,1.,0.707106781186548,1.,0.707106781186548,1.,
0.707106781186548,1.),(1.,0.707106781186547,1.,0.707106781186547,1.,0.707106781186547,
1.,0.707106781186547,1.),(1.,0.707106781186548,1.,0.707106781186548,1.,
0.707106781186548,1.,0.707106781186548,1.),(1.,0.707106781186547,1.,0.707106781186547,
1.,0.707106781186547,1.,0.707106781186547,1.),(1.,0.707106781186547,1.,
0.707106781186547,1.,0.707106781186547,1.,0.707106781186547,1.),(1.,0.707106781186548,
1.,0.707106781186548,1.,0.707106781186548,1.,0.707106781186548,1.),(1.,
0.707106781186547,1.,0.707106781186547,1.,0.707106781186547,1.,0.707106781186547,
1.),(1.,0.707106781186547,1.,0.707106781186547,1.,0.707106781186547,1.,
0.707106781186547,1.),(1.,0.707106781186547,1.,0.707106781186547,1.,0.707106781186547,
1.,0.707106781186547,1.),(1.,0.707106781186548,1.,0.707106781186548,1.,
0.707106781186548,1.,0.707106781186548,1.),(1.,0.707106781186547,1.,0.707106781186547,
1.,0.707106781186547,1.,0.707106781186547,1.),(1.,0.707106781186547,1.,
0.707106781186547,1.,0.707106781186547,1.,0.707106781186547,1.),(1.,0.707106781186547,
1.,0.707106781186547,1.,0.707106781186547,1.,0.707106781186547,1.),(1.,
0.707106781186547,1.,0.707106781186547,1.,0.707106781186547,1.,0.707106781186547,
1.),(1.,0.707106781186547,1.,0.707106781186547,1.,0.707106781186547,1.,
0.707106781186547,1.),(1.,0.707106781186547,1.,0.707106781186547,1.,0.707106781186547,
1.,0.707106781186547,1.),(1.,0.707106781186548,1.,0.707106781186548,1.,
0.707106781186548,1.,0.707106781186548,1.),(1.,0.707106781186548,1.,0.707106781186548,
1.,0.707106781186548,1.,0.707106781186548,1.),(1.,0.707106781186547,1.,
0.707106781186547,1.,0.707106781186547,1.,0.707106781186547,1.),(1.,0.707106781186548,
1.,0.707106781186548,1.,0.707106781186548,1.,0.707106781186548,1.),(1.,
0.707106781186547,1.,0.707106781186547,1.,0.707106781186547,1.,0.707106781186547,
1.),(1.,0.707106781186548,1.,0.707106781186548,1.,0.707106781186548,1.,
0.707106781186548,1.),(1.,0.707106781186548,1.,0.707106781186548,1.,0.707106781186548,
1.,0.707106781186548,1.),(1.,0.707106781186547,1.,0.707106781186547,1.,
0.707106781186547,1.,0.707106781186547,1.),(1.,0.707106781186548,1.,0.707106781186548,
1.,0.707106781186548,1.,0.707106781186548,1.),(1.,0.707106781186548,1.,
0.707106781186548,1.,0.707106781186548,1.,0.707106781186548,1.),(1.,0.707106781186548,
1.,0.707106781186548,1.,0.707106781186548,1.,0.707106781186548,1.),(1.,
0.707106781186547,1.,0.707106781186547,1.,0.707106781186547,1.,0.707106781186547,
1.),(1.,0.707106781186548,1.,0.707106781186548,1.,0.707106781186548,1.,
0.707106781186548,1.),(1.,0.707106781186547,1.,0.707106781186547,1.,0.707106781186547,
1.,0.707106781186547,1.),(1.,0.707106781186548,1.,0.707106781186548,1.,
0.707106781186548,1.,0.707106781186548,1.),(1.,0.707106781186548,1.,0.707106781186548,
1.,0.707106781186548,1.,0.707106781186548,1.),(1.,0.707106781186548,1.,
0.707106781186548,1.,0.707106781186548,1.,0.707106781186548,1.),(1.,0.707106781186547,
1.,0.707106781186547,1.,0.707106781186547,1.,0.707106781186547,1.),(1.,
0.707106781186547,1.,0.707106781186547,1.,0.707106781186547,1.,0.707106781186547,
1.),(1.,0.707106781186547,1.,0.707106781186547,1.,0.707106781186547,1.,
0.707106781186547,1.),(1.,0.707106781186548,1.,0.707106781186548,1.,0.707106781186548,
1.,0.707106781186548,1.),(1.,0.707106781186548,1.,0.707106781186548,1.,
0.707106781186548,1.,0.707106781186548,1.),(1.,0.707106781186548,1.,0.707106781186548,
1.,0.707106781186548,1.,0.707106781186548,1.),(1.,0.707106781186547,1.,
0.707106781186547,1.,0.707106781186547,1.,0.707106781186547,1.),(1.,0.707106781186547,
1.,0.707106781186547,1.,0.707106781186547,1.,0.707106781186547,1.),(1.,
0.707106781186547,1.,0.707106781186547,1.,0.707106781186547,1.,0.707106781186547,
1.),(1.,0.707106781186548,1.,0.707106781186548,1.,0.707106781186548,1.,
0.707106781186548,1.),(1.,0.707106781186548,1.,0.707106781186548,1.,0.707106781186548,
1.,0.707106781186548,1.),(1.,0.707106781186547,1.,0.707106781186547,1.,
0.707106781186547,1.,0.707106781186547,1.),(1.,0.707106781186547,1.,0.707106781186547,
1.,0.707106781186547,1.,0.707106781186547,1.),(1.,0.707106781186548,1.,
0.707106781186548,1.,0.707106781186548,1.,0.707106781186548,1.),(1.,0.707106781186547,
1.,0.707106781186547,1.,0.707106781186547,1.,0.707106781186547,1.),(1.,
0.707106781186547,1.,0.707106781186547,1.,0.707106781186547,1.,0.707106781186547,
1.),(1.,0.707106781186547,1.,0.707106781186547,1.,0.707106781186547,1.,
0.707106781186547,1.),(1.,0.707106781186547,1.,0.707106781186547,1.,0.707106781186547,
1.,0.707106781186547,1.),(1.,0.707106781186548,1.,0.707106781186548,1.,
0.707106781186548,1.,0.707106781186548,1.),(1.,0.707106781186547,1.,0.707106781186547,
1.,0.707106781186547,1.,0.707106781186547,1.),(1.,0.707106781186548,1.,
0.707106781186548,1.,0.707106781186548,1.,0.707106781186548,1.),(1.,0.707106781186547,
1.,0.707106781186547,1.,0.707106781186547,1.,0.707106781186547,1.),(1.,
0.707106781186547,1.,0.707106781186547,1.,0.707106781186547,1.,0.707106781186547,
1.),(1.,0.707106781186547,1.,0.707106781186547,1.,0.707106781186547,1.,
0.707106781186547,1.),(1.,0.707106781186548,1.,0.707106781186548,1.,0.707106781186548,
1.,0.707106781186548,1.),(1.,0.707106781186548,1.,0.707106781186548,1.,
0.707106781186548,1.,0.707106781186548,1.),(1.,0.707106781186547,1.,0.707106781186547,
1.,0.707106781186547,1.,0.707106781186547,1.),(1.,0.707106781186548,1.,
0.707106781186548,1.,0.707106781186548,1.,0.707106781186548,1.),(1.,0.707106781186548,
1.,0.707106781186548,1.,0.707106781186548,1.,0.707106781186548,1.),(1.,
0.707106781186547,1.,0.707106781186547,1.,0.707106781186547,1.,0.707106781186547,
1.),(1.,0.707106781186548,1.,0.707106781186548,1.,0.707106781186548,1.,
0.707106781186548,1.),(1.,0.707106781186547,1.,0.707106781186547,1.,0.707106781186547,
1.,0.707106781186547,1.),(1.,0.707106781186548,1.,0.707106781186548,1.,
0.707106781186548,1.,0.707106781186548,1.),(1.,0.707106781186547,1.,0.707106781186547,
1.,0.707106781186547,1.,0.707106781186547,1.),(1.,0.707106781186548,1.,
0.707106781186548,1.,0.707106781186548,1.,0.707106781186548,1.),(1.,0.707106781186547,
1.,0.707106781186547,1.,0.707106781186547,1.,0.707106781186547,1.),(1.,
0.707106781186547,1.,0.707106781186547,1.,0.707106781186547,1.,0.707106781186547,
1.),(1.,0.707106781186548,1.,0.707106781186548,1.,0.707106781186548,1.,
0.707106781186548,1.),(1.,0.707106781186547,1.,0.707106781186547,1.,0.707106781186547,
1.,0.707106781186547,1.),(1.,0.707106781186547,1.,0.707106781186547,1.,
0.707106781186547,1.,0.707106781186547,1.),(1.,0.707106781186548,1.,0.707106781186548,
1.,0.707106781186548,1.,0.707106781186548,1.),(1.,0.707106781186547,1.,
0.707106781186547,1.,0.707106781186547,1.,0.707106781186547,1.),(1.,0.707106781186547,
1.,0.707106781186547,1.,0.707106781186547,1.,0.707106781186547,1.),(1.,
0.707106781186548,1.,0.707106781186548,1.,0.707106781186548,1.,0.707106781186548,
1.),(1.,0.707106781186547,1.,0.707106781186547,1.,0.707106781186547,1.,
0.707106781186547,1.),(1.,0.707106781186548,1.,0.707106781186548,1.,0.707106781186548,
1.,0.707106781186548,1.),(1.,0.707106781186547,1.,0.707106781186547,1.,
0.707106781186547,1.,0.707106781186547,1.),(1.,0.707106781186547,1.,0.707106781186547,
1.,0.707106781186547,1.,0.707106781186547,1.),(1.,0.707106781186548,1.,
0.707106781186548,1.,0.707106781186548,1.,0.707106781186548,1.),(1.,0.707106781186548,
1.,0.707106781186548,1.,0.707106781186548,1.,0.707106781186548,1.),(1.,
0.707106781186547,1.,0.707106781186547,1.,0.707106781186547,1.,0.707106781186547,
1.),(1.,0.707106781186548,1.,0.707106781186548,1.,0.707106781186548,1.,
0.707106781186548,1.),(1.,0.707106781186547,1.,0.707106781186547,1.,0.707106781186547,
1.,0.707106781186547,1.),(1.,0.707106781186548,1.,0.707106781186548,1.,
0.707106781186548,1.,0.707106781186548,1.),(1.,0.707106781186547,1.,0.707106781186547,
1.,0.707106781186547,1.,0.707106781186547,1.),(1.,0.707106781186548,1.,
0.707106781186548,1.,0.707106781186548,1.,0.707106781186548,1.),(1.,0.707106781186547,
1.,0.707106781186547,1.,0.707106781186547,1.,0.707106781186547,1.),(1.,
0.707106781186548,1.,0.707106781186548,1.,0.707106781186548,1.,0.707106781186548,
1.),(1.,0.707106781186547,1.,0.707106781186547,1.,0.707106781186547,1.,
0.707106781186547,1.),(1.,0.707106781186548,1.,0.707106781186548,1.,0.707106781186548,
1.,0.707106781186548,1.),(1.,0.707106781186547,1.,0.707106781186547,1.,
0.707106781186547,1.,0.707106781186547,1.),(1.,0.707106781186548,1.,0.707106781186548,
1.,0.707106781186548,1.,0.707106781186548,1.),(1.,0.707106781186547,1.,
0.707106781186547,1.,0.707106781186547,1.,0.707106781186547,1.),(1.,0.707106781186548,
1.,0.707106781186548,1.,0.707106781186548,1.,0.707106781186548,1.),(1.,
0.707106781186547,1.,0.707106781186547,1.,0.707106781186547,1.,0.707106781186547,
1.),(1.,0.707106781186547,1.,0.707106781186547,1.,0.707106781186547,1.,
0.707106781186547,1.),(1.,0.707106781186548,1.,0.707106781186548,1.,0.707106781186548,
1.,0.707106781186548,1.),(1.,0.707106781186547,1.,0.707106781186547,1.,
0.707106781186547,1.,0.707106781186547,1.),(1.,0.707106781186548,1.,0.707106781186548,
1.,0.707106781186548,1.,0.707106781186548,1.),(1.,0.707106781186547,1.,
0.707106781186547,1.,0.707106781186547,1.,0.707106781186547,1.),(1.,0.707106781186548,
1.,0.707106781186548,1.,0.707106781186548,1.,0.707106781186548,1.),(1.,
0.707106781186547,1.,0.707106781186547,1.,0.707106781186547,1.,0.707106781186547,
1.),(1.,0.707106781186548,1.,0.707106781186548,1.,0.707106781186548,1.,
0.707106781186548,1.),(1.,0.707106781186547,1.,0.707106781186547,1.,0.707106781186547,
1.,0.707106781186547,1.),(1.,0.707106781186547,1.,0.707106781186547,1.,
0.707106781186547,1.,0.707106781186547,1.),(1.,0.707106781186548,1.,0.707106781186548,
1.,0.707106781186548,1.,0.707106781186548,1.),(1.,0.707106781186547,1.,
0.707106781186547,1.,0.707106781186547,1.,0.707106781186547,1.),(1.,0.707106781186548,
1.,0.707106781186548,1.,0.707106781186548,1.,0.707106781186548,1.),(1.,
0.707106781186548,1.,0.707106781186548,1.,0.707106781186548,1.,0.707106781186548,
1.),(1.,0.707106781186548,1.,0.707106781186548,1.,0.707106781186548,1.,
0.707106781186548,1.),(1.,0.707106781186547,1.,0.707106781186547,1.,0.707106781186547,
1.,0.707106781186547,1.),(1.,0.707106781186547,1.,0.707106781186547,1.,
0.707106781186547,1.,0.707106781186547,1.),(1.,0.707106781186547,1.,0.707106781186547,
1.,0.707106781186547,1.,0.707106781186547,1.),(1.,0.707106781186547,1.,
0.707106781186547,1.,0.707106781186547,1.,0.707106781186547,1.),(1.,0.707106781186548,
1.,0.707106781186548,1.,0.707106781186548,1.,0.707106781186548,1.),(1.,
0.707106781186547,1.,0.707106781186547,1.,0.707106781186547,1.,0.707106781186547,
1.),(1.,0.707106781186548,1.,0.707106781186548,1.,0.707106781186548,1.,
0.707106781186548,1.),(1.,0.707106781186548,1.,0.707106781186548,1.,0.707106781186548,
1.,0.707106781186548,1.),(1.,0.707106781186547,1.,0.707106781186547,1.,
0.707106781186547,1.,0.707106781186547,1.),(1.,0.707106781186547,1.,0.707106781186547,
1.,0.707106781186547,1.,0.707106781186547,1.),(1.,0.707106781186548,1.,
0.707106781186548,1.,0.707106781186548,1.,0.707106781186548,1.),(1.,0.707106781186548,
1.,0.707106781186548,1.,0.707106781186548,1.,0.707106781186548,1.),(1.,
0.707106781186547,1.,0.707106781186547,1.,0.707106781186547,1.,0.707106781186547,
1.),(1.,0.707106781186547,1.,0.707106781186547,1.,0.707106781186547,1.,
0.707106781186547,1.),(1.,0.707106781186548,1.,0.707106781186548,1.,0.707106781186548,
1.,0.707106781186548,1.),(1.,0.707106781186547,1.,0.707106781186547,1.,
0.707106781186547,1.,0.707106781186547,1.),(1.,0.707106781186548,1.,0.707106781186548,
1.,0.707106781186548,1.,0.707106781186548,1.),(1.,0.707106781186547,1.,
0.707106781186547,1.,0.707106781186547,1.,0.707106781186547,1.),(1.,0.707106781186547,
1.,0.707106781186547,1.,0.707106781186547,1.,0.707106781186547,1.),(1.,
0.707106781186547,1.,0.707106781186547,1.,0.707106781186547,1.,0.707106781186547,
1.),(1.,0.707106781186547,1.,0.707106781186547,1.,0.707106781186547,1.,
0.707106781186547,1.),(1.,0.707106781186547,1.,0.707106781186547,1.,0.707106781186547,
1.,0.707106781186547,1.),(1.,0.707106781186547,1.,0.707106781186547,1.,
0.707106781186547,1.,0.707106781186547,1.),(1.,0.707106781186547,1.,0.707106781186547,
1.,0.707106781186547,1.,0.707106781186547,1.),(1.,0.707106781186548,1.,
0.707106781186548,1.,0.707106781186548,1.,0.707106781186548,1.),(1.,0.707106781186547,
1.,0.707106781186547,1.,0.707106781186547,1.,0.707106781186547,1.),(1.,
0.707106781186548,1.,0.707106781186548,1.,0.707106781186548,1.,0.707106781186548,
1.),(1.,0.707106781186547,1.,0.707106781186547,1.,0.707106781186547,1.,
0.707106781186547,1.),(1.,0.707106781186548,1.,0.707106781186548,1.,0.707106781186548,
1.,0.707106781186548,1.),(1.,0.707106781186548,1.,0.707106781186548,1.,
0.707106781186548,1.,0.707106781186548,1.),(1.,0.707106781186547,1.,0.707106781186547,
1.,0.707106781186547,1.,0.707106781186547,1.),(1.,0.707106781186548,1.,
0.707106781186548,1.,0.707106781186548,1.,0.707106781186548,1.),(1.,0.707106781186548,
1.,0.707106781186548,1.,0.707106781186548,1.,0.707106781186548,1.),(1.,
0.707106781186548,1.,0.707106781186548,1.,0.707106781186548,1.,0.707106781186548,
1.),(1.,0.707106781186548,1.,0.707106781186548,1.,0.707106781186548,1.,
0.707106781186548,1.),(1.,0.707106781186547,1.,0.707106781186547,1.,0.707106781186547,
1.,0.707106781186547,1.),(1.,0.707106781186548,1.,0.707106781186548,1.,
0.707106781186548,1.,0.707106781186548,1.),(1.,0.707106781186547,1.,0.707106781186547,
1.,0.707106781186547,1.,0.707106781186547,1.),(1.,0.707106781186548,1.,
0.707106781186548,1.,0.707106781186548,1.,0.707106781186548,1.),(1.,0.707106781186547,
1.,0.707106781186547,1.,0.707106781186547,1.,0.707106781186547,1.),(1.,
0.707106781186547,1.,0.707106781186547,1.,0.707106781186547,1.,0.707106781186547,
1.),(1.,0.707106781186548,1.,0.707106781186548,1.,0.707106781186548,1.,
0.707106781186548,1.),(1.,0.707106781186548,1.,0.707106781186548,1.,0.707106781186548,
1.,0.707106781186548,1.),(1.,0.707106781186547,1.,0.707106781186547,1.,
0.707106781186547,1.,0.707106781186547,1.),(1.,0.707106781186547,1.,0.707106781186547,
1.,0.707106781186547,1.,0.707106781186547,1.),(1.,0.707106781186547,1.,
0.707106781186547,1.,0.707106781186547,1.,0.707106781186547,1.),(1.,0.707106781186547,
1.,0.707106781186547,1.,0.707106781186547,1.,0.707106781186547,1.),(1.,
0.707106781186547,1.,0.707106781186547,1.,0.707106781186547,1.,0.707106781186547,
1.),(1.,0.707106781186548,1.,0.707106781186548,1.,0.707106781186548,1.,
0.707106781186548,1.),(1.,0.707106781186548,1.,0.707106781186548,1.,0.707106781186548,
1.,0.707106781186548,1.),(1.,0.707106781186547,1.,0.707106781186547,1.,
0.707106781186547,1.,0.707106781186547,1.),(1.,0.707106781186547,1.,0.707106781186547,
1.,0.707106781186547,1.,0.707106781186547,1.),(1.,0.707106781186548,1.,
0.707106781186548,1.,0.707106781186548,1.,0.707106781186548,1.),(1.,0.707106781186548,
1.,0.707106781186548,1.,0.707106781186548,1.,0.707106781186548,1.),(1.,
0.707106781186547,1.,0.707106781186547,1.,0.707106781186547,1.,0.707106781186547,
1.),(1.,0.707106781186548,1.,0.707106781186548,1.,0.707106781186548,1.,
0.707106781186548,1.),(1.,0.707106781186547,1.,0.707106781186547,1.,0.707106781186547,
1.,0.707106781186547,1.),(1.,0.707106781186548,1.,0.707106781186548,1.,
0.707106781186548,1.,0.707106781186548,1.),(1.,0.707106781186548,1.,0.707106781186548,
1.,0.707106781186548,1.,0.707106781186548,1.),(1.,0.707106781186547,1.,
0.707106781186547,1.,0.707106781186547,1.,0.707106781186547,1.),(1.,0.707106781186547,
1.,0.707106781186547,1.,0.707106781186547,1.,0.707106781186547,1.),(1.,
0.707106781186548,1.,0.707106781186548,1.,0.707106781186548,1.,0.707106781186548,
1.),(1.,0.707106781186547,1.,0.707106781186547,1.,0.707106781186547,1.,
0.707106781186547,1.),(1.,0.707106781186547,1.,0.707106781186547,1.,0.707106781186547,
1.,0.707106781186547,1.),(1.,0.707106781186548,1.,0.707106781186548,1.,
0.707106781186548,1.,0.707106781186548,1.),(1.,0.707106781186547,1.,0.707106781186547,
1.,0.707106781186547,1.,0.707106781186547,1.),(1.,0.707106781186548,1.,
0.707106781186548,1.,0.707106781186548,1.,0.707106781186548,1.),(1.,0.707106781186547,
1.,0.707106781186547,1.,0.707106781186547,1.,0.707106781186547,1.),(1.,
0.707106781186548,1.,0.707106781186548,1.,0.707106781186548,1.,0.707106781186548,
1.),(1.,0.707106781186547,1.,0.707106781186547,1.,0.707106781186547,1.,
0.707106781186547,1.),(1.,0.707106781186547,1.,0.707106781186547,1.,0.707106781186547,
1.,0.707106781186547,1.),(1.,0.707106781186548,1.,0.707106781186548,1.,
0.707106781186548,1.,0.707106781186548,1.),(1.,0.707106781186548,1.,0.707106781186548,
1.,0.707106781186548,1.,0.707106781186548,1.),(1.,0.707106781186547,1.,
0.707106781186547,1.,0.707106781186547,1.,0.707106781186547,1.),(1.,0.707106781186547,
1.,0.707106781186547,1.,0.707106781186547,1.,0.707106781186547,1.),(1.,
0.707106781186548,1.,0.707106781186548,1.,0.707106781186548,1.,0.707106781186548,
1.),(1.,0.707106781186547,1.,0.707106781186547,1.,0.707106781186547,1.,
0.707106781186547,1.),(1.,0.707106781186547,1.,0.707106781186547,1.,0.707106781186547,
1.,0.707106781186547,1.),(1.,0.707106781186548,1.,0.707106781186548,1.,
0.707106781186548,1.,0.707106781186548,1.),(1.,0.707106781186547,1.,0.707106781186547,
1.,0.707106781186547,1.,0.707106781186547,1.),(1.,0.707106781186548,1.,
0.707106781186548,1.,0.707106781186548,1.,0.707106781186548,1.),(1.,0.707106781186547,
1.,0.707106781186547,1.,0.707106781186547,1.,0.707106781186547,1.),(1.,
0.707106781186548,1.,0.707106781186548,1.,0.707106781186548,1.,0.707106781186548,
1.),(1.,0.707106781186547,1.,0.707106781186547,1.,0.707106781186547,1.,
0.707106781186547,1.),(1.,0.707106781186548,1.,0.707106781186548,1.,0.707106781186548,
1.,0.707106781186548,1.),(1.,0.707106781186547,1.,0.707106781186547,1.,
0.707106781186547,1.,0.707106781186547,1.),(1.,0.707106781186547,1.,0.707106781186547,
1.,0.707106781186547,1.,0.707106781186547,1.),(1.,0.707106781186547,1.,
0.707106781186547,1.,0.707106781186547,1.,0.707106781186547,1.),(1.,0.707106781186547,
1.,0.707106781186547,1.,0.707106781186547,1.,0.707106781186547,1.),(1.,
0.707106781186547,1.,0.707106781186547,1.,0.707106781186547,1.,0.707106781186547,
1.),(1.,0.707106781186547,1.,0.707106781186547,1.,0.707106781186547,1.,
0.707106781186547,1.),(1.,0.707106781186548,1.,0.707106781186548,1.,0.707106781186548,
1.,0.707106781186548,1.),(1.,0.707106781186547,1.,0.707106781186547,1.,
0.707106781186547,1.,0.707106781186547,1.),(1.,0.707106781186548,1.,0.707106781186548,
1.,0.707106781186548,1.,0.707106781186548,1.),(1.,0.707106781186547,1.,
0.707106781186547,1.,0.707106781186547,1.,0.707106781186547,1.),(1.,0.707106781186548,
1.,0.707106781186548,1.,0.707106781186548,1.,0.707106781186548,1.),(1.,
0.707106781186548,1.,0.707106781186548,1.,0.707106781186548,1.,0.707106781186548,
1.),(1.,0.707106781186547,1.,0.707106781186547,1.,0.707106781186547,1.,
0.707106781186547,1.),(1.,0.707106781186548,1.,0.707106781186548,1.,0.707106781186548,
1.,0.707106781186548,1.),(1.,0.707106781186548,1.,0.707106781186548,1.,
0.707106781186548,1.,0.707106781186548,1.),(1.,0.707106781186547,1.,0.707106781186547,
1.,0.707106781186547,1.,0.707106781186547,1.),(1.,0.707106781186548,1.,
0.707106781186548,1.,0.707106781186548,1.,0.707106781186548,1.),(1.,0.707106781186547,
1.,0.707106781186547,1.,0.707106781186547,1.,0.707106781186547,1.),(1.,
0.707106781186547,1.,0.707106781186547,1.,0.707106781186547,1.,0.707106781186547,
1.),(1.,0.707106781186547,1.,0.707106781186547,1.,0.707106781186547,1.,
0.707106781186547,1.),(1.,0.707106781186548,1.,0.707106781186548,1.,0.707106781186548,
1.,0.707106781186548,1.),(1.,0.707106781186547,1.,0.707106781186547,1.,
0.707106781186547,1.,0.707106781186547,1.),(1.,0.707106781186547,1.,0.707106781186547,
1.,0.707106781186547,1.,0.707106781186547,1.),(1.,0.707106781186548,1.,
0.707106781186548,1.,0.707106781186548,1.,0.707106781186548,1.),(1.,0.707106781186547,
1.,0.707106781186547,1.,0.707106781186547,1.,0.707106781186547,1.),(1.,
0.707106781186548,1.,0.707106781186548,1.,0.707106781186548,1.,0.707106781186548,
1.),(1.,0.707106781186547,1.,0.707106781186547,1.,0.707106781186547,1.,
0.707106781186547,1.),(1.,0.707106781186547,1.,0.707106781186547,1.,0.707106781186547,
1.,0.707106781186547,1.),(1.,0.707106781186547,1.,0.707106781186547,1.,
0.707106781186547,1.,0.707106781186547,1.),(1.,0.707106781186548,1.,0.707106781186548,
1.,0.707106781186548,1.,0.707106781186548,1.),(1.,0.707106781186548,1.,
0.707106781186548,1.,0.707106781186548,1.,0.707106781186548,1.),(1.,0.707106781186547,
1.,0.707106781186547,1.,0.707106781186547,1.,0.707106781186547,1.),(1.,
0.707106781186548,1.,0.707106781186548,1.,0.707106781186548,1.,0.707106781186548,
1.),(1.,0.707106781186548,1.,0.707106781186548,1.,0.707106781186548,1.,
0.707106781186548,1.),(1.,0.707106781186547,1.,0.707106781186547,1.,0.707106781186547,
1.,0.707106781186547,1.),(1.,0.707106781186548,1.,0.707106781186548,1.,
0.707106781186548,1.,0.707106781186548,1.),(1.,0.707106781186547,1.,0.707106781186547,
1.,0.707106781186547,1.,0.707106781186547,1.),(1.,0.707106781186548,1.,
0.707106781186548,1.,0.707106781186548,1.,0.707106781186548,1.),(1.,0.707106781186548,
1.,0.707106781186548,1.,0.707106781186548,1.,0.707106781186548,1.),(1.,
0.707106781186547,1.,0.707106781186547,1.,0.707106781186547,1.,0.707106781186547,
1.),(1.,0.707106781186548,1.,0.707106781186548,1.,0.707106781186548,1.,
0.707106781186548,1.),(1.,0.707106781186548,1.,0.707106781186548,1.,0.707106781186548,
1.,0.707106781186548,1.),(1.,0.707106781186548,1.,0.707106781186548,1.,
0.707106781186548,1.,0.707106781186548,1.),(1.,0.707106781186547,1.,0.707106781186547,
1.,0.707106781186547,1.,0.707106781186547,1.),(1.,0.707106781186547,1.,
0.707106781186547,1.,0.707106781186547,1.,0.707106781186547,1.),(1.,0.707106781186548,
1.,0.707106781186548,1.,0.707106781186548,1.,0.707106781186548,1.),(1.,
0.707106781186547,1.,0.707106781186547,1.,0.707106781186547,1.,0.707106781186547,
1.),(1.,0.707106781186548,1.,0.707106781186548,1.,0.707106781186548,1.,
0.707106781186548,1.),(1.,0.707106781186547,1.,0.707106781186547,1.,0.707106781186547,
1.,0.707106781186547,1.),(1.,0.707106781186547,1.,0.707106781186547,1.,
0.707106781186547,1.,0.707106781186547,1.),(1.,0.707106781186548,1.,0.707106781186548,
1.,0.707106781186548,1.,0.707106781186548,1.),(1.,0.707106781186548,1.,
0.707106781186548,1.,0.707106781186548,1.,0.707106781186548,1.),(1.,0.707106781186548,
1.,0.707106781186548,1.,0.707106781186548,1.,0.707106781186548,1.),(1.,
0.707106781186547,1.,0.707106781186547,1.,0.707106781186547,1.,0.707106781186547,
1.),(1.,0.707106781186547,1.,0.707106781186547,1.,0.707106781186547,1.,
0.707106781186547,1.),(1.,0.707106781186548,1.,0.707106781186548,1.,0.707106781186548,
1.,0.707106781186548,1.),(1.,0.707106781186548,1.,0.707106781186548,1.,
0.707106781186548,1.,0.707106781186548,1.),(1.,0.707106781186547,1.,0.707106781186547,
1.,0.707106781186547,1.,0.707106781186547,1.),(1.,0.707106781186547,1.,
0.707106781186547,1.,0.707106781186547,1.,0.707106781186547,1.),(1.,0.707106781186548,
1.,0.707106781186548,1.,0.707106781186548,1.,0.707106781186548,1.),(1.,
0.707106781186547,1.,0.707106781186547,1.,0.707106781186547,1.,0.707106781186547,
1.),(1.,0.707106781186547,1.,0.707106781186547,1.,0.707106781186547,1.,
0.707106781186547,1.),(1.,0.707106781186548,1.,0.707106781186548,1.,0.707106781186548,
1.,0.707106781186548,1.),(1.,0.707106781186548,1.,0.707106781186548,1.,
0.707106781186548,1.,0.707106781186548,1.),(1.,0.707106781186547,1.,0.707106781186547,
1.,0.707106781186547,1.,0.707106781186547,1.),(1.,0.707106781186547,1.,
0.707106781186547,1.,0.707106781186547,1.,0.707106781186547,1.),(1.,0.707106781186547,
1.,0.707106781186547,1.,0.707106781186547,1.,0.707106781186547,1.),(1.,
0.707106781186548,1.,0.707106781186548,1.,0.707106781186548,1.,0.707106781186548,
1.),(1.,0.707106781186547,1.,0.707106781186547,1.,0.707106781186547,1.,
0.707106781186547,1.),(1.,0.707106781186547,1.,0.707106781186547,1.,0.707106781186547,
1.,0.707106781186547,1.),(1.,0.707106781186547,1.,0.707106781186547,1.,
0.707106781186547,1.,0.707106781186547,1.),(1.,0.707106781186548,1.,0.707106781186548,
1.,0.707106781186548,1.,0.707106781186548,1.),(1.,0.707106781186548,1.,
0.707106781186548,1.,0.707106781186548,1.,0.707106781186548,1.),(1.,0.707106781186547,
1.,0.707106781186547,1.,0.707106781186547,1.,0.707106781186547,1.),(1.,
0.707106781186548,1.,0.707106781186548,1.,0.707106781186548,1.,0.707106781186548,
1.),(1.,0.707106781186547,1.,0.707106781186547,1.,0.707106781186547,1.,
0.707106781186547,1.),(1.,0.707106781186548,1.,0.707106781186548,1.,0.707106781186548,
1.,0.707106781186548,1.),(1.,0.707106781186547,1.,0.707106781186547,1.,
0.707106781186547,1.,0.707106781186547,1.),(1.,0.707106781186548,1.,0.707106781186548,
1.,0.707106781186548,1.,0.707106781186548,1.),(1.,0.707106781186548,1.,
0.707106781186548,1.,0.707106781186548,1.,0.707106781186548,1.),(1.,0.707106781186547,
1.,0.707106781186547,1.,0.707106781186547,1.,0.707106781186547,1.),(1.,
0.707106781186547,1.,0.707106781186547,1.,0.707106781186547,1.,0.707106781186547,
1.),(1.,0.707106781186548,1.,0.707106781186548,1.,0.707106781186548,1.,
0.707106781186548,1.),(1.,0.707106781186547,1.,0.707106781186547,1.,0.707106781186547,
1.,0.707106781186547,1.),(1.,0.707106781186547,1.,0.707106781186547,1.,
0.707106781186547,1.,0.707106781186547,1.),(1.,0.707106781186548,1.,0.707106781186548,
1.,0.707106781186548,1.,0.707106781186548,1.),(1.,0.707106781186547,1.,
0.707106781186547,1.,0.707106781186547,1.,0.707106781186547,1.),(1.,0.707106781186548,
1.,0.707106781186548,1.,0.707106781186548,1.,0.707106781186548,1.),(1.,
0.707106781186548,1.,0.707106781186548,1.,0.707106781186548,1.,0.707106781186548,
1.),(1.,0.707106781186547,1.,0.707106781186547,1.,0.707106781186547,1.,
0.707106781186547,1.),(1.,0.707106781186548,1.,0.707106781186548,1.,0.707106781186548,
1.,0.707106781186548,1.),(1.,0.707106781186547,1.,0.707106781186547,1.,
0.707106781186547,1.,0.707106781186547,1.),(1.,0.707106781186547,1.,0.707106781186547,
1.,0.707106781186547,1.,0.707106781186547,1.),(1.,0.707106781186547,1.,
0.707106781186547,1.,0.707106781186547,1.,0.707106781186547,1.),(1.,0.707106781186548,
1.,0.707106781186548,1.,0.707106781186548,1.,0.707106781186548,1.),(1.,
0.707106781186548,1.,0.707106781186548,1.,0.707106781186548,1.,0.707106781186548,
1.),(1.,0.707106781186548,1.,0.707106781186548,1.,0.707106781186548,1.,
0.707106781186548,1.),(1.,0.707106781186547,1.,0.707106781186547,1.,0.707106781186547,
1.,0.707106781186547,1.),(1.,0.707106781186548,1.,0.707106781186548,1.,
0.707106781186548,1.,0.707106781186548,1.),(1.,0.707106781186547,1.,0.707106781186547,
1.,0.707106781186547,1.,0.707106781186547,1.),(1.,0.707106781186548,1.,
0.707106781186548,1.,0.707106781186548,1.,0.707106781186548,1.),(1.,0.707106781186547,
1.,0.707106781186547,1.,0.707106781186547,1.,0.707106781186547,1.),(1.,
0.707106781186547,1.,0.707106781186547,1.,0.707106781186547,1.,0.707106781186547,
1.),(1.,0.707106781186547,1.,0.707106781186547,1.,0.707106781186547,1.,
0.707106781186547,1.),(1.,0.707106781186547,1.,0.707106781186547,1.,0.707106781186547,
1.,0.707106781186547,1.),(1.,0.707106781186548,1.,0.707106781186548,1.,
0.707106781186548,1.,0.707106781186548,1.),(1.,0.707106781186548,1.,0.707106781186548,
1.,0.707106781186548,1.,0.707106781186548,1.),(1.,0.707106781186547,1.,
0.707106781186547,1.,0.707106781186547,1.,0.707106781186547,1.),(1.,0.707106781186547,
1.,0.707106781186547,1.,0.707106781186547,1.,0.707106781186547,1.),(1.,
0.707106781186548,1.,0.707106781186548,1.,0.707106781186548,1.,0.707106781186548,
1.),(1.,0.707106781186547,1.,0.707106781186547,1.,0.707106781186547,1.,
0.707106781186547,1.),(1.,0.707106781186548,1.,0.707106781186548,1.,0.707106781186548,
1.,0.707106781186548,1.),(1.,0.707106781186547,1.,0.707106781186547,1.,
0.707106781186547,1.,0.707106781186547,1.),(1.,0.707106781186548,1.,0.707106781186548,
1.,0.707106781186548,1.,0.707106781186548,1.),(1.,0.707106781186547,1.,
0.707106781186547,1.,0.707106781186547,1.,0.707106781186547,1.),(1.,0.707106781186547,
1.,0.707106781186547,1.,0.707106781186547,1.,0.707106781186547,1.),(1.,
0.707106781186548,1.,0.707106781186548,1.,0.707106781186548,1.,0.707106781186548,
1.),(1.,0.707106781186547,1.,0.707106781186547,1.,0.707106781186547,1.,
0.707106781186547,1.),(1.,0.707106781186548,1.,0.707106781186548,1.,0.707106781186548,
1.,0.707106781186548,1.),(1.,0.707106781186547,1.,0.707106781186547,1.,
0.707106781186547,1.,0.707106781186547,1.),(1.,0.707106781186548,1.,0.707106781186548,
1.,0.707106781186548,1.,0.707106781186548,1.),(1.,0.707106781186548,1.,
0.707106781186548,1.,0.707106781186548,1.,0.707106781186548,1.),(1.,0.707106781186547,
1.,0.707106781186547,1.,0.707106781186547,1.,0.707106781186547,1.),(1.,
0.707106781186548,1.,0.707106781186548,1.,0.707106781186548,1.,0.707106781186548,
1.),(1.,0.707106781186547,1.,0.707106781186547,1.,0.707106781186547,1.,
0.707106781186547,1.),(1.,0.707106781186548,1.,0.707106781186548,1.,0.707106781186548,
1.,0.707106781186548,1.),(1.,0.707106781186548,1.,0.707106781186548,1.,
0.707106781186548,1.,0.707106781186548,1.),(1.,0.707106781186547,1.,0.707106781186547,
1.,0.707106781186547,1.,0.707106781186547,1.),(1.,0.707106781186548,1.,
0.707106781186548,1.,0.707106781186548,1.,0.707106781186548,1.),(1.,0.707106781186547,
1.,0.707106781186547,1.,0.707106781186547,1.,0.707106781186547,1.),(1.,
0.707106781186547,1.,0.707106781186547,1.,0.707106781186547,1.,0.707106781186547,
1.),(1.,0.707106781186548,1.,0.707106781186548,1.,0.707106781186548,1.,
0.707106781186548,1.),(1.,0.707106781186547,1.,0.707106781186547,1.,0.707106781186547,
1.,0.707106781186547,1.),(1.,0.707106781186548,1.,0.707106781186548,1.,
0.707106781186548,1.,0.707106781186548,1.),(1.,0.707106781186547,1.,0.707106781186547,
1.,0.707106781186547,1.,0.707106781186547,1.),(1.,0.707106781186548,1.,
0.707106781186548,1.,0.707106781186548,1.,0.707106781186548,1.),(1.,0.707106781186547,
1.,0.707106781186547,1.,0.707106781186547,1.,0.707106781186547,1.),(1.,
0.707106781186547,1.,0.707106781186547,1.,0.707106781186547,1.,0.707106781186547,
1.),(1.,0.707106781186548,1.,0.707106781186548,1.,0.707106781186548,1.,
0.707106781186548,1.),(1.,0.707106781186548,1.,0.707106781186548,1.,0.707106781186548,
1.,0.707106781186548,1.),(1.,0.707106781186548,1.,0.707106781186548,1.,
0.707106781186548,1.,0.707106781186548,1.),(1.,0.707106781186548,1.,0.707106781186548,
1.,0.707106781186548,1.,0.707106781186548,1.),(1.,0.707106781186547,1.,
0.707106781186547,1.,0.707106781186547,1.,0.707106781186547,1.),(1.,0.707106781186548,
1.,0.707106781186548,1.,0.707106781186548,1.,0.707106781186548,1.),(1.,
0.707106781186548,1.,0.707106781186548,1.,0.707106781186548,1.,0.707106781186548,
1.),(1.,0.707106781186548,1.,0.707106781186548,1.,0.707106781186548,1.,
0.707106781186548,1.),(1.,0.707106781186547,1.,0.707106781186547,1.,0.707106781186547,
1.,0.707106781186547,1.),(1.,0.707106781186548,1.,0.707106781186548,1.,
0.707106781186548,1.,0.707106781186548,1.),(1.,0.707106781186548,1.,0.707106781186548,
1.,0.707106781186548,1.,0.707106781186548,1.),(1.,0.707106781186548,1.,
0.707106781186548,1.,0.707106781186548,1.,0.707106781186548,1.),(1.,0.707106781186547,
1.,0.707106781186547,1.,0.707106781186547,1.,0.707106781186547,1.),(1.,
0.707106781186547,1.,0.707106781186547,1.,0.707106781186547,1.,0.707106781186547,
1.),(1.,0.707106781186548,1.,0.707106781186548,1.,0.707106781186548,1.,
0.707106781186548,1.),(1.,0.707106781186547,1.,0.707106781186547,1.,0.707106781186547,
1.,0.707106781186547,1.),(1.,0.707106781186548,1.,0.707106781186548,1.,
0.707106781186548,1.,0.707106781186548,1.),(1.,0.707106781186547,1.,0.707106781186547,
1.,0.707106781186547,1.,0.707106781186547,1.),(1.,0.707106781186548,1.,
0.707106781186548,1.,0.707106781186548,1.,0.707106781186548,1.),(1.,0.707106781186548,
1.,0.707106781186548,1.,0.707106781186548,1.,0.707106781186548,1.),(1.,
0.707106781186547,1.,0.707106781186547,1.,0.707106781186547,1.,0.707106781186547,
1.),(1.,0.707106781186547,1.,0.707106781186547,1.,0.707106781186547,1.,
0.707106781186547,1.),(1.,0.707106781186548,1.,0.707106781186548,1.,0.707106781186548,
1.,0.707106781186548,1.),(1.,0.707106781186547,1.,0.707106781186547,1.,
0.707106781186547,1.,0.707106781186547,1.),(1.,0.707106781186548,1.,0.707106781186548,
1.,0.707106781186548,1.,0.707106781186548,1.),(1.,0.707106781186547,1.,
0.707106781186547,1.,0.707106781186547,1.,0.707106781186547,1.),(1.,0.707106781186548,
1.,0.707106781186548,1.,0.707106781186548,1.,0.707106781186548,1.),(1.,
0.707106781186548,1.,0.707106781186548,1.,0.707106781186548,1.,0.707106781186548,
1.),(1.,0.707106781186547,1.,0.707106781186547,1.,0.707106781186547,1.,
0.707106781186547,1.),(1.,0.707106781186547,1.,0.707106781186547,1.,0.707106781186547,
1.,0.707106781186547,1.),(1.,0.707106781186547,1.,0.707106781186547,1.,
0.707106781186547,1.,0.707106781186547,1.),(1.,0.707106781186548,1.,0.707106781186548,
1.,0.707106781186548,1.,0.707106781186548,1.),(1.,0.707106781186548,1.,
0.707106781186548,1.,0.707106781186548,1.,0.707106781186548,1.),(1.,0.707106781186547,
1.,0.707106781186547,1.,0.707106781186547,1.,0.707106781186547,1.),(1.,
0.707106781186547,1.,0.707106781186547,1.,0.707106781186547,1.,0.707106781186547,
1.),(1.,0.707106781186548,1.,0.707106781186548,1.,0.707106781186548,1.,
0.707106781186548,1.),(1.,0.707106781186548,1.,0.707106781186548,1.,0.707106781186548,
1.,0.707106781186548,1.),(1.,0.707106781186548,1.,0.707106781186548,1.,
0.707106781186548,1.,0.707106781186548,1.),(1.,0.707106781186548,1.,0.707106781186548,
1.,0.707106781186548,1.,0.707106781186548,1.),(1.,0.707106781186547,1.,
0.707106781186547,1.,0.707106781186547,1.,0.707106781186547,1.),(1.,0.707106781186547,
1.,0.707106781186547,1.,0.707106781186547,1.,0.707106781186547,1.),(1.,
0.707106781186548,1.,0.707106781186548,1.,0.707106781186548,1.,0.707106781186548,
1.),(1.,0.707106781186548,1.,0.707106781186548,1.,0.707106781186548,1.,
0.707106781186548,1.),(1.,0.707106781186547,1.,0.707106781186547,1.,0.707106781186547,
1.,0.707106781186547,1.),(1.,0.707106781186548,1.,0.707106781186548,1.,
0.707106781186548,1.,0.707106781186548,1.),(1.,0.707106781186547,1.,0.707106781186547,
1.,0.707106781186547,1.,0.707106781186547,1.),(1.,0.707106781186548,1.,
0.707106781186548,1.,0.707106781186548,1.,0.707106781186548,1.),(1.,0.707106781186547,
1.,0.707106781186547,1.,0.707106781186547,1.,0.707106781186547,1.),(1.,
0.707106781186548,1.,0.707106781186548,1.,0.707106781186548,1.,0.707106781186548,
1.),(1.,0.707106781186547,1.,0.707106781186547,1.,0.707106781186547,1.,
0.707106781186547,1.),(1.,0.707106781186547,1.,0.707106781186547,1.,0.707106781186547,
1.,0.707106781186547,1.),(1.,0.707106781186548,1.,0.707106781186548,1.,
0.707106781186548,1.,0.707106781186548,1.),(1.,0.707106781186547,1.,0.707106781186547,
1.,0.707106781186547,1.,0.707106781186547,1.),(1.,0.707106781186547,1.,
0.707106781186547,1.,0.707106781186547,1.,0.707106781186547,1.),(1.,0.707106781186548,
1.,0.707106781186548,1.,0.707106781186548,1.,0.707106781186548,1.),(1.,
0.707106781186547,1.,0.707106781186547,1.,0.707106781186547,1.,0.707106781186547,
1.),(1.,0.707106781186548,1.,0.707106781186548,1.,0.707106781186548,1.,
0.707106781186548,1.),(1.,0.707106781186547,1.,0.707106781186547,1.,0.707106781186547,
1.,0.707106781186547,1.),(1.,0.707106781186548,1.,0.707106781186548,1.,
0.707106781186548,1.,0.707106781186548,1.),(1.,0.707106781186547,1.,0.707106781186547,
1.,0.707106781186547,1.,0.707106781186547,1.),(1.,0.707106781186548,1.,
0.707106781186548,1.,0.707106781186548,1.,0.707106781186548,1.),(1.,0.707106781186547,
1.,0.707106781186547,1.,0.707106781186547,1.,0.707106781186547,1.),(1.,
0.707106781186548,1.,0.707106781186548,1.,0.707106781186548,1.,0.707106781186548,
1.),(1.,0.707106781186547,1.,0.707106781186547,1.,0.707106781186547,1.,
0.707106781186547,1.),(1.,0.707106781186548,1.,0.707106781186548,1.,0.707106781186548,
1.,0.707106781186548,1.),(1.,0.707106781186547,1.,0.707106781186547,1.,
0.707106781186547,1.,0.707106781186547,1.),(1.,0.707106781186547,1.,0.707106781186547,
1.,0.707106781186547,1.,0.707106781186547,1.),(1.,0.707106781186548,1.,
0.707106781186548,1.,0.707106781186548,1.,0.707106781186548,1.),(1.,0.707106781186548,
1.,0.707106781186548,1.,0.707106781186548,1.,0.707106781186548,1.),(1.,
0.707106781186547,1.,0.707106781186547,1.,0.707106781186547,1.,0.707106781186547,
1.),(1.,0.707106781186547,1.,0.707106781186547,1.,0.707106781186547,1.,
0.707106781186547,1.),(1.,0.707106781186547,1.,0.707106781186547,1.,0.707106781186547,
1.,0.707106781186547,1.),(1.,0.707106781186548,1.,0.707106781186548,1.,
0.707106781186548,1.,0.707106781186548,1.),(1.,0.707106781186547,1.,0.707106781186547,
1.,0.707106781186547,1.,0.707106781186547,1.),(1.,0.707106781186548,1.,
0.707106781186548,1.,0.707106781186548,1.,0.707106781186548,1.),(1.,0.707106781186547,
1.,0.707106781186547,1.,0.707106781186547,1.,0.707106781186547,1.),(1.,
0.707106781186548,1.,0.707106781186548,1.,0.707106781186548,1.,0.707106781186548,
1.),(1.,0.707106781186547,1.,0.707106781186547,1.,0.707106781186547,1.,
0.707106781186547,1.),(1.,0.707106781186548,1.,0.707106781186548,1.,0.707106781186548,
1.,0.707106781186548,1.),(1.,0.707106781186547,1.,0.707106781186547,1.,
0.707106781186547,1.,0.707106781186547,1.),(1.,0.707106781186547,1.,0.707106781186547,
1.,0.707106781186547,1.,0.707106781186547,1.),(1.,0.707106781186547,1.,
0.707106781186547,1.,0.707106781186547,1.,0.707106781186547,1.),(1.,0.707106781186548,
1.,0.707106781186548,1.,0.707106781186548,1.,0.707106781186548,1.),(1.,
0.707106781186547,1.,0.707106781186547,1.,0.707106781186547,1.,0.707106781186547,
1.),(1.,0.707106781186548,1.,0.707106781186548,1.,0.707106781186548,1.,
0.707106781186548,1.),(1.,0.707106781186548,1.,0.707106781186548,1.,0.707106781186548,
1.,0.707106781186548,1.),(1.,0.707106781186547,1.,0.707106781186547,1.,
0.707106781186547,1.,0.707106781186547,1.),(1.,0.707106781186548,1.,0.707106781186548,
1.,0.707106781186548,1.,0.707106781186548,1.),(1.,0.707106781186547,1.,
0.707106781186547,1.,0.707106781186547,1.,0.707106781186547,1.),(1.,0.707106781186547,
1.,0.707106781186547,1.,0.707106781186547,1.,0.707106781186547,1.),(1.,
0.707106781186548,1.,0.707106781186548,1.,0.707106781186548,1.,0.707106781186548,
1.),(1.,0.707106781186547,1.,0.707106781186547,1.,0.707106781186547,1.,
0.707106781186547,1.),(1.,0.707106781186547,1.,0.707106781186547,1.,0.707106781186547,
1.,0.707106781186547,1.),(1.,0.707106781186548,1.,0.707106781186548,1.,
0.707106781186548,1.,0.707106781186548,1.),(1.,0.707106781186547,1.,0.707106781186547,
1.,0.707106781186547,1.,0.707106781186547,1.),(1.,0.707106781186547,1.,
0.707106781186547,1.,0.707106781186547,1.,0.707106781186547,1.),(1.,0.707106781186547,
1.,0.707106781186547,1.,0.707106781186547,1.,0.707106781186547,1.),(1.,
0.707106781186547,1.,0.707106781186547,1.,0.707106781186547,1.,0.707106781186547,
1.),(1.,0.707106781186548,1.,0.707106781186548,1.,0.707106781186548,1.,
0.707106781186548,1.),(1.,0.707106781186547,1.,0.707106781186547,1.,0.707106781186547,
1.,0.707106781186547,1.),(1.,0.707106781186547,1.,0.707106781186547,1.,
0.707106781186547,1.,0.707106781186547,1.),(1.,0.707106781186547,1.,0.707106781186547,
1.,0.707106781186547,1.,0.707106781186547,1.),(1.,0.707106781186548,1.,
0.707106781186548,1.,0.707106781186548,1.,0.707106781186548,1.),(1.,0.707106781186547,
1.,0.707106781186547,1.,0.707106781186547,1.,0.707106781186547,1.),(1.,
0.707106781186547,1.,0.707106781186547,1.,0.707106781186547,1.,0.707106781186547,
1.),(1.,0.707106781186548,1.,0.707106781186548,1.,0.707106781186548,1.,
0.707106781186548,1.),(1.,0.707106781186548,1.,0.707106781186548,1.,0.707106781186548,
1.,0.707106781186548,1.),(1.,0.707106781186547,1.,0.707106781186547,1.,
0.707106781186547,1.,0.707106781186547,1.),(1.,0.707106781186548,1.,0.707106781186548,
1.,0.707106781186548,1.,0.707106781186548,1.),(1.,0.707106781186548,1.,
0.707106781186548,1.,0.707106781186548,1.,0.707106781186548,1.),(1.,0.707106781186547,
1.,0.707106781186547,1.,0.707106781186547,1.,0.707106781186547,1.),(1.,
0.707106781186547,1.,0.707106781186547,1.,0.707106781186547,1.,0.707106781186547,
1.),(1.,0.707106781186548,1.,0.707106781186548,1.,0.707106781186548,1.,
0.707106781186548,1.),(1.,0.707106781186547,1.,0.707106781186547,1.,0.707106781186547,
1.,0.707106781186547,1.),(1.,0.707106781186547,1.,0.707106781186547,1.,
0.707106781186547,1.,0.707106781186547,1.),(1.,0.707106781186548,1.,0.707106781186548,
1.,0.707106781186548,1.,0.707106781186548,1.),(1.,0.707106781186547,1.,
0.707106781186547,1.,0.707106781186547,1.,0.707106781186547,1.),(1.,0.707106781186547,
1.,0.707106781186547,1.,0.707106781186547,1.,0.707106781186547,1.),(1.,
0.707106781186547,1.,0.707106781186547,1.,0.707106781186547,1.,0.707106781186547,
1.),(1.,0.707106781186548,1.,0.707106781186548,1.,0.707106781186548,1.,
0.707106781186548,1.),(1.,0.707106781186547,1.,0.707106781186547,1.,0.707106781186547,
1.,0.707106781186547,1.),(1.,0.707106781186548,1.,0.707106781186548,1.,
0.707106781186548,1.,0.707106781186548,1.),(1.,0.707106781186547,1.,0.707106781186547,
1.,0.707106781186547,1.,0.707106781186547,1.),(1.,0.707106781186548,1.,
0.707106781186548,1.,0.707106781186548,1.,0.707106781186548,1.),(1.,0.707106781186547,
1.,0.707106781186547,1.,0.707106781186547,1.,0.707106781186547,1.),(1.,
0.707106781186548,1.,0.707106781186548,1.,0.707106781186548,1.,0.707106781186548,
1.),(1.,0.707106781186547,1.,0.707106781186547,1.,0.707106781186547,1.,
0.707106781186547,1.),(1.,0.707106781186548,1.,0.707106781186548,1.,0.707106781186548,
1.,0.707106781186548,1.),(1.,0.707106781186547,1.,0.707106781186547,1.,
0.707106781186547,1.,0.707106781186547,1.),(1.,0.707106781186548,1.,0.707106781186548,
1.,0.707106781186548,1.,0.707106781186548,1.),(1.,0.707106781186548,1.,
0.707106781186548,1.,0.707106781186548,1.,0.707106781186548,1.),(1.,0.707106781186547,
1.,0.707106781186547,1.,0.707106781186547,1.,0.707106781186547,1.),(1.,
0.707106781186547,1.,0.707106781186547,1.,0.707106781186547,1.,0.707106781186547,
1.),(1.,0.707106781186548,1.,0.707106781186548,1.,0.707106781186548,1.,
0.707106781186548,1.),(1.,0.707106781186547,1.,0.707106781186547,1.,0.707106781186547,
1.,0.707106781186547,1.),(1.,0.707106781186548,1.,0.707106781186548,1.,
0.707106781186548,1.,0.707106781186548,1.),(1.,0.707106781186547,1.,0.707106781186547,
1.,0.707106781186547,1.,0.707106781186547,1.),(1.,0.707106781186548,1.,
0.707106781186548,1.,0.707106781186548,1.,0.707106781186548,1.),(1.,0.707106781186548,
1.,0.707106781186548,1.,0.707106781186548,1.,0.707106781186548,1.),(1.,
0.707106781186547,1.,0.707106781186547,1.,0.707106781186547,1.,0.707106781186547,
1.),(1.,0.707106781186548,1.,0.707106781186548,1.,0.707106781186548,1.,
0.707106781186548,1.),(1.,0.707106781186547,1.,0.707106781186547,1.,0.707106781186547,
1.,0.707106781186547,1.),(1.,0.707106781186548,1.,0.707106781186548,1.,
0.707106781186548,1.,0.707106781186548,1.),(1.,0.707106781186548,1.,0.707106781186548,
1.,0.707106781186548,1.,0.707106781186548,1.),(1.,0.707106781186547,1.,
0.707106781186547,1.,0.707106781186547,1.,0.707106781186547,1.),(1.,0.707106781186547,
1.,0.707106781186547,1.,0.707106781186547,1.,0.707106781186547,1.),(1.,
0.707106781186548,1.,0.707106781186548,1.,0.707106781186548,1.,0.707106781186548,
1.),(1.,0.707106781186547,1.,0.707106781186547,1.,0.707106781186547,1.,
0.707106781186547,1.),(1.,0.707106781186548,1.,0.707106781186548,1.,0.707106781186548,
1.,0.707106781186548,1.),(1.,0.707106781186547,1.,0.707106781186547,1.,
0.707106781186547,1.,0.707106781186547,1.),(1.,0.707106781186548,1.,0.707106781186548,
1.,0.707106781186548,1.,0.707106781186548,1.),(1.,0.707106781186547,1.,
0.707106781186547,1.,0.707106781186547,1.,0.707106781186547,1.),(1.,0.707106781186548,
1.,0.707106781186548,1.,0.707106781186548,1.,0.707106781186548,1.),(1.,
0.707106781186547,1.,0.707106781186547,1.,0.707106781186547,1.,0.707106781186547,
1.),(1.,0.707106781186547,1.,0.707106781186547,1.,0.707106781186547,1.,
0.707106781186547,1.),(1.,0.707106781186547,1.,0.707106781186547,1.,0.707106781186547,
1.,0.707106781186547,1.),(1.,0.707106781186547,1.,0.707106781186547,1.,
0.707106781186547,1.,0.707106781186547,1.),(1.,0.707106781186547,1.,0.707106781186547,
1.,0.707106781186547,1.,0.707106781186547,1.),(1.,0.707106781186547,1.,
0.707106781186547,1.,0.707106781186547,1.,0.707106781186547,1.),(1.,0.707106781186547,
1.,0.707106781186547,1.,0.707106781186547,1.,0.707106781186547,1.),(1.,
0.707106781186547,1.,0.707106781186547,1.,0.707106781186547,1.,0.707106781186547,
1.),(1.,0.707106781186548,1.,0.707106781186548,1.,0.707106781186548,1.,
0.707106781186548,1.),(1.,0.707106781186547,1.,0.707106781186547,1.,0.707106781186547,
1.,0.707106781186547,1.),(1.,0.707106781186548,1.,0.707106781186548,1.,
0.707106781186548,1.,0.707106781186548,1.),(1.,0.707106781186547,1.,0.707106781186547,
1.,0.707106781186547,1.,0.707106781186547,1.),(1.,0.707106781186547,1.,
0.707106781186547,1.,0.707106781186547,1.,0.707106781186547,1.),(1.,0.707106781186548,
1.,0.707106781186548,1.,0.707106781186548,1.,0.707106781186548,1.),(1.,
0.707106781186547,1.,0.707106781186547,1.,0.707106781186547,1.,0.707106781186547,
1.),(1.,0.707106781186548,1.,0.707106781186548,1.,0.707106781186548,1.,
0.707106781186548,1.),(1.,0.707106781186547,1.,0.707106781186547,1.,0.707106781186547,
1.,0.707106781186547,1.),(1.,0.707106781186547,1.,0.707106781186547,1.,
0.707106781186547,1.,0.707106781186547,1.),(1.,0.707106781186548,1.,0.707106781186548,
1.,0.707106781186548,1.,0.707106781186548,1.),(1.,0.707106781186547,1.,
0.707106781186547,1.,0.707106781186547,1.,0.707106781186547,1.),(1.,0.707106781186548,
1.,0.707106781186548,1.,0.707106781186548,1.,0.707106781186548,1.),(1.,
0.707106781186547,1.,0.707106781186547,1.,0.707106781186547,1.,0.707106781186547,
1.),(1.,0.707106781186548,1.,0.707106781186548,1.,0.707106781186548,1.,
0.707106781186548,1.),(1.,0.707106781186547,1.,0.707106781186547,1.,0.707106781186547,
1.,0.707106781186547,1.),(1.,0.707106781186548,1.,0.707106781186548,1.,
0.707106781186548,1.,0.707106781186548,1.),(1.,0.707106781186547,1.,0.707106781186547,
1.,0.707106781186547,1.,0.707106781186547,1.),(1.,0.707106781186548,1.,
0.707106781186548,1.,0.707106781186548,1.,0.707106781186548,1.),(1.,0.707106781186547,
1.,0.707106781186547,1.,0.707106781186547,1.,0.707106781186547,1.),(1.,
0.707106781186548,1.,0.707106781186548,1.,0.707106781186548,1.,0.707106781186548,
1.),(1.,0.707106781186547,1.,0.707106781186547,1.,0.707106781186547,1.,
0.707106781186547,1.),(1.,0.707106781186548,1.,0.707106781186548,1.,0.707106781186548,
1.,0.707106781186548,1.),(1.,0.707106781186548,1.,0.707106781186548,1.,
0.707106781186548,1.,0.707106781186548,1.),(1.,0.707106781186547,1.,0.707106781186547,
1.,0.707106781186547,1.,0.707106781186547,1.),(1.,0.707106781186548,1.,
0.707106781186548,1.,0.707106781186548,1.,0.707106781186548,1.),(1.,0.707106781186547,
1.,0.707106781186547,1.,0.707106781186547,1.,0.707106781186547,1.),(1.,
0.707106781186547,1.,0.707106781186547,1.,0.707106781186547,1.,0.707106781186547,
1.),(1.,0.707106781186547,1.,0.707106781186547,1.,0.707106781186547,1.,
0.707106781186547,1.),(1.,0.707106781186548,1.,0.707106781186548,1.,0.707106781186548,
1.,0.707106781186548,1.),(1.,0.707106781186547,1.,0.707106781186547,1.,
0.707106781186547,1.,0.707106781186547,1.),(1.,0.707106781186547,1.,0.707106781186547,
1.,0.707106781186547,1.,0.707106781186547,1.),(1.,0.707106781186547,1.,
0.707106781186547,1.,0.707106781186547,1.,0.707106781186547,1.),(1.,0.707106781186548,
1.,0.707106781186548,1.,0.707106781186548,1.,0.707106781186548,1.),(1.,
0.707106781186547,1.,0.707106781186547,1.,0.707106781186547,1.,0.707106781186547,
1.),(1.,0.707106781186547,1.,0.707106781186547,1.,0.707106781186547,1.,
0.707106781186547,1.),(1.,0.707106781186548,1.,0.707106781186548,1.,0.707106781186548,
1.,0.707106781186548,1.),(1.,0.707106781186547,1.,0.707106781186547,1.,
0.707106781186547,1.,0.707106781186547,1.),(1.,0.707106781186547,1.,0.707106781186547,
1.,0.707106781186547,1.,0.707106781186547,1.),(1.,0.707106781186547,1.,
0.707106781186547,1.,0.707106781186547,1.,0.707106781186547,1.),(1.,0.707106781186547,
1.,0.707106781186547,1.,0.707106781186547,1.,0.707106781186547,1.),(1.,
0.707106781186548,1.,0.707106781186548,1.,0.707106781186548,1.,0.707106781186548,
1.),(1.,0.707106781186547,1.,0.707106781186547,1.,0.707106781186547,1.,
0.707106781186547,1.),(1.,0.707106781186547,1.,0.707106781186547,1.,0.707106781186547,
1.,0.707106781186547,1.),(1.,0.707106781186547,1.,0.707106781186547,1.,
0.707106781186547,1.,0.707106781186547,1.),(1.,0.707106781186548,1.,0.707106781186548,
1.,0.707106781186548,1.,0.707106781186548,1.),(1.,0.707106781186548,1.,
0.707106781186548,1.,0.707106781186548,1.,0.707106781186548,1.),(1.,0.707106781186548,
1.,0.707106781186548,1.,0.707106781186548,1.,0.707106781186548,1.),(1.,
0.707106781186548,1.,0.707106781186548,1.,0.707106781186548,1.,0.707106781186548,
1.),(1.,0.707106781186547,1.,0.707106781186547,1.,0.707106781186547,1.,
0.707106781186547,1.),(1.,0.707106781186548,1.,0.707106781186548,1.,0.707106781186548,
1.,0.707106781186548,1.),(1.,0.707106781186547,1.,0.707106781186547,1.,
0.707106781186547,1.,0.707106781186547,1.),(1.,0.707106781186547,1.,0.707106781186547,
1.,0.707106781186547,1.,0.707106781186547,1.),(1.,0.707106781186548,1.,
0.707106781186548,1.,0.707106781186548,1.,0.707106781186548,1.),(1.,0.707106781186547,
1.,0.707106781186547,1.,0.707106781186547,1.,0.707106781186547,1.),(1.,
0.707106781186548,1.,0.707106781186548,1.,0.707106781186548,1.,0.707106781186548,
1.),(1.,0.707106781186547,1.,0.707106781186547,1.,0.707106781186547,1.,
0.707106781186547,1.),(1.,0.707106781186547,1.,0.707106781186547,1.,0.707106781186547,
1.,0.707106781186547,1.),(1.,0.707106781186548,1.,0.707106781186548,1.,
0.707106781186548,1.,0.707106781186548,1.),(1.,0.707106781186547,1.,0.707106781186547,
1.,0.707106781186547,1.,0.707106781186547,1.),(1.,0.707106781186547,1.,
0.707106781186547,1.,0.707106781186547,1.,0.707106781186547,1.),(1.,0.707106781186547,
1.,0.707106781186547,1.,0.707106781186547,1.,0.707106781186547,1.),(1.,
0.707106781186547,1.,0.707106781186547,1.,0.707106781186547,1.,0.707106781186547,
1.),(1.,0.707106781186548,1.,0.707106781186548,1.,0.707106781186548,1.,
0.707106781186548,1.),(1.,0.707106781186548,1.,0.707106781186548,1.,0.707106781186548,
1.,0.707106781186548,1.),(1.,0.707106781186547,1.,0.707106781186547,1.,
0.707106781186547,1.,0.707106781186547,1.),(1.,0.707106781186547,1.,0.707106781186547,
1.,0.707106781186547,1.,0.707106781186547,1.),(1.,0.707106781186548,1.,
0.707106781186548,1.,0.707106781186548,1.,0.707106781186548,1.),(1.,0.707106781186547,
1.,0.707106781186547,1.,0.707106781186547,1.,0.707106781186547,1.),(1.,
0.707106781186548,1.,0.707106781186548,1.,0.707106781186548,1.,0.707106781186548,
1.),(1.,0.707106781186547,1.,0.707106781186547,1.,0.707106781186547,1.,
0.707106781186547,1.),(1.,0.707106781186548,1.,0.707106781186548,1.,0.707106781186548,
1.,0.707106781186548,1.),(1.,0.707106781186548,1.,0.707106781186548,1.,
0.707106781186548,1.,0.707106781186548,1.),(1.,0.707106781186547,1.,0.707106781186547,
1.,0.707106781186547,1.,0.707106781186547,1.),(1.,0.707106781186547,1.,
0.707106781186547,1.,0.707106781186547,1.,0.707106781186547,1.),(1.,0.707106781186548,
1.,0.707106781186548,1.,0.707106781186548,1.,0.707106781186548,1.),(1.,
0.707106781186548,1.,0.707106781186548,1.,0.707106781186548,1.,0.707106781186548,
1.),(1.,0.707106781186547,1.,0.707106781186547,1.,0.707106781186547,1.,
0.707106781186547,1.),(1.,0.707106781186548,1.,0.707106781186548,1.,0.707106781186548,
1.,0.707106781186548,1.),(1.,0.707106781186548,1.,0.707106781186548,1.,
0.707106781186548,1.,0.707106781186548,1.),(1.,0.707106781186547,1.,0.707106781186547,
1.,0.707106781186547,1.,0.707106781186547,1.),(1.,0.707106781186548,1.,
0.707106781186548,1.,0.707106781186548,1.,0.707106781186548,1.),(1.,0.707106781186548,
1.,0.707106781186548,1.,0.707106781186548,1.,0.707106781186548,1.),(1.,
0.707106781186548,1.,0.707106781186548,1.,0.707106781186548,1.,0.707106781186548,
1.),(1.,0.707106781186547,1.,0.707106781186547,1.,0.707106781186547,1.,
0.707106781186547,1.),(1.,0.707106781186548,1.,0.707106781186548,1.,0.707106781186548,
1.,0.707106781186548,1.),(1.,0.707106781186547,1.,0.707106781186547,1.,
0.707106781186547,1.,0.707106781186547,1.),(1.,0.707106781186548,1.,0.707106781186548,
1.,0.707106781186548,1.,0.707106781186548,1.),(1.,0.707106781186547,1.,
0.707106781186547,1.,0.707106781186547,1.,0.707106781186547,1.),(1.,0.707106781186548,
1.,0.707106781186548,1.,0.707106781186548,1.,0.707106781186548,1.),(1.,
0.707106781186547,1.,0.707106781186547,1.,0.707106781186547,1.,0.707106781186547,
1.),(1.,0.707106781186548,1.,0.707106781186548,1.,0.707106781186548,1.,
0.707106781186548,1.),(1.,0.707106781186547,1.,0.707106781186547,1.,0.707106781186547,
1.,0.707106781186547,1.),(1.,0.707106781186548,1.,0.707106781186548,1.,
0.707106781186548,1.,0.707106781186548,1.),(1.,0.707106781186548,1.,0.707106781186548,
1.,0.707106781186548,1.,0.707106781186548,1.),(1.,0.707106781186547,1.,
0.707106781186547,1.,0.707106781186547,1.,0.707106781186547,1.),(1.,0.707106781186547,
1.,0.707106781186547,1.,0.707106781186547,1.,0.707106781186547,1.),(1.,
0.707106781186548,1.,0.707106781186548,1.,0.707106781186548,1.,0.707106781186548,
1.),(1.,0.707106781186547,1.,0.707106781186547,1.,0.707106781186547,1.,
0.707106781186547,1.),(1.,0.707106781186548,1.,0.707106781186548,1.,0.707106781186548,
1.,0.707106781186548,1.),(1.,0.707106781186547,1.,0.707106781186547,1.,
0.707106781186547,1.,0.707106781186547,1.),(1.,0.707106781186548,1.,0.707106781186548,
1.,0.707106781186548,1.,0.707106781186548,1.),(1.,0.707106781186548,1.,
0.707106781186548,1.,0.707106781186548,1.,0.707106781186548,1.),(1.,0.707106781186548,
1.,0.707106781186548,1.,0.707106781186548,1.,0.707106781186548,1.),(1.,
0.707106781186548,1.,0.707106781186548,1.,0.707106781186548,1.,0.707106781186548,
1.),(1.,0.707106781186548,1.,0.707106781186548,1.,0.707106781186548,1.,
0.707106781186548,1.),(1.,0.707106781186547,1.,0.707106781186547,1.,0.707106781186547,
1.,0.707106781186547,1.),(1.,0.707106781186547,1.,0.707106781186547,1.,
0.707106781186547,1.,0.707106781186547,1.),(1.,0.707106781186547,1.,0.707106781186547,
1.,0.707106781186547,1.,0.707106781186547,1.),(1.,0.707106781186547,1.,
0.707106781186547,1.,0.707106781186547,1.,0.707106781186547,1.),(1.,0.707106781186548,
1.,0.707106781186548,1.,0.707106781186548,1.,0.707106781186548,1.),(1.,
0.707106781186547,1.,0.707106781186547,1.,0.707106781186547,1.,0.707106781186547,
1.),(1.,0.707106781186548,1.,0.707106781186548,1.,0.707106781186548,1.,
0.707106781186548,1.),(1.,0.707106781186547,1.,0.707106781186547,1.,0.707106781186547,
1.,0.707106781186547,1.),(1.,0.707106781186547,1.,0.707106781186547,1.,
0.707106781186547,1.,0.707106781186547,1.),(1.,0.707106781186548,1.,0.707106781186548,
1.,0.707106781186548,1.,0.707106781186548,1.),(1.,0.707106781186548,1.,
0.707106781186548,1.,0.707106781186548,1.,0.707106781186548,1.),(1.,0.707106781186547,
1.,0.707106781186547,1.,0.707106781186547,1.,0.707106781186547,1.),(1.,
0.707106781186548,1.,0.707106781186548,1.,0.707106781186548,1.,0.707106781186548,
1.),(1.,0.707106781186547,1.,0.707106781186547,1.,0.707106781186547,1.,
0.707106781186547,1.),(1.,0.707106781186548,1.,0.707106781186548,1.,0.707106781186548,
1.,0.707106781186548,1.),(1.,0.707106781186548,1.,0.707106781186548,1.,
0.707106781186548,1.,0.707106781186548,1.),(1.,0.707106781186547,1.,0.707106781186547,
1.,0.707106781186547,1.,0.707106781186547,1.),(1.,0.707106781186547,1.,
0.707106781186547,1.,0.707106781186547,1.,0.707106781186547,1.),(1.,0.707106781186548,
1.,0.707106781186548,1.,0.707106781186548,1.,0.707106781186548,1.),(1.,
0.707106781186547,1.,0.707106781186547,1.,0.707106781186547,1.,0.707106781186547,
1.),(1.,0.707106781186548,1.,0.707106781186548,1.,0.707106781186548,1.,
0.707106781186548,1.),(1.,0.707106781186547,1.,0.707106781186547,1.,0.707106781186547,
1.,0.707106781186547,1.),(1.,0.707106781186548,1.,0.707106781186548,1.,
0.707106781186548,1.,0.707106781186548,1.),(1.,0.707106781186547,1.,0.707106781186547,
1.,0.707106781186547,1.,0.707106781186547,1.),(1.,0.707106781186548,1.,
0.707106781186548,1.,0.707106781186548,1.,0.707106781186548,1.),(1.,0.707106781186547,
1.,0.707106781186547,1.,0.707106781186547,1.,0.707106781186547,1.),(1.,
0.707106781186548,1.,0.707106781186548,1.,0.707106781186548,1.,0.707106781186548,
1.),(1.,0.707106781186547,1.,0.707106781186547,1.,0.707106781186547,1.,
0.707106781186547,1.),(1.,0.707106781186548,1.,0.707106781186548,1.,0.707106781186548,
1.,0.707106781186548,1.),(1.,0.707106781186547,1.,0.707106781186547,1.,
0.707106781186547,1.,0.707106781186547,1.),(1.,0.707106781186548,1.,0.707106781186548,
1.,0.707106781186548,1.,0.707106781186548,1.),(1.,0.707106781186548,1.,
0.707106781186548,1.,0.707106781186548,1.,0.707106781186548,1.),(1.,0.707106781186547,
1.,0.707106781186547,1.,0.707106781186547,1.,0.707106781186547,1.),(1.,
0.707106781186548,1.,0.707106781186548,1.,0.707106781186548,1.,0.707106781186548,
1.),(1.,0.707106781186547,1.,0.707106781186547,1.,0.707106781186547,1.,
0.707106781186547,1.),(1.,0.707106781186548,1.,0.707106781186548,1.,0.707106781186548,
1.,0.707106781186548,1.),(1.,0.707106781186547,1.,0.707106781186547,1.,
0.707106781186547,1.,0.707106781186547,1.),(1.,0.707106781186548,1.,0.707106781186548,
1.,0.707106781186548,1.,0.707106781186548,1.),(1.,0.707106781186548,1.,
0.707106781186548,1.,0.707106781186548,1.,0.707106781186548,1.),(1.,0.707106781186548,
1.,0.707106781186548,1.,0.707106781186548,1.,0.707106781186548,1.),(1.,
0.707106781186547,1.,0.707106781186547,1.,0.707106781186547,1.,0.707106781186547,
1.),(1.,0.707106781186547,1.,0.707106781186547,1.,0.707106781186547,1.,
0.707106781186547,1.),(1.,0.707106781186548,1.,0.707106781186548,1.,0.707106781186548,
1.,0.707106781186548,1.),(1.,0.707106781186548,1.,0.707106781186548,1.,
0.707106781186548,1.,0.707106781186548,1.),(1.,0.707106781186547,1.,0.707106781186547,
1.,0.707106781186547,1.,0.707106781186547,1.),(1.,0.707106781186547,1.,
0.707106781186547,1.,0.707106781186547,1.,0.707106781186547,1.),(1.,0.707106781186547,
1.,0.707106781186547,1.,0.707106781186547,1.,0.707106781186547,1.),(1.,
0.707106781186548,1.,0.707106781186548,1.,0.707106781186548,1.,0.707106781186548,
1.),(1.,0.707106781186547,1.,0.707106781186547,1.,0.707106781186547,1.,
0.707106781186547,1.),(1.,0.707106781186548,1.,0.707106781186548,1.,0.707106781186548,
1.,0.707106781186548,1.),(1.,0.707106781186547,1.,0.707106781186547,1.,
0.707106781186547,1.,0.707106781186547,1.),(1.,0.707106781186548,1.,0.707106781186548,
1.,0.707106781186548,1.,0.707106781186548,1.),(1.,0.707106781186547,1.,
0.707106781186547,1.,0.707106781186547,1.,0.707106781186547,1.),(1.,0.707106781186547,
1.,0.707106781186547,1.,0.707106781186547,1.,0.707106781186547,1.),(1.,
0.707106781186547,1.,0.707106781186547,1.,0.707106781186547,1.,0.707106781186547,
1.),(1.,0.707106781186548,1.,0.707106781186548,1.,0.707106781186548,1.,
0.707106781186548,1.),(1.,0.707106781186547,1.,0.707106781186547,1.,0.707106781186547,
1.,0.707106781186547,1.),(1.,0.707106781186548,1.,0.707106781186548,1.,
0.707106781186548,1.,0.707106781186548,1.),(1.,0.707106781186547,1.,0.707106781186547,
1.,0.707106781186547,1.,0.707106781186547,1.),(1.,0.707106781186548,1.,
0.707106781186548,1.,0.707106781186548,1.,0.707106781186548,1.),(1.,0.707106781186547,
1.,0.707106781186547,1.,0.707106781186547,1.,0.707106781186547,1.),(1.,
0.707106781186548,1.,0.707106781186548,1.,0.707106781186548,1.,0.707106781186548,
1.),(1.,0.707106781186547,1.,0.707106781186547,1.,0.707106781186547,1.,
0.707106781186547,1.),(1.,0.707106781186547,1.,0.707106781186547,1.,0.707106781186547,
1.,0.707106781186547,1.),(1.,0.707106781186548,1.,0.707106781186548,1.,
0.707106781186548,1.,0.707106781186548,1.),(1.,0.707106781186547,1.,0.707106781186547,
1.,0.707106781186547,1.,0.707106781186547,1.),(1.,0.707106781186547,1.,
0.707106781186547,1.,0.707106781186547,1.,0.707106781186547,1.),(1.,0.707106781186548,
1.,0.707106781186548,1.,0.707106781186548,1.,0.707106781186548,1.),(1.,
0.707106781186547,1.,0.707106781186547,1.,0.707106781186547,1.,0.707106781186547,
1.),(1.,0.707106781186547,1.,0.707106781186547,1.,0.707106781186547,1.,
0.707106781186547,1.),(1.,0.707106781186548,1.,0.707106781186548,1.,0.707106781186548,
1.,0.707106781186548,1.),(1.,0.707106781186547,1.,0.707106781186547,1.,
0.707106781186547,1.,0.707106781186547,1.),(1.,0.707106781186547,1.,0.707106781186547,
1.,0.707106781186547,1.,0.707106781186547,1.),(1.,0.707106781186547,1.,
0.707106781186547,1.,0.707106781186547,1.,0.707106781186547,1.),(1.,0.707106781186548,
1.,0.707106781186548,1.,0.707106781186548,1.,0.707106781186548,1.),(1.,
0.707106781186547,1.,0.707106781186547,1.,0.707106781186547,1.,0.707106781186547,
1.),(1.,0.707106781186548,1.,0.707106781186548,1.,0.707106781186548,1.,
0.707106781186548,1.),(1.,0.707106781186547,1.,0.707106781186547,1.,0.707106781186547,
1.,0.707106781186547,1.),(1.,0.707106781186547,1.,0.707106781186547,1.,
0.707106781186547,1.,0.707106781186547,1.),(1.,0.707106781186547,1.,0.707106781186547,
1.,0.707106781186547,1.,0.707106781186547,1.),(1.,0.707106781186548,1.,
0.707106781186548,1.,0.707106781186548,1.,0.707106781186548,1.),(1.,0.707106781186548,
1.,0.707106781186548,1.,0.707106781186548,1.,0.707106781186548,1.),(1.,
0.707106781186547,1.,0.707106781186547,1.,0.707106781186547,1.,0.707106781186547,
1.),(1.,0.707106781186547,1.,0.707106781186547,1.,0.707106781186547,1.,
0.707106781186547,1.),(1.,0.707106781186548,1.,0.707106781186548,1.,0.707106781186548,
1.,0.707106781186548,1.),(1.,0.707106781186548,1.,0.707106781186548,1.,
0.707106781186548,1.,0.707106781186548,1.),(1.,0.707106781186548,1.,0.707106781186548,
1.,0.707106781186548,1.,0.707106781186548,1.),(1.,0.707106781186547,1.,
0.707106781186547,1.,0.707106781186547,1.,0.707106781186547,1.),(1.,0.707106781186548,
1.,0.707106781186548,1.,0.707106781186548,1.,0.707106781186548,1.),(1.,
0.707106781186547,1.,0.707106781186547,1.,0.707106781186547,1.,0.707106781186547,
1.),(1.,0.707106781186548,1.,0.707106781186548,1.,0.707106781186548,1.,
0.707106781186548,1.),(1.,0.707106781186547,1.,0.707106781186547,1.,0.707106781186547,
1.,0.707106781186547,1.),(1.,0.707106781186548,1.,0.707106781186548,1.,
0.707106781186548,1.,0.707106781186548,1.),(1.,0.707106781186547,1.,0.707106781186547,
1.,0.707106781186547,1.,0.707106781186547,1.),(1.,0.707106781186547,1.,
0.707106781186547,1.,0.707106781186547,1.,0.707106781186547,1.),(1.,0.707106781186547,
1.,0.707106781186547,1.,0.707106781186547,1.,0.707106781186547,1.),(1.,
0.707106781186547,1.,0.707106781186547,1.,0.707106781186547,1.,0.707106781186547,
1.),(1.,0.707106781186548,1.,0.707106781186548,1.,0.707106781186548,1.,
0.707106781186548,1.),(1.,0.707106781186547,1.,0.707106781186547,1.,0.707106781186547,
1.,0.707106781186547,1.),(1.,0.707106781186548,1.,0.707106781186548,1.,
0.707106781186548,1.,0.707106781186548,1.),(1.,0.707106781186548,1.,0.707106781186548,
1.,0.707106781186548,1.,0.707106781186548,1.),(1.,0.707106781186547,1.,
0.707106781186547,1.,0.707106781186547,1.,0.707106781186547,1.),(1.,0.707106781186548,
1.,0.707106781186548,1.,0.707106781186548,1.,0.707106781186548,1.),(1.,
0.707106781186547,1.,0.707106781186547,1.,0.707106781186547,1.,0.707106781186547,
1.),(1.,0.707106781186547,1.,0.707106781186547,1.,0.707106781186547,1.,
0.707106781186547,1.),(1.,0.707106781186547,1.,0.707106781186547,1.,0.707106781186547,
1.,0.707106781186547,1.),(1.,0.707106781186547,1.,0.707106781186547,1.,
0.707106781186547,1.,0.707106781186547,1.),(1.,0.707106781186548,1.,0.707106781186548,
1.,0.707106781186548,1.,0.707106781186548,1.),(1.,0.707106781186547,1.,
0.707106781186547,1.,0.707106781186547,1.,0.707106781186547,1.),(1.,0.707106781186548,
1.,0.707106781186548,1.,0.707106781186548,1.,0.707106781186548,1.),(1.,
0.707106781186547,1.,0.707106781186547,1.,0.707106781186547,1.,0.707106781186547,
1.),(1.,0.707106781186548,1.,0.707106781186548,1.,0.707106781186548,1.,
0.707106781186548,1.),(1.,0.707106781186548,1.,0.707106781186548,1.,0.707106781186548,
1.,0.707106781186548,1.),(1.,0.707106781186547,1.,0.707106781186547,1.,
0.707106781186547,1.,0.707106781186547,1.),(1.,0.707106781186548,1.,0.707106781186548,
1.,0.707106781186548,1.,0.707106781186548,1.),(1.,0.707106781186547,1.,
0.707106781186547,1.,0.707106781186547,1.,0.707106781186547,1.),(1.,0.707106781186547,
1.,0.707106781186547,1.,0.707106781186547,1.,0.707106781186547,1.),(1.,
0.707106781186547,1.,0.707106781186547,1.,0.707106781186547,1.,0.707106781186547,
1.),(1.,0.707106781186547,1.,0.707106781186547,1.,0.707106781186547,1.,
0.707106781186547,1.),(1.,0.707106781186548,1.,0.707106781186548,1.,0.707106781186548,
1.,0.707106781186548,1.),(1.,0.707106781186547,1.,0.707106781186547,1.,
0.707106781186547,1.,0.707106781186547,1.),(1.,0.707106781186548,1.,0.707106781186548,
1.,0.707106781186548,1.,0.707106781186548,1.),(1.,0.707106781186548,1.,
0.707106781186548,1.,0.707106781186548,1.,0.707106781186548,1.),(1.,0.707106781186547,
1.,0.707106781186547,1.,0.707106781186547,1.,0.707106781186547,1.),(1.,
0.707106781186548,1.,0.707106781186548,1.,0.707106781186548,1.,0.707106781186548,
1.),(1.,0.707106781186547,1.,0.707106781186547,1.,0.707106781186547,1.,
0.707106781186547,1.),(1.,0.707106781186548,1.,0.707106781186548,1.,0.707106781186548,
1.,0.707106781186548,1.),(1.,0.707106781186547,1.,0.707106781186547,1.,
0.707106781186547,1.,0.707106781186547,1.),(1.,0.707106781186547,1.,0.707106781186547,
1.,0.707106781186547,1.,0.707106781186547,1.),(1.,0.707106781186548,1.,
0.707106781186548,1.,0.707106781186548,1.,0.707106781186548,1.),(1.,0.707106781186547,
1.,0.707106781186547,1.,0.707106781186547,1.,0.707106781186547,1.),(1.,
0.707106781186548,1.,0.707106781186548,1.,0.707106781186548,1.,0.707106781186548,
1.),(1.,0.707106781186548,1.,0.707106781186548,1.,0.707106781186548,1.,
0.707106781186548,1.),(1.,0.707106781186547,1.,0.707106781186547,1.,0.707106781186547,
1.,0.707106781186547,1.),(1.,0.707106781186547,1.,0.707106781186547,1.,
0.707106781186547,1.,0.707106781186547,1.),(1.,0.707106781186548,1.,0.707106781186548,
1.,0.707106781186548,1.,0.707106781186548,1.),(1.,0.707106781186548,1.,
0.707106781186548,1.,0.707106781186548,1.,0.707106781186548,1.),(1.,0.707106781186547,
1.,0.707106781186547,1.,0.707106781186547,1.,0.707106781186547,1.),(1.,
0.707106781186547,1.,0.707106781186547,1.,0.707106781186547,1.,0.707106781186547,
1.),(1.,0.707106781186548,1.,0.707106781186548,1.,0.707106781186548,1.,
0.707106781186548,1.),(1.,0.707106781186547,1.,0.707106781186547,1.,0.707106781186547,
1.,0.707106781186547,1.),(1.,0.707106781186547,1.,0.707106781186547,1.,
0.707106781186547,1.,0.707106781186547,1.),(1.,0.707106781186548,1.,0.707106781186548,
1.,0.707106781186548,1.,0.707106781186548,1.),(1.,0.707106781186547,1.,
0.707106781186547,1.,0.707106781186547,1.,0.707106781186547,1.),(1.,0.707106781186547,
1.,0.707106781186547,1.,0.707106781186547,1.,0.707106781186547,1.),(1.,
0.707106781186548,1.,0.707106781186548,1.,0.707106781186548,1.,0.707106781186548,
1.),(1.,0.707106781186547,1.,0.707106781186547,1.,0.707106781186547,1.,
0.707106781186547,1.),(1.,0.707106781186548,1.,0.707106781186548,1.,0.707106781186548,
1.,0.707106781186548,1.),(1.,0.707106781186547,1.,0.707106781186547,1.,
0.707106781186547,1.,0.707106781186547,1.),(1.,0.707106781186547,1.,0.707106781186547,
1.,0.707106781186547,1.,0.707106781186547,1.),(1.,0.707106781186548,1.,
0.707106781186548,1.,0.707106781186548,1.,0.707106781186548,1.),(1.,0.707106781186547,
1.,0.707106781186547,1.,0.707106781186547,1.,0.707106781186547,1.),(1.,
0.707106781186548,1.,0.707106781186548,1.,0.707106781186548,1.,0.707106781186548,
1.),(1.,0.707106781186547,1.,0.707106781186547,1.,0.707106781186547,1.,
0.707106781186547,1.),(1.,0.707106781186548,1.,0.707106781186548,1.,0.707106781186548,
1.,0.707106781186548,1.),(1.,0.707106781186547,1.,0.707106781186547,1.,
0.707106781186547,1.,0.707106781186547,1.),(1.,0.707106781186547,1.,0.707106781186547,
1.,0.707106781186547,1.,0.707106781186547,1.),(1.,0.707106781186547,1.,
0.707106781186547,1.,0.707106781186547,1.,0.707106781186547,1.),(1.,0.707106781186548,
1.,0.707106781186548,1.,0.707106781186548,1.,0.707106781186548,1.),(1.,
0.707106781186547,1.,0.707106781186547,1.,0.707106781186547,1.,0.707106781186547,
1.),(1.,0.707106781186548,1.,0.707106781186548,1.,0.707106781186548,1.,
0.707106781186548,1.),(1.,0.707106781186547,1.,0.707106781186547,1.,0.707106781186547,
1.,0.707106781186547,1.),(1.,0.707106781186548,1.,0.707106781186548,1.,
0.707106781186548,1.,0.707106781186548,1.),(1.,0.707106781186548,1.,0.707106781186548,
1.,0.707106781186548,1.,0.707106781186548,1.),(1.,0.707106781186548,1.,
0.707106781186548,1.,0.707106781186548,1.,0.707106781186548,1.),(1.,0.707106781186548,
1.,0.707106781186548,1.,0.707106781186548,1.,0.707106781186548,1.),(1.,
0.707106781186547,1.,0.707106781186547,1.,0.707106781186547,1.,0.707106781186547,
1.),(1.,0.707106781186547,1.,0.707106781186547,1.,0.707106781186547,1.,
0.707106781186547,1.),(1.,0.707106781186547,1.,0.707106781186547,1.,0.707106781186547,
1.,0.707106781186547,1.),(1.,0.707106781186548,1.,0.707106781186548,1.,
0.707106781186548,1.,0.707106781186548,1.),(1.,0.707106781186547,1.,0.707106781186547,
1.,0.707106781186547,1.,0.707106781186547,1.),(1.,0.707106781186548,1.,
0.707106781186548,1.,0.707106781186548,1.,0.707106781186548,1.),(1.,0.707106781186547,
1.,0.707106781186547,1.,0.707106781186547,1.,0.707106781186547,1.),(1.,
0.707106781186547,1.,0.707106781186547,1.,0.707106781186547,1.,0.707106781186547,
1.),(1.,0.707106781186548,1.,0.707106781186548,1.,0.707106781186548,1.,
0.707106781186548,1.),(1.,0.707106781186547,1.,0.707106781186547,1.,0.707106781186547,
1.,0.707106781186547,1.),(1.,0.707106781186547,1.,0.707106781186547,1.,
0.707106781186547,1.,0.707106781186547,1.),(1.,0.707106781186548,1.,0.707106781186548,
1.,0.707106781186548,1.,0.707106781186548,1.),(1.,0.707106781186547,1.,
0.707106781186547,1.,0.707106781186547,1.,0.707106781186547,1.),(1.,0.707106781186547,
1.,0.707106781186547,1.,0.707106781186547,1.,0.707106781186547,1.),(1.,
0.707106781186548,1.,0.707106781186548,1.,0.707106781186548,1.,0.707106781186548,
1.),(1.,0.707106781186548,1.,0.707106781186548,1.,0.707106781186548,1.,
0.707106781186548,1.),(1.,0.707106781186547,1.,0.707106781186547,1.,0.707106781186547,
1.,0.707106781186547,1.),(1.,0.707106781186548,1.,0.707106781186548,1.,
0.707106781186548,1.,0.707106781186548,1.),(1.,0.707106781186547,1.,0.707106781186547,
1.,0.707106781186547,1.,0.707106781186547,1.),(1.,0.707106781186547,1.,
0.707106781186547,1.,0.707106781186547,1.,0.707106781186547,1.),(1.,0.707106781186548,
1.,0.707106781186548,1.,0.707106781186548,1.,0.707106781186548,1.),(1.,
0.707106781186547,1.,0.707106781186547,1.,0.707106781186547,1.,0.707106781186547,
1.),(1.,0.707106781186548,1.,0.707106781186548,1.,0.707106781186548,1.,
0.707106781186548,1.),(1.,0.707106781186547,1.,0.707106781186547,1.,0.707106781186547,
1.,0.707106781186547,1.),(1.,0.707106781186548,1.,0.707106781186548,1.,
0.707106781186548,1.,0.707106781186548,1.),(1.,0.707106781186547,1.,0.707106781186547,
1.,0.707106781186547,1.,0.707106781186547,1.),(1.,0.707106781186547,1.,
0.707106781186547,1.,0.707106781186547,1.,0.707106781186547,1.),(1.,0.707106781186547,
1.,0.707106781186547,1.,0.707106781186547,1.,0.707106781186547,1.),(1.,
0.707106781186548,1.,0.707106781186548,1.,0.707106781186548,1.,0.707106781186548,
1.),(1.,0.707106781186547,1.,0.707106781186547,1.,0.707106781186547,1.,
0.707106781186547,1.),(1.,0.707106781186548,1.,0.707106781186548,1.,0.707106781186548,
1.,0.707106781186548,1.),(1.,0.707106781186547,1.,0.707106781186547,1.,
0.707106781186547,1.,0.707106781186547,1.),(1.,0.707106781186548,1.,0.707106781186548,
1.,0.707106781186548,1.,0.707106781186548,1.),(1.,0.707106781186547,1.,
0.707106781186547,1.,0.707106781186547,1.,0.707106781186547,1.),(1.,0.707106781186547,
1.,0.707106781186547,1.,0.707106781186547,1.,0.707106781186547,1.),(1.,
0.707106781186548,1.,0.707106781186548,1.,0.707106781186548,1.,0.707106781186548,
1.),(1.,0.707106781186548,1.,0.707106781186548,1.,0.707106781186548,1.,
0.707106781186548,1.),(1.,0.707106781186548,1.,0.707106781186548,1.,0.707106781186548,
1.,0.707106781186548,1.),(1.,0.707106781186547,1.,0.707106781186547,1.,
0.707106781186547,1.,0.707106781186547,1.),(1.,0.707106781186548,1.,0.707106781186548,
1.,0.707106781186548,1.,0.707106781186548,1.),(1.,0.707106781186547,1.,
0.707106781186547,1.,0.707106781186547,1.,0.707106781186547,1.),(1.,0.707106781186548,
1.,0.707106781186548,1.,0.707106781186548,1.,0.707106781186548,1.),(1.,
0.707106781186547,1.,0.707106781186547,1.,0.707106781186547,1.,0.707106781186547,
1.),(1.,0.707106781186548,1.,0.707106781186548,1.,0.707106781186548,1.,
0.707106781186548,1.),(1.,0.707106781186547,1.,0.707106781186547,1.,0.707106781186547,
1.,0.707106781186547,1.),(1.,0.707106781186548,1.,0.707106781186548,1.,
0.707106781186548,1.,0.707106781186548,1.),(1.,0.707106781186548,1.,0.707106781186548,
1.,0.707106781186548,1.,0.707106781186548,1.),(1.,0.707106781186547,1.,
0.707106781186547,1.,0.707106781186547,1.,0.707106781186547,1.),(1.,0.707106781186547,
1.,0.707106781186547,1.,0.707106781186547,1.,0.707106781186547,1.),(1.,
0.707106781186547,1.,0.707106781186547,1.,0.707106781186547,1.,0.707106781186547,
1.),(1.,0.707106781186548,1.,0.707106781186548,1.,0.707106781186548,1.,
0.707106781186548,1.),(1.,0.707106781186547,1.,0.707106781186547,1.,0.707106781186547,
1.,0.707106781186547,1.),(1.,0.707106781186547,1.,0.707106781186547,1.,
0.707106781186547,1.,0.707106781186547,1.),(1.,0.707106781186548,1.,0.707106781186548,
1.,0.707106781186548,1.,0.707106781186548,1.),(1.,0.707106781186547,1.,
0.707106781186547,1.,0.707106781186547,1.,0.707106781186547,1.),(1.,0.707106781186547,
1.,0.707106781186547,1.,0.707106781186547,1.,0.707106781186547,1.),(1.,
0.707106781186548,1.,0.707106781186548,1.,0.707106781186548,1.,0.707106781186548,
1.),(1.,0.707106781186547,1.,0.707106781186547,1.,0.707106781186547,1.,
0.707106781186547,1.),(1.,0.707106781186548,1.,0.707106781186548,1.,0.707106781186548,
1.,0.707106781186548,1.),(1.,0.707106781186548,1.,0.707106781186548,1.,
0.707106781186548,1.,0.707106781186548,1.),(1.,0.707106781186548,1.,0.707106781186548,
1.,0.707106781186548,1.,0.707106781186548,1.),(1.,0.707106781186547,1.,
0.707106781186547,1.,0.707106781186547,1.,0.707106781186547,1.),(1.,0.707106781186548,
1.,0.707106781186548,1.,0.707106781186548,1.,0.707106781186548,1.),(1.,
0.707106781186547,1.,0.707106781186547,1.,0.707106781186547,1.,0.707106781186547,
1.),(1.,0.707106781186548,1.,0.707106781186548,1.,0.707106781186548,1.,
0.707106781186548,1.),(1.,0.707106781186547,1.,0.707106781186547,1.,0.707106781186547,
1.,0.707106781186547,1.),(1.,0.707106781186548,1.,0.707106781186548,1.,
0.707106781186548,1.,0.707106781186548,1.),(1.,0.707106781186547,1.,0.707106781186547,
1.,0.707106781186547,1.,0.707106781186547,1.),(1.,0.707106781186548,1.,
0.707106781186548,1.,0.707106781186548,1.,0.707106781186548,1.),(1.,0.707106781186547,
1.,0.707106781186547,1.,0.707106781186547,1.,0.707106781186547,1.),(1.,
0.707106781186548,1.,0.707106781186548,1.,0.707106781186548,1.,0.707106781186548,
1.),(1.,0.707106781186547,1.,0.707106781186547,1.,0.707106781186547,1.,
0.707106781186547,1.),(1.,0.707106781186548,1.,0.707106781186548,1.,0.707106781186548,
1.,0.707106781186548,1.),(1.,0.707106781186548,1.,0.707106781186548,1.,
0.707106781186548,1.,0.707106781186548,1.),(1.,0.707106781186547,1.,0.707106781186547,
1.,0.707106781186547,1.,0.707106781186547,1.),(1.,0.707106781186548,1.,
0.707106781186548,1.,0.707106781186548,1.,0.707106781186548,1.),(1.,0.707106781186547,
1.,0.707106781186547,1.,0.707106781186547,1.,0.707106781186547,1.),(1.,
0.707106781186548,1.,0.707106781186548,1.,0.707106781186548,1.,0.707106781186548,
1.),(1.,0.707106781186548,1.,0.707106781186548,1.,0.707106781186548,1.,
0.707106781186548,1.),(1.,0.707106781186547,1.,0.707106781186547,1.,0.707106781186547,
1.,0.707106781186547,1.),(1.,0.707106781186547,1.,0.707106781186547,1.,
0.707106781186547,1.,0.707106781186547,1.),(1.,0.707106781186548,1.,0.707106781186548,
1.,0.707106781186548,1.,0.707106781186548,1.),(1.,0.707106781186547,1.,
0.707106781186547,1.,0.707106781186547,1.,0.707106781186547,1.),(1.,0.707106781186547,
1.,0.707106781186547,1.,0.707106781186547,1.,0.707106781186547,1.),(1.,
0.707106781186548,1.,0.707106781186548,1.,0.707106781186548,1.,0.707106781186548,
1.),(1.,0.707106781186547,1.,0.707106781186547,1.,0.707106781186547,1.,
0.707106781186547,1.),(1.,0.707106781186548,1.,0.707106781186548,1.,0.707106781186548,
1.,0.707106781186548,1.),(1.,0.707106781186548,1.,0.707106781186548,1.,
0.707106781186548,1.,0.707106781186548,1.),(1.,0.707106781186547,1.,0.707106781186547,
1.,0.707106781186547,1.,0.707106781186547,1.),(1.,0.707106781186548,1.,
0.707106781186548,1.,0.707106781186548,1.,0.707106781186548,1.),(1.,0.707106781186548,
1.,0.707106781186548,1.,0.707106781186548,1.,0.707106781186548,1.),(1.,
0.707106781186548,1.,0.707106781186548,1.,0.707106781186548,1.,0.707106781186548,
1.),(1.,0.707106781186548,1.,0.707106781186548,1.,0.707106781186548,1.,
0.707106781186548,1.),(1.,0.707106781186548,1.,0.707106781186548,1.,0.707106781186548,
1.,0.707106781186548,1.),(1.,0.707106781186547,1.,0.707106781186547,1.,
0.707106781186547,1.,0.707106781186547,1.),(1.,0.707106781186548,1.,0.707106781186548,
1.,0.707106781186548,1.,0.707106781186548,1.),(1.,0.707106781186548,1.,
0.707106781186548,1.,0.707106781186548,1.,0.707106781186548,1.),(1.,0.707106781186548,
1.,0.707106781186548,1.,0.707106781186548,1.,0.707106781186548,1.),(1.,
0.707106781186547,1.,0.707106781186547,1.,0.707106781186547,1.,0.707106781186547,
1.),(1.,0.707106781186548,1.,0.707106781186548,1.,0.707106781186548,1.,
0.707106781186548,1.),(1.,0.707106781186547,1.,0.707106781186547,1.,0.707106781186547,
1.,0.707106781186547,1.),(1.,0.707106781186548,1.,0.707106781186548,1.,
0.707106781186548,1.,0.707106781186548,1.),(1.,0.707106781186547,1.,0.707106781186547,
1.,0.707106781186547,1.,0.707106781186547,1.),(1.,0.707106781186548,1.,
0.707106781186548,1.,0.707106781186548,1.,0.707106781186548,1.),(1.,0.707106781186547,
1.,0.707106781186547,1.,0.707106781186547,1.,0.707106781186547,1.),(1.,
0.707106781186548,1.,0.707106781186548,1.,0.707106781186548,1.,0.707106781186548,
1.),(1.,0.707106781186547,1.,0.707106781186547,1.,0.707106781186547,1.,
0.707106781186547,1.),(1.,0.707106781186548,1.,0.707106781186548,1.,0.707106781186548,
1.,0.707106781186548,1.),(1.,0.707106781186547,1.,0.707106781186547,1.,
0.707106781186547,1.,0.707106781186547,1.),(1.,0.707106781186547,1.,0.707106781186547,
1.,0.707106781186547,1.,0.707106781186547,1.),(1.,0.707106781186548,1.,
0.707106781186548,1.,0.707106781186548,1.,0.707106781186548,1.),(1.,0.707106781186547,
1.,0.707106781186547,1.,0.707106781186547,1.,0.707106781186547,1.),(1.,
0.707106781186547,1.,0.707106781186547,1.,0.707106781186547,1.,0.707106781186547,
1.),(1.,0.707106781186548,1.,0.707106781186548,1.,0.707106781186548,1.,
0.707106781186548,1.),(1.,0.707106781186547,1.,0.707106781186547,1.,0.707106781186547,
1.,0.707106781186547,1.),(1.,0.707106781186548,1.,0.707106781186548,1.,
0.707106781186548,1.,0.707106781186548,1.),(1.,0.707106781186547,1.,0.707106781186547,
1.,0.707106781186547,1.,0.707106781186547,1.),(1.,0.707106781186548,1.,
0.707106781186548,1.,0.707106781186548,1.,0.707106781186548,1.),(1.,0.707106781186547,
1.,0.707106781186547,1.,0.707106781186547,1.,0.707106781186547,1.),(1.,
0.707106781186548,1.,0.707106781186548,1.,0.707106781186548,1.,0.707106781186548,
1.),(1.,0.707106781186547,1.,0.707106781186547,1.,0.707106781186547,1.,
0.707106781186547,1.),(1.,0.707106781186547,1.,0.707106781186547,1.,0.707106781186547,
1.,0.707106781186547,1.),(1.,0.707106781186548,1.,0.707106781186548,1.,
0.707106781186548,1.,0.707106781186548,1.),(1.,0.707106781186547,1.,0.707106781186547,
1.,0.707106781186547,1.,0.707106781186547,1.),(1.,0.707106781186547,1.,
0.707106781186547,1.,0.707106781186547,1.,0.707106781186547,1.),(1.,0.707106781186548,
1.,0.707106781186548,1.,0.707106781186548,1.,0.707106781186548,1.),(1.,
0.707106781186547,1.,0.707106781186547,1.,0.707106781186547,1.,0.707106781186547,
1.),(1.,0.707106781186548,1.,0.707106781186548,1.,0.707106781186548,1.,
0.707106781186548,1.),(1.,0.707106781186547,1.,0.707106781186547,1.,0.707106781186547,
1.,0.707106781186547,1.),(1.,0.707106781186547,1.,0.707106781186547,1.,
0.707106781186547,1.,0.707106781186547,1.),(1.,0.707106781186548,1.,0.707106781186548,
1.,0.707106781186548,1.,0.707106781186548,1.),(1.,0.707106781186548,1.,
0.707106781186548,1.,0.707106781186548,1.,0.707106781186548,1.),(1.,0.707106781186547,
1.,0.707106781186547,1.,0.707106781186547,1.,0.707106781186547,1.),(1.,
0.707106781186548,1.,0.707106781186548,1.,0.707106781186548,1.,0.707106781186548,
1.),(1.,0.707106781186547,1.,0.707106781186547,1.,0.707106781186547,1.,
0.707106781186547,1.),(1.,0.707106781186547,1.,0.707106781186547,1.,0.707106781186547,
1.,0.707106781186547,1.),(1.,0.707106781186547,1.,0.707106781186547,1.,
0.707106781186547,1.,0.707106781186547,1.),(1.,0.707106781186548,1.,0.707106781186548,
1.,0.707106781186548,1.,0.707106781186548,1.),(1.,0.707106781186547,1.,
0.707106781186547,1.,0.707106781186547,1.,0.707106781186547,1.),(1.,0.707106781186547,
1.,0.707106781186547,1.,0.707106781186547,1.,0.707106781186547,1.),(1.,
0.707106781186548,1.,0.707106781186548,1.,0.707106781186548,1.,0.707106781186548,
1.),(1.,0.707106781186547,1.,0.707106781186547,1.,0.707106781186547,1.,
0.707106781186547,1.),(1.,0.707106781186547,1.,0.707106781186547,1.,0.707106781186547,
1.,0.707106781186547,1.),(1.,0.707106781186547,1.,0.707106781186547,1.,
0.707106781186547,1.,0.707106781186547,1.),(1.,0.707106781186548,1.,0.707106781186548,
1.,0.707106781186548,1.,0.707106781186548,1.),(1.,0.707106781186548,1.,
0.707106781186548,1.,0.707106781186548,1.,0.707106781186548,1.),(1.,0.707106781186547,
1.,0.707106781186547,1.,0.707106781186547,1.,0.707106781186547,1.),(1.,
0.707106781186548,1.,0.707106781186548,1.,0.707106781186548,1.,0.707106781186548,
1.),(1.,0.707106781186547,1.,0.707106781186547,1.,0.707106781186547,1.,
0.707106781186547,1.),(1.,0.707106781186548,1.,0.707106781186548,1.,0.707106781186548,
1.,0.707106781186548,1.),(1.,0.707106781186547,1.,0.707106781186547,1.,
0.707106781186547,1.,0.707106781186547,1.),(1.,0.707106781186547,1.,0.707106781186547,
1.,0.707106781186547,1.,0.707106781186547,1.),(1.,0.707106781186548,1.,
0.707106781186548,1.,0.707106781186548,1.,0.707106781186548,1.),(1.,0.707106781186547,
1.,0.707106781186547,1.,0.707106781186547,1.,0.707106781186547,1.),(1.,
0.707106781186548,1.,0.707106781186548,1.,0.707106781186548,1.,0.707106781186548,
1.),(1.,0.707106781186547,1.,0.707106781186547,1.,0.707106781186547,1.,
0.707106781186547,1.),(1.,0.707106781186547,1.,0.707106781186547,1.,0.707106781186547,
1.,0.707106781186547,1.),(1.,0.707106781186547,1.,0.707106781186547,1.,
0.707106781186547,1.,0.707106781186547,1.),(1.,0.707106781186547,1.,0.707106781186547,
1.,0.707106781186547,1.,0.707106781186547,1.),(1.,0.707106781186548,1.,
0.707106781186548,1.,0.707106781186548,1.,0.707106781186548,1.),(1.,0.707106781186547,
1.,0.707106781186547,1.,0.707106781186547,1.,0.707106781186547,1.),(1.,
0.707106781186547,1.,0.707106781186547,1.,0.707106781186547,1.,0.707106781186547,
1.),(1.,0.707106781186547,1.,0.707106781186547,1.,0.707106781186547,1.,
0.707106781186547,1.),(1.,0.707106781186547,1.,0.707106781186547,1.,0.707106781186547,
1.,0.707106781186547,1.),(1.,0.707106781186547,1.,0.707106781186547,1.,
0.707106781186547,1.,0.707106781186547,1.),(1.,0.707106781186548,1.,0.707106781186548,
1.,0.707106781186548,1.,0.707106781186548,1.),(1.,0.707106781186547,1.,
0.707106781186547,1.,0.707106781186547,1.,0.707106781186547,1.),(1.,0.707106781186547,
1.,0.707106781186547,1.,0.707106781186547,1.,0.707106781186547,1.),(1.,
0.707106781186547,1.,0.707106781186547,1.,0.707106781186547,1.,0.707106781186547,
1.),(1.,0.707106781186547,1.,0.707106781186547,1.,0.707106781186547,1.,
0.707106781186547,1.),(1.,0.707106781186548,1.,0.707106781186548,1.,0.707106781186548,
1.,0.707106781186548,1.),(1.,0.707106781186547,1.,0.707106781186547,1.,
0.707106781186547,1.,0.707106781186547,1.),(1.,0.707106781186548,1.,0.707106781186548,
1.,0.707106781186548,1.,0.707106781186548,1.),(1.,0.707106781186547,1.,
0.707106781186547,1.,0.707106781186547,1.,0.707106781186547,1.),(1.,0.707106781186547,
1.,0.707106781186547,1.,0.707106781186547,1.,0.707106781186547,1.),(1.,
0.707106781186548,1.,0.707106781186548,1.,0.707106781186548,1.,0.707106781186548,
1.),(1.,0.707106781186547,1.,0.707106781186547,1.,0.707106781186547,1.,
0.707106781186547,1.),(1.,0.707106781186548,1.,0.707106781186548,1.,0.707106781186548,
1.,0.707106781186548,1.),(1.,0.707106781186547,1.,0.707106781186547,1.,
0.707106781186547,1.,0.707106781186547,1.),(1.,0.707106781186547,1.,0.707106781186547,
1.,0.707106781186547,1.,0.707106781186547,1.),(1.,0.707106781186548,1.,
0.707106781186548,1.,0.707106781186548,1.,0.707106781186548,1.),(1.,0.707106781186547,
1.,0.707106781186547,1.,0.707106781186547,1.,0.707106781186547,1.),(1.,
0.707106781186547,1.,0.707106781186547,1.,0.707106781186547,1.,0.707106781186547,
1.),(1.,0.707106781186548,1.,0.707106781186548,1.,0.707106781186548,1.,
0.707106781186548,1.),(1.,0.707106781186547,1.,0.707106781186547,1.,0.707106781186547,
1.,0.707106781186547,1.),(1.,0.707106781186547,1.,0.707106781186547,1.,
0.707106781186547,1.,0.707106781186547,1.),(1.,0.707106781186547,1.,0.707106781186547,
1.,0.707106781186547,1.,0.707106781186547,1.),(1.,0.707106781186547,1.,
0.707106781186547,1.,0.707106781186547,1.,0.707106781186547,1.),(1.,0.707106781186548,
1.,0.707106781186548,1.,0.707106781186548,1.,0.707106781186548,1.),(1.,
0.707106781186547,1.,0.707106781186547,1.,0.707106781186547,1.,0.707106781186547,
1.),(1.,0.707106781186548,1.,0.707106781186548,1.,0.707106781186548,1.,
0.707106781186548,1.),(1.,0.707106781186548,1.,0.707106781186548,1.,0.707106781186548,
1.,0.707106781186548,1.),(1.,0.707106781186547,1.,0.707106781186547,1.,
0.707106781186547,1.,0.707106781186547,1.),(1.,0.707106781186548,1.,0.707106781186548,
1.,0.707106781186548,1.,0.707106781186548,1.),(1.,0.707106781186548,1.,
0.707106781186548,1.,0.707106781186548,1.,0.707106781186548,1.),(1.,0.707106781186547,
1.,0.707106781186547,1.,0.707106781186547,1.,0.707106781186547,1.),(1.,
0.707106781186547,1.,0.707106781186547,1.,0.707106781186547,1.,0.707106781186547,
1.),(1.,0.707106781186548,1.,0.707106781186548,1.,0.707106781186548,1.,
0.707106781186548,1.),(1.,0.707106781186547,1.,0.707106781186547,1.,0.707106781186547,
1.,0.707106781186547,1.),(1.,0.707106781186547,1.,0.707106781186547,1.,
0.707106781186547,1.,0.707106781186547,1.),(1.,0.707106781186547,1.,0.707106781186547,
1.,0.707106781186547,1.,0.707106781186547,1.),(1.,0.707106781186548,1.,
0.707106781186548,1.,0.707106781186548,1.,0.707106781186548,1.),(1.,0.707106781186547,
1.,0.707106781186547,1.,0.707106781186547,1.,0.707106781186547,1.),(1.,
0.707106781186547,1.,0.707106781186547,1.,0.707106781186547,1.,0.707106781186547,
1.),(1.,0.707106781186548,1.,0.707106781186548,1.,0.707106781186548,1.,
0.707106781186548,1.),(1.,0.707106781186547,1.,0.707106781186547,1.,0.707106781186547,
1.,0.707106781186547,1.),(1.,0.707106781186548,1.,0.707106781186548,1.,
0.707106781186548,1.,0.707106781186548,1.),(1.,0.707106781186547,1.,0.707106781186547,
1.,0.707106781186547,1.,0.707106781186547,1.),(1.,0.707106781186548,1.,
0.707106781186548,1.,0.707106781186548,1.,0.707106781186548,1.),(1.,0.707106781186547,
1.,0.707106781186547,1.,0.707106781186547,1.,0.707106781186547,1.),(1.,
0.707106781186547,1.,0.707106781186547,1.,0.707106781186547,1.,0.707106781186547,
1.),(1.,0.707106781186548,1.,0.707106781186548,1.,0.707106781186548,1.,
0.707106781186548,1.),(1.,0.707106781186547,1.,0.707106781186547,1.,0.707106781186547,
1.,0.707106781186547,1.),(1.,0.707106781186548,1.,0.707106781186548,1.,
0.707106781186548,1.,0.707106781186548,1.),(1.,0.707106781186547,1.,0.707106781186547,
1.,0.707106781186547,1.,0.707106781186547,1.),(1.,0.707106781186548,1.,
0.707106781186548,1.,0.707106781186548,1.,0.707106781186548,1.),(1.,0.707106781186547,
1.,0.707106781186547,1.,0.707106781186547,1.,0.707106781186547,1.),(1.,
0.707106781186548,1.,0.707106781186548,1.,0.707106781186548,1.,0.707106781186548,
1.),(1.,0.707106781186547,1.,0.707106781186547,1.,0.707106781186547,1.,
0.707106781186547,1.),(1.,0.707106781186548,1.,0.707106781186548,1.,0.707106781186548,
1.,0.707106781186548,1.),(1.,0.707106781186547,1.,0.707106781186547,1.,
0.707106781186547,1.,0.707106781186547,1.),(1.,0.707106781186547,1.,0.707106781186547,
1.,0.707106781186547,1.,0.707106781186547,1.),(1.,0.707106781186547,1.,
0.707106781186547,1.,0.707106781186547,1.,0.707106781186547,1.),(1.,0.707106781186547,
1.,0.707106781186547,1.,0.707106781186547,1.,0.707106781186547,1.),(1.,
0.707106781186548,1.,0.707106781186548,1.,0.707106781186548,1.,0.707106781186548,
1.),(1.,0.707106781186548,1.,0.707106781186548,1.,0.707106781186548,1.,
0.707106781186548,1.),(1.,0.707106781186547,1.,0.707106781186547,1.,0.707106781186547,
1.,0.707106781186547,1.),(1.,0.707106781186548,1.,0.707106781186548,1.,
0.707106781186548,1.,0.707106781186548,1.),(1.,0.707106781186548,1.,0.707106781186548,
1.,0.707106781186548,1.,0.707106781186548,1.),(1.,0.707106781186547,1.,
0.707106781186547,1.,0.707106781186547,1.,0.707106781186547,1.),(1.,0.707106781186548,
1.,0.707106781186548,1.,0.707106781186548,1.,0.707106781186548,1.),(1.,
0.707106781186547,1.,0.707106781186547,1.,0.707106781186547,1.,0.707106781186547,
1.),(1.,0.707106781186547,1.,0.707106781186547,1.,0.707106781186547,1.,
0.707106781186547,1.),(1.,0.707106781186548,1.,0.707106781186548,1.,0.707106781186548,
1.,0.707106781186548,1.),(1.,0.707106781186547,1.,0.707106781186547,1.,
0.707106781186547,1.,0.707106781186547,1.),(1.,0.707106781186547,1.,0.707106781186547,
1.,0.707106781186547,1.,0.707106781186547,1.),(1.,0.707106781186547,1.,
0.707106781186547,1.,0.707106781186547,1.,0.707106781186547,1.),(1.,0.707106781186547,
1.,0.707106781186547,1.,0.707106781186547,1.,0.707106781186547,1.),(1.,
0.707106781186548,1.,0.707106781186548,1.,0.707106781186548,1.,0.707106781186548,
1.),(1.,0.707106781186547,1.,0.707106781186547,1.,0.707106781186547,1.,
0.707106781186547,1.),(1.,0.707106781186547,1.,0.707106781186547,1.,0.707106781186547,
1.,0.707106781186547,1.),(1.,0.707106781186547,1.,0.707106781186547,1.,
0.707106781186547,1.,0.707106781186547,1.),(1.,0.707106781186548,1.,0.707106781186548,
1.,0.707106781186548,1.,0.707106781186548,1.),(1.,0.707106781186547,1.,
0.707106781186547,1.,0.707106781186547,1.,0.707106781186547,1.),(1.,0.707106781186547,
1.,0.707106781186547,1.,0.707106781186547,1.,0.707106781186547,1.),(1.,
0.707106781186548,1.,0.707106781186548,1.,0.707106781186548,1.,0.707106781186548,
1.),(1.,0.707106781186547,1.,0.707106781186547,1.,0.707106781186547,1.,
0.707106781186547,1.),(1.,0.707106781186548,1.,0.707106781186548,1.,0.707106781186548,
1.,0.707106781186548,1.),(1.,0.707106781186548,1.,0.707106781186548,1.,
0.707106781186548,1.,0.707106781186548,1.),(1.,0.707106781186547,1.,0.707106781186547,
1.,0.707106781186547,1.,0.707106781186547,1.),(1.,0.707106781186548,1.,
0.707106781186548,1.,0.707106781186548,1.,0.707106781186548,1.),(1.,0.707106781186547,
1.,0.707106781186547,1.,0.707106781186547,1.,0.707106781186547,1.),(1.,
0.707106781186548,1.,0.707106781186548,1.,0.707106781186548,1.,0.707106781186548,
1.),(1.,0.707106781186547,1.,0.707106781186547,1.,0.707106781186547,1.,
0.707106781186547,1.),(1.,0.707106781186548,1.,0.707106781186548,1.,0.707106781186548,
1.,0.707106781186548,1.),(1.,0.707106781186547,1.,0.707106781186547,1.,
0.707106781186547,1.,0.707106781186547,1.),(1.,0.707106781186547,1.,0.707106781186547,
1.,0.707106781186547,1.,0.707106781186547,1.),(1.,0.707106781186548,1.,
0.707106781186548,1.,0.707106781186548,1.,0.707106781186548,1.),(1.,0.707106781186547,
1.,0.707106781186547,1.,0.707106781186547,1.,0.707106781186547,1.),(1.,
0.707106781186548,1.,0.707106781186548,1.,0.707106781186548,1.,0.707106781186548,
1.),(1.,0.707106781186548,1.,0.707106781186548,1.,0.707106781186548,1.,
0.707106781186548,1.),(1.,0.707106781186547,1.,0.707106781186547,1.,0.707106781186547,
1.,0.707106781186547,1.),(1.,0.707106781186547,1.,0.707106781186547,1.,
0.707106781186547,1.,0.707106781186547,1.),(1.,0.707106781186548,1.,0.707106781186548,
1.,0.707106781186548,1.,0.707106781186548,1.),(1.,0.707106781186547,1.,
0.707106781186547,1.,0.707106781186547,1.,0.707106781186547,1.),(1.,0.707106781186548,
1.,0.707106781186548,1.,0.707106781186548,1.,0.707106781186548,1.),(1.,
0.707106781186547,1.,0.707106781186547,1.,0.707106781186547,1.,0.707106781186547,
1.),(1.,0.707106781186548,1.,0.707106781186548,1.,0.707106781186548,1.,
0.707106781186548,1.),(1.,0.707106781186547,1.,0.707106781186547,1.,0.707106781186547,
1.,0.707106781186547,1.),(1.,0.707106781186547,1.,0.707106781186547,1.,
0.707106781186547,1.,0.707106781186547,1.),(1.,0.707106781186548,1.,0.707106781186548,
1.,0.707106781186548,1.,0.707106781186548,1.),(1.,0.707106781186548,1.,
0.707106781186548,1.,0.707106781186548,1.,0.707106781186548,1.),(1.,0.707106781186547,
1.,0.707106781186547,1.,0.707106781186547,1.,0.707106781186547,1.),(1.,
0.707106781186548,1.,0.707106781186548,1.,0.707106781186548,1.,0.707106781186548,
1.),(1.,0.707106781186548,1.,0.707106781186548,1.,0.707106781186548,1.,
0.707106781186548,1.),(1.,0.707106781186547,1.,0.707106781186547,1.,0.707106781186547,
1.,0.707106781186547,1.),(1.,0.707106781186548,1.,0.707106781186548,1.,
0.707106781186548,1.,0.707106781186548,1.),(1.,0.707106781186548,1.,0.707106781186548,
1.,0.707106781186548,1.,0.707106781186548,1.),(1.,0.707106781186547,1.,
0.707106781186547,1.,0.707106781186547,1.,0.707106781186547,1.),(1.,0.707106781186548,
1.,0.707106781186548,1.,0.707106781186548,1.,0.707106781186548,1.),(1.,
0.707106781186547,1.,0.707106781186547,1.,0.707106781186547,1.,0.707106781186547,
1.),(1.,0.707106781186548,1.,0.707106781186548,1.,0.707106781186548,1.,
0.707106781186548,1.),(1.,0.707106781186547,1.,0.707106781186547,1.,0.707106781186547,
1.,0.707106781186547,1.),(1.,0.707106781186548,1.,0.707106781186548,1.,
0.707106781186548,1.,0.707106781186548,1.),(1.,0.707106781186547,1.,0.707106781186547,
1.,0.707106781186547,1.,0.707106781186547,1.),(1.,0.707106781186548,1.,
0.707106781186548,1.,0.707106781186548,1.,0.707106781186548,1.),(1.,0.707106781186547,
1.,0.707106781186547,1.,0.707106781186547,1.,0.707106781186547,1.),(1.,
0.707106781186547,1.,0.707106781186547,1.,0.707106781186547,1.,0.707106781186547,
1.),(1.,0.707106781186548,1.,0.707106781186548,1.,0.707106781186548,1.,
0.707106781186548,1.),(1.,0.707106781186547,1.,0.707106781186547,1.,0.707106781186547,
1.,0.707106781186547,1.),(1.,0.707106781186547,1.,0.707106781186547,1.,
0.707106781186547,1.,0.707106781186547,1.),(1.,0.707106781186548,1.,0.707106781186548,
1.,0.707106781186548,1.,0.707106781186548,1.),(1.,0.707106781186547,1.,
0.707106781186547,1.,0.707106781186547,1.,0.707106781186547,1.),(1.,0.707106781186548,
1.,0.707106781186548,1.,0.707106781186548,1.,0.707106781186548,1.),(1.,
0.707106781186548,1.,0.707106781186548,1.,0.707106781186548,1.,0.707106781186548,
1.),(1.,0.707106781186547,1.,0.707106781186547,1.,0.707106781186547,1.,
0.707106781186547,1.),(1.,0.707106781186547,1.,0.707106781186547,1.,0.707106781186547,
1.,0.707106781186547,1.),(1.,0.707106781186547,1.,0.707106781186547,1.,
0.707106781186547,1.,0.707106781186547,1.),(1.,0.707106781186548,1.,0.707106781186548,
1.,0.707106781186548,1.,0.707106781186548,1.),(1.,0.707106781186547,1.,
0.707106781186547,1.,0.707106781186547,1.,0.707106781186547,1.),(1.,0.707106781186548,
1.,0.707106781186548,1.,0.707106781186548,1.,0.707106781186548,1.),(1.,
0.707106781186548,1.,0.707106781186548,1.,0.707106781186548,1.,0.707106781186548,
1.),(1.,0.707106781186547,1.,0.707106781186547,1.,0.707106781186547,1.,
0.707106781186547,1.),(1.,0.707106781186548,1.,0.707106781186548,1.,0.707106781186548,
1.,0.707106781186548,1.),(1.,0.707106781186547,1.,0.707106781186547,1.,
0.707106781186547,1.,0.707106781186547,1.),(1.,0.707106781186548,1.,0.707106781186548,
1.,0.707106781186548,1.,0.707106781186548,1.),(1.,0.707106781186547,1.,
0.707106781186547,1.,0.707106781186547,1.,0.707106781186547,1.),(1.,0.707106781186548,
1.,0.707106781186548,1.,0.707106781186548,1.,0.707106781186548,1.),(1.,
0.707106781186547,1.,0.707106781186547,1.,0.707106781186547,1.,0.707106781186547,
1.),(1.,0.707106781186547,1.,0.707106781186547,1.,0.707106781186547,1.,
0.707106781186547,1.),(1.,0.707106781186548,1.,0.707106781186548,1.,0.707106781186548,
1.,0.707106781186548,1.),(1.,0.707106781186548,1.,0.707106781186548,1.,
0.707106781186548,1.,0.707106781186548,1.),(1.,0.707106781186548,1.,0.707106781186548,
1.,0.707106781186548,1.,0.707106781186548,1.),(1.,0.707106781186547,1.,
0.707106781186547,1.,0.707106781186547,1.,0.707106781186547,1.),(1.,0.707106781186548,
1.,0.707106781186548,1.,0.707106781186548,1.,0.707106781186548,1.),(1.,
0.707106781186548,1.,0.707106781186548,1.,0.707106781186548,1.,0.707106781186548,
1.),(1.,0.707106781186547,1.,0.707106781186547,1.,0.707106781186547,1.,
0.707106781186547,1.),(1.,0.707106781186548,1.,0.707106781186548,1.,0.707106781186548,
1.,0.707106781186548,1.),(1.,0.707106781186547,1.,0.707106781186547,1.,
0.707106781186547,1.,0.707106781186547,1.),(1.,0.707106781186548,1.,0.707106781186548,
1.,0.707106781186548,1.,0.707106781186548,1.),(1.,0.707106781186548,1.,
0.707106781186548,1.,0.707106781186548,1.,0.707106781186548,1.),(1.,0.707106781186548,
1.,0.707106781186548,1.,0.707106781186548,1.,0.707106781186548,1.),(1.,
0.707106781186548,1.,0.707106781186548,1.,0.707106781186548,1.,0.707106781186548,
1.),(1.,0.707106781186548,1.,0.707106781186548,1.,0.707106781186548,1.,
0.707106781186548,1.),(1.,0.707106781186548,1.,0.707106781186548,1.,0.707106781186548,
1.,0.707106781186548,1.),(1.,0.707106781186547,1.,0.707106781186547,1.,
0.707106781186547,1.,0.707106781186547,1.),(1.,0.707106781186547,1.,0.707106781186547,
1.,0.707106781186547,1.,0.707106781186547,1.),(1.,0.707106781186548,1.,
0.707106781186548,1.,0.707106781186548,1.,0.707106781186548,1.),(1.,0.707106781186547,
1.,0.707106781186547,1.,0.707106781186547,1.,0.707106781186547,1.),(1.,
0.707106781186547,1.,0.707106781186547,1.,0.707106781186547,1.,0.707106781186547,
1.),(1.,0.707106781186548,1.,0.707106781186548,1.,0.707106781186548,1.,
0.707106781186548,1.),(1.,0.707106781186547,1.,0.707106781186547,1.,0.707106781186547,
1.,0.707106781186547,1.),(1.,0.707106781186547,1.,0.707106781186547,1.,
0.707106781186547,1.,0.707106781186547,1.),(1.,0.707106781186548,1.,0.707106781186548,
1.,0.707106781186548,1.,0.707106781186548,1.),(1.,0.707106781186547,1.,
0.707106781186547,1.,0.707106781186547,1.,0.707106781186547,1.),(1.,0.707106781186548,
1.,0.707106781186548,1.,0.707106781186548,1.,0.707106781186548,1.),(1.,
0.707106781186547,1.,0.707106781186547,1.,0.707106781186547,1.,0.707106781186547,
1.),(1.,0.707106781186548,1.,0.707106781186548,1.,0.707106781186548,1.,
0.707106781186548,1.),(1.,0.707106781186547,1.,0.707106781186547,1.,0.707106781186547,
1.,0.707106781186547,1.),(1.,0.707106781186547,1.,0.707106781186547,1.,
0.707106781186547,1.,0.707106781186547,1.),(1.,0.707106781186547,1.,0.707106781186547,
1.,0.707106781186547,1.,0.707106781186547,1.),(1.,0.707106781186548,1.,
0.707106781186548,1.,0.707106781186548,1.,0.707106781186548,1.),(1.,0.707106781186547,
1.,0.707106781186547,1.,0.707106781186547,1.,0.707106781186547,1.),(1.,
0.707106781186547,1.,0.707106781186547,1.,0.707106781186547,1.,0.707106781186547,
1.),(1.,0.707106781186548,1.,0.707106781186548,1.,0.707106781186548,1.,
0.707106781186548,1.),(1.,0.707106781186547,1.,0.707106781186547,1.,0.707106781186547,
1.,0.707106781186547,1.),(1.,0.707106781186548,1.,0.707106781186548,1.,
0.707106781186548,1.,0.707106781186548,1.),(1.,0.707106781186547,1.,0.707106781186547,
1.,0.707106781186547,1.,0.707106781186547,1.),(1.,0.707106781186548,1.,
0.707106781186548,1.,0.707106781186548,1.,0.707106781186548,1.),(1.,0.707106781186547,
1.,0.707106781186547,1.,0.707106781186547,1.,0.707106781186547,1.),(1.,
0.707106781186547,1.,0.707106781186547,1.,0.707106781186547,1.,0.707106781186547,
1.),(1.,0.707106781186547,1.,0.707106781186547,1.,0.707106781186547,1.,
0.707106781186547,1.),(1.,0.707106781186547,1.,0.707106781186547,1.,0.707106781186547,
1.,0.707106781186547,1.),(1.,0.707106781186548,1.,0.707106781186548,1.,
0.707106781186548,1.,0.707106781186548,1.),(1.,0.707106781186547,1.,0.707106781186547,
1.,0.707106781186547,1.,0.707106781186547,1.),(1.,0.707106781186547,1.,
0.707106781186547,1.,0.707106781186547,1.,0.707106781186547,1.),(1.,0.707106781186548,
1.,0.707106781186548,1.,0.707106781186548,1.,0.707106781186548,1.),(1.,
0.707106781186548,1.,0.707106781186548,1.,0.707106781186548,1.,0.707106781186548,
1.),(1.,0.707106781186547,1.,0.707106781186547,1.,0.707106781186547,1.,
0.707106781186547,1.),(1.,0.707106781186548,1.,0.707106781186548,1.,0.707106781186548,
1.,0.707106781186548,1.),(1.,0.707106781186547,1.,0.707106781186547,1.,
0.707106781186547,1.,0.707106781186547,1.),(1.,0.707106781186548,1.,0.707106781186548,
1.,0.707106781186548,1.,0.707106781186548,1.),(1.,0.707106781186547,1.,
0.707106781186547,1.,0.707106781186547,1.,0.707106781186547,1.),(1.,0.707106781186547,
1.,0.707106781186547,1.,0.707106781186547,1.,0.707106781186547,1.),(1.,
0.707106781186548,1.,0.707106781186548,1.,0.707106781186548,1.,0.707106781186548,
1.),(1.,0.707106781186547,1.,0.707106781186547,1.,0.707106781186547,1.,
0.707106781186547,1.),(1.,0.707106781186548,1.,0.707106781186548,1.,0.707106781186548,
1.,0.707106781186548,1.),(1.,0.707106781186547,1.,0.707106781186547,1.,
0.707106781186547,1.,0.707106781186547,1.),(1.,0.707106781186548,1.,0.707106781186548,
1.,0.707106781186548,1.,0.707106781186548,1.),(1.,0.707106781186547,1.,
0.707106781186547,1.,0.707106781186547,1.,0.707106781186547,1.),(1.,0.707106781186548,
1.,0.707106781186548,1.,0.707106781186548,1.,0.707106781186548,1.),(1.,
0.707106781186548,1.,0.707106781186548,1.,0.707106781186548,1.,0.707106781186548,
1.),(1.,0.707106781186547,1.,0.707106781186547,1.,0.707106781186547,1.,
0.707106781186547,1.),(1.,0.707106781186548,1.,0.707106781186548,1.,0.707106781186548,
1.,0.707106781186548,1.),(1.,0.707106781186547,1.,0.707106781186547,1.,
0.707106781186547,1.,0.707106781186547,1.),(1.,0.707106781186547,1.,0.707106781186547,
1.,0.707106781186547,1.,0.707106781186547,1.),(1.,0.707106781186548,1.,
0.707106781186548,1.,0.707106781186548,1.,0.707106781186548,1.),(1.,0.707106781186547,
1.,0.707106781186547,1.,0.707106781186547,1.,0.707106781186547,1.),(1.,
0.707106781186547,1.,0.707106781186547,1.,0.707106781186547,1.,0.707106781186547,
1.),(1.,0.707106781186548,1.,0.707106781186548,1.,0.707106781186548,1.,
0.707106781186548,1.),(1.,0.707106781186548,1.,0.707106781186548,1.,0.707106781186548,
1.,0.707106781186548,1.),(1.,0.707106781186548,1.,0.707106781186548,1.,
0.707106781186548,1.,0.707106781186548,1.),(1.,0.707106781186547,1.,0.707106781186547,
1.,0.707106781186547,1.,0.707106781186547,1.),(1.,0.707106781186548,1.,
0.707106781186548,1.,0.707106781186548,1.,0.707106781186548,1.),(1.,0.707106781186547,
1.,0.707106781186547,1.,0.707106781186547,1.,0.707106781186547,1.),(1.,
0.707106781186547,1.,0.707106781186547,1.,0.707106781186547,1.,0.707106781186547,
1.),(1.,0.707106781186547,1.,0.707106781186547,1.,0.707106781186547,1.,
0.707106781186547,1.),(1.,0.707106781186548,1.,0.707106781186548,1.,0.707106781186548,
1.,0.707106781186548,1.),(1.,0.707106781186547,1.,0.707106781186547,1.,
0.707106781186547,1.,0.707106781186547,1.),(1.,0.707106781186548,1.,0.707106781186548,
1.,0.707106781186548,1.,0.707106781186548,1.),(1.,0.707106781186548,1.,
0.707106781186548,1.,0.707106781186548,1.,0.707106781186548,1.),(1.,0.707106781186548,
1.,0.707106781186548,1.,0.707106781186548,1.,0.707106781186548,1.),(1.,
0.707106781186547,1.,0.707106781186547,1.,0.707106781186547,1.,0.707106781186547,
1.),(1.,0.707106781186547,1.,0.707106781186547,1.,0.707106781186547,1.,
0.707106781186547,1.),(1.,0.707106781186547,1.,0.707106781186547,1.,0.707106781186547,
1.,0.707106781186547,1.),(1.,0.707106781186547,1.,0.707106781186547,1.,
0.707106781186547,1.,0.707106781186547,1.),(1.,0.707106781186548,1.,0.707106781186548,
1.,0.707106781186548,1.,0.707106781186548,1.),(1.,0.707106781186547,1.,
0.707106781186547,1.,0.707106781186547,1.,0.707106781186547,1.),(1.,0.707106781186547,
1.,0.707106781186547,1.,0.707106781186547,1.,0.707106781186547,1.),(1.,
0.707106781186548,1.,0.707106781186548,1.,0.707106781186548,1.,0.707106781186548,
1.),(1.,0.707106781186547,1.,0.707106781186547,1.,0.707106781186547,1.,
0.707106781186547,1.),(1.,0.707106781186548,1.,0.707106781186548,1.,0.707106781186548,
1.,0.707106781186548,1.),(1.,0.707106781186547,1.,0.707106781186547,1.,
0.707106781186547,1.,0.707106781186547,1.),(1.,0.707106781186547,1.,0.707106781186547,
1.,0.707106781186547,1.,0.707106781186547,1.),(1.,0.707106781186548,1.,
0.707106781186548,1.,0.707106781186548,1.,0.707106781186548,1.),(1.,0.707106781186547,
1.,0.707106781186547,1.,0.707106781186547,1.,0.707106781186547,1.),(1.,
0.707106781186548,1.,0.707106781186548,1.,0.707106781186548,1.,0.707106781186548,
1.),(1.,0.707106781186547,1.,0.707106781186547,1.,0.707106781186547,1.,
0.707106781186547,1.),(1.,0.707106781186548,1.,0.707106781186548,1.,0.707106781186548,
1.,0.707106781186548,1.),(1.,0.707106781186547,1.,0.707106781186547,1.,
0.707106781186547,1.,0.707106781186547,1.),(1.,0.707106781186547,1.,0.707106781186547,
1.,0.707106781186547,1.,0.707106781186547,1.),(1.,0.707106781186547,1.,
0.707106781186547,1.,0.707106781186547,1.,0.707106781186547,1.),(1.,0.707106781186547,
1.,0.707106781186547,1.,0.707106781186547,1.,0.707106781186547,1.),(1.,
0.707106781186547,1.,0.707106781186547,1.,0.707106781186547,1.,0.707106781186547,
1.),(1.,0.707106781186547,1.,0.707106781186547,1.,0.707106781186547,1.,
0.707106781186547,1.),(1.,0.707106781186548,1.,0.707106781186548,1.,0.707106781186548,
1.,0.707106781186548,1.),(1.,0.707106781186547,1.,0.707106781186547,1.,
0.707106781186547,1.,0.707106781186547,1.),(1.,0.707106781186547,1.,0.707106781186547,
1.,0.707106781186547,1.,0.707106781186547,1.),(1.,0.707106781186548,1.,
0.707106781186548,1.,0.707106781186548,1.,0.707106781186548,1.),(1.,0.707106781186548,
1.,0.707106781186548,1.,0.707106781186548,1.,0.707106781186548,1.),(1.,
0.707106781186547,1.,0.707106781186547,1.,0.707106781186547,1.,0.707106781186547,
1.),(1.,0.707106781186548,1.,0.707106781186548,1.,0.707106781186548,1.,
0.707106781186548,1.),(1.,0.707106781186548,1.,0.707106781186548,1.,0.707106781186548,
1.,0.707106781186548,1.),(1.,0.707106781186547,1.,0.707106781186547,1.,
0.707106781186547,1.,0.707106781186547,1.),(1.,0.707106781186547,1.,0.707106781186547,
1.,0.707106781186547,1.,0.707106781186547,1.),(1.,0.707106781186548,1.,
0.707106781186548,1.,0.707106781186548,1.,0.707106781186548,1.),(1.,0.707106781186547,
1.,0.707106781186547,1.,0.707106781186547,1.,0.707106781186547,1.),(1.,
0.707106781186547,1.,0.707106781186547,1.,0.707106781186547,1.,0.707106781186547,
1.),(1.,0.707106781186548,1.,0.707106781186548,1.,0.707106781186548,1.,
0.707106781186548,1.),(1.,0.707106781186547,1.,0.707106781186547,1.,0.707106781186547,
1.,0.707106781186547,1.),(1.,0.707106781186548,1.,0.707106781186548,1.,
0.707106781186548,1.,0.707106781186548,1.),(1.,0.707106781186548,1.,0.707106781186548,
1.,0.707106781186548,1.,0.707106781186548,1.),(1.,0.707106781186548,1.,
0.707106781186548,1.,0.707106781186548,1.,0.707106781186548,1.),(1.,0.707106781186547,
1.,0.707106781186547,1.,0.707106781186547,1.,0.707106781186547,1.),(1.,
0.707106781186547,1.,0.707106781186547,1.,0.707106781186547,1.,0.707106781186547,
1.),(1.,0.707106781186547,1.,0.707106781186547,1.,0.707106781186547,1.,
0.707106781186547,1.),(1.,0.707106781186547,1.,0.707106781186547,1.,0.707106781186547,
1.,0.707106781186547,1.),(1.,0.707106781186548,1.,0.707106781186548,1.,
0.707106781186548,1.,0.707106781186548,1.),(1.,0.707106781186548,1.,0.707106781186548,
1.,0.707106781186548,1.,0.707106781186548,1.),(1.,0.707106781186548,1.,
0.707106781186548,1.,0.707106781186548,1.,0.707106781186548,1.),(1.,0.707106781186547,
1.,0.707106781186547,1.,0.707106781186547,1.,0.707106781186547,1.),(1.,
0.707106781186548,1.,0.707106781186548,1.,0.707106781186548,1.,0.707106781186548,
1.),(1.,0.707106781186547,1.,0.707106781186547,1.,0.707106781186547,1.,
0.707106781186547,1.),(1.,0.707106781186548,1.,0.707106781186548,1.,0.707106781186548,
1.,0.707106781186548,1.),(1.,0.707106781186548,1.,0.707106781186548,1.,
0.707106781186548,1.,0.707106781186548,1.),(1.,0.707106781186547,1.,0.707106781186547,
1.,0.707106781186547,1.,0.707106781186547,1.),(1.,0.707106781186548,1.,
0.707106781186548,1.,0.707106781186548,1.,0.707106781186548,1.),(1.,0.707106781186547,
1.,0.707106781186547,1.,0.707106781186547,1.,0.707106781186547,1.),(1.,
0.707106781186548,1.,0.707106781186548,1.,0.707106781186548,1.,0.707106781186548,
1.),(1.,0.707106781186548,1.,0.707106781186548,1.,0.707106781186548,1.,
0.707106781186548,1.),(1.,0.707106781186547,1.,0.707106781186547,1.,0.707106781186547,
1.,0.707106781186547,1.),(1.,0.707106781186547,1.,0.707106781186547,1.,
0.707106781186547,1.,0.707106781186547,1.),(1.,0.707106781186548,1.,0.707106781186548,
1.,0.707106781186548,1.,0.707106781186548,1.),(1.,0.707106781186547,1.,
0.707106781186547,1.,0.707106781186547,1.,0.707106781186547,1.),(1.,0.707106781186548,
1.,0.707106781186548,1.,0.707106781186548,1.,0.707106781186548,1.),(1.,
0.707106781186547,1.,0.707106781186547,1.,0.707106781186547,1.,0.707106781186547,
1.),(1.,0.707106781186548,1.,0.707106781186548,1.,0.707106781186548,1.,
0.707106781186548,1.),(1.,0.707106781186548,1.,0.707106781186548,1.,0.707106781186548,
1.,0.707106781186548,1.),(1.,0.707106781186548,1.,0.707106781186548,1.,
0.707106781186548,1.,0.707106781186548,1.),(1.,0.707106781186547,1.,0.707106781186547,
1.,0.707106781186547,1.,0.707106781186547,1.),(1.,0.707106781186548,1.,
0.707106781186548,1.,0.707106781186548,1.,0.707106781186548,1.),(1.,0.707106781186547,
1.,0.707106781186547,1.,0.707106781186547,1.,0.707106781186547,1.),(1.,
0.707106781186547,1.,0.707106781186547,1.,0.707106781186547,1.,0.707106781186547,
1.),(1.,0.707106781186547,1.,0.707106781186547,1.,0.707106781186547,1.,
0.707106781186547,1.),(1.,0.707106781186547,1.,0.707106781186547,1.,0.707106781186547,
1.,0.707106781186547,1.),(1.,0.707106781186548,1.,0.707106781186548,1.,
0.707106781186548,1.,0.707106781186548,1.),(1.,0.707106781186548,1.,0.707106781186548,
1.,0.707106781186548,1.,0.707106781186548,1.),(1.,0.707106781186547,1.,
0.707106781186547,1.,0.707106781186547,1.,0.707106781186547,1.),(1.,0.707106781186547,
1.,0.707106781186547,1.,0.707106781186547,1.,0.707106781186547,1.),(1.,
0.707106781186547,1.,0.707106781186547,1.,0.707106781186547,1.,0.707106781186547,
1.),(1.,0.707106781186548,1.,0.707106781186548,1.,0.707106781186548,1.,
0.707106781186548,1.),(1.,0.707106781186547,1.,0.707106781186547,1.,0.707106781186547,
1.,0.707106781186547,1.),(1.,0.707106781186547,1.,0.707106781186547,1.,
0.707106781186547,1.,0.707106781186547,1.),(1.,0.707106781186548,1.,0.707106781186548,
1.,0.707106781186548,1.,0.707106781186548,1.),(1.,0.707106781186547,1.,
0.707106781186547,1.,0.707106781186547,1.,0.707106781186547,1.),(1.,0.707106781186548,
1.,0.707106781186548,1.,0.707106781186548,1.,0.707106781186548,1.),(1.,
0.707106781186548,1.,0.707106781186548,1.,0.707106781186548,1.,0.707106781186548,
1.),(1.,0.707106781186548,1.,0.707106781186548,1.,0.707106781186548,1.,
0.707106781186548,1.),(1.,0.707106781186547,1.,0.707106781186547,1.,0.707106781186547,
1.,0.707106781186547,1.),(1.,0.707106781186547,1.,0.707106781186547,1.,
0.707106781186547,1.,0.707106781186547,1.),(1.,0.707106781186547,1.,0.707106781186547,
1.,0.707106781186547,1.,0.707106781186547,1.),(1.,0.707106781186547,1.,
0.707106781186547,1.,0.707106781186547,1.,0.707106781186547,1.),(1.,0.707106781186548,
1.,0.707106781186548,1.,0.707106781186548,1.,0.707106781186548,1.),(1.,
0.707106781186548,1.,0.707106781186548,1.,0.707106781186548,1.,0.707106781186548,
1.),(1.,0.707106781186547,1.,0.707106781186547,1.,0.707106781186547,1.,
0.707106781186547,1.),(1.,0.707106781186548,1.,0.707106781186548,1.,0.707106781186548,
1.,0.707106781186548,1.),(1.,0.707106781186547,1.,0.707106781186547,1.,
0.707106781186547,1.,0.707106781186547,1.),(1.,0.707106781186548,1.,0.707106781186548,
1.,0.707106781186548,1.,0.707106781186548,1.),(1.,0.707106781186548,1.,
0.707106781186548,1.,0.707106781186548,1.,0.707106781186548,1.),(1.,0.707106781186547,
1.,0.707106781186547,1.,0.707106781186547,1.,0.707106781186547,1.),(1.,
0.707106781186548,1.,0.707106781186548,1.,0.707106781186548,1.,0.707106781186548,
1.),(1.,0.707106781186547,1.,0.707106781186547,1.,0.707106781186547,1.,
0.707106781186547,1.),(1.,0.707106781186548,1.,0.707106781186548,1.,0.707106781186548,
1.,0.707106781186548,1.),(1.,0.707106781186547,1.,0.707106781186547,1.,
0.707106781186547,1.,0.707106781186547,1.),(1.,0.707106781186547,1.,0.707106781186547,
1.,0.707106781186547,1.,0.707106781186547,1.),(1.,0.707106781186547,1.,
0.707106781186547,1.,0.707106781186547,1.,0.707106781186547,1.),(1.,0.707106781186548,
1.,0.707106781186548,1.,0.707106781186548,1.,0.707106781186548,1.),(1.,
0.707106781186547,1.,0.707106781186547,1.,0.707106781186547,1.,0.707106781186547,
1.),(1.,0.707106781186548,1.,0.707106781186548,1.,0.707106781186548,1.,
0.707106781186548,1.),(1.,0.707106781186547,1.,0.707106781186547,1.,0.707106781186547,
1.,0.707106781186547,1.),(1.,0.707106781186548,1.,0.707106781186548,1.,
0.707106781186548,1.,0.707106781186548,1.),(1.,0.707106781186547,1.,0.707106781186547,
1.,0.707106781186547,1.,0.707106781186547,1.),(1.,0.707106781186548,1.,
0.707106781186548,1.,0.707106781186548,1.,0.707106781186548,1.),(1.,0.707106781186547,
1.,0.707106781186547,1.,0.707106781186547,1.,0.707106781186547,1.),(1.,
0.707106781186548,1.,0.707106781186548,1.,0.707106781186548,1.,0.707106781186548,
1.),(1.,0.707106781186547,1.,0.707106781186547,1.,0.707106781186547,1.,
0.707106781186547,1.),(1.,0.707106781186547,1.,0.707106781186547,1.,0.707106781186547,
1.,0.707106781186547,1.),(1.,0.707106781186548,1.,0.707106781186548,1.,
0.707106781186548,1.,0.707106781186548,1.),(1.,0.707106781186547,1.,0.707106781186547,
1.,0.707106781186547,1.,0.707106781186547,1.),(1.,0.707106781186548,1.,
0.707106781186548,1.,0.707106781186548,1.,0.707106781186548,1.),(1.,0.707106781186547,
1.,0.707106781186547,1.,0.707106781186547,1.,0.707106781186547,1.),(1.,
0.707106781186547,1.,0.707106781186547,1.,0.707106781186547,1.,0.707106781186547,
1.),(1.,0.707106781186548,1.,0.707106781186548,1.,0.707106781186548,1.,
0.707106781186548,1.),(1.,0.707106781186548,1.,0.707106781186548,1.,0.707106781186548,
1.,0.707106781186548,1.),(1.,0.707106781186547,1.,0.707106781186547,1.,
0.707106781186547,1.,0.707106781186547,1.),(1.,0.707106781186548,1.,0.707106781186548,
1.,0.707106781186548,1.,0.707106781186548,1.),(1.,0.707106781186548,1.,
0.707106781186548,1.,0.707106781186548,1.,0.707106781186548,1.),(1.,0.707106781186547,
1.,0.707106781186547,1.,0.707106781186547,1.,0.707106781186547,1.),(1.,
0.707106781186548,1.,0.707106781186548,1.,0.707106781186548,1.,0.707106781186548,
1.),(1.,0.707106781186547,1.,0.707106781186547,1.,0.707106781186547,1.,
0.707106781186547,1.),(1.,0.707106781186548,1.,0.707106781186548,1.,0.707106781186548,
1.,0.707106781186548,1.),(1.,0.707106781186547,1.,0.707106781186547,1.,
0.707106781186547,1.,0.707106781186547,1.),(1.,0.707106781186547,1.,0.707106781186547,
1.,0.707106781186547,1.,0.707106781186547,1.),(1.,0.707106781186547,1.,
0.707106781186547,1.,0.707106781186547,1.,0.707106781186547,1.),(1.,0.707106781186548,
1.,0.707106781186548,1.,0.707106781186548,1.,0.707106781186548,1.),(1.,
0.707106781186547,1.,0.707106781186547,1.,0.707106781186547,1.,0.707106781186547,
1.),(1.,0.707106781186547,1.,0.707106781186547,1.,0.707106781186547,1.,
0.707106781186547,1.),(1.,0.707106781186548,1.,0.707106781186548,1.,0.707106781186548,
1.,0.707106781186548,1.),(1.,0.707106781186547,1.,0.707106781186547,1.,
0.707106781186547,1.,0.707106781186547,1.),(1.,0.707106781186548,1.,0.707106781186548,
1.,0.707106781186548,1.,0.707106781186548,1.),(1.,0.707106781186547,1.,
0.707106781186547,1.,0.707106781186547,1.,0.707106781186547,1.),(1.,0.707106781186548,
1.,0.707106781186548,1.,0.707106781186548,1.,0.707106781186548,1.),(1.,
0.707106781186548,1.,0.707106781186548,1.,0.707106781186548,1.,0.707106781186548,
1.),(1.,0.707106781186547,1.,0.707106781186547,1.,0.707106781186547,1.,
0.707106781186547,1.),(1.,0.707106781186548,1.,0.707106781186548,1.,0.707106781186548,
1.,0.707106781186548,1.),(1.,0.707106781186547,1.,0.707106781186547,1.,
0.707106781186547,1.,0.707106781186547,1.),(1.,0.707106781186548,1.,0.707106781186548,
1.,0.707106781186548,1.,0.707106781186548,1.),(1.,0.707106781186548,1.,
0.707106781186548,1.,0.707106781186548,1.,0.707106781186548,1.),(1.,0.707106781186548,
1.,0.707106781186548,1.,0.707106781186548,1.,0.707106781186548,1.),(1.,
0.707106781186548,1.,0.707106781186548,1.,0.707106781186548,1.,0.707106781186548,
1.),(1.,0.707106781186547,1.,0.707106781186547,1.,0.707106781186547,1.,
0.707106781186547,1.),(1.,0.707106781186547,1.,0.707106781186547,1.,0.707106781186547,
1.,0.707106781186547,1.),(1.,0.707106781186548,1.,0.707106781186548,1.,
0.707106781186548,1.,0.707106781186548,1.),(1.,0.707106781186547,1.,0.707106781186547,
1.,0.707106781186547,1.,0.707106781186547,1.),(1.,0.707106781186547,1.,
0.707106781186547,1.,0.707106781186547,1.,0.707106781186547,1.),(1.,0.707106781186548,
1.,0.707106781186548,1.,0.707106781186548,1.,0.707106781186548,1.),(1.,
0.707106781186548,1.,0.707106781186548,1.,0.707106781186548,1.,0.707106781186548,
1.),(1.,0.707106781186547,1.,0.707106781186547,1.,0.707106781186547,1.,
0.707106781186547,1.),(1.,0.707106781186547,1.,0.707106781186547,1.,0.707106781186547,
1.,0.707106781186547,1.),(1.,0.707106781186548,1.,0.707106781186548,1.,
0.707106781186548,1.,0.707106781186548,1.),(1.,0.707106781186547,1.,0.707106781186547,
1.,0.707106781186547,1.,0.707106781186547,1.),(1.,0.707106781186547,1.,
0.707106781186547,1.,0.707106781186547,1.,0.707106781186547,1.),(1.,0.707106781186548,
1.,0.707106781186548,1.,0.707106781186548,1.,0.707106781186548,1.),(1.,
0.707106781186547,1.,0.707106781186547,1.,0.707106781186547,1.,0.707106781186547,
1.),(1.,0.707106781186548,1.,0.707106781186548,1.,0.707106781186548,1.,
0.707106781186548,1.),(1.,0.707106781186547,1.,0.707106781186547,1.,0.707106781186547,
1.,0.707106781186547,1.),(1.,0.707106781186548,1.,0.707106781186548,1.,
0.707106781186548,1.,0.707106781186548,1.),(1.,0.707106781186547,1.,0.707106781186547,
1.,0.707106781186547,1.,0.707106781186547,1.),(1.,0.707106781186547,1.,
0.707106781186547,1.,0.707106781186547,1.,0.707106781186547,1.),(1.,0.707106781186547,
1.,0.707106781186547,1.,0.707106781186547,1.,0.707106781186547,1.),(1.,
0.707106781186548,1.,0.707106781186548,1.,0.707106781186548,1.,0.707106781186548,
1.),(1.,0.707106781186547,1.,0.707106781186547,1.,0.707106781186547,1.,
0.707106781186547,1.),(1.,0.707106781186547,1.,0.707106781186547,1.,0.707106781186547,
1.,0.707106781186547,1.),(1.,0.707106781186548,1.,0.707106781186548,1.,
0.707106781186548,1.,0.707106781186548,1.),(1.,0.707106781186547,1.,0.707106781186547,
1.,0.707106781186547,1.,0.707106781186547,1.),(1.,0.707106781186548,1.,
0.707106781186548,1.,0.707106781186548,1.,0.707106781186548,1.),(1.,0.707106781186548,
1.,0.707106781186548,1.,0.707106781186548,1.,0.707106781186548,1.),(1.,
0.707106781186548,1.,0.707106781186548,1.,0.707106781186548,1.,0.707106781186548,
1.),(1.,0.707106781186547,1.,0.707106781186547,1.,0.707106781186547,1.,
0.707106781186547,1.),(1.,0.707106781186547,1.,0.707106781186547,1.,0.707106781186547,
1.,0.707106781186547,1.),(1.,0.707106781186547,1.,0.707106781186547,1.,
0.707106781186547,1.,0.707106781186547,1.),(1.,0.707106781186548,1.,0.707106781186548,
1.,0.707106781186548,1.,0.707106781186548,1.),(1.,0.707106781186548,1.,
0.707106781186548,1.,0.707106781186548,1.,0.707106781186548,1.),(1.,0.707106781186547,
1.,0.707106781186547,1.,0.707106781186547,1.,0.707106781186547,1.),(1.,
0.707106781186547,1.,0.707106781186547,1.,0.707106781186547,1.,0.707106781186547,
1.),(1.,0.707106781186547,1.,0.707106781186547,1.,0.707106781186547,1.,
0.707106781186547,1.),(1.,0.707106781186547,1.,0.707106781186547,1.,0.707106781186547,
1.,0.707106781186547,1.),(1.,0.707106781186548,1.,0.707106781186548,1.,
0.707106781186548,1.,0.707106781186548,1.),(1.,0.707106781186548,1.,0.707106781186548,
1.,0.707106781186548,1.,0.707106781186548,1.),(1.,0.707106781186547,1.,
0.707106781186547,1.,0.707106781186547,1.,0.707106781186547,1.),(1.,0.707106781186547,
1.,0.707106781186547,1.,0.707106781186547,1.,0.707106781186547,1.),(1.,
0.707106781186547,1.,0.707106781186547,1.,0.707106781186547,1.,0.707106781186547,
1.),(1.,0.707106781186548,1.,0.707106781186548,1.,0.707106781186548,1.,
0.707106781186548,1.),(1.,0.707106781186548,1.,0.707106781186548,1.,0.707106781186548,
1.,0.707106781186548,1.),(1.,0.707106781186547,1.,0.707106781186547,1.,
0.707106781186547,1.,0.707106781186547,1.),(1.,0.707106781186548,1.,0.707106781186548,
1.,0.707106781186548,1.,0.707106781186548,1.),(1.,0.707106781186547,1.,
0.707106781186547,1.,0.707106781186547,1.,0.707106781186547,1.),(1.,0.707106781186548,
1.,0.707106781186548,1.,0.707106781186548,1.,0.707106781186548,1.),(1.,
0.707106781186547,1.,0.707106781186547,1.,0.707106781186547,1.,0.707106781186547,
1.),(1.,0.707106781186548,1.,0.707106781186548,1.,0.707106781186548,1.,
0.707106781186548,1.),(1.,0.707106781186548,1.,0.707106781186548,1.,0.707106781186548,
1.,0.707106781186548,1.),(1.,0.707106781186547,1.,0.707106781186547,1.,
0.707106781186547,1.,0.707106781186547,1.),(1.,0.707106781186548,1.,0.707106781186548,
1.,0.707106781186548,1.,0.707106781186548,1.),(1.,0.707106781186548,1.,
0.707106781186548,1.,0.707106781186548,1.,0.707106781186548,1.),(1.,0.707106781186548,
1.,0.707106781186548,1.,0.707106781186548,1.,0.707106781186548,1.),(1.,
0.707106781186547,1.,0.707106781186547,1.,0.707106781186547,1.,0.707106781186547,
1.),(1.,0.707106781186547,1.,0.707106781186547,1.,0.707106781186547,1.,
0.707106781186547,1.),(1.,0.707106781186547,1.,0.707106781186547,1.,0.707106781186547,
1.,0.707106781186547,1.),(1.,0.707106781186548,1.,0.707106781186548,1.,
0.707106781186548,1.,0.707106781186548,1.),(1.,0.707106781186548,1.,0.707106781186548,
1.,0.707106781186548,1.,0.707106781186548,1.),(1.,0.707106781186548,1.,
0.707106781186548,1.,0.707106781186548,1.,0.707106781186548,1.),(1.,0.707106781186547,
1.,0.707106781186547,1.,0.707106781186547,1.,0.707106781186547,1.),(1.,
0.707106781186547,1.,0.707106781186547,1.,0.707106781186547,1.,0.707106781186547,
1.),(1.,0.707106781186548,1.,0.707106781186548,1.,0.707106781186548,1.,
0.707106781186548,1.),(1.,0.707106781186548,1.,0.707106781186548,1.,0.707106781186548,
1.,0.707106781186548,1.),(1.,0.707106781186547,1.,0.707106781186547,1.,
0.707106781186547,1.,0.707106781186547,1.),(1.,0.707106781186548,1.,0.707106781186548,
1.,0.707106781186548,1.,0.707106781186548,1.),(1.,0.707106781186547,1.,
0.707106781186547,1.,0.707106781186547,1.,0.707106781186547,1.),(1.,0.707106781186547,
1.,0.707106781186547,1.,0.707106781186547,1.,0.707106781186547,1.),(1.,
0.707106781186548,1.,0.707106781186548,1.,0.707106781186548,1.,0.707106781186548,
1.),(1.,0.707106781186547,1.,0.707106781186547,1.,0.707106781186547,1.,
0.707106781186547,1.),(1.,0.707106781186548,1.,0.707106781186548,1.,0.707106781186548,
1.,0.707106781186548,1.),(1.,0.707106781186547,1.,0.707106781186547,1.,
0.707106781186547,1.,0.707106781186547,1.),(1.,0.707106781186547,1.,0.707106781186547,
1.,0.707106781186547,1.,0.707106781186547,1.),(1.,0.707106781186548,1.,
0.707106781186548,1.,0.707106781186548,1.,0.707106781186548,1.),(1.,0.707106781186547,
1.,0.707106781186547,1.,0.707106781186547,1.,0.707106781186547,1.),(1.,
0.707106781186548,1.,0.707106781186548,1.,0.707106781186548,1.,0.707106781186548,
1.),(1.,0.707106781186548,1.,0.707106781186548,1.,0.707106781186548,1.,
0.707106781186548,1.),(1.,0.707106781186547,1.,0.707106781186547,1.,0.707106781186547,
1.,0.707106781186547,1.),(1.,0.707106781186547,1.,0.707106781186547,1.,
0.707106781186547,1.,0.707106781186547,1.),(1.,0.707106781186548,1.,0.707106781186548,
1.,0.707106781186548,1.,0.707106781186548,1.),(1.,0.707106781186547,1.,
0.707106781186547,1.,0.707106781186547,1.,0.707106781186547,1.),(1.,0.707106781186548,
1.,0.707106781186548,1.,0.707106781186548,1.,0.707106781186548,1.),(1.,
0.707106781186547,1.,0.707106781186547,1.,0.707106781186547,1.,0.707106781186547,
1.),(1.,0.707106781186547,1.,0.707106781186547,1.,0.707106781186547,1.,
0.707106781186547,1.),(1.,0.707106781186548,1.,0.707106781186548,1.,0.707106781186548,
1.,0.707106781186548,1.),(1.,0.707106781186547,1.,0.707106781186547,1.,
0.707106781186547,1.,0.707106781186547,1.),(1.,0.707106781186548,1.,0.707106781186548,
1.,0.707106781186548,1.,0.707106781186548,1.),(1.,0.707106781186547,1.,
0.707106781186547,1.,0.707106781186547,1.,0.707106781186547,1.),(1.,0.707106781186548,
1.,0.707106781186548,1.,0.707106781186548,1.,0.707106781186548,1.),(1.,
0.707106781186547,1.,0.707106781186547,1.,0.707106781186547,1.,0.707106781186547,
1.),(1.,0.707106781186547,1.,0.707106781186547,1.,0.707106781186547,1.,
0.707106781186547,1.),(1.,0.707106781186548,1.,0.707106781186548,1.,0.707106781186548,
1.,0.707106781186548,1.),(1.,0.707106781186547,1.,0.707106781186547,1.,
0.707106781186547,1.,0.707106781186547,1.),(1.,0.707106781186547,1.,0.707106781186547,
1.,0.707106781186547,1.,0.707106781186547,1.),(1.,0.707106781186547,1.,
0.707106781186547,1.,0.707106781186547,1.,0.707106781186547,1.),(1.,0.707106781186547,
1.,0.707106781186547,1.,0.707106781186547,1.,0.707106781186547,1.),(1.,
0.707106781186547,1.,0.707106781186547,1.,0.707106781186547,1.,0.707106781186547,
1.),(1.,0.707106781186547,1.,0.707106781186547,1.,0.707106781186547,1.,
0.707106781186547,1.),(1.,0.707106781186548,1.,0.707106781186548,1.,0.707106781186548,
1.,0.707106781186548,1.),(1.,0.707106781186547,1.,0.707106781186547,1.,
0.707106781186547,1.,0.707106781186547,1.),(1.,0.707106781186548,1.,0.707106781186548,
1.,0.707106781186548,1.,0.707106781186548,1.),(1.,0.707106781186548,1.,
0.707106781186548,1.,0.707106781186548,1.,0.707106781186548,1.),(1.,0.707106781186548,
1.,0.707106781186548,1.,0.707106781186548,1.,0.707106781186548,1.),(1.,
0.707106781186547,1.,0.707106781186547,1.,0.707106781186547,1.,0.707106781186547,
1.),(1.,0.707106781186547,1.,0.707106781186547,1.,0.707106781186547,1.,
0.707106781186547,1.),(1.,0.707106781186547,1.,0.707106781186547,1.,0.707106781186547,
1.,0.707106781186547,1.),(1.,0.707106781186548,1.,0.707106781186548,1.,
0.707106781186548,1.,0.707106781186548,1.),(1.,0.707106781186547,1.,0.707106781186547,
1.,0.707106781186547,1.,0.707106781186547,1.),(1.,0.707106781186548,1.,
0.707106781186548,1.,0.707106781186548,1.,0.707106781186548,1.),(1.,0.707106781186547,
1.,0.707106781186547,1.,0.707106781186547,1.,0.707106781186547,1.),(1.,
0.707106781186547,1.,0.707106781186547,1.,0.707106781186547,1.,0.707106781186547,
1.),(1.,0.707106781186548,1.,0.707106781186548,1.,0.707106781186548,1.,
0.707106781186548,1.),(1.,0.707106781186547,1.,0.707106781186547,1.,0.707106781186547,
1.,0.707106781186547,1.),(1.,0.707106781186547,1.,0.707106781186547,1.,
0.707106781186547,1.,0.707106781186547,1.),(1.,0.707106781186547,1.,0.707106781186547,
1.,0.707106781186547,1.,0.707106781186547,1.),(1.,0.707106781186547,1.,
0.707106781186547,1.,0.707106781186547,1.,0.707106781186547,1.),(1.,0.707106781186547,
1.,0.707106781186547,1.,0.707106781186547,1.,0.707106781186547,1.),(1.,
0.707106781186548,1.,0.707106781186548,1.,0.707106781186548,1.,0.707106781186548,
1.),(1.,0.707106781186547,1.,0.707106781186547,1.,0.707106781186547,1.,
0.707106781186547,1.),(1.,0.707106781186548,1.,0.707106781186548,1.,0.707106781186548,
1.,0.707106781186548,1.),(1.,0.707106781186547,1.,0.707106781186547,1.,
0.707106781186547,1.,0.707106781186547,1.),(1.,0.707106781186547,1.,0.707106781186547,
1.,0.707106781186547,1.,0.707106781186547,1.),(1.,0.707106781186548,1.,
0.707106781186548,1.,0.707106781186548,1.,0.707106781186548,1.),(1.,0.707106781186548,
1.,0.707106781186548,1.,0.707106781186548,1.,0.707106781186548,1.),(1.,
0.707106781186547,1.,0.707106781186547,1.,0.707106781186547,1.,0.707106781186547,
1.),(1.,0.707106781186547,1.,0.707106781186547,1.,0.707106781186547,1.,
0.707106781186547,1.),(1.,0.707106781186547,1.,0.707106781186547,1.,0.707106781186547,
1.,0.707106781186547,1.),(1.,0.707106781186548,1.,0.707106781186548,1.,
0.707106781186548,1.,0.707106781186548,1.),(1.,0.707106781186547,1.,0.707106781186547,
1.,0.707106781186547,1.,0.707106781186547,1.),(1.,0.707106781186547,1.,
0.707106781186547,1.,0.707106781186547,1.,0.707106781186547,1.),(1.,0.707106781186548,
1.,0.707106781186548,1.,0.707106781186548,1.,0.707106781186548,1.),(1.,
0.707106781186548,1.,0.707106781186548,1.,0.707106781186548,1.,0.707106781186548,
1.),(1.,0.707106781186547,1.,0.707106781186547,1.,0.707106781186547,1.,
0.707106781186547,1.),(1.,0.707106781186548,1.,0.707106781186548,1.,0.707106781186548,
1.,0.707106781186548,1.),(1.,0.707106781186547,1.,0.707106781186547,1.,
0.707106781186547,1.,0.707106781186547,1.),(1.,0.707106781186548,1.,0.707106781186548,
1.,0.707106781186548,1.,0.707106781186548,1.),(1.,0.707106781186548,1.,
0.707106781186548,1.,0.707106781186548,1.,0.707106781186548,1.),(1.,0.707106781186547,
1.,0.707106781186547,1.,0.707106781186547,1.,0.707106781186547,1.),(1.,
0.707106781186547,1.,0.707106781186547,1.,0.707106781186547,1.,0.707106781186547,
1.),(1.,0.707106781186547,1.,0.707106781186547,1.,0.707106781186547,1.,
0.707106781186547,1.),(1.,0.707106781186548,1.,0.707106781186548,1.,0.707106781186548,
1.,0.707106781186548,1.),(1.,0.707106781186548,1.,0.707106781186548,1.,
0.707106781186548,1.,0.707106781186548,1.),(1.,0.707106781186547,1.,0.707106781186547,
1.,0.707106781186547,1.,0.707106781186547,1.),(1.,0.707106781186548,1.,
0.707106781186548,1.,0.707106781186548,1.,0.707106781186548,1.),(1.,0.707106781186547,
1.,0.707106781186547,1.,0.707106781186547,1.,0.707106781186547,1.),(1.,
0.707106781186548,1.,0.707106781186548,1.,0.707106781186548,1.,0.707106781186548,
1.),(1.,0.707106781186548,1.,0.707106781186548,1.,0.707106781186548,1.,
0.707106781186548,1.),(1.,0.707106781186547,1.,0.707106781186547,1.,0.707106781186547,
1.,0.707106781186547,1.),(1.,0.707106781186548,1.,0.707106781186548,1.,
0.707106781186548,1.,0.707106781186548,1.),(1.,0.707106781186547,1.,0.707106781186547,
1.,0.707106781186547,1.,0.707106781186547,1.),(1.,0.707106781186547,1.,
0.707106781186547,1.,0.707106781186547,1.,0.707106781186547,1.),(1.,0.707106781186547,
1.,0.707106781186547,1.,0.707106781186547,1.,0.707106781186547,1.),(1.,
0.707106781186548,1.,0.707106781186548,1.,0.707106781186548,1.,0.707106781186548,
1.),(1.,0.707106781186547,1.,0.707106781186547,1.,0.707106781186547,1.,
0.707106781186547,1.),(1.,0.707106781186548,1.,0.707106781186548,1.,0.707106781186548,
1.,0.707106781186548,1.),(1.,0.707106781186547,1.,0.707106781186547,1.,
0.707106781186547,1.,0.707106781186547,1.),(1.,0.707106781186548,1.,0.707106781186548,
1.,0.707106781186548,1.,0.707106781186548,1.),(1.,0.707106781186547,1.,
0.707106781186547,1.,0.707106781186547,1.,0.707106781186547,1.),(1.,0.707106781186547,
1.,0.707106781186547,1.,0.707106781186547,1.,0.707106781186547,1.),(1.,
0.707106781186547,1.,0.707106781186547,1.,0.707106781186547,1.,0.707106781186547,
1.),(1.,0.707106781186547,1.,0.707106781186547,1.,0.707106781186547,1.,
0.707106781186547,1.),(1.,0.707106781186547,1.,0.707106781186547,1.,0.707106781186547,
1.,0.707106781186547,1.),(1.,0.707106781186548,1.,0.707106781186548,1.,
0.707106781186548,1.,0.707106781186548,1.),(1.,0.707106781186547,1.,0.707106781186547,
1.,0.707106781186547,1.,0.707106781186547,1.),(1.,0.707106781186548,1.,
0.707106781186548,1.,0.707106781186548,1.,0.707106781186548,1.),(1.,0.707106781186547,
1.,0.707106781186547,1.,0.707106781186547,1.,0.707106781186547,1.),(1.,
0.707106781186548,1.,0.707106781186548,1.,0.707106781186548,1.,0.707106781186548,
1.),(1.,0.707106781186547,1.,0.707106781186547,1.,0.707106781186547,1.,
0.707106781186547,1.),(1.,0.707106781186548,1.,0.707106781186548,1.,0.707106781186548,
1.,0.707106781186548,1.),(1.,0.707106781186547,1.,0.707106781186547,1.,
0.707106781186547,1.,0.707106781186547,1.),(1.,0.707106781186547,1.,0.707106781186547,
1.,0.707106781186547,1.,0.707106781186547,1.),(1.,0.707106781186547,1.,
0.707106781186547,1.,0.707106781186547,1.,0.707106781186547,1.),(1.,0.707106781186547,
1.,0.707106781186547,1.,0.707106781186547,1.,0.707106781186547,1.),(1.,
0.707106781186547,1.,0.707106781186547,1.,0.707106781186547,1.,0.707106781186547,
1.),(1.,0.707106781186548,1.,0.707106781186548,1.,0.707106781186548,1.,
0.707106781186548,1.),(1.,0.707106781186548,1.,0.707106781186548,1.,0.707106781186548,
1.,0.707106781186548,1.),(1.,0.707106781186548,1.,0.707106781186548,1.,
0.707106781186548,1.,0.707106781186548,1.),(1.,0.707106781186547,1.,0.707106781186547,
1.,0.707106781186547,1.,0.707106781186547,1.),(1.,0.707106781186548,1.,
0.707106781186548,1.,0.707106781186548,1.,0.707106781186548,1.),(1.,0.707106781186547,
1.,0.707106781186547,1.,0.707106781186547,1.,0.707106781186547,1.),(1.,
0.707106781186548,1.,0.707106781186548,1.,0.707106781186548,1.,0.707106781186548,
1.),(1.,0.707106781186547,1.,0.707106781186547,1.,0.707106781186547,1.,
0.707106781186547,1.),(1.,0.707106781186547,1.,0.707106781186547,1.,0.707106781186547,
1.,0.707106781186547,1.),(1.,0.707106781186548,1.,0.707106781186548,1.,
0.707106781186548,1.,0.707106781186548,1.),(1.,0.707106781186547,1.,0.707106781186547,
1.,0.707106781186547,1.,0.707106781186547,1.),(1.,0.707106781186548,1.,
0.707106781186548,1.,0.707106781186548,1.,0.707106781186548,1.),(1.,0.707106781186547,
1.,0.707106781186547,1.,0.707106781186547,1.,0.707106781186547,1.),(1.,
0.707106781186547,1.,0.707106781186547,1.,0.707106781186547,1.,0.707106781186547,
1.),(1.,0.707106781186547,1.,0.707106781186547,1.,0.707106781186547,1.,
0.707106781186547,1.),(1.,0.707106781186548,1.,0.707106781186548,1.,0.707106781186548,
1.,0.707106781186548,1.),(1.,0.707106781186548,1.,0.707106781186548,1.,
0.707106781186548,1.,0.707106781186548,1.),(1.,0.707106781186547,1.,0.707106781186547,
1.,0.707106781186547,1.,0.707106781186547,1.),(1.,0.707106781186548,1.,
0.707106781186548,1.,0.707106781186548,1.,0.707106781186548,1.),(1.,0.707106781186547,
1.,0.707106781186547,1.,0.707106781186547,1.,0.707106781186547,1.),(1.,
0.707106781186548,1.,0.707106781186548,1.,0.707106781186548,1.,0.707106781186548,
1.),(1.,0.707106781186548,1.,0.707106781186548,1.,0.707106781186548,1.,
0.707106781186548,1.),(1.,0.707106781186547,1.,0.707106781186547,1.,0.707106781186547,
1.,0.707106781186547,1.),(1.,0.707106781186548,1.,0.707106781186548,1.,
0.707106781186548,1.,0.707106781186548,1.),(1.,0.707106781186547,1.,0.707106781186547,
1.,0.707106781186547,1.,0.707106781186547,1.),(1.,0.707106781186548,1.,
0.707106781186548,1.,0.707106781186548,1.,0.707106781186548,1.),(1.,0.707106781186548,
1.,0.707106781186548,1.,0.707106781186548,1.,0.707106781186548,1.),(1.,
0.707106781186547,1.,0.707106781186547,1.,0.707106781186547,1.,0.707106781186547,
1.),(1.,0.707106781186547,1.,0.707106781186547,1.,0.707106781186547,1.,
0.707106781186547,1.),(1.,0.707106781186547,1.,0.707106781186547,1.,0.707106781186547,
1.,0.707106781186547,1.),(1.,0.707106781186547,1.,0.707106781186547,1.,
0.707106781186547,1.,0.707106781186547,1.),(1.,0.707106781186547,1.,0.707106781186547,
1.,0.707106781186547,1.,0.707106781186547,1.),(1.,0.707106781186547,1.,
0.707106781186547,1.,0.707106781186547,1.,0.707106781186547,1.),(1.,0.707106781186548,
1.,0.707106781186548,1.,0.707106781186548,1.,0.707106781186548,1.),(1.,
0.707106781186548,1.,0.707106781186548,1.,0.707106781186548,1.,0.707106781186548,
1.),(1.,0.707106781186547,1.,0.707106781186547,1.,0.707106781186547,1.,
0.707106781186547,1.),(1.,0.707106781186548,1.,0.707106781186548,1.,0.707106781186548,
1.,0.707106781186548,1.),(1.,0.707106781186547,1.,0.707106781186547,1.,
0.707106781186547,1.,0.707106781186547,1.),(1.,0.707106781186547,1.,0.707106781186547,
1.,0.707106781186547,1.,0.707106781186547,1.),(1.,0.707106781186548,1.,
0.707106781186548,1.,0.707106781186548,1.,0.707106781186548,1.),(1.,0.707106781186547,
1.,0.707106781186547,1.,0.707106781186547,1.,0.707106781186547,1.),(1.,
0.707106781186547,1.,0.707106781186547,1.,0.707106781186547,1.,0.707106781186547,
1.),(1.,0.707106781186548,1.,0.707106781186548,1.,0.707106781186548,1.,
0.707106781186548,1.),(1.,0.707106781186547,1.,0.707106781186547,1.,0.707106781186547,
1.,0.707106781186547,1.),(1.,0.707106781186547,1.,0.707106781186547,1.,
0.707106781186547,1.,0.707106781186547,1.),(1.,0.707106781186547,1.,0.707106781186547,
1.,0.707106781186547,1.,0.707106781186547,1.),(1.,0.707106781186548,1.,
0.707106781186548,1.,0.707106781186548,1.,0.707106781186548,1.),(1.,0.707106781186547,
1.,0.707106781186547,1.,0.707106781186547,1.,0.707106781186547,1.),(1.,
0.707106781186547,1.,0.707106781186547,1.,0.707106781186547,1.,0.707106781186547,
1.),(1.,0.707106781186548,1.,0.707106781186548,1.,0.707106781186548,1.,
0.707106781186548,1.),(1.,0.707106781186547,1.,0.707106781186547,1.,0.707106781186547,
1.,0.707106781186547,1.),(1.,0.707106781186548,1.,0.707106781186548,1.,
0.707106781186548,1.,0.707106781186548,1.),(1.,0.707106781186548,1.,0.707106781186548,
1.,0.707106781186548,1.,0.707106781186548,1.),(1.,0.707106781186547,1.,
0.707106781186547,1.,0.707106781186547,1.,0.707106781186547,1.),(1.,0.707106781186547,
1.,0.707106781186547,1.,0.707106781186547,1.,0.707106781186547,1.),(1.,
0.707106781186547,1.,0.707106781186547,1.,0.707106781186547,1.,0.707106781186547,
1.),(1.,0.707106781186548,1.,0.707106781186548,1.,0.707106781186548,1.,
0.707106781186548,1.),(1.,0.707106781186547,1.,0.707106781186547,1.,0.707106781186547,
1.,0.707106781186547,1.),(1.,0.707106781186547,1.,0.707106781186547,1.,
0.707106781186547,1.,0.707106781186547,1.),(1.,0.707106781186548,1.,0.707106781186548,
1.,0.707106781186548,1.,0.707106781186548,1.),(1.,0.707106781186548,1.,
0.707106781186548,1.,0.707106781186548,1.,0.707106781186548,1.),(1.,0.707106781186548,
1.,0.707106781186548,1.,0.707106781186548,1.,0.707106781186548,1.),(1.,
0.707106781186548,1.,0.707106781186548,1.,0.707106781186548,1.,0.707106781186548,
1.),(1.,0.707106781186547,1.,0.707106781186547,1.,0.707106781186547,1.,
0.707106781186547,1.),(1.,0.707106781186548,1.,0.707106781186548,1.,0.707106781186548,
1.,0.707106781186548,1.),(1.,0.707106781186548,1.,0.707106781186548,1.,
0.707106781186548,1.,0.707106781186548,1.),(1.,0.707106781186547,1.,0.707106781186547,
1.,0.707106781186547,1.,0.707106781186547,1.),(1.,0.707106781186547,1.,
0.707106781186547,1.,0.707106781186547,1.,0.707106781186547,1.),(1.,0.707106781186548,
1.,0.707106781186548,1.,0.707106781186548,1.,0.707106781186548,1.),(1.,
0.707106781186547,1.,0.707106781186547,1.,0.707106781186547,1.,0.707106781186547,
1.),(1.,0.707106781186548,1.,0.707106781186548,1.,0.707106781186548,1.,
0.707106781186548,1.),(1.,0.707106781186547,1.,0.707106781186547,1.,0.707106781186547,
1.,0.707106781186547,1.),(1.,0.707106781186547,1.,0.707106781186547,1.,
0.707106781186547,1.,0.707106781186547,1.),(1.,0.707106781186548,1.,0.707106781186548,
1.,0.707106781186548,1.,0.707106781186548,1.),(1.,0.707106781186547,1.,
0.707106781186547,1.,0.707106781186547,1.,0.707106781186547,1.),(1.,0.707106781186547,
1.,0.707106781186547,1.,0.707106781186547,1.,0.707106781186547,1.),(1.,
0.707106781186548,1.,0.707106781186548,1.,0.707106781186548,1.,0.707106781186548,
1.),(1.,0.707106781186547,1.,0.707106781186547,1.,0.707106781186547,1.,
0.707106781186547,1.),(1.,0.707106781186548,1.,0.707106781186548,1.,0.707106781186548,
1.,0.707106781186548,1.),(1.,0.707106781186547,1.,0.707106781186547,1.,
0.707106781186547,1.,0.707106781186547,1.),(1.,0.707106781186548,1.,0.707106781186548,
1.,0.707106781186548,1.,0.707106781186548,1.),(1.,0.707106781186547,1.,
0.707106781186547,1.,0.707106781186547,1.,0.707106781186547,1.),(1.,0.707106781186548,
1.,0.707106781186548,1.,0.707106781186548,1.,0.707106781186548,1.),(1.,
0.707106781186547,1.,0.707106781186547,1.,0.707106781186547,1.,0.707106781186547,
1.),(1.,0.707106781186548,1.,0.707106781186548,1.,0.707106781186548,1.,
0.707106781186548,1.),(1.,0.707106781186547,1.,0.707106781186547,1.,0.707106781186547,
1.,0.707106781186547,1.),(1.,0.707106781186548,1.,0.707106781186548,1.,
0.707106781186548,1.,0.707106781186548,1.),(1.,0.707106781186548,1.,0.707106781186548,
1.,0.707106781186548,1.,0.707106781186548,1.),(1.,0.707106781186547,1.,
0.707106781186547,1.,0.707106781186547,1.,0.707106781186547,1.),(1.,0.707106781186547,
1.,0.707106781186547,1.,0.707106781186547,1.,0.707106781186547,1.),(1.,
0.707106781186548,1.,0.707106781186548,1.,0.707106781186548,1.,0.707106781186548,
1.),(1.,0.707106781186548,1.,0.707106781186548,1.,0.707106781186548,1.,
0.707106781186548,1.),(1.,0.707106781186547,1.,0.707106781186547,1.,0.707106781186547,
1.,0.707106781186547,1.),(1.,0.707106781186547,1.,0.707106781186547,1.,
0.707106781186547,1.,0.707106781186547,1.),(1.,0.707106781186547,1.,0.707106781186547,
1.,0.707106781186547,1.,0.707106781186547,1.),(1.,0.707106781186547,1.,
0.707106781186547,1.,0.707106781186547,1.,0.707106781186547,1.),(1.,0.707106781186547,
1.,0.707106781186547,1.,0.707106781186547,1.,0.707106781186547,1.),(1.,
0.707106781186548,1.,0.707106781186548,1.,0.707106781186548,1.,0.707106781186548,
1.),(1.,0.707106781186547,1.,0.707106781186547,1.,0.707106781186547,1.,
0.707106781186547,1.),(1.,0.707106781186547,1.,0.707106781186547,1.,0.707106781186547,
1.,0.707106781186547,1.),(1.,0.707106781186548,1.,0.707106781186548,1.,
0.707106781186548,1.,0.707106781186548,1.),(1.,0.707106781186547,1.,0.707106781186547,
1.,0.707106781186547,1.,0.707106781186547,1.),(1.,0.707106781186548,1.,
0.707106781186548,1.,0.707106781186548,1.,0.707106781186548,1.),(1.,0.707106781186548,
1.,0.707106781186548,1.,0.707106781186548,1.,0.707106781186548,1.),(1.,
0.707106781186547,1.,0.707106781186547,1.,0.707106781186547,1.,0.707106781186547,
1.),(1.,0.707106781186548,1.,0.707106781186548,1.,0.707106781186548,1.,
0.707106781186548,1.),(1.,0.707106781186547,1.,0.707106781186547,1.,0.707106781186547,
1.,0.707106781186547,1.),(1.,0.707106781186548,1.,0.707106781186548,1.,
0.707106781186548,1.,0.707106781186548,1.),(1.,0.707106781186547,1.,0.707106781186547,
1.,0.707106781186547,1.,0.707106781186547,1.),(1.,0.707106781186548,1.,
0.707106781186548,1.,0.707106781186548,1.,0.707106781186548,1.),(1.,0.707106781186547,
1.,0.707106781186547,1.,0.707106781186547,1.,0.707106781186547,1.),(1.,
0.707106781186547,1.,0.707106781186547,1.,0.707106781186547,1.,0.707106781186547,
1.),(1.,0.707106781186547,1.,0.707106781186547,1.,0.707106781186547,1.,
0.707106781186547,1.),(1.,0.707106781186547,1.,0.707106781186547,1.,0.707106781186547,
1.,0.707106781186547,1.),(1.,0.707106781186547,1.,0.707106781186547,1.,
0.707106781186547,1.,0.707106781186547,1.),(1.,0.707106781186547,1.,0.707106781186547,
1.,0.707106781186547,1.,0.707106781186547,1.),(1.,0.707106781186548,1.,
0.707106781186548,1.,0.707106781186548,1.,0.707106781186548,1.),(1.,0.707106781186547,
1.,0.707106781186547,1.,0.707106781186547,1.,0.707106781186547,1.),(1.,
0.707106781186548,1.,0.707106781186548,1.,0.707106781186548,1.,0.707106781186548,
1.),(1.,0.707106781186547,1.,0.707106781186547,1.,0.707106781186547,1.,
0.707106781186547,1.),(1.,0.707106781186547,1.,0.707106781186547,1.,0.707106781186547,
1.,0.707106781186547,1.),(1.,0.707106781186547,1.,0.707106781186547,1.,
0.707106781186547,1.,0.707106781186547,1.),(1.,0.707106781186548,1.,0.707106781186548,
1.,0.707106781186548,1.,0.707106781186548,1.),(1.,0.707106781186547,1.,
0.707106781186547,1.,0.707106781186547,1.,0.707106781186547,1.),(1.,0.707106781186548,
1.,0.707106781186548,1.,0.707106781186548,1.,0.707106781186548,1.),(1.,
0.707106781186548,1.,0.707106781186548,1.,0.707106781186548,1.,0.707106781186548,
1.),(1.,0.707106781186547,1.,0.707106781186547,1.,0.707106781186547,1.,
0.707106781186547,1.),(1.,0.707106781186547,1.,0.707106781186547,1.,0.707106781186547,
1.,0.707106781186547,1.),(1.,0.707106781186548,1.,0.707106781186548,1.,
0.707106781186548,1.,0.707106781186548,1.),(1.,0.707106781186547,1.,0.707106781186547,
1.,0.707106781186547,1.,0.707106781186547,1.),(1.,0.707106781186548,1.,
0.707106781186548,1.,0.707106781186548,1.,0.707106781186548,1.),(1.,0.707106781186547,
1.,0.707106781186547,1.,0.707106781186547,1.,0.707106781186547,1.),(1.,
0.707106781186548,1.,0.707106781186548,1.,0.707106781186548,1.,0.707106781186548,
1.),(1.,0.707106781186547,1.,0.707106781186547,1.,0.707106781186547,1.,
0.707106781186547,1.),(1.,0.707106781186548,1.,0.707106781186548,1.,0.707106781186548,
1.,0.707106781186548,1.),(1.,0.707106781186547,1.,0.707106781186547,1.,
0.707106781186547,1.,0.707106781186547,1.),(1.,0.707106781186547,1.,0.707106781186547,
1.,0.707106781186547,1.,0.707106781186547,1.),(1.,0.707106781186548,1.,
0.707106781186548,1.,0.707106781186548,1.,0.707106781186548,1.),(1.,0.707106781186547,
1.,0.707106781186547,1.,0.707106781186547,1.,0.707106781186547,1.),(1.,
0.707106781186548,1.,0.707106781186548,1.,0.707106781186548,1.,0.707106781186548,
1.),(1.,0.707106781186547,1.,0.707106781186547,1.,0.707106781186547,1.,
0.707106781186547,1.),(1.,0.707106781186548,1.,0.707106781186548,1.,0.707106781186548,
1.,0.707106781186548,1.),(1.,0.707106781186548,1.,0.707106781186548,1.,
0.707106781186548,1.,0.707106781186548,1.),(1.,0.707106781186548,1.,0.707106781186548,
1.,0.707106781186548,1.,0.707106781186548,1.),(1.,0.707106781186548,1.,
0.707106781186548,1.,0.707106781186548,1.,0.707106781186548,1.),(1.,0.707106781186547,
1.,0.707106781186547,1.,0.707106781186547,1.,0.707106781186547,1.),(1.,
0.707106781186548,1.,0.707106781186548,1.,0.707106781186548,1.,0.707106781186548,
1.),(1.,0.707106781186548,1.,0.707106781186548,1.,0.707106781186548,1.,
0.707106781186548,1.),(1.,0.707106781186548,1.,0.707106781186548,1.,0.707106781186548,
1.,0.707106781186548,1.),(1.,0.707106781186547,1.,0.707106781186547,1.,
0.707106781186547,1.,0.707106781186547,1.),(1.,0.707106781186548,1.,0.707106781186548,
1.,0.707106781186548,1.,0.707106781186548,1.),(1.,0.707106781186548,1.,
0.707106781186548,1.,0.707106781186548,1.,0.707106781186548,1.),(1.,0.707106781186547,
1.,0.707106781186547,1.,0.707106781186547,1.,0.707106781186547,1.),(1.,
0.707106781186548,1.,0.707106781186548,1.,0.707106781186548,1.,0.707106781186548,
1.),(1.,0.707106781186547,1.,0.707106781186547,1.,0.707106781186547,1.,
0.707106781186547,1.),(1.,0.707106781186548,1.,0.707106781186548,1.,0.707106781186548,
1.,0.707106781186548,1.),(1.,0.707106781186547,1.,0.707106781186547,1.,
0.707106781186547,1.,0.707106781186547,1.),(1.,0.707106781186547,1.,0.707106781186547,
1.,0.707106781186547,1.,0.707106781186547,1.),(1.,0.707106781186547,1.,
0.707106781186547,1.,0.707106781186547,1.,0.707106781186547,1.),(1.,0.707106781186548,
1.,0.707106781186548,1.,0.707106781186548,1.,0.707106781186548,1.),(1.,
0.707106781186548,1.,0.707106781186548,1.,0.707106781186548,1.,0.707106781186548,
1.),(1.,0.707106781186547,1.,0.707106781186547,1.,0.707106781186547,1.,
0.707106781186547,1.),(1.,0.707106781186548,1.,0.707106781186548,1.,0.707106781186548,
1.,0.707106781186548,1.),(1.,0.707106781186547,1.,0.707106781186547,1.,
0.707106781186547,1.,0.707106781186547,1.),(1.,0.707106781186548,1.,0.707106781186548,
1.,0.707106781186548,1.,0.707106781186548,1.),(1.,0.707106781186547,1.,
0.707106781186547,1.,0.707106781186547,1.,0.707106781186547,1.),(1.,0.707106781186548,
1.,0.707106781186548,1.,0.707106781186548,1.,0.707106781186548,1.),(1.,
0.707106781186548,1.,0.707106781186548,1.,0.707106781186548,1.,0.707106781186548,
1.),(1.,0.707106781186547,1.,0.707106781186547,1.,0.707106781186547,1.,
0.707106781186547,1.),(1.,0.707106781186548,1.,0.707106781186548,1.,0.707106781186548,
1.,0.707106781186548,1.),(1.,0.707106781186547,1.,0.707106781186547,1.,
0.707106781186547,1.,0.707106781186547,1.),(1.,0.707106781186547,1.,0.707106781186547,
1.,0.707106781186547,1.,0.707106781186547,1.),(1.,0.707106781186548,1.,
0.707106781186548,1.,0.707106781186548,1.,0.707106781186548,1.),(1.,0.707106781186547,
1.,0.707106781186547,1.,0.707106781186547,1.,0.707106781186547,1.),(1.,
0.707106781186547,1.,0.707106781186547,1.,0.707106781186547,1.,0.707106781186547,
1.),(1.,0.707106781186547,1.,0.707106781186547,1.,0.707106781186547,1.,
0.707106781186547,1.),(1.,0.707106781186548,1.,0.707106781186548,1.,0.707106781186548,
1.,0.707106781186548,1.),(1.,0.707106781186547,1.,0.707106781186547,1.,
0.707106781186547,1.,0.707106781186547,1.),(1.,0.707106781186548,1.,0.707106781186548,
1.,0.707106781186548,1.,0.707106781186548,1.),(1.,0.707106781186548,1.,
0.707106781186548,1.,0.707106781186548,1.,0.707106781186548,1.),(1.,0.707106781186547,
1.,0.707106781186547,1.,0.707106781186547,1.,0.707106781186547,1.),(1.,
0.707106781186548,1.,0.707106781186548,1.,0.707106781186548,1.,0.707106781186548,
1.),(1.,0.707106781186547,1.,0.707106781186547,1.,0.707106781186547,1.,
0.707106781186547,1.),(1.,0.707106781186548,1.,0.707106781186548,1.,0.707106781186548,
1.,0.707106781186548,1.),(1.,0.707106781186548,1.,0.707106781186548,1.,
0.707106781186548,1.,0.707106781186548,1.),(1.,0.707106781186548,1.,0.707106781186548,
1.,0.707106781186548,1.,0.707106781186548,1.),(1.,0.707106781186548,1.,
0.707106781186548,1.,0.707106781186548,1.,0.707106781186548,1.),(1.,0.707106781186547,
1.,0.707106781186547,1.,0.707106781186547,1.,0.707106781186547,1.),(1.,
0.707106781186548,1.,0.707106781186548,1.,0.707106781186548,1.,0.707106781186548,
1.),(1.,0.707106781186547,1.,0.707106781186547,1.,0.707106781186547,1.,
0.707106781186547,1.),(1.,0.707106781186548,1.,0.707106781186548,1.,0.707106781186548,
1.,0.707106781186548,1.),(1.,0.707106781186547,1.,0.707106781186547,1.,
0.707106781186547,1.,0.707106781186547,1.),(1.,0.707106781186548,1.,0.707106781186548,
1.,0.707106781186548,1.,0.707106781186548,1.),(1.,0.707106781186547,1.,
0.707106781186547,1.,0.707106781186547,1.,0.707106781186547,1.),(1.,0.707106781186547,
1.,0.707106781186547,1.,0.707106781186547,1.,0.707106781186547,1.),(1.,
0.707106781186547,1.,0.707106781186547,1.,0.707106781186547,1.,0.707106781186547,
1.),(1.,0.707106781186547,1.,0.707106781186547,1.,0.707106781186547,1.,
0.707106781186547,1.),(1.,0.707106781186548,1.,0.707106781186548,1.,0.707106781186548,
1.,0.707106781186548,1.),(1.,0.707106781186547,1.,0.707106781186547,1.,
0.707106781186547,1.,0.707106781186547,1.),(1.,0.707106781186548,1.,0.707106781186548,
1.,0.707106781186548,1.,0.707106781186548,1.),(1.,0.707106781186547,1.,
0.707106781186547,1.,0.707106781186547,1.,0.707106781186547,1.),(1.,0.707106781186547,
1.,0.707106781186547,1.,0.707106781186547,1.,0.707106781186547,1.),(1.,
0.707106781186548,1.,0.707106781186548,1.,0.707106781186548,1.,0.707106781186548,
1.),(1.,0.707106781186547,1.,0.707106781186547,1.,0.707106781186547,1.,
0.707106781186547,1.),(1.,0.707106781186548,1.,0.707106781186548,1.,0.707106781186548,
1.,0.707106781186548,1.),(1.,0.707106781186547,1.,0.707106781186547,1.,
0.707106781186547,1.,0.707106781186547,1.),(1.,0.707106781186548,1.,0.707106781186548,
1.,0.707106781186548,1.,0.707106781186548,1.),(1.,0.707106781186547,1.,
0.707106781186547,1.,0.707106781186547,1.,0.707106781186547,1.),(1.,0.707106781186548,
1.,0.707106781186548,1.,0.707106781186548,1.,0.707106781186548,1.),(1.,
0.707106781186548,1.,0.707106781186548,1.,0.707106781186548,1.,0.707106781186548,
1.),(1.,0.707106781186548,1.,0.707106781186548,1.,0.707106781186548,1.,
0.707106781186548,1.),(1.,0.707106781186548,1.,0.707106781186548,1.,0.707106781186548,
1.,0.707106781186548,1.),(1.,0.707106781186547,1.,0.707106781186547,1.,
0.707106781186547,1.,0.707106781186547,1.),(1.,0.707106781186548,1.,0.707106781186548,
1.,0.707106781186548,1.,0.707106781186548,1.),(1.,0.707106781186548,1.,
0.707106781186548,1.,0.707106781186548,1.,0.707106781186548,1.),(1.,0.707106781186547,
1.,0.707106781186547,1.,0.707106781186547,1.,0.707106781186547,1.),(1.,
0.707106781186548,1.,0.707106781186548,1.,0.707106781186548,1.,0.707106781186548,
1.),(1.,0.707106781186547,1.,0.707106781186547,1.,0.707106781186547,1.,
0.707106781186547,1.),(1.,0.707106781186548,1.,0.707106781186548,1.,0.707106781186548,
1.,0.707106781186548,1.),(1.,0.707106781186547,1.,0.707106781186547,1.,
0.707106781186547,1.,0.707106781186547,1.),(1.,0.707106781186548,1.,0.707106781186548,
1.,0.707106781186548,1.,0.707106781186548,1.),(1.,0.707106781186547,1.,
0.707106781186547,1.,0.707106781186547,1.,0.707106781186547,1.),(1.,0.707106781186547,
1.,0.707106781186547,1.,0.707106781186547,1.,0.707106781186547,1.),(1.,
0.707106781186548,1.,0.707106781186548,1.,0.707106781186548,1.,0.707106781186548,
1.),(1.,0.707106781186547,1.,0.707106781186547,1.,0.707106781186547,1.,
0.707106781186547,1.),(1.,0.707106781186548,1.,0.707106781186548,1.,0.707106781186548,
1.,0.707106781186548,1.),(1.,0.707106781186547,1.,0.707106781186547,1.,
0.707106781186547,1.,0.707106781186547,1.),(1.,0.707106781186547,1.,0.707106781186547,
1.,0.707106781186547,1.,0.707106781186547,1.),(1.,0.707106781186548,1.,
0.707106781186548,1.,0.707106781186548,1.,0.707106781186548,1.),(1.,0.707106781186547,
1.,0.707106781186547,1.,0.707106781186547,1.,0.707106781186547,1.),(1.,
0.707106781186548,1.,0.707106781186548,1.,0.707106781186548,1.,0.707106781186548,
1.),(1.,0.707106781186547,1.,0.707106781186547,1.,0.707106781186547,1.,
0.707106781186547,1.),(1.,0.707106781186547,1.,0.707106781186547,1.,0.707106781186547,
1.,0.707106781186547,1.),(1.,0.707106781186548,1.,0.707106781186548,1.,
0.707106781186548,1.,0.707106781186548,1.),(1.,0.707106781186548,1.,0.707106781186548,
1.,0.707106781186548,1.,0.707106781186548,1.),(1.,0.707106781186548,1.,
0.707106781186548,1.,0.707106781186548,1.,0.707106781186548,1.),(1.,0.707106781186548,
1.,0.707106781186548,1.,0.707106781186548,1.,0.707106781186548,1.),(1.,
0.707106781186548,1.,0.707106781186548,1.,0.707106781186548,1.,0.707106781186548,
1.),(1.,0.707106781186548,1.,0.707106781186548,1.,0.707106781186548,1.,
0.707106781186548,1.),(1.,0.707106781186548,1.,0.707106781186548,1.,0.707106781186548,
1.,0.707106781186548,1.),(1.,0.707106781186548,1.,0.707106781186548,1.,
0.707106781186548,1.,0.707106781186548,1.),(1.,0.707106781186548,1.,0.707106781186548,
1.,0.707106781186548,1.,0.707106781186548,1.),(1.,0.707106781186547,1.,
0.707106781186547,1.,0.707106781186547,1.,0.707106781186547,1.),(1.,0.707106781186548,
1.,0.707106781186548,1.,0.707106781186548,1.,0.707106781186548,1.),(1.,
0.707106781186547,1.,0.707106781186547,1.,0.707106781186547,1.,0.707106781186547,
1.),(1.,0.707106781186547,1.,0.707106781186547,1.,0.707106781186547,1.,
0.707106781186547,1.),(1.,0.707106781186548,1.,0.707106781186548,1.,0.707106781186548,
1.,0.707106781186548,1.),(1.,0.707106781186547,1.,0.707106781186547,1.,
0.707106781186547,1.,0.707106781186547,1.),(1.,0.707106781186548,1.,0.707106781186548,
1.,0.707106781186548,1.,0.707106781186548,1.),(1.,0.707106781186548,1.,
0.707106781186548,1.,0.707106781186548,1.,0.707106781186548,1.),(1.,0.707106781186547,
1.,0.707106781186547,1.,0.707106781186547,1.,0.707106781186547,1.),(1.,
0.707106781186547,1.,0.707106781186547,1.,0.707106781186547,1.,0.707106781186547,
1.),(1.,0.707106781186548,1.,0.707106781186548,1.,0.707106781186548,1.,
0.707106781186548,1.),(1.,0.707106781186548,1.,0.707106781186548,1.,0.707106781186548,
1.,0.707106781186548,1.),(1.,0.707106781186547,1.,0.707106781186547,1.,
0.707106781186547,1.,0.707106781186547,1.),(1.,0.707106781186547,1.,0.707106781186547,
1.,0.707106781186547,1.,0.707106781186547,1.),(1.,0.707106781186547,1.,
0.707106781186547,1.,0.707106781186547,1.,0.707106781186547,1.),(1.,0.707106781186547,
1.,0.707106781186547,1.,0.707106781186547,1.,0.707106781186547,1.),(1.,
0.707106781186547,1.,0.707106781186547,1.,0.707106781186547,1.,0.707106781186547,
1.),(1.,0.707106781186548,1.,0.707106781186548,1.,0.707106781186548,1.,
0.707106781186548,1.),(1.,0.707106781186547,1.,0.707106781186547,1.,0.707106781186547,
1.,0.707106781186547,1.),(1.,0.707106781186548,1.,0.707106781186548,1.,
0.707106781186548,1.,0.707106781186548,1.),(1.,0.707106781186548,1.,0.707106781186548,
1.,0.707106781186548,1.,0.707106781186548,1.),(1.,0.707106781186548,1.,
0.707106781186548,1.,0.707106781186548,1.,0.707106781186548,1.),(1.,0.707106781186547,
1.,0.707106781186547,1.,0.707106781186547,1.,0.707106781186547,1.),(1.,
0.707106781186548,1.,0.707106781186548,1.,0.707106781186548,1.,0.707106781186548,
1.),(1.,0.707106781186547,1.,0.707106781186547,1.,0.707106781186547,1.,
0.707106781186547,1.),(1.,0.707106781186548,1.,0.707106781186548,1.,0.707106781186548,
1.,0.707106781186548,1.),(1.,0.707106781186547,1.,0.707106781186547,1.,
0.707106781186547,1.,0.707106781186547,1.),(1.,0.707106781186548,1.,0.707106781186548,
1.,0.707106781186548,1.,0.707106781186548,1.),(1.,0.707106781186547,1.,
0.707106781186547,1.,0.707106781186547,1.,0.707106781186547,1.),(1.,0.707106781186548,
1.,0.707106781186548,1.,0.707106781186548,1.,0.707106781186548,1.),(1.,
0.707106781186548,1.,0.707106781186548,1.,0.707106781186548,1.,0.707106781186548,
1.),(1.,0.707106781186547,1.,0.707106781186547,1.,0.707106781186547,1.,
0.707106781186547,1.),(1.,0.707106781186547,1.,0.707106781186547,1.,0.707106781186547,
1.,0.707106781186547,1.),(1.,0.707106781186548,1.,0.707106781186548,1.,
0.707106781186548,1.,0.707106781186548,1.),(1.,0.707106781186548,1.,0.707106781186548,
1.,0.707106781186548,1.,0.707106781186548,1.),(1.,0.707106781186548,1.,
0.707106781186548,1.,0.707106781186548,1.,0.707106781186548,1.),(1.,0.707106781186547,
1.,0.707106781186547,1.,0.707106781186547,1.,0.707106781186547,1.),(1.,
0.707106781186547,1.,0.707106781186547,1.,0.707106781186547,1.,0.707106781186547,
1.),(1.,0.707106781186548,1.,0.707106781186548,1.,0.707106781186548,1.,
0.707106781186548,1.),(1.,0.707106781186547,1.,0.707106781186547,1.,0.707106781186547,
1.,0.707106781186547,1.),(1.,0.707106781186547,1.,0.707106781186547,1.,
0.707106781186547,1.,0.707106781186547,1.),(1.,0.707106781186548,1.,0.707106781186548,
1.,0.707106781186548,1.,0.707106781186548,1.),(1.,0.707106781186547,1.,
0.707106781186547,1.,0.707106781186547,1.,0.707106781186547,1.),(1.,0.707106781186548,
1.,0.707106781186548,1.,0.707106781186548,1.,0.707106781186548,1.),(1.,
0.707106781186547,1.,0.707106781186547,1.,0.707106781186547,1.,0.707106781186547,
1.),(1.,0.707106781186547,1.,0.707106781186547,1.,0.707106781186547,1.,
0.707106781186547,1.),(1.,0.707106781186548,1.,0.707106781186548,1.,0.707106781186548,
1.,0.707106781186548,1.),(1.,0.707106781186548,1.,0.707106781186548,1.,
0.707106781186548,1.,0.707106781186548,1.),(1.,0.707106781186548,1.,0.707106781186548,
1.,0.707106781186548,1.,0.707106781186548,1.),(1.,0.707106781186547,1.,
0.707106781186547,1.,0.707106781186547,1.,0.707106781186547,1.),(1.,0.707106781186547,
1.,0.707106781186547,1.,0.707106781186547,1.,0.707106781186547,1.),(1.,
0.707106781186548,1.,0.707106781186548,1.,0.707106781186548,1.,0.707106781186548,
1.),(1.,0.707106781186547,1.,0.707106781186547,1.,0.707106781186547,1.,
0.707106781186547,1.),(1.,0.707106781186548,1.,0.707106781186548,1.,0.707106781186548,
1.,0.707106781186548,1.),(1.,0.707106781186547,1.,0.707106781186547,1.,
0.707106781186547,1.,0.707106781186547,1.),(1.,0.707106781186548,1.,0.707106781186548,
1.,0.707106781186548,1.,0.707106781186548,1.),(1.,0.707106781186547,1.,
0.707106781186547,1.,0.707106781186547,1.,0.707106781186547,1.),(1.,0.707106781186548,
1.,0.707106781186548,1.,0.707106781186548,1.,0.707106781186548,1.),(1.,
0.707106781186548,1.,0.707106781186548,1.,0.707106781186548,1.,0.707106781186548,
1.),(1.,0.707106781186547,1.,0.707106781186547,1.,0.707106781186547,1.,
0.707106781186547,1.),(1.,0.707106781186548,1.,0.707106781186548,1.,0.707106781186548,
1.,0.707106781186548,1.),(1.,0.707106781186547,1.,0.707106781186547,1.,
0.707106781186547,1.,0.707106781186547,1.),(1.,0.707106781186548,1.,0.707106781186548,
1.,0.707106781186548,1.,0.707106781186548,1.),(1.,0.707106781186547,1.,
0.707106781186547,1.,0.707106781186547,1.,0.707106781186547,1.),(1.,0.707106781186547,
1.,0.707106781186547,1.,0.707106781186547,1.,0.707106781186547,1.),(1.,
0.707106781186547,1.,0.707106781186547,1.,0.707106781186547,1.,0.707106781186547,
1.),(1.,0.707106781186548,1.,0.707106781186548,1.,0.707106781186548,1.,
0.707106781186548,1.),(1.,0.707106781186547,1.,0.707106781186547,1.,0.707106781186547,
1.,0.707106781186547,1.),(1.,0.707106781186548,1.,0.707106781186548,1.,
0.707106781186548,1.,0.707106781186548,1.),(1.,0.707106781186547,1.,0.707106781186547,
1.,0.707106781186547,1.,0.707106781186547,1.),(1.,0.707106781186547,1.,
0.707106781186547,1.,0.707106781186547,1.,0.707106781186547,1.),(1.,0.707106781186547,
1.,0.707106781186547,1.,0.707106781186547,1.,0.707106781186547,1.),(1.,
0.707106781186548,1.,0.707106781186548,1.,0.707106781186548,1.,0.707106781186548,
1.),(1.,0.707106781186547,1.,0.707106781186547,1.,0.707106781186547,1.,
0.707106781186547,1.),(1.,0.707106781186547,1.,0.707106781186547,1.,0.707106781186547,
1.,0.707106781186547,1.),(1.,0.707106781186548,1.,0.707106781186548,1.,
0.707106781186548,1.,0.707106781186548,1.),(1.,0.707106781186548,1.,0.707106781186548,
1.,0.707106781186548,1.,0.707106781186548,1.),(1.,0.707106781186547,1.,
0.707106781186547,1.,0.707106781186547,1.,0.707106781186547,1.),(1.,0.707106781186548,
1.,0.707106781186548,1.,0.707106781186548,1.,0.707106781186548,1.),(1.,
0.707106781186547,1.,0.707106781186547,1.,0.707106781186547,1.,0.707106781186547,
1.),(1.,0.707106781186548,1.,0.707106781186548,1.,0.707106781186548,1.,
0.707106781186548,1.),(1.,0.707106781186548,1.,0.707106781186548,1.,0.707106781186548,
1.,0.707106781186548,1.),(1.,0.707106781186547,1.,0.707106781186547,1.,
0.707106781186547,1.,0.707106781186547,1.),(1.,0.707106781186548,1.,0.707106781186548,
1.,0.707106781186548,1.,0.707106781186548,1.),(1.,0.707106781186547,1.,
0.707106781186547,1.,0.707106781186547,1.,0.707106781186547,1.),(1.,0.707106781186547,
1.,0.707106781186547,1.,0.707106781186547,1.,0.707106781186547,1.),(1.,
0.707106781186548,1.,0.707106781186548,1.,0.707106781186548,1.,0.707106781186548,
1.),(1.,0.707106781186547,1.,0.707106781186547,1.,0.707106781186547,1.,
0.707106781186547,1.),(1.,0.707106781186547,1.,0.707106781186547,1.,0.707106781186547,
1.,0.707106781186547,1.),(1.,0.707106781186547,1.,0.707106781186547,1.,
0.707106781186547,1.,0.707106781186547,1.),(1.,0.707106781186548,1.,0.707106781186548,
1.,0.707106781186548,1.,0.707106781186548,1.),(1.,0.707106781186547,1.,
0.707106781186547,1.,0.707106781186547,1.,0.707106781186547,1.),(1.,0.707106781186548,
1.,0.707106781186548,1.,0.707106781186548,1.,0.707106781186548,1.),(1.,
0.707106781186547,1.,0.707106781186547,1.,0.707106781186547,1.,0.707106781186547,
1.),(1.,0.707106781186548,1.,0.707106781186548,1.,0.707106781186548,1.,
0.707106781186548,1.),(1.,0.707106781186548,1.,0.707106781186548,1.,0.707106781186548,
1.,0.707106781186548,1.),(1.,0.707106781186548,1.,0.707106781186548,1.,
0.707106781186548,1.,0.707106781186548,1.),(1.,0.707106781186547,1.,0.707106781186547,
1.,0.707106781186547,1.,0.707106781186547,1.),(1.,0.707106781186548,1.,
0.707106781186548,1.,0.707106781186548,1.,0.707106781186548,1.),(1.,0.707106781186548,
1.,0.707106781186548,1.,0.707106781186548,1.,0.707106781186548,1.),(1.,
0.707106781186548,1.,0.707106781186548,1.,0.707106781186548,1.,0.707106781186548,
1.),(1.,0.707106781186547,1.,0.707106781186547,1.,0.707106781186547,1.,
0.707106781186547,1.),(1.,0.707106781186548,1.,0.707106781186548,1.,0.707106781186548,
1.,0.707106781186548,1.),(1.,0.707106781186547,1.,0.707106781186547,1.,
0.707106781186547,1.,0.707106781186547,1.),(1.,0.707106781186547,1.,0.707106781186547,
1.,0.707106781186547,1.,0.707106781186547,1.),(1.,0.707106781186548,1.,
0.707106781186548,1.,0.707106781186548,1.,0.707106781186548,1.),(1.,0.707106781186547,
1.,0.707106781186547,1.,0.707106781186547,1.,0.707106781186547,1.),(1.,
0.707106781186547,1.,0.707106781186547,1.,0.707106781186547,1.,0.707106781186547,
1.),(1.,0.707106781186548,1.,0.707106781186548,1.,0.707106781186548,1.,
0.707106781186548,1.),(1.,0.707106781186548,1.,0.707106781186548,1.,0.707106781186548,
1.,0.707106781186548,1.),(1.,0.707106781186547,1.,0.707106781186547,1.,
0.707106781186547,1.,0.707106781186547,1.),(1.,0.707106781186548,1.,0.707106781186548,
1.,0.707106781186548,1.,0.707106781186548,1.),(1.,0.707106781186547,1.,
0.707106781186547,1.,0.707106781186547,1.,0.707106781186547,1.),(1.,0.707106781186548,
1.,0.707106781186548,1.,0.707106781186548,1.,0.707106781186548,1.),(1.,
0.707106781186548,1.,0.707106781186548,1.,0.707106781186548,1.,0.707106781186548,
1.),(1.,0.707106781186547,1.,0.707106781186547,1.,0.707106781186547,1.,
0.707106781186547,1.),(1.,0.707106781186548,1.,0.707106781186548,1.,0.707106781186548,
1.,0.707106781186548,1.),(1.,0.707106781186547,1.,0.707106781186547,1.,
0.707106781186547,1.,0.707106781186547,1.),(1.,0.707106781186548,1.,0.707106781186548,
1.,0.707106781186548,1.,0.707106781186548,1.),(1.,0.707106781186547,1.,
0.707106781186547,1.,0.707106781186547,1.,0.707106781186547,1.),(1.,0.707106781186548,
1.,0.707106781186548,1.,0.707106781186548,1.,0.707106781186548,1.),(1.,
0.707106781186547,1.,0.707106781186547,1.,0.707106781186547,1.,0.707106781186547,
1.),(1.,0.707106781186548,1.,0.707106781186548,1.,0.707106781186548,1.,
0.707106781186548,1.),(1.,0.707106781186548,1.,0.707106781186548,1.,0.707106781186548,
1.,0.707106781186548,1.),(1.,0.707106781186548,1.,0.707106781186548,1.,
0.707106781186548,1.,0.707106781186548,1.),(1.,0.707106781186547,1.,0.707106781186547,
1.,0.707106781186547,1.,0.707106781186547,1.),(1.,0.707106781186548,1.,
0.707106781186548,1.,0.707106781186548,1.,0.707106781186548,1.),(1.,0.707106781186548,
1.,0.707106781186548,1.,0.707106781186548,1.,0.707106781186548,1.),(1.,
0.707106781186547,1.,0.707106781186547,1.,0.707106781186547,1.,0.707106781186547,
1.),(1.,0.707106781186547,1.,0.707106781186547,1.,0.707106781186547,1.,
0.707106781186547,1.),(1.,0.707106781186548,1.,0.707106781186548,1.,0.707106781186548,
1.,0.707106781186548,1.),(1.,0.707106781186547,1.,0.707106781186547,1.,
0.707106781186547,1.,0.707106781186547,1.),(1.,0.707106781186548,1.,0.707106781186548,
1.,0.707106781186548,1.,0.707106781186548,1.),(1.,0.707106781186548,1.,
0.707106781186548,1.,0.707106781186548,1.,0.707106781186548,1.),(1.,0.707106781186547,
1.,0.707106781186547,1.,0.707106781186547,1.,0.707106781186547,1.),(1.,
0.707106781186548,1.,0.707106781186548,1.,0.707106781186548,1.,0.707106781186548,
1.),(1.,0.707106781186548,1.,0.707106781186548,1.,0.707106781186548,1.,
0.707106781186548,1.),(1.,0.707106781186547,1.,0.707106781186547,1.,0.707106781186547,
1.,0.707106781186547,1.),(1.,0.707106781186548,1.,0.707106781186548,1.,
0.707106781186548,1.,0.707106781186548,1.),(1.,0.707106781186548,1.,0.707106781186548,
1.,0.707106781186548,1.,0.707106781186548,1.),(1.,0.707106781186547,1.,
0.707106781186547,1.,0.707106781186547,1.,0.707106781186547,1.),(1.,0.707106781186547,
1.,0.707106781186547,1.,0.707106781186547,1.,0.707106781186547,1.),(1.,
0.707106781186548,1.,0.707106781186548,1.,0.707106781186548,1.,0.707106781186548,
1.),(1.,0.707106781186547,1.,0.707106781186547,1.,0.707106781186547,1.,
0.707106781186547,1.),(1.,0.707106781186548,1.,0.707106781186548,1.,0.707106781186548,
1.,0.707106781186548,1.),(1.,0.707106781186547,1.,0.707106781186547,1.,
0.707106781186547,1.,0.707106781186547,1.),(1.,0.707106781186548,1.,0.707106781186548,
1.,0.707106781186548,1.,0.707106781186548,1.),(1.,0.707106781186547,1.,
0.707106781186547,1.,0.707106781186547,1.,0.707106781186547,1.),(1.,0.707106781186548,
1.,0.707106781186548,1.,0.707106781186548,1.,0.707106781186548,1.),(1.,
0.707106781186548,1.,0.707106781186548,1.,0.707106781186548,1.,0.707106781186548,
1.),(1.,0.707106781186548,1.,0.707106781186548,1.,0.707106781186548,1.,
0.707106781186548,1.),(1.,0.707106781186547,1.,0.707106781186547,1.,0.707106781186547,
1.,0.707106781186547,1.),(1.,0.707106781186548,1.,0.707106781186548,1.,
0.707106781186548,1.,0.707106781186548,1.),(1.,0.707106781186547,1.,0.707106781186547,
1.,0.707106781186547,1.,0.707106781186547,1.),(1.,0.707106781186548,1.,
0.707106781186548,1.,0.707106781186548,1.,0.707106781186548,1.),(1.,0.707106781186547,
1.,0.707106781186547,1.,0.707106781186547,1.,0.707106781186547,1.),(1.,
0.707106781186548,1.,0.707106781186548,1.,0.707106781186548,1.,0.707106781186548,
1.),(1.,0.707106781186547,1.,0.707106781186547,1.,0.707106781186547,1.,
0.707106781186547,1.),(1.,0.707106781186548,1.,0.707106781186548,1.,0.707106781186548,
1.,0.707106781186548,1.),(1.,0.707106781186547,1.,0.707106781186547,1.,
0.707106781186547,1.,0.707106781186547,1.),(1.,0.707106781186548,1.,0.707106781186548,
1.,0.707106781186548,1.,0.707106781186548,1.),(1.,0.707106781186547,1.,
0.707106781186547,1.,0.707106781186547,1.,0.707106781186547,1.),(1.,0.707106781186548,
1.,0.707106781186548,1.,0.707106781186548,1.,0.707106781186548,1.),(1.,
0.707106781186547,1.,0.707106781186547,1.,0.707106781186547,1.,0.707106781186547,
1.),(1.,0.707106781186547,1.,0.707106781186547,1.,0.707106781186547,1.,
0.707106781186547,1.),(1.,0.707106781186547,1.,0.707106781186547,1.,0.707106781186547,
1.,0.707106781186547,1.),(1.,0.707106781186548,1.,0.707106781186548,1.,
0.707106781186548,1.,0.707106781186548,1.),(1.,0.707106781186547,1.,0.707106781186547,
1.,0.707106781186547,1.,0.707106781186547,1.),(1.,0.707106781186548,1.,
0.707106781186548,1.,0.707106781186548,1.,0.707106781186548,1.),(1.,0.707106781186547,
1.,0.707106781186547,1.,0.707106781186547,1.,0.707106781186547,1.),(1.,
0.707106781186548,1.,0.707106781186548,1.,0.707106781186548,1.,0.707106781186548,
1.),(1.,0.707106781186547,1.,0.707106781186547,1.,0.707106781186547,1.,
0.707106781186547,1.),(1.,0.707106781186548,1.,0.707106781186548,1.,0.707106781186548,
1.,0.707106781186548,1.),(1.,0.707106781186547,1.,0.707106781186547,1.,
0.707106781186547,1.,0.707106781186547,1.),(1.,0.707106781186548,1.,0.707106781186548,
1.,0.707106781186548,1.,0.707106781186548,1.),(1.,0.707106781186548,1.,
0.707106781186548,1.,0.707106781186548,1.,0.707106781186548,1.),(1.,0.707106781186548,
1.,0.707106781186548,1.,0.707106781186548,1.,0.707106781186548,1.),(1.,
0.707106781186547,1.,0.707106781186547,1.,0.707106781186547,1.,0.707106781186547,
1.),(1.,0.707106781186548,1.,0.707106781186548,1.,0.707106781186548,1.,
0.707106781186548,1.),(1.,0.707106781186547,1.,0.707106781186547,1.,0.707106781186547,
1.,0.707106781186547,1.),(1.,0.707106781186548,1.,0.707106781186548,1.,
0.707106781186548,1.,0.707106781186548,1.),(1.,0.707106781186548,1.,0.707106781186548,
1.,0.707106781186548,1.,0.707106781186548,1.),(1.,0.707106781186547,1.,
0.707106781186547,1.,0.707106781186547,1.,0.707106781186547,1.),(1.,0.707106781186548,
1.,0.707106781186548,1.,0.707106781186548,1.,0.707106781186548,1.),(1.,
0.707106781186547,1.,0.707106781186547,1.,0.707106781186547,1.,0.707106781186547,
1.),(1.,0.707106781186548,1.,0.707106781186548,1.,0.707106781186548,1.,
0.707106781186548,1.),(1.,0.707106781186547,1.,0.707106781186547,1.,0.707106781186547,
1.,0.707106781186547,1.),(1.,0.707106781186548,1.,0.707106781186548,1.,
0.707106781186548,1.,0.707106781186548,1.),(1.,0.707106781186547,1.,0.707106781186547,
1.,0.707106781186547,1.,0.707106781186547,1.),(1.,0.707106781186548,1.,
0.707106781186548,1.,0.707106781186548,1.,0.707106781186548,1.),(1.,0.707106781186547,
1.,0.707106781186547,1.,0.707106781186547,1.,0.707106781186547,1.),(1.,
0.707106781186547,1.,0.707106781186547,1.,0.707106781186547,1.,0.707106781186547,
1.),(1.,0.707106781186547,1.,0.707106781186547,1.,0.707106781186547,1.,
0.707106781186547,1.),(1.,0.707106781186548,1.,0.707106781186548,1.,0.707106781186548,
1.,0.707106781186548,1.),(1.,0.707106781186547,1.,0.707106781186547,1.,
0.707106781186547,1.,0.707106781186547,1.),(1.,0.707106781186547,1.,0.707106781186547,
1.,0.707106781186547,1.,0.707106781186547,1.),(1.,0.707106781186548,1.,
0.707106781186548,1.,0.707106781186548,1.,0.707106781186548,1.),(1.,0.707106781186547,
1.,0.707106781186547,1.,0.707106781186547,1.,0.707106781186547,1.),(1.,
0.707106781186548,1.,0.707106781186548,1.,0.707106781186548,1.,0.707106781186548,
1.),(1.,0.707106781186547,1.,0.707106781186547,1.,0.707106781186547,1.,
0.707106781186547,1.),(1.,0.707106781186547,1.,0.707106781186547,1.,0.707106781186547,
1.,0.707106781186547,1.),(1.,0.707106781186548,1.,0.707106781186548,1.,
0.707106781186548,1.,0.707106781186548,1.),(1.,0.707106781186547,1.,0.707106781186547,
1.,0.707106781186547,1.,0.707106781186547,1.),(1.,0.707106781186548,1.,
0.707106781186548,1.,0.707106781186548,1.,0.707106781186548,1.),(1.,0.707106781186547,
1.,0.707106781186547,1.,0.707106781186547,1.,0.707106781186547,1.),(1.,
0.707106781186548,1.,0.707106781186548,1.,0.707106781186548,1.,0.707106781186548,
1.),(1.,0.707106781186548,1.,0.707106781186548,1.,0.707106781186548,1.,
0.707106781186548,1.),(1.,0.707106781186548,1.,0.707106781186548,1.,0.707106781186548,
1.,0.707106781186548,1.),(1.,0.707106781186547,1.,0.707106781186547,1.,
0.707106781186547,1.,0.707106781186547,1.),(1.,0.707106781186547,1.,0.707106781186547,
1.,0.707106781186547,1.,0.707106781186547,1.),(1.,0.707106781186548,1.,
0.707106781186548,1.,0.707106781186548,1.,0.707106781186548,1.),(1.,0.707106781186548,
1.,0.707106781186548,1.,0.707106781186548,1.,0.707106781186548,1.),(1.,
0.707106781186547,1.,0.707106781186547,1.,0.707106781186547,1.,0.707106781186547,
1.),(1.,0.707106781186548,1.,0.707106781186548,1.,0.707106781186548,1.,
0.707106781186548,1.),(1.,0.707106781186547,1.,0.707106781186547,1.,0.707106781186547,
1.,0.707106781186547,1.),(1.,0.707106781186547,1.,0.707106781186547,1.,
0.707106781186547,1.,0.707106781186547,1.),(1.,0.707106781186547,1.,0.707106781186547,
1.,0.707106781186547,1.,0.707106781186547,1.),(1.,0.707106781186548,1.,
0.707106781186548,1.,0.707106781186548,1.,0.707106781186548,1.),(1.,0.707106781186547,
1.,0.707106781186547,1.,0.707106781186547,1.,0.707106781186547,1.),(1.,
0.707106781186548,1.,0.707106781186548,1.,0.707106781186548,1.,0.707106781186548,
1.),(1.,0.707106781186547,1.,0.707106781186547,1.,0.707106781186547,1.,
0.707106781186547,1.),(1.,0.707106781186548,1.,0.707106781186548,1.,0.707106781186548,
1.,0.707106781186548,1.),(1.,0.707106781186548,1.,0.707106781186548,1.,
0.707106781186548,1.,0.707106781186548,1.),(1.,0.707106781186548,1.,0.707106781186548,
1.,0.707106781186548,1.,0.707106781186548,1.),(1.,0.707106781186547,1.,
0.707106781186547,1.,0.707106781186547,1.,0.707106781186547,1.),(1.,0.707106781186547,
1.,0.707106781186547,1.,0.707106781186547,1.,0.707106781186547,1.),(1.,
0.707106781186547,1.,0.707106781186547,1.,0.707106781186547,1.,0.707106781186547,
1.),(1.,0.707106781186547,1.,0.707106781186547,1.,0.707106781186547,1.,
0.707106781186547,1.),(1.,0.707106781186547,1.,0.707106781186547,1.,0.707106781186547,
1.,0.707106781186547,1.),(1.,0.707106781186547,1.,0.707106781186547,1.,
0.707106781186547,1.,0.707106781186547,1.),(1.,0.707106781186548,1.,0.707106781186548,
1.,0.707106781186548,1.,0.707106781186548,1.),(1.,0.707106781186547,1.,
0.707106781186547,1.,0.707106781186547,1.,0.707106781186547,1.),(1.,0.707106781186548,
1.,0.707106781186548,1.,0.707106781186548,1.,0.707106781186548,1.),(1.,
0.707106781186547,1.,0.707106781186547,1.,0.707106781186547,1.,0.707106781186547,
1.),(1.,0.707106781186548,1.,0.707106781186548,1.,0.707106781186548,1.,
0.707106781186548,1.),(1.,0.707106781186547,1.,0.707106781186547,1.,0.707106781186547,
1.,0.707106781186547,1.),(1.,0.707106781186547,1.,0.707106781186547,1.,
0.707106781186547,1.,0.707106781186547,1.),(1.,0.707106781186548,1.,0.707106781186548,
1.,0.707106781186548,1.,0.707106781186548,1.),(1.,0.707106781186547,1.,
0.707106781186547,1.,0.707106781186547,1.,0.707106781186547,1.),(1.,0.707106781186547,
1.,0.707106781186547,1.,0.707106781186547,1.,0.707106781186547,1.),(1.,
0.707106781186548,1.,0.707106781186548,1.,0.707106781186548,1.,0.707106781186548,
1.),(1.,0.707106781186548,1.,0.707106781186548,1.,0.707106781186548,1.,
0.707106781186548,1.),(1.,0.707106781186547,1.,0.707106781186547,1.,0.707106781186547,
1.,0.707106781186547,1.),(1.,0.707106781186547,1.,0.707106781186547,1.,
0.707106781186547,1.,0.707106781186547,1.),(1.,0.707106781186547,1.,0.707106781186547,
1.,0.707106781186547,1.,0.707106781186547,1.),(1.,0.707106781186548,1.,
0.707106781186548,1.,0.707106781186548,1.,0.707106781186548,1.),(1.,0.707106781186547,
1.,0.707106781186547,1.,0.707106781186547,1.,0.707106781186547,1.),(1.,
0.707106781186547,1.,0.707106781186547,1.,0.707106781186547,1.,0.707106781186547,
1.),(1.,0.707106781186548,1.,0.707106781186548,1.,0.707106781186548,1.,
0.707106781186548,1.),(1.,0.707106781186548,1.,0.707106781186548,1.,0.707106781186548,
1.,0.707106781186548,1.)))
REPRESENTATION_ITEM('')
SURFACE()
) ;
#66=(
BOUNDED_SURFACE()
B_SPLINE_SURFACE(2,3,((#194404,#194405,#194406,#194407,#194408,#194409,
#194410),(#194411,#194412,#194413,#194414,#194415,#194416,#194417),(#194418,
#194419,#194420,#194421,#194422,#194423,#194424),(#194425,#194426,#194427,
#194428,#194429,#194430,#194431),(#194432,#194433,#194434,#194435,#194436,
#194437,#194438),(#194439,#194440,#194441,#194442,#194443,#194444,#194445),
(#194446,#194447,#194448,#194449,#194450,#194451,#194452),(#194453,#194454,
#194455,#194456,#194457,#194458,#194459),(#194460,#194461,#194462,#194463,
#194464,#194465,#194466)),.UNSPECIFIED.,.T.,.F.,.F.)
B_SPLINE_SURFACE_WITH_KNOTS((3,2,2,2,3),(4,1,1,1,4),(0.,0.117809724509617,
0.235619449019234,0.353429173528852,0.471238898038469),(0.,0.0911446219616379,
0.182289243923276,0.273433865884915,0.364578487846551),.UNSPECIFIED.)
GEOMETRIC_REPRESENTATION_ITEM()
RATIONAL_B_SPLINE_SURFACE(((1.,1.,1.,1.,1.,1.,1.),(0.707106781186548,0.707106781186548,
0.707106781186547,0.707106781186548,0.707106781186547,0.707106781186548,
0.707106781186548),(1.,1.,1.,1.,1.,1.,1.),(0.707106781186548,0.707106781186548,
0.707106781186547,0.707106781186548,0.707106781186547,0.707106781186548,
0.707106781186548),(1.,1.,1.,1.,1.,1.,1.),(0.707106781186548,0.707106781186548,
0.707106781186547,0.707106781186548,0.707106781186547,0.707106781186548,
0.707106781186548),(1.,1.,1.,1.,1.,1.,1.),(0.707106781186548,0.707106781186548,
0.707106781186547,0.707106781186548,0.707106781186547,0.707106781186548,
0.707106781186548),(1.,1.,1.,1.,1.,1.,1.)))
REPRESENTATION_ITEM('')
SURFACE()
) ;
#67=(
BOUNDED_SURFACE()
B_SPLINE_SURFACE(2,3,((#194476,#194477,#194478,#194479),(#194480,#194481,
#194482,#194483),(#194484,#194485,#194486,#194487),(#194488,#194489,#194490,
#194491),(#194492,#194493,#194494,#194495),(#194496,#194497,#194498,#194499),
(#194500,#194501,#194502,#194503),(#194504,#194505,#194506,#194507),(#194508,
#194509,#194510,#194511)),.UNSPECIFIED.,.T.,.F.,.F.)
B_SPLINE_SURFACE_WITH_KNOTS((3,2,2,2,3),(4,4),(0.,0.117809724509617,0.235619449019234,
0.353429173528852,0.471238898038469),(0.,1.1454147408364),.UNSPECIFIED.)
GEOMETRIC_REPRESENTATION_ITEM()
RATIONAL_B_SPLINE_SURFACE(((1.,1.,1.,1.),(0.707106781186548,0.707106781186548,
0.707106781186547,0.707106781186548),(1.,1.,1.,1.),(0.707106781186548,0.707106781186548,
0.707106781186547,0.707106781186548),(1.,1.,1.,1.),(0.707106781186548,0.707106781186548,
0.707106781186547,0.707106781186548),(1.,1.,1.,1.),(0.707106781186548,0.707106781186548,
0.707106781186547,0.707106781186548),(1.,1.,1.,1.)))
REPRESENTATION_ITEM('')
SURFACE()
) ;
#68=(
BOUNDED_SURFACE()
B_SPLINE_SURFACE(2,3,((#194519,#194520,#194521,#194522,#194523,#194524,
#194525,#194526,#194527,#194528,#194529,#194530,#194531,#194532,#194533,
#194534,#194535,#194536,#194537),(#194538,#194539,#194540,#194541,#194542,
#194543,#194544,#194545,#194546,#194547,#194548,#194549,#194550,#194551,
#194552,#194553,#194554,#194555,#194556),(#194557,#194558,#194559,#194560,
#194561,#194562,#194563,#194564,#194565,#194566,#194567,#194568,#194569,
#194570,#194571,#194572,#194573,#194574,#194575),(#194576,#194577,#194578,
#194579,#194580,#194581,#194582,#194583,#194584,#194585,#194586,#194587,
#194588,#194589,#194590,#194591,#194592,#194593,#194594),(#194595,#194596,
#194597,#194598,#194599,#194600,#194601,#194602,#194603,#194604,#194605,
#194606,#194607,#194608,#194609,#194610,#194611,#194612,#194613),(#194614,
#194615,#194616,#194617,#194618,#194619,#194620,#194621,#194622,#194623,
#194624,#194625,#194626,#194627,#194628,#194629,#194630,#194631,#194632),
(#194633,#194634,#194635,#194636,#194637,#194638,#194639,#194640,#194641,
#194642,#194643,#194644,#194645,#194646,#194647,#194648,#194649,#194650,
#194651),(#194652,#194653,#194654,#194655,#194656,#194657,#194658,#194659,
#194660,#194661,#194662,#194663,#194664,#194665,#194666,#194667,#194668,
#194669,#194670),(#194671,#194672,#194673,#194674,#194675,#194676,#194677,
#194678,#194679,#194680,#194681,#194682,#194683,#194684,#194685,#194686,
#194687,#194688,#194689)),.UNSPECIFIED.,.T.,.F.,.F.)
B_SPLINE_SURFACE_WITH_KNOTS((3,2,2,2,3),(4,1,1,1,1,1,1,1,1,1,1,1,1,1,1,
1,4),(0.,0.117809724509617,0.235619449019234,0.353429173528852,0.471238898038469),
(0.,0.226732296973331,0.464902013928651,0.70307173088397,0.9298040278573,
1.15653632483063,1.39470604178595,1.63287575874127,1.8596080557146,2.08634035268793,
2.32451006964325,2.56267978659857,2.7894120835719,3.01614438054523,3.25431409750055,
3.49248381445586,3.7192161114292),.UNSPECIFIED.)
GEOMETRIC_REPRESENTATION_ITEM()
RATIONAL_B_SPLINE_SURFACE(((1.,1.,1.,1.,1.,1.,1.,1.,1.,1.,1.,1.,1.,1.,1.,
1.,1.,1.,1.),(0.707106781186548,0.707106781186547,0.707106781186548,0.707106781186547,
0.707106781186548,0.707106781186547,0.707106781186548,0.707106781186547,
0.707106781186547,0.707106781186547,0.707106781186548,0.707106781186547,
0.707106781186547,0.707106781186547,0.707106781186547,0.707106781186547,
0.707106781186548,0.707106781186547,0.707106781186548),(1.,1.,1.,1.,1.,
1.,1.,1.,1.,1.,1.,1.,1.,1.,1.,1.,1.,1.,1.),(0.707106781186548,0.707106781186547,
0.707106781186548,0.707106781186547,0.707106781186548,0.707106781186547,
0.707106781186548,0.707106781186547,0.707106781186547,0.707106781186547,
0.707106781186548,0.707106781186547,0.707106781186547,0.707106781186547,
0.707106781186547,0.707106781186547,0.707106781186548,0.707106781186547,
0.707106781186548),(1.,1.,1.,1.,1.,1.,1.,1.,1.,1.,1.,1.,1.,1.,1.,1.,1.,
1.,1.),(0.707106781186548,0.707106781186547,0.707106781186548,0.707106781186547,
0.707106781186548,0.707106781186547,0.707106781186548,0.707106781186547,
0.707106781186547,0.707106781186547,0.707106781186548,0.707106781186547,
0.707106781186547,0.707106781186547,0.707106781186547,0.707106781186547,
0.707106781186548,0.707106781186547,0.707106781186548),(1.,1.,1.,1.,1.,
1.,1.,1.,1.,1.,1.,1.,1.,1.,1.,1.,1.,1.,1.),(0.707106781186548,0.707106781186547,
0.707106781186548,0.707106781186547,0.707106781186548,0.707106781186547,
0.707106781186548,0.707106781186547,0.707106781186547,0.707106781186547,
0.707106781186548,0.707106781186547,0.707106781186547,0.707106781186547,
0.707106781186547,0.707106781186547,0.707106781186548,0.707106781186547,
0.707106781186548),(1.,1.,1.,1.,1.,1.,1.,1.,1.,1.,1.,1.,1.,1.,1.,1.,1.,
1.,1.)))
REPRESENTATION_ITEM('')
SURFACE()
) ;
#175=ELLIPSE('',#9023,0.075909797816342,0.0750000000000059) ;
#176=ELLIPSE('',#9024,0.0776797958593107,0.0750000000000013) ;
#177=ELLIPSE('',#9025,0.0776797958593107,0.0750000000000013) ;
#178=ELLIPSE('',#9026,0.0776797958593107,0.0750000000000013) ;
#179=ELLIPSE('',#9027,0.0773330605240012,0.0750000000000033) ;
#180=ELLIPSE('',#9028,0.0773330605239995,0.0750000000000025) ;
#181=ELLIPSE('',#9029,0.0773330605239995,0.0750000000000025) ;
#182=ELLIPSE('',#9030,0.0773330605239995,0.0750000000000025) ;
#183=ELLIPSE('',#9032,0.0759097978163331,0.0750000000000011) ;
#184=ELLIPSE('',#9033,0.0776797958593144,0.0750000000000244) ;
#185=ELLIPSE('',#9034,0.0776797958593144,0.0750000000000244) ;
#186=ELLIPSE('',#9035,0.0776797958593144,0.0750000000000244) ;
#187=ELLIPSE('',#9036,0.0773330605240056,0.0750000000000024) ;
#188=ELLIPSE('',#9037,0.077333060524004,0.0750000000000015) ;
#189=ELLIPSE('',#9038,0.077333060524004,0.0750000000000015) ;
#190=ELLIPSE('',#9039,0.077333060524004,0.0750000000000015) ;
#334=STYLED_ITEM('',(#196765),#353) ;
#353=MANIFOLD_SOLID_BREP('Exit Return Spring',#8730) ;
#406=PLANE('',#9022) ;
#407=PLANE('',#9031) ;
#408=PLANE('',#9040) ;
#409=PLANE('',#9041) ;
#1066=FACE_OUTER_BOUND('',#1575,.T.) ;
#1067=FACE_OUTER_BOUND('',#1576,.T.) ;
#1068=FACE_OUTER_BOUND('',#1577,.T.) ;
#1069=FACE_OUTER_BOUND('',#1578,.T.) ;
#1070=FACE_OUTER_BOUND('',#1579,.T.) ;
#1071=FACE_OUTER_BOUND('',#1580,.T.) ;
#1072=FACE_OUTER_BOUND('',#1581,.T.) ;
#1073=FACE_OUTER_BOUND('',#1582,.T.) ;
#1074=FACE_OUTER_BOUND('',#1583,.T.) ;
#1075=FACE_OUTER_BOUND('',#1584,.T.) ;
#1076=FACE_OUTER_BOUND('',#1585,.T.) ;
#1077=FACE_OUTER_BOUND('',#1586,.T.) ;
#1575=EDGE_LOOP('',(#6596)) ;
#1576=EDGE_LOOP('',(#6597,#6598,#6599,#6600,#6601,#6602,#6603,#6604)) ;
#1577=EDGE_LOOP('',(#6605,#6606,#6607,#6608,#6609,#6610)) ;
#1578=EDGE_LOOP('',(#6611,#6612,#6613,#6614,#6615,#6616)) ;
#1579=EDGE_LOOP('',(#6617,#6618,#6619,#6620,#6621,#6622)) ;
#1580=EDGE_LOOP('',(#6623)) ;
#1581=EDGE_LOOP('',(#6624,#6625,#6626,#6627,#6628,#6629,#6630,#6631)) ;
#1582=EDGE_LOOP('',(#6632,#6633,#6634,#6635,#6636,#6637)) ;
#1583=EDGE_LOOP('',(#6638,#6639,#6640,#6641,#6642,#6643)) ;
#1584=EDGE_LOOP('',(#6644,#6645,#6646,#6647,#6648,#6649)) ;
#1585=EDGE_LOOP('',(#6650,#6651,#6652)) ;
#1586=EDGE_LOOP('',(#6653,#6654,#6655)) ;
#2052=LINE('',#174526,#2755) ;
#2053=LINE('',#194513,#2756) ;
#2755=VECTOR('',#10208,10.) ;
#2756=VECTOR('',#10227,10.) ;
#3441=B_SPLINE_CURVE_WITH_KNOTS('',3,(#173197,#173198,#173199,#173200,#173201,
#173202,#173203,#173204,#173205,#173206,#173207,#173208,#173209,#173210,
#173211,#173212,#173213,#173214,#173215,#173216,#173217,#173218,#173219,
#173220),.UNSPECIFIED.,.F.,.F.,(4,2,2,2,2,2,2,2,2,2,2,4),(1.00031199612268E-6,
0.000119735576117112,0.000254804132751259,0.00059289635728083,0.00141995080467776,
0.00328477655390897,0.00771007580557226,0.0150743060490529,0.0244362537133422,
0.034502869975532,0.0421294348106346,0.0495174324242607),.UNSPECIFIED.) ;
#3442=B_SPLINE_CURVE_WITH_KNOTS('',3,(#173222,#173223,#173224,#173225,#173226,
#173227,#173228,#173229,#173230,#173231,#173232,#173233,#173234,#173235,
#173236,#173237,#173238,#173239,#173240,#173241,#173242,#173243,#173244,
#173245,#173246,#173247,#173248,#173249,#173250,#173251,#173252,#173253,
#173254,#173255,#173256,#173257,#173258,#173259,#173260,#173261),
 .UNSPECIFIED.,.F.,.F.,(4,2,2,2,2,2,2,2,2,2,2,2,2,2,2,2,2,2,2,4),(1.00000084760866E-6,
0.0356408539522558,0.0716339726729334,0.115839657841778,0.158216981743479,
0.204242565336012,0.226773462184898,0.231866667251746,0.233211898655665,
0.234024688708034,0.23470594245746,0.235469634878188,0.236733298374843,
0.239629242314517,0.248630132692209,0.305025417214415,0.356714542868905,
0.408516103190126,0.448230914032676,0.487460271649596),.UNSPECIFIED.) ;
#3443=B_SPLINE_CURVE_WITH_KNOTS('',3,(#173262,#173263,#173264,#173265,#173266,
#173267,#173268,#173269,#173270,#173271,#173272,#173273,#173274,#173275,
#173276,#173277,#173278,#173279,#173280,#173281,#173282,#173283,#173284,
#173285,#173286,#173287,#173288,#173289,#173290,#173291,#173292,#173293,
#173294,#173295,#173296,#173297,#173298,#173299,#173300,#173301,#173302,
#173303,#173304,#173305,#173306,#173307,#173308,#173309,#173310,#173311,
#173312,#173313,#173314,#173315,#173316,#173317,#173318,#173319,#173320,
#173321,#173322,#173323,#173324,#173325,#173326,#173327,#173328,#173329,
#173330,#173331,#173332,#173333,#173334,#173335,#173336,#173337,#173338,
#173339,#173340,#173341,#173342,#173343,#173344,#173345,#173346,#173347,
#173348,#173349,#173350,#173351,#173352),.UNSPECIFIED.,.F.,.F.,(4,3,3,3,
3,3,3,3,3,3,3,3,3,3,3,3,3,3,3,3,3,3,3,3,3,3,3,3,3,3,4),(5.88213542013056,
6.01172757014424,6.06553319243455,6.31789845245754,6.37548924090185,6.63205227957284,
6.68416207138069,6.92308957797642,6.99256132469663,7.21322502396329,7.29931351804432,
7.37778610061133,7.45630345780951,7.53485664750583,7.60445173491709,7.66483122117882,
7.72511128058719,7.78447080698424,7.84521113289827,7.9059514588123,7.9450455134496,
7.98442846700658,8.02381142056356,8.05269948781751,8.08176212724297,8.08494149672526,
8.10686730859982,8.11737739318286,8.13530591783441,8.14584296460486,8.16217407354799),
 .UNSPECIFIED.) ;
#3444=B_SPLINE_CURVE_WITH_KNOTS('',3,(#193185,#193186,#193187,#193188,#193189,
#193190,#193191,#193192,#193193,#193194,#193195,#193196,#193197,#193198,
#193199,#193200,#193201,#193202,#193203,#193204,#193205,#193206,#193207,
#193208),.UNSPECIFIED.,.F.,.F.,(4,2,2,2,2,2,2,2,2,2,2,4),(1.00031199566413E-6,
0.000119735576065817,0.000254804132477893,0.000592896355756741,0.0014199507976843,
0.00328477653422319,0.00771007575652981,0.0150743059510554,0.0244362535529347,
0.0345028697479965,0.0421294345322319,0.0495174320965966),.UNSPECIFIED.) ;
#3445=B_SPLINE_CURVE_WITH_KNOTS('',3,(#193209,#193210,#193211,#193212,#193213,
#193214,#193215,#193216,#193217,#193218,#193219,#193220,#193221,#193222,
#193223,#193224,#193225,#193226,#193227,#193228,#193229,#193230,#193231,
#193232,#193233,#193234,#193235,#193236,#193237,#193238,#193239,#193240,
#193241,#193242,#193243,#193244,#193245,#193246,#193247,#193248),
 .UNSPECIFIED.,.F.,.F.,(4,2,2,2,2,2,2,2,2,2,2,2,2,2,2,2,2,2,2,4),(-0.487460274297177,
-0.44823091626508,-0.408516105002165,-0.356714544130802,-0.305025417927037,
-0.248630132802184,-0.23962924233009,-0.236733298377342,-0.235469634879205,
-0.234705942460026,-0.234024688710982,-0.233211898657874,-0.231866667252239,
-0.22677346218541,-0.204242565336273,-0.158216981743476,-0.115839657841771,
-0.071633972672922,-0.0356408539523076,-1.00000084793567E-6),
 .UNSPECIFIED.) ;
#3446=B_SPLINE_CURVE_WITH_KNOTS('',3,(#193249,#193250,#193251,#193252,#193253,
#193254,#193255,#193256,#193257,#193258,#193259,#193260,#193261,#193262,
#193263,#193264,#193265,#193266,#193267,#193268,#193269,#193270,#193271,
#193272,#193273,#193274,#193275,#193276,#193277,#193278,#193279,#193280,
#193281,#193282,#193283,#193284,#193285,#193286,#193287,#193288,#193289,
#193290,#193291,#193292,#193293,#193294,#193295,#193296,#193297,#193298,
#193299,#193300,#193301,#193302,#193303,#193304,#193305,#193306,#193307,
#193308,#193309,#193310,#193311,#193312,#193313,#193314,#193315,#193316,
#193317,#193318,#193319,#193320,#193321,#193322,#193323,#193324,#193325,
#193326,#193327,#193328,#193329,#193330,#193331,#193332,#193333,#193334,
#193335,#193336,#193337,#193338,#193339),.UNSPECIFIED.,.F.,.F.,(4,3,3,3,
3,3,3,3,3,3,3,3,3,3,3,3,3,3,3,3,3,3,3,3,3,3,3,3,3,3,4),(5.88213542013066,
6.01172757014427,6.06553319243458,6.31789845246383,6.37548924090187,6.63205227957771,
6.68416207138071,6.92308957798153,6.99256132469664,7.21322502396281,7.29931351804433,
7.37778610061136,7.45630345780724,7.53485664750453,7.6044517349171,7.66483122117873,
7.72511128058713,7.78447080698428,7.84521113289829,7.90595145881231,7.94504551344955,
7.98442846700656,8.02381142056356,8.05269948781744,8.08176212725545,8.08494149672526,
8.10686730859978,8.11737739318286,8.13530591783441,8.14584296460486,8.16217407354799),
 .UNSPECIFIED.) ;
#3784=VERTEX_POINT('',#154734) ;
#3785=VERTEX_POINT('',#173195) ;
#3786=VERTEX_POINT('',#173196) ;
#3787=VERTEX_POINT('',#173221) ;
#3788=VERTEX_POINT('',#173353) ;
#3789=VERTEX_POINT('',#174412) ;
#3790=VERTEX_POINT('',#174414) ;
#3791=VERTEX_POINT('',#174480) ;
#3792=VERTEX_POINT('',#174525) ;
#3793=VERTEX_POINT('',#174527) ;
#3794=VERTEX_POINT('',#174529) ;
#3795=VERTEX_POINT('',#174723) ;
#3796=VERTEX_POINT('',#193184) ;
#3797=VERTEX_POINT('',#193340) ;
#3798=VERTEX_POINT('',#194399) ;
#3799=VERTEX_POINT('',#194401) ;
#3800=VERTEX_POINT('',#194467) ;
#3801=VERTEX_POINT('',#194512) ;
#3802=VERTEX_POINT('',#194514) ;
#3803=VERTEX_POINT('',#194516) ;
#4806=EDGE_CURVE('',#3784,#3784,#175,.T.) ;
#4807=EDGE_CURVE('',#3785,#3786,#3441,.T.) ;
#4808=EDGE_CURVE('',#3787,#3786,#3442,.T.) ;
#4809=EDGE_CURVE('',#3787,#3785,#3443,.T.) ;
#4810=EDGE_CURVE('',#3788,#3785,#27,.T.) ;
#4811=EDGE_CURVE('',#3788,#3789,#176,.T.) ;
#4812=EDGE_CURVE('',#3789,#3790,#177,.T.) ;
#4813=EDGE_CURVE('',#3790,#3788,#178,.T.) ;
#4814=EDGE_CURVE('',#3788,#3791,#28,.T.) ;
#4815=EDGE_CURVE('',#3791,#3791,#179,.T.) ;
#4816=EDGE_CURVE('',#3791,#3792,#2052,.T.) ;
#4817=EDGE_CURVE('',#3793,#3792,#180,.T.) ;
#4818=EDGE_CURVE('',#3794,#3793,#181,.T.) ;
#4819=EDGE_CURVE('',#3792,#3794,#182,.T.) ;
#4820=EDGE_CURVE('',#3792,#3784,#29,.T.) ;
#4821=EDGE_CURVE('',#3795,#3795,#183,.T.) ;
#4822=EDGE_CURVE('',#3796,#3786,#3444,.T.) ;
#4823=EDGE_CURVE('',#3786,#3787,#3445,.T.) ;
#4824=EDGE_CURVE('',#3787,#3796,#3446,.T.) ;
#4825=EDGE_CURVE('',#3797,#3796,#30,.T.) ;
#4826=EDGE_CURVE('',#3797,#3798,#184,.T.) ;
#4827=EDGE_CURVE('',#3798,#3799,#185,.T.) ;
#4828=EDGE_CURVE('',#3799,#3797,#186,.T.) ;
#4829=EDGE_CURVE('',#3797,#3800,#31,.T.) ;
#4830=EDGE_CURVE('',#3800,#3800,#187,.T.) ;
#4831=EDGE_CURVE('',#3800,#3801,#2053,.T.) ;
#4832=EDGE_CURVE('',#3802,#3801,#188,.T.) ;
#4833=EDGE_CURVE('',#3803,#3802,#189,.T.) ;
#4834=EDGE_CURVE('',#3801,#3803,#190,.T.) ;
#4835=EDGE_CURVE('',#3801,#3795,#32,.T.) ;
#6596=ORIENTED_EDGE('',*,*,#4806,.T.) ;
#6597=ORIENTED_EDGE('',*,*,#4807,.T.) ;
#6598=ORIENTED_EDGE('',*,*,#4808,.F.) ;
#6599=ORIENTED_EDGE('',*,*,#4809,.T.) ;
#6600=ORIENTED_EDGE('',*,*,#4810,.F.) ;
#6601=ORIENTED_EDGE('',*,*,#4811,.T.) ;
#6602=ORIENTED_EDGE('',*,*,#4812,.T.) ;
#6603=ORIENTED_EDGE('',*,*,#4813,.T.) ;
#6604=ORIENTED_EDGE('',*,*,#4810,.T.) ;
#6605=ORIENTED_EDGE('',*,*,#4811,.F.) ;
#6606=ORIENTED_EDGE('',*,*,#4814,.T.) ;
#6607=ORIENTED_EDGE('',*,*,#4815,.F.) ;
#6608=ORIENTED_EDGE('',*,*,#4814,.F.) ;
#6609=ORIENTED_EDGE('',*,*,#4813,.F.) ;
#6610=ORIENTED_EDGE('',*,*,#4812,.F.) ;
#6611=ORIENTED_EDGE('',*,*,#4815,.T.) ;
#6612=ORIENTED_EDGE('',*,*,#4816,.T.) ;
#6613=ORIENTED_EDGE('',*,*,#4817,.F.) ;
#6614=ORIENTED_EDGE('',*,*,#4818,.F.) ;
#6615=ORIENTED_EDGE('',*,*,#4819,.F.) ;
#6616=ORIENTED_EDGE('',*,*,#4816,.F.) ;
#6617=ORIENTED_EDGE('',*,*,#4819,.T.) ;
#6618=ORIENTED_EDGE('',*,*,#4818,.T.) ;
#6619=ORIENTED_EDGE('',*,*,#4817,.T.) ;
#6620=ORIENTED_EDGE('',*,*,#4820,.T.) ;
#6621=ORIENTED_EDGE('',*,*,#4806,.F.) ;
#6622=ORIENTED_EDGE('',*,*,#4820,.F.) ;
#6623=ORIENTED_EDGE('',*,*,#4821,.T.) ;
#6624=ORIENTED_EDGE('',*,*,#4822,.T.) ;
#6625=ORIENTED_EDGE('',*,*,#4823,.T.) ;
#6626=ORIENTED_EDGE('',*,*,#4824,.T.) ;
#6627=ORIENTED_EDGE('',*,*,#4825,.F.) ;
#6628=ORIENTED_EDGE('',*,*,#4826,.T.) ;
#6629=ORIENTED_EDGE('',*,*,#4827,.T.) ;
#6630=ORIENTED_EDGE('',*,*,#4828,.T.) ;
#6631=ORIENTED_EDGE('',*,*,#4825,.T.) ;
#6632=ORIENTED_EDGE('',*,*,#4826,.F.) ;
#6633=ORIENTED_EDGE('',*,*,#4829,.T.) ;
#6634=ORIENTED_EDGE('',*,*,#4830,.F.) ;
#6635=ORIENTED_EDGE('',*,*,#4829,.F.) ;
#6636=ORIENTED_EDGE('',*,*,#4828,.F.) ;
#6637=ORIENTED_EDGE('',*,*,#4827,.F.) ;
#6638=ORIENTED_EDGE('',*,*,#4830,.T.) ;
#6639=ORIENTED_EDGE('',*,*,#4831,.T.) ;
#6640=ORIENTED_EDGE('',*,*,#4832,.F.) ;
#6641=ORIENTED_EDGE('',*,*,#4833,.F.) ;
#6642=ORIENTED_EDGE('',*,*,#4834,.F.) ;
#6643=ORIENTED_EDGE('',*,*,#4831,.F.) ;
#6644=ORIENTED_EDGE('',*,*,#4834,.T.) ;
#6645=ORIENTED_EDGE('',*,*,#4833,.T.) ;
#6646=ORIENTED_EDGE('',*,*,#4832,.T.) ;
#6647=ORIENTED_EDGE('',*,*,#4835,.T.) ;
#6648=ORIENTED_EDGE('',*,*,#4821,.F.) ;
#6649=ORIENTED_EDGE('',*,*,#4835,.F.) ;
#6650=ORIENTED_EDGE('',*,*,#4808,.T.) ;
#6651=ORIENTED_EDGE('',*,*,#4822,.F.) ;
#6652=ORIENTED_EDGE('',*,*,#4824,.F.) ;
#6653=ORIENTED_EDGE('',*,*,#4807,.F.) ;
#6654=ORIENTED_EDGE('',*,*,#4809,.F.) ;
#6655=ORIENTED_EDGE('',*,*,#4823,.F.) ;
#8449=ADVANCED_FACE('',(#1066),#406,.T.) ;
#8450=ADVANCED_FACE('',(#1067),#61,.T.) ;
#8451=ADVANCED_FACE('',(#1068),#62,.T.) ;
#8452=ADVANCED_FACE('',(#1069),#63,.T.) ;
#8453=ADVANCED_FACE('',(#1070),#64,.T.) ;
#8454=ADVANCED_FACE('',(#1071),#407,.T.) ;
#8455=ADVANCED_FACE('',(#1072),#65,.T.) ;
#8456=ADVANCED_FACE('',(#1073),#66,.T.) ;
#8457=ADVANCED_FACE('',(#1074),#67,.T.) ;
#8458=ADVANCED_FACE('',(#1075),#68,.T.) ;
#8459=ADVANCED_FACE('',(#1076),#408,.T.) ;
#8460=ADVANCED_FACE('',(#1077),#409,.T.) ;
#8730=CLOSED_SHELL('',(#8449,#8450,#8451,#8452,#8453,#8454,#8455,#8456,
#8457,#8458,#8459,#8460)) ;
#9022=AXIS2_PLACEMENT_3D('',#154733,#10196,#10197) ;
#9023=AXIS2_PLACEMENT_3D('',#154735,#10198,#10199) ;
#9024=AXIS2_PLACEMENT_3D('',#174413,#10200,#10201) ;
#9025=AXIS2_PLACEMENT_3D('',#174415,#10202,#10203) ;
#9026=AXIS2_PLACEMENT_3D('',#174416,#10204,#10205) ;
#9027=AXIS2_PLACEMENT_3D('',#174488,#10206,#10207) ;
#9028=AXIS2_PLACEMENT_3D('',#174528,#10209,#10210) ;
#9029=AXIS2_PLACEMENT_3D('',#174530,#10211,#10212) ;
#9030=AXIS2_PLACEMENT_3D('',#174531,#10213,#10214) ;
#9031=AXIS2_PLACEMENT_3D('',#174722,#10215,#10216) ;
#9032=AXIS2_PLACEMENT_3D('',#174724,#10217,#10218) ;
#9033=AXIS2_PLACEMENT_3D('',#194400,#10219,#10220) ;
#9034=AXIS2_PLACEMENT_3D('',#194402,#10221,#10222) ;
#9035=AXIS2_PLACEMENT_3D('',#194403,#10223,#10224) ;
#9036=AXIS2_PLACEMENT_3D('',#194475,#10225,#10226) ;
#9037=AXIS2_PLACEMENT_3D('',#194515,#10228,#10229) ;
#9038=AXIS2_PLACEMENT_3D('',#194517,#10230,#10231) ;
#9039=AXIS2_PLACEMENT_3D('',#194518,#10232,#10233) ;
#9040=AXIS2_PLACEMENT_3D('',#194709,#10234,#10235) ;
#9041=AXIS2_PLACEMENT_3D('',#194710,#10236,#10237) ;
#10196=DIRECTION('center_axis',(-0.94996636698286,0.0212343718222728,0.311629592713367)) ;
#10197=DIRECTION('ref_axis',(0.311699873146498,0.,0.950180608663667)) ;
#10198=DIRECTION('center_axis',(-0.94996636698287,0.0212343718222707,0.311629592713338)) ;
#10199=DIRECTION('ref_axis',(0.312152280469402,0.0288488649901466,0.949593964169177)) ;
#10200=DIRECTION('center_axis',(-0.0760882816615384,0.969794458779537,0.231752629142151)) ;
#10201=DIRECTION('ref_axis',(0.950103467612754,-2.02102068934678E-14,0.311934930442585)) ;
#10202=DIRECTION('center_axis',(-0.0760882816615384,0.969794458779537,0.231752629142151)) ;
#10203=DIRECTION('ref_axis',(0.950103467612754,-2.02102068934678E-14,0.311934930442585)) ;
#10204=DIRECTION('center_axis',(-0.0760882816615384,0.969794458779537,0.231752629142151)) ;
#10205=DIRECTION('ref_axis',(0.950103467612754,-2.02102068934678E-14,0.311934930442585)) ;
#10206=DIRECTION('center_axis',(0.0420144257474089,0.020843567561995,0.998899561377621)) ;
#10207=DIRECTION('ref_axis',(0.999092865779137,-0.00782614817447476,-0.0418592517131076)) ;
#10208=DIRECTION('',(0.0252238094988886,-2.33710244054272E-6,0.999681829098089)) ;
#10209=DIRECTION('center_axis',(0.0420144257475537,0.0208435675618864,0.998899561377617)) ;
#10210=DIRECTION('ref_axis',(0.999092865779119,-0.00782614817623618,-0.041859251713216)) ;
#10211=DIRECTION('center_axis',(0.0420144257475537,0.0208435675618864,0.998899561377617)) ;
#10212=DIRECTION('ref_axis',(0.999092865779119,-0.00782614817623618,-0.041859251713216)) ;
#10213=DIRECTION('center_axis',(0.0420144257475537,0.0208435675618864,0.998899561377617)) ;
#10214=DIRECTION('ref_axis',(0.999092865779119,-0.00782614817623618,-0.041859251713216)) ;
#10215=DIRECTION('center_axis',(0.949966366982867,0.0212343718222273,-0.311629592713352)) ;
#10216=DIRECTION('ref_axis',(-0.311699873146483,0.,-0.950180608663672)) ;
#10217=DIRECTION('center_axis',(0.949966366982847,0.0212343718222471,-0.31162959271341)) ;
#10218=DIRECTION('ref_axis',(0.312152280468722,-0.0288488649229102,0.949593964171443)) ;
#10219=DIRECTION('center_axis',(0.0760882816615399,0.969794458779565,-0.231752629142034)) ;
#10220=DIRECTION('ref_axis',(0.950103467611678,8.48549543021553E-13,0.311934930445863)) ;
#10221=DIRECTION('center_axis',(0.0760882816615399,0.969794458779565,-0.231752629142034)) ;
#10222=DIRECTION('ref_axis',(0.950103467611678,8.48549543021553E-13,0.311934930445863)) ;
#10223=DIRECTION('center_axis',(0.0760882816615399,0.969794458779565,-0.231752629142034)) ;
#10224=DIRECTION('ref_axis',(0.950103467611678,8.48549543021553E-13,0.311934930445863)) ;
#10225=DIRECTION('center_axis',(-0.0420144257478324,0.0208435675616726,
-0.99889956137761)) ;
#10226=DIRECTION('ref_axis',(0.999092865779128,0.00782614817325717,-0.0418592517135592)) ;
#10227=DIRECTION('',(-0.0252238094988909,-2.33710244054257E-6,-0.999681829098089)) ;
#10228=DIRECTION('center_axis',(-0.0420144257474992,0.0208435675615805,
-0.998899561377626)) ;
#10229=DIRECTION('ref_axis',(0.999092865779118,0.00782614817675116,-0.0418592517131527)) ;
#10230=DIRECTION('center_axis',(-0.0420144257474992,0.0208435675615805,
-0.998899561377626)) ;
#10231=DIRECTION('ref_axis',(0.999092865779118,0.00782614817675116,-0.0418592517131527)) ;
#10232=DIRECTION('center_axis',(-0.0420144257474992,0.0208435675615805,
-0.998899561377626)) ;
#10233=DIRECTION('ref_axis',(0.999092865779118,0.00782614817675116,-0.0418592517131527)) ;
#10234=DIRECTION('center_axis',(0.950103467612781,0.,0.311934930442502)) ;
#10235=DIRECTION('ref_axis',(0.311934930442502,0.,-0.950103467612781)) ;
#10236=DIRECTION('center_axis',(-0.950103467612781,0.,-0.311934930442503)) ;
#10237=DIRECTION('ref_axis',(-0.311934930442503,0.,0.950103467612781)) ;
#154733=CARTESIAN_POINT('Origin',(-5.91338286987807,-13.4878920043255,119.207537192558)) ;
#154734=CARTESIAN_POINT('',(-5.85699395434883,-13.4607154515732,119.377580402306)) ;
#154735=CARTESIAN_POINT('Origin',(-5.8796005086299,-13.4878920043255,119.310518769832)) ;
#154736=CARTESIAN_POINT('Ctrl Pts',(-6.34456572554058,-13.1500241806476,
118.666226584225)) ;
#154737=CARTESIAN_POINT('Ctrl Pts',(-6.36725418306881,-13.1683184483544,
118.735331965087)) ;
#154738=CARTESIAN_POINT('Ctrl Pts',(-6.44105802647819,-13.1683184483544,
118.711100923369)) ;
#154739=CARTESIAN_POINT('Ctrl Pts',(-6.51486186988758,-13.1683184483544,
118.686869881651)) ;
#154740=CARTESIAN_POINT('Ctrl Pts',(-6.49217341235936,-13.1500241806476,
118.617764500789)) ;
#154741=CARTESIAN_POINT('Ctrl Pts',(-6.46948495483114,-13.1317299129408,
118.548659119927)) ;
#154742=CARTESIAN_POINT('Ctrl Pts',(-6.39568111142176,-13.1317299129408,
118.572890161645)) ;
#154743=CARTESIAN_POINT('Ctrl Pts',(-6.32187726801236,-13.1317299129408,
118.597121203363)) ;
#154744=CARTESIAN_POINT('Ctrl Pts',(-6.34456572554058,-13.1500241806476,
118.666226584225)) ;
#154745=CARTESIAN_POINT('Ctrl Pts',(-6.34529362630125,-13.1438552129684,
118.667661018198)) ;
#154746=CARTESIAN_POINT('Ctrl Pts',(-6.36794803444601,-13.1625827638083,
118.736662689976)) ;
#154747=CARTESIAN_POINT('Ctrl Pts',(-6.44175187709088,-13.1625827713816,
118.712431645929)) ;
#154748=CARTESIAN_POINT('Ctrl Pts',(-6.51555571973573,-13.1625827789549,
118.688200601882)) ;
#154749=CARTESIAN_POINT('Ctrl Pts',(-6.49290131159096,-13.143855228115,
118.619198930104)) ;
#154750=CARTESIAN_POINT('Ctrl Pts',(-6.4702469034462,-13.1251276772751,
118.550197258326)) ;
#154751=CARTESIAN_POINT('Ctrl Pts',(-6.39644306080134,-13.1251276697018,
118.574428302373)) ;
#154752=CARTESIAN_POINT('Ctrl Pts',(-6.32263921815648,-13.1251276621286,
118.59865934642)) ;
#154753=CARTESIAN_POINT('Ctrl Pts',(-6.34529362630125,-13.1438552129684,
118.667661018198)) ;
#154754=CARTESIAN_POINT('Ctrl Pts',(-6.35716264371204,-13.045472096163,
118.691303794064)) ;
#154755=CARTESIAN_POINT('Ctrl Pts',(-6.37925822797836,-13.0710887780094,
118.758603382009)) ;
#154756=CARTESIAN_POINT('Ctrl Pts',(-6.45306208999897,-13.0710886158947,
118.734372396978)) ;
#154757=CARTESIAN_POINT('Ctrl Pts',(-6.52686595201958,-13.07108845378,118.710141411947)) ;
#154758=CARTESIAN_POINT('Ctrl Pts',(-6.50477036775327,-13.0454717719336,
118.642841824001)) ;
#154759=CARTESIAN_POINT('Ctrl Pts',(-6.48267478348697,-13.0198550900872,
118.575542236056)) ;
#154760=CARTESIAN_POINT('Ctrl Pts',(-6.40887092146635,-13.0198552522019,
118.599773221087)) ;
#154761=CARTESIAN_POINT('Ctrl Pts',(-6.33506705944574,-13.0198554143166,
118.624004206118)) ;
#154762=CARTESIAN_POINT('Ctrl Pts',(-6.35716264371204,-13.045472096163,
118.691303794064)) ;
#154763=CARTESIAN_POINT('Ctrl Pts',(-6.38921314251039,-12.8597742993635,
118.764325222303)) ;
#154764=CARTESIAN_POINT('Ctrl Pts',(-6.40960406991293,-12.8983625293638,
118.826432695618)) ;
#154765=CARTESIAN_POINT('Ctrl Pts',(-6.48340790505723,-12.8983626007157,
118.802201628725)) ;
#154766=CARTESIAN_POINT('Ctrl Pts',(-6.55721174020152,-12.8983626720675,
118.777970561833)) ;
#154767=CARTESIAN_POINT('Ctrl Pts',(-6.53682081279897,-12.8597744420672,
118.715863088518)) ;
#154768=CARTESIAN_POINT('Ctrl Pts',(-6.51642988539642,-12.821186212067,
118.653755615204)) ;
#154769=CARTESIAN_POINT('Ctrl Pts',(-6.44262605025212,-12.8211861407151,
118.677986682097)) ;
#154770=CARTESIAN_POINT('Ctrl Pts',(-6.36882221510784,-12.8211860693632,
118.702217748989)) ;
#154771=CARTESIAN_POINT('Ctrl Pts',(-6.38921314251039,-12.8597742993635,
118.764325222303)) ;
#154772=CARTESIAN_POINT('Ctrl Pts',(-6.45615197626408,-12.6327839415056,
118.932852707777)) ;
#154773=CARTESIAN_POINT('Ctrl Pts',(-6.47262988951442,-12.6872840912264,
118.983041773343)) ;
#154774=CARTESIAN_POINT('Ctrl Pts',(-6.54643373625563,-12.6872840678826,
118.958810741773)) ;
#154775=CARTESIAN_POINT('Ctrl Pts',(-6.62023758299684,-12.6872840445389,
118.934579710203)) ;
#154776=CARTESIAN_POINT('Ctrl Pts',(-6.6037596697465,-12.6327838948181,
118.884390644637)) ;
#154777=CARTESIAN_POINT('Ctrl Pts',(-6.58728175649615,-12.5782837450973,
118.834201579071)) ;
#154778=CARTESIAN_POINT('Ctrl Pts',(-6.51347790975495,-12.578283768441,
118.858432610641)) ;
#154779=CARTESIAN_POINT('Ctrl Pts',(-6.43967406301373,-12.5782837917848,
118.882663642211)) ;
#154780=CARTESIAN_POINT('Ctrl Pts',(-6.45615197626408,-12.6327839415056,
118.932852707777)) ;
#154781=CARTESIAN_POINT('Ctrl Pts',(-6.53996330725217,-12.4610780963096,
119.152681494851)) ;
#154782=CARTESIAN_POINT('Ctrl Pts',(-6.55134680489055,-12.5276451730564,
119.187353792041)) ;
#154783=CARTESIAN_POINT('Ctrl Pts',(-6.62515065062138,-12.52764517241,119.163122757393)) ;
#154784=CARTESIAN_POINT('Ctrl Pts',(-6.6989544963522,-12.5276451717636,
119.138891722746)) ;
#154785=CARTESIAN_POINT('Ctrl Pts',(-6.68757099871382,-12.4610780950169,
119.104219425556)) ;
#154786=CARTESIAN_POINT('Ctrl Pts',(-6.67618750107543,-12.3945110182701,
119.069547128366)) ;
#154787=CARTESIAN_POINT('Ctrl Pts',(-6.60238365534461,-12.3945110189165,
119.093778163013)) ;
#154788=CARTESIAN_POINT('Ctrl Pts',(-6.52857980961378,-12.3945110195628,
119.11800919766)) ;
#154789=CARTESIAN_POINT('Ctrl Pts',(-6.53996330725217,-12.4610780963096,
119.152681494851)) ;
#154790=CARTESIAN_POINT('Ctrl Pts',(-6.63588982776904,-12.3578311300529,
119.409231710552)) ;
#154791=CARTESIAN_POINT('Ctrl Pts',(-6.64132916621594,-12.431704833434,
119.425799058233)) ;
#154792=CARTESIAN_POINT('Ctrl Pts',(-6.71513301565431,-12.4317048270663,
119.401568034878)) ;
#154793=CARTESIAN_POINT('Ctrl Pts',(-6.78893686509269,-12.4317048206985,
119.377337011523)) ;
#154794=CARTESIAN_POINT('Ctrl Pts',(-6.78349752664579,-12.3578311173174,
119.360769663843)) ;
#154795=CARTESIAN_POINT('Ctrl Pts',(-6.7780581881989,-12.2839574139363,
119.344202316162)) ;
#154796=CARTESIAN_POINT('Ctrl Pts',(-6.70425433876052,-12.283957420304,
119.368433339517)) ;
#154797=CARTESIAN_POINT('Ctrl Pts',(-6.63045048932215,-12.2839574266718,
119.392664362872)) ;
#154798=CARTESIAN_POINT('Ctrl Pts',(-6.63588982776904,-12.3578311300529,
119.409231710552)) ;
#154799=CARTESIAN_POINT('Ctrl Pts',(-6.736259431342,-12.3309709098726,119.679683383479)) ;
#154800=CARTESIAN_POINT('Ctrl Pts',(-6.73542828981625,-12.4068262743209,
119.677151860981)) ;
#154801=CARTESIAN_POINT('Ctrl Pts',(-6.80923214114053,-12.4068262750749,
119.65292084337)) ;
#154802=CARTESIAN_POINT('Ctrl Pts',(-6.88303599246479,-12.4068262758288,
119.62868982576)) ;
#154803=CARTESIAN_POINT('Ctrl Pts',(-6.88386713399053,-12.3309709113806,
119.631221348258)) ;
#154804=CARTESIAN_POINT('Ctrl Pts',(-6.88469827551626,-12.2551155469323,
119.633752870756)) ;
#154805=CARTESIAN_POINT('Ctrl Pts',(-6.81089442419199,-12.2551155461783,
119.657983888367)) ;
#154806=CARTESIAN_POINT('Ctrl Pts',(-6.73709057286772,-12.2551155454244,
119.682214905978)) ;
#154807=CARTESIAN_POINT('Ctrl Pts',(-6.736259431342,-12.3309709098726,119.679683383479)) ;
#154808=CARTESIAN_POINT('Ctrl Pts',(-6.83652100223137,-12.3817310335918,
119.949488204916)) ;
#154809=CARTESIAN_POINT('Ctrl Pts',(-6.82942443523005,-12.4541523823842,
119.927873207533)) ;
#154810=CARTESIAN_POINT('Ctrl Pts',(-6.90322828907729,-12.4541523921254,
119.903642197606)) ;
#154811=CARTESIAN_POINT('Ctrl Pts',(-6.97703214292451,-12.4541524018665,
119.87941118768)) ;
#154812=CARTESIAN_POINT('Ctrl Pts',(-6.98412870992583,-12.3817310530741,
119.901026185064)) ;
#154813=CARTESIAN_POINT('Ctrl Pts',(-6.99122527692713,-12.3093097042818,
119.922641182447)) ;
#154814=CARTESIAN_POINT('Ctrl Pts',(-6.9174214230799,-12.3093096945406,
119.946872192373)) ;
#154815=CARTESIAN_POINT('Ctrl Pts',(-6.84361756923268,-12.3093096847995,
119.971103202299)) ;
#154816=CARTESIAN_POINT('Ctrl Pts',(-6.83652100223137,-12.3817310335918,
119.949488204916)) ;
#154817=CARTESIAN_POINT('Ctrl Pts',(-6.92897537929249,-12.5067458714326,
120.195657155914)) ;
#154818=CARTESIAN_POINT('Ctrl Pts',(-6.91614658582664,-12.5705432422448,
120.15658272177)) ;
#154819=CARTESIAN_POINT('Ctrl Pts',(-6.98995044064887,-12.57054326527,120.132351714814)) ;
#154820=CARTESIAN_POINT('Ctrl Pts',(-7.06375429547111,-12.5705432882951,
120.108120707857)) ;
#154821=CARTESIAN_POINT('Ctrl Pts',(-7.07658308893695,-12.5067459174828,
120.147195142002)) ;
#154822=CARTESIAN_POINT('Ctrl Pts',(-7.08941188240279,-12.4429485466705,
120.186269576146)) ;
#154823=CARTESIAN_POINT('Ctrl Pts',(-7.01560802758057,-12.4429485236454,
120.210500583102)) ;
#154824=CARTESIAN_POINT('Ctrl Pts',(-6.94180417275833,-12.4429485006203,
120.234731590059)) ;
#154825=CARTESIAN_POINT('Ctrl Pts',(-6.92897537929249,-12.5067458714326,
120.195657155914)) ;
#154826=CARTESIAN_POINT('Ctrl Pts',(-7.00828982195215,-12.6971218835384,
120.401748881771)) ;
#154827=CARTESIAN_POINT('Ctrl Pts',(-6.99063912619378,-12.7477196021645,
120.347987711428)) ;
#154828=CARTESIAN_POINT('Ctrl Pts',(-7.06444298055982,-12.7477196406968,
120.323756703082)) ;
#154829=CARTESIAN_POINT('Ctrl Pts',(-7.13824683492587,-12.7477196792291,
120.299525694736)) ;
#154830=CARTESIAN_POINT('Ctrl Pts',(-7.15589753068423,-12.697121960603,
120.353286865079)) ;
#154831=CARTESIAN_POINT('Ctrl Pts',(-7.17354822644261,-12.646524241977,
120.407048035422)) ;
#154832=CARTESIAN_POINT('Ctrl Pts',(-7.09974437207656,-12.6465242034447,
120.431279043767)) ;
#154833=CARTESIAN_POINT('Ctrl Pts',(-7.02594051771052,-12.6465241649123,
120.455510052113)) ;
#154834=CARTESIAN_POINT('Ctrl Pts',(-7.00828982195215,-12.6971218835384,
120.401748881771)) ;
#154835=CARTESIAN_POINT('Ctrl Pts',(-7.06933695913004,-12.9391053860727,
120.552223222998)) ;
#154836=CARTESIAN_POINT('Ctrl Pts',(-7.04813238576582,-12.9728813246928,
120.48763751505)) ;
#154837=CARTESIAN_POINT('Ctrl Pts',(-7.1219362377198,-12.9728813789312,
120.463406499357)) ;
#154838=CARTESIAN_POINT('Ctrl Pts',(-7.19574008967378,-12.9728814331696,
120.439175483665)) ;
#154839=CARTESIAN_POINT('Ctrl Pts',(-7.21694466303801,-12.9391054945495,
120.503761191613)) ;
#154840=CARTESIAN_POINT('Ctrl Pts',(-7.23814923640224,-12.9053295559293,
120.568346899561)) ;
#154841=CARTESIAN_POINT('Ctrl Pts',(-7.16434538444827,-12.9053295016909,
120.592577915254)) ;
#154842=CARTESIAN_POINT('Ctrl Pts',(-7.09054153249427,-12.9053294474525,
120.616808930946)) ;
#154843=CARTESIAN_POINT('Ctrl Pts',(-7.06933695913004,-12.9391053860727,
120.552223222998)) ;
#154844=CARTESIAN_POINT('Ctrl Pts',(-7.10853205803656,-13.2152764852227,
120.63614997259)) ;
#154845=CARTESIAN_POINT('Ctrl Pts',(-7.08529393427628,-13.2298195844166,
120.565370398405)) ;
#154846=CARTESIAN_POINT('Ctrl Pts',(-7.1590977818874,-13.2298196519975,
120.541139369485)) ;
#154847=CARTESIAN_POINT('Ctrl Pts',(-7.2329016294985,-13.2298197195784,
120.516908340565)) ;
#154848=CARTESIAN_POINT('Ctrl Pts',(-7.25613975325877,-13.2152766203844,
120.587687914749)) ;
#154849=CARTESIAN_POINT('Ctrl Pts',(-7.27937787701905,-13.2007335211905,
120.658467488933)) ;
#154850=CARTESIAN_POINT('Ctrl Pts',(-7.20557402940794,-13.2007334536096,
120.682698517854)) ;
#154851=CARTESIAN_POINT('Ctrl Pts',(-7.13177018179683,-13.2007333860287,
120.706929546774)) ;
#154852=CARTESIAN_POINT('Ctrl Pts',(-7.10853205803656,-13.2152764852227,
120.63614997259)) ;
#154853=CARTESIAN_POINT('Ctrl Pts',(-7.12391162690117,-13.505784356226,
120.64756404441)) ;
#154854=CARTESIAN_POINT('Ctrl Pts',(-7.10029921937121,-13.5000660445819,
120.5756444624)) ;
#154855=CARTESIAN_POINT('Ctrl Pts',(-7.17410306107907,-13.5000661208921,
120.5514134155)) ;
#154856=CARTESIAN_POINT('Ctrl Pts',(-7.24790690278691,-13.5000661972022,
120.527182368599)) ;
#154857=CARTESIAN_POINT('Ctrl Pts',(-7.27151931031687,-13.5057845088464,
120.599101950609)) ;
#154858=CARTESIAN_POINT('Ctrl Pts',(-7.29513171784683,-13.5115028204905,
120.671021532619)) ;
#154859=CARTESIAN_POINT('Ctrl Pts',(-7.22132787613898,-13.5115027441803,
120.69525257952)) ;
#154860=CARTESIAN_POINT('Ctrl Pts',(-7.14752403443112,-13.5115026678702,
120.719483626421)) ;
#154861=CARTESIAN_POINT('Ctrl Pts',(-7.12391162690117,-13.505784356226,
120.64756404441)) ;
#154862=CARTESIAN_POINT('Ctrl Pts',(-7.11491785946518,-13.7916119971123,
120.584527953854)) ;
#154863=CARTESIAN_POINT('Ctrl Pts',(-7.09263642037673,-13.7659297998844,
120.516662287132)) ;
#154864=CARTESIAN_POINT('Ctrl Pts',(-7.16644025484466,-13.7659298799449,
120.492431218179)) ;
#154865=CARTESIAN_POINT('Ctrl Pts',(-7.2402440893126,-13.7659299600053,
120.468200149227)) ;
#154866=CARTESIAN_POINT('Ctrl Pts',(-7.26252552840107,-13.7916121572332,
120.53606581595)) ;
#154867=CARTESIAN_POINT('Ctrl Pts',(-7.28480696748951,-13.817294354461,
120.603931482673)) ;
#154868=CARTESIAN_POINT('Ctrl Pts',(-7.21100313302158,-13.8172942744006,
120.628162551625)) ;
#154869=CARTESIAN_POINT('Ctrl Pts',(-7.13719929855364,-13.8172941943401,
120.652393620577)) ;
#154870=CARTESIAN_POINT('Ctrl Pts',(-7.11491785946518,-13.7916119971123,
120.584527953854)) ;
#154871=CARTESIAN_POINT('Ctrl Pts',(-7.08327931847018,-14.0480477215918,
120.452871020505)) ;
#154872=CARTESIAN_POINT('Ctrl Pts',(-7.06390476968655,-14.00442476396,120.393859272724)) ;
#154873=CARTESIAN_POINT('Ctrl Pts',(-7.13770859691392,-14.0044248376781,
120.369628181718)) ;
#154874=CARTESIAN_POINT('Ctrl Pts',(-7.21151242414129,-14.0044249113963,
120.345397090713)) ;
#154875=CARTESIAN_POINT('Ctrl Pts',(-7.23088697292491,-14.0480478690281,
120.404408838494)) ;
#154876=CARTESIAN_POINT('Ctrl Pts',(-7.25026152170854,-14.0916708266599,
120.463420586275)) ;
#154877=CARTESIAN_POINT('Ctrl Pts',(-7.17645769448117,-14.0916707529417,
120.48765167728)) ;
#154878=CARTESIAN_POINT('Ctrl Pts',(-7.10265386725381,-14.0916706792236,
120.511882768286)) ;
#154879=CARTESIAN_POINT('Ctrl Pts',(-7.08327931847018,-14.0480477215918,
120.452871020505)) ;
#154880=CARTESIAN_POINT('Ctrl Pts',(-7.03177476396055,-14.2608003622883,
120.260526319525)) ;
#154881=CARTESIAN_POINT('Ctrl Pts',(-7.01670175571782,-14.2022602348381,
120.214616370291)) ;
#154882=CARTESIAN_POINT('Ctrl Pts',(-7.09050557606073,-14.2022602957698,
120.190385258316)) ;
#154883=CARTESIAN_POINT('Ctrl Pts',(-7.16430939640363,-14.2022603567015,
120.166154146341)) ;
#154884=CARTESIAN_POINT('Ctrl Pts',(-7.17938240464634,-14.2608004841518,
120.212064095575)) ;
#154885=CARTESIAN_POINT('Ctrl Pts',(-7.19445541288906,-14.319340611602,
120.25797404481)) ;
#154886=CARTESIAN_POINT('Ctrl Pts',(-7.12065159254616,-14.3193405506703,
120.282205156785)) ;
#154887=CARTESIAN_POINT('Ctrl Pts',(-7.04684777220326,-14.3193404897386,
120.306436268759)) ;
#154888=CARTESIAN_POINT('Ctrl Pts',(-7.03177476396055,-14.2608003622883,
120.260526319525)) ;
#154889=CARTESIAN_POINT('Ctrl Pts',(-6.96488777055259,-14.4130997833176,
120.021344897526)) ;
#154890=CARTESIAN_POINT('Ctrl Pts',(-6.9551961334502,-14.3438411557226,
119.991825736593)) ;
#154891=CARTESIAN_POINT('Ctrl Pts',(-7.02899994823942,-14.3438411966561,
119.967594607703)) ;
#154892=CARTESIAN_POINT('Ctrl Pts',(-7.10280376302866,-14.3438412375897,
119.943363478813)) ;
#154893=CARTESIAN_POINT('Ctrl Pts',(-7.11249540013105,-14.4130998651847,
119.972882639745)) ;
#154894=CARTESIAN_POINT('Ctrl Pts',(-7.12218703723345,-14.4823584927798,
120.002401800678)) ;
#154895=CARTESIAN_POINT('Ctrl Pts',(-7.04838322244423,-14.4823584518462,
120.026632929568)) ;
#154896=CARTESIAN_POINT('Ctrl Pts',(-6.974579407655,-14.4823584109127,120.050864058458)) ;
#154897=CARTESIAN_POINT('Ctrl Pts',(-6.96488777055259,-14.4130997833176,
120.021344897526)) ;
#154898=CARTESIAN_POINT('Ctrl Pts',(-6.88794749547868,-14.494276858583,
119.751438472986)) ;
#154899=CARTESIAN_POINT('Ctrl Pts',(-6.88434901109577,-14.419248986888,
119.740478072188)) ;
#154900=CARTESIAN_POINT('Ctrl Pts',(-6.95815282228635,-14.4192490024428,
119.716246932336)) ;
#154901=CARTESIAN_POINT('Ctrl Pts',(-7.03195663347692,-14.4192490179976,
119.692015792485)) ;
#154902=CARTESIAN_POINT('Ctrl Pts',(-7.03555511785984,-14.4942768896926,
119.702976193283)) ;
#154903=CARTESIAN_POINT('Ctrl Pts',(-7.03915360224275,-14.5693047613875,
119.713936594082)) ;
#154904=CARTESIAN_POINT('Ctrl Pts',(-6.96534979105218,-14.5693047458327,
119.738167733933)) ;
#154905=CARTESIAN_POINT('Ctrl Pts',(-6.8915459798616,-14.569304730278,119.762398873784)) ;
#154906=CARTESIAN_POINT('Ctrl Pts',(-6.88794749547868,-14.494276858583,
119.751438472986)) ;
#154907=CARTESIAN_POINT('Ctrl Pts',(-6.80764424999997,-14.4979516536895,
119.471388070987)) ;
#154908=CARTESIAN_POINT('Ctrl Pts',(-6.81038065083614,-14.4225568687656,
119.479722708482)) ;
#154909=CARTESIAN_POINT('Ctrl Pts',(-6.88418446115919,-14.4225568559479,
119.455491565989)) ;
#154910=CARTESIAN_POINT('Ctrl Pts',(-6.95798827148224,-14.4225568431301,
119.431260423495)) ;
#154911=CARTESIAN_POINT('Ctrl Pts',(-6.9552518706461,-14.497951628054,119.422925786)) ;
#154912=CARTESIAN_POINT('Ctrl Pts',(-6.95251546980995,-14.5733464129779,
119.414591148505)) ;
#154913=CARTESIAN_POINT('Ctrl Pts',(-6.87871165948689,-14.5733464257956,
119.438822290999)) ;
#154914=CARTESIAN_POINT('Ctrl Pts',(-6.80490784916383,-14.5733464386134,
119.463053433492)) ;
#154915=CARTESIAN_POINT('Ctrl Pts',(-6.80764424999997,-14.4979516536895,
119.471388070987)) ;
#154916=CARTESIAN_POINT('Ctrl Pts',(-6.73039780792071,-14.4245500702158,
119.200701305624)) ;
#154917=CARTESIAN_POINT('Ctrl Pts',(-6.73926391619148,-14.3541688694618,
119.227706042965)) ;
#154918=CARTESIAN_POINT('Ctrl Pts',(-6.81306772839461,-14.3541688284501,
119.203474906198)) ;
#154919=CARTESIAN_POINT('Ctrl Pts',(-6.88687154059774,-14.3541687874384,
119.179243769431)) ;
#154920=CARTESIAN_POINT('Ctrl Pts',(-6.87800543232696,-14.4245499881925,
119.15223903209)) ;
#154921=CARTESIAN_POINT('Ctrl Pts',(-6.86913932405619,-14.4949311889465,
119.125234294749)) ;
#154922=CARTESIAN_POINT('Ctrl Pts',(-6.79533551185306,-14.4949312299582,
119.149465431516)) ;
#154923=CARTESIAN_POINT('Ctrl Pts',(-6.72153169964993,-14.4949312709699,
119.173696568283)) ;
#154924=CARTESIAN_POINT('Ctrl Pts',(-6.73039780792071,-14.4245500702158,
119.200701305624)) ;
#154925=CARTESIAN_POINT('Ctrl Pts',(-6.66228119436863,-14.27912481409,118.957786696)) ;
#154926=CARTESIAN_POINT('Ctrl Pts',(-6.67664941802772,-14.2187925848184,
119.001549989056)) ;
#154927=CARTESIAN_POINT('Ctrl Pts',(-6.75045323468118,-14.2187925185092,
118.977318865844)) ;
#154928=CARTESIAN_POINT('Ctrl Pts',(-6.82425705133464,-14.2187924522,118.953087742632)) ;
#154929=CARTESIAN_POINT('Ctrl Pts',(-6.80988882767555,-14.2791246814716,
118.909324449576)) ;
#154930=CARTESIAN_POINT('Ctrl Pts',(-6.79552060401646,-14.3394569107431,
118.865561156519)) ;
#154931=CARTESIAN_POINT('Ctrl Pts',(-6.72171678736299,-14.3394569770523,
118.889792279731)) ;
#154932=CARTESIAN_POINT('Ctrl Pts',(-6.64791297070954,-14.3394570433615,
118.914023402943)) ;
#154933=CARTESIAN_POINT('Ctrl Pts',(-6.66228119436863,-14.27912481409,118.957786696)) ;
#154934=CARTESIAN_POINT('Ctrl Pts',(-6.60891474419106,-14.0717728276009,
118.75974735927)) ;
#154935=CARTESIAN_POINT('Ctrl Pts',(-6.62776457270004,-14.0258274816855,
118.817160897579)) ;
#154936=CARTESIAN_POINT('Ctrl Pts',(-6.70156839599648,-14.0258273955752,
118.7929297946)) ;
#154937=CARTESIAN_POINT('Ctrl Pts',(-6.7753722192929,-14.025827309465,118.768698691621)) ;
#154938=CARTESIAN_POINT('Ctrl Pts',(-6.7565223907839,-14.0717726553804,
118.711285153312)) ;
#154939=CARTESIAN_POINT('Ctrl Pts',(-6.73767256227492,-14.1177180012958,
118.653871615004)) ;
#154940=CARTESIAN_POINT('Ctrl Pts',(-6.66386873897849,-14.1177180874061,
118.678102717983)) ;
#154941=CARTESIAN_POINT('Ctrl Pts',(-6.59006491568207,-14.1177181735163,
118.702333820961)) ;
#154942=CARTESIAN_POINT('Ctrl Pts',(-6.60891474419106,-14.0717728276009,
118.75974735927)) ;
#154943=CARTESIAN_POINT('Ctrl Pts',(-6.57501586876472,-13.8168218187551,
118.62092447149)) ;
#154944=CARTESIAN_POINT('Ctrl Pts',(-6.59699661459439,-13.7886075890761,
118.687874278739)) ;
#154945=CARTESIAN_POINT('Ctrl Pts',(-6.67080044605695,-13.7886074911404,
118.663643200633)) ;
#154946=CARTESIAN_POINT('Ctrl Pts',(-6.7446042775195,-13.7886073932047,
118.639412122527)) ;
#154947=CARTESIAN_POINT('Ctrl Pts',(-6.72262353168983,-13.8168216228837,
118.572462315278)) ;
#154948=CARTESIAN_POINT('Ctrl Pts',(-6.70064278586015,-13.8450358525627,
118.505512508029)) ;
#154949=CARTESIAN_POINT('Ctrl Pts',(-6.6268389543976,-13.8450359504984,
118.529743586135)) ;
#154950=CARTESIAN_POINT('Ctrl Pts',(-6.55303512293504,-13.8450360484341,
118.553974664241)) ;
#154951=CARTESIAN_POINT('Ctrl Pts',(-6.57501586876472,-13.8168218187551,
118.62092447149)) ;
#154952=CARTESIAN_POINT('Ctrl Pts',(-6.56385556381707,-13.535324035321,
118.551622243501)) ;
#154953=CARTESIAN_POINT('Ctrl Pts',(-6.58737882351097,-13.5267213387171,
118.623270299046)) ;
#154954=CARTESIAN_POINT('Ctrl Pts',(-6.6611826635699,-13.5267212367711,
118.599039247123)) ;
#154955=CARTESIAN_POINT('Ctrl Pts',(-6.73498650362882,-13.526721134825,
118.5748081952)) ;
#154956=CARTESIAN_POINT('Ctrl Pts',(-6.71146324393492,-13.5353238314288,
118.503160139655)) ;
#154957=CARTESIAN_POINT('Ctrl Pts',(-6.68793998424103,-13.5439265280327,
118.43151208411)) ;
#154958=CARTESIAN_POINT('Ctrl Pts',(-6.61413614418211,-13.5439266299788,
118.455743136033)) ;
#154959=CARTESIAN_POINT('Ctrl Pts',(-6.54033230412318,-13.5439267319248,
118.479974187956)) ;
#154960=CARTESIAN_POINT('Ctrl Pts',(-6.56385556381707,-13.535324035321,
118.551622243501)) ;
#154961=CARTESIAN_POINT('Ctrl Pts',(-6.57670200274292,-13.2440746292406,
118.55526577413)) ;
#154962=CARTESIAN_POINT('Ctrl Pts',(-6.60009785377443,-13.2557932048074,
118.626525763366)) ;
#154963=CARTESIAN_POINT('Ctrl Pts',(-6.67390170224611,-13.2557931077727,
118.602294737067)) ;
#154964=CARTESIAN_POINT('Ctrl Pts',(-6.74770555071778,-13.2557930107381,
118.578063710768)) ;
#154965=CARTESIAN_POINT('Ctrl Pts',(-6.72430969968627,-13.2440744351713,
118.506803721532)) ;
#154966=CARTESIAN_POINT('Ctrl Pts',(-6.70091384865477,-13.2323558596045,
118.435543732295)) ;
#154967=CARTESIAN_POINT('Ctrl Pts',(-6.62711000018308,-13.2323559566392,
118.459774758594)) ;
#154968=CARTESIAN_POINT('Ctrl Pts',(-6.55330615171141,-13.2323560536738,
118.484005784893)) ;
#154969=CARTESIAN_POINT('Ctrl Pts',(-6.57670200274292,-13.2440746292406,
118.55526577413)) ;
#154970=CARTESIAN_POINT('Ctrl Pts',(-6.61375984173444,-12.9648031401168,
118.632582291307)) ;
#154971=CARTESIAN_POINT('Ctrl Pts',(-6.63533936183605,-12.9960374765742,
118.698310029483)) ;
#154972=CARTESIAN_POINT('Ctrl Pts',(-6.7091432174225,-12.9960373926029,
118.674079024855)) ;
#154973=CARTESIAN_POINT('Ctrl Pts',(-6.78294707300893,-12.9960373086315,
118.649848020226)) ;
#154974=CARTESIAN_POINT('Ctrl Pts',(-6.76136755290732,-12.964802972174,
118.58412028205)) ;
#154975=CARTESIAN_POINT('Ctrl Pts',(-6.73978803280568,-12.9335686357166,
118.518392543873)) ;
#154976=CARTESIAN_POINT('Ctrl Pts',(-6.66598417721924,-12.933568719688,
118.542623548502)) ;
#154977=CARTESIAN_POINT('Ctrl Pts',(-6.5921803216328,-12.9335688036593,
118.56685455313)) ;
#154978=CARTESIAN_POINT('Ctrl Pts',(-6.61375984173444,-12.9648031401168,
118.632582291307)) ;
#154979=CARTESIAN_POINT('Ctrl Pts',(-6.67258342631208,-12.7194345507308,
118.776404079392)) ;
#154980=CARTESIAN_POINT('Ctrl Pts',(-6.69081973876519,-12.7678470581872,
118.831948946394)) ;
#154981=CARTESIAN_POINT('Ctrl Pts',(-6.76462359980993,-12.7678469916176,
118.80771795839)) ;
#154982=CARTESIAN_POINT('Ctrl Pts',(-6.83842746085466,-12.767846925048,
118.783486970387)) ;
#154983=CARTESIAN_POINT('Ctrl Pts',(-6.82019114840154,-12.7194344175916,
118.727942103385)) ;
#154984=CARTESIAN_POINT('Ctrl Pts',(-6.80195483594844,-12.6710219101352,
118.672397236382)) ;
#154985=CARTESIAN_POINT('Ctrl Pts',(-6.72815097490371,-12.6710219767048,
118.696628224386)) ;
#154986=CARTESIAN_POINT('Ctrl Pts',(-6.65434711385897,-12.6710220432744,
118.720859212389)) ;
#154987=CARTESIAN_POINT('Ctrl Pts',(-6.67258342631208,-12.7194345507308,
118.776404079392)) ;
#154988=CARTESIAN_POINT('Ctrl Pts',(-6.75039015970557,-12.5228537207888,
118.97784552327)) ;
#154989=CARTESIAN_POINT('Ctrl Pts',(-6.76395720799441,-12.5850644655665,
119.019168564866)) ;
#154990=CARTESIAN_POINT('Ctrl Pts',(-6.83776107202866,-12.5850644207041,
118.994937585968)) ;
#154991=CARTESIAN_POINT('Ctrl Pts',(-6.91156493606291,-12.5850643758416,
118.97070660707)) ;
#154992=CARTESIAN_POINT('Ctrl Pts',(-6.89799788777407,-12.522853631064,
118.929383565474)) ;
#154993=CARTESIAN_POINT('Ctrl Pts',(-6.88443083948523,-12.4606428862864,
118.888060523877)) ;
#154994=CARTESIAN_POINT('Ctrl Pts',(-6.81062697545099,-12.4606429311488,
118.912291502775)) ;
#154995=CARTESIAN_POINT('Ctrl Pts',(-6.73682311141673,-12.4606429760112,
118.936522481673)) ;
#154996=CARTESIAN_POINT('Ctrl Pts',(-6.75039015970557,-12.5228537207888,
118.97784552327)) ;
#154997=CARTESIAN_POINT('Ctrl Pts',(-6.84171874623714,-12.3910219564108,
119.220611387595)) ;
#154998=CARTESIAN_POINT('Ctrl Pts',(-6.84966241347004,-12.4625310700348,
119.244806517688)) ;
#154999=CARTESIAN_POINT('Ctrl Pts',(-6.92346627839763,-12.4625310467126,
119.220575541511)) ;
#155000=CARTESIAN_POINT('Ctrl Pts',(-6.99727014332522,-12.4625310233905,
119.196344565334)) ;
#155001=CARTESIAN_POINT('Ctrl Pts',(-6.98932647609232,-12.3910219097665,
119.172149435241)) ;
#155002=CARTESIAN_POINT('Ctrl Pts',(-6.98138280885941,-12.3195127961425,
119.147954305148)) ;
#155003=CARTESIAN_POINT('Ctrl Pts',(-6.90757894393183,-12.3195128194647,
119.172185281325)) ;
#155004=CARTESIAN_POINT('Ctrl Pts',(-6.83377507900424,-12.3195128427868,
119.196416257502)) ;
#155005=CARTESIAN_POINT('Ctrl Pts',(-6.84171874623714,-12.3910219564108,
119.220611387595)) ;
#155006=CARTESIAN_POINT('Ctrl Pts',(-6.94152390518599,-12.3324946198483,
119.489024176868)) ;
#155007=CARTESIAN_POINT('Ctrl Pts',(-6.94324743147265,-12.408198760168,
119.494273761078)) ;
#155008=CARTESIAN_POINT('Ctrl Pts',(-7.01705129472505,-12.4081987566325,
119.470042779798)) ;
#155009=CARTESIAN_POINT('Ctrl Pts',(-7.09085515797744,-12.4081987530971,
119.445811798519)) ;
#155010=CARTESIAN_POINT('Ctrl Pts',(-7.08913163169077,-12.3324946127775,
119.440562214309)) ;
#155011=CARTESIAN_POINT('Ctrl Pts',(-7.08740810540409,-12.2567904724578,
119.435312630098)) ;
#155012=CARTESIAN_POINT('Ctrl Pts',(-7.01360424215171,-12.2567904759932,
119.459543611378)) ;
#155013=CARTESIAN_POINT('Ctrl Pts',(-6.93980037889931,-12.2567904795287,
119.483774592657)) ;
#155014=CARTESIAN_POINT('Ctrl Pts',(-6.94152390518599,-12.3324946198483,
119.489024176868)) ;
#155015=CARTESIAN_POINT('Ctrl Pts',(-7.04230587420137,-12.3517941049946,
119.760653819778)) ;
#155016=CARTESIAN_POINT('Ctrl Pts',(-7.03772653183689,-12.426265134033,
119.746705882901)) ;
#155017=CARTESIAN_POINT('Ctrl Pts',(-7.11153039244817,-12.426265145997,
119.722474893577)) ;
#155018=CARTESIAN_POINT('Ctrl Pts',(-7.18533425305945,-12.4262651579609,
119.698243904253)) ;
#155019=CARTESIAN_POINT('Ctrl Pts',(-7.18991359542393,-12.3517941289225,
119.71219184113)) ;
#155020=CARTESIAN_POINT('Ctrl Pts',(-7.19449293778842,-12.2773230998841,
119.726139778008)) ;
#155021=CARTESIAN_POINT('Ctrl Pts',(-7.12068907717713,-12.2773230879201,
119.750370767332)) ;
#155022=CARTESIAN_POINT('Ctrl Pts',(-7.04688521656585,-12.2773230759562,
119.774601756655)) ;
#155023=CARTESIAN_POINT('Ctrl Pts',(-7.04230587420137,-12.3517941049946,
119.760653819778)) ;
#155024=CARTESIAN_POINT('Ctrl Pts',(-7.13886766534031,-12.4476532719571,
120.019204540318)) ;
#155025=CARTESIAN_POINT('Ctrl Pts',(-7.12827513854447,-12.5155445566341,
119.986941413701)) ;
#155026=CARTESIAN_POINT('Ctrl Pts',(-7.2020789948579,-12.5155445785794,
119.962710411286)) ;
#155027=CARTESIAN_POINT('Ctrl Pts',(-7.27588285117132,-12.5155446005247,
119.938479408872)) ;
#155028=CARTESIAN_POINT('Ctrl Pts',(-7.28647537796717,-12.4476533158478,
119.970742535489)) ;
#155029=CARTESIAN_POINT('Ctrl Pts',(-7.297067904763,-12.3797620311708,120.003005662107)) ;
#155030=CARTESIAN_POINT('Ctrl Pts',(-7.22326404844958,-12.3797620092255,
120.027236664521)) ;
#155031=CARTESIAN_POINT('Ctrl Pts',(-7.14946019213615,-12.3797619872802,
120.051467666936)) ;
#155032=CARTESIAN_POINT('Ctrl Pts',(-7.13886766534031,-12.4476532719571,
120.019204540318)) ;
#155033=CARTESIAN_POINT('Ctrl Pts',(-7.22405843886179,-12.6128436094032,
120.24325293471)) ;
#155034=CARTESIAN_POINT('Ctrl Pts',(-7.20823477368357,-12.6693038141033,
120.195056604459)) ;
#155035=CARTESIAN_POINT('Ctrl Pts',(-7.28203862582447,-12.669303840492,
120.170825589336)) ;
#155036=CARTESIAN_POINT('Ctrl Pts',(-7.35584247796537,-12.6693038668807,
120.146594574213)) ;
#155037=CARTESIAN_POINT('Ctrl Pts',(-7.3716661431436,-12.6128436621805,
120.194790904463)) ;
#155038=CARTESIAN_POINT('Ctrl Pts',(-7.38748980832182,-12.5563834574804,
120.242987234714)) ;
#155039=CARTESIAN_POINT('Ctrl Pts',(-7.31368595618093,-12.5563834310917,
120.267218249837)) ;
#155040=CARTESIAN_POINT('Ctrl Pts',(-7.23988210404002,-12.556383404703,
120.29144926496)) ;
#155041=CARTESIAN_POINT('Ctrl Pts',(-7.22405843886179,-12.6128436094032,
120.24325293471)) ;
#155042=CARTESIAN_POINT('Ctrl Pts',(-7.29301191518833,-12.8354722898284,
120.417835047233)) ;
#155043=CARTESIAN_POINT('Ctrl Pts',(-7.27308310321733,-12.8764735343339,
120.357135102054)) ;
#155044=CARTESIAN_POINT('Ctrl Pts',(-7.34688695143518,-12.8764735602594,
120.332904074982)) ;
#155045=CARTESIAN_POINT('Ctrl Pts',(-7.42069079965303,-12.8764735861849,
120.308673047909)) ;
#155046=CARTESIAN_POINT('Ctrl Pts',(-7.44061961162404,-12.8354723416794,
120.369372993088)) ;
#155047=CARTESIAN_POINT('Ctrl Pts',(-7.46054842359504,-12.794471097174,
120.430072938267)) ;
#155048=CARTESIAN_POINT('Ctrl Pts',(-7.38674457537718,-12.7944710712485,
120.454303965339)) ;
#155049=CARTESIAN_POINT('Ctrl Pts',(-7.31294072715933,-12.794471045323,
120.478534992412)) ;
#155050=CARTESIAN_POINT('Ctrl Pts',(-7.29301191518833,-12.8354722898284,
120.417835047233)) ;
#155051=CARTESIAN_POINT('Ctrl Pts',(-7.34159724157024,-13.101408894203,
120.530187095211)) ;
#155052=CARTESIAN_POINT('Ctrl Pts',(-7.31898299520702,-13.1239035578376,
120.461307749982)) ;
#155053=CARTESIAN_POINT('Ctrl Pts',(-7.39278684027698,-13.1239035777503,
120.437076713321)) ;
#155054=CARTESIAN_POINT('Ctrl Pts',(-7.46659068534692,-13.1239035976629,
120.412845676661)) ;
#155055=CARTESIAN_POINT('Ctrl Pts',(-7.48920493171014,-13.1014089340283,
120.48172502189)) ;
#155056=CARTESIAN_POINT('Ctrl Pts',(-7.51181917807333,-13.0789142703937,
120.550604367119)) ;
#155057=CARTESIAN_POINT('Ctrl Pts',(-7.43801533300339,-13.078914250481,
120.574835403779)) ;
#155058=CARTESIAN_POINT('Ctrl Pts',(-7.36421148793344,-13.0789142305684,
120.59906644044)) ;
#155059=CARTESIAN_POINT('Ctrl Pts',(-7.34159724157024,-13.101408894203,
120.530187095211)) ;
#155060=CARTESIAN_POINT('Ctrl Pts',(-7.36657138807077,-13.3874022195482,
120.570964865022)) ;
#155061=CARTESIAN_POINT('Ctrl Pts',(-7.34290959708444,-13.3899614744304,
120.498894867778)) ;
#155062=CARTESIAN_POINT('Ctrl Pts',(-7.41671344046239,-13.389961489155,
120.474663825964)) ;
#155063=CARTESIAN_POINT('Ctrl Pts',(-7.49051728384033,-13.3899615038795,
120.45043278415)) ;
#155064=CARTESIAN_POINT('Ctrl Pts',(-7.51417907482665,-13.3874022489973,
120.522502781394)) ;
#155065=CARTESIAN_POINT('Ctrl Pts',(-7.53784086581298,-13.384842994115,
120.594572778638)) ;
#155066=CARTESIAN_POINT('Ctrl Pts',(-7.46403702243505,-13.3848429793905,
120.618803820452)) ;
#155067=CARTESIAN_POINT('Ctrl Pts',(-7.3902331790571,-13.3848429646659,
120.643034862266)) ;
#155068=CARTESIAN_POINT('Ctrl Pts',(-7.36657138807077,-13.3874022195482,
120.570964865022)) ;
#155069=CARTESIAN_POINT('Ctrl Pts',(-7.36752626591963,-13.6768759171903,
120.538418289664)) ;
#155070=CARTESIAN_POINT('Ctrl Pts',(-7.34449582013555,-13.6592264507691,
120.468271267912)) ;
#155071=CARTESIAN_POINT('Ctrl Pts',(-7.41829966275664,-13.6592264585441,
120.444040223793)) ;
#155072=CARTESIAN_POINT('Ctrl Pts',(-7.49210350537773,-13.6592264663191,
120.419809179674)) ;
#155073=CARTESIAN_POINT('Ctrl Pts',(-7.51513395116179,-13.6768759327404,
120.489956201426)) ;
#155074=CARTESIAN_POINT('Ctrl Pts',(-7.53816439694586,-13.6945253991617,
120.560103223178)) ;
#155075=CARTESIAN_POINT('Ctrl Pts',(-7.46436055432477,-13.6945253913867,
120.584334267297)) ;
#155076=CARTESIAN_POINT('Ctrl Pts',(-7.39055671170369,-13.6945253836116,
120.608565311417)) ;
#155077=CARTESIAN_POINT('Ctrl Pts',(-7.36752626591963,-13.6768759171903,
120.538418289664)) ;
#155078=CARTESIAN_POINT('Ctrl Pts',(-7.34470605061851,-13.948608493865,
120.433347699827)) ;
#155079=CARTESIAN_POINT('Ctrl Pts',(-7.32397035086195,-13.9119580024122,
120.370190104105)) ;
#155080=CARTESIAN_POINT('Ctrl Pts',(-7.39777419381241,-13.9119580041773,
120.345959060989)) ;
#155081=CARTESIAN_POINT('Ctrl Pts',(-7.47157803676287,-13.9119580059424,
120.321728017873)) ;
#155082=CARTESIAN_POINT('Ctrl Pts',(-7.49231373651943,-13.9486084973951,
120.384885613595)) ;
#155083=CARTESIAN_POINT('Ctrl Pts',(-7.51304943627599,-13.9852589888479,
120.448043209317)) ;
#155084=CARTESIAN_POINT('Ctrl Pts',(-7.43924559332553,-13.9852589870828,
120.472274252433)) ;
#155085=CARTESIAN_POINT('Ctrl Pts',(-7.36544175037507,-13.9852589853178,
120.496505295549)) ;
#155086=CARTESIAN_POINT('Ctrl Pts',(-7.34470605061851,-13.948608493865,
120.433347699827)) ;
#155087=CARTESIAN_POINT('Ctrl Pts',(-7.30074221590675,-14.181257681225,
120.264014178484)) ;
#155088=CARTESIAN_POINT('Ctrl Pts',(-7.28377855552149,-14.12830707033,120.212345606003)) ;
#155089=CARTESIAN_POINT('Ctrl Pts',(-7.35758239915043,-14.1283070692883,
120.188114564954)) ;
#155090=CARTESIAN_POINT('Ctrl Pts',(-7.43138624277937,-14.1283070682466,
120.163883523905)) ;
#155091=CARTESIAN_POINT('Ctrl Pts',(-7.44834990316463,-14.1812576791416,
120.215552096385)) ;
#155092=CARTESIAN_POINT('Ctrl Pts',(-7.46531356354989,-14.2342082900366,
120.267220668866)) ;
#155093=CARTESIAN_POINT('Ctrl Pts',(-7.39150971992095,-14.2342082910783,
120.291451709916)) ;
#155094=CARTESIAN_POINT('Ctrl Pts',(-7.31770587629201,-14.23420829212,120.315682750965)) ;
#155095=CARTESIAN_POINT('Ctrl Pts',(-7.30074221590675,-14.181257681225,
120.264014178484)) ;
#155096=CARTESIAN_POINT('Ctrl Pts',(-7.23958451504645,-14.3592650506284,
120.042343425265)) ;
#155097=CARTESIAN_POINT('Ctrl Pts',(-7.22759862181639,-14.2938058183535,
120.005836328342)) ;
#155098=CARTESIAN_POINT('Ctrl Pts',(-7.30140246605262,-14.2938058167003,
119.981605289143)) ;
#155099=CARTESIAN_POINT('Ctrl Pts',(-7.37520631028883,-14.293805815047,
119.957374249943)) ;
#155100=CARTESIAN_POINT('Ctrl Pts',(-7.38719220351889,-14.359265047322,
119.993881346865)) ;
#155101=CARTESIAN_POINT('Ctrl Pts',(-7.39917809674894,-14.4247242795969,
120.030388443787)) ;
#155102=CARTESIAN_POINT('Ctrl Pts',(-7.32537425251272,-14.4247242812501,
120.054619482987)) ;
#155103=CARTESIAN_POINT('Ctrl Pts',(-7.2515704082765,-14.4247242829034,
120.078850522187)) ;
#155104=CARTESIAN_POINT('Ctrl Pts',(-7.23958451504645,-14.3592650506284,
120.042343425265)) ;
#155105=CARTESIAN_POINT('Ctrl Pts',(-7.16614529781219,-14.4703402370834,
119.783202402502)) ;
#155106=CARTESIAN_POINT('Ctrl Pts',(-7.16000368885189,-14.3970277006435,
119.764496052493)) ;
#155107=CARTESIAN_POINT('Ctrl Pts',(-7.23380753322604,-14.3970276999611,
119.740265013713)) ;
#155108=CARTESIAN_POINT('Ctrl Pts',(-7.30761137760024,-14.3970276992787,
119.716033974934)) ;
#155109=CARTESIAN_POINT('Ctrl Pts',(-7.31375298656054,-14.4703402357187,
119.734740324943)) ;
#155110=CARTESIAN_POINT('Ctrl Pts',(-7.31989459552087,-14.5436527721586,
119.753446674952)) ;
#155111=CARTESIAN_POINT('Ctrl Pts',(-7.24609075114669,-14.543652772841,
119.777677713732)) ;
#155112=CARTESIAN_POINT('Ctrl Pts',(-7.17228690677252,-14.5436527735234,
119.801908752511)) ;
#155113=CARTESIAN_POINT('Ctrl Pts',(-7.16614529781219,-14.4703402370834,
119.783202402502)) ;
#155114=CARTESIAN_POINT('Ctrl Pts',(-7.08630537122041,-14.5059089260168,
119.504470384707)) ;
#155115=CARTESIAN_POINT('Ctrl Pts',(-7.08646558971183,-14.4300045540626,
119.504958384369)) ;
#155116=CARTESIAN_POINT('Ctrl Pts',(-7.16026943329858,-14.4300045543585,
119.480727343191)) ;
#155117=CARTESIAN_POINT('Ctrl Pts',(-7.23407327688532,-14.4300045546544,
119.456496302013)) ;
#155118=CARTESIAN_POINT('Ctrl Pts',(-7.2339130583939,-14.5059089266086,
119.456008302351)) ;
#155119=CARTESIAN_POINT('Ctrl Pts',(-7.23375283990247,-14.5818132985628,
119.455520302688)) ;
#155120=CARTESIAN_POINT('Ctrl Pts',(-7.15994899631572,-14.5818132982669,
119.479751343866)) ;
#155121=CARTESIAN_POINT('Ctrl Pts',(-7.08614515272898,-14.581813297971,
119.503982385044)) ;
#155122=CARTESIAN_POINT('Ctrl Pts',(-7.08630537122041,-14.5059089260168,
119.504470384707)) ;
#155123=CARTESIAN_POINT('Ctrl Pts',(-7.00714711584661,-14.4635906108697,
119.22798980315)) ;
#155124=CARTESIAN_POINT('Ctrl Pts',(-7.01356694457032,-14.3905302812958,
119.247543565668)) ;
#155125=CARTESIAN_POINT('Ctrl Pts',(-7.08737078700817,-14.3905302808225,
119.22331252099)) ;
#155126=CARTESIAN_POINT('Ctrl Pts',(-7.16117462944603,-14.3905302803492,
119.199081476313)) ;
#155127=CARTESIAN_POINT('Ctrl Pts',(-7.15475480072232,-14.4635906099231,
119.179527713796)) ;
#155128=CARTESIAN_POINT('Ctrl Pts',(-7.14833497199862,-14.536650939497,
119.159973951278)) ;
#155129=CARTESIAN_POINT('Ctrl Pts',(-7.07453112956076,-14.5366509399703,
119.184204995956)) ;
#155130=CARTESIAN_POINT('Ctrl Pts',(-7.0007272871229,-14.5366509404436,
119.208436040633)) ;
#155131=CARTESIAN_POINT('Ctrl Pts',(-7.00714711584661,-14.4635906108697,
119.22798980315)) ;
#155132=CARTESIAN_POINT('Ctrl Pts',(-6.9343979792678,-14.3462861335646,
118.970893409468)) ;
#155133=CARTESIAN_POINT('Ctrl Pts',(-6.94664184382201,-14.2813098903358,
119.008186245531)) ;
#155134=CARTESIAN_POINT('Ctrl Pts',(-7.02044568477505,-14.2813098862363,
118.983955196331)) ;
#155135=CARTESIAN_POINT('Ctrl Pts',(-7.0942495257281,-14.2813098821367,
118.959724147132)) ;
#155136=CARTESIAN_POINT('Ctrl Pts',(-7.0820056611739,-14.3462861253655,
118.922431311069)) ;
#155137=CARTESIAN_POINT('Ctrl Pts',(-7.06976179661971,-14.4112623685942,
118.885138475006)) ;
#155138=CARTESIAN_POINT('Ctrl Pts',(-6.99595795566666,-14.4112623726938,
118.909369524205)) ;
#155139=CARTESIAN_POINT('Ctrl Pts',(-6.9221541147136,-14.4112623767934,
118.933600573405)) ;
#155140=CARTESIAN_POINT('Ctrl Pts',(-6.9343979792678,-14.3462861335646,
118.970893409468)) ;
#155141=CARTESIAN_POINT('Ctrl Pts',(-6.87439561306881,-14.1620807273187,
118.752616009014)) ;
#155142=CARTESIAN_POINT('Ctrl Pts',(-6.8915819369104,-14.1098718676652,
118.804962778742)) ;
#155143=CARTESIAN_POINT('Ctrl Pts',(-6.96538577675959,-14.1098718563613,
118.780731726181)) ;
#155144=CARTESIAN_POINT('Ctrl Pts',(-7.03918961660877,-14.1098718450575,
118.756500673619)) ;
#155145=CARTESIAN_POINT('Ctrl Pts',(-7.02200329276718,-14.162080704711,
118.70415390389)) ;
#155146=CARTESIAN_POINT('Ctrl Pts',(-7.00481696892557,-14.2142895643646,
118.651807134161)) ;
#155147=CARTESIAN_POINT('Ctrl Pts',(-6.9310131290764,-14.2142895756684,
118.676038186723)) ;
#155148=CARTESIAN_POINT('Ctrl Pts',(-6.8572092892272,-14.2142895869723,
118.700269239285)) ;
#155149=CARTESIAN_POINT('Ctrl Pts',(-6.87439561306881,-14.1620807273187,
118.752616009014)) ;
#155150=CARTESIAN_POINT('Ctrl Pts',(-6.83231279792918,-13.9257450561724,
118.589088105333)) ;
#155151=CARTESIAN_POINT('Ctrl Pts',(-6.85319376491815,-13.8899621379748,
118.652688162088)) ;
#155152=CARTESIAN_POINT('Ctrl Pts',(-6.92699760485068,-13.8899621182589,
118.62845710978)) ;
#155153=CARTESIAN_POINT('Ctrl Pts',(-7.0008014447832,-13.889962098543,118.604226057471)) ;
#155154=CARTESIAN_POINT('Ctrl Pts',(-6.97992047779423,-13.9257450167406,
118.540626000717)) ;
#155155=CARTESIAN_POINT('Ctrl Pts',(-6.95903951080526,-13.9615279349381,
118.477025943963)) ;
#155156=CARTESIAN_POINT('Ctrl Pts',(-6.88523567087274,-13.961527954654,
118.501256996271)) ;
#155157=CARTESIAN_POINT('Ctrl Pts',(-6.81143183094022,-13.9615279743699,
118.525488048579)) ;
#155158=CARTESIAN_POINT('Ctrl Pts',(-6.83231279792918,-13.9257450561724,
118.589088105333)) ;
#155159=CARTESIAN_POINT('Ctrl Pts',(-6.81152149947454,-13.6518932520307,
118.490235528419)) ;
#155160=CARTESIAN_POINT('Ctrl Pts',(-6.83461955364127,-13.6351791904555,
118.560588475159)) ;
#155161=CARTESIAN_POINT('Ctrl Pts',(-6.90842339470331,-13.6351791600229,
118.536357426292)) ;
#155162=CARTESIAN_POINT('Ctrl Pts',(-6.98222723576535,-13.6351791295903,
118.512126377424)) ;
#155163=CARTESIAN_POINT('Ctrl Pts',(-6.95912918159862,-13.6518931911655,
118.441773430683)) ;
#155164=CARTESIAN_POINT('Ctrl Pts',(-6.93603112743188,-13.6686072527407,
118.371420483943)) ;
#155165=CARTESIAN_POINT('Ctrl Pts',(-6.86222728636984,-13.6686072831733,
118.395651532811)) ;
#155166=CARTESIAN_POINT('Ctrl Pts',(-6.78842344530779,-13.6686073136059,
118.419882581678)) ;
#155167=CARTESIAN_POINT('Ctrl Pts',(-6.81152149947454,-13.6518932520307,
118.490235528419)) ;
#155168=CARTESIAN_POINT('Ctrl Pts',(-6.81458866379034,-13.361350209501,
118.464074361768)) ;
#155169=CARTESIAN_POINT('Ctrl Pts',(-6.83824065261878,-13.3648978107094,
118.536114504284)) ;
#155170=CARTESIAN_POINT('Ctrl Pts',(-6.91204449644649,-13.3648977704052,
118.51188346384)) ;
#155171=CARTESIAN_POINT('Ctrl Pts',(-6.9858483402742,-13.364897730101,118.487652423396)) ;
#155172=CARTESIAN_POINT('Ctrl Pts',(-6.96219635144575,-13.3613501288926,
118.41561228088)) ;
#155173=CARTESIAN_POINT('Ctrl Pts',(-6.9385443626173,-13.3578025276842,
118.343572138364)) ;
#155174=CARTESIAN_POINT('Ctrl Pts',(-6.86474051878959,-13.3578025679884,
118.367803178808)) ;
#155175=CARTESIAN_POINT('Ctrl Pts',(-6.79093667496188,-13.3578026082926,
118.392034219252)) ;
#155176=CARTESIAN_POINT('Ctrl Pts',(-6.81458866379034,-13.361350209501,
118.464074361768)) ;
#155177=CARTESIAN_POINT('Ctrl Pts',(-6.84190912425954,-13.0754523993138,
118.511850887542)) ;
#155178=CARTESIAN_POINT('Ctrl Pts',(-6.86442104202547,-13.0989663539562,
118.580418557715)) ;
#155179=CARTESIAN_POINT('Ctrl Pts',(-6.93822489001608,-13.0989663074807,
118.556187529951)) ;
#155180=CARTESIAN_POINT('Ctrl Pts',(-7.01202873800668,-13.0989662610053,
118.531956502186)) ;
#155181=CARTESIAN_POINT('Ctrl Pts',(-6.98951682024076,-13.0754523063629,
118.463388832014)) ;
#155182=CARTESIAN_POINT('Ctrl Pts',(-6.96700490247481,-13.0519383517206,
118.394821161841)) ;
#155183=CARTESIAN_POINT('Ctrl Pts',(-6.89320105448421,-13.051938398196,
118.419052189605)) ;
#155184=CARTESIAN_POINT('Ctrl Pts',(-6.8193972064936,-13.0519384446715,
118.44328321737)) ;
#155185=CARTESIAN_POINT('Ctrl Pts',(-6.84190912425954,-13.0754523993138,
118.511850887542)) ;
#155186=CARTESIAN_POINT('Ctrl Pts',(-6.89221998106671,-12.8139381990977,
118.629651920743)) ;
#155187=CARTESIAN_POINT('Ctrl Pts',(-6.91198505624896,-12.8557446579336,
118.68985315177)) ;
#155188=CARTESIAN_POINT('Ctrl Pts',(-6.98578890934624,-12.8557446099044,
118.66562213956)) ;
#155189=CARTESIAN_POINT('Ctrl Pts',(-7.05959276244351,-12.8557445618753,
118.641391127349)) ;
#155190=CARTESIAN_POINT('Ctrl Pts',(-7.03982768726127,-12.8139381030394,
118.581189896322)) ;
#155191=CARTESIAN_POINT('Ctrl Pts',(-7.02006261207903,-12.7721316442036,
118.520988665295)) ;
#155192=CARTESIAN_POINT('Ctrl Pts',(-6.94625875898175,-12.7721316922327,
118.545219677506)) ;
#155193=CARTESIAN_POINT('Ctrl Pts',(-6.87245490588448,-12.7721317402619,
118.569450689716)) ;
#155194=CARTESIAN_POINT('Ctrl Pts',(-6.89221998106671,-12.8139381990977,
118.629651920743)) ;
#155195=CARTESIAN_POINT('Ctrl Pts',(-6.96317166541847,-12.5948180944483,
118.810143346469)) ;
#155196=CARTESIAN_POINT('Ctrl Pts',(-6.97874870279201,-12.6519838381849,
118.857588490258)) ;
#155197=CARTESIAN_POINT('Ctrl Pts',(-7.05255256187162,-12.6519837938663,
118.833357496269)) ;
#155198=CARTESIAN_POINT('Ctrl Pts',(-7.12635642095122,-12.6519837495477,
118.80912650228)) ;
#155199=CARTESIAN_POINT('Ctrl Pts',(-7.11077938357767,-12.5948180058111,
118.761681358491)) ;
#155200=CARTESIAN_POINT('Ctrl Pts',(-7.09520234620412,-12.5376522620745,
118.714236214702)) ;
#155201=CARTESIAN_POINT('Ctrl Pts',(-7.02139848712452,-12.537652306393,
118.738467208691)) ;
#155202=CARTESIAN_POINT('Ctrl Pts',(-6.94759462804491,-12.5376523507116,
118.76269820268)) ;
#155203=CARTESIAN_POINT('Ctrl Pts',(-6.96317166541847,-12.5948180944483,
118.810143346469)) ;
#155204=CARTESIAN_POINT('Ctrl Pts',(-7.04930238281719,-12.4362800048722,
119.037190426179)) ;
#155205=CARTESIAN_POINT('Ctrl Pts',(-7.05961869911306,-12.5045968794166,
119.068612262503)) ;
#155206=CARTESIAN_POINT('Ctrl Pts',(-7.13342256311478,-12.5045968472639,
119.044381283506)) ;
#155207=CARTESIAN_POINT('Ctrl Pts',(-7.20722642711649,-12.5045968151111,
119.020150304509)) ;
#155208=CARTESIAN_POINT('Ctrl Pts',(-7.19691011082063,-12.4362799405667,
118.988728468185)) ;
#155209=CARTESIAN_POINT('Ctrl Pts',(-7.18659379452477,-12.3679630660223,
118.95730663186)) ;
#155210=CARTESIAN_POINT('Ctrl Pts',(-7.11278993052304,-12.367963098175,
118.981537610857)) ;
#155211=CARTESIAN_POINT('Ctrl Pts',(-7.03898606652133,-12.3679631303278,
119.005768589854)) ;
#155212=CARTESIAN_POINT('Ctrl Pts',(-7.04930238281719,-12.4362800048722,
119.037190426179)) ;
#155213=CARTESIAN_POINT('Ctrl Pts',(-7.14639896583729,-12.346922078608,
119.29741677471)) ;
#155214=CARTESIAN_POINT('Ctrl Pts',(-7.15068612719803,-12.4215768384595,
119.310474778056)) ;
#155215=CARTESIAN_POINT('Ctrl Pts',(-7.22448999554273,-12.4215768235296,
119.286243812287)) ;
#155216=CARTESIAN_POINT('Ctrl Pts',(-7.29829386388744,-12.4215768085998,
119.262012846518)) ;
#155217=CARTESIAN_POINT('Ctrl Pts',(-7.2940067025267,-12.3469220487482,
119.248954843172)) ;
#155218=CARTESIAN_POINT('Ctrl Pts',(-7.28971954116596,-12.2722672888967,
119.235896839826)) ;
#155219=CARTESIAN_POINT('Ctrl Pts',(-7.21591567282126,-12.2722673038266,
119.260127805595)) ;
#155220=CARTESIAN_POINT('Ctrl Pts',(-7.14211180447654,-12.2722673187564,
119.284358771364)) ;
#155221=CARTESIAN_POINT('Ctrl Pts',(-7.14639896583729,-12.346922078608,
119.29741677471)) ;
#155222=CARTESIAN_POINT('Ctrl Pts',(-7.24765406779605,-12.3346186385411,
119.570362985162)) ;
#155223=CARTESIAN_POINT('Ctrl Pts',(-7.24561188999,-12.4102408597983,119.56414284277)) ;
#155224=CARTESIAN_POINT('Ctrl Pts',(-7.3194157607563,-12.4102408673589,
119.539911884376)) ;
#155225=CARTESIAN_POINT('Ctrl Pts',(-7.3932196315226,-12.4102408749196,
119.515680925983)) ;
#155226=CARTESIAN_POINT('Ctrl Pts',(-7.39526180932864,-12.3346186536624,
119.521901068375)) ;
#155227=CARTESIAN_POINT('Ctrl Pts',(-7.3973039871347,-12.2589964324052,
119.528121210767)) ;
#155228=CARTESIAN_POINT('Ctrl Pts',(-7.3235001163684,-12.2589964248446,
119.55235216916)) ;
#155229=CARTESIAN_POINT('Ctrl Pts',(-7.24969624560211,-12.2589964172839,
119.576583127554)) ;
#155230=CARTESIAN_POINT('Ctrl Pts',(-7.24765406779605,-12.3346186385411,
119.570362985162)) ;
#155231=CARTESIAN_POINT('Ctrl Pts',(-7.34665382402801,-12.3998225687949,
119.836445852581)) ;
#155232=CARTESIAN_POINT('Ctrl Pts',(-7.33843046780754,-12.4710025852177,
119.811398838181)) ;
#155233=CARTESIAN_POINT('Ctrl Pts',(-7.41223433866837,-12.4710026178869,
119.787167880076)) ;
#155234=CARTESIAN_POINT('Ctrl Pts',(-7.48603820952917,-12.4710026505561,
119.762936921971)) ;
#155235=CARTESIAN_POINT('Ctrl Pts',(-7.49426156574964,-12.3998226341332,
119.78798393637)) ;
#155236=CARTESIAN_POINT('Ctrl Pts',(-7.5024849219701,-12.3286426177104,
119.81303095077)) ;
#155237=CARTESIAN_POINT('Ctrl Pts',(-7.42868105110929,-12.3286425850412,
119.837261908875)) ;
#155238=CARTESIAN_POINT('Ctrl Pts',(-7.35487718024847,-12.328642552372,
119.861492866981)) ;
#155239=CARTESIAN_POINT('Ctrl Pts',(-7.34665382402801,-12.3998225687949,
119.836445852581)) ;
#155240=CARTESIAN_POINT('Ctrl Pts',(-7.4370740592955,-12.5378477500096,
120.076408147661)) ;
#155241=CARTESIAN_POINT('Ctrl Pts',(-7.42325927266372,-12.599495230749,
120.034330538498)) ;
#155242=CARTESIAN_POINT('Ctrl Pts',(-7.497063141071,-12.5994952885301,120.01009957292)) ;
#155243=CARTESIAN_POINT('Ctrl Pts',(-7.57086700947827,-12.5994953463112,
119.985868607341)) ;
#155244=CARTESIAN_POINT('Ctrl Pts',(-7.58468179611005,-12.5378478655717,
120.027946216505)) ;
#155245=CARTESIAN_POINT('Ctrl Pts',(-7.59849658274182,-12.4762003848323,
120.070023825668)) ;
#155246=CARTESIAN_POINT('Ctrl Pts',(-7.52469271433454,-12.4762003270512,
120.094254791246)) ;
#155247=CARTESIAN_POINT('Ctrl Pts',(-7.45088884592727,-12.4762002692701,
120.118485756825)) ;
#155248=CARTESIAN_POINT('Ctrl Pts',(-7.4370740592955,-12.5378477500096,
120.076408147661)) ;
#155249=CARTESIAN_POINT('Ctrl Pts',(-7.5133452204639,-12.7392396507352,
120.273212489585)) ;
#155250=CARTESIAN_POINT('Ctrl Pts',(-7.49491989486196,-12.7869171442881,
120.217091922708)) ;
#155251=CARTESIAN_POINT('Ctrl Pts',(-7.56872375838898,-12.7869172246325,
120.192860942265)) ;
#155252=CARTESIAN_POINT('Ctrl Pts',(-7.64252762191598,-12.786917304977,
120.168629961822)) ;
#155253=CARTESIAN_POINT('Ctrl Pts',(-7.66095294751793,-12.7392398114241,
120.2247505287)) ;
#155254=CARTESIAN_POINT('Ctrl Pts',(-7.67937827311986,-12.6915623178712,
120.280871095577)) ;
#155255=CARTESIAN_POINT('Ctrl Pts',(-7.60557440959285,-12.6915622375267,
120.30510207602)) ;
#155256=CARTESIAN_POINT('Ctrl Pts',(-7.53177054606584,-12.6915621571823,
120.329333056462)) ;
#155257=CARTESIAN_POINT('Ctrl Pts',(-7.5133452204639,-12.7392396507352,
120.273212489585)) ;
#155258=CARTESIAN_POINT('Ctrl Pts',(-7.57051158312834,-12.989236405783,
120.411850909373)) ;
#155259=CARTESIAN_POINT('Ctrl Pts',(-7.54880219935677,-13.019530175167,
120.345727631249)) ;
#155260=CARTESIAN_POINT('Ctrl Pts',(-7.62260605583471,-13.019530272485,
120.321496629336)) ;
#155261=CARTESIAN_POINT('Ctrl Pts',(-7.69640991231264,-13.0195303698031,
120.297265627423)) ;
#155262=CARTESIAN_POINT('Ctrl Pts',(-7.71811929608421,-12.9892366004191,
120.363388905547)) ;
#155263=CARTESIAN_POINT('Ctrl Pts',(-7.7398286798558,-12.9589428310352,
120.429512183671)) ;
#155264=CARTESIAN_POINT('Ctrl Pts',(-7.66602482337786,-12.9589427337171,
120.453743185585)) ;
#155265=CARTESIAN_POINT('Ctrl Pts',(-7.59222096689992,-12.9589426363991,
120.477974187498)) ;
#155266=CARTESIAN_POINT('Ctrl Pts',(-7.57051158312834,-12.989236405783,
120.411850909373)) ;
#155267=CARTESIAN_POINT('Ctrl Pts',(-7.60526793750275,-13.269049028932,
120.482338834054)) ;
#155268=CARTESIAN_POINT('Ctrl Pts',(-7.58183203791737,-13.279851801729,
120.410956867366)) ;
#155269=CARTESIAN_POINT('Ctrl Pts',(-7.65563588594552,-13.2798519083315,
120.386725839716)) ;
#155270=CARTESIAN_POINT('Ctrl Pts',(-7.7294397339737,-13.279852014934,120.362494812066)) ;
#155271=CARTESIAN_POINT('Ctrl Pts',(-7.75287563355908,-13.269049242137,
120.433876778754)) ;
#155272=CARTESIAN_POINT('Ctrl Pts',(-7.77631153314448,-13.2582464693401,
120.505258745443)) ;
#155273=CARTESIAN_POINT('Ctrl Pts',(-7.7025076851163,-13.2582463627375,
120.529489773093)) ;
#155274=CARTESIAN_POINT('Ctrl Pts',(-7.62870383708814,-13.258246256135,
120.553720800743)) ;
#155275=CARTESIAN_POINT('Ctrl Pts',(-7.60526793750275,-13.269049028932,
120.482338834054)) ;
#155276=CARTESIAN_POINT('Ctrl Pts',(-7.61610217928452,-13.560604521515,
120.479829556645)) ;
#155277=CARTESIAN_POINT('Ctrl Pts',(-7.59260992748901,-13.5510680943663,
120.408275950233)) ;
#155278=CARTESIAN_POINT('Ctrl Pts',(-7.66641376645151,-13.5510682019353,
120.384044894971)) ;
#155279=CARTESIAN_POINT('Ctrl Pts',(-7.74021760541402,-13.5510683095042,
120.359813839708)) ;
#155280=CARTESIAN_POINT('Ctrl Pts',(-7.76370985720953,-13.5606047366529,
120.43136744612)) ;
#155281=CARTESIAN_POINT('Ctrl Pts',(-7.78720210900504,-13.5701411638016,
120.502921052531)) ;
#155282=CARTESIAN_POINT('Ctrl Pts',(-7.71339827004254,-13.5701410562327,
120.527152107794)) ;
#155283=CARTESIAN_POINT('Ctrl Pts',(-7.63959443108004,-13.5701409486637,
120.551383163056)) ;
#155284=CARTESIAN_POINT('Ctrl Pts',(-7.61610217928452,-13.560604521515,
120.479829556645)) ;
#155285=CARTESIAN_POINT('Ctrl Pts',(-7.60265701261583,-13.8423158077137,
120.4033105886)) ;
#155286=CARTESIAN_POINT('Ctrl Pts',(-7.58080443900952,-13.8130971975032,
120.33675117738)) ;
#155287=CARTESIAN_POINT('Ctrl Pts',(-7.65460826925647,-13.8130972967894,
120.312520095571)) ;
#155288=CARTESIAN_POINT('Ctrl Pts',(-7.72841209950342,-13.8130973960757,
120.288289013763)) ;
#155289=CARTESIAN_POINT('Ctrl Pts',(-7.75026467310974,-13.8423160062862,
120.354848424983)) ;
#155290=CARTESIAN_POINT('Ctrl Pts',(-7.77211724671606,-13.8715346164967,
120.421407836203)) ;
#155291=CARTESIAN_POINT('Ctrl Pts',(-7.6983134164691,-13.8715345172104,
120.445638918011)) ;
#155292=CARTESIAN_POINT('Ctrl Pts',(-7.62450958622215,-13.8715344179242,
120.46986999982)) ;
#155293=CARTESIAN_POINT('Ctrl Pts',(-7.60265701261583,-13.8423158077137,
120.4033105886)) ;
#155294=CARTESIAN_POINT('Ctrl Pts',(-7.56703031046435,-14.0920492190499,
120.259455200578)) ;
#155295=CARTESIAN_POINT('Ctrl Pts',(-7.5483639780729,-14.0453516515009,
120.202600565973)) ;
#155296=CARTESIAN_POINT('Ctrl Pts',(-7.62216780084486,-14.0453517349523,
120.178369461397)) ;
#155297=CARTESIAN_POINT('Ctrl Pts',(-7.69597162361682,-14.0453518184037,
120.154138356821)) ;
#155298=CARTESIAN_POINT('Ctrl Pts',(-7.71463795600827,-14.0920493859528,
120.210992991425)) ;
#155299=CARTESIAN_POINT('Ctrl Pts',(-7.73330428839972,-14.1387469535018,
120.26784762603)) ;
#155300=CARTESIAN_POINT('Ctrl Pts',(-7.65950046562776,-14.1387468700504,
120.292078730606)) ;
#155301=CARTESIAN_POINT('Ctrl Pts',(-7.5856966428558,-14.138746786599,120.316309835182)) ;
#155302=CARTESIAN_POINT('Ctrl Pts',(-7.56703031046435,-14.0920492190499,
120.259455200578)) ;
#155303=CARTESIAN_POINT('Ctrl Pts',(-7.51204303377268,-14.2950965364046,
120.056387264096)) ;
#155304=CARTESIAN_POINT('Ctrl Pts',(-7.49792407955998,-14.2341530477557,
120.013383209649)) ;
#155305=CARTESIAN_POINT('Ctrl Pts',(-7.57172789688386,-14.2341531086755,
119.989152088479)) ;
#155306=CARTESIAN_POINT('Ctrl Pts',(-7.64553171420774,-14.2341531695953,
119.964920967308)) ;
#155307=CARTESIAN_POINT('Ctrl Pts',(-7.65965066842044,-14.2950966582441,
120.007925021756)) ;
#155308=CARTESIAN_POINT('Ctrl Pts',(-7.67376962263314,-14.3560401468929,
120.050929076204)) ;
#155309=CARTESIAN_POINT('Ctrl Pts',(-7.59996580530926,-14.3560400859732,
120.075160197374)) ;
#155310=CARTESIAN_POINT('Ctrl Pts',(-7.52616198798538,-14.3560400250534,
120.099391318544)) ;
#155311=CARTESIAN_POINT('Ctrl Pts',(-7.51204303377268,-14.2950965364046,
120.056387264096)) ;
#155312=CARTESIAN_POINT('Ctrl Pts',(-7.44273831121475,-14.434335219557,
119.809815786678)) ;
#155313=CARTESIAN_POINT('Ctrl Pts',(-7.43417104149911,-14.3635791231233,
119.783721267369)) ;
#155314=CARTESIAN_POINT('Ctrl Pts',(-7.50797485590469,-14.3635791582218,
119.75949013731)) ;
#155315=CARTESIAN_POINT('Ctrl Pts',(-7.58177867031028,-14.3635791933204,
119.735259007251)) ;
#155316=CARTESIAN_POINT('Ctrl Pts',(-7.59034594002593,-14.4343352897541,
119.76135352656)) ;
#155317=CARTESIAN_POINT('Ctrl Pts',(-7.59891320974157,-14.5050913861879,
119.787448045869)) ;
#155318=CARTESIAN_POINT('Ctrl Pts',(-7.52510939533598,-14.5050913510893,
119.811679175928)) ;
#155319=CARTESIAN_POINT('Ctrl Pts',(-7.45130558093039,-14.5050913159907,
119.835910305987)) ;
#155320=CARTESIAN_POINT('Ctrl Pts',(-7.44273831121475,-14.434335219557,
119.809815786678)) ;
#155321=CARTESIAN_POINT('Ctrl Pts',(-7.36521040000063,-14.5007530721094,
119.538381721836)) ;
#155322=CARTESIAN_POINT('Ctrl Pts',(-7.36277354008315,-14.4252541131167,
119.530959441559)) ;
#155323=CARTESIAN_POINT('Ctrl Pts',(-7.4365773538254,-14.4252541219683,
119.50672830948)) ;
#155324=CARTESIAN_POINT('Ctrl Pts',(-7.51038116756764,-14.4252541308198,
119.482497177401)) ;
#155325=CARTESIAN_POINT('Ctrl Pts',(-7.51281802748512,-14.5007530898126,
119.489919457677)) ;
#155326=CARTESIAN_POINT('Ctrl Pts',(-7.51525488740261,-14.5762520488053,
119.497341737954)) ;
#155327=CARTESIAN_POINT('Ctrl Pts',(-7.44145107366037,-14.5762520399537,
119.521572870033)) ;
#155328=CARTESIAN_POINT('Ctrl Pts',(-7.36764725991812,-14.5762520311022,
119.545804002113)) ;
#155329=CARTESIAN_POINT('Ctrl Pts',(-7.36521040000063,-14.5007530721094,
119.538381721836)) ;
#155330=CARTESIAN_POINT('Ctrl Pts',(-7.28479809434297,-14.4901437351793,
119.257926243117)) ;
#155331=CARTESIAN_POINT('Ctrl Pts',(-7.28870699471344,-14.415271701562,
119.269832124676)) ;
#155332=CARTESIAN_POINT('Ctrl Pts',(-7.36251081065682,-14.4152716856427,
119.245600999301)) ;
#155333=CARTESIAN_POINT('Ctrl Pts',(-7.43631462660021,-14.4152716697234,
119.221369873926)) ;
#155334=CARTESIAN_POINT('Ctrl Pts',(-7.43240572622976,-14.4901437033406,
119.209463992367)) ;
#155335=CARTESIAN_POINT('Ctrl Pts',(-7.42849682585929,-14.5650157369579,
119.197558110808)) ;
#155336=CARTESIAN_POINT('Ctrl Pts',(-7.3546930099159,-14.5650157528772,
119.221789236183)) ;
#155337=CARTESIAN_POINT('Ctrl Pts',(-7.28088919397251,-14.5650157687965,
119.246020361558)) ;
#155338=CARTESIAN_POINT('Ctrl Pts',(-7.28479809434297,-14.4901437351793,
119.257926243117)) ;
#155339=CARTESIAN_POINT('Ctrl Pts',(-7.20843821052364,-14.402041943339,
118.989761053497)) ;
#155340=CARTESIAN_POINT('Ctrl Pts',(-7.21842069556288,-14.3332076954044,
119.020166093841)) ;
#155341=CARTESIAN_POINT('Ctrl Pts',(-7.29222451596317,-14.3332076598222,
118.995934982041)) ;
#155342=CARTESIAN_POINT('Ctrl Pts',(-7.36602833636344,-14.33320762424,118.971703870241)) ;
#155343=CARTESIAN_POINT('Ctrl Pts',(-7.3560458513242,-14.4020418721746,
118.941298829897)) ;
#155344=CARTESIAN_POINT('Ctrl Pts',(-7.34606336628494,-14.4708761201093,
118.910893789552)) ;
#155345=CARTESIAN_POINT('Ctrl Pts',(-7.27225954588466,-14.4708761556915,
118.935124901352)) ;
#155346=CARTESIAN_POINT('Ctrl Pts',(-7.19845572548438,-14.4708761912736,
118.959356013152)) ;
#155347=CARTESIAN_POINT('Ctrl Pts',(-7.20843821052364,-14.402041943339,
118.989761053497)) ;
#155348=CARTESIAN_POINT('Ctrl Pts',(-7.1427835920666,-14.243691286176,118.754343222241)) ;
#155349=CARTESIAN_POINT('Ctrl Pts',(-7.15809856623828,-14.18580899599,118.800990163949)) ;
#155350=CARTESIAN_POINT('Ctrl Pts',(-7.23190239210298,-14.1858089469242,
118.776759068792)) ;
#155351=CARTESIAN_POINT('Ctrl Pts',(-7.30570621796767,-14.1858088978584,
118.752527973636)) ;
#155352=CARTESIAN_POINT('Ctrl Pts',(-7.290391243796,-14.2436911880444,118.705881031928)) ;
#155353=CARTESIAN_POINT('Ctrl Pts',(-7.27507626962433,-14.3015734782304,
118.659234090221)) ;
#155354=CARTESIAN_POINT('Ctrl Pts',(-7.20127244375963,-14.3015735272962,
118.683465185377)) ;
#155355=CARTESIAN_POINT('Ctrl Pts',(-7.12746861789493,-14.301573576362,
118.707696280533)) ;
#155356=CARTESIAN_POINT('Ctrl Pts',(-7.1427835920666,-14.243691286176,118.754343222241)) ;
#155357=CARTESIAN_POINT('Ctrl Pts',(-7.09305076334606,-14.0272168477211,
118.567541759605)) ;
#155358=CARTESIAN_POINT('Ctrl Pts',(-7.11259210256672,-13.9843615039812,
118.627061527202)) ;
#155359=CARTESIAN_POINT('Ctrl Pts',(-7.18639593427092,-13.9843614472663,
118.602830449832)) ;
#155360=CARTESIAN_POINT('Ctrl Pts',(-7.26019976597513,-13.9843613905514,
118.578599372462)) ;
#155361=CARTESIAN_POINT('Ctrl Pts',(-7.24065842675446,-14.0272167342913,
118.519079604865)) ;
#155362=CARTESIAN_POINT('Ctrl Pts',(-7.22111708753381,-14.0700720780313,
118.459559837268)) ;
#155363=CARTESIAN_POINT('Ctrl Pts',(-7.1473132558296,-14.0700721347462,
118.483790914638)) ;
#155364=CARTESIAN_POINT('Ctrl Pts',(-7.0735094241254,-14.0700721914611,
118.508021992008)) ;
#155365=CARTESIAN_POINT('Ctrl Pts',(-7.09305076334606,-14.0272168477211,
118.567541759605)) ;
#155366=CARTESIAN_POINT('Ctrl Pts',(-7.06320365437595,-13.7664028194368,
118.441170630651)) ;
#155367=CARTESIAN_POINT('Ctrl Pts',(-7.08559233431929,-13.7416926429616,
118.509362938513)) ;
#155368=CARTESIAN_POINT('Ctrl Pts',(-7.15939617199936,-13.7416925860971,
118.485131879344)) ;
#155369=CARTESIAN_POINT('Ctrl Pts',(-7.23320000967943,-13.7416925292327,
118.460900820176)) ;
#155370=CARTESIAN_POINT('Ctrl Pts',(-7.21081132973608,-13.7664027057079,
118.392708512314)) ;
#155371=CARTESIAN_POINT('Ctrl Pts',(-7.18842264979274,-13.791112882183,
118.324516204452)) ;
#155372=CARTESIAN_POINT('Ctrl Pts',(-7.11461881211266,-13.7911129390475,
118.348747263621)) ;
#155373=CARTESIAN_POINT('Ctrl Pts',(-7.0408149744326,-13.7911129959119,
118.37297832279)) ;
#155374=CARTESIAN_POINT('Ctrl Pts',(-7.06320365437595,-13.7664028194368,
118.441170630651)) ;
#155375=CARTESIAN_POINT('Ctrl Pts',(-7.05638533636368,-13.4798811075686,
118.384860283325)) ;
#155376=CARTESIAN_POINT('Ctrl Pts',(-7.08001960465576,-13.4751386073872,
118.456846452141)) ;
#155377=CARTESIAN_POINT('Ctrl Pts',(-7.15382344746782,-13.4751385570953,
118.432615408603)) ;
#155378=CARTESIAN_POINT('Ctrl Pts',(-7.22762729027988,-13.4751385068035,
118.408384365066)) ;
#155379=CARTESIAN_POINT('Ctrl Pts',(-7.2039930219878,-13.4798810069848,
118.33639819625)) ;
#155380=CARTESIAN_POINT('Ctrl Pts',(-7.18035875369573,-13.4846235071661,
118.264412027435)) ;
#155381=CARTESIAN_POINT('Ctrl Pts',(-7.10655491088367,-13.484623557458,
118.288643070972)) ;
#155382=CARTESIAN_POINT('Ctrl Pts',(-7.03275106807161,-13.4846236077499,
118.31287411451)) ;
#155383=CARTESIAN_POINT('Ctrl Pts',(-7.05638533636368,-13.4798811075686,
118.384860283325)) ;
#155384=CARTESIAN_POINT('Ctrl Pts',(-7.07408092560861,-13.1885796838075,
118.403166688914)) ;
#155385=CARTESIAN_POINT('Ctrl Pts',(-7.09725213348969,-13.2041693777773,
118.473742450239)) ;
#155386=CARTESIAN_POINT('Ctrl Pts',(-7.17105597976469,-13.2041693384602,
118.449511417249)) ;
#155387=CARTESIAN_POINT('Ctrl Pts',(-7.24485982603969,-13.2041692991432,
118.425280384259)) ;
#155388=CARTESIAN_POINT('Ctrl Pts',(-7.2216886181586,-13.1885796051734,
118.354704622934)) ;
#155389=CARTESIAN_POINT('Ctrl Pts',(-7.19851741027751,-13.1729899112036,
118.284128861609)) ;
#155390=CARTESIAN_POINT('Ctrl Pts',(-7.12471356400251,-13.1729899505207,
118.308359894599)) ;
#155391=CARTESIAN_POINT('Ctrl Pts',(-7.05090971772751,-13.1729899898377,
118.332590927589)) ;
#155392=CARTESIAN_POINT('Ctrl Pts',(-7.07408092560861,-13.1885796838075,
118.403166688914)) ;
#155393=CARTESIAN_POINT('Ctrl Pts',(-7.11507198338345,-12.9166253502417,
118.492814113544)) ;
#155394=CARTESIAN_POINT('Ctrl Pts',(-7.13614450236063,-12.9512269476541,
118.556997606973)) ;
#155395=CARTESIAN_POINT('Ctrl Pts',(-7.209948350884,-12.951226917539,118.532766580832)) ;
#155396=CARTESIAN_POINT('Ctrl Pts',(-7.28375219940736,-12.951226887424,
118.50853555469)) ;
#155397=CARTESIAN_POINT('Ctrl Pts',(-7.26267968043019,-12.9166252900117,
118.444352061261)) ;
#155398=CARTESIAN_POINT('Ctrl Pts',(-7.241607161453,-12.8820236925993,118.380168567832)) ;
#155399=CARTESIAN_POINT('Ctrl Pts',(-7.16780331292964,-12.8820237227144,
118.404399593974)) ;
#155400=CARTESIAN_POINT('Ctrl Pts',(-7.09399946440627,-12.8820237528294,
118.428630620115)) ;
#155401=CARTESIAN_POINT('Ctrl Pts',(-7.11507198338345,-12.9166253502417,
118.492814113544)) ;
#155402=CARTESIAN_POINT('Ctrl Pts',(-7.1780574208389,-12.6775835687805,
118.649064501798)) ;
#155403=CARTESIAN_POINT('Ctrl Pts',(-7.19550067995718,-12.7289285556427,
118.70219385509)) ;
#155404=CARTESIAN_POINT('Ctrl Pts',(-7.26930452881846,-12.728928538127,
118.677962829978)) ;
#155405=CARTESIAN_POINT('Ctrl Pts',(-7.34310837767973,-12.7289285206112,
118.653731804865)) ;
#155406=CARTESIAN_POINT('Ctrl Pts',(-7.32566511856146,-12.6775835337489,
118.600602451572)) ;
#155407=CARTESIAN_POINT('Ctrl Pts',(-7.30822185944318,-12.6262385468866,
118.54747309828)) ;
#155408=CARTESIAN_POINT('Ctrl Pts',(-7.2344180105819,-12.6262385644024,
118.571704123392)) ;
#155409=CARTESIAN_POINT('Ctrl Pts',(-7.16061416172062,-12.6262385819182,
118.595935148505)) ;
#155410=CARTESIAN_POINT('Ctrl Pts',(-7.1780574208389,-12.6775835687805,
118.649064501798)) ;
#155411=CARTESIAN_POINT('Ctrl Pts',(-7.25891893918462,-12.4925681740676,
118.859833268336)) ;
#155412=CARTESIAN_POINT('Ctrl Pts',(-7.27147756279767,-12.5569096995895,
118.898084809856)) ;
#155413=CARTESIAN_POINT('Ctrl Pts',(-7.34528141070538,-12.5569096913385,
118.873853781839)) ;
#155414=CARTESIAN_POINT('Ctrl Pts',(-7.4190852586131,-12.5569096830874,
118.849622753822)) ;
#155415=CARTESIAN_POINT('Ctrl Pts',(-7.40652663500005,-12.4925681575655,
118.811371212302)) ;
#155416=CARTESIAN_POINT('Ctrl Pts',(-7.393968011387,-12.4282266320435,118.773119670782)) ;
#155417=CARTESIAN_POINT('Ctrl Pts',(-7.32016416347927,-12.4282266402946,
118.797350698799)) ;
#155418=CARTESIAN_POINT('Ctrl Pts',(-7.24636031557156,-12.4282266485456,
118.821581726816)) ;
#155419=CARTESIAN_POINT('Ctrl Pts',(-7.25891893918462,-12.4925681740676,
118.859833268336)) ;
#155420=CARTESIAN_POINT('Ctrl Pts',(-7.35188793041178,-12.3743553948694,
119.107715107246)) ;
#155421=CARTESIAN_POINT('Ctrl Pts',(-7.35870415945858,-12.4470477080891,
119.128476241342)) ;
#155422=CARTESIAN_POINT('Ctrl Pts',(-7.43250800622119,-12.447047705519,
119.104245209837)) ;
#155423=CARTESIAN_POINT('Ctrl Pts',(-7.50631185298381,-12.4470477029489,
119.080014178332)) ;
#155424=CARTESIAN_POINT('Ctrl Pts',(-7.49949562393702,-12.3743553897291,
119.059253044237)) ;
#155425=CARTESIAN_POINT('Ctrl Pts',(-7.49267939489023,-12.3016630765093,
119.038491910141)) ;
#155426=CARTESIAN_POINT('Ctrl Pts',(-7.41887554812762,-12.3016630790795,
119.062722941646)) ;
#155427=CARTESIAN_POINT('Ctrl Pts',(-7.345071701365,-12.3016630816496,119.086953973151)) ;
#155428=CARTESIAN_POINT('Ctrl Pts',(-7.35188793041178,-12.3743553948694,
119.107715107246)) ;
#155429=CARTESIAN_POINT('Ctrl Pts',(-7.45265031525607,-12.3300586716913,
119.37899047094)) ;
#155430=CARTESIAN_POINT('Ctrl Pts',(-7.45317826435854,-12.4059540802535,
119.3805985188)) ;
#155431=CARTESIAN_POINT('Ctrl Pts',(-7.52698210902912,-12.4059540807321,
119.356367480923)) ;
#155432=CARTESIAN_POINT('Ctrl Pts',(-7.60078595369971,-12.4059540812107,
119.332136443046)) ;
#155433=CARTESIAN_POINT('Ctrl Pts',(-7.60025800459724,-12.3300586726485,
119.330528395187)) ;
#155434=CARTESIAN_POINT('Ctrl Pts',(-7.59973005549478,-12.2541632640863,
119.328920347327)) ;
#155435=CARTESIAN_POINT('Ctrl Pts',(-7.52592621082419,-12.2541632636077,
119.353151385204)) ;
#155436=CARTESIAN_POINT('Ctrl Pts',(-7.4521223661536,-12.254163263129,119.37738242308)) ;
#155437=CARTESIAN_POINT('Ctrl Pts',(-7.45265031525607,-12.3300586716913,
119.37899047094)) ;
#155438=CARTESIAN_POINT('Ctrl Pts',(-7.55337524562207,-12.3643855283945,
119.650314676817)) ;
#155439=CARTESIAN_POINT('Ctrl Pts',(-7.54760458625465,-12.4379977305632,
119.632738179473)) ;
#155440=CARTESIAN_POINT('Ctrl Pts',(-7.62140842959395,-12.4379977307755,
119.608507137542)) ;
#155441=CARTESIAN_POINT('Ctrl Pts',(-7.69521227293323,-12.4379977309879,
119.58427609561)) ;
#155442=CARTESIAN_POINT('Ctrl Pts',(-7.70098293230066,-12.3643855288192,
119.601852592954)) ;
#155443=CARTESIAN_POINT('Ctrl Pts',(-7.70675359166808,-12.2907733266505,
119.619429090297)) ;
#155444=CARTESIAN_POINT('Ctrl Pts',(-7.63294974832878,-12.2907733264382,
119.643660132229)) ;
#155445=CARTESIAN_POINT('Ctrl Pts',(-7.55914590498948,-12.2907733262258,
119.66789117416)) ;
#155446=CARTESIAN_POINT('Ctrl Pts',(-7.55337524562207,-12.3643855283945,
119.650314676817)) ;
#155447=CARTESIAN_POINT('Ctrl Pts',(-7.64773366833853,-12.4735026256636,
119.902366613272)) ;
#155448=CARTESIAN_POINT('Ctrl Pts',(-7.63609718343747,-12.5396050352221,
119.866923757755)) ;
#155449=CARTESIAN_POINT('Ctrl Pts',(-7.70990102613766,-12.5396050341181,
119.842692713877)) ;
#155450=CARTESIAN_POINT('Ctrl Pts',(-7.78370486883785,-12.5396050330141,
119.818461669998)) ;
#155451=CARTESIAN_POINT('Ctrl Pts',(-7.79534135373891,-12.4735026234556,
119.853904525516)) ;
#155452=CARTESIAN_POINT('Ctrl Pts',(-7.80697783863996,-12.4074002138971,
119.889347381033)) ;
#155453=CARTESIAN_POINT('Ctrl Pts',(-7.73317399593978,-12.4074002150011,
119.913578424911)) ;
#155454=CARTESIAN_POINT('Ctrl Pts',(-7.65937015323959,-12.4074002161051,
119.93780946879)) ;
#155455=CARTESIAN_POINT('Ctrl Pts',(-7.64773366833853,-12.4735026256636,
119.902366613272)) ;
#155456=CARTESIAN_POINT('Ctrl Pts',(-7.73041986817396,-12.6505044221707,
120.118738891923)) ;
#155457=CARTESIAN_POINT('Ctrl Pts',(-7.71372634252646,-12.7043450691342,
120.067893106223)) ;
#155458=CARTESIAN_POINT('Ctrl Pts',(-7.7875301851787,-12.7043450666146,
120.043662062199)) ;
#155459=CARTESIAN_POINT('Ctrl Pts',(-7.86133402783094,-12.7043450640951,
120.019431018175)) ;
#155460=CARTESIAN_POINT('Ctrl Pts',(-7.87802755347846,-12.6505044171317,
120.070276803874)) ;
#155461=CARTESIAN_POINT('Ctrl Pts',(-7.89472107912596,-12.5966637701682,
120.121122589574)) ;
#155462=CARTESIAN_POINT('Ctrl Pts',(-7.82091723647372,-12.5966637726878,
120.145353633598)) ;
#155463=CARTESIAN_POINT('Ctrl Pts',(-7.74711339382147,-12.5966637752073,
120.169584677622)) ;
#155464=CARTESIAN_POINT('Ctrl Pts',(-7.73041986817396,-12.6505044221707,
120.118738891923)) ;
#155465=CARTESIAN_POINT('Ctrl Pts',(-7.79595012127722,-12.883421947767,
120.282755379935)) ;
#155466=CARTESIAN_POINT('Ctrl Pts',(-7.77539224983967,-12.9210776018657,
120.220139420507)) ;
#155467=CARTESIAN_POINT('Ctrl Pts',(-7.84919609306675,-12.9210776004055,
120.195908378234)) ;
#155468=CARTESIAN_POINT('Ctrl Pts',(-7.92299993629382,-12.9210775989452,
120.17167733596)) ;
#155469=CARTESIAN_POINT('Ctrl Pts',(-7.94355780773136,-12.8834219448465,
120.234293295388)) ;
#155470=CARTESIAN_POINT('Ctrl Pts',(-7.96411567916889,-12.8457662907479,
120.296909254817)) ;
#155471=CARTESIAN_POINT('Ctrl Pts',(-7.89031183594182,-12.8457662922081,
120.32114029709)) ;
#155472=CARTESIAN_POINT('Ctrl Pts',(-7.81650799271475,-12.8457662936684,
120.345371339364)) ;
#155473=CARTESIAN_POINT('Ctrl Pts',(-7.79595012127722,-12.883421947767,
120.282755379935)) ;
#155474=CARTESIAN_POINT('Ctrl Pts',(-7.83999077408972,-13.1527514798463,
120.381574983125)) ;
#155475=CARTESIAN_POINT('Ctrl Pts',(-7.81705865500437,-13.1716560829413,
120.3117274485)) ;
#155476=CARTESIAN_POINT('Ctrl Pts',(-7.8908624986358,-13.1716560841151,
120.287496407458)) ;
#155477=CARTESIAN_POINT('Ctrl Pts',(-7.96466634226723,-13.1716560852888,
120.263265366416)) ;
#155478=CARTESIAN_POINT('Ctrl Pts',(-7.98759846135258,-13.1527514821937,
120.333112901041)) ;
#155479=CARTESIAN_POINT('Ctrl Pts',(-8.01053058043792,-13.1338468790986,
120.402960435666)) ;
#155480=CARTESIAN_POINT('Ctrl Pts',(-7.93672673680649,-13.1338468779249,
120.427191476708)) ;
#155481=CARTESIAN_POINT('Ctrl Pts',(-7.86292289317506,-13.1338468767512,
120.451422517749)) ;
#155482=CARTESIAN_POINT('Ctrl Pts',(-7.83999077408972,-13.1527514798463,
120.381574983125)) ;
#155483=CARTESIAN_POINT('Ctrl Pts',(-7.86072974007722,-13.4437023579035,
120.40908356129)) ;
#155484=CARTESIAN_POINT('Ctrl Pts',(-7.83705375696572,-13.4423185568972,
120.336970336981)) ;
#155485=CARTESIAN_POINT('Ctrl Pts',(-7.91085760050323,-13.442318564338,
120.312739295653)) ;
#155486=CARTESIAN_POINT('Ctrl Pts',(-7.98466144404073,-13.4423185717788,
120.288508254326)) ;
#155487=CARTESIAN_POINT('Ctrl Pts',(-8.00833742715221,-13.443702372785,
120.360621478634)) ;
#155488=CARTESIAN_POINT('Ctrl Pts',(-8.0320134102637,-13.4450861737913,
120.432734702942)) ;
#155489=CARTESIAN_POINT('Ctrl Pts',(-7.95820956672621,-13.4450861663505,
120.45696574427)) ;
#155490=CARTESIAN_POINT('Ctrl Pts',(-7.88440572318869,-13.4450861589097,
120.481196785598)) ;
#155491=CARTESIAN_POINT('Ctrl Pts',(-7.86072974007722,-13.4437023579035,
120.40908356129)) ;
#155492=CARTESIAN_POINT('Ctrl Pts',(-7.85692244140455,-13.7306193771303,
120.362100112163)) ;
#155493=CARTESIAN_POINT('Ctrl Pts',(-7.83421023585808,-13.7091999974399,
120.292922398928)) ;
#155494=CARTESIAN_POINT('Ctrl Pts',(-7.90801407820719,-13.7092000104109,
120.268691353981)) ;
#155495=CARTESIAN_POINT('Ctrl Pts',(-7.9818179205563,-13.7092000233819,
120.244460309033)) ;
#155496=CARTESIAN_POINT('Ctrl Pts',(-8.00453012610277,-13.7306194030722,
120.313638022267)) ;
#155497=CARTESIAN_POINT('Ctrl Pts',(-8.02724233164922,-13.7520387827626,
120.382815735502)) ;
#155498=CARTESIAN_POINT('Ctrl Pts',(-7.95343848930012,-13.7520387697916,
120.40704678045)) ;
#155499=CARTESIAN_POINT('Ctrl Pts',(-7.87963464695101,-13.7520387568206,
120.431277825397)) ;
#155500=CARTESIAN_POINT('Ctrl Pts',(-7.85692244140455,-13.7306193771303,
120.362100112163)) ;
#155501=CARTESIAN_POINT('Ctrl Pts',(-7.83012410737516,-13.9949086675026,
120.245151518457)) ;
#155502=CARTESIAN_POINT('Ctrl Pts',(-7.80998117065526,-13.9550051326843,
120.183799383634)) ;
#155503=CARTESIAN_POINT('Ctrl Pts',(-7.8837850110375,-13.9550051495312,
120.159568332696)) ;
#155504=CARTESIAN_POINT('Ctrl Pts',(-7.95758885141974,-13.9550051663781,
120.135337281758)) ;
#155505=CARTESIAN_POINT('Ctrl Pts',(-7.97773178813963,-13.9949087011963,
120.19668941658)) ;
#155506=CARTESIAN_POINT('Ctrl Pts',(-7.99787472485951,-14.0348122360146,
120.258041551403)) ;
#155507=CARTESIAN_POINT('Ctrl Pts',(-7.92407088447728,-14.0348122191677,
120.282272602341)) ;
#155508=CARTESIAN_POINT('Ctrl Pts',(-7.85026704409504,-14.0348122023208,
120.306503653279)) ;
#155509=CARTESIAN_POINT('Ctrl Pts',(-7.83012410737516,-13.9949086675026,
120.245151518457)) ;
#155510=CARTESIAN_POINT('Ctrl Pts',(-7.78237083717385,-14.2196906214034,
120.06409456817)) ;
#155511=CARTESIAN_POINT('Ctrl Pts',(-7.76626970535942,-14.1640342666894,
120.015053119126)) ;
#155512=CARTESIAN_POINT('Ctrl Pts',(-7.84007354233546,-14.1640342866179,
119.990822057813)) ;
#155513=CARTESIAN_POINT('Ctrl Pts',(-7.91387737931149,-14.1640343065465,
119.9665909965)) ;
#155514=CARTESIAN_POINT('Ctrl Pts',(-7.9299785111259,-14.2196906612605,
120.015632445544)) ;
#155515=CARTESIAN_POINT('Ctrl Pts',(-7.94607964294033,-14.2753470159745,
120.064673894588)) ;
#155516=CARTESIAN_POINT('Ctrl Pts',(-7.8722758059643,-14.275346996046,120.088904955901)) ;
#155517=CARTESIAN_POINT('Ctrl Pts',(-7.79847196898827,-14.2753469761174,
120.113136017214)) ;
#155518=CARTESIAN_POINT('Ctrl Pts',(-7.78237083717385,-14.2196906214034,
120.06409456817)) ;
#155519=CARTESIAN_POINT('Ctrl Pts',(-7.71854875724072,-14.3856064052365,
119.834353268658)) ;
#155520=CARTESIAN_POINT('Ctrl Pts',(-7.70761197878153,-14.3182855334349,
119.801041606811)) ;
#155521=CARTESIAN_POINT('Ctrl Pts',(-7.78141581228379,-14.3182855505584,
119.776810534917)) ;
#155522=CARTESIAN_POINT('Ctrl Pts',(-7.85521964578606,-14.318285567682,
119.752579463024)) ;
#155523=CARTESIAN_POINT('Ctrl Pts',(-7.86615642424525,-14.3856064394836,
119.785891124871)) ;
#155524=CARTESIAN_POINT('Ctrl Pts',(-7.87709320270443,-14.4529273112853,
119.819202786718)) ;
#155525=CARTESIAN_POINT('Ctrl Pts',(-7.80328936920217,-14.4529272941617,
119.843433858612)) ;
#155526=CARTESIAN_POINT('Ctrl Pts',(-7.7294855356999,-14.4529272770382,
119.867664930505)) ;
#155527=CARTESIAN_POINT('Ctrl Pts',(-7.71854875724072,-14.3856064052365,
119.834353268658)) ;
#155528=CARTESIAN_POINT('Ctrl Pts',(-7.64334502750247,-14.4829720573525,
119.569777363778)) ;
#155529=CARTESIAN_POINT('Ctrl Pts',(-7.63837808621904,-14.4087556909408,
119.554648862916)) ;
#155530=CARTESIAN_POINT('Ctrl Pts',(-7.71218191587185,-14.4087557009118,
119.530417779298)) ;
#155531=CARTESIAN_POINT('Ctrl Pts',(-7.78598574552467,-14.4087557108828,
119.506186695679)) ;
#155532=CARTESIAN_POINT('Ctrl Pts',(-7.7909526868081,-14.4829720772946,
119.521315196541)) ;
#155533=CARTESIAN_POINT('Ctrl Pts',(-7.79591962809152,-14.5571884437063,
119.536443697403)) ;
#155534=CARTESIAN_POINT('Ctrl Pts',(-7.7221157984387,-14.5571884337353,
119.560674781022)) ;
#155535=CARTESIAN_POINT('Ctrl Pts',(-7.64831196878589,-14.5571884237643,
119.58490586464)) ;
#155536=CARTESIAN_POINT('Ctrl Pts',(-7.64334502750247,-14.4829720573525,
119.569777363778)) ;
#155537=CARTESIAN_POINT('Ctrl Pts',(-7.56338289868114,-14.5039687036518,
119.290821303275)) ;
#155538=CARTESIAN_POINT('Ctrl Pts',(-7.56472425461539,-14.4281793222941,
119.294906858056)) ;
#155539=CARTESIAN_POINT('Ctrl Pts',(-7.63852808138411,-14.4281793198172,
119.270675765653)) ;
#155540=CARTESIAN_POINT('Ctrl Pts',(-7.71233190815282,-14.4281793173403,
119.24644467325)) ;
#155541=CARTESIAN_POINT('Ctrl Pts',(-7.71099055221857,-14.503968698698,
119.242359118469)) ;
#155542=CARTESIAN_POINT('Ctrl Pts',(-7.7096491962843,-14.5797580800556,
119.238273563689)) ;
#155543=CARTESIAN_POINT('Ctrl Pts',(-7.63584536951559,-14.5797580825325,
119.262504656092)) ;
#155544=CARTESIAN_POINT('Ctrl Pts',(-7.56204154274688,-14.5797580850095,
119.286735748495)) ;
#155545=CARTESIAN_POINT('Ctrl Pts',(-7.56338289868114,-14.5039687036518,
119.290821303275)) ;
#155546=CARTESIAN_POINT('Ctrl Pts',(-7.48437547453331,-14.4466173797893,
119.014508165448)) ;
#155547=CARTESIAN_POINT('Ctrl Pts',(-7.49197302414555,-14.3747219587681,
119.037649076942)) ;
#155548=CARTESIAN_POINT('Ctrl Pts',(-7.56577684864369,-14.3747219386736,
119.013417977623)) ;
#155549=CARTESIAN_POINT('Ctrl Pts',(-7.63958067314183,-14.3747219185791,
118.989186878304)) ;
#155550=CARTESIAN_POINT('Ctrl Pts',(-7.63198312352959,-14.4466173396002,
118.966045966811)) ;
#155551=CARTESIAN_POINT('Ctrl Pts',(-7.62438557391735,-14.5185127606213,
118.942905055318)) ;
#155552=CARTESIAN_POINT('Ctrl Pts',(-7.55058174941921,-14.5185127807159,
118.967136154636)) ;
#155553=CARTESIAN_POINT('Ctrl Pts',(-7.47677792492107,-14.5185128008104,
118.991367253955)) ;
#155554=CARTESIAN_POINT('Ctrl Pts',(-7.48437547453331,-14.4466173797893,
119.014508165448)) ;
#155555=CARTESIAN_POINT('Ctrl Pts',(-7.41403834460529,-14.3162716014842,
118.764955621569)) ;
#155556=CARTESIAN_POINT('Ctrl Pts',(-7.42728841454722,-14.2533730380978,
118.805313198086)) ;
#155557=CARTESIAN_POINT('Ctrl Pts',(-7.50109223966777,-14.2533729987048,
118.781082100663)) ;
#155558=CARTESIAN_POINT('Ctrl Pts',(-7.57489606478832,-14.2533729593119,
118.75685100324)) ;
#155559=CARTESIAN_POINT('Ctrl Pts',(-7.56164599484638,-14.3162715226984,
118.716493426723)) ;
#155560=CARTESIAN_POINT('Ctrl Pts',(-7.54839592490445,-14.3791700860849,
118.676135850206)) ;
#155561=CARTESIAN_POINT('Ctrl Pts',(-7.4745920997839,-14.3791701254778,
118.700366947629)) ;
#155562=CARTESIAN_POINT('Ctrl Pts',(-7.40078827466335,-14.3791701648707,
118.724598045051)) ;
#155563=CARTESIAN_POINT('Ctrl Pts',(-7.41403834460529,-14.3162716014842,
118.764955621569)) ;
#155564=CARTESIAN_POINT('Ctrl Pts',(-7.35704039989976,-14.1214968775469,
118.555885778132)) ;
#155565=CARTESIAN_POINT('Ctrl Pts',(-7.37502288865875,-14.0721057771866,
118.610657538943)) ;
#155566=CARTESIAN_POINT('Ctrl Pts',(-7.44882671608949,-14.0721057178665,
118.586426448556)) ;
#155567=CARTESIAN_POINT('Ctrl Pts',(-7.52263054352023,-14.0721056585463,
118.56219535817)) ;
#155568=CARTESIAN_POINT('Ctrl Pts',(-7.50464805476125,-14.1214967589066,
118.507423597359)) ;
#155569=CARTESIAN_POINT('Ctrl Pts',(-7.48666556600226,-14.170887859267,
118.452651836549)) ;
#155570=CARTESIAN_POINT('Ctrl Pts',(-7.41286173857152,-14.1708879185871,
118.476882926935)) ;
#155571=CARTESIAN_POINT('Ctrl Pts',(-7.33905791114077,-14.1708879779072,
118.501114017322)) ;
#155572=CARTESIAN_POINT('Ctrl Pts',(-7.35704039989976,-14.1214968775469,
118.555885778132)) ;
#155573=CARTESIAN_POINT('Ctrl Pts',(-7.31852311276589,-13.8749956323593,
118.402954989973)) ;
#155574=CARTESIAN_POINT('Ctrl Pts',(-7.33995787032347,-13.8427423803111,
118.46824180468)) ;
#155575=CARTESIAN_POINT('Ctrl Pts',(-7.4137617022352,-13.8427423020325,
118.444010727942)) ;
#155576=CARTESIAN_POINT('Ctrl Pts',(-7.48756553414692,-13.8427422237539,
118.419779651204)) ;
#155577=CARTESIAN_POINT('Ctrl Pts',(-7.46613077658935,-13.8749954758022,
118.354492836497)) ;
#155578=CARTESIAN_POINT('Ctrl Pts',(-7.44469601903177,-13.9072487278505,
118.28920602179)) ;
#155579=CARTESIAN_POINT('Ctrl Pts',(-7.37089218712003,-13.907248806129,
118.313437098528)) ;
#155580=CARTESIAN_POINT('Ctrl Pts',(-7.2970883552083,-13.9072488844076,
118.337668175266)) ;
#155581=CARTESIAN_POINT('Ctrl Pts',(-7.31852311276589,-13.8749956323593,
118.402954989973)) ;
#155582=CARTESIAN_POINT('Ctrl Pts',(-7.30231103568058,-13.5974682752699,
118.318202627209)) ;
#155583=CARTESIAN_POINT('Ctrl Pts',(-7.32564071440279,-13.5845442893725,
118.389261066145)) ;
#155584=CARTESIAN_POINT('Ctrl Pts',(-7.39944455296119,-13.584544198723,
118.365030009652)) ;
#155585=CARTESIAN_POINT('Ctrl Pts',(-7.4732483915196,-13.5845441080735,
118.340798953159)) ;
#155586=CARTESIAN_POINT('Ctrl Pts',(-7.4499187127974,-13.597468093971,118.269740514223)) ;
#155587=CARTESIAN_POINT('Ctrl Pts',(-7.42658903407519,-13.6103920798684,
118.198682075287)) ;
#155588=CARTESIAN_POINT('Ctrl Pts',(-7.35278519551678,-13.6103921705179,
118.22291313178)) ;
#155589=CARTESIAN_POINT('Ctrl Pts',(-7.27898135695837,-13.6103922611673,
118.247144188274)) ;
#155590=CARTESIAN_POINT('Ctrl Pts',(-7.30231103568058,-13.5974682752699,
118.318202627209)) ;
#155591=CARTESIAN_POINT('Ctrl Pts',(-7.30987663537963,-13.3070931499256,
118.305860700972)) ;
#155592=CARTESIAN_POINT('Ctrl Pts',(-7.33344423912749,-13.3144232873773,
118.377643821243)) ;
#155593=CARTESIAN_POINT('Ctrl Pts',(-7.40724808549206,-13.3144231909102,
118.353412788526)) ;
#155594=CARTESIAN_POINT('Ctrl Pts',(-7.48105193185662,-13.314423094443,
118.329181755809)) ;
#155595=CARTESIAN_POINT('Ctrl Pts',(-7.45748432810876,-13.3070929569913,
118.257398635538)) ;
#155596=CARTESIAN_POINT('Ctrl Pts',(-7.43391672436091,-13.2997628195396,
118.185615515268)) ;
#155597=CARTESIAN_POINT('Ctrl Pts',(-7.36011287799634,-13.2997629160068,
118.209846547985)) ;
#155598=CARTESIAN_POINT('Ctrl Pts',(-7.28630903163177,-13.2997630124739,
118.234077580702)) ;
#155599=CARTESIAN_POINT('Ctrl Pts',(-7.30987663537963,-13.3070931499256,
118.305860700972)) ;
#155600=CARTESIAN_POINT('Ctrl Pts',(-7.34175942853511,-13.0233508116479,
118.36742076646)) ;
#155601=CARTESIAN_POINT('Ctrl Pts',(-7.36387123793272,-13.0505014151777,
118.434769772124)) ;
#155602=CARTESIAN_POINT('Ctrl Pts',(-7.43767509276429,-13.0505013202395,
118.410538765196)) ;
#155603=CARTESIAN_POINT('Ctrl Pts',(-7.51147894759584,-13.0505012253013,
118.386307758269)) ;
#155604=CARTESIAN_POINT('Ctrl Pts',(-7.48936713819821,-13.0233506217714,
118.318958752604)) ;
#155605=CARTESIAN_POINT('Ctrl Pts',(-7.4672553288006,-12.9962000182415,
118.25160974694)) ;
#155606=CARTESIAN_POINT('Ctrl Pts',(-7.39345147396905,-12.9962001131797,
118.275840753868)) ;
#155607=CARTESIAN_POINT('Ctrl Pts',(-7.31964761913749,-12.996200208118,
118.300071760795)) ;
#155608=CARTESIAN_POINT('Ctrl Pts',(-7.34175942853511,-13.0233508116479,
118.36742076646)) ;
#155609=CARTESIAN_POINT('Ctrl Pts',(-7.39618528009665,-12.7688607554056,
118.497769967232)) ;
#155610=CARTESIAN_POINT('Ctrl Pts',(-7.41526264461118,-12.8138186885295,
118.55587654345)) ;
#155611=CARTESIAN_POINT('Ctrl Pts',(-7.48906650749834,-12.8138186042271,
118.531645561058)) ;
#155612=CARTESIAN_POINT('Ctrl Pts',(-7.56287037038549,-12.8138185199248,
118.507414578666)) ;
#155613=CARTESIAN_POINT('Ctrl Pts',(-7.54379300587095,-12.7688605868009,
118.449308002449)) ;
#155614=CARTESIAN_POINT('Ctrl Pts',(-7.52471564135643,-12.723902653677,
118.391201426231)) ;
#155615=CARTESIAN_POINT('Ctrl Pts',(-7.45091177846927,-12.7239027379794,
118.415432408623)) ;
#155616=CARTESIAN_POINT('Ctrl Pts',(-7.37710791558212,-12.7239028222818,
118.439663391015)) ;
#155617=CARTESIAN_POINT('Ctrl Pts',(-7.39618528009665,-12.7688607554056,
118.497769967232)) ;
#155618=CARTESIAN_POINT('Ctrl Pts',(-7.47020228300154,-12.5604071436069,
118.687726339368)) ;
#155619=CARTESIAN_POINT('Ctrl Pts',(-7.4848744582239,-12.6199846631104,
118.732415419821)) ;
#155620=CARTESIAN_POINT('Ctrl Pts',(-7.5586783279789,-12.6199845970407,
118.708184458347)) ;
#155621=CARTESIAN_POINT('Ctrl Pts',(-7.63248219773388,-12.6199845309711,
118.683953496874)) ;
#155622=CARTESIAN_POINT('Ctrl Pts',(-7.61781002251153,-12.5604070114677,
118.639264416421)) ;
#155623=CARTESIAN_POINT('Ctrl Pts',(-7.60313784728917,-12.5008294919642,
118.594575335968)) ;
#155624=CARTESIAN_POINT('Ctrl Pts',(-7.52933397753417,-12.5008295580339,
118.618806297441)) ;
#155625=CARTESIAN_POINT('Ctrl Pts',(-7.45553010777918,-12.5008296241035,
118.643037258915)) ;
#155626=CARTESIAN_POINT('Ctrl Pts',(-7.47020228300154,-12.5604071436069,
118.687726339368)) ;
#155627=CARTESIAN_POINT('Ctrl Pts',(-7.55906350518853,-12.4137261008746,
118.922952330464)) ;
#155628=CARTESIAN_POINT('Ctrl Pts',(-7.56828647533281,-12.4836322376362,
118.951044011495)) ;
#155629=CARTESIAN_POINT('Ctrl Pts',(-7.64209034991756,-12.4836321960017,
118.926813064733)) ;
#155630=CARTESIAN_POINT('Ctrl Pts',(-7.71589422450231,-12.4836321543672,
118.90258211797)) ;
#155631=CARTESIAN_POINT('Ctrl Pts',(-7.70667125435802,-12.4137260176056,
118.874490436939)) ;
#155632=CARTESIAN_POINT('Ctrl Pts',(-7.69744828421375,-12.343819880844,
118.846398755907)) ;
#155633=CARTESIAN_POINT('Ctrl Pts',(-7.623644409629,-12.3438199224785,118.87062970267)) ;
#155634=CARTESIAN_POINT('Ctrl Pts',(-7.54984053504425,-12.343819964113,
118.894860649433)) ;
#155635=CARTESIAN_POINT('Ctrl Pts',(-7.55906350518853,-12.4137261008746,
118.922952330464)) ;
#155636=CARTESIAN_POINT('Ctrl Pts',(-7.65717245038672,-12.3387040702925,
119.186368813652)) ;
#155637=CARTESIAN_POINT('Ctrl Pts',(-7.66029208335573,-12.4139513070211,
119.195870714419)) ;
#155638=CARTESIAN_POINT('Ctrl Pts',(-7.7340959603037,-12.4139512934304,
119.171639774854)) ;
#155639=CARTESIAN_POINT('Ctrl Pts',(-7.80789983725165,-12.4139512798397,
119.147408835289)) ;
#155640=CARTESIAN_POINT('Ctrl Pts',(-7.80478020428264,-12.3387040431111,
119.137906934522)) ;
#155641=CARTESIAN_POINT('Ctrl Pts',(-7.80166057131362,-12.2634568063825,
119.128405033755)) ;
#155642=CARTESIAN_POINT('Ctrl Pts',(-7.72785669436566,-12.2634568199732,
119.15263597332)) ;
#155643=CARTESIAN_POINT('Ctrl Pts',(-7.65405281741769,-12.2634568335639,
119.176866912885)) ;
#155644=CARTESIAN_POINT('Ctrl Pts',(-7.65717245038672,-12.3387040702925,
119.186368813652)) ;
#155645=CARTESIAN_POINT('Ctrl Pts',(-7.75884035692309,-12.3410592400664,
119.460451576393)) ;
#155646=CARTESIAN_POINT('Ctrl Pts',(-7.75560281377236,-12.4162542159503,
119.450590544401)) ;
#155647=CARTESIAN_POINT('Ctrl Pts',(-7.8294066902323,-12.4162542313705,
119.426359603349)) ;
#155648=CARTESIAN_POINT('Ctrl Pts',(-7.90321056669223,-12.4162542467908,
119.402128662298)) ;
#155649=CARTESIAN_POINT('Ctrl Pts',(-7.90644810984295,-12.3410592709069,
119.41198969429)) ;
#155650=CARTESIAN_POINT('Ctrl Pts',(-7.90968565299367,-12.265864295023,
119.421850726283)) ;
#155651=CARTESIAN_POINT('Ctrl Pts',(-7.83588177653374,-12.2658642796027,
119.446081667334)) ;
#155652=CARTESIAN_POINT('Ctrl Pts',(-7.76207790007381,-12.2658642641825,
119.470312608385)) ;
#155653=CARTESIAN_POINT('Ctrl Pts',(-7.75884035692309,-12.3410592400664,
119.460451576393)) ;
#155654=CARTESIAN_POINT('Ctrl Pts',(-7.85654736634483,-12.4205041979803,
119.722651987663)) ;
#155655=CARTESIAN_POINT('Ctrl Pts',(-7.84721586315474,-12.4902644552577,
119.694229736606)) ;
#155656=CARTESIAN_POINT('Ctrl Pts',(-7.92101973652683,-12.4902644973908,
119.66999878615)) ;
#155657=CARTESIAN_POINT('Ctrl Pts',(-7.99482360989893,-12.4902645395239,
119.645767835693)) ;
#155658=CARTESIAN_POINT('Ctrl Pts',(-8.00415511308902,-12.4205042822464,
119.674190086751)) ;
#155659=CARTESIAN_POINT('Ctrl Pts',(-8.0134866162791,-12.350744024969,119.702612337808)) ;
#155660=CARTESIAN_POINT('Ctrl Pts',(-7.939682742907,-12.3507439828359,119.726843288264)) ;
#155661=CARTESIAN_POINT('Ctrl Pts',(-7.86587886953491,-12.3507439407028,
119.751074238721)) ;
#155662=CARTESIAN_POINT('Ctrl Pts',(-7.85654736634483,-12.4205041979803,
119.722651987663)) ;
#155663=CARTESIAN_POINT('Ctrl Pts',(-7.94481318053513,-12.5715202421064,
119.956000118428)) ;
#155664=CARTESIAN_POINT('Ctrl Pts',(-7.93003972839049,-12.6308413998765,
119.911002568843)) ;
#155665=CARTESIAN_POINT('Ctrl Pts',(-8.00384359633958,-12.6308414639116,
119.886771601869)) ;
#155666=CARTESIAN_POINT('Ctrl Pts',(-8.07764746428867,-12.6308415279467,
119.862540634895)) ;
#155667=CARTESIAN_POINT('Ctrl Pts',(-8.09242091643331,-12.5715203701767,
119.90753818448)) ;
#155668=CARTESIAN_POINT('Ctrl Pts',(-8.10719436857796,-12.5121992124066,
119.952535734065)) ;
#155669=CARTESIAN_POINT('Ctrl Pts',(-8.03339050062888,-12.5121991483715,
119.976766701039)) ;
#155670=CARTESIAN_POINT('Ctrl Pts',(-7.95958663267978,-12.5121990843364,
120.000997668012)) ;
#155671=CARTESIAN_POINT('Ctrl Pts',(-7.94481318053513,-12.5715202421064,
119.956000118428)) ;
#155672=CARTESIAN_POINT('Ctrl Pts',(-8.01771408381364,-12.7831706996134,
120.142578445181)) ;
#155673=CARTESIAN_POINT('Ctrl Pts',(-7.99856257426153,-12.827803906149,
120.084246039043)) ;
#155674=CARTESIAN_POINT('Ctrl Pts',(-8.07236643520165,-12.8278039851649,
120.060015050721)) ;
#155675=CARTESIAN_POINT('Ctrl Pts',(-8.14617029614177,-12.8278040641808,
120.035784062399)) ;
#155676=CARTESIAN_POINT('Ctrl Pts',(-8.16532180569389,-12.7831708576452,
120.094116468536)) ;
#155677=CARTESIAN_POINT('Ctrl Pts',(-8.18447331524599,-12.7385376511096,
120.152448874673)) ;
#155678=CARTESIAN_POINT('Ctrl Pts',(-8.11066945430587,-12.7385375720937,
120.176679862995)) ;
#155679=CARTESIAN_POINT('Ctrl Pts',(-8.03686559336574,-12.7385374930778,
120.200910851318)) ;
#155680=CARTESIAN_POINT('Ctrl Pts',(-8.01771408381364,-12.7831706996134,
120.142578445181)) ;
#155681=CARTESIAN_POINT('Ctrl Pts',(-8.07085503105618,-13.0400861903177,
120.268992723008)) ;
#155682=CARTESIAN_POINT('Ctrl Pts',(-8.04869796956498,-13.0668491450616,
120.201505890507)) ;
#155683=CARTESIAN_POINT('Ctrl Pts',(-8.12250182275097,-13.0668492312408,
120.177274878567)) ;
#155684=CARTESIAN_POINT('Ctrl Pts',(-8.19630567593696,-13.06684931742,120.153043866627)) ;
#155685=CARTESIAN_POINT('Ctrl Pts',(-8.21846273742817,-13.0400863626762,
120.220530699128)) ;
#155686=CARTESIAN_POINT('Ctrl Pts',(-8.24061979891935,-13.0133234079323,
120.288017531629)) ;
#155687=CARTESIAN_POINT('Ctrl Pts',(-8.16681594573337,-13.0133233217531,
120.312248543569)) ;
#155688=CARTESIAN_POINT('Ctrl Pts',(-8.09301209254737,-13.0133232355738,
120.336479555509)) ;
#155689=CARTESIAN_POINT('Ctrl Pts',(-8.07085503105618,-13.0400861903177,
120.268992723008)) ;
#155690=CARTESIAN_POINT('Ctrl Pts',(-8.1012449479731,-13.3242719779506,
120.326083671067)) ;
#155691=CARTESIAN_POINT('Ctrl Pts',(-8.0776667011033,-13.3312338876365,
120.254268137088)) ;
#155692=CARTESIAN_POINT('Ctrl Pts',(-8.15147054661026,-13.3312339727679,
120.230037101759)) ;
#155693=CARTESIAN_POINT('Ctrl Pts',(-8.22527439211721,-13.3312340578993,
120.20580606643)) ;
#155694=CARTESIAN_POINT('Ctrl Pts',(-8.24885263898701,-13.3242721482135,
120.277621600409)) ;
#155695=CARTESIAN_POINT('Ctrl Pts',(-8.2724308858568,-13.3173102385276,
120.349437134388)) ;
#155696=CARTESIAN_POINT('Ctrl Pts',(-8.19862704034984,-13.3173101533962,
120.373668169717)) ;
#155697=CARTESIAN_POINT('Ctrl Pts',(-8.12482319484289,-13.3173100682647,
120.397899205046)) ;
#155698=CARTESIAN_POINT('Ctrl Pts',(-8.1012449479731,-13.3242719779506,
120.326083671067)) ;
#155699=CARTESIAN_POINT('Ctrl Pts',(-8.10739844779683,-13.6152878377403,
120.309341878199)) ;
#155700=CARTESIAN_POINT('Ctrl Pts',(-8.08408919078993,-13.601941852712,
120.238345643802)) ;
#155701=CARTESIAN_POINT('Ctrl Pts',(-8.15789302956165,-13.6019419294696,
120.214114587959)) ;
#155702=CARTESIAN_POINT('Ctrl Pts',(-8.23169686833337,-13.6019420062272,
120.189883532115)) ;
#155703=CARTESIAN_POINT('Ctrl Pts',(-8.25500612534027,-13.6152879912555,
120.260879766512)) ;
#155704=CARTESIAN_POINT('Ctrl Pts',(-8.27831538234716,-13.6286339762838,
120.33187600091)) ;
#155705=CARTESIAN_POINT('Ctrl Pts',(-8.20451154357544,-13.6286338995262,
120.356107056753)) ;
#155706=CARTESIAN_POINT('Ctrl Pts',(-8.13070770480371,-13.6286338227686,
120.380338112597)) ;
#155707=CARTESIAN_POINT('Ctrl Pts',(-8.10739844779683,-13.6152878377403,
120.309341878199)) ;
#155708=CARTESIAN_POINT('Ctrl Pts',(-8.08962004095609,-13.8920338673762,
120.219720905231)) ;
#155709=CARTESIAN_POINT('Ctrl Pts',(-8.06825077036232,-13.8593453805719,
120.154633556283)) ;
#155710=CARTESIAN_POINT('Ctrl Pts',(-8.14205460400106,-13.8593454436439,
120.130402484805)) ;
#155711=CARTESIAN_POINT('Ctrl Pts',(-8.21585843763983,-13.859345506716,
120.106171413327)) ;
#155712=CARTESIAN_POINT('Ctrl Pts',(-8.23722770823361,-13.8920339935203,
120.171258762276)) ;
#155713=CARTESIAN_POINT('Ctrl Pts',(-8.2585969788274,-13.9247224803246,
120.236346111225)) ;
#155714=CARTESIAN_POINT('Ctrl Pts',(-8.18479314518863,-13.9247224172525,
120.260577182702)) ;
#155715=CARTESIAN_POINT('Ctrl Pts',(-8.11098931154989,-13.9247223541804,
120.28480825418)) ;
#155716=CARTESIAN_POINT('Ctrl Pts',(-8.08962004095609,-13.8920338673762,
120.219720905231)) ;
#155717=CARTESIAN_POINT('Ctrl Pts',(-8.05001723486067,-14.1346381572922,
120.063660745971)) ;
#155718=CARTESIAN_POINT('Ctrl Pts',(-8.03211395972011,-14.0849615058488,
120.009130259783)) ;
#155719=CARTESIAN_POINT('Ctrl Pts',(-8.10591779010873,-14.0849615523416,
119.984899178406)) ;
#155720=CARTESIAN_POINT('Ctrl Pts',(-8.17972162049735,-14.0849615988343,
119.960668097028)) ;
#155721=CARTESIAN_POINT('Ctrl Pts',(-8.19762489563791,-14.1346382502777,
120.015198583216)) ;
#155722=CARTESIAN_POINT('Ctrl Pts',(-8.21552817077847,-14.1843149017211,
120.069729069404)) ;
#155723=CARTESIAN_POINT('Ctrl Pts',(-8.14172434038985,-14.1843148552283,
120.093960150781)) ;
#155724=CARTESIAN_POINT('Ctrl Pts',(-8.06792051000123,-14.1843148087356,
120.118191232158)) ;
#155725=CARTESIAN_POINT('Ctrl Pts',(-8.05001723486067,-14.1346381572922,
120.063660745971)) ;
#155726=CARTESIAN_POINT('Ctrl Pts',(-7.992024762362,-14.3262307223465,119.85152566265)) ;
#155727=CARTESIAN_POINT('Ctrl Pts',(-7.97887798500129,-14.263101480961,
119.81148270107)) ;
#155728=CARTESIAN_POINT('Ctrl Pts',(-8.05268181432158,-14.2631015098285,
119.787251616438)) ;
#155729=CARTESIAN_POINT('Ctrl Pts',(-8.12648564364185,-14.263101538696,
119.763020531807)) ;
#155730=CARTESIAN_POINT('Ctrl Pts',(-8.13963242100255,-14.3262307800815,
119.803063493387)) ;
#155731=CARTESIAN_POINT('Ctrl Pts',(-8.15277919836325,-14.3893600214671,
119.843106454968)) ;
#155732=CARTESIAN_POINT('Ctrl Pts',(-8.07897536904298,-14.3893599925996,
119.867337539599)) ;
#155733=CARTESIAN_POINT('Ctrl Pts',(-8.00517153972269,-14.3893599637321,
119.89156862423)) ;
#155734=CARTESIAN_POINT('Ctrl Pts',(-7.992024762362,-14.3262307223465,119.85152566265)) ;
#155735=CARTESIAN_POINT('Ctrl Pts',(-7.92087420413947,-14.4523301137118,
119.599430244914)) ;
#155736=CARTESIAN_POINT('Ctrl Pts',(-7.913407539792,-14.380300846747,119.576687990937)) ;
#155737=CARTESIAN_POINT('Ctrl Pts',(-7.98721136957771,-14.3803008602231,
119.552456907723)) ;
#155738=CARTESIAN_POINT('Ctrl Pts',(-8.06101519936343,-14.3803008736991,
119.52822582451)) ;
#155739=CARTESIAN_POINT('Ctrl Pts',(-8.0684818637109,-14.4523301406639,
119.550968078487)) ;
#155740=CARTESIAN_POINT('Ctrl Pts',(-8.07594852805837,-14.5243594076287,
119.573710332464)) ;
#155741=CARTESIAN_POINT('Ctrl Pts',(-8.00214469827266,-14.5243593941527,
119.597941415678)) ;
#155742=CARTESIAN_POINT('Ctrl Pts',(-7.92834086848694,-14.5243593806767,
119.622172498891)) ;
#155743=CARTESIAN_POINT('Ctrl Pts',(-7.92087420413947,-14.4523301137118,
119.599430244914)) ;
#155744=CARTESIAN_POINT('Ctrl Pts',(-7.84204196997817,-14.5048566464616,
119.323854472488)) ;
#155745=CARTESIAN_POINT('Ctrl Pts',(-7.84080211163026,-14.4290505733795,
119.320078064726)) ;
#155746=CARTESIAN_POINT('Ctrl Pts',(-7.91460594349901,-14.4290505742608,
119.295846987857)) ;
#155747=CARTESIAN_POINT('Ctrl Pts',(-7.98840977536776,-14.429050575142,
119.271615910988)) ;
#155748=CARTESIAN_POINT('Ctrl Pts',(-7.98964963371567,-14.5048566482241,
119.27539231875)) ;
#155749=CARTESIAN_POINT('Ctrl Pts',(-7.99088949206357,-14.5806627213062,
119.279168726512)) ;
#155750=CARTESIAN_POINT('Ctrl Pts',(-7.91708566019482,-14.580662720425,
119.303399803381)) ;
#155751=CARTESIAN_POINT('Ctrl Pts',(-7.84328182832607,-14.5806627195438,
119.32763088025)) ;
#155752=CARTESIAN_POINT('Ctrl Pts',(-7.84204196997817,-14.5048566464616,
119.323854472488)) ;
#155753=CARTESIAN_POINT('Ctrl Pts',(-7.76186601911956,-14.4792282215674,
119.044096181178)) ;
#155754=CARTESIAN_POINT('Ctrl Pts',(-7.76695821637415,-14.405096385773,
119.059606192928)) ;
#155755=CARTESIAN_POINT('Ctrl Pts',(-7.84076205141397,-14.4050963789129,
119.035375125717)) ;
#155756=CARTESIAN_POINT('Ctrl Pts',(-7.91456588645379,-14.4050963720528,
119.011144058507)) ;
#155757=CARTESIAN_POINT('Ctrl Pts',(-7.9094736891992,-14.4792282078472,
118.995634046757)) ;
#155758=CARTESIAN_POINT('Ctrl Pts',(-7.90438149194462,-14.5533600436416,
118.980124035008)) ;
#155759=CARTESIAN_POINT('Ctrl Pts',(-7.8305776569048,-14.5533600505017,
119.004355102218)) ;
#155760=CARTESIAN_POINT('Ctrl Pts',(-7.75677382186498,-14.5533600573618,
119.028586169429)) ;
#155761=CARTESIAN_POINT('Ctrl Pts',(-7.76186601911956,-14.4792282215674,
119.044096181178)) ;
#155762=CARTESIAN_POINT('Ctrl Pts',(-7.68732567425835,-14.3776591931245,
118.781625479166)) ;
#155763=CARTESIAN_POINT('Ctrl Pts',(-7.69836352724098,-14.3105071713144,
118.815244998788)) ;
#155764=CARTESIAN_POINT('Ctrl Pts',(-7.77216736523883,-14.3105071612984,
118.791013940587)) ;
#155765=CARTESIAN_POINT('Ctrl Pts',(-7.84597120323668,-14.3105071512824,
118.766782882386)) ;
#155766=CARTESIAN_POINT('Ctrl Pts',(-7.83493335025406,-14.3776591730925,
118.733163362765)) ;
#155767=CARTESIAN_POINT('Ctrl Pts',(-7.82389549727142,-14.4448111949025,
118.699543843143)) ;
#155768=CARTESIAN_POINT('Ctrl Pts',(-7.75009165927358,-14.4448112049185,
118.723774901344)) ;
#155769=CARTESIAN_POINT('Ctrl Pts',(-7.67628782127572,-14.4448112149345,
118.748005959545)) ;
#155770=CARTESIAN_POINT('Ctrl Pts',(-7.68732567425835,-14.3776591931245,
118.781625479166)) ;
#155771=CARTESIAN_POINT('Ctrl Pts',(-7.62415597339361,-14.2073582471136,
118.553754081591)) ;
#155772=CARTESIAN_POINT('Ctrl Pts',(-7.64035528068796,-14.1519959883529,
118.603094558107)) ;
#155773=CARTESIAN_POINT('Ctrl Pts',(-7.71415912134421,-14.1519959791231,
118.578863508004)) ;
#155774=CARTESIAN_POINT('Ctrl Pts',(-7.78796296200047,-14.1519959698933,
118.5546324579)) ;
#155775=CARTESIAN_POINT('Ctrl Pts',(-7.77176365470613,-14.207358228654,
118.505291981383)) ;
#155776=CARTESIAN_POINT('Ctrl Pts',(-7.75556434741179,-14.2627204874147,
118.455951504867)) ;
#155777=CARTESIAN_POINT('Ctrl Pts',(-7.68176050675553,-14.2627204966445,
118.48018255497)) ;
#155778=CARTESIAN_POINT('Ctrl Pts',(-7.60795666609927,-14.2627205058743,
118.504413605074)) ;
#155779=CARTESIAN_POINT('Ctrl Pts',(-7.62415597339361,-14.2073582471136,
118.553754081591)) ;
#155780=CARTESIAN_POINT('Ctrl Pts',(-7.57772822356053,-13.980463190757,
118.376876023582)) ;
#155781=CARTESIAN_POINT('Ctrl Pts',(-7.59792777189917,-13.9408606598198,
118.438400588762)) ;
#155782=CARTESIAN_POINT('Ctrl Pts',(-7.67173161439476,-13.9408606539983,
118.41416954426)) ;
#155783=CARTESIAN_POINT('Ctrl Pts',(-7.74553545689033,-13.9408606481768,
118.389938499759)) ;
#155784=CARTESIAN_POINT('Ctrl Pts',(-7.72533590855169,-13.9804631791139,
118.328413934579)) ;
#155785=CARTESIAN_POINT('Ctrl Pts',(-7.70513636021303,-14.0200657100511,
118.266889369399)) ;
#155786=CARTESIAN_POINT('Ctrl Pts',(-7.63133251771746,-14.0200657158726,
118.2911204139)) ;
#155787=CARTESIAN_POINT('Ctrl Pts',(-7.55752867522188,-14.0200657216941,
118.315351458402)) ;
#155788=CARTESIAN_POINT('Ctrl Pts',(-7.57772822356053,-13.980463190757,
118.376876023582)) ;
#155789=CARTESIAN_POINT('Ctrl Pts',(-7.55211423680401,-13.7134648384933,
118.263415580786)) ;
#155790=CARTESIAN_POINT('Ctrl Pts',(-7.57486615867029,-13.6924464842837,
118.332714263813)) ;
#155791=CARTESIAN_POINT('Ctrl Pts',(-7.64867000205498,-13.6924464826294,
118.308483222019)) ;
#155792=CARTESIAN_POINT('Ctrl Pts',(-7.72247384543967,-13.6924464809751,
118.284252180226)) ;
#155793=CARTESIAN_POINT('Ctrl Pts',(-7.69972192357337,-13.7134648351847,
118.214953497199)) ;
#155794=CARTESIAN_POINT('Ctrl Pts',(-7.67697000170707,-13.7344831893942,
118.145654814172)) ;
#155795=CARTESIAN_POINT('Ctrl Pts',(-7.60316615832239,-13.7344831910485,
118.169885855965)) ;
#155796=CARTESIAN_POINT('Ctrl Pts',(-7.5293623149377,-13.7344831927028,
118.194116897759)) ;
#155797=CARTESIAN_POINT('Ctrl Pts',(-7.55211423680401,-13.7134648384933,
118.263415580786)) ;
#155798=CARTESIAN_POINT('Ctrl Pts',(-7.54988396928805,-13.4252028157263,
118.221162235282)) ;
#155799=CARTESIAN_POINT('Ctrl Pts',(-7.57355949818283,-13.4242817506044,
118.293274076228)) ;
#155800=CARTESIAN_POINT('Ctrl Pts',(-7.64736334166818,-13.4242817523867,
118.269043034742)) ;
#155801=CARTESIAN_POINT('Ctrl Pts',(-7.72116718515352,-13.4242817541689,
118.244811993255)) ;
#155802=CARTESIAN_POINT('Ctrl Pts',(-7.69749165625874,-13.4252028192908,
118.172700152308)) ;
#155803=CARTESIAN_POINT('Ctrl Pts',(-7.67381612736396,-13.4261238844127,
118.100588311361)) ;
#155804=CARTESIAN_POINT('Ctrl Pts',(-7.60001228387861,-13.4261238826305,
118.124819352848)) ;
#155805=CARTESIAN_POINT('Ctrl Pts',(-7.52620844039326,-13.4261238808483,
118.149050394335)) ;
#155806=CARTESIAN_POINT('Ctrl Pts',(-7.54988396928805,-13.4252028157263,
118.221162235282)) ;
#155807=CARTESIAN_POINT('Ctrl Pts',(-7.57190400588021,-13.136660084581,
118.252804065339)) ;
#155808=CARTESIAN_POINT('Ctrl Pts',(-7.59481029167102,-13.1558861878268,
118.322572915877)) ;
#155809=CARTESIAN_POINT('Ctrl Pts',(-7.66861413481843,-13.1558861911127,
118.298341873361)) ;
#155810=CARTESIAN_POINT('Ctrl Pts',(-7.74241797796585,-13.1558861943986,
118.274110830845)) ;
#155811=CARTESIAN_POINT('Ctrl Pts',(-7.71951169217504,-13.1366600911528,
118.204341980307)) ;
#155812=CARTESIAN_POINT('Ctrl Pts',(-7.69660540638423,-13.117433987907,
118.134573129769)) ;
#155813=CARTESIAN_POINT('Ctrl Pts',(-7.62280156323682,-13.1174339846211,
118.158804172285)) ;
#155814=CARTESIAN_POINT('Ctrl Pts',(-7.54899772008939,-13.1174339813352,
118.183035214801)) ;
#155815=CARTESIAN_POINT('Ctrl Pts',(-7.57190400588021,-13.136660084581,
118.252804065339)) ;
#155816=CARTESIAN_POINT('Ctrl Pts',(-7.61755830701388,-12.8674128564449,
118.356315160482)) ;
#155817=CARTESIAN_POINT('Ctrl Pts',(-7.63804609281463,-12.9054690960976,
118.418717650288)) ;
#155818=CARTESIAN_POINT('Ctrl Pts',(-7.71184993576395,-12.9054690982831,
118.394486607169)) ;
#155819=CARTESIAN_POINT('Ctrl Pts',(-7.78565377871326,-12.9054691004687,
118.370255564049)) ;
#155820=CARTESIAN_POINT('Ctrl Pts',(-7.7651659929125,-12.867412860816,118.307853074243)) ;
#155821=CARTESIAN_POINT('Ctrl Pts',(-7.74467820711173,-12.8293566211633,
118.245450584436)) ;
#155822=CARTESIAN_POINT('Ctrl Pts',(-7.67087436416242,-12.8293566189777,
118.269681627556)) ;
#155823=CARTESIAN_POINT('Ctrl Pts',(-7.59707052121311,-12.8293566167922,
118.293912670675)) ;
#155824=CARTESIAN_POINT('Ctrl Pts',(-7.61755830701388,-12.8674128564449,
118.356315160482)) ;
#155825=CARTESIAN_POINT('Ctrl Pts',(-7.68406859821228,-12.6383938778605,
118.523453892796)) ;
#155826=CARTESIAN_POINT('Ctrl Pts',(-7.70067567677603,-12.6924977231703,
118.574036374563)) ;
#155827=CARTESIAN_POINT('Ctrl Pts',(-7.77447952014917,-12.6924977228183,
118.549805332734)) ;
#155828=CARTESIAN_POINT('Ctrl Pts',(-7.84828336352231,-12.6924977224664,
118.525574290905)) ;
#155829=CARTESIAN_POINT('Ctrl Pts',(-7.83167628495855,-12.6383938771567,
118.474991809139)) ;
#155830=CARTESIAN_POINT('Ctrl Pts',(-7.8150692063948,-12.5842900318469,
118.424409327373)) ;
#155831=CARTESIAN_POINT('Ctrl Pts',(-7.74126536302167,-12.5842900321988,
118.448640369202)) ;
#155832=CARTESIAN_POINT('Ctrl Pts',(-7.66746151964852,-12.5842900325507,
118.47287141103)) ;
#155833=CARTESIAN_POINT('Ctrl Pts',(-7.68406859821228,-12.6383938778605,
118.523453892796)) ;
#155834=CARTESIAN_POINT('Ctrl Pts',(-7.76755837693475,-12.465038874388,
118.74228416299)) ;
#155835=CARTESIAN_POINT('Ctrl Pts',(-7.77909394316923,-12.531326536537,
118.777419636573)) ;
#155836=CARTESIAN_POINT('Ctrl Pts',(-7.85289778777235,-12.5313265339241,
118.753188598491)) ;
#155837=CARTESIAN_POINT('Ctrl Pts',(-7.92670163237547,-12.5313265313111,
118.728957560409)) ;
#155838=CARTESIAN_POINT('Ctrl Pts',(-7.91516606614098,-12.4650388691621,
118.693822086826)) ;
#155839=CARTESIAN_POINT('Ctrl Pts',(-7.90363049990651,-12.3987512070131,
118.658686613243)) ;
#155840=CARTESIAN_POINT('Ctrl Pts',(-7.82982665530339,-12.3987512096261,
118.682917651325)) ;
#155841=CARTESIAN_POINT('Ctrl Pts',(-7.75602281070027,-12.398751212239,
118.707148689407)) ;
#155842=CARTESIAN_POINT('Ctrl Pts',(-7.76755837693475,-12.465038874388,
118.74228416299)) ;
#155843=CARTESIAN_POINT('Ctrl Pts',(-7.86272316977547,-12.3599344396702,
118.99669592537)) ;
#155844=CARTESIAN_POINT('Ctrl Pts',(-7.86836420348592,-12.4336574817887,
119.013877604073)) ;
#155845=CARTESIAN_POINT('Ctrl Pts',(-7.94216804997685,-12.4336574787988,
118.989646571741)) ;
#155846=CARTESIAN_POINT('Ctrl Pts',(-8.01597189646776,-12.4336574758088,
118.965415539409)) ;
#155847=CARTESIAN_POINT('Ctrl Pts',(-8.01033086275732,-12.3599344336902,
118.948233860705)) ;
#155848=CARTESIAN_POINT('Ctrl Pts',(-8.00468982904687,-12.2862113915716,
118.931052182002)) ;
#155849=CARTESIAN_POINT('Ctrl Pts',(-7.93088598255596,-12.2862113945616,
118.955283214334)) ;
#155850=CARTESIAN_POINT('Ctrl Pts',(-7.85708213606502,-12.2862113975516,
118.979514246666)) ;
#155851=CARTESIAN_POINT('Ctrl Pts',(-7.86272316977547,-12.3599344396702,
118.99669592537)) ;
#155852=CARTESIAN_POINT('Ctrl Pts',(-7.96381251944024,-12.3306429195518,
119.269059347859)) ;
#155853=CARTESIAN_POINT('Ctrl Pts',(-7.9631387544268,-12.4065184959483,
119.267007168685)) ;
#155854=CARTESIAN_POINT('Ctrl Pts',(-8.0369426034021,-12.4065184959014,
119.24277614392)) ;
#155855=CARTESIAN_POINT('Ctrl Pts',(-8.11074645237739,-12.4065184958546,
119.218545119154)) ;
#155856=CARTESIAN_POINT('Ctrl Pts',(-8.11142021739083,-12.330642919458,
119.220597298329)) ;
#155857=CARTESIAN_POINT('Ctrl Pts',(-8.11209398240426,-12.2547673430615,
119.222649477503)) ;
#155858=CARTESIAN_POINT('Ctrl Pts',(-8.03829013342897,-12.2547673431084,
119.246880502269)) ;
#155859=CARTESIAN_POINT('Ctrl Pts',(-7.96448628445367,-12.2547673431553,
119.271111527034)) ;
#155860=CARTESIAN_POINT('Ctrl Pts',(-7.96381251944024,-12.3306429195518,
119.269059347859)) ;
#155861=CARTESIAN_POINT('Ctrl Pts',(-8.06368380821921,-12.3792038030185,
119.537856629935)) ;
#155862=CARTESIAN_POINT('Ctrl Pts',(-8.05676830195218,-12.4517984874487,
119.516793114142)) ;
#155863=CARTESIAN_POINT('Ctrl Pts',(-8.13057215287077,-12.4517984942269,
119.492562095296)) ;
#155864=CARTESIAN_POINT('Ctrl Pts',(-8.20437600378937,-12.4517985010052,
119.468331076449)) ;
#155865=CARTESIAN_POINT('Ctrl Pts',(-8.2112915100564,-12.379203816575,119.489394592243)) ;
#155866=CARTESIAN_POINT('Ctrl Pts',(-8.21820701632344,-12.3066091321447,
119.510458108036)) ;
#155867=CARTESIAN_POINT('Ctrl Pts',(-8.14440316540483,-12.3066091253665,
119.534689126882)) ;
#155868=CARTESIAN_POINT('Ctrl Pts',(-8.07059931448624,-12.3066091185883,
119.558920145729)) ;
#155869=CARTESIAN_POINT('Ctrl Pts',(-8.06368380821921,-12.3792038030185,
119.537856629935)) ;
#155870=CARTESIAN_POINT('Ctrl Pts',(-8.15659748944132,-12.502250920438,
119.785364900155)) ;
#155871=CARTESIAN_POINT('Ctrl Pts',(-8.14391906293416,-12.5663594268052,
119.746748459319)) ;
#155872=CARTESIAN_POINT('Ctrl Pts',(-8.21772291527402,-12.5663594442773,
119.722517444801)) ;
#155873=CARTESIAN_POINT('Ctrl Pts',(-8.29152676761388,-12.5663594617495,
119.698286430284)) ;
#155874=CARTESIAN_POINT('Ctrl Pts',(-8.30420519412103,-12.5022509553824,
119.73690287112)) ;
#155875=CARTESIAN_POINT('Ctrl Pts',(-8.31688362062818,-12.4381424490152,
119.775519311956)) ;
#155876=CARTESIAN_POINT('Ctrl Pts',(-8.24307976828833,-12.4381424315431,
119.799750326474)) ;
#155877=CARTESIAN_POINT('Ctrl Pts',(-8.16927591594847,-12.4381424140709,
119.823981340991)) ;
#155878=CARTESIAN_POINT('Ctrl Pts',(-8.15659748944132,-12.502250920438,
119.785364900155)) ;
#155879=CARTESIAN_POINT('Ctrl Pts',(-8.23623754753109,-12.690704289041,
119.992502391065)) ;
#155880=CARTESIAN_POINT('Ctrl Pts',(-8.21871354461729,-12.7417475393675,
119.939127106486)) ;
#155881=CARTESIAN_POINT('Ctrl Pts',(-8.29251739692174,-12.7417475700136,
119.914896091861)) ;
#155882=CARTESIAN_POINT('Ctrl Pts',(-8.36632124922617,-12.7417476006596,
119.890665077235)) ;
#155883=CARTESIAN_POINT('Ctrl Pts',(-8.38384525213997,-12.6907043503331,
119.944040361814)) ;
#155884=CARTESIAN_POINT('Ctrl Pts',(-8.40136925505376,-12.6396611000066,
119.997415646394)) ;
#155885=CARTESIAN_POINT('Ctrl Pts',(-8.32756540274933,-12.6396610693606,
120.021646661019)) ;
#155886=CARTESIAN_POINT('Ctrl Pts',(-8.25376155044489,-12.6396610387145,
120.045877675644)) ;
#155887=CARTESIAN_POINT('Ctrl Pts',(-8.23623754753109,-12.690704289041,
119.992502391065)) ;
#155888=CARTESIAN_POINT('Ctrl Pts',(-8.29787978612712,-12.9312491813812,
120.144802031741)) ;
#155889=CARTESIAN_POINT('Ctrl Pts',(-8.27676025616477,-12.9655714979513,
120.080475352075)) ;
#155890=CARTESIAN_POINT('Ctrl Pts',(-8.35056410683368,-12.9655715427417,
120.056244332468)) ;
#155891=CARTESIAN_POINT('Ctrl Pts',(-8.42436795750258,-12.9655715875322,
120.032013312861)) ;
#155892=CARTESIAN_POINT('Ctrl Pts',(-8.44548748746493,-12.9312492709622,
120.096339992527)) ;
#155893=CARTESIAN_POINT('Ctrl Pts',(-8.46660701742727,-12.8969269543922,
120.160666672194)) ;
#155894=CARTESIAN_POINT('Ctrl Pts',(-8.39280316675835,-12.8969269096017,
120.184897691801)) ;
#155895=CARTESIAN_POINT('Ctrl Pts',(-8.31899931608945,-12.8969268648112,
120.209128711407)) ;
#155896=CARTESIAN_POINT('Ctrl Pts',(-8.29787978612712,-12.9312491813812,
120.144802031741)) ;
#155897=CARTESIAN_POINT('Ctrl Pts',(-8.33778763616187,-13.2069304836541,
120.230868966777)) ;
#155898=CARTESIAN_POINT('Ctrl Pts',(-8.31458553285275,-13.2220547357584,
120.160199104889)) ;
#155899=CARTESIAN_POINT('Ctrl Pts',(-8.38838938005927,-13.2220547937704,
120.135968074736)) ;
#155900=CARTESIAN_POINT('Ctrl Pts',(-8.46219322726581,-13.2220548517825,
120.111737044583)) ;
#155901=CARTESIAN_POINT('Ctrl Pts',(-8.48539533057494,-13.2069305996783,
120.182406906472)) ;
#155902=CARTESIAN_POINT('Ctrl Pts',(-8.50859743388407,-13.191806347574,
120.25307676836)) ;
#155903=CARTESIAN_POINT('Ctrl Pts',(-8.43479358667754,-13.191806289562,
120.277307798513)) ;
#155904=CARTESIAN_POINT('Ctrl Pts',(-8.36098973947101,-13.1918062315499,
120.301538828665)) ;
#155905=CARTESIAN_POINT('Ctrl Pts',(-8.33778763616187,-13.2069304836541,
120.230868966777)) ;
#155906=CARTESIAN_POINT('Ctrl Pts',(-8.35386611104003,-13.4971323588194,
120.244433805866)) ;
#155907=CARTESIAN_POINT('Ctrl Pts',(-8.33024059213342,-13.4920171795336,
120.172474288537)) ;
#155908=CARTESIAN_POINT('Ctrl Pts',(-8.40404443425814,-13.4920172465716,
120.148243242906)) ;
#155909=CARTESIAN_POINT('Ctrl Pts',(-8.47784827638287,-13.4920173136096,
120.124012197275)) ;
#155910=CARTESIAN_POINT('Ctrl Pts',(-8.50147379528949,-13.4971324928954,
120.195971714604)) ;
#155911=CARTESIAN_POINT('Ctrl Pts',(-8.52509931419611,-13.5022476721812,
120.267931231933)) ;
#155912=CARTESIAN_POINT('Ctrl Pts',(-8.45129547207138,-13.5022476051432,
120.292162277563)) ;
#155913=CARTESIAN_POINT('Ctrl Pts',(-8.37749162994666,-13.5022475381053,
120.316393323194)) ;
#155914=CARTESIAN_POINT('Ctrl Pts',(-8.35386611104003,-13.4971323588194,
120.244433805866)) ;
#155915=CARTESIAN_POINT('Ctrl Pts',(-8.34559176606117,-13.7832858649534,
120.183607286869)) ;
#155916=CARTESIAN_POINT('Ctrl Pts',(-8.32324669305239,-13.7581847544607,
120.115547801325)) ;
#155917=CARTESIAN_POINT('Ctrl Pts',(-8.39705052864382,-13.7581848266256,
120.091316735795)) ;
#155918=CARTESIAN_POINT('Ctrl Pts',(-8.47085436423525,-13.7581848987905,
120.067085670265)) ;
#155919=CARTESIAN_POINT('Ctrl Pts',(-8.49319943724403,-13.7832860092831,
120.135145155809)) ;
#155920=CARTESIAN_POINT('Ctrl Pts',(-8.51554451025281,-13.8083871197758,
120.203204641352)) ;
#155921=CARTESIAN_POINT('Ctrl Pts',(-8.44174067466138,-13.808387047611,
120.227435706883)) ;
#155922=CARTESIAN_POINT('Ctrl Pts',(-8.36793683906994,-13.8083869754461,
120.251666772413)) ;
#155923=CARTESIAN_POINT('Ctrl Pts',(-8.34559176606117,-13.7832858649534,
120.183607286869)) ;
#155924=CARTESIAN_POINT('Ctrl Pts',(-8.31464185127322,-14.0408293277911,
120.054056184709)) ;
#155925=CARTESIAN_POINT('Ctrl Pts',(-8.29515542606811,-13.9977110227071,
119.994703679246)) ;
#155926=CARTESIAN_POINT('Ctrl Pts',(-8.36895925493502,-13.997711090453,
119.970472593234)) ;
#155927=CARTESIAN_POINT('Ctrl Pts',(-8.44276308380194,-13.9977111581989,
119.946241507222)) ;
#155928=CARTESIAN_POINT('Ctrl Pts',(-8.46224950900705,-14.0408294632829,
120.005594012685)) ;
#155929=CARTESIAN_POINT('Ctrl Pts',(-8.48173593421216,-14.0839477683669,
120.064946518147)) ;
#155930=CARTESIAN_POINT('Ctrl Pts',(-8.40793210534524,-14.083947700621,
120.089177604159)) ;
#155931=CARTESIAN_POINT('Ctrl Pts',(-8.33412827647834,-14.0839476328751,
120.113408690171)) ;
#155932=CARTESIAN_POINT('Ctrl Pts',(-8.31464185127322,-14.0408293277911,
120.054056184709)) ;
#155933=CARTESIAN_POINT('Ctrl Pts',(-8.26340664177902,-14.255952322556,
119.862377902584)) ;
#155934=CARTESIAN_POINT('Ctrl Pts',(-8.24820592875809,-14.1977519640159,
119.816078985087)) ;
#155935=CARTESIAN_POINT('Ctrl Pts',(-8.32200975066257,-14.1977520218044,
119.791847877869)) ;
#155936=CARTESIAN_POINT('Ctrl Pts',(-8.39581357256705,-14.1977520795929,
119.76761677065)) ;
#155937=CARTESIAN_POINT('Ctrl Pts',(-8.41101428558798,-14.2559524381331,
119.813915688147)) ;
#155938=CARTESIAN_POINT('Ctrl Pts',(-8.4262149986089,-14.3141527966732,
119.860214605644)) ;
#155939=CARTESIAN_POINT('Ctrl Pts',(-8.35241117670443,-14.3141527388846,
119.884445712862)) ;
#155940=CARTESIAN_POINT('Ctrl Pts',(-8.27860735479995,-14.3141526810961,
119.908676820081)) ;
#155941=CARTESIAN_POINT('Ctrl Pts',(-8.26340664177902,-14.255952322556,
119.862377902584)) ;
#155942=CARTESIAN_POINT('Ctrl Pts',(-8.1971249772834,-14.4094466686143,
119.625180693076)) ;
#155943=CARTESIAN_POINT('Ctrl Pts',(-8.18726048315509,-14.3404453655438,
119.595135037421)) ;
#155944=CARTESIAN_POINT('Ctrl Pts',(-8.26106429969089,-14.3404454048825,
119.570903913851)) ;
#155945=CARTESIAN_POINT('Ctrl Pts',(-8.33486811622669,-14.3404454442213,
119.54667279028)) ;
#155946=CARTESIAN_POINT('Ctrl Pts',(-8.344732610355,-14.4094467472918,119.576718445934)) ;
#155947=CARTESIAN_POINT('Ctrl Pts',(-8.35459710448329,-14.4784480503623,
119.606764101589)) ;
#155948=CARTESIAN_POINT('Ctrl Pts',(-8.2807932879475,-14.4784480110235,
119.630995225159)) ;
#155949=CARTESIAN_POINT('Ctrl Pts',(-8.20698947141171,-14.4784479716848,
119.65522634873)) ;
#155950=CARTESIAN_POINT('Ctrl Pts',(-8.1971249772834,-14.4094466686143,
119.625180693076)) ;
#155951=CARTESIAN_POINT('Ctrl Pts',(-8.12040152389499,-14.4929694646286,
119.35593056019)) ;
#155952=CARTESIAN_POINT('Ctrl Pts',(-8.11661493104229,-14.4180358803258,
119.34439721126)) ;
#155953=CARTESIAN_POINT('Ctrl Pts',(-8.19041874362283,-14.4180358961808,
119.320166075642)) ;
#155954=CARTESIAN_POINT('Ctrl Pts',(-8.26422255620336,-14.4180359120358,
119.295934940024)) ;
#155955=CARTESIAN_POINT('Ctrl Pts',(-8.26800914905606,-14.4929694963386,
119.307468288954)) ;
#155956=CARTESIAN_POINT('Ctrl Pts',(-8.27179574190875,-14.5679030806414,
119.319001637885)) ;
#155957=CARTESIAN_POINT('Ctrl Pts',(-8.19799192932821,-14.5679030647864,
119.343232773502)) ;
#155958=CARTESIAN_POINT('Ctrl Pts',(-8.12418811674768,-14.5679030489314,
119.36746390912)) ;
#155959=CARTESIAN_POINT('Ctrl Pts',(-8.12040152389499,-14.4929694646286,
119.35593056019)) ;
#155960=CARTESIAN_POINT('Ctrl Pts',(-8.04009022848257,-14.4990155260453,
119.075851461994)) ;
#155961=CARTESIAN_POINT('Ctrl Pts',(-8.04263890692783,-14.4235500005798,
119.083614327317)) ;
#155962=CARTESIAN_POINT('Ctrl Pts',(-8.11644271815056,-14.4235499890681,
119.059383187563)) ;
#155963=CARTESIAN_POINT('Ctrl Pts',(-8.19024652937329,-14.4235499775565,
119.03515204781)) ;
#155964=CARTESIAN_POINT('Ctrl Pts',(-8.18769785092804,-14.499015503022,
119.027389182487)) ;
#155965=CARTESIAN_POINT('Ctrl Pts',(-8.18514917248278,-14.5744810284875,
119.019626317164)) ;
#155966=CARTESIAN_POINT('Ctrl Pts',(-8.11134536126006,-14.5744810399991,
119.043857456918)) ;
#155967=CARTESIAN_POINT('Ctrl Pts',(-8.03754155003731,-14.5744810515108,
119.068088596671)) ;
#155968=CARTESIAN_POINT('Ctrl Pts',(-8.04009022848257,-14.4990155260453,
119.075851461994)) ;
#155969=CARTESIAN_POINT('Ctrl Pts',(-7.9625098388441,-14.4275804860338,
118.804068220134)) ;
#155970=CARTESIAN_POINT('Ctrl Pts',(-7.97121287685695,-14.3569912762542,
118.830576271749)) ;
#155971=CARTESIAN_POINT('Ctrl Pts',(-8.04501668942195,-14.3569912367052,
118.806345136084)) ;
#155972=CARTESIAN_POINT('Ctrl Pts',(-8.11882050198696,-14.3569911971563,
118.782114000419)) ;
#155973=CARTESIAN_POINT('Ctrl Pts',(-8.11011746397412,-14.4275804069359,
118.755605948804)) ;
#155974=CARTESIAN_POINT('Ctrl Pts',(-8.10141442596128,-14.4981696167155,
118.729097897188)) ;
#155975=CARTESIAN_POINT('Ctrl Pts',(-8.02761061339627,-14.4981696562644,
118.753329032853)) ;
#155976=CARTESIAN_POINT('Ctrl Pts',(-7.95380680083127,-14.4981696958134,
118.777560168518)) ;
#155977=CARTESIAN_POINT('Ctrl Pts',(-7.9625098388441,-14.4275804860338,
118.804068220134)) ;
#155978=CARTESIAN_POINT('Ctrl Pts',(-7.8941100124004,-14.284309082368,118.560336785865)) ;
#155979=CARTESIAN_POINT('Ctrl Pts',(-7.90833367643576,-14.223618657059,
118.603659773624)) ;
#155980=CARTESIAN_POINT('Ctrl Pts',(-7.98213749300733,-14.2236185917218,
118.579428650163)) ;
#155981=CARTESIAN_POINT('Ctrl Pts',(-8.05594130957889,-14.2236185263845,
118.555197526701)) ;
#155982=CARTESIAN_POINT('Ctrl Pts',(-8.04171764554352,-14.2843089516935,
118.511874538942)) ;
#155983=CARTESIAN_POINT('Ctrl Pts',(-8.02749398150816,-14.3449993770025,
118.468551551182)) ;
#155984=CARTESIAN_POINT('Ctrl Pts',(-7.95369016493661,-14.3449994423398,
118.492782674643)) ;
#155985=CARTESIAN_POINT('Ctrl Pts',(-7.87988634836503,-14.3449995076771,
118.517013798105)) ;
#155986=CARTESIAN_POINT('Ctrl Pts',(-7.8941100124004,-14.284309082368,118.560336785865)) ;
#155987=CARTESIAN_POINT('Ctrl Pts',(-7.84012347499757,-14.0775350374868,
118.360268383229)) ;
#155988=CARTESIAN_POINT('Ctrl Pts',(-7.85887471453744,-14.0311904705444,
118.417381635461)) ;
#155989=CARTESIAN_POINT('Ctrl Pts',(-7.93267853746199,-14.0311903843125,
118.39315053135)) ;
#155990=CARTESIAN_POINT('Ctrl Pts',(-8.00648236038654,-14.0311902980806,
118.368919427238)) ;
#155991=CARTESIAN_POINT('Ctrl Pts',(-7.98773112084667,-14.0775348650229,
118.311806175006)) ;
#155992=CARTESIAN_POINT('Ctrl Pts',(-7.96897988130681,-14.1238794319653,
118.254692922774)) ;
#155993=CARTESIAN_POINT('Ctrl Pts',(-7.89517605838225,-14.1238795181972,
118.278924026886)) ;
#155994=CARTESIAN_POINT('Ctrl Pts',(-7.8213722354577,-14.1238796044292,
118.303155130997)) ;
#155995=CARTESIAN_POINT('Ctrl Pts',(-7.84012347499757,-14.0775350374868,
118.360268383229)) ;
#155996=CARTESIAN_POINT('Ctrl Pts',(-7.80588583848825,-13.8261134335288,
118.220747745965)) ;
#155997=CARTESIAN_POINT('Ctrl Pts',(-7.82778425353249,-13.7972540806325,
118.287446786978)) ;
#155998=CARTESIAN_POINT('Ctrl Pts',(-7.90158808437181,-13.7972539806286,
118.263215706973)) ;
#155999=CARTESIAN_POINT('Ctrl Pts',(-7.97539191521112,-13.7972538806247,
118.238984626969)) ;
#156000=CARTESIAN_POINT('Ctrl Pts',(-7.95349350016687,-13.826113233521,
118.172285585957)) ;
#156001=CARTESIAN_POINT('Ctrl Pts',(-7.93159508512261,-13.8549725864173,
118.105586544944)) ;
#156002=CARTESIAN_POINT('Ctrl Pts',(-7.85779125428331,-13.8549726864212,
118.129817624949)) ;
#156003=CARTESIAN_POINT('Ctrl Pts',(-7.78398742344399,-13.8549727864252,
118.154048704953)) ;
#156004=CARTESIAN_POINT('Ctrl Pts',(-7.80588583848825,-13.8261134335288,
118.220747745965)) ;
#156005=CARTESIAN_POINT('Ctrl Pts',(-7.79385768957157,-13.5428648342343,
118.148500404782)) ;
#156006=CARTESIAN_POINT('Ctrl Pts',(-7.81736543683943,-13.5337376171051,
118.220101212043)) ;
#156007=CARTESIAN_POINT('Ctrl Pts',(-7.89116927654803,-13.5337375120109,
118.195870159053)) ;
#156008=CARTESIAN_POINT('Ctrl Pts',(-7.96497311625663,-13.5337374069167,
118.171639106063)) ;
#156009=CARTESIAN_POINT('Ctrl Pts',(-7.94146536898876,-13.5428646240459,
118.100038298802)) ;
#156010=CARTESIAN_POINT('Ctrl Pts',(-7.9179576217209,-13.551991841175,118.028437491541)) ;
#156011=CARTESIAN_POINT('Ctrl Pts',(-7.84415378201231,-13.5519919462692,
118.052668544531)) ;
#156012=CARTESIAN_POINT('Ctrl Pts',(-7.7703499423037,-13.5519920513634,
118.076899597521)) ;
#156013=CARTESIAN_POINT('Ctrl Pts',(-7.79385768957157,-13.5428648342343,
118.148500404782)) ;
#156014=CARTESIAN_POINT('Ctrl Pts',(-7.80612682657335,-13.252182353688,
118.150461687266)) ;
#156015=CARTESIAN_POINT('Ctrl Pts',(-7.82954570480992,-13.263336213575,
118.22179181374)) ;
#156016=CARTESIAN_POINT('Ctrl Pts',(-7.90334955320528,-13.2633361119795,
118.197560787209)) ;
#156017=CARTESIAN_POINT('Ctrl Pts',(-7.97715340160061,-13.2633360103841,
118.173329760677)) ;
#156018=CARTESIAN_POINT('Ctrl Pts',(-7.95373452336405,-13.2521821504971,
118.101999634203)) ;
#156019=CARTESIAN_POINT('Ctrl Pts',(-7.93031564512747,-13.2410282906101,
118.030669507729)) ;
#156020=CARTESIAN_POINT('Ctrl Pts',(-7.85651179673213,-13.2410283922056,
118.05490053426)) ;
#156021=CARTESIAN_POINT('Ctrl Pts',(-7.78270794833677,-13.241028493801,
118.079131560792)) ;
#156022=CARTESIAN_POINT('Ctrl Pts',(-7.80612682657335,-13.252182353688,
118.150461687266)) ;
#156023=CARTESIAN_POINT('Ctrl Pts',(-7.84228893480843,-12.9730234465435,
118.225161565708)) ;
#156024=CARTESIAN_POINT('Ctrl Pts',(-7.86395152537764,-13.0036840588297,
118.29114232325)) ;
#156025=CARTESIAN_POINT('Ctrl Pts',(-7.9377553815644,-13.0036839686776,
118.26691132045)) ;
#156026=CARTESIAN_POINT('Ctrl Pts',(-8.01155923775114,-13.0036838785254,
118.242680317649)) ;
#156027=CARTESIAN_POINT('Ctrl Pts',(-7.98989664718192,-12.9730232662392,
118.176699560108)) ;
#156028=CARTESIAN_POINT('Ctrl Pts',(-7.9682340566127,-12.9423626539529,
118.110718802566)) ;
#156029=CARTESIAN_POINT('Ctrl Pts',(-7.89443020042595,-12.942362744105,
118.134949805366)) ;
#156030=CARTESIAN_POINT('Ctrl Pts',(-7.8206263442392,-12.9423628342572,
118.159180808167)) ;
#156031=CARTESIAN_POINT('Ctrl Pts',(-7.84228893480843,-12.9730234465435,
118.225161565708)) ;
#156032=CARTESIAN_POINT('Ctrl Pts',(-7.90103421558884,-12.724731390434,
118.368470996422)) ;
#156033=CARTESIAN_POINT('Ctrl Pts',(-7.91936506739964,-12.77277340565,118.424303815163)) ;
#156034=CARTESIAN_POINT('Ctrl Pts',(-7.99316892941168,-12.7727733343003,
118.400072830106)) ;
#156035=CARTESIAN_POINT('Ctrl Pts',(-8.06697279142372,-12.7727732629506,
118.375841845048)) ;
#156036=CARTESIAN_POINT('Ctrl Pts',(-8.04864193961291,-12.7247312477346,
118.320009026308)) ;
#156037=CARTESIAN_POINT('Ctrl Pts',(-8.0303110878021,-12.6766892325185,
118.264176207567)) ;
#156038=CARTESIAN_POINT('Ctrl Pts',(-7.95650722579007,-12.6766893038683,
118.288407192625)) ;
#156039=CARTESIAN_POINT('Ctrl Pts',(-7.88270336377803,-12.676689375218,
118.312638177682)) ;
#156040=CARTESIAN_POINT('Ctrl Pts',(-7.90103421558884,-12.724731390434,
118.368470996422)) ;
#156041=CARTESIAN_POINT('Ctrl Pts',(-7.97782116130876,-12.5280561031159,
118.567077843843)) ;
#156042=CARTESIAN_POINT('Ctrl Pts',(-7.99154820293211,-12.5899016984486,
118.608888199484)) ;
#156043=CARTESIAN_POINT('Ctrl Pts',(-8.06535206896777,-12.5899016481567,
118.584657226682)) ;
#156044=CARTESIAN_POINT('Ctrl Pts',(-8.13915593500343,-12.5899015978648,
118.56042625388)) ;
#156045=CARTESIAN_POINT('Ctrl Pts',(-8.12542889338008,-12.5280560025322,
118.518615898239)) ;
#156046=CARTESIAN_POINT('Ctrl Pts',(-8.11170185175672,-12.4662104071995,
118.476805542598)) ;
#156047=CARTESIAN_POINT('Ctrl Pts',(-8.03789798572106,-12.4662104574914,
118.5010365154)) ;
#156048=CARTESIAN_POINT('Ctrl Pts',(-7.96409411968541,-12.4662105077833,
118.525267488202)) ;
#156049=CARTESIAN_POINT('Ctrl Pts',(-7.97782116130876,-12.5280561031159,
118.567077843843)) ;
#156050=CARTESIAN_POINT('Ctrl Pts',(-8.0692686377754,-12.3935893009494,
118.810023631757)) ;
#156051=CARTESIAN_POINT('Ctrl Pts',(-8.07736813977987,-12.4649167907205,
118.834693409571)) ;
#156052=CARTESIAN_POINT('Ctrl Pts',(-8.15117200694027,-12.464916764178,
118.810462440194)) ;
#156053=CARTESIAN_POINT('Ctrl Pts',(-8.22497587410067,-12.4649167376354,
118.786231470818)) ;
#156054=CARTESIAN_POINT('Ctrl Pts',(-8.21687637209619,-12.3935892478642,
118.761561693005)) ;
#156055=CARTESIAN_POINT('Ctrl Pts',(-8.20877687009171,-12.322261758093,
118.736891915191)) ;
#156056=CARTESIAN_POINT('Ctrl Pts',(-8.13497300293131,-12.3222617846356,
118.761122884567)) ;
#156057=CARTESIAN_POINT('Ctrl Pts',(-8.06116913577091,-12.3222618111782,
118.785353853944)) ;
#156058=CARTESIAN_POINT('Ctrl Pts',(-8.0692686377754,-12.3935893009494,
118.810023631757)) ;
#156059=CARTESIAN_POINT('Ctrl Pts',(-8.16837016553241,-12.333081965445,
119.076502994386)) ;
#156060=CARTESIAN_POINT('Ctrl Pts',(-8.17029452669112,-12.4087416290775,
119.08236428941)) ;
#156061=CARTESIAN_POINT('Ctrl Pts',(-8.24409839311102,-12.4087416242859,
119.058133317778)) ;
#156062=CARTESIAN_POINT('Ctrl Pts',(-8.31790225953092,-12.4087416194943,
119.033902346147)) ;
#156063=CARTESIAN_POINT('Ctrl Pts',(-8.31597789837221,-12.3330819558618,
119.028041051122)) ;
#156064=CARTESIAN_POINT('Ctrl Pts',(-8.31405353721349,-12.2574222922293,
119.022179756098)) ;
#156065=CARTESIAN_POINT('Ctrl Pts',(-8.24024967079359,-12.2574222970209,
119.04641072773)) ;
#156066=CARTESIAN_POINT('Ctrl Pts',(-8.16644580437368,-12.2574223018125,
119.070641699362)) ;
#156067=CARTESIAN_POINT('Ctrl Pts',(-8.16837016553241,-12.333081965445,
119.076502994386)) ;
#156068=CARTESIAN_POINT('Ctrl Pts',(-8.27009279108481,-12.3505128306963,
119.350670896121)) ;
#156069=CARTESIAN_POINT('Ctrl Pts',(-8.26565575692453,-12.4250706656238,
119.33715640722)) ;
#156070=CARTESIAN_POINT('Ctrl Pts',(-8.33945961991325,-12.4250706786686,
119.312925425138)) ;
#156071=CARTESIAN_POINT('Ctrl Pts',(-8.41326348290199,-12.4250706917134,
119.288694443055)) ;
#156072=CARTESIAN_POINT('Ctrl Pts',(-8.41770051706228,-12.3505128567859,
119.302208931956)) ;
#156073=CARTESIAN_POINT('Ctrl Pts',(-8.42213755122257,-12.2759550218584,
119.315723420857)) ;
#156074=CARTESIAN_POINT('Ctrl Pts',(-8.34833368823383,-12.2759550088136,
119.33995440294)) ;
#156075=CARTESIAN_POINT('Ctrl Pts',(-8.2745298252451,-12.2759549957688,
119.364185385022)) ;
#156076=CARTESIAN_POINT('Ctrl Pts',(-8.27009279108481,-12.3505128306963,
119.350670896121)) ;
#156077=CARTESIAN_POINT('Ctrl Pts',(-8.3658449010965,-12.4433828921911,
119.60714075347)) ;
#156078=CARTESIAN_POINT('Ctrl Pts',(-8.35544359845222,-12.5115686405398,
119.575460064988)) ;
#156079=CARTESIAN_POINT('Ctrl Pts',(-8.42924745806618,-12.5115686671103,
119.551229072627)) ;
#156080=CARTESIAN_POINT('Ctrl Pts',(-8.50305131768015,-12.5115686936807,
119.526998080265)) ;
#156081=CARTESIAN_POINT('Ctrl Pts',(-8.51345262032444,-12.443382945332,
119.558678768747)) ;
#156082=CARTESIAN_POINT('Ctrl Pts',(-8.52385392296872,-12.3751971969833,
119.590359457229)) ;
#156083=CARTESIAN_POINT('Ctrl Pts',(-8.45005006335476,-12.3751971704129,
119.614590449591)) ;
#156084=CARTESIAN_POINT('Ctrl Pts',(-8.37624620374079,-12.3751971438424,
119.638821441952)) ;
#156085=CARTESIAN_POINT('Ctrl Pts',(-8.3658449010965,-12.4433828921911,
119.60714075347)) ;
#156086=CARTESIAN_POINT('Ctrl Pts',(-8.45197505795687,-12.607349424796,
119.833841108759)) ;
#156087=CARTESIAN_POINT('Ctrl Pts',(-8.43628164446657,-12.6641907157574,
119.786041504319)) ;
#156088=CARTESIAN_POINT('Ctrl Pts',(-8.51008549888229,-12.6641907484467,
119.761810496124)) ;
#156089=CARTESIAN_POINT('Ctrl Pts',(-8.58388935329801,-12.664190781136,
119.73757948793)) ;
#156090=CARTESIAN_POINT('Ctrl Pts',(-8.59958276678831,-12.6073494901747,
119.78537909237)) ;
#156091=CARTESIAN_POINT('Ctrl Pts',(-8.6152761802786,-12.5505081992133,
119.83317869681)) ;
#156092=CARTESIAN_POINT('Ctrl Pts',(-8.54147232586288,-12.5505081665239,
119.857409705004)) ;
#156093=CARTESIAN_POINT('Ctrl Pts',(-8.46766847144716,-12.5505081338346,
119.881640713199)) ;
#156094=CARTESIAN_POINT('Ctrl Pts',(-8.45197505795687,-12.607349424796,
119.833841108759)) ;
#156095=CARTESIAN_POINT('Ctrl Pts',(-8.52120977492203,-12.8279036385121,
120.00940010572)) ;
#156096=CARTESIAN_POINT('Ctrl Pts',(-8.50138939635353,-12.8694313461383,
119.949030431395)) ;
#156097=CARTESIAN_POINT('Ctrl Pts',(-8.57519324644018,-12.8694313807778,
119.924799410014)) ;
#156098=CARTESIAN_POINT('Ctrl Pts',(-8.64899709652682,-12.8694314154173,
119.900568388634)) ;
#156099=CARTESIAN_POINT('Ctrl Pts',(-8.66881747509531,-12.8279037077911,
119.96093806296)) ;
#156100=CARTESIAN_POINT('Ctrl Pts',(-8.68863785366382,-12.7863760001649,
120.021307737286)) ;
#156101=CARTESIAN_POINT('Ctrl Pts',(-8.61483400357718,-12.7863759655254,
120.045538758666)) ;
#156102=CARTESIAN_POINT('Ctrl Pts',(-8.54103015349054,-12.7863759308859,
120.069769780046)) ;
#156103=CARTESIAN_POINT('Ctrl Pts',(-8.52120977492203,-12.8279036385121,
120.00940010572)) ;
#156104=CARTESIAN_POINT('Ctrl Pts',(-8.57055325895007,-13.0930059035689,
120.124025527535)) ;
#156105=CARTESIAN_POINT('Ctrl Pts',(-8.54799540220528,-13.1160865947577,
120.055317936172)) ;
#156106=CARTESIAN_POINT('Ctrl Pts',(-8.62179924818873,-13.1160866238806,
120.031086902294)) ;
#156107=CARTESIAN_POINT('Ctrl Pts',(-8.69560309417219,-13.1160866530036,
120.006855868416)) ;
#156108=CARTESIAN_POINT('Ctrl Pts',(-8.71816095091697,-13.0930059618148,
120.075563459779)) ;
#156109=CARTESIAN_POINT('Ctrl Pts',(-8.74071880766174,-13.069925270626,
120.144271051143)) ;
#156110=CARTESIAN_POINT('Ctrl Pts',(-8.6669149616783,-13.069925241503,120.168502085021)) ;
#156111=CARTESIAN_POINT('Ctrl Pts',(-8.59311111569484,-13.0699252123801,
120.192733118899)) ;
#156112=CARTESIAN_POINT('Ctrl Pts',(-8.57055325895007,-13.0930059035689,
120.124025527535)) ;
#156113=CARTESIAN_POINT('Ctrl Pts',(-8.59625204583721,-13.3789266137586,
120.166977376249)) ;
#156114=CARTESIAN_POINT('Ctrl Pts',(-8.57259671566402,-13.3820781397035,
120.094927057768)) ;
#156115=CARTESIAN_POINT('Ctrl Pts',(-8.64640055914781,-13.3820781631016,
120.070696016276)) ;
#156116=CARTESIAN_POINT('Ctrl Pts',(-8.72020440263158,-13.3820781864996,
120.046464974784)) ;
#156117=CARTESIAN_POINT('Ctrl Pts',(-8.74385973280477,-13.3789266605547,
120.118515293266)) ;
#156118=CARTESIAN_POINT('Ctrl Pts',(-8.76751506297795,-13.3757751346097,
120.190565611747)) ;
#156119=CARTESIAN_POINT('Ctrl Pts',(-8.69371121949417,-13.3757751112117,
120.214796653239)) ;
#156120=CARTESIAN_POINT('Ctrl Pts',(-8.61990737601039,-13.3757750878137,
120.239027694731)) ;
#156121=CARTESIAN_POINT('Ctrl Pts',(-8.59625204583721,-13.3789266137586,
120.166977376249)) ;
#156122=CARTESIAN_POINT('Ctrl Pts',(-8.59788852250651,-13.6686885717782,
120.136495690536)) ;
#156123=CARTESIAN_POINT('Ctrl Pts',(-8.57481707676371,-13.6516124113894,
120.066223789672)) ;
#156124=CARTESIAN_POINT('Ctrl Pts',(-8.64862091882858,-13.6516124266104,
120.041992743859)) ;
#156125=CARTESIAN_POINT('Ctrl Pts',(-8.72242476089344,-13.6516124418314,
120.017761698045)) ;
#156126=CARTESIAN_POINT('Ctrl Pts',(-8.74549620663624,-13.6686886022201,
120.088033598909)) ;
#156127=CARTESIAN_POINT('Ctrl Pts',(-8.76856765237905,-13.6857647626089,
120.158305499772)) ;
#156128=CARTESIAN_POINT('Ctrl Pts',(-8.69476381031418,-13.6857647473879,
120.182536545585)) ;
#156129=CARTESIAN_POINT('Ctrl Pts',(-8.62095996824932,-13.6857647321669,
120.206767591399)) ;
#156130=CARTESIAN_POINT('Ctrl Pts',(-8.59788852250651,-13.6686885717782,
120.136495690536)) ;
#156131=CARTESIAN_POINT('Ctrl Pts',(-8.57580906244584,-13.9407698971193,
120.033752331659)) ;
#156132=CARTESIAN_POINT('Ctrl Pts',(-8.55497897586174,-13.9046696710089,
119.970307249017)) ;
#156133=CARTESIAN_POINT('Ctrl Pts',(-8.62878281778872,-13.904669678464,
119.946076202783)) ;
#156134=CARTESIAN_POINT('Ctrl Pts',(-8.70258665971571,-13.9046696859191,
119.92184515655)) ;
#156135=CARTESIAN_POINT('Ctrl Pts',(-8.72341674629981,-13.9407699120296,
119.985290239192)) ;
#156136=CARTESIAN_POINT('Ctrl Pts',(-8.74424683288391,-13.97687013814,120.048735321835)) ;
#156137=CARTESIAN_POINT('Ctrl Pts',(-8.67044299095692,-13.9768701306849,
120.072966368068)) ;
#156138=CARTESIAN_POINT('Ctrl Pts',(-8.59663914902995,-13.9768701232298,
120.097197414301)) ;
#156139=CARTESIAN_POINT('Ctrl Pts',(-8.57580906244584,-13.9407698971193,
120.033752331659)) ;
#156140=CARTESIAN_POINT('Ctrl Pts',(-8.53228870836988,-14.1754452261927,
119.865663575393)) ;
#156141=CARTESIAN_POINT('Ctrl Pts',(-8.51520149123549,-14.122903887043,
119.813618669073)) ;
#156142=CARTESIAN_POINT('Ctrl Pts',(-8.58900533389292,-14.1229038889288,
119.789387625064)) ;
#156143=CARTESIAN_POINT('Ctrl Pts',(-8.66280917655036,-14.1229038908147,
119.765156581056)) ;
#156144=CARTESIAN_POINT('Ctrl Pts',(-8.67989639368476,-14.1754452299645,
119.817201487376)) ;
#156145=CARTESIAN_POINT('Ctrl Pts',(-8.69698361081914,-14.2279865691142,
119.869246393697)) ;
#156146=CARTESIAN_POINT('Ctrl Pts',(-8.6231797681617,-14.2279865672284,
119.893477437705)) ;
#156147=CARTESIAN_POINT('Ctrl Pts',(-8.54937592550426,-14.2279865653425,
119.917708481714)) ;
#156148=CARTESIAN_POINT('Ctrl Pts',(-8.53228870836988,-14.1754452261927,
119.865663575393)) ;
#156149=CARTESIAN_POINT('Ctrl Pts',(-8.47162858688881,-14.3550939223612,
119.645549235714)) ;
#156150=CARTESIAN_POINT('Ctrl Pts',(-8.45948313829748,-14.2899298530335,
119.608556158953)) ;
#156151=CARTESIAN_POINT('Ctrl Pts',(-8.5332869818319,-14.2899298524596,
119.584325117616)) ;
#156152=CARTESIAN_POINT('Ctrl Pts',(-8.60709082536632,-14.2899298518858,
119.560094076279)) ;
#156153=CARTESIAN_POINT('Ctrl Pts',(-8.61923627395765,-14.3550939212134,
119.597087153039)) ;
#156154=CARTESIAN_POINT('Ctrl Pts',(-8.63138172254897,-14.4202579905411,
119.634080229799)) ;
#156155=CARTESIAN_POINT('Ctrl Pts',(-8.55757787901455,-14.420257991115,
119.658311271137)) ;
#156156=CARTESIAN_POINT('Ctrl Pts',(-8.48377403548013,-14.4202579916889,
119.682542312474)) ;
#156157=CARTESIAN_POINT('Ctrl Pts',(-8.47162858688881,-14.3550939223612,
119.645549235714)) ;
#156158=CARTESIAN_POINT('Ctrl Pts',(-8.39799248590873,-14.468598908444,
119.385596001449)) ;
#156159=CARTESIAN_POINT('Ctrl Pts',(-8.3917090967398,-14.3954110161889,
119.366457811798)) ;
#156160=CARTESIAN_POINT('Ctrl Pts',(-8.46551294113031,-14.3954110152214,
119.342226773068)) ;
#156161=CARTESIAN_POINT('Ctrl Pts',(-8.53931678552082,-14.395411014254,
119.317995734338)) ;
#156162=CARTESIAN_POINT('Ctrl Pts',(-8.54560017468974,-14.4685989065091,
119.337133923989)) ;
#156163=CARTESIAN_POINT('Ctrl Pts',(-8.55188356385866,-14.5417867987642,
119.35627211364)) ;
#156164=CARTESIAN_POINT('Ctrl Pts',(-8.47807971946816,-14.5417867997317,
119.38050315237)) ;
#156165=CARTESIAN_POINT('Ctrl Pts',(-8.40427587507765,-14.5417868006991,
119.4047341911)) ;
#156166=CARTESIAN_POINT('Ctrl Pts',(-8.39799248590873,-14.468598908444,
119.385596001449)) ;
#156167=CARTESIAN_POINT('Ctrl Pts',(-8.31877491440371,-14.5058659881171,
119.109007145666)) ;
#156168=CARTESIAN_POINT('Ctrl Pts',(-8.31874453084561,-14.4299679241318,
119.108914602191)) ;
#156169=CARTESIAN_POINT('Ctrl Pts',(-8.39254837521704,-14.4299679242476,
119.084683563403)) ;
#156170=CARTESIAN_POINT('Ctrl Pts',(-8.46635221958846,-14.4299679243634,
119.060452524615)) ;
#156171=CARTESIAN_POINT('Ctrl Pts',(-8.46638260314656,-14.5058659883488,
119.06054506809)) ;
#156172=CARTESIAN_POINT('Ctrl Pts',(-8.46641298670466,-14.5817640523341,
119.060637611565)) ;
#156173=CARTESIAN_POINT('Ctrl Pts',(-8.39260914233323,-14.5817640522183,
119.084868650353)) ;
#156174=CARTESIAN_POINT('Ctrl Pts',(-8.31880529796181,-14.5817640521025,
119.109099689141)) ;
#156175=CARTESIAN_POINT('Ctrl Pts',(-8.31877491440371,-14.5058659881171,
119.109007145666)) ;
#156176=CARTESIAN_POINT('Ctrl Pts',(-8.23941378855136,-14.465907705861,
118.831859781048)) ;
#156177=CARTESIAN_POINT('Ctrl Pts',(-8.24565808732545,-14.3926881487027,
118.850878907574)) ;
#156178=CARTESIAN_POINT('Ctrl Pts',(-8.31946193110952,-14.3926881492861,
118.826647866997)) ;
#156179=CARTESIAN_POINT('Ctrl Pts',(-8.3932657748936,-14.3926881498695,
118.80241682642)) ;
#156180=CARTESIAN_POINT('Ctrl Pts',(-8.38702147611951,-14.4659077070278,
118.783397699894)) ;
#156181=CARTESIAN_POINT('Ctrl Pts',(-8.38077717734542,-14.5391272641861,
118.764378573367)) ;
#156182=CARTESIAN_POINT('Ctrl Pts',(-8.30697333356135,-14.5391272636027,
118.788609613944)) ;
#156183=CARTESIAN_POINT('Ctrl Pts',(-8.23316948977728,-14.5391272630193,
118.812840654521)) ;
#156184=CARTESIAN_POINT('Ctrl Pts',(-8.23941378855136,-14.465907705861,
118.831859781048)) ;
#156185=CARTESIAN_POINT('Ctrl Pts',(-8.16647270185438,-14.3507454275659,
118.574221540228)) ;
#156186=CARTESIAN_POINT('Ctrl Pts',(-8.17855345341657,-14.2854599330561,
118.611017560312)) ;
#156187=CARTESIAN_POINT('Ctrl Pts',(-8.25235729609328,-14.2854599321569,
118.586786516362)) ;
#156188=CARTESIAN_POINT('Ctrl Pts',(-8.32616113876998,-14.2854599312576,
118.562555472413)) ;
#156189=CARTESIAN_POINT('Ctrl Pts',(-8.31408038720779,-14.3507454257675,
118.525759452328)) ;
#156190=CARTESIAN_POINT('Ctrl Pts',(-8.30199963564559,-14.4160309202774,
118.488963432244)) ;
#156191=CARTESIAN_POINT('Ctrl Pts',(-8.22819579296889,-14.4160309211766,
118.513194476194)) ;
#156192=CARTESIAN_POINT('Ctrl Pts',(-8.15439195029218,-14.4160309220758,
118.537425520144)) ;
#156193=CARTESIAN_POINT('Ctrl Pts',(-8.16647270185438,-14.3507454275659,
118.574221540228)) ;
#156194=CARTESIAN_POINT('Ctrl Pts',(-8.10601871451368,-14.1684902162708,
118.354580107972)) ;
#156195=CARTESIAN_POINT('Ctrl Pts',(-8.12307315420655,-14.1158354027091,
118.406525179709)) ;
#156196=CARTESIAN_POINT('Ctrl Pts',(-8.19687699576229,-14.1158353972228,
118.382294132345)) ;
#156197=CARTESIAN_POINT('Ctrl Pts',(-8.27068083731801,-14.1158353917364,
118.358063084981)) ;
#156198=CARTESIAN_POINT('Ctrl Pts',(-8.25362639762513,-14.1684902052981,
118.306118013244)) ;
#156199=CARTESIAN_POINT('Ctrl Pts',(-8.23657195793224,-14.2211450188598,
118.254172941506)) ;
#156200=CARTESIAN_POINT('Ctrl Pts',(-8.16276811637651,-14.2211450243462,
118.278403988871)) ;
#156201=CARTESIAN_POINT('Ctrl Pts',(-8.08896427482079,-14.2211450298325,
118.302635036235)) ;
#156202=CARTESIAN_POINT('Ctrl Pts',(-8.10601871451368,-14.1684902162708,
118.354580107972)) ;
#156203=CARTESIAN_POINT('Ctrl Pts',(-8.06327379464778,-13.9330107336615,
118.188967146787)) ;
#156204=CARTESIAN_POINT('Ctrl Pts',(-8.08407054318253,-13.8967214466837,
118.252310687557)) ;
#156205=CARTESIAN_POINT('Ctrl Pts',(-8.15787438431086,-13.8967214344113,
118.228079638891)) ;
#156206=CARTESIAN_POINT('Ctrl Pts',(-8.23167822543917,-13.8967214221389,
118.203848590225)) ;
#156207=CARTESIAN_POINT('Ctrl Pts',(-8.21088147690444,-13.9330107091168,
118.140505049456)) ;
#156208=CARTESIAN_POINT('Ctrl Pts',(-8.19008472836968,-13.9692999960946,
118.077161508686)) ;
#156209=CARTESIAN_POINT('Ctrl Pts',(-8.11628088724137,-13.969300008367,
118.101392557352)) ;
#156210=CARTESIAN_POINT('Ctrl Pts',(-8.04247704611305,-13.9693000206394,
118.125623606018)) ;
#156211=CARTESIAN_POINT('Ctrl Pts',(-8.06327379464778,-13.9330107336615,
118.188967146787)) ;
#156212=CARTESIAN_POINT('Ctrl Pts',(-8.04188464728271,-13.6600763512271,
118.088315145107)) ;
#156213=CARTESIAN_POINT('Ctrl Pts',(-8.06493974041926,-13.6427914121404,
118.158537239301)) ;
#156214=CARTESIAN_POINT('Ctrl Pts',(-8.13874358210421,-13.6427913908253,
118.134306192331)) ;
#156215=CARTESIAN_POINT('Ctrl Pts',(-8.21254742378915,-13.6427913695102,
118.11007514536)) ;
#156216=CARTESIAN_POINT('Ctrl Pts',(-8.18949233065261,-13.6600763085969,
118.039853051166)) ;
#156217=CARTESIAN_POINT('Ctrl Pts',(-8.16643723751604,-13.6773612476836,
117.969630956972)) ;
#156218=CARTESIAN_POINT('Ctrl Pts',(-8.09263339583109,-13.6773612689987,
117.993862003942)) ;
#156219=CARTESIAN_POINT('Ctrl Pts',(-8.01882955414613,-13.6773612903137,
118.018093050913)) ;
#156220=CARTESIAN_POINT('Ctrl Pts',(-8.04188464728271,-13.6600763512271,
118.088315145107)) ;
#156221=CARTESIAN_POINT('Ctrl Pts',(-8.04415984284868,-13.3704757504778,
118.059833665652)) ;
#156222=CARTESIAN_POINT('Ctrl Pts',(-8.06782216910361,-13.3733860820227,
118.131905294094)) ;
#156223=CARTESIAN_POINT('Ctrl Pts',(-8.1416260126549,-13.3733860523621,
118.107674252808)) ;
#156224=CARTESIAN_POINT('Ctrl Pts',(-8.21542985620619,-13.3733860227015,
118.083443211523)) ;
#156225=CARTESIAN_POINT('Ctrl Pts',(-8.19176752995126,-13.3704756911566,
118.01137158308)) ;
#156226=CARTESIAN_POINT('Ctrl Pts',(-8.16810520369634,-13.3675653596117,
117.939299954637)) ;
#156227=CARTESIAN_POINT('Ctrl Pts',(-8.09430136014505,-13.3675653892723,
117.963530995923)) ;
#156228=CARTESIAN_POINT('Ctrl Pts',(-8.02049751659377,-13.3675654189329,
117.987762037209)) ;
#156229=CARTESIAN_POINT('Ctrl Pts',(-8.04415984284868,-13.3704757504778,
118.059833665652)) ;
#156230=CARTESIAN_POINT('Ctrl Pts',(-8.07098859328993,-13.0823700026988,
118.105885959188)) ;
#156231=CARTESIAN_POINT('Ctrl Pts',(-8.09355009795567,-13.1054004112685,
118.17460466289)) ;
#156232=CARTESIAN_POINT('Ctrl Pts',(-8.16735394500072,-13.1054003729185,
118.150373632246)) ;
#156233=CARTESIAN_POINT('Ctrl Pts',(-8.24115779204577,-13.1054003345686,
118.126142601601)) ;
#156234=CARTESIAN_POINT('Ctrl Pts',(-8.21859628738003,-13.0823699259989,
118.057423897899)) ;
#156235=CARTESIAN_POINT('Ctrl Pts',(-8.19603478271429,-13.0593395174292,
117.988705194198)) ;
#156236=CARTESIAN_POINT('Ctrl Pts',(-8.12223093566923,-13.0593395557792,
118.012936224842)) ;
#156237=CARTESIAN_POINT('Ctrl Pts',(-8.04842708862418,-13.0593395941291,
118.037167255487)) ;
#156238=CARTESIAN_POINT('Ctrl Pts',(-8.07098859328993,-13.0823700026988,
118.105885959188)) ;
#156239=CARTESIAN_POINT('Ctrl Pts',(-8.120503467602,-12.8213180178566,118.221441446184)) ;
#156240=CARTESIAN_POINT('Ctrl Pts',(-8.14036987651576,-12.8626079589609,
118.281951323206)) ;
#156241=CARTESIAN_POINT('Ctrl Pts',(-8.21417372776093,-12.862607919451,
118.257720305355)) ;
#156242=CARTESIAN_POINT('Ctrl Pts',(-8.2879775790061,-12.8626078799411,
118.233489287503)) ;
#156243=CARTESIAN_POINT('Ctrl Pts',(-8.26811117009233,-12.8213179388368,
118.172979410481)) ;
#156244=CARTESIAN_POINT('Ctrl Pts',(-8.24824476117856,-12.7800279977325,
118.112469533458)) ;
#156245=CARTESIAN_POINT('Ctrl Pts',(-8.1744409099334,-12.7800280372424,
118.13670055131)) ;
#156246=CARTESIAN_POINT('Ctrl Pts',(-8.10063705868823,-12.7800280767523,
118.160931569162)) ;
#156247=CARTESIAN_POINT('Ctrl Pts',(-8.120503467602,-12.8213180178566,118.221441446184)) ;
#156248=CARTESIAN_POINT('Ctrl Pts',(-8.19068066224925,-12.6009816910039,
118.399651162582)) ;
#156249=CARTESIAN_POINT('Ctrl Pts',(-8.20641152323964,-12.6577150521394,
118.44756482808)) ;
#156250=CARTESIAN_POINT('Ctrl Pts',(-8.28021537965013,-12.6577150144821,
118.423333825961)) ;
#156251=CARTESIAN_POINT('Ctrl Pts',(-8.35401923606062,-12.6577149768248,
118.399102823842)) ;
#156252=CARTESIAN_POINT('Ctrl Pts',(-8.33828837507023,-12.6009816156892,
118.351189158345)) ;
#156253=CARTESIAN_POINT('Ctrl Pts',(-8.32255751407984,-12.5442482545536,
118.303275492847)) ;
#156254=CARTESIAN_POINT('Ctrl Pts',(-8.24875365766935,-12.5442482922109,
118.327506494966)) ;
#156255=CARTESIAN_POINT('Ctrl Pts',(-8.17494980125887,-12.5442483298683,
118.351737497085)) ;
#156256=CARTESIAN_POINT('Ctrl Pts',(-8.19068066224925,-12.6009816910039,
118.399651162582)) ;
#156257=CARTESIAN_POINT('Ctrl Pts',(-8.27663038654765,-12.4399155910324,
118.626049746092)) ;
#156258=CARTESIAN_POINT('Ctrl Pts',(-8.28711539330814,-12.5079761461326,
118.657985386172)) ;
#156259=CARTESIAN_POINT('Ctrl Pts',(-8.36091925456453,-12.5079761174331,
118.633754398813)) ;
#156260=CARTESIAN_POINT('Ctrl Pts',(-8.43472311582091,-12.5079760887335,
118.609523411454)) ;
#156261=CARTESIAN_POINT('Ctrl Pts',(-8.42423810906042,-12.4399155336333,
118.577587771374)) ;
#156262=CARTESIAN_POINT('Ctrl Pts',(-8.41375310229993,-12.3718549785331,
118.545652131295)) ;
#156263=CARTESIAN_POINT('Ctrl Pts',(-8.33994924104354,-12.3718550072327,
118.569883118654)) ;
#156264=CARTESIAN_POINT('Ctrl Pts',(-8.26614537978715,-12.3718550359322,
118.594114106013)) ;
#156265=CARTESIAN_POINT('Ctrl Pts',(-8.27663038654765,-12.4399155910324,
118.626049746092)) ;
#156266=CARTESIAN_POINT('Ctrl Pts',(-8.37377653671491,-12.3483508718252,
118.886335164228)) ;
#156267=CARTESIAN_POINT('Ctrl Pts',(-8.3782310343859,-12.4229031690547,
118.899902846821)) ;
#156268=CARTESIAN_POINT('Ctrl Pts',(-8.45203490024531,-12.4229031549688,
118.875671873482)) ;
#156269=CARTESIAN_POINT('Ctrl Pts',(-8.52583876610469,-12.4229031408829,
118.851440900143)) ;
#156270=CARTESIAN_POINT('Ctrl Pts',(-8.5213842684337,-12.3483508436534,
118.83787321755)) ;
#156271=CARTESIAN_POINT('Ctrl Pts',(-8.51692977076269,-12.2737985464239,
118.824305534957)) ;
#156272=CARTESIAN_POINT('Ctrl Pts',(-8.4431259049033,-12.2737985605098,
118.848536508296)) ;
#156273=CARTESIAN_POINT('Ctrl Pts',(-8.3693220390439,-12.2737985745957,
118.872767481635)) ;
#156274=CARTESIAN_POINT('Ctrl Pts',(-8.37377653671491,-12.3483508718252,
118.886335164228)) ;
#156275=CARTESIAN_POINT('Ctrl Pts',(-8.47470424960895,-12.3338872424077,
119.158388022071)) ;
#156276=CARTESIAN_POINT('Ctrl Pts',(-8.47285027545596,-12.4095571114995,
119.152741117483)) ;
#156277=CARTESIAN_POINT('Ctrl Pts',(-8.54665414372756,-12.4095571176329,
119.128510151491)) ;
#156278=CARTESIAN_POINT('Ctrl Pts',(-8.62045801199916,-12.4095571237664,
119.1042791855)) ;
#156279=CARTESIAN_POINT('Ctrl Pts',(-8.62231198615215,-12.3338872546745,
119.109926090087)) ;
#156280=CARTESIAN_POINT('Ctrl Pts',(-8.62416596030512,-12.2582173855827,
119.115572994675)) ;
#156281=CARTESIAN_POINT('Ctrl Pts',(-8.55036209203353,-12.2582173794493,
119.139803960667)) ;
#156282=CARTESIAN_POINT('Ctrl Pts',(-8.47655822376192,-12.2582173733159,
119.164034926658)) ;
#156283=CARTESIAN_POINT('Ctrl Pts',(-8.47470424960895,-12.3338872424077,
119.158388022071)) ;
#156284=CARTESIAN_POINT('Ctrl Pts',(-8.5740859453798,-12.396923495094,119.425556245681)) ;
#156285=CARTESIAN_POINT('Ctrl Pts',(-8.5660260133282,-12.4683025104667,
119.401006994805)) ;
#156286=CARTESIAN_POINT('Ctrl Pts',(-8.63982988237598,-12.4683025400751,
119.376776031178)) ;
#156287=CARTESIAN_POINT('Ctrl Pts',(-8.71363375142374,-12.4683025696834,
119.35254506755)) ;
#156288=CARTESIAN_POINT('Ctrl Pts',(-8.72169368347534,-12.3969235543106,
119.377094318426)) ;
#156289=CARTESIAN_POINT('Ctrl Pts',(-8.72975361552693,-12.3255445389379,
119.401643569301)) ;
#156290=CARTESIAN_POINT('Ctrl Pts',(-8.65594974647916,-12.3255445093296,
119.425874532929)) ;
#156291=CARTESIAN_POINT('Ctrl Pts',(-8.58214587743139,-12.3255444797213,
119.450105496557)) ;
#156292=CARTESIAN_POINT('Ctrl Pts',(-8.5740859453798,-12.396923495094,119.425556245681)) ;
#156293=CARTESIAN_POINT('Ctrl Pts',(-8.6649277864638,-12.5334553693914,
119.666748762957)) ;
#156294=CARTESIAN_POINT('Ctrl Pts',(-8.65124833264428,-12.595406254364,
119.625083355602)) ;
#156295=CARTESIAN_POINT('Ctrl Pts',(-8.72505219984459,-12.5954063084814,
119.600852386347)) ;
#156296=CARTESIAN_POINT('Ctrl Pts',(-8.79885606704489,-12.5954063625988,
119.576621417092)) ;
#156297=CARTESIAN_POINT('Ctrl Pts',(-8.81253552086441,-12.5334554776262,
119.618286824447)) ;
#156298=CARTESIAN_POINT('Ctrl Pts',(-8.82621497468392,-12.4715045926535,
119.659952231802)) ;
#156299=CARTESIAN_POINT('Ctrl Pts',(-8.75241110748362,-12.4715045385361,
119.684183201057)) ;
#156300=CARTESIAN_POINT('Ctrl Pts',(-8.67860724028331,-12.4715044844187,
119.708414170312)) ;
#156301=CARTESIAN_POINT('Ctrl Pts',(-8.6649277864638,-12.5334553693914,
119.666748762957)) ;
#156302=CARTESIAN_POINT('Ctrl Pts',(-8.74128429943828,-12.7322215761211,
119.863992617795)) ;
#156303=CARTESIAN_POINT('Ctrl Pts',(-8.72298495132889,-12.7803853400704,
119.808255757934)) ;
#156304=CARTESIAN_POINT('Ctrl Pts',(-8.7967888140635,-12.7803854158274,
119.784024775078)) ;
#156305=CARTESIAN_POINT('Ctrl Pts',(-8.8705926767981,-12.7803854915845,
119.759793792221)) ;
#156306=CARTESIAN_POINT('Ctrl Pts',(-8.88889202490748,-12.7322217276352,
119.815530652082)) ;
#156307=CARTESIAN_POINT('Ctrl Pts',(-8.90719137301686,-12.6840579636859,
119.871267511943)) ;
#156308=CARTESIAN_POINT('Ctrl Pts',(-8.83338751028226,-12.6840578879289,
119.895498494799)) ;
#156309=CARTESIAN_POINT('Ctrl Pts',(-8.75958364754765,-12.6840578121718,
119.919729477656)) ;
#156310=CARTESIAN_POINT('Ctrl Pts',(-8.74128429943828,-12.7322215761211,
119.863992617795)) ;
#156311=CARTESIAN_POINT('Ctrl Pts',(-8.79916573819104,-12.9810049412899,
120.004790749052)) ;
#156312=CARTESIAN_POINT('Ctrl Pts',(-8.77753307281271,-13.0118702151138,
119.938901142704)) ;
#156313=CARTESIAN_POINT('Ctrl Pts',(-8.85133692912627,-13.0118703086727,
119.91467014029)) ;
#156314=CARTESIAN_POINT('Ctrl Pts',(-8.92514078543982,-13.0118704022315,
119.890439137876)) ;
#156315=CARTESIAN_POINT('Ctrl Pts',(-8.94677345081817,-12.9810051284076,
119.956328744224)) ;
#156316=CARTESIAN_POINT('Ctrl Pts',(-8.96840611619649,-12.9501398545836,
120.022218350571)) ;
#156317=CARTESIAN_POINT('Ctrl Pts',(-8.89460225988293,-12.9501397610248,
120.046449352985)) ;
#156318=CARTESIAN_POINT('Ctrl Pts',(-8.82079840356937,-12.9501396674659,
120.070680355399)) ;
#156319=CARTESIAN_POINT('Ctrl Pts',(-8.79916573819104,-12.9810049412899,
120.004790749052)) ;
#156320=CARTESIAN_POINT('Ctrl Pts',(-8.83469320205863,-13.2609753303157,
120.077533333241)) ;
#156321=CARTESIAN_POINT('Ctrl Pts',(-8.81128227802888,-13.2723394892272,
120.006227438023)) ;
#156322=CARTESIAN_POINT('Ctrl Pts',(-8.88508612624132,-13.2723395935458,
119.981996410934)) ;
#156323=CARTESIAN_POINT('Ctrl Pts',(-8.95888997445376,-13.2723396978644,
119.957765383845)) ;
#156324=CARTESIAN_POINT('Ctrl Pts',(-8.9823008984835,-13.260975538953,120.029071279063)) ;
#156325=CARTESIAN_POINT('Ctrl Pts',(-9.00571182251326,-13.2496113800415,
120.100377174282)) ;
#156326=CARTESIAN_POINT('Ctrl Pts',(-8.93190797430082,-13.2496112757229,
120.12460820137)) ;
#156327=CARTESIAN_POINT('Ctrl Pts',(-8.85810412608837,-13.2496111714043,
120.148839228459)) ;
#156328=CARTESIAN_POINT('Ctrl Pts',(-8.83469320205863,-13.2609753303157,
120.077533333241)) ;
#156329=CARTESIAN_POINT('Ctrl Pts',(-8.84616539838749,-13.5522070361543,
120.07700191012)) ;
#156330=CARTESIAN_POINT('Ctrl Pts',(-8.82265305360655,-13.5432552863656,
120.005387103697)) ;
#156331=CARTESIAN_POINT('Ctrl Pts',(-8.89645689290648,-13.5432553930549,
119.981156049463)) ;
#156332=CARTESIAN_POINT('Ctrl Pts',(-8.97026073220642,-13.5432554997441,
119.956924995228)) ;
#156333=CARTESIAN_POINT('Ctrl Pts',(-8.99377307698736,-13.5522072495328,
120.02853980165)) ;
#156334=CARTESIAN_POINT('Ctrl Pts',(-9.0172854217683,-13.5611589993214,
120.100154608073)) ;
#156335=CARTESIAN_POINT('Ctrl Pts',(-8.94348158246836,-13.5611588926322,
120.124385662307)) ;
#156336=CARTESIAN_POINT('Ctrl Pts',(-8.86967774316843,-13.5611587859429,
120.148616716542)) ;
#156337=CARTESIAN_POINT('Ctrl Pts',(-8.84616539838749,-13.5522070361543,
120.07700191012)) ;
#156338=CARTESIAN_POINT('Ctrl Pts',(-8.83352879857719,-13.8335794690488,
120.003072712917)) ;
#156339=CARTESIAN_POINT('Ctrl Pts',(-8.81159729377728,-13.8049701426201,
119.936272890026)) ;
#156340=CARTESIAN_POINT('Ctrl Pts',(-8.88540112426656,-13.8049702427903,
119.912041808956)) ;
#156341=CARTESIAN_POINT('Ctrl Pts',(-8.95920495475583,-13.8049703429605,
119.887810727885)) ;
#156342=CARTESIAN_POINT('Ctrl Pts',(-8.98113645955575,-13.8335796693892,
119.954610550776)) ;
#156343=CARTESIAN_POINT('Ctrl Pts',(-9.00306796435566,-13.862188995818,
120.021410373666)) ;
#156344=CARTESIAN_POINT('Ctrl Pts',(-8.92926413386639,-13.8621888956478,
120.045641454737)) ;
#156345=CARTESIAN_POINT('Ctrl Pts',(-8.8554603033771,-13.8621887954776,
120.069872535807)) ;
#156346=CARTESIAN_POINT('Ctrl Pts',(-8.83352879857719,-13.8335794690488,
120.003072712917)) ;
#156347=CARTESIAN_POINT('Ctrl Pts',(-8.79840525558534,-14.0854850074698,
119.86061077159)) ;
#156348=CARTESIAN_POINT('Ctrl Pts',(-8.77962758865732,-14.0392461681425,
119.803417029983)) ;
#156349=CARTESIAN_POINT('Ctrl Pts',(-8.85343141133836,-14.0392462534928,
119.77918592513)) ;
#156350=CARTESIAN_POINT('Ctrl Pts',(-8.92723523401938,-14.039246338843,
119.754954820277)) ;
#156351=CARTESIAN_POINT('Ctrl Pts',(-8.94601290094739,-14.0854851781703,
119.812148561884)) ;
#156352=CARTESIAN_POINT('Ctrl Pts',(-8.96479056787539,-14.1317240174977,
119.869342303491)) ;
#156353=CARTESIAN_POINT('Ctrl Pts',(-8.89098674519436,-14.1317239321474,
119.893573408344)) ;
#156354=CARTESIAN_POINT('Ctrl Pts',(-8.81718292251333,-14.1317238467972,
119.917804513197)) ;
#156355=CARTESIAN_POINT('Ctrl Pts',(-8.79840525558534,-14.0854850074698,
119.86061077159)) ;
#156356=CARTESIAN_POINT('Ctrl Pts',(-8.74411665331808,-14.2893882283517,
119.659805611785)) ;
#156357=CARTESIAN_POINT('Ctrl Pts',(-8.72983485738257,-14.2288448467623,
119.616305567789)) ;
#156358=CARTESIAN_POINT('Ctrl Pts',(-8.80363867406561,-14.2288449105474,
119.592074444667)) ;
#156359=CARTESIAN_POINT('Ctrl Pts',(-8.87744249074863,-14.2288449743324,
119.567843321545)) ;
#156360=CARTESIAN_POINT('Ctrl Pts',(-8.89172428668414,-14.2893883559219,
119.611343365541)) ;
#156361=CARTESIAN_POINT('Ctrl Pts',(-8.90600608261964,-14.3499317375113,
119.654843409537)) ;
#156362=CARTESIAN_POINT('Ctrl Pts',(-8.83220226593662,-14.3499316737262,
119.679074532659)) ;
#156363=CARTESIAN_POINT('Ctrl Pts',(-8.75839844925359,-14.3499316099411,
119.703305655781)) ;
#156364=CARTESIAN_POINT('Ctrl Pts',(-8.74411665331808,-14.2893882283517,
119.659805611785)) ;
#156365=CARTESIAN_POINT('Ctrl Pts',(-8.67521497823715,-14.4310416708449,
119.414456500244)) ;
#156366=CARTESIAN_POINT('Ctrl Pts',(-8.66645661513697,-14.3605181681089,
119.387779941412)) ;
#156367=CARTESIAN_POINT('Ctrl Pts',(-8.74026042822641,-14.3605182058442,
119.363548807345)) ;
#156368=CARTESIAN_POINT('Ctrl Pts',(-8.81406424131583,-14.3605182435796,
119.339317673277)) ;
#156369=CARTESIAN_POINT('Ctrl Pts',(-8.82282260441602,-14.4310417463156,
119.365994232109)) ;
#156370=CARTESIAN_POINT('Ctrl Pts',(-8.83158096751619,-14.5015652490516,
119.39267079094)) ;
#156371=CARTESIAN_POINT('Ctrl Pts',(-8.75777715442677,-14.5015652113162,
119.416901925008)) ;
#156372=CARTESIAN_POINT('Ctrl Pts',(-8.68397334133732,-14.5015651735809,
119.441133059075)) ;
#156373=CARTESIAN_POINT('Ctrl Pts',(-8.67521497823715,-14.4310416708449,
119.414456500244)) ;
#156374=CARTESIAN_POINT('Ctrl Pts',(-8.59746348536126,-14.4999960091202,
119.142167399687)) ;
#156375=CARTESIAN_POINT('Ctrl Pts',(-8.5948543547224,-14.4245527843061,
119.134220410688)) ;
#156376=CARTESIAN_POINT('Ctrl Pts',(-8.66865816690361,-14.4245527944394,
119.109989273854)) ;
#156377=CARTESIAN_POINT('Ctrl Pts',(-8.74246197908482,-14.4245528045727,
119.08575813702)) ;
#156378=CARTESIAN_POINT('Ctrl Pts',(-8.74507110972368,-14.4999960293868,
119.093705126019)) ;
#156379=CARTESIAN_POINT('Ctrl Pts',(-8.74768024036255,-14.5754392542009,
119.101652115019)) ;
#156380=CARTESIAN_POINT('Ctrl Pts',(-8.67387642818134,-14.5754392440676,
119.125883251853)) ;
#156381=CARTESIAN_POINT('Ctrl Pts',(-8.60007261600012,-14.5754392339344,
119.150114388687)) ;
#156382=CARTESIAN_POINT('Ctrl Pts',(-8.59746348536126,-14.4999960091202,
119.142167399687)) ;
#156383=CARTESIAN_POINT('Ctrl Pts',(-8.51725220866625,-14.4914668725251,
118.862420893709)) ;
#156384=CARTESIAN_POINT('Ctrl Pts',(-8.52097256831155,-14.4165060453907,
118.873752510769)) ;
#156385=CARTESIAN_POINT('Ctrl Pts',(-8.59477638215005,-14.4165060293028,
118.849521378983)) ;
#156386=CARTESIAN_POINT('Ctrl Pts',(-8.66858019598853,-14.416506013215,
118.825290247197)) ;
#156387=CARTESIAN_POINT('Ctrl Pts',(-8.66485983634323,-14.4914668403494,
118.813958630137)) ;
#156388=CARTESIAN_POINT('Ctrl Pts',(-8.6611394766979,-14.5664276674838,
118.802627013077)) ;
#156389=CARTESIAN_POINT('Ctrl Pts',(-8.58733566285942,-14.5664276835716,
118.826858144863)) ;
#156390=CARTESIAN_POINT('Ctrl Pts',(-8.51353184902093,-14.5664276996595,
118.851089276649)) ;
#156391=CARTESIAN_POINT('Ctrl Pts',(-8.51725220866625,-14.4914668725251,
118.862420893709)) ;
#156392=CARTESIAN_POINT('Ctrl Pts',(-8.44094453814601,-14.4062237339893,
118.594550823069)) ;
#156393=CARTESIAN_POINT('Ctrl Pts',(-8.45073164518584,-14.3371017134928,
118.624360773722)) ;
#156394=CARTESIAN_POINT('Ctrl Pts',(-8.52453546296583,-14.337101674971,
118.600129653941)) ;
#156395=CARTESIAN_POINT('Ctrl Pts',(-8.59833928074581,-14.3371016364492,
118.57589853416)) ;
#156396=CARTESIAN_POINT('Ctrl Pts',(-8.58855217370597,-14.4062236569457,
118.546088583507)) ;
#156397=CARTESIAN_POINT('Ctrl Pts',(-8.57876506666614,-14.4753456774423,
118.516278632854)) ;
#156398=CARTESIAN_POINT('Ctrl Pts',(-8.50496124888616,-14.4753457159641,
118.540509752635)) ;
#156399=CARTESIAN_POINT('Ctrl Pts',(-8.43115743110617,-14.4753457544858,
118.564740872416)) ;
#156400=CARTESIAN_POINT('Ctrl Pts',(-8.44094453814601,-14.4062237339893,
118.594550823069)) ;
#156401=CARTESIAN_POINT('Ctrl Pts',(-8.37461958404781,-14.2495321967945,
118.356968882225)) ;
#156402=CARTESIAN_POINT('Ctrl Pts',(-8.38978814218742,-14.1912456004984,
118.403169864494)) ;
#156403=CARTESIAN_POINT('Ctrl Pts',(-8.46359196581185,-14.1912455461204,
118.378938762515)) ;
#156404=CARTESIAN_POINT('Ctrl Pts',(-8.53739578943627,-14.1912454917425,
118.354707660535)) ;
#156405=CARTESIAN_POINT('Ctrl Pts',(-8.52222723129668,-14.2495320880387,
118.308506678265)) ;
#156406=CARTESIAN_POINT('Ctrl Pts',(-8.50705867315707,-14.3078186843349,
118.262305695995)) ;
#156407=CARTESIAN_POINT('Ctrl Pts',(-8.43325484953264,-14.3078187387128,
118.286536797975)) ;
#156408=CARTESIAN_POINT('Ctrl Pts',(-8.3594510259082,-14.3078187930907,
118.310767899955)) ;
#156409=CARTESIAN_POINT('Ctrl Pts',(-8.37461958404781,-14.2495321967945,
118.356968882225)) ;
#156410=CARTESIAN_POINT('Ctrl Pts',(-8.32425634296907,-14.0340281298451,
118.168167653125)) ;
#156411=CARTESIAN_POINT('Ctrl Pts',(-8.34369668060544,-13.990699945468,
118.227379786363)) ;
#156412=CARTESIAN_POINT('Ctrl Pts',(-8.41750051062051,-13.9906998817967,
118.203148703848)) ;
#156413=CARTESIAN_POINT('Ctrl Pts',(-8.49130434063558,-13.9906998181254,
118.178917621333)) ;
#156414=CARTESIAN_POINT('Ctrl Pts',(-8.47186400299921,-14.0340280025025,
118.119705488095)) ;
#156415=CARTESIAN_POINT('Ctrl Pts',(-8.45242366536283,-14.0773561868796,
118.060493354857)) ;
#156416=CARTESIAN_POINT('Ctrl Pts',(-8.37861983534776,-14.0773562505509,
118.084724437372)) ;
#156417=CARTESIAN_POINT('Ctrl Pts',(-8.30481600533269,-14.0773563142222,
118.108955519887)) ;
#156418=CARTESIAN_POINT('Ctrl Pts',(-8.32425634296907,-14.0340281298451,
118.168167653125)) ;
#156419=CARTESIAN_POINT('Ctrl Pts',(-8.29382206288613,-13.7742259092907,
118.040014681808)) ;
#156420=CARTESIAN_POINT('Ctrl Pts',(-8.31615037608938,-13.7489714833696,
118.108023122501)) ;
#156421=CARTESIAN_POINT('Ctrl Pts',(-8.38995421264838,-13.7489714178304,
118.083792059918)) ;
#156422=CARTESIAN_POINT('Ctrl Pts',(-8.46375804920739,-13.7489713522911,
118.059560997334)) ;
#156423=CARTESIAN_POINT('Ctrl Pts',(-8.44142973600415,-13.7742257782122,
117.991552556642)) ;
#156424=CARTESIAN_POINT('Ctrl Pts',(-8.4191014228009,-13.7994802041333,
117.923544115949)) ;
#156425=CARTESIAN_POINT('Ctrl Pts',(-8.34529758624189,-13.7994802696726,
117.947775178532)) ;
#156426=CARTESIAN_POINT('Ctrl Pts',(-8.27149374968289,-13.7994803352118,
117.972006241116)) ;
#156427=CARTESIAN_POINT('Ctrl Pts',(-8.29382206288613,-13.7742259092907,
118.040014681808)) ;
#156428=CARTESIAN_POINT('Ctrl Pts',(-8.28631480334285,-13.488993839479,
117.981708548653)) ;
#156429=CARTESIAN_POINT('Ctrl Pts',(-8.30993444408831,-13.4836161224244,
118.053650164529)) ;
#156430=CARTESIAN_POINT('Ctrl Pts',(-8.38373828651983,-13.4836160614426,
118.029419119833)) ;
#156431=CARTESIAN_POINT('Ctrl Pts',(-8.45754212895135,-13.4836160004609,
118.005188075136)) ;
#156432=CARTESIAN_POINT('Ctrl Pts',(-8.43392248820588,-13.4889937175154,
117.93324645926)) ;
#156433=CARTESIAN_POINT('Ctrl Pts',(-8.41030284746041,-13.49437143457,117.861304843384)) ;
#156434=CARTESIAN_POINT('Ctrl Pts',(-8.33649900502889,-13.4943714955518,
117.885535888081)) ;
#156435=CARTESIAN_POINT('Ctrl Pts',(-8.26269516259738,-13.4943715565336,
117.909766932777)) ;
#156436=CARTESIAN_POINT('Ctrl Pts',(-8.28631480334285,-13.488993839479,
117.981708548653)) ;
#156437=CARTESIAN_POINT('Ctrl Pts',(-8.30320195637338,-13.1975717487405,
117.997560479062)) ;
#156438=CARTESIAN_POINT('Ctrl Pts',(-8.32641478554093,-13.2125333094721,
118.068263012322)) ;
#156439=CARTESIAN_POINT('Ctrl Pts',(-8.40021863242881,-13.2125332593627,
118.044031981199)) ;
#156440=CARTESIAN_POINT('Ctrl Pts',(-8.4740224793167,-13.2125332092533,
118.019800950075)) ;
#156441=CARTESIAN_POINT('Ctrl Pts',(-8.45080965014914,-13.1975716485217,
117.949098416815)) ;
#156442=CARTESIAN_POINT('Ctrl Pts',(-8.42759682098158,-13.1826100877902,
117.878395883556)) ;
#156443=CARTESIAN_POINT('Ctrl Pts',(-8.35379297409371,-13.1826101378995,
117.902626914679)) ;
#156444=CARTESIAN_POINT('Ctrl Pts',(-8.27998912720583,-13.1826101880089,
117.926857945802)) ;
#156445=CARTESIAN_POINT('Ctrl Pts',(-8.30320195637338,-13.1975717487405,
117.997560479062)) ;
#156446=CARTESIAN_POINT('Ctrl Pts',(-8.3436703131233,-12.9237175982201,
118.085475777875)) ;
#156447=CARTESIAN_POINT('Ctrl Pts',(-8.36482407973362,-12.9578227208983,
118.149906738669)) ;
#156448=CARTESIAN_POINT('Ctrl Pts',(-8.43862792956874,-12.9578226823066,
118.125675716522)) ;
#156449=CARTESIAN_POINT('Ctrl Pts',(-8.51243177940384,-12.9578226437149,
118.101444694376)) ;
#156450=CARTESIAN_POINT('Ctrl Pts',(-8.49127801279351,-12.9237175210368,
118.037013733583)) ;
#156451=CARTESIAN_POINT('Ctrl Pts',(-8.47012424618317,-12.8896123983586,
117.972582772789)) ;
#156452=CARTESIAN_POINT('Ctrl Pts',(-8.39632039634807,-12.8896124369503,
117.996813794936)) ;
#156453=CARTESIAN_POINT('Ctrl Pts',(-8.32251654651295,-12.889612475542,
118.021044817082)) ;
#156454=CARTESIAN_POINT('Ctrl Pts',(-8.3436703131233,-12.9237175982201,
118.085475777875)) ;
#156455=CARTESIAN_POINT('Ctrl Pts',(-8.4062239104521,-12.6833926232874,
118.240377888327)) ;
#156456=CARTESIAN_POINT('Ctrl Pts',(-8.4237794536085,-12.7343299181759,
118.293849240853)) ;
#156457=CARTESIAN_POINT('Ctrl Pts',(-8.49758330427195,-12.7343298939571,
118.26961822123)) ;
#156458=CARTESIAN_POINT('Ctrl Pts',(-8.57138715493539,-12.7343298697383,
118.245387201606)) ;
#156459=CARTESIAN_POINT('Ctrl Pts',(-8.553831611779,-12.6833925748499,118.19191584908)) ;
#156460=CARTESIAN_POINT('Ctrl Pts',(-8.5362760686226,-12.6324552799614,
118.138444496554)) ;
#156461=CARTESIAN_POINT('Ctrl Pts',(-8.46247221795915,-12.6324553041802,
118.162675516177)) ;
#156462=CARTESIAN_POINT('Ctrl Pts',(-8.38866836729569,-12.632455328399,
118.186906535801)) ;
#156463=CARTESIAN_POINT('Ctrl Pts',(-8.4062239104521,-12.6833926232874,
118.240377888327)) ;
#156464=CARTESIAN_POINT('Ctrl Pts',(-8.48615190099208,-12.4975233316372,
118.448503252107)) ;
#156465=CARTESIAN_POINT('Ctrl Pts',(-8.4988840715495,-12.5615155230103,
118.48728338981)) ;
#156466=CARTESIAN_POINT('Ctrl Pts',(-8.57268792207089,-12.5615155094136,
118.463052369754)) ;
#156467=CARTESIAN_POINT('Ctrl Pts',(-8.64649177259229,-12.561515495817,
118.438821349698)) ;
#156468=CARTESIAN_POINT('Ctrl Pts',(-8.63375960203489,-12.4975233044439,
118.400041211994)) ;
#156469=CARTESIAN_POINT('Ctrl Pts',(-8.62102743147748,-12.4335311130708,
118.361261074291)) ;
#156470=CARTESIAN_POINT('Ctrl Pts',(-8.54722358095607,-12.4335311266674,
118.385492094347)) ;
#156471=CARTESIAN_POINT('Ctrl Pts',(-8.47341973043468,-12.433531140264,
118.409723114404)) ;
#156472=CARTESIAN_POINT('Ctrl Pts',(-8.48615190099208,-12.4975233316372,
118.448503252107)) ;
#156473=CARTESIAN_POINT('Ctrl Pts',(-8.57934667074232,-12.3765652756753,
118.696871045336)) ;
#156474=CARTESIAN_POINT('Ctrl Pts',(-8.58632526391847,-12.4491001941253,
118.718126714516)) ;
#156475=CARTESIAN_POINT('Ctrl Pts',(-8.66012911291596,-12.44910018943,118.693895689818)) ;
#156476=CARTESIAN_POINT('Ctrl Pts',(-8.73393296191344,-12.4491001847347,
118.66966466512)) ;
#156477=CARTESIAN_POINT('Ctrl Pts',(-8.72695436873729,-12.3765652662847,
118.64840899594)) ;
#156478=CARTESIAN_POINT('Ctrl Pts',(-8.71997577556115,-12.3040303478347,
118.62715332676)) ;
#156479=CARTESIAN_POINT('Ctrl Pts',(-8.64617192656366,-12.30403035253,118.651384351458)) ;
#156480=CARTESIAN_POINT('Ctrl Pts',(-8.57236807756618,-12.3040303572253,
118.675615376155)) ;
#156481=CARTESIAN_POINT('Ctrl Pts',(-8.57934667074232,-12.3765652756753,
118.696871045336)) ;
#156482=CARTESIAN_POINT('Ctrl Pts',(-8.67942447659642,-12.3303669115662,
118.966269185261)) ;
#156483=CARTESIAN_POINT('Ctrl Pts',(-8.68015871203297,-12.4062370893219,
118.968505548159)) ;
#156484=CARTESIAN_POINT('Ctrl Pts',(-8.75396255910231,-12.4062370896233,
118.944274517589)) ;
#156485=CARTESIAN_POINT('Ctrl Pts',(-8.82776640617164,-12.4062370899248,
118.920043487018)) ;
#156486=CARTESIAN_POINT('Ctrl Pts',(-8.82703217073509,-12.3303669121692,
118.91780712412)) ;
#156487=CARTESIAN_POINT('Ctrl Pts',(-8.82629793529853,-12.2544967344135,
118.915570761222)) ;
#156488=CARTESIAN_POINT('Ctrl Pts',(-8.7524940882292,-12.2544967341121,
118.939801791793)) ;
#156489=CARTESIAN_POINT('Ctrl Pts',(-8.67869024115987,-12.2544967338106,
118.964032822363)) ;
#156490=CARTESIAN_POINT('Ctrl Pts',(-8.67942447659642,-12.3303669115662,
118.966269185261)) ;
#156491=CARTESIAN_POINT('Ctrl Pts',(-8.78046560292115,-12.3620831181533,
119.23847587387)) ;
#156492=CARTESIAN_POINT('Ctrl Pts',(-8.77488124433053,-12.4358532268962,
119.221466818734)) ;
#156493=CARTESIAN_POINT('Ctrl Pts',(-8.84868508924219,-12.4358532286459,
119.197235781592)) ;
#156494=CARTESIAN_POINT('Ctrl Pts',(-8.92248893415383,-12.4358532303956,
119.173004744449)) ;
#156495=CARTESIAN_POINT('Ctrl Pts',(-8.92807329274446,-12.3620831216526,
119.190013799585)) ;
#156496=CARTESIAN_POINT('Ctrl Pts',(-8.93365765133506,-12.2883130129096,
119.20702285472)) ;
#156497=CARTESIAN_POINT('Ctrl Pts',(-8.85985380642342,-12.28831301116,119.231253891863)) ;
#156498=CARTESIAN_POINT('Ctrl Pts',(-8.78604996151176,-12.2883130094103,
119.255484929005)) ;
#156499=CARTESIAN_POINT('Ctrl Pts',(-8.78046560292115,-12.3620831181533,
119.23847587387)) ;
#156500=CARTESIAN_POINT('Ctrl Pts',(-8.87549407917763,-12.4697592102098,
119.49241363428)) ;
#156501=CARTESIAN_POINT('Ctrl Pts',(-8.86400045518284,-12.536121336536,
119.457405910088)) ;
#156502=CARTESIAN_POINT('Ctrl Pts',(-8.93780429864287,-12.5361213369903,
119.433174868524)) ;
#156503=CARTESIAN_POINT('Ctrl Pts',(-9.0116081421029,-12.5361213374447,
119.40894382696)) ;
#156504=CARTESIAN_POINT('Ctrl Pts',(-9.02310176609769,-12.4697592111185,
119.443951551152)) ;
#156505=CARTESIAN_POINT('Ctrl Pts',(-9.03459539009248,-12.4033970847922,
119.478959275343)) ;
#156506=CARTESIAN_POINT('Ctrl Pts',(-8.96079154663245,-12.4033970843379,
119.503190316907)) ;
#156507=CARTESIAN_POINT('Ctrl Pts',(-8.88698770317242,-12.4033970838835,
119.527421358471)) ;
#156508=CARTESIAN_POINT('Ctrl Pts',(-8.87549407917763,-12.4697592102098,
119.49241363428)) ;
#156509=CARTESIAN_POINT('Ctrl Pts',(-8.95832054343873,-12.6447797711106,
119.709301795168)) ;
#156510=CARTESIAN_POINT('Ctrl Pts',(-8.94175857502336,-12.6990195583039,
119.658856711595)) ;
#156511=CARTESIAN_POINT('Ctrl Pts',(-9.0155624178882,-12.69901955683,119.634625668218)) ;
#156512=CARTESIAN_POINT('Ctrl Pts',(-9.08936626075305,-12.6990195553562,
119.610394624842)) ;
#156513=CARTESIAN_POINT('Ctrl Pts',(-9.10592822916841,-12.6447797681629,
119.660839708415)) ;
#156514=CARTESIAN_POINT('Ctrl Pts',(-9.1224901975838,-12.5905399809696,
119.711284791988)) ;
#156515=CARTESIAN_POINT('Ctrl Pts',(-9.04868635471895,-12.5905399824434,
119.735515835365)) ;
#156516=CARTESIAN_POINT('Ctrl Pts',(-8.97488251185411,-12.5905399839173,
119.759746878742)) ;
#156517=CARTESIAN_POINT('Ctrl Pts',(-8.95832054343873,-12.6447797711106,
119.709301795168)) ;
#156518=CARTESIAN_POINT('Ctrl Pts',(-9.02420754409074,-12.8750273852739,
119.874571217192)) ;
#156519=CARTESIAN_POINT('Ctrl Pts',(-9.00375303558084,-12.9132697898462,
119.812270084526)) ;
#156520=CARTESIAN_POINT('Ctrl Pts',(-9.0775568784528,-12.9132697868245,
119.788039041171)) ;
#156521=CARTESIAN_POINT('Ctrl Pts',(-9.15136072132475,-12.9132697838028,
119.763807997816)) ;
#156522=CARTESIAN_POINT('Ctrl Pts',(-9.17181522983464,-12.8750273792305,
119.826109130482)) ;
#156523=CARTESIAN_POINT('Ctrl Pts',(-9.19226973834453,-12.8367849746583,
119.888410263147)) ;
#156524=CARTESIAN_POINT('Ctrl Pts',(-9.11846589547259,-12.8367849776799,
119.912641306503)) ;
#156525=CARTESIAN_POINT('Ctrl Pts',(-9.04466205260062,-12.8367849807016,
119.936872349858)) ;
#156526=CARTESIAN_POINT('Ctrl Pts',(-9.02420754409074,-12.8750273852739,
119.874571217192)) ;
#156527=CARTESIAN_POINT('Ctrl Pts',(-9.06917668282671,-13.1453257818208,
119.975977828757)) ;
#156528=CARTESIAN_POINT('Ctrl Pts',(-9.04628767891136,-13.1647498113274,
119.906261615918)) ;
#156529=CARTESIAN_POINT('Ctrl Pts',(-9.12009152221,-13.1647498092517,119.882030573863)) ;
#156530=CARTESIAN_POINT('Ctrl Pts',(-9.19389536550866,-13.164749807176,
119.857799531807)) ;
#156531=CARTESIAN_POINT('Ctrl Pts',(-9.21678436942402,-13.1453257776693,
119.927515744647)) ;
#156532=CARTESIAN_POINT('Ctrl Pts',(-9.23967337333938,-13.1259017481627,
119.997231957486)) ;
#156533=CARTESIAN_POINT('Ctrl Pts',(-9.16586953004072,-13.1259017502384,
120.021462999541)) ;
#156534=CARTESIAN_POINT('Ctrl Pts',(-9.09206568674207,-13.1259017523141,
120.045694041597)) ;
#156535=CARTESIAN_POINT('Ctrl Pts',(-9.06917668282671,-13.1453257818208,
119.975977828757)) ;
#156536=CARTESIAN_POINT('Ctrl Pts',(-9.09047067571145,-13.4336234546741,
120.005474883971)) ;
#156537=CARTESIAN_POINT('Ctrl Pts',(-9.06679306728316,-13.4329452228824,
119.933356709079)) ;
#156538=CARTESIAN_POINT('Ctrl Pts',(-9.14059691081299,-13.4329452235498,
119.909125667728)) ;
#156539=CARTESIAN_POINT('Ctrl Pts',(-9.21440075434283,-13.4329452242172,
119.884894626377)) ;
#156540=CARTESIAN_POINT('Ctrl Pts',(-9.23807836277112,-13.433623456009,
119.957012801268)) ;
#156541=CARTESIAN_POINT('Ctrl Pts',(-9.2617559711994,-13.4343016878008,
120.02913097616)) ;
#156542=CARTESIAN_POINT('Ctrl Pts',(-9.18795212766956,-13.4343016871333,
120.053362017511)) ;
#156543=CARTESIAN_POINT('Ctrl Pts',(-9.11414828413973,-13.4343016864659,
120.077593058863)) ;
#156544=CARTESIAN_POINT('Ctrl Pts',(-9.09047067571145,-13.4336234546741,
120.005474883971)) ;
#156545=CARTESIAN_POINT('Ctrl Pts',(-9.08746787607695,-13.7229316022969,
119.960694301127)) ;
#156546=CARTESIAN_POINT('Ctrl Pts',(-9.06470262091767,-13.7020508739217,
119.891355007195)) ;
#156547=CARTESIAN_POINT('Ctrl Pts',(-9.13850646392357,-13.7020508801849,
119.867123964248)) ;
#156548=CARTESIAN_POINT('Ctrl Pts',(-9.21231030692947,-13.7020508864481,
119.842892921301)) ;
#156549=CARTESIAN_POINT('Ctrl Pts',(-9.23507556208875,-13.7229316148234,
119.912232215233)) ;
#156550=CARTESIAN_POINT('Ctrl Pts',(-9.25784081724804,-13.7438123431986,
119.981571509164)) ;
#156551=CARTESIAN_POINT('Ctrl Pts',(-9.18403697424214,-13.7438123369354,
120.005802552111)) ;
#156552=CARTESIAN_POINT('Ctrl Pts',(-9.11023313123624,-13.7438123306722,
120.030033595058)) ;
#156553=CARTESIAN_POINT('Ctrl Pts',(-9.08746787607695,-13.7229316022969,
119.960694301127)) ;
#156554=CARTESIAN_POINT('Ctrl Pts',(-9.06117191970581,-13.9881204584926,
119.845257989114)) ;
#156555=CARTESIAN_POINT('Ctrl Pts',(-9.0409411018076,-13.948693047744,119.783638182254)) ;
#156556=CARTESIAN_POINT('Ctrl Pts',(-9.11474494342789,-13.9486930580491,
119.759407135087)) ;
#156557=CARTESIAN_POINT('Ctrl Pts',(-9.18854878504819,-13.9486930683542,
119.735176087919)) ;
#156558=CARTESIAN_POINT('Ctrl Pts',(-9.2087796029464,-13.9881204791028,
119.796795894779)) ;
#156559=CARTESIAN_POINT('Ctrl Pts',(-9.2290104208446,-14.0275478898515,
119.858415701639)) ;
#156560=CARTESIAN_POINT('Ctrl Pts',(-9.1552065792243,-14.0275478795464,
119.882646748806)) ;
#156561=CARTESIAN_POINT('Ctrl Pts',(-9.081402737604,-14.0275478692412,119.906877795974)) ;
#156562=CARTESIAN_POINT('Ctrl Pts',(-9.06117191970581,-13.9881204584926,
119.845257989114)) ;
#156563=CARTESIAN_POINT('Ctrl Pts',(-9.01419630762022,-14.2135626266573,
119.66671241156)) ;
#156564=CARTESIAN_POINT('Ctrl Pts',(-8.99794998984458,-14.1583369427659,
119.617228749313)) ;
#156565=CARTESIAN_POINT('Ctrl Pts',(-9.07175382911603,-14.1583369561378,
119.592997694991)) ;
#156566=CARTESIAN_POINT('Ctrl Pts',(-9.14555766838748,-14.1583369695098,
119.568766640669)) ;
#156567=CARTESIAN_POINT('Ctrl Pts',(-9.16180398616311,-14.2135626534012,
119.618250302917)) ;
#156568=CARTESIAN_POINT('Ctrl Pts',(-9.17805030393876,-14.2687883372926,
119.667733965164)) ;
#156569=CARTESIAN_POINT('Ctrl Pts',(-9.10424646466731,-14.2687883239207,
119.691965019485)) ;
#156570=CARTESIAN_POINT('Ctrl Pts',(-9.03044262539586,-14.2687883105487,
119.716196073807)) ;
#156571=CARTESIAN_POINT('Ctrl Pts',(-9.01419630762022,-14.2135626266573,
119.66671241156)) ;
#156572=CARTESIAN_POINT('Ctrl Pts',(-8.95045579816424,-14.3820856851378,
119.437041610208)) ;
#156573=CARTESIAN_POINT('Ctrl Pts',(-8.93937158994986,-14.3150132250762,
119.403280900945)) ;
#156574=CARTESIAN_POINT('Ctrl Pts',(-9.01317542591036,-14.3150132383268,
119.379049836539)) ;
#156575=CARTESIAN_POINT('Ctrl Pts',(-9.08697926187084,-14.3150132515775,
119.354818772132)) ;
#156576=CARTESIAN_POINT('Ctrl Pts',(-9.09806347008522,-14.3820857116392,
119.388579481395)) ;
#156577=CARTESIAN_POINT('Ctrl Pts',(-9.10914767829959,-14.4491581717009,
119.422340190658)) ;
#156578=CARTESIAN_POINT('Ctrl Pts',(-9.0353438423391,-14.4491581584502,
119.446571255064)) ;
#156579=CARTESIAN_POINT('Ctrl Pts',(-8.96154000637861,-14.4491581451995,
119.47080231947)) ;
#156580=CARTESIAN_POINT('Ctrl Pts',(-8.95045579816424,-14.3820856851378,
119.437041610208)) ;
#156581=CARTESIAN_POINT('Ctrl Pts',(-8.87581727914137,-14.4811007735871,
119.174352555604)) ;
#156582=CARTESIAN_POINT('Ctrl Pts',(-8.8706599200612,-14.4070183383993,
119.158644072651)) ;
#156583=CARTESIAN_POINT('Ctrl Pts',(-8.94446375296266,-14.4070183464706,
119.134412998928)) ;
#156584=CARTESIAN_POINT('Ctrl Pts',(-9.0182675858641,-14.4070183545419,
119.110181925204)) ;
#156585=CARTESIAN_POINT('Ctrl Pts',(-9.02342494494427,-14.4811007897297,
119.125890408156)) ;
#156586=CARTESIAN_POINT('Ctrl Pts',(-9.02858230402444,-14.5551832249176,
119.141598891109)) ;
#156587=CARTESIAN_POINT('Ctrl Pts',(-8.95477847112299,-14.5551832168463,
119.165829964832)) ;
#156588=CARTESIAN_POINT('Ctrl Pts',(-8.88097463822153,-14.555183208775,
119.190061038556)) ;
#156589=CARTESIAN_POINT('Ctrl Pts',(-8.87581727914137,-14.4811007735871,
119.174352555604)) ;
#156590=CARTESIAN_POINT('Ctrl Pts',(-8.79562316232527,-14.5043853087956,
118.894554465702)) ;
#156591=CARTESIAN_POINT('Ctrl Pts',(-8.79679290375713,-14.4285698473868,
118.898117310217)) ;
#156592=CARTESIAN_POINT('Ctrl Pts',(-8.87059673344941,-14.4285698457663,
118.873886226719)) ;
#156593=CARTESIAN_POINT('Ctrl Pts',(-8.9444005631417,-14.4285698441458,
118.849655143221)) ;
#156594=CARTESIAN_POINT('Ctrl Pts',(-8.94323082170984,-14.5043853055546,
118.846092298706)) ;
#156595=CARTESIAN_POINT('Ctrl Pts',(-8.94206108027798,-14.5802007669634,
118.842529454191)) ;
#156596=CARTESIAN_POINT('Ctrl Pts',(-8.86825725058571,-14.5802007685839,
118.866760537689)) ;
#156597=CARTESIAN_POINT('Ctrl Pts',(-8.79445342089341,-14.5802007702044,
118.890991621187)) ;
#156598=CARTESIAN_POINT('Ctrl Pts',(-8.79562316232527,-14.5043853087956,
118.894554465702)) ;
#156599=CARTESIAN_POINT('Ctrl Pts',(-8.71698219857194,-14.4497319209782,
118.619592459032)) ;
#156600=CARTESIAN_POINT('Ctrl Pts',(-8.72437748963348,-14.3776228604659,
118.642117323393)) ;
#156601=CARTESIAN_POINT('Ctrl Pts',(-8.79818131745724,-14.3776228445383,
118.617886234204)) ;
#156602=CARTESIAN_POINT('Ctrl Pts',(-8.87198514528099,-14.3776228286107,
118.593655145014)) ;
#156603=CARTESIAN_POINT('Ctrl Pts',(-8.86458985421945,-14.449731889123,
118.571130280654)) ;
#156604=CARTESIAN_POINT('Ctrl Pts',(-8.85719456315791,-14.5218409496353,
118.548605416293)) ;
#156605=CARTESIAN_POINT('Ctrl Pts',(-8.78339073533415,-14.5218409655629,
118.572836505482)) ;
#156606=CARTESIAN_POINT('Ctrl Pts',(-8.7095869075104,-14.5218409814906,
118.597067594671)) ;
#156607=CARTESIAN_POINT('Ctrl Pts',(-8.71698219857194,-14.4497319209782,
118.619592459032)) ;
#156608=CARTESIAN_POINT('Ctrl Pts',(-8.64580441276013,-14.3208489038209,
118.36724001526)) ;
#156609=CARTESIAN_POINT('Ctrl Pts',(-8.65891567247647,-14.25763373208,118.407174798059)) ;
#156610=CARTESIAN_POINT('Ctrl Pts',(-8.73271949971065,-14.2576336982123,
118.382943707073)) ;
#156611=CARTESIAN_POINT('Ctrl Pts',(-8.80652332694482,-14.2576336643446,
118.358712616088)) ;
#156612=CARTESIAN_POINT('Ctrl Pts',(-8.79341206722847,-14.3208488360855,
118.318777833289)) ;
#156613=CARTESIAN_POINT('Ctrl Pts',(-8.78030080751211,-14.3840640078265,
118.278843050491)) ;
#156614=CARTESIAN_POINT('Ctrl Pts',(-8.70649698027795,-14.3840640416942,
118.303074141476)) ;
#156615=CARTESIAN_POINT('Ctrl Pts',(-8.63269315304377,-14.3840640755619,
118.327305232461)) ;
#156616=CARTESIAN_POINT('Ctrl Pts',(-8.64580441276013,-14.3208489038209,
118.36724001526)) ;
#156617=CARTESIAN_POINT('Ctrl Pts',(-8.5883553866719,-14.1269083086763,
118.156726837458)) ;
#156618=CARTESIAN_POINT('Ctrl Pts',(-8.60623187044661,-14.0771420046429,
118.211175724042)) ;
#156619=CARTESIAN_POINT('Ctrl Pts',(-8.68003569934284,-14.0771419513953,
118.18694463812)) ;
#156620=CARTESIAN_POINT('Ctrl Pts',(-8.75383952823908,-14.0771418981477,
118.162713552197)) ;
#156621=CARTESIAN_POINT('Ctrl Pts',(-8.73596304446436,-14.1269082021811,
118.108264665612)) ;
#156622=CARTESIAN_POINT('Ctrl Pts',(-8.71808656068964,-14.1766745062146,
118.053815779028)) ;
#156623=CARTESIAN_POINT('Ctrl Pts',(-8.64428273179342,-14.1766745594622,
118.07804686495)) ;
#156624=CARTESIAN_POINT('Ctrl Pts',(-8.57047890289718,-14.1766746127098,
118.102277950873)) ;
#156625=CARTESIAN_POINT('Ctrl Pts',(-8.5883553866719,-14.1269083086763,
118.156726837458)) ;
#156626=CARTESIAN_POINT('Ctrl Pts',(-8.54955936673305,-13.8839530008224,
118.003271664693)) ;
#156627=CARTESIAN_POINT('Ctrl Pts',(-8.5709004469701,-13.8510774674815,
118.068273153212)) ;
#156628=CARTESIAN_POINT('Ctrl Pts',(-8.64470427993426,-13.8510773982051,
118.044042079679)) ;
#156629=CARTESIAN_POINT('Ctrl Pts',(-8.71850811289841,-13.8510773289287,
118.019811006147)) ;
#156630=CARTESIAN_POINT('Ctrl Pts',(-8.69716703266136,-13.8839528622696,
117.954809517628)) ;
#156631=CARTESIAN_POINT('Ctrl Pts',(-8.6758259524243,-13.9168283956105,
117.88980802911)) ;
#156632=CARTESIAN_POINT('Ctrl Pts',(-8.60202211946015,-13.9168284648869,
117.914039102643)) ;
#156633=CARTESIAN_POINT('Ctrl Pts',(-8.52821828649599,-13.9168285341632,
117.938270176175)) ;
#156634=CARTESIAN_POINT('Ctrl Pts',(-8.54955936673305,-13.8839530008224,
118.003271664693)) ;
#156635=CARTESIAN_POINT('Ctrl Pts',(-8.53248329253628,-13.6058131007772,
117.915704634662)) ;
#156636=CARTESIAN_POINT('Ctrl Pts',(-8.55578333401837,-13.592308546656,
117.986672803208)) ;
#156637=CARTESIAN_POINT('Ctrl Pts',(-8.62958717268441,-13.5923084632408,
117.962441747043)) ;
#156638=CARTESIAN_POINT('Ctrl Pts',(-8.70339101135044,-13.5923083798256,
117.938210690877)) ;
#156639=CARTESIAN_POINT('Ctrl Pts',(-8.68009096986836,-13.6058129339469,
117.867242522331)) ;
#156640=CARTESIAN_POINT('Ctrl Pts',(-8.65679092838625,-13.6193174880682,
117.796274353786)) ;
#156641=CARTESIAN_POINT('Ctrl Pts',(-8.58298708972022,-13.6193175714834,
117.820505409951)) ;
#156642=CARTESIAN_POINT('Ctrl Pts',(-8.50918325105419,-13.6193176548985,
117.844736466117)) ;
#156643=CARTESIAN_POINT('Ctrl Pts',(-8.53248329253628,-13.6058131007772,
117.915704634662)) ;
#156644=CARTESIAN_POINT('Ctrl Pts',(-8.53937026013509,-13.3154623494247,
117.901296893058)) ;
#156645=CARTESIAN_POINT('Ctrl Pts',(-8.56295544834905,-13.3222095128514,
117.973133572653)) ;
#156646=CARTESIAN_POINT('Ctrl Pts',(-8.63675929426366,-13.3222094225439,
117.948902538566)) ;
#156647=CARTESIAN_POINT('Ctrl Pts',(-8.71056314017827,-13.3222093322365,
117.924671504478)) ;
#156648=CARTESIAN_POINT('Ctrl Pts',(-8.68697795196431,-13.3154621688099,
117.852834824883)) ;
#156649=CARTESIAN_POINT('Ctrl Pts',(-8.66339276375033,-13.3087150053832,
117.780998145287)) ;
#156650=CARTESIAN_POINT('Ctrl Pts',(-8.58958891783573,-13.3087150956907,
117.805229179375)) ;
#156651=CARTESIAN_POINT('Ctrl Pts',(-8.51578507192111,-13.3087151859981,
117.829460213462)) ;
#156652=CARTESIAN_POINT('Ctrl Pts',(-8.53937026013509,-13.3154623494247,
117.901296893058)) ;
#156653=CARTESIAN_POINT('Ctrl Pts',(-8.57069168239456,-13.0305252756843,
117.961054033285)) ;
#156654=CARTESIAN_POINT('Ctrl Pts',(-8.59286220817367,-13.057175468413,
118.028581879486)) ;
#156655=CARTESIAN_POINT('Ctrl Pts',(-8.66666606225781,-13.0571753774731,
118.004350870281)) ;
#156656=CARTESIAN_POINT('Ctrl Pts',(-8.74046991634194,-13.0571752865332,
117.980119861077)) ;
#156657=CARTESIAN_POINT('Ctrl Pts',(-8.71829939056283,-13.0305250938045,
117.912592014877)) ;
#156658=CARTESIAN_POINT('Ctrl Pts',(-8.69612886478371,-13.0038749010759,
117.845064168676)) ;
#156659=CARTESIAN_POINT('Ctrl Pts',(-8.62232501069957,-13.0038749920158,
117.869295177881)) ;
#156660=CARTESIAN_POINT('Ctrl Pts',(-8.54852115661543,-13.0038750829557,
117.893526187085)) ;
#156661=CARTESIAN_POINT('Ctrl Pts',(-8.57069168239456,-13.0305252756843,
117.961054033285)) ;
#156662=CARTESIAN_POINT('Ctrl Pts',(-8.62430702145784,-12.7760411077928,
118.089081673625)) ;
#156663=CARTESIAN_POINT('Ctrl Pts',(-8.64349646537957,-12.8204973460342,
118.147529625551)) ;
#156664=CARTESIAN_POINT('Ctrl Pts',(-8.71730032725692,-12.8204972646132,
118.123298640083)) ;
#156665=CARTESIAN_POINT('Ctrl Pts',(-8.79110418913424,-12.8204971831922,
118.099067654616)) ;
#156666=CARTESIAN_POINT('Ctrl Pts',(-8.77191474521251,-12.7760409449508,
118.04061970269)) ;
#156667=CARTESIAN_POINT('Ctrl Pts',(-8.75272530129079,-12.7315847067095,
117.982171750764)) ;
#156668=CARTESIAN_POINT('Ctrl Pts',(-8.67892143941345,-12.7315847881305,
118.006402736232)) ;
#156669=CARTESIAN_POINT('Ctrl Pts',(-8.60511757753611,-12.7315848695515,
118.030633721699)) ;
#156670=CARTESIAN_POINT('Ctrl Pts',(-8.62430702145784,-12.7760411077928,
118.089081673625)) ;
#156671=CARTESIAN_POINT('Ctrl Pts',(-8.69778013803695,-12.5658693797106,
118.277375059853)) ;
#156672=CARTESIAN_POINT('Ctrl Pts',(-8.71260256265765,-12.6250641545161,
118.322521775676)) ;
#156673=CARTESIAN_POINT('Ctrl Pts',(-8.78640643152489,-12.6250640894152,
118.298290811498)) ;
#156674=CARTESIAN_POINT('Ctrl Pts',(-8.86021030039212,-12.6250640243143,
118.274059847321)) ;
#156675=CARTESIAN_POINT('Ctrl Pts',(-8.84538787577142,-12.5658692495088,
118.228913131498)) ;
#156676=CARTESIAN_POINT('Ctrl Pts',(-8.83056545115072,-12.5066744747032,
118.183766415675)) ;
#156677=CARTESIAN_POINT('Ctrl Pts',(-8.75676158228349,-12.5066745398042,
118.207997379852)) ;
#156678=CARTESIAN_POINT('Ctrl Pts',(-8.68295771341625,-12.506674604905,
118.232228344029)) ;
#156679=CARTESIAN_POINT('Ctrl Pts',(-8.69778013803695,-12.5658693797106,
118.277375059853)) ;
#156680=CARTESIAN_POINT('Ctrl Pts',(-8.78628545767639,-12.4170609140262,
118.511509776539)) ;
#156681=CARTESIAN_POINT('Ctrl Pts',(-8.79568383392516,-12.4867319202062,
118.540135716234)) ;
#156682=CARTESIAN_POINT('Ctrl Pts',(-8.86948770797218,-12.4867318782286,
118.515904767834)) ;
#156683=CARTESIAN_POINT('Ctrl Pts',(-8.94329158201918,-12.4867318362511,
118.491673819433)) ;
#156684=CARTESIAN_POINT('Ctrl Pts',(-8.9338932057704,-12.4170608300712,
118.463047879737)) ;
#156685=CARTESIAN_POINT('Ctrl Pts',(-8.92449482952162,-12.3473898238912,
118.434421940042)) ;
#156686=CARTESIAN_POINT('Ctrl Pts',(-8.85069095547461,-12.3473898658687,
118.458652888443)) ;
#156687=CARTESIAN_POINT('Ctrl Pts',(-8.7768870814276,-12.3473899078463,
118.482883836843)) ;
#156688=CARTESIAN_POINT('Ctrl Pts',(-8.78628545767639,-12.4170609140262,
118.511509776539)) ;
#156689=CARTESIAN_POINT('Ctrl Pts',(-8.88463232709871,-12.3396249333132,
118.775501151269)) ;
#156690=CARTESIAN_POINT('Ctrl Pts',(-8.8879141833157,-12.4148052434578,
118.785497157874)) ;
#156691=CARTESIAN_POINT('Ctrl Pts',(-8.9617180602112,-12.4148052290128,
118.761266218149)) ;
#156692=CARTESIAN_POINT('Ctrl Pts',(-9.0355219371067,-12.4148052145678,
118.737035278425)) ;
#156693=CARTESIAN_POINT('Ctrl Pts',(-9.03224008088971,-12.3396249044232,
118.72703927182)) ;
#156694=CARTESIAN_POINT('Ctrl Pts',(-9.02895822467271,-12.2644445942785,
118.717043265215)) ;
#156695=CARTESIAN_POINT('Ctrl Pts',(-8.95515434777721,-12.2644446087235,
118.74127420494)) ;
#156696=CARTESIAN_POINT('Ctrl Pts',(-8.88135047088172,-12.2644446231686,
118.765505144665)) ;
#156697=CARTESIAN_POINT('Ctrl Pts',(-8.88463232709871,-12.3396249333132,
118.775501151269)) ;
#156698=CARTESIAN_POINT('Ctrl Pts',(-8.9861492359783,-12.340046412335,119.04917803503)) ;
#156699=CARTESIAN_POINT('Ctrl Pts',(-8.98308354184458,-12.4153088432885,
119.03984042744)) ;
#156700=CARTESIAN_POINT('Ctrl Pts',(-9.05688741871824,-12.4153088579802,
119.015609487649)) ;
#156701=CARTESIAN_POINT('Ctrl Pts',(-9.13069129559191,-12.4153088726718,
118.991378547857)) ;
#156702=CARTESIAN_POINT('Ctrl Pts',(-9.13375698972563,-12.3400464417183,
119.000716155448)) ;
#156703=CARTESIAN_POINT('Ctrl Pts',(-9.13682268385935,-12.2647840107648,
119.010053763039)) ;
#156704=CARTESIAN_POINT('Ctrl Pts',(-9.06301880698568,-12.2647839960732,
119.03428470283)) ;
#156705=CARTESIAN_POINT('Ctrl Pts',(-8.98921493011202,-12.2647839813815,
119.058515642621)) ;
#156706=CARTESIAN_POINT('Ctrl Pts',(-8.9861492359783,-12.340046412335,119.04917803503)) ;
#156707=CARTESIAN_POINT('Ctrl Pts',(-9.08378193823022,-12.4170460254182,
119.311248494083)) ;
#156708=CARTESIAN_POINT('Ctrl Pts',(-9.07462576737877,-12.4870438442232,
119.283360277089)) ;
#156709=CARTESIAN_POINT('Ctrl Pts',(-9.14842964160796,-12.487043886487,
119.259129329243)) ;
#156710=CARTESIAN_POINT('Ctrl Pts',(-9.22223351583714,-12.4870439287509,
119.234898381398)) ;
#156711=CARTESIAN_POINT('Ctrl Pts',(-9.23138968668858,-12.4170461099459,
119.262786598391)) ;
#156712=CARTESIAN_POINT('Ctrl Pts',(-9.24054585754002,-12.3470482911409,
119.290674815385)) ;
#156713=CARTESIAN_POINT('Ctrl Pts',(-9.16674198331085,-12.3470482488771,
119.314905763231)) ;
#156714=CARTESIAN_POINT('Ctrl Pts',(-9.09293810908166,-12.3470482066133,
119.339136711077)) ;
#156715=CARTESIAN_POINT('Ctrl Pts',(-9.08378193823022,-12.4170460254182,
119.311248494083)) ;
#156716=CARTESIAN_POINT('Ctrl Pts',(-9.17250255530307,-12.5662136094611,
119.545947051563)) ;
#156717=CARTESIAN_POINT('Ctrl Pts',(-9.1578737421701,-12.625901534808,119.501390049144)) ;
#156718=CARTESIAN_POINT('Ctrl Pts',(-9.23167761123566,-12.6259016005162,
119.477159085571)) ;
#156719=CARTESIAN_POINT('Ctrl Pts',(-9.3054814803012,-12.6259016662244,
119.452928121997)) ;
#156720=CARTESIAN_POINT('Ctrl Pts',(-9.32011029343416,-12.5662137408776,
119.497485124416)) ;
#156721=CARTESIAN_POINT('Ctrl Pts',(-9.33473910656713,-12.5065258155307,
119.542042126834)) ;
#156722=CARTESIAN_POINT('Ctrl Pts',(-9.26093523750158,-12.5065257498225,
119.566273090408)) ;
#156723=CARTESIAN_POINT('Ctrl Pts',(-9.18713136843604,-12.5065256841143,
119.590504053981)) ;
#156724=CARTESIAN_POINT('Ctrl Pts',(-9.17250255530307,-12.5662136094611,
119.545947051563)) ;
#156725=CARTESIAN_POINT('Ctrl Pts',(-9.24585112857785,-12.7760199991739,
119.733930887948)) ;
#156726=CARTESIAN_POINT('Ctrl Pts',(-9.22681247363185,-12.8211489416697,
119.675942218833)) ;
#156727=CARTESIAN_POINT('Ctrl Pts',(-9.30061633575258,-12.8211490243987,
119.651711234107)) ;
#156728=CARTESIAN_POINT('Ctrl Pts',(-9.37442019787332,-12.8211491071278,
119.627480249381)) ;
#156729=CARTESIAN_POINT('Ctrl Pts',(-9.39345885281933,-12.776020164632,
119.685468918496)) ;
#156730=CARTESIAN_POINT('Ctrl Pts',(-9.41249750776533,-12.7308912221363,
119.743457587611)) ;
#156731=CARTESIAN_POINT('Ctrl Pts',(-9.33869364564458,-12.7308911394072,
119.767688572337)) ;
#156732=CARTESIAN_POINT('Ctrl Pts',(-9.26488978352385,-12.7308910566782,
119.791919557063)) ;
#156733=CARTESIAN_POINT('Ctrl Pts',(-9.24585112857785,-12.7760199991739,
119.733930887948)) ;
#156734=CARTESIAN_POINT('Ctrl Pts',(-9.29969159508292,-13.0322696653641,
119.862416821601)) ;
#156735=CARTESIAN_POINT('Ctrl Pts',(-9.27760000870786,-13.0595756323769,
119.795129415856)) ;
#156736=CARTESIAN_POINT('Ctrl Pts',(-9.35140386280755,-13.059575723918,
119.770898406699)) ;
#156737=CARTESIAN_POINT('Ctrl Pts',(-9.42520771690725,-13.0595758154591,
119.746667397542)) ;
#156738=CARTESIAN_POINT('Ctrl Pts',(-9.44729930328231,-13.0322698484462,
119.813954803287)) ;
#156739=CARTESIAN_POINT('Ctrl Pts',(-9.46939088965738,-13.0049638814334,
119.881242209032)) ;
#156740=CARTESIAN_POINT('Ctrl Pts',(-9.39558703555768,-13.0049637898923,
119.905473218189)) ;
#156741=CARTESIAN_POINT('Ctrl Pts',(-9.32178318145799,-13.0049636983512,
119.929704227346)) ;
#156742=CARTESIAN_POINT('Ctrl Pts',(-9.29969159508292,-13.0322696653641,
119.862416821601)) ;
#156743=CARTESIAN_POINT('Ctrl Pts',(-9.33072971583805,-13.3151090323585,
119.921587753964)) ;
#156744=CARTESIAN_POINT('Ctrl Pts',(-9.30716980380042,-13.3227086607463,
119.849828065076)) ;
#156745=CARTESIAN_POINT('Ctrl Pts',(-9.38097364977465,-13.3227087535366,
119.82559703117)) ;
#156746=CARTESIAN_POINT('Ctrl Pts',(-9.4547774957489,-13.3227088463268,
119.801365997264)) ;
#156747=CARTESIAN_POINT('Ctrl Pts',(-9.47833740778652,-13.315109217939,
119.873125686152)) ;
#156748=CARTESIAN_POINT('Ctrl Pts',(-9.50189731982416,-13.3075095895512,
119.944885375041)) ;
#156749=CARTESIAN_POINT('Ctrl Pts',(-9.42809347384992,-13.307509496761,
119.969116408947)) ;
#156750=CARTESIAN_POINT('Ctrl Pts',(-9.35428962787569,-13.3075094039707,
119.993347442852)) ;
#156751=CARTESIAN_POINT('Ctrl Pts',(-9.33072971583805,-13.3151090323585,
119.921587753964)) ;
#156752=CARTESIAN_POINT('Ctrl Pts',(-9.33762134165996,-13.6075492018493,
119.906927850832)) ;
#156753=CARTESIAN_POINT('Ctrl Pts',(-9.31428227870287,-13.5947427678056,
119.835840832465)) ;
#156754=CARTESIAN_POINT('Ctrl Pts',(-9.38808611725758,-13.5947428521219,
119.81160977596)) ;
#156755=CARTESIAN_POINT('Ctrl Pts',(-9.4618899558123,-13.594742936438,119.787378719456)) ;
#156756=CARTESIAN_POINT('Ctrl Pts',(-9.48522901876938,-13.6075493704817,
119.858465737822)) ;
#156757=CARTESIAN_POINT('Ctrl Pts',(-9.50856808172646,-13.6203558045254,
119.929552756189)) ;
#156758=CARTESIAN_POINT('Ctrl Pts',(-9.43476424317175,-13.6203557202092,
119.953783812694)) ;
#156759=CARTESIAN_POINT('Ctrl Pts',(-9.36096040461704,-13.620355635893,
119.978014869198)) ;
#156760=CARTESIAN_POINT('Ctrl Pts',(-9.33762134165996,-13.6075492018493,
119.906927850832)) ;
#156761=CARTESIAN_POINT('Ctrl Pts',(-9.32055446084888,-13.8839937911961,
119.819605029903)) ;
#156762=CARTESIAN_POINT('Ctrl Pts',(-9.29910313304257,-13.8518669319433,
119.754267748105)) ;
#156763=CARTESIAN_POINT('Ctrl Pts',(-9.37290696562471,-13.8518670036745,
119.730036673409)) ;
#156764=CARTESIAN_POINT('Ctrl Pts',(-9.44671079820685,-13.8518670754058,
119.705805598712)) ;
#156765=CARTESIAN_POINT('Ctrl Pts',(-9.46816212601316,-13.8839939346586,
119.771142880511)) ;
#156766=CARTESIAN_POINT('Ctrl Pts',(-9.48961345381948,-13.9161207939113,
119.83648016231)) ;
#156767=CARTESIAN_POINT('Ctrl Pts',(-9.41580962123734,-13.9161207221801,
119.860711237006)) ;
#156768=CARTESIAN_POINT('Ctrl Pts',(-9.3420057886552,-13.9161206504489,
119.884942311702)) ;
#156769=CARTESIAN_POINT('Ctrl Pts',(-9.32055446084888,-13.8839937911961,
119.819605029903)) ;
#156770=CARTESIAN_POINT('Ctrl Pts',(-9.28147726722591,-14.1283418739825,
119.665069210431)) ;
#156771=CARTESIAN_POINT('Ctrl Pts',(-9.2634566491389,-14.0791061363548,
119.610181316741)) ;
#156772=CARTESIAN_POINT('Ctrl Pts',(-9.33726047777319,-14.079106190233,
119.58595023002)) ;
#156773=CARTESIAN_POINT('Ctrl Pts',(-9.41106430640748,-14.0791062441112,
119.561719143299)) ;
#156774=CARTESIAN_POINT('Ctrl Pts',(-9.42908492449449,-14.1283419817388,
119.61660703699)) ;
#156775=CARTESIAN_POINT('Ctrl Pts',(-9.44710554258149,-14.1775777193664,
119.671494930681)) ;
#156776=CARTESIAN_POINT('Ctrl Pts',(-9.37330171394721,-14.1775776654883,
119.695726017402)) ;
#156777=CARTESIAN_POINT('Ctrl Pts',(-9.29949788531291,-14.1775776116101,
119.719957104122)) ;
#156778=CARTESIAN_POINT('Ctrl Pts',(-9.28147726722591,-14.1283418739825,
119.665069210431)) ;
#156779=CARTESIAN_POINT('Ctrl Pts',(-9.22417716238159,-14.321085337762,
119.455168775729)) ;
#156780=CARTESIAN_POINT('Ctrl Pts',(-9.21086198390688,-14.2583178356259,
119.414612891736)) ;
#156781=CARTESIAN_POINT('Ctrl Pts',(-9.28466581049705,-14.2583178709165,
119.390381798789)) ;
#156782=CARTESIAN_POINT('Ctrl Pts',(-9.35846963708723,-14.2583179062071,
119.366150705843)) ;
#156783=CARTESIAN_POINT('Ctrl Pts',(-9.37178481556196,-14.3210854083432,
119.406706589835)) ;
#156784=CARTESIAN_POINT('Ctrl Pts',(-9.38509999403666,-14.3838529104793,
119.447262473828)) ;
#156785=CARTESIAN_POINT('Ctrl Pts',(-9.31129616744649,-14.3838528751887,
119.471493566774)) ;
#156786=CARTESIAN_POINT('Ctrl Pts',(-9.23749234085631,-14.3838528398981,
119.495724659721)) ;
#156787=CARTESIAN_POINT('Ctrl Pts',(-9.22417716238159,-14.321085337762,
119.455168775729)) ;
#156788=CARTESIAN_POINT('Ctrl Pts',(-9.1528918141783,-14.4501544762085,
119.202433516862)) ;
#156789=CARTESIAN_POINT('Ctrl Pts',(-9.1452704554292,-14.3782797175252,
119.179220088868)) ;
#156790=CARTESIAN_POINT('Ctrl Pts',(-9.21907428260848,-14.378279733915,
119.154988997716)) ;
#156791=CARTESIAN_POINT('Ctrl Pts',(-9.29287810978775,-14.3782797503047,
119.130757906563)) ;
#156792=CARTESIAN_POINT('Ctrl Pts',(-9.30049946853686,-14.450154508988,
119.153971334557)) ;
#156793=CARTESIAN_POINT('Ctrl Pts',(-9.30812082728596,-14.5220292676713,
119.177184762551)) ;
#156794=CARTESIAN_POINT('Ctrl Pts',(-9.23431700010668,-14.5220292512815,
119.201415853704)) ;
#156795=CARTESIAN_POINT('Ctrl Pts',(-9.1605131729274,-14.5220292348918,
119.225646944856)) ;
#156796=CARTESIAN_POINT('Ctrl Pts',(-9.1528918141783,-14.4501544762085,
119.202433516862)) ;
#156797=CARTESIAN_POINT('Ctrl Pts',(-9.07410157725992,-14.504350239421,
118.926962323926)) ;
#156798=CARTESIAN_POINT('Ctrl Pts',(-9.07270431240989,-14.4285822954382,
118.922706481521)) ;
#156799=CARTESIAN_POINT('Ctrl Pts',(-9.14650814161148,-14.4285822971821,
118.898475396528)) ;
#156800=CARTESIAN_POINT('Ctrl Pts',(-9.22031197081306,-14.4285822989259,
118.874244311535)) ;
#156801=CARTESIAN_POINT('Ctrl Pts',(-9.2217092356631,-14.5043502429086,
118.87850015394)) ;
#156802=CARTESIAN_POINT('Ctrl Pts',(-9.22310650051312,-14.5801181868914,
118.882755996344)) ;
#156803=CARTESIAN_POINT('Ctrl Pts',(-9.14930267131155,-14.5801181851475,
118.906987081337)) ;
#156804=CARTESIAN_POINT('Ctrl Pts',(-9.07549884210995,-14.5801181834037,
118.93121816633)) ;
#156805=CARTESIAN_POINT('Ctrl Pts',(-9.07410157725992,-14.504350239421,
118.926962323926)) ;
#156806=CARTESIAN_POINT('Ctrl Pts',(-8.99439714763998,-14.4811635345991,
118.648874617531)) ;
#156807=CARTESIAN_POINT('Ctrl Pts',(-8.99929378974257,-14.4069000332384,
118.663789000046)) ;
#156808=CARTESIAN_POINT('Ctrl Pts',(-9.0730976215289,-14.4069000243761,
118.639557922925)) ;
#156809=CARTESIAN_POINT('Ctrl Pts',(-9.14690145331523,-14.4069000155138,
118.615326845805)) ;
#156810=CARTESIAN_POINT('Ctrl Pts',(-9.14200481121263,-14.4811635168746,
118.600412463291)) ;
#156811=CARTESIAN_POINT('Ctrl Pts',(-9.13710816911003,-14.5554270182353,
118.585498080776)) ;
#156812=CARTESIAN_POINT('Ctrl Pts',(-9.0633043373237,-14.5554270270976,
118.609729157896)) ;
#156813=CARTESIAN_POINT('Ctrl Pts',(-8.98950050553737,-14.5554270359599,
118.633960235017)) ;
#156814=CARTESIAN_POINT('Ctrl Pts',(-8.99439714763998,-14.4811635345991,
118.648874617531)) ;
#156815=CARTESIAN_POINT('Ctrl Pts',(-8.91938092952298,-14.3816036851556,
118.384850057937)) ;
#156816=CARTESIAN_POINT('Ctrl Pts',(-8.93025827732114,-14.3141789361096,
118.417980704839)) ;
#156817=CARTESIAN_POINT('Ctrl Pts',(-9.00406211280163,-14.3141789218921,
118.393749638971)) ;
#156818=CARTESIAN_POINT('Ctrl Pts',(-9.0778659482821,-14.3141789076745,
118.369518573102)) ;
#156819=CARTESIAN_POINT('Ctrl Pts',(-9.06698860048393,-14.3816036567204,
118.3363879262)) ;
#156820=CARTESIAN_POINT('Ctrl Pts',(-9.05611125268575,-14.4490284057664,
118.303257279298)) ;
#156821=CARTESIAN_POINT('Ctrl Pts',(-8.98230741720528,-14.449028419984,
118.327488345167)) ;
#156822=CARTESIAN_POINT('Ctrl Pts',(-8.9085035817248,-14.4490284342016,
118.351719411035)) ;
#156823=CARTESIAN_POINT('Ctrl Pts',(-8.91938092952298,-14.3816036851556,
118.384850057937)) ;
#156824=CARTESIAN_POINT('Ctrl Pts',(-8.8558492241993,-14.2132115910195,
118.155902462999)) ;
#156825=CARTESIAN_POINT('Ctrl Pts',(-8.8719124615394,-14.1574425718006,
118.204828492554)) ;
#156826=CARTESIAN_POINT('Ctrl Pts',(-8.94571630025698,-14.1574425567691,
118.180597436545)) ;
#156827=CARTESIAN_POINT('Ctrl Pts',(-9.01952013897455,-14.1574425417376,
118.156366380536)) ;
#156828=CARTESIAN_POINT('Ctrl Pts',(-9.00345690163445,-14.2132115609565,
118.107440350981)) ;
#156829=CARTESIAN_POINT('Ctrl Pts',(-8.98739366429436,-14.2689805801753,
118.058514321426)) ;
#156830=CARTESIAN_POINT('Ctrl Pts',(-8.91358982557679,-14.2689805952068,
118.082745377435)) ;
#156831=CARTESIAN_POINT('Ctrl Pts',(-8.8397859868592,-14.2689806102383,
118.106976433443)) ;
#156832=CARTESIAN_POINT('Ctrl Pts',(-8.8558492241993,-14.2132115910195,
118.155902462999)) ;
#156833=CARTESIAN_POINT('Ctrl Pts',(-8.80875359263179,-13.9871283531687,
117.97689596451)) ;
#156834=CARTESIAN_POINT('Ctrl Pts',(-8.8288655504278,-13.9470611393289,
118.038153743158)) ;
#156835=CARTESIAN_POINT('Ctrl Pts',(-8.9026693918761,-13.9470611278095,
118.013922695466)) ;
#156836=CARTESIAN_POINT('Ctrl Pts',(-8.97647323332439,-13.9470611162902,
117.989691647775)) ;
#156837=CARTESIAN_POINT('Ctrl Pts',(-8.95636127552838,-13.98712833013,117.928433869127)) ;
#156838=CARTESIAN_POINT('Ctrl Pts',(-8.93624931773237,-14.0271955439699,
117.86717609048)) ;
#156839=CARTESIAN_POINT('Ctrl Pts',(-8.86244547628407,-14.0271955554892,
117.891407138171)) ;
#156840=CARTESIAN_POINT('Ctrl Pts',(-8.78864163483579,-14.0271955670085,
117.915638185862)) ;
#156841=CARTESIAN_POINT('Ctrl Pts',(-8.80875359263179,-13.9871283531687,
117.97689596451)) ;
#156842=CARTESIAN_POINT('Ctrl Pts',(-8.78260162901795,-13.7209751384546,
117.86180531742)) ;
#156843=CARTESIAN_POINT('Ctrl Pts',(-8.80530328477739,-13.6994320003675,
117.930950898101)) ;
#156844=CARTESIAN_POINT('Ctrl Pts',(-8.87910712770323,-13.6994319934453,
117.90671985491)) ;
#156845=CARTESIAN_POINT('Ctrl Pts',(-8.95291097062908,-13.699431986523,
117.882488811719)) ;
#156846=CARTESIAN_POINT('Ctrl Pts',(-8.93020931486964,-13.72097512461,117.813343231038)) ;
#156847=CARTESIAN_POINT('Ctrl Pts',(-8.9075076591102,-13.7425182626971,
117.744197650356)) ;
#156848=CARTESIAN_POINT('Ctrl Pts',(-8.83370381618435,-13.7425182696194,
117.768428693547)) ;
#156849=CARTESIAN_POINT('Ctrl Pts',(-8.75989997325851,-13.7425182765416,
117.792659736738)) ;
#156850=CARTESIAN_POINT('Ctrl Pts',(-8.78260162901795,-13.7209751384546,
117.86180531742)) ;
#156851=CARTESIAN_POINT('Ctrl Pts',(-8.7796418761099,-13.4341833204507,
117.817471206849)) ;
#156852=CARTESIAN_POINT('Ctrl Pts',(-8.80331509092212,-13.4326332891495,
117.889575999558)) ;
#156853=CARTESIAN_POINT('Ctrl Pts',(-8.87711893444489,-13.4326332865185,
117.865344958186)) ;
#156854=CARTESIAN_POINT('Ctrl Pts',(-8.95092277796765,-13.4326332838874,
117.841113916813)) ;
#156855=CARTESIAN_POINT('Ctrl Pts',(-8.92724956315542,-13.4341833151887,
117.769009124103)) ;
#156856=CARTESIAN_POINT('Ctrl Pts',(-8.90357634834319,-13.4357333464899,
117.696904331393)) ;
#156857=CARTESIAN_POINT('Ctrl Pts',(-8.82977250482043,-13.435733349121,
117.721135372766)) ;
#156858=CARTESIAN_POINT('Ctrl Pts',(-8.75596866129766,-13.435733351752,
117.745366414139)) ;
#156859=CARTESIAN_POINT('Ctrl Pts',(-8.7796418761099,-13.4341833204507,
117.817471206849)) ;
#156860=CARTESIAN_POINT('Ctrl Pts',(-8.80108831291345,-13.1440226446982,
117.847195297999)) ;
#156861=CARTESIAN_POINT('Ctrl Pts',(-8.82403622680466,-13.1627318776024,
117.917090941048)) ;
#156862=CARTESIAN_POINT('Ctrl Pts',(-8.89784007017418,-13.1627318792492,
117.892859899208)) ;
#156863=CARTESIAN_POINT('Ctrl Pts',(-8.97164391354369,-13.1627318808959,
117.868628857369)) ;
#156864=CARTESIAN_POINT('Ctrl Pts',(-8.94869599965246,-13.1440226479917,
117.79873321432)) ;
#156865=CARTESIAN_POINT('Ctrl Pts',(-8.92574808576123,-13.1253134150875,
117.72883757127)) ;
#156866=CARTESIAN_POINT('Ctrl Pts',(-8.85194424239172,-13.1253134134407,
117.75306861311)) ;
#156867=CARTESIAN_POINT('Ctrl Pts',(-8.7781403990222,-13.125313411794,117.77729965495)) ;
#156868=CARTESIAN_POINT('Ctrl Pts',(-8.80108831291345,-13.1440226446982,
117.847195297999)) ;
#156869=CARTESIAN_POINT('Ctrl Pts',(-8.84592426043001,-12.8750223963181,
117.948364040509)) ;
#156870=CARTESIAN_POINT('Ctrl Pts',(-8.86650795627559,-12.9125432630704,
118.011058656823)) ;
#156871=CARTESIAN_POINT('Ctrl Pts',(-8.94031179917461,-12.9125432659671,
117.986827613551)) ;
#156872=CARTESIAN_POINT('Ctrl Pts',(-9.01411564207361,-12.9125432688638,
117.962596570278)) ;
#156873=CARTESIAN_POINT('Ctrl Pts',(-8.99353194622804,-12.8750224021116,
117.899901953963)) ;
#156874=CARTESIAN_POINT('Ctrl Pts',(-8.97294825038245,-12.8375015353593,
117.837207337649)) ;
#156875=CARTESIAN_POINT('Ctrl Pts',(-8.89914440748345,-12.8375015324626,
117.861438380922)) ;
#156876=CARTESIAN_POINT('Ctrl Pts',(-8.82534056458443,-12.8375015295659,
117.885669424194)) ;
#156877=CARTESIAN_POINT('Ctrl Pts',(-8.84592426043001,-12.8750223963181,
117.948364040509)) ;
#156878=CARTESIAN_POINT('Ctrl Pts',(-8.91216833972909,-12.6437154561283,
118.114539740324)) ;
#156879=CARTESIAN_POINT('Ctrl Pts',(-8.92889332303276,-12.6974444198838,
118.165481340849)) ;
#156880=CARTESIAN_POINT('Ctrl Pts',(-9.00269716581704,-12.6974444216942,
118.141250297227)) ;
#156881=CARTESIAN_POINT('Ctrl Pts',(-9.07650100860129,-12.6974444235046,
118.117019253605)) ;
#156882=CARTESIAN_POINT('Ctrl Pts',(-9.05977602529763,-12.6437154597491,
118.06607765308)) ;
#156883=CARTESIAN_POINT('Ctrl Pts',(-9.04305104199395,-12.5899864959936,
118.015136052555)) ;
#156884=CARTESIAN_POINT('Ctrl Pts',(-8.96924719920968,-12.5899864941832,
118.039367096177)) ;
#156885=CARTESIAN_POINT('Ctrl Pts',(-8.89544335642542,-12.5899864923728,
118.063598139799)) ;
#156886=CARTESIAN_POINT('Ctrl Pts',(-8.91216833972909,-12.6437154561283,
118.114539740324)) ;
#156887=CARTESIAN_POINT('Ctrl Pts',(-8.99483011325719,-12.4695015573388,
118.331032618802)) ;
#156888=CARTESIAN_POINT('Ctrl Pts',(-9.00653775971677,-12.5354737259947,
118.366692220884)) ;
#156889=CARTESIAN_POINT('Ctrl Pts',(-9.08034160291349,-12.5354737260558,
118.342461178518)) ;
#156890=CARTESIAN_POINT('Ctrl Pts',(-9.15414544611019,-12.5354737261168,
118.318230136152)) ;
#156891=CARTESIAN_POINT('Ctrl Pts',(-9.1424377996506,-12.4695015574609,
118.28257053407)) ;
#156892=CARTESIAN_POINT('Ctrl Pts',(-9.130730153191,-12.403529388805,118.246910931988)) ;
#156893=CARTESIAN_POINT('Ctrl Pts',(-9.0569263099943,-12.403529388744,118.271141974354)) ;
#156894=CARTESIAN_POINT('Ctrl Pts',(-8.98312246679759,-12.4035293886829,
118.29537301672)) ;
#156895=CARTESIAN_POINT('Ctrl Pts',(-8.99483011325719,-12.4695015573388,
118.331032618802)) ;
#156896=CARTESIAN_POINT('Ctrl Pts',(-9.08998111303647,-12.3618253102505,
118.585299380963)) ;
#156897=CARTESIAN_POINT('Ctrl Pts',(-9.09579750273664,-12.4354130130407,
118.603015165592)) ;
#156898=CARTESIAN_POINT('Ctrl Pts',(-9.16960134725352,-12.4354130116483,
118.578784127247)) ;
#156899=CARTESIAN_POINT('Ctrl Pts',(-9.2434051917704,-12.4354130102558,
118.554553088902)) ;
#156900=CARTESIAN_POINT('Ctrl Pts',(-9.23758880207023,-12.3618253074657,
118.536837304273)) ;
#156901=CARTESIAN_POINT('Ctrl Pts',(-9.23177241237007,-12.2882376046756,
118.519121519645)) ;
#156902=CARTESIAN_POINT('Ctrl Pts',(-9.15796856785319,-12.288237606068,
118.543352557989)) ;
#156903=CARTESIAN_POINT('Ctrl Pts',(-9.0841647233363,-12.2882376074604,
118.567583596334)) ;
#156904=CARTESIAN_POINT('Ctrl Pts',(-9.08998111303647,-12.3618253102505,
118.585299380963)) ;
#156905=CARTESIAN_POINT('Ctrl Pts',(-9.1909709333649,-12.3304086987919,
118.857374561843)) ;
#156906=CARTESIAN_POINT('Ctrl Pts',(-9.19047930770828,-12.406297480682,
118.855877149609)) ;
#156907=CARTESIAN_POINT('Ctrl Pts',(-9.26428315423005,-12.4062974803833,
118.83164611737)) ;
#156908=CARTESIAN_POINT('Ctrl Pts',(-9.3380870007518,-12.4062974800845,
118.807415085132)) ;
#156909=CARTESIAN_POINT('Ctrl Pts',(-9.33857862640842,-12.3304086981944,
118.808912497366)) ;
#156910=CARTESIAN_POINT('Ctrl Pts',(-9.33907025206503,-12.2545199163043,
118.8104099096)) ;
#156911=CARTESIAN_POINT('Ctrl Pts',(-9.26526640554327,-12.2545199166031,
118.834640941838)) ;
#156912=CARTESIAN_POINT('Ctrl Pts',(-9.19146255902151,-12.2545199169019,
118.858871974077)) ;
#156913=CARTESIAN_POINT('Ctrl Pts',(-9.1909709333649,-12.3304086987919,
118.857374561843)) ;
#156914=CARTESIAN_POINT('Ctrl Pts',(-9.29090632432286,-12.3767667157857,
119.126380154863)) ;
#156915=CARTESIAN_POINT('Ctrl Pts',(-9.28416836803978,-12.4495286298161,
119.105857427502)) ;
#156916=CARTESIAN_POINT('Ctrl Pts',(-9.35797221631645,-12.4495286339673,
119.081626400609)) ;
#156917=CARTESIAN_POINT('Ctrl Pts',(-9.43177606459311,-12.4495286381184,
119.057395373716)) ;
#156918=CARTESIAN_POINT('Ctrl Pts',(-9.4385140208762,-12.376766724088,119.077918101077)) ;
#156919=CARTESIAN_POINT('Ctrl Pts',(-9.4452519771593,-12.3040048100576,
119.098440828438)) ;
#156920=CARTESIAN_POINT('Ctrl Pts',(-9.37144812888264,-12.3040048059064,
119.122671855331)) ;
#156921=CARTESIAN_POINT('Ctrl Pts',(-9.29764428060597,-12.3040048017553,
119.146902882224)) ;
#156922=CARTESIAN_POINT('Ctrl Pts',(-9.29090632432286,-12.3767667157857,
119.126380154863)) ;
#156923=CARTESIAN_POINT('Ctrl Pts',(-9.38394796937826,-12.4973266925111,
119.374354583408)) ;
#156924=CARTESIAN_POINT('Ctrl Pts',(-9.37143676374085,-12.5617762145597,
119.336247470161)) ;
#156925=CARTESIAN_POINT('Ctrl Pts',(-9.44524061342147,-12.5617762263117,
119.312016447545)) ;
#156926=CARTESIAN_POINT('Ctrl Pts',(-9.51904446310207,-12.5617762380637,
119.287785424927)) ;
#156927=CARTESIAN_POINT('Ctrl Pts',(-9.53155566873948,-12.497326716015,
119.325892538174)) ;
#156928=CARTESIAN_POINT('Ctrl Pts',(-9.54406687437688,-12.4328771939664,
119.36399965142)) ;
#156929=CARTESIAN_POINT('Ctrl Pts',(-9.47026302469627,-12.4328771822144,
119.388230674037)) ;
#156930=CARTESIAN_POINT('Ctrl Pts',(-9.39645917501566,-12.4328771704624,
119.412461696654)) ;
#156931=CARTESIAN_POINT('Ctrl Pts',(-9.38394796937826,-12.4973266925111,
119.374354583408)) ;
#156932=CARTESIAN_POINT('Ctrl Pts',(-9.4644362377349,-12.6849702880242,
119.583900943341)) ;
#156933=CARTESIAN_POINT('Ctrl Pts',(-9.4470238617794,-12.7364118506539,
119.530865656292)) ;
#156934=CARTESIAN_POINT('Ctrl Pts',(-9.52082771227271,-12.7364118743968,
119.506634636151)) ;
#156935=CARTESIAN_POINT('Ctrl Pts',(-9.59463156276601,-12.7364118981397,
119.482403616009)) ;
#156936=CARTESIAN_POINT('Ctrl Pts',(-9.61204393872151,-12.68497033551,119.535438903058)) ;
#156937=CARTESIAN_POINT('Ctrl Pts',(-9.62945631467699,-12.6335287728803,
119.588474190107)) ;
#156938=CARTESIAN_POINT('Ctrl Pts',(-9.5556524641837,-12.6335287491374,
119.612705210249)) ;
#156939=CARTESIAN_POINT('Ctrl Pts',(-9.48184861369038,-12.6335287253945,
119.63693623039)) ;
#156940=CARTESIAN_POINT('Ctrl Pts',(-9.4644362377349,-12.6849702880242,
119.583900943341)) ;
#156941=CARTESIAN_POINT('Ctrl Pts',(-9.5264642676195,-12.9239536141708,
119.737443599299)) ;
#156942=CARTESIAN_POINT('Ctrl Pts',(-9.50542818056897,-12.958783516276,
119.67337107309)) ;
#156943=CARTESIAN_POINT('Ctrl Pts',(-9.57923202992662,-12.9587835522301,
119.649140049489)) ;
#156944=CARTESIAN_POINT('Ctrl Pts',(-9.65303587928429,-12.9587835881843,
119.624909025889)) ;
#156945=CARTESIAN_POINT('Ctrl Pts',(-9.67407196633483,-12.9239536860792,
119.688981552098)) ;
#156946=CARTESIAN_POINT('Ctrl Pts',(-9.69510805338537,-12.889123783974,
119.753054078307)) ;
#156947=CARTESIAN_POINT('Ctrl Pts',(-9.6213042040277,-12.8891237480199,
119.777285101908)) ;
#156948=CARTESIAN_POINT('Ctrl Pts',(-9.54750035467004,-12.8891237120657,
119.801516125509)) ;
#156949=CARTESIAN_POINT('Ctrl Pts',(-9.5264642676195,-12.9239536141708,
119.737443599299)) ;
#156950=CARTESIAN_POINT('Ctrl Pts',(-9.56699499377198,-13.198264514804,
119.825482569648)) ;
#156951=CARTESIAN_POINT('Ctrl Pts',(-9.54383147105243,-13.2139924714054,
119.754930217809)) ;
#156952=CARTESIAN_POINT('Ctrl Pts',(-9.61763531776289,-13.2139925191053,
119.730699186145)) ;
#156953=CARTESIAN_POINT('Ctrl Pts',(-9.69143916447335,-13.2139925668051,
119.706468154482)) ;
#156954=CARTESIAN_POINT('Ctrl Pts',(-9.71460268719289,-13.1982646102037,
119.777020506321)) ;
#156955=CARTESIAN_POINT('Ctrl Pts',(-9.73776620991244,-13.1825366536022,
119.847572858159)) ;
#156956=CARTESIAN_POINT('Ctrl Pts',(-9.66396236320198,-13.1825366059024,
119.871803889823)) ;
#156957=CARTESIAN_POINT('Ctrl Pts',(-9.59015851649152,-13.1825365582025,
119.896034921487)) ;
#156958=CARTESIAN_POINT('Ctrl Pts',(-9.56699499377198,-13.198264514804,
119.825482569648)) ;
#156959=CARTESIAN_POINT('Ctrl Pts',(-9.58379794756891,-13.4887696764051,
119.841196258796)) ;
#156960=CARTESIAN_POINT('Ctrl Pts',(-9.56016164623923,-13.4842376804655,
119.769203899761)) ;
#156961=CARTESIAN_POINT('Ctrl Pts',(-9.63396548872277,-13.4842377379434,
119.744972855222)) ;
#156962=CARTESIAN_POINT('Ctrl Pts',(-9.70776933120628,-13.4842377954214,
119.720741810684)) ;
#156963=CARTESIAN_POINT('Ctrl Pts',(-9.73140563253596,-13.488769791361,
119.792734169719)) ;
#156964=CARTESIAN_POINT('Ctrl Pts',(-9.75504193386563,-13.4933017873006,
119.864726528754)) ;
#156965=CARTESIAN_POINT('Ctrl Pts',(-9.68123809138211,-13.4933017298226,
119.888957573292)) ;
#156966=CARTESIAN_POINT('Ctrl Pts',(-9.60743424889859,-13.4933016723446,
119.91318861783)) ;
#156967=CARTESIAN_POINT('Ctrl Pts',(-9.58379794756891,-13.4887696764051,
119.841196258796)) ;
#156968=CARTESIAN_POINT('Ctrl Pts',(-9.57628694483019,-13.7747050880232,
119.782787604556)) ;
#156969=CARTESIAN_POINT('Ctrl Pts',(-9.55387601395397,-13.7502030722453,
119.714527526385)) ;
#156970=CARTESIAN_POINT('Ctrl Pts',(-9.62767985077114,-13.7502031353853,
119.690296464588)) ;
#156971=CARTESIAN_POINT('Ctrl Pts',(-9.70148368758833,-13.7502031985253,
119.666065402791)) ;
#156972=CARTESIAN_POINT('Ctrl Pts',(-9.72389461846455,-13.7747052143032,
119.734325480963)) ;
#156973=CARTESIAN_POINT('Ctrl Pts',(-9.74630554934077,-13.7992072300811,
119.802585559134)) ;
#156974=CARTESIAN_POINT('Ctrl Pts',(-9.67250171252359,-13.7992071669411,
119.826816620931)) ;
#156975=CARTESIAN_POINT('Ctrl Pts',(-9.59869787570641,-13.7992071038011,
119.851047682728)) ;
#156976=CARTESIAN_POINT('Ctrl Pts',(-9.57628694483019,-13.7747050880232,
119.782787604556)) ;
#156977=CARTESIAN_POINT('Ctrl Pts',(-9.54578275574017,-14.0346989777519,
119.65439454944)) ;
#156978=CARTESIAN_POINT('Ctrl Pts',(-9.5262032717922,-13.9920093582588,
119.594758601917)) ;
#156979=CARTESIAN_POINT('Ctrl Pts',(-9.60000710216503,-13.9920094202152,
119.570527520491)) ;
#156980=CARTESIAN_POINT('Ctrl Pts',(-9.67381093253786,-13.9920094821717,
119.546296439066)) ;
#156981=CARTESIAN_POINT('Ctrl Pts',(-9.69339041648583,-14.0346991016648,
119.605932386589)) ;
#156982=CARTESIAN_POINT('Ctrl Pts',(-9.71296990043381,-14.077388721158,
119.665568334113)) ;
#156983=CARTESIAN_POINT('Ctrl Pts',(-9.63916607006098,-14.0773886592015,
119.689799415538)) ;
#156984=CARTESIAN_POINT('Ctrl Pts',(-9.56536223968815,-14.077388597245,
119.714030496963)) ;
#156985=CARTESIAN_POINT('Ctrl Pts',(-9.54578275574017,-14.0346989777519,
119.65439454944)) ;
#156986=CARTESIAN_POINT('Ctrl Pts',(-9.49516719411495,-14.2504823475427,
119.464718649369)) ;
#156987=CARTESIAN_POINT('Ctrl Pts',(-9.47982784694189,-14.1926653559339,
119.417997474467)) ;
#156988=CARTESIAN_POINT('Ctrl Pts',(-9.5536316707946,-14.192665409366,119.393766373183)) ;
#156989=CARTESIAN_POINT('Ctrl Pts',(-9.62743549464732,-14.1926654627981,
119.369535271898)) ;
#156990=CARTESIAN_POINT('Ctrl Pts',(-9.64277484182037,-14.2504824544068,
119.4162564468)) ;
#156991=CARTESIAN_POINT('Ctrl Pts',(-9.65811418899341,-14.3082994460156,
119.462977621703)) ;
#156992=CARTESIAN_POINT('Ctrl Pts',(-9.58431036514069,-14.3082993925835,
119.487208722987)) ;
#156993=CARTESIAN_POINT('Ctrl Pts',(-9.51050654128798,-14.3082993391515,
119.511439824272)) ;
#156994=CARTESIAN_POINT('Ctrl Pts',(-9.49516719411495,-14.2504823475427,
119.464718649369)) ;
#156995=CARTESIAN_POINT('Ctrl Pts',(-9.42925750378619,-14.4061007577842,
119.228637274552)) ;
#156996=CARTESIAN_POINT('Ctrl Pts',(-9.41922861107984,-14.3373352952271,
119.198090887228)) ;
#156997=CARTESIAN_POINT('Ctrl Pts',(-9.49303242959301,-14.3373353326338,
119.17385976968)) ;
#156998=CARTESIAN_POINT('Ctrl Pts',(-9.56683624810616,-14.3373353700405,
119.149628652132)) ;
#156999=CARTESIAN_POINT('Ctrl Pts',(-9.57686514081249,-14.4061008325976,
119.180175039457)) ;
#157000=CARTESIAN_POINT('Ctrl Pts',(-9.58689403351884,-14.4748662951547,
119.210721426781)) ;
#157001=CARTESIAN_POINT('Ctrl Pts',(-9.51309021500568,-14.474866257748,
119.234952544329)) ;
#157002=CARTESIAN_POINT('Ctrl Pts',(-9.43928639649253,-14.4748662203413,
119.259183661877)) ;
#157003=CARTESIAN_POINT('Ctrl Pts',(-9.42925750378619,-14.4061007577842,
119.228637274552)) ;
#157004=CARTESIAN_POINT('Ctrl Pts',(-9.35244000585146,-14.4917978275685,
118.958975475398)) ;
#157005=CARTESIAN_POINT('Ctrl Pts',(-9.34849792368344,-14.4169485235802,
118.946968531011)) ;
#157006=CARTESIAN_POINT('Ctrl Pts',(-9.42230173775408,-14.4169485394119,
118.922737399932)) ;
#157007=CARTESIAN_POINT('Ctrl Pts',(-9.49610555182472,-14.4169485552436,
118.898506268853)) ;
#157008=CARTESIAN_POINT('Ctrl Pts',(-9.50004763399274,-14.4917978592319,
118.91051321324)) ;
#157009=CARTESIAN_POINT('Ctrl Pts',(-9.50398971616077,-14.5666471632202,
118.922520157628)) ;
#157010=CARTESIAN_POINT('Ctrl Pts',(-9.43018590209014,-14.5666471473885,
118.946751288707)) ;
#157011=CARTESIAN_POINT('Ctrl Pts',(-9.35638208801949,-14.5666471315568,
118.970982419786)) ;
#157012=CARTESIAN_POINT('Ctrl Pts',(-9.35244000585146,-14.4917978275685,
118.958975475398)) ;
#157013=CARTESIAN_POINT('Ctrl Pts',(-9.27254720983972,-14.4998539330622,
118.680348428381)) ;
#157014=CARTESIAN_POINT('Ctrl Pts',(-9.27490739751976,-14.4243333592347,
118.687537181156)) ;
#157015=CARTESIAN_POINT('Ctrl Pts',(-9.34871121015168,-14.4243333490761,
118.663306045695)) ;
#157016=CARTESIAN_POINT('Ctrl Pts',(-9.42251502278361,-14.4243333389175,
118.639074910234)) ;
#157017=CARTESIAN_POINT('Ctrl Pts',(-9.42015483510357,-14.4998539127449,
118.631886157459)) ;
#157018=CARTESIAN_POINT('Ctrl Pts',(-9.41779464742353,-14.5753744865724,
118.624697404683)) ;
#157019=CARTESIAN_POINT('Ctrl Pts',(-9.3439908347916,-14.575374496731,118.648928540144)) ;
#157020=CARTESIAN_POINT('Ctrl Pts',(-9.27018702215968,-14.5753745068897,
118.673159675605)) ;
#157021=CARTESIAN_POINT('Ctrl Pts',(-9.27254720983972,-14.4998539330622,
118.680348428381)) ;
#157022=CARTESIAN_POINT('Ctrl Pts',(-9.19483422021103,-14.4309092256038,
118.408185227294)) ;
#157023=CARTESIAN_POINT('Ctrl Pts',(-9.20335723096026,-14.3600915226302,
118.434144944847)) ;
#157024=CARTESIAN_POINT('Ctrl Pts',(-9.27716104438173,-14.3600914852358,
118.409913811791)) ;
#157025=CARTESIAN_POINT('Ctrl Pts',(-9.35096485780319,-14.3600914478414,
118.385682678734)) ;
#157026=CARTESIAN_POINT('Ctrl Pts',(-9.34244184705396,-14.430909150815,
118.359722961181)) ;
#157027=CARTESIAN_POINT('Ctrl Pts',(-9.33391883630474,-14.5017268537886,
118.333763243628)) ;
#157028=CARTESIAN_POINT('Ctrl Pts',(-9.26011502288327,-14.501726891183,
118.357994376684)) ;
#157029=CARTESIAN_POINT('Ctrl Pts',(-9.1863112094618,-14.5017269285774,
118.38222550974)) ;
#157030=CARTESIAN_POINT('Ctrl Pts',(-9.19483422021103,-14.4309092256038,
118.408185227294)) ;
#157031=CARTESIAN_POINT('Ctrl Pts',(-9.12600873086239,-14.2894596882656,
118.163115988674)) ;
#157032=CARTESIAN_POINT('Ctrl Pts',(-9.14008263562817,-14.2284134835687,
118.205982833824)) ;
#157033=CARTESIAN_POINT('Ctrl Pts',(-9.21388645251701,-14.2284134202247,
118.181751711328)) ;
#157034=CARTESIAN_POINT('Ctrl Pts',(-9.28769026940583,-14.2284133568807,
118.157520588833)) ;
#157035=CARTESIAN_POINT('Ctrl Pts',(-9.27361636464005,-14.2894595615776,
118.114653743684)) ;
#157036=CARTESIAN_POINT('Ctrl Pts',(-9.25954245987426,-14.3505057662746,
118.071786898535)) ;
#157037=CARTESIAN_POINT('Ctrl Pts',(-9.18573864298543,-14.3505058296186,
118.09601802103)) ;
#157038=CARTESIAN_POINT('Ctrl Pts',(-9.1119348260966,-14.3505058929625,
118.120249143525)) ;
#157039=CARTESIAN_POINT('Ctrl Pts',(-9.12600873086239,-14.2894596882656,
118.163115988674)) ;
#157040=CARTESIAN_POINT('Ctrl Pts',(-9.07154849099475,-14.0846391379262,
117.961648450783)) ;
#157041=CARTESIAN_POINT('Ctrl Pts',(-9.09018180458957,-14.0378023203219,
118.018402519606)) ;
#157042=CARTESIAN_POINT('Ctrl Pts',(-9.16398562735108,-14.0378022350358,
117.994171414998)) ;
#157043=CARTESIAN_POINT('Ctrl Pts',(-9.23778945011258,-14.0378021497496,
117.96994031039)) ;
#157044=CARTESIAN_POINT('Ctrl Pts',(-9.21915613651776,-14.0846389673539,
117.913186241567)) ;
#157045=CARTESIAN_POINT('Ctrl Pts',(-9.20052282292294,-14.1314757849582,
117.856432172745)) ;
#157046=CARTESIAN_POINT('Ctrl Pts',(-9.12671900016143,-14.1314758702443,
117.880663277353)) ;
#157047=CARTESIAN_POINT('Ctrl Pts',(-9.05291517739992,-14.1314759555304,
117.904894381961)) ;
#157048=CARTESIAN_POINT('Ctrl Pts',(-9.07154849099475,-14.0846391379262,
117.961648450783)) ;
#157049=CARTESIAN_POINT('Ctrl Pts',(-9.036633988908,-13.833584389583,117.819961399887)) ;
#157050=CARTESIAN_POINT('Ctrl Pts',(-9.05846369099851,-13.8042063937381,
117.88645115234)) ;
#157051=CARTESIAN_POINT('Ctrl Pts',(-9.13226752150254,-13.8042062935713,
117.862220071314)) ;
#157052=CARTESIAN_POINT('Ctrl Pts',(-9.20607135200658,-13.8042061934045,
117.837988990289)) ;
#157053=CARTESIAN_POINT('Ctrl Pts',(-9.18424164991607,-13.8335841892493,
117.771499237836)) ;
#157054=CARTESIAN_POINT('Ctrl Pts',(-9.16241194782554,-13.8629621850941,
117.705009485383)) ;
#157055=CARTESIAN_POINT('Ctrl Pts',(-9.08860811732153,-13.862962285261,
117.729240566409)) ;
#157056=CARTESIAN_POINT('Ctrl Pts',(-9.01480428681749,-13.8629623854278,
117.753471647434)) ;
#157057=CARTESIAN_POINT('Ctrl Pts',(-9.036633988908,-13.833584389583,117.819961399887)) ;
#157058=CARTESIAN_POINT('Ctrl Pts',(-9.02391466502751,-13.5522887119168,
117.745782719323)) ;
#157059=CARTESIAN_POINT('Ctrl Pts',(-9.04739797225372,-13.5425061564868,
117.817309086205)) ;
#157060=CARTESIAN_POINT('Ctrl Pts',(-9.1212018115543,-13.542506049205,117.793078031972)) ;
#157061=CARTESIAN_POINT('Ctrl Pts',(-9.19500565085488,-13.5425059419231,
117.768846977739)) ;
#157062=CARTESIAN_POINT('Ctrl Pts',(-9.17152234362867,-13.5522884973531,
117.697320610857)) ;
#157063=CARTESIAN_POINT('Ctrl Pts',(-9.14803903640246,-13.5620710527831,
117.625794243975)) ;
#157064=CARTESIAN_POINT('Ctrl Pts',(-9.07423519710187,-13.5620711600649,
117.650025298208)) ;
#157065=CARTESIAN_POINT('Ctrl Pts',(-9.0004313578013,-13.5620712673468,
117.67425635244)) ;
#157066=CARTESIAN_POINT('Ctrl Pts',(-9.02391466502751,-13.5522887119168,
117.745782719323)) ;
#157067=CARTESIAN_POINT('Ctrl Pts',(-9.03557274648368,-13.2592972529684,
117.745601612871)) ;
#157068=CARTESIAN_POINT('Ctrl Pts',(-9.05901578034276,-13.2699555383047,
117.817005313531)) ;
#157069=CARTESIAN_POINT('Ctrl Pts',(-9.13281962864124,-13.2699554336479,
117.792774286704)) ;
#157070=CARTESIAN_POINT('Ctrl Pts',(-9.20662347693971,-13.2699553289911,
117.768543259878)) ;
#157071=CARTESIAN_POINT('Ctrl Pts',(-9.18318044308064,-13.2592970436547,
117.697139559218)) ;
#157072=CARTESIAN_POINT('Ctrl Pts',(-9.15973740922156,-13.2486387583184,
117.625735858557)) ;
#157073=CARTESIAN_POINT('Ctrl Pts',(-9.08593356092309,-13.2486388629752,
117.649966885384)) ;
#157074=CARTESIAN_POINT('Ctrl Pts',(-9.0121297126246,-13.248638967632,117.67419791221)) ;
#157075=CARTESIAN_POINT('Ctrl Pts',(-9.03557274648368,-13.2592972529684,
117.745601612871)) ;
#157076=CARTESIAN_POINT('Ctrl Pts',(-9.07098090557538,-12.9811038250668,
117.818197097558)) ;
#157077=CARTESIAN_POINT('Ctrl Pts',(-9.09271605071885,-13.0112007681919,
117.884398844714)) ;
#157078=CARTESIAN_POINT('Ctrl Pts',(-9.166519907195,-13.0112006734562,117.860167842795)) ;
#157079=CARTESIAN_POINT('Ctrl Pts',(-9.24032376367114,-13.0112005787204,
117.835936840877)) ;
#157080=CARTESIAN_POINT('Ctrl Pts',(-9.21858861852767,-12.9811036355953,
117.76973509372)) ;
#157081=CARTESIAN_POINT('Ctrl Pts',(-9.19685347338419,-12.9510066924703,
117.703533346564)) ;
#157082=CARTESIAN_POINT('Ctrl Pts',(-9.12304961690805,-12.951006787206,
117.727764348482)) ;
#157083=CARTESIAN_POINT('Ctrl Pts',(-9.0492457604319,-12.9510068819417,
117.751995350401)) ;
#157084=CARTESIAN_POINT('Ctrl Pts',(-9.07098090557538,-12.9811038250668,
117.818197097558)) ;
#157085=CARTESIAN_POINT('Ctrl Pts',(-9.1288816653457,-12.7319954339599,
117.959013661815)) ;
#157086=CARTESIAN_POINT('Ctrl Pts',(-9.14734233324813,-12.7795294847017,
118.015241879551)) ;
#157087=CARTESIAN_POINT('Ctrl Pts',(-9.22114619632656,-12.7795294077386,
117.991010897742)) ;
#157088=CARTESIAN_POINT('Ctrl Pts',(-9.29495005940499,-12.7795293307755,
117.966779915932)) ;
#157089=CARTESIAN_POINT('Ctrl Pts',(-9.27648939150257,-12.7319952800337,
117.910551698197)) ;
#157090=CARTESIAN_POINT('Ctrl Pts',(-9.25802872360013,-12.6844612292919,
117.854323480461)) ;
#157091=CARTESIAN_POINT('Ctrl Pts',(-9.1842248605217,-12.684461306255,117.87855446227)) ;
#157092=CARTESIAN_POINT('Ctrl Pts',(-9.11042099744327,-12.6844613832181,
117.902785444079)) ;
#157093=CARTESIAN_POINT('Ctrl Pts',(-9.1288816653457,-12.7319954339599,
117.959013661815)) ;
#157094=CARTESIAN_POINT('Ctrl Pts',(-9.20542108821079,-12.5329045763516,
118.156747660811)) ;
#157095=CARTESIAN_POINT('Ctrl Pts',(-9.21929794557474,-12.5944099452727,
118.199014331155)) ;
#157096=CARTESIAN_POINT('Ctrl Pts',(-9.2931018131911,-12.5944098904592,
118.174783363168)) ;
#157097=CARTESIAN_POINT('Ctrl Pts',(-9.36690568080745,-12.5944098356456,
118.15055239518)) ;
#157098=CARTESIAN_POINT('Ctrl Pts',(-9.3530288234435,-12.5329044667245,
118.108285724836)) ;
#157099=CARTESIAN_POINT('Ctrl Pts',(-9.33915196607953,-12.4713990978033,
118.066019054492)) ;
#157100=CARTESIAN_POINT('Ctrl Pts',(-9.26534809846318,-12.4713991526168,
118.090250022479)) ;
#157101=CARTESIAN_POINT('Ctrl Pts',(-9.19154423084681,-12.4713992074304,
118.114480990467)) ;
#157102=CARTESIAN_POINT('Ctrl Pts',(-9.20542108821079,-12.5329045763516,
118.156747660811)) ;
#157103=CARTESIAN_POINT('Ctrl Pts',(-9.2965722776736,-12.3964115152595,
118.398783809131)) ;
#157104=CARTESIAN_POINT('Ctrl Pts',(-9.30484266398313,-12.467539433598,
118.423974073115)) ;
#157105=CARTESIAN_POINT('Ctrl Pts',(-9.37864653333808,-12.4675394037743,
118.399743110423)) ;
#157106=CARTESIAN_POINT('Ctrl Pts',(-9.45245040269302,-12.4675393739507,
118.375512147731)) ;
#157107=CARTESIAN_POINT('Ctrl Pts',(-9.44418001638348,-12.3964114556122,
118.350321883747)) ;
#157108=CARTESIAN_POINT('Ctrl Pts',(-9.43590963007394,-12.3252835372738,
118.325131619762)) ;
#157109=CARTESIAN_POINT('Ctrl Pts',(-9.36210576071901,-12.3252835670974,
118.349362582454)) ;
#157110=CARTESIAN_POINT('Ctrl Pts',(-9.28830189136406,-12.3252835969211,
118.373593545146)) ;
#157111=CARTESIAN_POINT('Ctrl Pts',(-9.2965722776736,-12.3964115152595,
118.398783809131)) ;
#157112=CARTESIAN_POINT('Ctrl Pts',(-9.39560158322444,-12.3338312624075,
118.665015098447)) ;
#157113=CARTESIAN_POINT('Ctrl Pts',(-9.39770272998261,-12.4094356003857,
118.671414854041)) ;
#157114=CARTESIAN_POINT('Ctrl Pts',(-9.47150659893981,-12.409435594184,
118.647183890138)) ;
#157115=CARTESIAN_POINT('Ctrl Pts',(-9.54531046789698,-12.4094355879822,
118.622952926234)) ;
#157116=CARTESIAN_POINT('Ctrl Pts',(-9.54320932113881,-12.333831250004,
118.61655317064)) ;
#157117=CARTESIAN_POINT('Ctrl Pts',(-9.54110817438061,-12.2582269120257,
118.610153415045)) ;
#157118=CARTESIAN_POINT('Ctrl Pts',(-9.46730430542344,-12.2582269182275,
118.634384378949)) ;
#157119=CARTESIAN_POINT('Ctrl Pts',(-9.39350043646624,-12.2582269244292,
118.658615342853)) ;
#157120=CARTESIAN_POINT('Ctrl Pts',(-9.39560158322444,-12.3338312624075,
118.665015098447)) ;
#157121=CARTESIAN_POINT('Ctrl Pts',(-9.4968318946719,-12.3486707517994,
118.937874104534)) ;
#157122=CARTESIAN_POINT('Ctrl Pts',(-9.49260239676129,-12.4233532981751,
118.92499173777)) ;
#157123=CARTESIAN_POINT('Ctrl Pts',(-9.56640626305169,-12.4233533125853,
118.900760765744)) ;
#157124=CARTESIAN_POINT('Ctrl Pts',(-9.64021012934211,-12.4233533269956,
118.876529793718)) ;
#157125=CARTESIAN_POINT('Ctrl Pts',(-9.64443962725272,-12.3486707806198,
118.889412160482)) ;
#157126=CARTESIAN_POINT('Ctrl Pts',(-9.64866912516332,-12.2739882342441,
118.902294527246)) ;
#157127=CARTESIAN_POINT('Ctrl Pts',(-9.5748652588729,-12.2739882198339,
118.926525499272)) ;
#157128=CARTESIAN_POINT('Ctrl Pts',(-9.5010613925825,-12.2739882054237,
118.950756471299)) ;
#157129=CARTESIAN_POINT('Ctrl Pts',(-9.4968318946719,-12.3486707517994,
118.937874104534)) ;
#157130=CARTESIAN_POINT('Ctrl Pts',(-9.59343723857601,-12.4397941697449,
119.196716726627)) ;
#157131=CARTESIAN_POINT('Ctrl Pts',(-9.58318893999786,-12.5082273902753,
119.165502064017)) ;
#157132=CARTESIAN_POINT('Ctrl Pts',(-9.65699280218564,-12.5082274205257,
119.141271079495)) ;
#157133=CARTESIAN_POINT('Ctrl Pts',(-9.73079666437343,-12.508227450776,
119.117040094973)) ;
#157134=CARTESIAN_POINT('Ctrl Pts',(-9.74104496295157,-12.4397942302456,
119.148254757583)) ;
#157135=CARTESIAN_POINT('Ctrl Pts',(-9.75129326152971,-12.3713610097152,
119.179469420192)) ;
#157136=CARTESIAN_POINT('Ctrl Pts',(-9.67748939934194,-12.3713609794648,
119.203700404715)) ;
#157137=CARTESIAN_POINT('Ctrl Pts',(-9.60368553715415,-12.3713609492144,
119.227931389237)) ;
#157138=CARTESIAN_POINT('Ctrl Pts',(-9.59343723857601,-12.4397941697449,
119.196716726627)) ;
#157139=CARTESIAN_POINT('Ctrl Pts',(-9.67989153670841,-12.6021170084136,
119.424415022172)) ;
#157140=CARTESIAN_POINT('Ctrl Pts',(-9.66432856763324,-12.6593209317561,
119.377012730555)) ;
#157141=CARTESIAN_POINT('Ctrl Pts',(-9.73813242432927,-12.6593209703252,
119.352781729306)) ;
#157142=CARTESIAN_POINT('Ctrl Pts',(-9.81193628102528,-12.6593210088944,
119.328550728057)) ;
#157143=CARTESIAN_POINT('Ctrl Pts',(-9.82749925010046,-12.6021170855519,
119.375953019674)) ;
#157144=CARTESIAN_POINT('Ctrl Pts',(-9.84306221917561,-12.5449131622094,
119.423355311291)) ;
#157145=CARTESIAN_POINT('Ctrl Pts',(-9.7692583624796,-12.5449131236403,
119.44758631254)) ;
#157146=CARTESIAN_POINT('Ctrl Pts',(-9.69545450578357,-12.5449130850712,
119.47181731379)) ;
#157147=CARTESIAN_POINT('Ctrl Pts',(-9.67989153670841,-12.6021170084136,
119.424415022172)) ;
#157148=CARTESIAN_POINT('Ctrl Pts',(-9.74951237514481,-12.8208593941247,
119.601209318802)) ;
#157149=CARTESIAN_POINT('Ctrl Pts',(-9.7297945436342,-12.862876765698,119.541151986463)) ;
#157150=CARTESIAN_POINT('Ctrl Pts',(-9.80359839554776,-12.8628768085356,
119.516920970647)) ;
#157151=CARTESIAN_POINT('Ctrl Pts',(-9.87740224746131,-12.8628768513732,
119.492689954831)) ;
#157152=CARTESIAN_POINT('Ctrl Pts',(-9.89712007897192,-12.8208594798,119.552747287171)) ;
#157153=CARTESIAN_POINT('Ctrl Pts',(-9.91683791048251,-12.7788421082267,
119.61280461951)) ;
#157154=CARTESIAN_POINT('Ctrl Pts',(-9.84303405856896,-12.7788420653891,
119.637035635326)) ;
#157155=CARTESIAN_POINT('Ctrl Pts',(-9.76923020665541,-12.7788420225515,
119.661266651141)) ;
#157156=CARTESIAN_POINT('Ctrl Pts',(-9.74951237514481,-12.8208593941247,
119.601209318802)) ;
#157157=CARTESIAN_POINT('Ctrl Pts',(-9.79944954754396,-13.084370773037,
119.717716848365)) ;
#157158=CARTESIAN_POINT('Ctrl Pts',(-9.77695151881111,-13.1080532494665,
119.649191483677)) ;
#157159=CARTESIAN_POINT('Ctrl Pts',(-9.85075536585704,-13.1080532886094,
119.624960453035)) ;
#157160=CARTESIAN_POINT('Ctrl Pts',(-9.92455921290298,-13.1080533277524,
119.600729422393)) ;
#157161=CARTESIAN_POINT('Ctrl Pts',(-9.94705724163583,-13.0843708513228,
119.669254787081)) ;
#157162=CARTESIAN_POINT('Ctrl Pts',(-9.96955527036869,-13.0606883748933,
119.737780151769)) ;
#157163=CARTESIAN_POINT('Ctrl Pts',(-9.89575142332274,-13.0606883357504,
119.762011182411)) ;
#157164=CARTESIAN_POINT('Ctrl Pts',(-9.82194757627682,-13.0606882966075,
119.786242213053)) ;
#157165=CARTESIAN_POINT('Ctrl Pts',(-9.79944954754396,-13.084370773037,
119.717716848365)) ;
#157166=CARTESIAN_POINT('Ctrl Pts',(-9.82597149657916,-13.3711928765175,
119.763016540292)) ;
#157167=CARTESIAN_POINT('Ctrl Pts',(-9.80232171969241,-13.3748845002412,
119.690983136391)) ;
#157168=CARTESIAN_POINT('Ctrl Pts',(-9.87612556329562,-13.3748845322642,
119.666752095263)) ;
#157169=CARTESIAN_POINT('Ctrl Pts',(-9.94992940689882,-13.3748845642871,
119.642521054136)) ;
#157170=CARTESIAN_POINT('Ctrl Pts',(-9.97357918378556,-13.3711929405634,
119.714554458036)) ;
#157171=CARTESIAN_POINT('Ctrl Pts',(-9.99722896067229,-13.3675013168397,
119.786587861936)) ;
#157172=CARTESIAN_POINT('Ctrl Pts',(-9.92342511706909,-13.3675012848167,
119.810818903064)) ;
#157173=CARTESIAN_POINT('Ctrl Pts',(-9.84962127346588,-13.3675012527938,
119.835049944192)) ;
#157174=CARTESIAN_POINT('Ctrl Pts',(-9.82597149657916,-13.3711928765175,
119.763016540292)) ;
#157175=CARTESIAN_POINT('Ctrl Pts',(-9.82819214417096,-13.6609866789311,
119.734331572361)) ;
#157176=CARTESIAN_POINT('Ctrl Pts',(-9.80508506706182,-13.644449399206,
119.663951144264)) ;
#157177=CARTESIAN_POINT('Ctrl Pts',(-9.87888890860554,-13.6444494224757,
119.639720096863)) ;
#157178=CARTESIAN_POINT('Ctrl Pts',(-9.95269275014925,-13.6444494457453,
119.615489049462)) ;
#157179=CARTESIAN_POINT('Ctrl Pts',(-9.97579982725838,-13.6609867254704,
119.68586947756)) ;
#157180=CARTESIAN_POINT('Ctrl Pts',(-9.99890690436752,-13.6775240051955,
119.756249905657)) ;
#157181=CARTESIAN_POINT('Ctrl Pts',(-9.9251030628238,-13.6775239819258,
119.780480953058)) ;
#157182=CARTESIAN_POINT('Ctrl Pts',(-9.85129922128009,-13.6775239586562,
119.804712000459)) ;
#157183=CARTESIAN_POINT('Ctrl Pts',(-9.82819214417096,-13.6609866789311,
119.734331572361)) ;
#157184=CARTESIAN_POINT('Ctrl Pts',(-9.8068991329201,-13.9327616913683,
119.63413267067)) ;
#157185=CARTESIAN_POINT('Ctrl Pts',(-9.785975348665,-13.8972231314794,119.570402200203)) ;
#157186=CARTESIAN_POINT('Ctrl Pts',(-9.85977918932944,-13.8972231463685,
119.546171150125)) ;
#157187=CARTESIAN_POINT('Ctrl Pts',(-9.9335830299939,-13.8972231612576,
119.521940100046)) ;
#157188=CARTESIAN_POINT('Ctrl Pts',(-9.954506814249,-13.9327617211465,119.585670570512)) ;
#157189=CARTESIAN_POINT('Ctrl Pts',(-9.9754305985041,-13.9683002810353,
119.649401040979)) ;
#157190=CARTESIAN_POINT('Ctrl Pts',(-9.90162675783965,-13.9683002661462,
119.673632091058)) ;
#157191=CARTESIAN_POINT('Ctrl Pts',(-9.8278229171752,-13.9683002512571,
119.697863141137)) ;
#157192=CARTESIAN_POINT('Ctrl Pts',(-9.8068991329201,-13.9327616913683,
119.63413267067)) ;
#157193=CARTESIAN_POINT('Ctrl Pts',(-9.76382464831486,-14.1696775509721,
119.467276311035)) ;
#157194=CARTESIAN_POINT('Ctrl Pts',(-9.74661479432104,-14.117542024341,
119.414857872744)) ;
#157195=CARTESIAN_POINT('Ctrl Pts',(-9.82041863565303,-14.1175420304562,
119.390626824698)) ;
#157196=CARTESIAN_POINT('Ctrl Pts',(-9.89422247698502,-14.1175420365713,
119.366395776653)) ;
#157197=CARTESIAN_POINT('Ctrl Pts',(-9.91143233097885,-14.1696775632024,
119.418814214944)) ;
#157198=CARTESIAN_POINT('Ctrl Pts',(-9.92864218497269,-14.2218130898334,
119.471232653236)) ;
#157199=CARTESIAN_POINT('Ctrl Pts',(-9.85483834364069,-14.2218130837183,
119.495463701281)) ;
#157200=CARTESIAN_POINT('Ctrl Pts',(-9.7810345023087,-14.2218130776032,
119.519694749327)) ;
#157201=CARTESIAN_POINT('Ctrl Pts',(-9.76382464831486,-14.1696775509721,
119.467276311035)) ;
#157202=CARTESIAN_POINT('Ctrl Pts',(-9.7036673139555,-14.3505522399701,
119.248758719857)) ;
#157203=CARTESIAN_POINT('Ctrl Pts',(-9.69136245748043,-14.2857090044566,
119.211280112503)) ;
#157204=CARTESIAN_POINT('Ctrl Pts',(-9.76516629961979,-14.2857090064648,
119.187049066917)) ;
#157205=CARTESIAN_POINT('Ctrl Pts',(-9.83897014175914,-14.285709008473,
119.16281802133)) ;
#157206=CARTESIAN_POINT('Ctrl Pts',(-9.8512749982342,-14.3505522439865,
119.200296628684)) ;
#157207=CARTESIAN_POINT('Ctrl Pts',(-9.86357985470927,-14.4153954795,119.237775236038)) ;
#157208=CARTESIAN_POINT('Ctrl Pts',(-9.78977601256991,-14.4153954774918,
119.262006281625)) ;
#157209=CARTESIAN_POINT('Ctrl Pts',(-9.71597217043056,-14.4153954754836,
119.286237327211)) ;
#157210=CARTESIAN_POINT('Ctrl Pts',(-9.7036673139555,-14.3505522399701,
119.248758719857)) ;
#157211=CARTESIAN_POINT('Ctrl Pts',(-9.63071094051081,-14.4659895814683,
118.991045032151)) ;
#157212=CARTESIAN_POINT('Ctrl Pts',(-9.62421662360605,-14.39298831287,118.97126439071)) ;
#157213=CARTESIAN_POINT('Ctrl Pts',(-9.69802046703066,-14.392988312459,
118.947033349038)) ;
#157214=CARTESIAN_POINT('Ctrl Pts',(-9.77182431045527,-14.3929883120481,
118.922802307366)) ;
#157215=CARTESIAN_POINT('Ctrl Pts',(-9.77831862736004,-14.4659895806463,
118.942582948807)) ;
#157216=CARTESIAN_POINT('Ctrl Pts',(-9.78481294426479,-14.5389908492445,
118.962363590248)) ;
#157217=CARTESIAN_POINT('Ctrl Pts',(-9.71100910084019,-14.5389908496555,
118.98659463192)) ;
#157218=CARTESIAN_POINT('Ctrl Pts',(-9.63720525741557,-14.5389908500665,
119.010825673591)) ;
#157219=CARTESIAN_POINT('Ctrl Pts',(-9.63071094051081,-14.4659895814683,
118.991045032151)) ;
#157220=CARTESIAN_POINT('Ctrl Pts',(-9.55101925277455,-14.5060552317741,
118.712756531787)) ;
#157221=CARTESIAN_POINT('Ctrl Pts',(-9.55081597857438,-14.4301469447621,
118.712137391313)) ;
#157222=CARTESIAN_POINT('Ctrl Pts',(-9.62461982292271,-14.4301469446393,
118.687906352455)) ;
#157223=CARTESIAN_POINT('Ctrl Pts',(-9.69842366727105,-14.4301469445164,
118.663675313597)) ;
#157224=CARTESIAN_POINT('Ctrl Pts',(-9.69862694147122,-14.5060552315285,
118.66429445407)) ;
#157225=CARTESIAN_POINT('Ctrl Pts',(-9.69883021567139,-14.5819635185405,
118.664913594544)) ;
#157226=CARTESIAN_POINT('Ctrl Pts',(-9.62502637132304,-14.5819635186633,
118.689144633402)) ;
#157227=CARTESIAN_POINT('Ctrl Pts',(-9.55122252697472,-14.5819635187861,
118.713375672261)) ;
#157228=CARTESIAN_POINT('Ctrl Pts',(-9.55101925277455,-14.5060552317741,
118.712756531787)) ;
#157229=CARTESIAN_POINT('Ctrl Pts',(-9.4714813916173,-14.4677867862301,
118.435025022222)) ;
#157230=CARTESIAN_POINT('Ctrl Pts',(-9.47756606505661,-14.3944382757636,
118.453557955699)) ;
#157231=CARTESIAN_POINT('Ctrl Pts',(-9.55136990941469,-14.3944382766233,
118.42932691687)) ;
#157232=CARTESIAN_POINT('Ctrl Pts',(-9.62517375377276,-14.3944382774829,
118.405095878042)) ;
#157233=CARTESIAN_POINT('Ctrl Pts',(-9.61908908033345,-14.4677867879495,
118.386562944565)) ;
#157234=CARTESIAN_POINT('Ctrl Pts',(-9.61300440689413,-14.541135298416,
118.368030011088)) ;
#157235=CARTESIAN_POINT('Ctrl Pts',(-9.53920056253606,-14.5411352975563,
118.392261049916)) ;
#157236=CARTESIAN_POINT('Ctrl Pts',(-9.46539671817799,-14.5411352966967,
118.416492088745)) ;
#157237=CARTESIAN_POINT('Ctrl Pts',(-9.4714813916173,-14.4677867862301,
118.435025022222)) ;
#157238=CARTESIAN_POINT('Ctrl Pts',(-9.39862983053746,-14.3553856703914,
118.177844077314)) ;
#157239=CARTESIAN_POINT('Ctrl Pts',(-9.41054063802838,-14.2897781146532,
118.214122475092)) ;
#157240=CARTESIAN_POINT('Ctrl Pts',(-9.4843444819206,-14.2897781158864,
118.189891434844)) ;
#157241=CARTESIAN_POINT('Ctrl Pts',(-9.55814832581283,-14.2897781171196,
118.165660394597)) ;
#157242=CARTESIAN_POINT('Ctrl Pts',(-9.54623751832192,-14.3553856728579,
118.129381996819)) ;
#157243=CARTESIAN_POINT('Ctrl Pts',(-9.534326710831,-14.4209932285961,118.093103599041)) ;
#157244=CARTESIAN_POINT('Ctrl Pts',(-9.46052286693878,-14.4209932273629,
118.117334639289)) ;
#157245=CARTESIAN_POINT('Ctrl Pts',(-9.38671902304655,-14.4209932261297,
118.141565679537)) ;
#157246=CARTESIAN_POINT('Ctrl Pts',(-9.39862983053746,-14.3553856703914,
118.177844077314)) ;
#157247=CARTESIAN_POINT('Ctrl Pts',(-9.33739442485482,-14.1738642018268,
117.955618487218)) ;
#157248=CARTESIAN_POINT('Ctrl Pts',(-9.3543378978728,-14.1208352191847,
118.007225572262)) ;
#157249=CARTESIAN_POINT('Ctrl Pts',(-9.42814174061825,-14.1208352175881,
117.982994528522)) ;
#157250=CARTESIAN_POINT('Ctrl Pts',(-9.50194558336371,-14.1208352159916,
117.958763484782)) ;
#157251=CARTESIAN_POINT('Ctrl Pts',(-9.48500211034573,-14.1738641986337,
117.907156399737)) ;
#157252=CARTESIAN_POINT('Ctrl Pts',(-9.46805863732774,-14.2268931812759,
117.855549314692)) ;
#157253=CARTESIAN_POINT('Ctrl Pts',(-9.39425479458228,-14.2268931828724,
117.879780358433)) ;
#157254=CARTESIAN_POINT('Ctrl Pts',(-9.32045095183683,-14.226893184469,
117.904011402173)) ;
#157255=CARTESIAN_POINT('Ctrl Pts',(-9.33739442485482,-14.1738642018268,
117.955618487218)) ;
#157256=CARTESIAN_POINT('Ctrl Pts',(-9.29429158603599,-13.9401973275635,
117.789022041494)) ;
#157257=CARTESIAN_POINT('Ctrl Pts',(-9.31500003079175,-13.9034069013251,
117.852096623063)) ;
#157258=CARTESIAN_POINT('Ctrl Pts',(-9.38880387300515,-13.9034068952956,
117.827865577702)) ;
#157259=CARTESIAN_POINT('Ctrl Pts',(-9.46260771521854,-13.903406889266,
117.803634532341)) ;
#157260=CARTESIAN_POINT('Ctrl Pts',(-9.44189927046278,-13.9401973155044,
117.740559950772)) ;
#157261=CARTESIAN_POINT('Ctrl Pts',(-9.42119082570701,-13.9769877417428,
117.677485369204)) ;
#157262=CARTESIAN_POINT('Ctrl Pts',(-9.34738698349362,-13.9769877477723,
117.701716414565)) ;
#157263=CARTESIAN_POINT('Ctrl Pts',(-9.27358314128022,-13.9769877538019,
117.725947459926)) ;
#157264=CARTESIAN_POINT('Ctrl Pts',(-9.29429158603599,-13.9401973275635,
117.789022041494)) ;
#157265=CARTESIAN_POINT('Ctrl Pts',(-9.27225194137694,-13.6684975496401,
117.686437026218)) ;
#157266=CARTESIAN_POINT('Ctrl Pts',(-9.29526311301215,-13.650624726406,
117.756525342438)) ;
#157267=CARTESIAN_POINT('Ctrl Pts',(-9.36906695530124,-13.6506247135771,
117.732294297308)) ;
#157268=CARTESIAN_POINT('Ctrl Pts',(-9.44287079759031,-13.6506247007482,
117.708063252177)) ;
#157269=CARTESIAN_POINT('Ctrl Pts',(-9.4198596259551,-13.6684975239824,
117.637974935957)) ;
#157270=CARTESIAN_POINT('Ctrl Pts',(-9.39684845431988,-13.6863703472165,
117.567886619738)) ;
#157271=CARTESIAN_POINT('Ctrl Pts',(-9.3230446120308,-13.6863703600454,
117.592117664868)) ;
#157272=CARTESIAN_POINT('Ctrl Pts',(-9.24924076974172,-13.6863703728742,
117.616348709998)) ;
#157273=CARTESIAN_POINT('Ctrl Pts',(-9.27225194137694,-13.6684975496401,
117.686437026218)) ;
#157274=CARTESIAN_POINT('Ctrl Pts',(-9.27379869131216,-13.3792258998284,
117.65575130022)) ;
#157275=CARTESIAN_POINT('Ctrl Pts',(-9.29746767065879,-13.3815248172849,
117.727843192722)) ;
#157276=CARTESIAN_POINT('Ctrl Pts',(-9.37127151404433,-13.3815247972218,
117.703612150931)) ;
#157277=CARTESIAN_POINT('Ctrl Pts',(-9.44507535742988,-13.3815247771587,
117.67938110914)) ;
#157278=CARTESIAN_POINT('Ctrl Pts',(-9.42140637808324,-13.3792258597022,
117.607289216639)) ;
#157279=CARTESIAN_POINT('Ctrl Pts',(-9.39773739873661,-13.3769269422458,
117.535197324138)) ;
#157280=CARTESIAN_POINT('Ctrl Pts',(-9.32393355535107,-13.3769269623089,
117.559428365928)) ;
#157281=CARTESIAN_POINT('Ctrl Pts',(-9.25012971196552,-13.3769269823719,
117.583659407719)) ;
#157282=CARTESIAN_POINT('Ctrl Pts',(-9.27379869131216,-13.3792258998284,
117.65575130022)) ;
#157283=CARTESIAN_POINT('Ctrl Pts',(-9.29992444127897,-13.0905267308239,
117.699639537515)) ;
#157284=CARTESIAN_POINT('Ctrl Pts',(-9.32254221362511,-13.1129867022683,
117.768529623299)) ;
#157285=CARTESIAN_POINT('Ctrl Pts',(-9.39634605964063,-13.1129866733618,
117.744298589519)) ;
#157286=CARTESIAN_POINT('Ctrl Pts',(-9.47014990565614,-13.1129866444553,
117.720067555738)) ;
#157287=CARTESIAN_POINT('Ctrl Pts',(-9.44753213330999,-13.0905266730108,
117.651177469954)) ;
#157288=CARTESIAN_POINT('Ctrl Pts',(-9.42491436096384,-13.0680667015663,
117.58228738417)) ;
#157289=CARTESIAN_POINT('Ctrl Pts',(-9.35111051494833,-13.0680667304729,
117.60651841795)) ;
#157290=CARTESIAN_POINT('Ctrl Pts',(-9.27730666893281,-13.0680667593794,
117.630749451731)) ;
#157291=CARTESIAN_POINT('Ctrl Pts',(-9.29992444127897,-13.0905267308239,
117.699639537515)) ;
#157292=CARTESIAN_POINT('Ctrl Pts',(-9.34881358143102,-12.8284630006125,
117.813282587224)) ;
#157293=CARTESIAN_POINT('Ctrl Pts',(-9.36878015715335,-12.8692525646979,
117.874097555988)) ;
#157294=CARTESIAN_POINT('Ctrl Pts',(-9.44258400659655,-12.869252533481,
117.849866532648)) ;
#157295=CARTESIAN_POINT('Ctrl Pts',(-9.51638785603974,-12.869252502264,
117.825635509308)) ;
#157296=CARTESIAN_POINT('Ctrl Pts',(-9.49642128031742,-12.8284629381786,
117.764820540543)) ;
#157297=CARTESIAN_POINT('Ctrl Pts',(-9.47645470459509,-12.7876733740933,
117.704005571779)) ;
#157298=CARTESIAN_POINT('Ctrl Pts',(-9.40265085515189,-12.7876734053102,
117.728236595119)) ;
#157299=CARTESIAN_POINT('Ctrl Pts',(-9.3288470057087,-12.7876734365271,
117.752467618459)) ;
#157300=CARTESIAN_POINT('Ctrl Pts',(-9.34881358143102,-12.8284630006125,
117.813282587224)) ;
#157301=CARTESIAN_POINT('Ctrl Pts',(-9.41846234787993,-12.6065365051644,
117.989873611575)) ;
#157302=CARTESIAN_POINT('Ctrl Pts',(-9.43433055933074,-12.6628800161341,
118.03820562422)) ;
#157303=CARTESIAN_POINT('Ctrl Pts',(-9.50813441331065,-12.6628799847594,
118.013974614698)) ;
#157304=CARTESIAN_POINT('Ctrl Pts',(-9.58193826729053,-12.6628799533848,
117.989743605176)) ;
#157305=CARTESIAN_POINT('Ctrl Pts',(-9.56607005583973,-12.6065364424151,
117.941411592531)) ;
#157306=CARTESIAN_POINT('Ctrl Pts',(-9.55020184438891,-12.5501929314454,
117.893079579885)) ;
#157307=CARTESIAN_POINT('Ctrl Pts',(-9.47639799040901,-12.5501929628201,
117.917310589407)) ;
#157308=CARTESIAN_POINT('Ctrl Pts',(-9.40259413642911,-12.5501929941947,
117.941541598929)) ;
#157309=CARTESIAN_POINT('Ctrl Pts',(-9.41846234787993,-12.6065365051644,
117.989873611575)) ;
#157310=CARTESIAN_POINT('Ctrl Pts',(-9.50417588053103,-12.4434900571409,
118.215497616744)) ;
#157311=CARTESIAN_POINT('Ctrl Pts',(-9.51481602660928,-12.5112986804866,
118.247905785975)) ;
#157312=CARTESIAN_POINT('Ctrl Pts',(-9.58861988520866,-12.5112986555149,
118.223674790523)) ;
#157313=CARTESIAN_POINT('Ctrl Pts',(-9.66242374380803,-12.5112986305432,
118.199443795071)) ;
#157314=CARTESIAN_POINT('Ctrl Pts',(-9.65178359772977,-12.4434900071976,
118.16703562584)) ;
#157315=CARTESIAN_POINT('Ctrl Pts',(-9.64114345165152,-12.3756813838519,
118.13462745661)) ;
#157316=CARTESIAN_POINT('Ctrl Pts',(-9.56733959305215,-12.3756814088236,
118.158858452062)) ;
#157317=CARTESIAN_POINT('Ctrl Pts',(-9.49353573445278,-12.3756814337953,
118.183089447514)) ;
#157318=CARTESIAN_POINT('Ctrl Pts',(-9.50417588053103,-12.4434900571409,
118.215497616744)) ;
#157319=CARTESIAN_POINT('Ctrl Pts',(-9.60073723451511,-12.3500508502058,
118.474134121631)) ;
#157320=CARTESIAN_POINT('Ctrl Pts',(-9.60538505037241,-12.4244812912888,
118.488290620034)) ;
#157321=CARTESIAN_POINT('Ctrl Pts',(-9.67918891312454,-12.424481278477,
118.464059637231)) ;
#157322=CARTESIAN_POINT('Ctrl Pts',(-9.75299277587668,-12.4244812656651,
118.439828654428)) ;
#157323=CARTESIAN_POINT('Ctrl Pts',(-9.74834496001938,-12.3500508245822,
118.425672156025)) ;
#157324=CARTESIAN_POINT('Ctrl Pts',(-9.74369714416208,-12.2756203834992,
118.411515657622)) ;
#157325=CARTESIAN_POINT('Ctrl Pts',(-9.66989328140994,-12.275620396311,
118.435746640425)) ;
#157326=CARTESIAN_POINT('Ctrl Pts',(-9.5960894186578,-12.2756204091229,
118.459977623229)) ;
#157327=CARTESIAN_POINT('Ctrl Pts',(-9.60073723451511,-12.3500508502058,
118.474134121631)) ;
#157328=CARTESIAN_POINT('Ctrl Pts',(-9.70194573753584,-12.3331953888952,
118.746927131276)) ;
#157329=CARTESIAN_POINT('Ctrl Pts',(-9.70026811438521,-12.4089103805945,
118.741817363225)) ;
#157330=CARTESIAN_POINT('Ctrl Pts',(-9.77407198005636,-12.4089103853774,
118.717586389313)) ;
#157331=CARTESIAN_POINT('Ctrl Pts',(-9.84787584572754,-12.4089103901604,
118.693355415401)) ;
#157332=CARTESIAN_POINT('Ctrl Pts',(-9.84955346887816,-12.3331953984611,
118.698465183452)) ;
#157333=CARTESIAN_POINT('Ctrl Pts',(-9.8512310920288,-12.2574804067618,
118.703574951503)) ;
#157334=CARTESIAN_POINT('Ctrl Pts',(-9.77742722635763,-12.2574804019789,
118.727805925415)) ;
#157335=CARTESIAN_POINT('Ctrl Pts',(-9.70362336068647,-12.2574803971959,
118.752036899327)) ;
#157336=CARTESIAN_POINT('Ctrl Pts',(-9.70194573753584,-12.3331953888952,
118.746927131276)) ;
#157337=CARTESIAN_POINT('Ctrl Pts',(-9.80131762641198,-12.3940161187778,
119.014124252987)) ;
#157338=CARTESIAN_POINT('Ctrl Pts',(-9.79343372369382,-12.4655945537366,
118.990111158902)) ;
#157339=CARTESIAN_POINT('Ctrl Pts',(-9.86723759044243,-12.4655945799172,
118.965880188271)) ;
#157340=CARTESIAN_POINT('Ctrl Pts',(-9.94104145719105,-12.4655946060978,
118.941649217641)) ;
#157341=CARTESIAN_POINT('Ctrl Pts',(-9.94892535990921,-12.3940161711391,
118.965662311726)) ;
#157342=CARTESIAN_POINT('Ctrl Pts',(-9.95680926262737,-12.3224377361804,
118.98967540581)) ;
#157343=CARTESIAN_POINT('Ctrl Pts',(-9.88300539587875,-12.3224377099997,
119.013906376441)) ;
#157344=CARTESIAN_POINT('Ctrl Pts',(-9.80920152913014,-12.3224376838191,
119.038137347071)) ;
#157345=CARTESIAN_POINT('Ctrl Pts',(-9.80131762641198,-12.3940161187778,
119.014124252987)) ;
#157346=CARTESIAN_POINT('Ctrl Pts',(-9.89248329484562,-12.5284976067023,
119.256301286483)) ;
#157347=CARTESIAN_POINT('Ctrl Pts',(-9.87895755535242,-12.5907910171459,
119.215104068027)) ;
#157348=CARTESIAN_POINT('Ctrl Pts',(-9.95276142087398,-12.590791066487,
119.190873093659)) ;
#157349=CARTESIAN_POINT('Ctrl Pts',(-10.0265652863955,-12.5907911158281,
119.166642119291)) ;
#157350=CARTESIAN_POINT('Ctrl Pts',(-10.0400910258887,-12.5284977053845,
119.207839337747)) ;
#157351=CARTESIAN_POINT('Ctrl Pts',(-10.0536167653819,-12.466204294941,
119.249036556204)) ;
#157352=CARTESIAN_POINT('Ctrl Pts',(-9.97981289986036,-12.4662042455999,
119.273267530572)) ;
#157353=CARTESIAN_POINT('Ctrl Pts',(-9.9060090343388,-12.4662041962588,
119.29749850494)) ;
#157354=CARTESIAN_POINT('Ctrl Pts',(-9.89248329484562,-12.5284976067023,
119.256301286483)) ;
#157355=CARTESIAN_POINT('Ctrl Pts',(-9.9693440763676,-12.7253590046235,
119.455101779986)) ;
#157356=CARTESIAN_POINT('Ctrl Pts',(-9.95116310647556,-12.7739984449888,
119.399725480954)) ;
#157357=CARTESIAN_POINT('Ctrl Pts',(-10.0249669682071,-12.7739985153053,
119.375494495042)) ;
#157358=CARTESIAN_POINT('Ctrl Pts',(-10.0987708299386,-12.7739985856217,
119.35126350913)) ;
#157359=CARTESIAN_POINT('Ctrl Pts',(-10.1169517998307,-12.7253591452565,
119.406639808163)) ;
#157360=CARTESIAN_POINT('Ctrl Pts',(-10.1351327697227,-12.6767197048912,
119.462016107195)) ;
#157361=CARTESIAN_POINT('Ctrl Pts',(-10.0613289079912,-12.6767196345747,
119.486247093107)) ;
#157362=CARTESIAN_POINT('Ctrl Pts',(-9.98752504625965,-12.6767195642582,
119.510478079019)) ;
#157363=CARTESIAN_POINT('Ctrl Pts',(-9.9693440763676,-12.7253590046235,
119.455101779986)) ;
#157364=CARTESIAN_POINT('Ctrl Pts',(-10.0281574646971,-12.9750336085797,
119.598466100957)) ;
#157365=CARTESIAN_POINT('Ctrl Pts',(-10.006583801685,-13.0063134744705,
119.532756206226)) ;
#157366=CARTESIAN_POINT('Ctrl Pts',(-10.0803876577271,-13.0063135643594,
119.508525202985)) ;
#157367=CARTESIAN_POINT('Ctrl Pts',(-10.1541915137692,-13.0063136542484,
119.484294199744)) ;
#157368=CARTESIAN_POINT('Ctrl Pts',(-10.1757651767812,-12.9750337883576,
119.550004094475)) ;
#157369=CARTESIAN_POINT('Ctrl Pts',(-10.1973388397932,-12.9437539224668,
119.615713989206)) ;
#157370=CARTESIAN_POINT('Ctrl Pts',(-10.1235349837511,-12.9437538325779,
119.639944992447)) ;
#157371=CARTESIAN_POINT('Ctrl Pts',(-10.0497311277091,-12.943753742689,
119.664175995688)) ;
#157372=CARTESIAN_POINT('Ctrl Pts',(-10.0281574646971,-12.9750336085797,
119.598466100957)) ;
#157373=CARTESIAN_POINT('Ctrl Pts',(-10.0639625581,-13.2518773391213,119.672384712737)) ;
#157374=CARTESIAN_POINT('Ctrl Pts',(-10.0405848667401,-13.2638740920304,
119.601180038788)) ;
#157375=CARTESIAN_POINT('Ctrl Pts',(-10.1143887150386,-13.2638741920649,
119.576949011961)) ;
#157376=CARTESIAN_POINT('Ctrl Pts',(-10.1881925633371,-13.2638742920995,
119.552717985135)) ;
#157377=CARTESIAN_POINT('Ctrl Pts',(-10.211570254697,-13.2518775391904,
119.623922659084)) ;
#157378=CARTESIAN_POINT('Ctrl Pts',(-10.2349479460568,-13.2398807862813,
119.695127333032)) ;
#157379=CARTESIAN_POINT('Ctrl Pts',(-10.1611440977583,-13.2398806862467,
119.719358359859)) ;
#157380=CARTESIAN_POINT('Ctrl Pts',(-10.0873402494598,-13.2398805862122,
119.743589386686)) ;
#157381=CARTESIAN_POINT('Ctrl Pts',(-10.0639625581,-13.2518773391213,119.672384712737)) ;
#157382=CARTESIAN_POINT('Ctrl Pts',(-10.0762711870781,-13.5442043587849,
119.674255680769)) ;
#157383=CARTESIAN_POINT('Ctrl Pts',(-10.052736732687,-13.5358098803519,
119.602573531998)) ;
#157384=CARTESIAN_POINT('Ctrl Pts',(-10.1265405723682,-13.5358099849276,
119.578342478924)) ;
#157385=CARTESIAN_POINT('Ctrl Pts',(-10.2003444120494,-13.5358100895033,
119.554111425851)) ;
#157386=CARTESIAN_POINT('Ctrl Pts',(-10.2238788664405,-13.5442045679364,
119.625793574622)) ;
#157387=CARTESIAN_POINT('Ctrl Pts',(-10.2474133208317,-13.5525990463694,
119.697475723393)) ;
#157388=CARTESIAN_POINT('Ctrl Pts',(-10.1736094811505,-13.5525989417936,
119.721706776466)) ;
#157389=CARTESIAN_POINT('Ctrl Pts',(-10.0998056414693,-13.5525988372179,
119.745937829539)) ;
#157390=CARTESIAN_POINT('Ctrl Pts',(-10.0762711870781,-13.5442043587849,
119.674255680769)) ;
#157391=CARTESIAN_POINT('Ctrl Pts',(-10.0642632265541,-13.8259451748865,
119.602266518667)) ;
#157392=CARTESIAN_POINT('Ctrl Pts',(-10.0422653073509,-13.7978682383242,
119.535264408198)) ;
#157393=CARTESIAN_POINT('Ctrl Pts',(-10.1160691382364,-13.7978683377893,
119.511033328335)) ;
#157394=CARTESIAN_POINT('Ctrl Pts',(-10.1898729691219,-13.7978684372543,
119.486802248471)) ;
#157395=CARTESIAN_POINT('Ctrl Pts',(-10.2118708883251,-13.8259453738167,
119.55380435894)) ;
#157396=CARTESIAN_POINT('Ctrl Pts',(-10.2338688075283,-13.8540223103791,
119.620806469409)) ;
#157397=CARTESIAN_POINT('Ctrl Pts',(-10.1600649766428,-13.854022210914,
119.645037549273)) ;
#157398=CARTESIAN_POINT('Ctrl Pts',(-10.0862611457573,-13.8540221114489,
119.669268629136)) ;
#157399=CARTESIAN_POINT('Ctrl Pts',(-10.0642632265541,-13.8259451748865,
119.602266518667)) ;
#157400=CARTESIAN_POINT('Ctrl Pts',(-10.0296964583947,-14.0792480619856,
119.461456237366)) ;
#157401=CARTESIAN_POINT('Ctrl Pts',(-10.0108143826101,-14.0334450409061,
119.403944483233)) ;
#157402=CARTESIAN_POINT('Ctrl Pts',(-10.0846182054714,-14.0334451269848,
119.379713378929)) ;
#157403=CARTESIAN_POINT('Ctrl Pts',(-10.1584220283326,-14.0334452130635,
119.355482274624)) ;
#157404=CARTESIAN_POINT('Ctrl Pts',(-10.1773041041172,-14.079248234143,
119.412994028758)) ;
#157405=CARTESIAN_POINT('Ctrl Pts',(-10.1961861799017,-14.1250512552225,
119.470505782891)) ;
#157406=CARTESIAN_POINT('Ctrl Pts',(-10.1223823570405,-14.1250511691438,
119.494736887195)) ;
#157407=CARTESIAN_POINT('Ctrl Pts',(-10.0485785341793,-14.1250510830651,
119.518967991499)) ;
#157408=CARTESIAN_POINT('Ctrl Pts',(-10.0296964583947,-14.0792480619856,
119.461456237366)) ;
#157409=CARTESIAN_POINT('Ctrl Pts',(-9.97588775903519,-14.2845087011992,
119.262132122512)) ;
#157410=CARTESIAN_POINT('Ctrl Pts',(-9.96146759893467,-14.2243072924303,
119.218210643622)) ;
#157411=CARTESIAN_POINT('Ctrl Pts',(-10.0352714154371,-14.2243073577872,
119.19397951995)) ;
#157412=CARTESIAN_POINT('Ctrl Pts',(-10.1090752319395,-14.2243074231441,
119.169748396277)) ;
#157413=CARTESIAN_POINT('Ctrl Pts',(-10.12349539204,-14.284508831913,119.213669875168)) ;
#157414=CARTESIAN_POINT('Ctrl Pts',(-10.1379155521406,-14.3447102406819,
119.257591354058)) ;
#157415=CARTESIAN_POINT('Ctrl Pts',(-10.0641117356382,-14.344710175325,
119.28182247773)) ;
#157416=CARTESIAN_POINT('Ctrl Pts',(-9.99030791913573,-14.3447101099681,
119.306053601403)) ;
#157417=CARTESIAN_POINT('Ctrl Pts',(-9.97588775903519,-14.2845087011992,
119.262132122512)) ;
#157418=CARTESIAN_POINT('Ctrl Pts',(-9.90744210014645,-14.4278905637469,
119.018229253178)) ;
#157419=CARTESIAN_POINT('Ctrl Pts',(-9.89851224393999,-14.3575893614837,
118.991030354069)) ;
#157420=CARTESIAN_POINT('Ctrl Pts',(-9.97231605632315,-14.3575894011323,
118.96679921785)) ;
#157421=CARTESIAN_POINT('Ctrl Pts',(-10.0461198687063,-14.3575894407809,
118.942568081632)) ;
#157422=CARTESIAN_POINT('Ctrl Pts',(-10.0550497249128,-14.4278906430441,
118.96976698074)) ;
#157423=CARTESIAN_POINT('Ctrl Pts',(-10.0639795811192,-14.4981918453073,
118.996965879848)) ;
#157424=CARTESIAN_POINT('Ctrl Pts',(-9.99017576873607,-14.4981918056587,
119.021197016067)) ;
#157425=CARTESIAN_POINT('Ctrl Pts',(-9.91637195635291,-14.4981917660102,
119.045428152286)) ;
#157426=CARTESIAN_POINT('Ctrl Pts',(-9.90744210014645,-14.4278905637469,
119.018229253178)) ;
#157427=CARTESIAN_POINT('Ctrl Pts',(-9.82982242385163,-14.49909499359,118.746322529544)) ;
#157428=CARTESIAN_POINT('Ctrl Pts',(-9.8270327331662,-14.4237176570017,
118.737825583854)) ;
#157429=CARTESIAN_POINT('Ctrl Pts',(-9.90083654412551,-14.4237176684641,
118.713594443298)) ;
#157430=CARTESIAN_POINT('Ctrl Pts',(-9.97464035508483,-14.4237176799264,
118.689363302743)) ;
#157431=CARTESIAN_POINT('Ctrl Pts',(-9.97743004577026,-14.4990950165147,
118.697860248433)) ;
#157432=CARTESIAN_POINT('Ctrl Pts',(-9.9802197364557,-14.5744723531029,
118.706357194123)) ;
#157433=CARTESIAN_POINT('Ctrl Pts',(-9.90641592549639,-14.5744723416406,
118.730588334679)) ;
#157434=CARTESIAN_POINT('Ctrl Pts',(-9.83261211453707,-14.5744723301783,
118.754819475234)) ;
#157435=CARTESIAN_POINT('Ctrl Pts',(-9.82982242385163,-14.49909499359,118.746322529544)) ;
#157436=CARTESIAN_POINT('Ctrl Pts',(-9.74956192660519,-14.492829252027,
118.466414353285)) ;
#157437=CARTESIAN_POINT('Ctrl Pts',(-9.75310509711621,-14.4177767154629,
118.477206280931)) ;
#157438=CARTESIAN_POINT('Ctrl Pts',(-9.82690890932998,-14.4177766993577,
118.452975144196)) ;
#157439=CARTESIAN_POINT('Ctrl Pts',(-9.90071272154373,-14.4177766832525,
118.428744007461)) ;
#157440=CARTESIAN_POINT('Ctrl Pts',(-9.8971695510327,-14.4928292198167,
118.417952079816)) ;
#157441=CARTESIAN_POINT('Ctrl Pts',(-9.89362638052167,-14.5678817563809,
118.40716015217)) ;
#157442=CARTESIAN_POINT('Ctrl Pts',(-9.81982256830792,-14.567881772486,
118.431391288905)) ;
#157443=CARTESIAN_POINT('Ctrl Pts',(-9.74601875609416,-14.5678817885912,
118.45562242564)) ;
#157444=CARTESIAN_POINT('Ctrl Pts',(-9.74956192660519,-14.492829252027,
118.466414353285)) ;
#157445=CARTESIAN_POINT('Ctrl Pts',(-9.67283879350772,-14.4093444300335,
118.197174970448)) ;
#157446=CARTESIAN_POINT('Ctrl Pts',(-9.68247953277884,-14.3400077238797,
118.226539108603)) ;
#157447=CARTESIAN_POINT('Ctrl Pts',(-9.75628334887631,-14.3400076836513,
118.202307983697)) ;
#157448=CARTESIAN_POINT('Ctrl Pts',(-9.8300871649738,-14.340007643423,118.178076858792)) ;
#157449=CARTESIAN_POINT('Ctrl Pts',(-9.82044642570268,-14.4093443495768,
118.148712720637)) ;
#157450=CARTESIAN_POINT('Ctrl Pts',(-9.81080568643156,-14.4786810557306,
118.119348582483)) ;
#157451=CARTESIAN_POINT('Ctrl Pts',(-9.73700187033407,-14.4786810959589,
118.143579707388)) ;
#157452=CARTESIAN_POINT('Ctrl Pts',(-9.66319805423659,-14.4786811361873,
118.167810832294)) ;
#157453=CARTESIAN_POINT('Ctrl Pts',(-9.67283879350772,-14.4093444300335,
118.197174970448)) ;
#157454=CARTESIAN_POINT('Ctrl Pts',(-9.60626579738372,-14.2544052422715,
117.958871810111)) ;
#157455=CARTESIAN_POINT('Ctrl Pts',(-9.62130430767447,-14.1957815883073,
118.004676687747)) ;
#157456=CARTESIAN_POINT('Ctrl Pts',(-9.69510812953136,-14.1957815301846,
117.980445580384)) ;
#157457=CARTESIAN_POINT('Ctrl Pts',(-9.76891195138824,-14.1957814720619,
117.95621447302)) ;
#157458=CARTESIAN_POINT('Ctrl Pts',(-9.75387344109749,-14.2544051260261,
117.910409595385)) ;
#157459=CARTESIAN_POINT('Ctrl Pts',(-9.73883493080673,-14.3130287799903,
117.864604717749)) ;
#157460=CARTESIAN_POINT('Ctrl Pts',(-9.66503110894986,-14.313028838113,
117.888835825112)) ;
#157461=CARTESIAN_POINT('Ctrl Pts',(-9.59122728709297,-14.3130288962357,
117.913066932476)) ;
#157462=CARTESIAN_POINT('Ctrl Pts',(-9.60626579738372,-14.2544052422715,
117.958871810111)) ;
#157463=CARTESIAN_POINT('Ctrl Pts',(-9.55553746479956,-14.0410991720381,
117.769068814144)) ;
#157464=CARTESIAN_POINT('Ctrl Pts',(-9.57487061302664,-13.9972803376337,
117.827954465898)) ;
#157465=CARTESIAN_POINT('Ctrl Pts',(-9.64867444137708,-13.9972802674836,
117.803723378313)) ;
#157466=CARTESIAN_POINT('Ctrl Pts',(-9.72247826972751,-13.9972801973335,
117.779492290728)) ;
#157467=CARTESIAN_POINT('Ctrl Pts',(-9.70314512150042,-14.0410990317379,
117.720606638974)) ;
#157468=CARTESIAN_POINT('Ctrl Pts',(-9.68381197327334,-14.0849178661423,
117.66172098722)) ;
#157469=CARTESIAN_POINT('Ctrl Pts',(-9.6100081449229,-14.0849179362924,
117.685952074805)) ;
#157470=CARTESIAN_POINT('Ctrl Pts',(-9.53620431657246,-14.0849180064424,
117.71018316239)) ;
#157471=CARTESIAN_POINT('Ctrl Pts',(-9.55553746479956,-14.0410991720381,
117.769068814144)) ;
#157472=CARTESIAN_POINT('Ctrl Pts',(-9.52441285793816,-13.7816895970119,
117.638727760598)) ;
#157473=CARTESIAN_POINT('Ctrl Pts',(-9.5466837632346,-13.7559161217153,
117.706561346231)) ;
#157474=CARTESIAN_POINT('Ctrl Pts',(-9.62048759876048,-13.7559160484501,
117.682330280501)) ;
#157475=CARTESIAN_POINT('Ctrl Pts',(-9.69429143428636,-13.7559159751849,
117.658099214771)) ;
#157476=CARTESIAN_POINT('Ctrl Pts',(-9.67202052898993,-13.7816894504815,
117.590265629138)) ;
#157477=CARTESIAN_POINT('Ctrl Pts',(-9.64974962369348,-13.8074629257781,
117.522432043505)) ;
#157478=CARTESIAN_POINT('Ctrl Pts',(-9.5759457881676,-13.8074629990433,
117.546663109235)) ;
#157479=CARTESIAN_POINT('Ctrl Pts',(-9.50214195264172,-13.8074630723084,
117.570894174964)) ;
#157480=CARTESIAN_POINT('Ctrl Pts',(-9.52441285793816,-13.7816895970119,
117.638727760598)) ;
#157481=CARTESIAN_POINT('Ctrl Pts',(-9.51628185017245,-13.4976199910735,
117.578613119079)) ;
#157482=CARTESIAN_POINT('Ctrl Pts',(-9.53988551258455,-13.4916413053213,
117.650506067717)) ;
#157483=CARTESIAN_POINT('Ctrl Pts',(-9.61368935460016,-13.4916412347082,
117.626275021754)) ;
#157484=CARTESIAN_POINT('Ctrl Pts',(-9.68749319661578,-13.4916411640951,
117.60204397579)) ;
#157485=CARTESIAN_POINT('Ctrl Pts',(-9.66388953420369,-13.4976198498473,
117.530151027152)) ;
#157486=CARTESIAN_POINT('Ctrl Pts',(-9.6402858717916,-13.5035985355994,
117.458258078514)) ;
#157487=CARTESIAN_POINT('Ctrl Pts',(-9.56648202977599,-13.5035986062125,
117.482489124477)) ;
#157488=CARTESIAN_POINT('Ctrl Pts',(-9.49267818776037,-13.5035986768257,
117.506720170441)) ;
#157489=CARTESIAN_POINT('Ctrl Pts',(-9.51628185017245,-13.4976199910735,
117.578613119079)) ;
#157490=CARTESIAN_POINT('Ctrl Pts',(-9.53237212691088,-13.2063007087737,
117.592070626438)) ;
#157491=CARTESIAN_POINT('Ctrl Pts',(-9.55562384876197,-13.2206528794354,
117.662891620739)) ;
#157492=CARTESIAN_POINT('Ctrl Pts',(-9.62942769617348,-13.2206528189828,
117.63866059121)) ;
#157493=CARTESIAN_POINT('Ctrl Pts',(-9.70323154358499,-13.2206527585302,
117.614429561682)) ;
#157494=CARTESIAN_POINT('Ctrl Pts',(-9.67997982173389,-13.2063005878686,
117.543608567381)) ;
#157495=CARTESIAN_POINT('Ctrl Pts',(-9.6567280998828,-13.1919484172069,
117.47278757308)) ;
#157496=CARTESIAN_POINT('Ctrl Pts',(-9.5829242524713,-13.1919484776594,
117.497018602609)) ;
#157497=CARTESIAN_POINT('Ctrl Pts',(-9.50912040505978,-13.191948538112,
117.521249632137)) ;
#157498=CARTESIAN_POINT('Ctrl Pts',(-9.53237212691088,-13.2063007087737,
117.592070626438)) ;
#157499=CARTESIAN_POINT('Ctrl Pts',(-9.57232919510587,-12.9308185504047,
117.678310643569)) ;
#157500=CARTESIAN_POINT('Ctrl Pts',(-9.5935601703269,-12.9644269321628,
117.742976769516)) ;
#157501=CARTESIAN_POINT('Ctrl Pts',(-9.66736402139537,-12.9644268849646,
117.718745751126)) ;
#157502=CARTESIAN_POINT('Ctrl Pts',(-9.74116787246387,-12.9644268377663,
117.694514732736)) ;
#157503=CARTESIAN_POINT('Ctrl Pts',(-9.71993689724284,-12.9308184560083,
117.62984860679)) ;
#157504=CARTESIAN_POINT('Ctrl Pts',(-9.69870592202183,-12.8972100742503,
117.565182480843)) ;
#157505=CARTESIAN_POINT('Ctrl Pts',(-9.62490207095333,-12.8972101214485,
117.589413499233)) ;
#157506=CARTESIAN_POINT('Ctrl Pts',(-9.55109821988485,-12.8972101686467,
117.613644517623)) ;
#157507=CARTESIAN_POINT('Ctrl Pts',(-9.57232919510587,-12.9308185504047,
117.678310643569)) ;
#157508=CARTESIAN_POINT('Ctrl Pts',(-9.634113078639,-12.690040453889,117.830986128613)) ;
#157509=CARTESIAN_POINT('Ctrl Pts',(-9.65179721230132,-12.7405114660654,
117.884849147276)) ;
#157510=CARTESIAN_POINT('Ctrl Pts',(-9.72560106508382,-12.7405114337976,
117.860618134107)) ;
#157511=CARTESIAN_POINT('Ctrl Pts',(-9.79940491786632,-12.7405114015298,
117.836387120937)) ;
#157512=CARTESIAN_POINT('Ctrl Pts',(-9.78172078420399,-12.6900403893535,
117.782524102275)) ;
#157513=CARTESIAN_POINT('Ctrl Pts',(-9.76403665054166,-12.6395693771771,
117.728661083612)) ;
#157514=CARTESIAN_POINT('Ctrl Pts',(-9.69023279775917,-12.6395694094449,
117.752892096781)) ;
#157515=CARTESIAN_POINT('Ctrl Pts',(-9.61642894497667,-12.6395694417127,
117.77712310995)) ;
#157516=CARTESIAN_POINT('Ctrl Pts',(-9.634113078639,-12.690040453889,117.830986128613)) ;
#157517=CARTESIAN_POINT('Ctrl Pts',(-9.713580692807,-12.5021903792694,118.037691814633)) ;
#157518=CARTESIAN_POINT('Ctrl Pts',(-9.72647426064452,-12.5658538076965,
118.076963542604)) ;
#157519=CARTESIAN_POINT('Ctrl Pts',(-9.80027811379014,-12.5658537885695,
118.052732530541)) ;
#157520=CARTESIAN_POINT('Ctrl Pts',(-9.87408196693574,-12.5658537694425,
118.028501518478)) ;
#157521=CARTESIAN_POINT('Ctrl Pts',(-9.86118839909822,-12.5021903410154,
117.989229790506)) ;
#157522=CARTESIAN_POINT('Ctrl Pts',(-9.84829483126071,-12.4385269125883,
117.949958062535)) ;
#157523=CARTESIAN_POINT('Ctrl Pts',(-9.77449097811509,-12.4385269317153,
117.974189074598)) ;
#157524=CARTESIAN_POINT('Ctrl Pts',(-9.70068712496948,-12.4385269508424,
117.998420086661)) ;
#157525=CARTESIAN_POINT('Ctrl Pts',(-9.713580692807,-12.5021903792694,118.037691814633)) ;
#157526=CARTESIAN_POINT('Ctrl Pts',(-9.80659684966496,-12.3790435207342,
118.285471103814)) ;
#157527=CARTESIAN_POINT('Ctrl Pts',(-9.81375059597936,-12.4514021719633,
118.307260261368)) ;
#157528=CARTESIAN_POINT('Ctrl Pts',(-9.887554447672,-12.4514021645019,118.283029244879)) ;
#157529=CARTESIAN_POINT('Ctrl Pts',(-9.96135829936465,-12.4514021570405,
118.25879822839)) ;
#157530=CARTESIAN_POINT('Ctrl Pts',(-9.95420455305025,-12.3790435058114,
118.237009070837)) ;
#157531=CARTESIAN_POINT('Ctrl Pts',(-9.94705080673585,-12.3066848545823,
118.215219913283)) ;
#157532=CARTESIAN_POINT('Ctrl Pts',(-9.87324695504321,-12.3066848620437,
118.239450929772)) ;
#157533=CARTESIAN_POINT('Ctrl Pts',(-9.79944310335057,-12.3066848695051,
118.263681946261)) ;
#157534=CARTESIAN_POINT('Ctrl Pts',(-9.80659684966496,-12.3790435207342,
118.285471103814)) ;
#157535=CARTESIAN_POINT('Ctrl Pts',(-9.90658661047469,-12.3305042760163,
118.554594905817)) ;
#157536=CARTESIAN_POINT('Ctrl Pts',(-9.90750267093768,-12.4063616289538,
118.557385078565)) ;
#157537=CARTESIAN_POINT('Ctrl Pts',(-9.98130652053492,-12.4063616290811,
118.533154055694)) ;
#157538=CARTESIAN_POINT('Ctrl Pts',(-10.0551103701321,-12.4063616292084,
118.508923032823)) ;
#157539=CARTESIAN_POINT('Ctrl Pts',(-10.0541943096692,-12.3305042762709,
118.506132860075)) ;
#157540=CARTESIAN_POINT('Ctrl Pts',(-10.0532782492062,-12.2546469233334,
118.503342687327)) ;
#157541=CARTESIAN_POINT('Ctrl Pts',(-9.97947439960893,-12.2546469232061,
118.527573710198)) ;
#157542=CARTESIAN_POINT('Ctrl Pts',(-9.9056705500117,-12.2546469230788,
118.551804733069)) ;
#157543=CARTESIAN_POINT('Ctrl Pts',(-9.90658661047469,-12.3305042760163,
118.554594905817)) ;
#157544=CARTESIAN_POINT('Ctrl Pts',(-10.008066495342,-12.3604684800267,
118.827998813982)) ;
#157545=CARTESIAN_POINT('Ctrl Pts',(-10.0026364882404,-12.434348796245,
118.811459888692)) ;
#157546=CARTESIAN_POINT('Ctrl Pts',(-10.0764403349558,-12.4343487994094,
118.787228857044)) ;
#157547=CARTESIAN_POINT('Ctrl Pts',(-10.1502441816713,-12.4343488025737,
118.762997825396)) ;
#157548=CARTESIAN_POINT('Ctrl Pts',(-10.1556741887729,-12.3604684863554,
118.779536750686)) ;
#157549=CARTESIAN_POINT('Ctrl Pts',(-10.1611041958745,-12.2865881701371,
118.796075675976)) ;
#157550=CARTESIAN_POINT('Ctrl Pts',(-10.087300349159,-12.2865881669728,
118.820306707624)) ;
#157551=CARTESIAN_POINT('Ctrl Pts',(-10.0134965024436,-12.2865881638084,
118.844537739272)) ;
#157552=CARTESIAN_POINT('Ctrl Pts',(-10.008066495342,-12.3604684800267,
118.827998813982)) ;
#157553=CARTESIAN_POINT('Ctrl Pts',(-10.1026122259296,-12.4650891112354,
119.080754567184)) ;
#157554=CARTESIAN_POINT('Ctrl Pts',(-10.0913012354726,-12.5317749496589,
119.0463031154)) ;
#157555=CARTESIAN_POINT('Ctrl Pts',(-10.1651050806005,-12.5317749532163,
119.022072078917)) ;
#157556=CARTESIAN_POINT('Ctrl Pts',(-10.2389089257285,-12.5317749567737,
118.997841042433)) ;
#157557=CARTESIAN_POINT('Ctrl Pts',(-10.2502199161856,-12.4650891183502,
119.032292494217)) ;
#157558=CARTESIAN_POINT('Ctrl Pts',(-10.2615309066426,-12.3984032799266,
119.066743946)) ;
#157559=CARTESIAN_POINT('Ctrl Pts',(-10.1877270615146,-12.3984032763692,
119.090974982484)) ;
#157560=CARTESIAN_POINT('Ctrl Pts',(-10.1139232163866,-12.3984032728119,
119.115206018967)) ;
#157561=CARTESIAN_POINT('Ctrl Pts',(-10.1026122259296,-12.4650891112354,
119.080754567184)) ;
#157562=CARTESIAN_POINT('Ctrl Pts',(-10.1865625678926,-12.6397680496829,
119.300758559966)) ;
#157563=CARTESIAN_POINT('Ctrl Pts',(-10.1701110588088,-12.6943569653302,
119.25064991775)) ;
#157564=CARTESIAN_POINT('Ctrl Pts',(-10.2439149022629,-12.6943569660359,
119.226418876168)) ;
#157565=CARTESIAN_POINT('Ctrl Pts',(-10.317718745717,-12.6943569667415,
119.202187834586)) ;
#157566=CARTESIAN_POINT('Ctrl Pts',(-10.3341702548008,-12.6397680510942,
119.252296476803)) ;
#157567=CARTESIAN_POINT('Ctrl Pts',(-10.3506217638846,-12.5851791354469,
119.302405119019)) ;
#157568=CARTESIAN_POINT('Ctrl Pts',(-10.2768179204305,-12.5851791347412,
119.326636160601)) ;
#157569=CARTESIAN_POINT('Ctrl Pts',(-10.2030140769763,-12.5851791340356,
119.350867202183)) ;
#157570=CARTESIAN_POINT('Ctrl Pts',(-10.1865625678926,-12.6397680496829,
119.300758559966)) ;
#157571=CARTESIAN_POINT('Ctrl Pts',(-10.2525551850904,-12.8673926753431,
119.466570849935)) ;
#157572=CARTESIAN_POINT('Ctrl Pts',(-10.2321995339973,-12.9061686393151,
119.404570821043)) ;
#157573=CARTESIAN_POINT('Ctrl Pts',(-10.3060033770812,-12.9061686378558,
119.380339778333)) ;
#157574=CARTESIAN_POINT('Ctrl Pts',(-10.379807220165,-12.9061686363964,
119.356108735624)) ;
#157575=CARTESIAN_POINT('Ctrl Pts',(-10.4001628712581,-12.8673926724244,
119.418108764515)) ;
#157576=CARTESIAN_POINT('Ctrl Pts',(-10.4205185223511,-12.8286167084523,
119.480108793406)) ;
#157577=CARTESIAN_POINT('Ctrl Pts',(-10.3467146792673,-12.8286167099117,
119.504339836116)) ;
#157578=CARTESIAN_POINT('Ctrl Pts',(-10.2729108361835,-12.828616711371,
119.528570878826)) ;
#157579=CARTESIAN_POINT('Ctrl Pts',(-10.2525551850904,-12.8673926753431,
119.466570849935)) ;
#157580=CARTESIAN_POINT('Ctrl Pts',(-10.2984413344148,-13.138383085188,
119.5705591487)) ;
#157581=CARTESIAN_POINT('Ctrl Pts',(-10.2755911957919,-13.1582932670834,
119.500961313244)) ;
#157582=CARTESIAN_POINT('Ctrl Pts',(-10.3493950389077,-13.15829326372,119.476730270631)) ;
#157583=CARTESIAN_POINT('Ctrl Pts',(-10.4231988820235,-13.1582932603565,
119.452499228019)) ;
#157584=CARTESIAN_POINT('Ctrl Pts',(-10.4460490206464,-13.1383830784611,
119.522097063476)) ;
#157585=CARTESIAN_POINT('Ctrl Pts',(-10.4688991592693,-13.1184728965658,
119.591694898932)) ;
#157586=CARTESIAN_POINT('Ctrl Pts',(-10.3950953161535,-13.1184728999292,
119.615925941545)) ;
#157587=CARTESIAN_POINT('Ctrl Pts',(-10.3212914730377,-13.1184729032926,
119.640156984157)) ;
#157588=CARTESIAN_POINT('Ctrl Pts',(-10.2984413344148,-13.138383085188,
119.5705591487)) ;
#157589=CARTESIAN_POINT('Ctrl Pts',(-10.3201874020919,-13.4250580301084,
119.601606079011)) ;
#157590=CARTESIAN_POINT('Ctrl Pts',(-10.2965135474119,-13.4249798616491,
119.52949933737)) ;
#157591=CARTESIAN_POINT('Ctrl Pts',(-10.3703173908735,-13.4249798591319,
119.50526829581)) ;
#157592=CARTESIAN_POINT('Ctrl Pts',(-10.444121234335,-13.4249798566146,
119.481037254251)) ;
#157593=CARTESIAN_POINT('Ctrl Pts',(-10.467795089015,-13.4250580250739,
119.553143995892)) ;
#157594=CARTESIAN_POINT('Ctrl Pts',(-10.491468943695,-13.4251361935332,
119.625250737534)) ;
#157595=CARTESIAN_POINT('Ctrl Pts',(-10.4176651002335,-13.4251361960505,
119.649481779093)) ;
#157596=CARTESIAN_POINT('Ctrl Pts',(-10.3438612567719,-13.4251361985678,
119.673712820652)) ;
#157597=CARTESIAN_POINT('Ctrl Pts',(-10.3201874020919,-13.4250580301084,
119.601606079011)) ;
#157598=CARTESIAN_POINT('Ctrl Pts',(-10.3180530372285,-13.713663843469,
119.559606091718)) ;
#157599=CARTESIAN_POINT('Ctrl Pts',(-10.2952280150007,-13.6934329579285,
119.490084756816)) ;
#157600=CARTESIAN_POINT('Ctrl Pts',(-10.3690318585251,-13.6934329580841,
119.465853715448)) ;
#157601=CARTESIAN_POINT('Ctrl Pts',(-10.4428357020495,-13.6934329582396,
119.441622674081)) ;
#157602=CARTESIAN_POINT('Ctrl Pts',(-10.4656607242774,-13.7136638437801,
119.511144008982)) ;
#157603=CARTESIAN_POINT('Ctrl Pts',(-10.4884857465052,-13.7338947293205,
119.580665343884)) ;
#157604=CARTESIAN_POINT('Ctrl Pts',(-10.4146819029808,-13.733894729165,
119.604896385251)) ;
#157605=CARTESIAN_POINT('Ctrl Pts',(-10.3408780594563,-13.7338947290095,
119.629127426619)) ;
#157606=CARTESIAN_POINT('Ctrl Pts',(-10.3180530372285,-13.713663843469,
119.559606091718)) ;
#157607=CARTESIAN_POINT('Ctrl Pts',(-10.2921786001434,-13.9818996954329,
119.445166371893)) ;
#157608=CARTESIAN_POINT('Ctrl Pts',(-10.2718641660542,-13.9429089187137,
119.383291883489)) ;
#157609=CARTESIAN_POINT('Ctrl Pts',(-10.3456680086685,-13.9429089238121,
119.359060839349)) ;
#157610=CARTESIAN_POINT('Ctrl Pts',(-10.4194718512827,-13.9429089289105,
119.334829795209)) ;
#157611=CARTESIAN_POINT('Ctrl Pts',(-10.4397862853719,-13.9818997056297,
119.396704283613)) ;
#157612=CARTESIAN_POINT('Ctrl Pts',(-10.4601007194611,-14.0208904823489,
119.458578772017)) ;
#157613=CARTESIAN_POINT('Ctrl Pts',(-10.3862968768469,-14.0208904772505,
119.482809816157)) ;
#157614=CARTESIAN_POINT('Ctrl Pts',(-10.3124930342326,-14.0208904721521,
119.507040860297)) ;
#157615=CARTESIAN_POINT('Ctrl Pts',(-10.2921786001434,-13.9818996954329,
119.445166371893)) ;
#157616=CARTESIAN_POINT('Ctrl Pts',(-10.245938215231,-14.2073240866329,
119.269059645356)) ;
#157617=CARTESIAN_POINT('Ctrl Pts',(-10.2295527871486,-14.1525370337597,
119.219152275396)) ;
#157618=CARTESIAN_POINT('Ctrl Pts',(-10.303356628324,-14.1525370412397,
119.194921226873)) ;
#157619=CARTESIAN_POINT('Ctrl Pts',(-10.3771604694994,-14.1525370487197,
119.170690178351)) ;
#157620=CARTESIAN_POINT('Ctrl Pts',(-10.3935458975818,-14.2073241015929,
119.220597548311)) ;
#157621=CARTESIAN_POINT('Ctrl Pts',(-10.4099313256642,-14.2621111544661,
119.270504918271)) ;
#157622=CARTESIAN_POINT('Ctrl Pts',(-10.3361274844888,-14.2621111469861,
119.294735966793)) ;
#157623=CARTESIAN_POINT('Ctrl Pts',(-10.2623236433134,-14.2621111395061,
119.318967015316)) ;
#157624=CARTESIAN_POINT('Ctrl Pts',(-10.245938215231,-14.2073240866329,
119.269059645356)) ;
#157625=CARTESIAN_POINT('Ctrl Pts',(-10.1827043131007,-14.3779496982449,
119.040941067964)) ;
#157626=CARTESIAN_POINT('Ctrl Pts',(-10.1714452553299,-14.3111692669398,
119.006647794977)) ;
#157627=CARTESIAN_POINT('Ctrl Pts',(-10.245249094003,-14.3111692758398,
118.982416738833)) ;
#157628=CARTESIAN_POINT('Ctrl Pts',(-10.3190529326762,-14.3111692847398,
118.958185682689)) ;
#157629=CARTESIAN_POINT('Ctrl Pts',(-10.330311990447,-14.3779497160448,
118.992478955676)) ;
#157630=CARTESIAN_POINT('Ctrl Pts',(-10.3415710482178,-14.4447301473499,
119.026772228663)) ;
#157631=CARTESIAN_POINT('Ctrl Pts',(-10.2677672095446,-14.4447301384499,
119.051003284807)) ;
#157632=CARTESIAN_POINT('Ctrl Pts',(-10.1939633708715,-14.4447301295499,
119.075234340951)) ;
#157633=CARTESIAN_POINT('Ctrl Pts',(-10.1827043131007,-14.3779496982449,
119.040941067964)) ;
#157634=CARTESIAN_POINT('Ctrl Pts',(-10.1079403524329,-14.4795452062324,
118.777702483988)) ;
#157635=CARTESIAN_POINT('Ctrl Pts',(-10.1026201618355,-14.405574238108,
118.761498042339)) ;
#157636=CARTESIAN_POINT('Ctrl Pts',(-10.1764239974123,-14.4055742445888,
118.737266976764)) ;
#157637=CARTESIAN_POINT('Ctrl Pts',(-10.250227832989,-14.4055742510696,
118.713035911189)) ;
#157638=CARTESIAN_POINT('Ctrl Pts',(-10.2555480235865,-14.4795452191939,
118.729240352838)) ;
#157639=CARTESIAN_POINT('Ctrl Pts',(-10.2608682141839,-14.5535161873183,
118.745444794488)) ;
#157640=CARTESIAN_POINT('Ctrl Pts',(-10.1870643786071,-14.5535161808375,
118.769675860063)) ;
#157641=CARTESIAN_POINT('Ctrl Pts',(-10.1132605430304,-14.5535161743567,
118.793906925638)) ;
#157642=CARTESIAN_POINT('Ctrl Pts',(-10.1079403524329,-14.4795452062324,
118.777702483988)) ;
#157643=CARTESIAN_POINT('Ctrl Pts',(-10.0277788315133,-14.504675613756,
118.497994836855)) ;
#157644=CARTESIAN_POINT('Ctrl Pts',(-10.0287835153218,-14.4288427645242,
118.501054942308)) ;
#157645=CARTESIAN_POINT('Ctrl Pts',(-10.1025873477986,-14.4288427635045,
118.476823867291)) ;
#157646=CARTESIAN_POINT('Ctrl Pts',(-10.1763911802754,-14.4288427624848,
118.452592792274)) ;
#157647=CARTESIAN_POINT('Ctrl Pts',(-10.1753864964669,-14.5046756117167,
118.449532686821)) ;
#157648=CARTESIAN_POINT('Ctrl Pts',(-10.1743818126584,-14.5805084609485,
118.446472581367)) ;
#157649=CARTESIAN_POINT('Ctrl Pts',(-10.1005779801816,-14.5805084619682,
118.470703656384)) ;
#157650=CARTESIAN_POINT('Ctrl Pts',(-10.0267741477048,-14.5805084629879,
118.494934731401)) ;
#157651=CARTESIAN_POINT('Ctrl Pts',(-10.0277788315133,-14.504675613756,
118.497994836855)) ;
#157652=CARTESIAN_POINT('Ctrl Pts',(-9.94934961424335,-14.4524935600785,
118.223832977652)) ;
#157653=CARTESIAN_POINT('Ctrl Pts',(-9.95656164691611,-14.3801950254555,
118.245799666326)) ;
#157654=CARTESIAN_POINT('Ctrl Pts',(-10.030365477824,-14.3801950131856,
118.22156858653)) ;
#157655=CARTESIAN_POINT('Ctrl Pts',(-10.1041693087319,-14.3801950009157,
118.197337506734)) ;
#157656=CARTESIAN_POINT('Ctrl Pts',(-10.0969572760591,-14.4524935355387,
118.175370818061)) ;
#157657=CARTESIAN_POINT('Ctrl Pts',(-10.0897452433863,-14.5247920701618,
118.153404129387)) ;
#157658=CARTESIAN_POINT('Ctrl Pts',(-10.0159414124784,-14.5247920824317,
118.177635209183)) ;
#157659=CARTESIAN_POINT('Ctrl Pts',(-9.94213758157056,-14.5247920947016,
118.201866288978)) ;
#157660=CARTESIAN_POINT('Ctrl Pts',(-9.94934961424335,-14.4524935600785,
118.223832977652)) ;
#157661=CARTESIAN_POINT('Ctrl Pts',(-9.8776805943081,-14.3253673837965,
117.969892660447)) ;
#157662=CARTESIAN_POINT('Ctrl Pts',(-9.89064463115639,-14.2618396984513,
118.009379025961)) ;
#157663=CARTESIAN_POINT('Ctrl Pts',(-9.96444846077423,-14.2618396702595,
117.985147942236)) ;
#157664=CARTESIAN_POINT('Ctrl Pts',(-10.0382522903921,-14.2618396420677,
117.960916858511)) ;
#157665=CARTESIAN_POINT('Ctrl Pts',(-10.0252882535438,-14.325367327413,
117.921430492997)) ;
#157666=CARTESIAN_POINT('Ctrl Pts',(-10.0123242166955,-14.3888950127582,
117.881944127484)) ;
#157667=CARTESIAN_POINT('Ctrl Pts',(-9.93852038707766,-14.38889504095,117.906175211209)) ;
#157668=CARTESIAN_POINT('Ctrl Pts',(-9.86471655745981,-14.3888950691418,
117.930406294933)) ;
#157669=CARTESIAN_POINT('Ctrl Pts',(-9.8776805943081,-14.3253673837965,
117.969892660447)) ;
#157670=CARTESIAN_POINT('Ctrl Pts',(-9.81989105535084,-14.1335026343525,
117.758421157027)) ;
#157671=CARTESIAN_POINT('Ctrl Pts',(-9.83764223195818,-14.0832788793335,
117.812488378008)) ;
#157672=CARTESIAN_POINT('Ctrl Pts',(-9.91144606272761,-14.0832788338596,
117.78825729779)) ;
#157673=CARTESIAN_POINT('Ctrl Pts',(-9.98524989349704,-14.0832787883857,
117.764026217573)) ;
#157674=CARTESIAN_POINT('Ctrl Pts',(-9.96749871688968,-14.1335025434047,
117.709958996592)) ;
#157675=CARTESIAN_POINT('Ctrl Pts',(-9.94974754028233,-14.1837262984236,
117.655891775611)) ;
#157676=CARTESIAN_POINT('Ctrl Pts',(-9.87594370951292,-14.1837263438975,
117.680122855828)) ;
#157677=CARTESIAN_POINT('Ctrl Pts',(-9.80213987874348,-14.1837263893715,
117.704353936045)) ;
#157678=CARTESIAN_POINT('Ctrl Pts',(-9.81989105535084,-14.1335026343525,
117.758421157027)) ;
#157679=CARTESIAN_POINT('Ctrl Pts',(-9.78045273451247,-13.8914689377216,
117.602957988204)) ;
#157680=CARTESIAN_POINT('Ctrl Pts',(-9.80171425934229,-13.8580710694063,
117.667717163616)) ;
#157681=CARTESIAN_POINT('Ctrl Pts',(-9.87551809334006,-13.8580710084392,
117.643486093231)) ;
#157682=CARTESIAN_POINT('Ctrl Pts',(-9.94932192733782,-13.8580709474722,
117.619255022847)) ;
#157683=CARTESIAN_POINT('Ctrl Pts',(-9.92806040250799,-13.8914688157875,
117.554495847435)) ;
#157684=CARTESIAN_POINT('Ctrl Pts',(-9.90679887767815,-13.9248666841028,
117.489736672023)) ;
#157685=CARTESIAN_POINT('Ctrl Pts',(-9.83299504368039,-13.9248667450698,
117.513967742407)) ;
#157686=CARTESIAN_POINT('Ctrl Pts',(-9.75919120968263,-13.9248668060369,
117.538198812791)) ;
#157687=CARTESIAN_POINT('Ctrl Pts',(-9.78045273451247,-13.8914689377216,
117.602957988204)) ;
#157688=CARTESIAN_POINT('Ctrl Pts',(-9.76271568007487,-13.6147208150664,
117.513467417372)) ;
#157689=CARTESIAN_POINT('Ctrl Pts',(-9.78598021616308,-13.6005963890855,
117.584327442045)) ;
#157690=CARTESIAN_POINT('Ctrl Pts',(-9.85978405508859,-13.6005963145347,
117.56009638667)) ;
#157691=CARTESIAN_POINT('Ctrl Pts',(-9.93358789401411,-13.600596239984,
117.535865331294)) ;
#157692=CARTESIAN_POINT('Ctrl Pts',(-9.91032335792589,-13.6147206659649,
117.465005306621)) ;
#157693=CARTESIAN_POINT('Ctrl Pts',(-9.88705882183766,-13.6288450919457,
117.394145281948)) ;
#157694=CARTESIAN_POINT('Ctrl Pts',(-9.81325498291215,-13.6288451664965,
117.418376337323)) ;
#157695=CARTESIAN_POINT('Ctrl Pts',(-9.73945114398663,-13.6288452410473,
117.442607392699)) ;
#157696=CARTESIAN_POINT('Ctrl Pts',(-9.76271568007487,-13.6147208150664,
117.513467417372)) ;
#157697=CARTESIAN_POINT('Ctrl Pts',(-9.76890870119331,-13.3237687258409,
117.4968563122)) ;
#157698=CARTESIAN_POINT('Ctrl Pts',(-9.7925086415556,-13.3299371797537,
117.568737924317)) ;
#157699=CARTESIAN_POINT('Ctrl Pts',(-9.86631248703233,-13.3299370967314,
117.544506888895)) ;
#157700=CARTESIAN_POINT('Ctrl Pts',(-9.94011633250904,-13.329937013709,
117.520275853474)) ;
#157701=CARTESIAN_POINT('Ctrl Pts',(-9.91651639214676,-13.3237685597962,
117.448394241357)) ;
#157702=CARTESIAN_POINT('Ctrl Pts',(-9.89291645178446,-13.3176001058834,
117.376512629241)) ;
#157703=CARTESIAN_POINT('Ctrl Pts',(-9.81911260630774,-13.3176001889057,
117.400743664662)) ;
#157704=CARTESIAN_POINT('Ctrl Pts',(-9.74530876083102,-13.3176002719281,
117.424974700083)) ;
#157705=CARTESIAN_POINT('Ctrl Pts',(-9.76890870119331,-13.3237687258409,
117.4968563122)) ;
#157706=CARTESIAN_POINT('Ctrl Pts',(-9.79936071736111,-13.0396242352637,
117.554132453179)) ;
#157707=CARTESIAN_POINT('Ctrl Pts',(-9.82160297578344,-13.0656396906541,
117.621878785295)) ;
#157708=CARTESIAN_POINT('Ctrl Pts',(-9.89540682880252,-13.0656396062825,
117.597647772846)) ;
#157709=CARTESIAN_POINT('Ctrl Pts',(-9.96921068182159,-13.0656395219109,
117.573416760398)) ;
#157710=CARTESIAN_POINT('Ctrl Pts',(-9.94696842339928,-13.0396240665205,
117.505670428282)) ;
#157711=CARTESIAN_POINT('Ctrl Pts',(-9.92472616497694,-13.0136086111301,
117.437924096167)) ;
#157712=CARTESIAN_POINT('Ctrl Pts',(-9.85092231195787,-13.0136086955017,
117.462155108615)) ;
#157713=CARTESIAN_POINT('Ctrl Pts',(-9.77711845893878,-13.0136087798733,
117.486386121064)) ;
#157714=CARTESIAN_POINT('Ctrl Pts',(-9.79936071736111,-13.0396242352637,
117.554132453179)) ;
#157715=CARTESIAN_POINT('Ctrl Pts',(-9.85239927743223,-12.7830678889279,
117.680294085095)) ;
#157716=CARTESIAN_POINT('Ctrl Pts',(-9.87170308697766,-12.8270330002595,
117.73909037615)) ;
#157717=CARTESIAN_POINT('Ctrl Pts',(-9.94550694758217,-12.8270329227443,
117.714859386806)) ;
#157718=CARTESIAN_POINT('Ctrl Pts',(-10.0193108081867,-12.8270328452292,
117.690628397462)) ;
#157719=CARTESIAN_POINT('Ctrl Pts',(-10.0000069986413,-12.7830677338975,
117.631832106406)) ;
#157720=CARTESIAN_POINT('Ctrl Pts',(-9.98070318909583,-12.7391026225659,
117.573035815351)) ;
#157721=CARTESIAN_POINT('Ctrl Pts',(-9.90689932849131,-12.739102700081,
117.597266804696)) ;
#157722=CARTESIAN_POINT('Ctrl Pts',(-9.83309546788681,-12.7391027775962,
117.62149779404)) ;
#157723=CARTESIAN_POINT('Ctrl Pts',(-9.85239927743223,-12.7830678889279,
117.680294085095)) ;
#157724=CARTESIAN_POINT('Ctrl Pts',(-9.9257847579806,-12.5704752635878,
117.868146840537)) ;
#157725=CARTESIAN_POINT('Ctrl Pts',(-9.94073149886832,-12.6293473017033,
117.913672203583)) ;
#157726=CARTESIAN_POINT('Ctrl Pts',(-10.0145353667142,-12.6293472382111,
117.889441236294)) ;
#157727=CARTESIAN_POINT('Ctrl Pts',(-10.0883392345601,-12.6293471747189,
117.865210269006)) ;
#157728=CARTESIAN_POINT('Ctrl Pts',(-10.0733924936724,-12.5704751366034,
117.819684905961)) ;
#157729=CARTESIAN_POINT('Ctrl Pts',(-10.0584457527847,-12.5116030984879,
117.774159542916)) ;
#157730=CARTESIAN_POINT('Ctrl Pts',(-9.9846418849388,-12.5116031619801,
117.798390510204)) ;
#157731=CARTESIAN_POINT('Ctrl Pts',(-9.91083801709289,-12.5116032254723,
117.822621477492)) ;
#157732=CARTESIAN_POINT('Ctrl Pts',(-9.9257847579806,-12.5704752635878,
117.868146840537)) ;
#157733=CARTESIAN_POINT('Ctrl Pts',(-10.0135422022618,-12.4206416986158,
118.100172237485)) ;
#157734=CARTESIAN_POINT('Ctrl Pts',(-10.0231135704383,-12.490060480766,
118.129325082619)) ;
#157735=CARTESIAN_POINT('Ctrl Pts',(-10.0969174434593,-12.4900604392227,
118.105094131093)) ;
#157736=CARTESIAN_POINT('Ctrl Pts',(-10.1707213164804,-12.4900603976793,
118.080863179567)) ;
#157737=CARTESIAN_POINT('Ctrl Pts',(-10.1611499483039,-12.4206416155292,
118.051710334434)) ;
#157738=CARTESIAN_POINT('Ctrl Pts',(-10.1515785801275,-12.351222833379,
118.0225574893)) ;
#157739=CARTESIAN_POINT('Ctrl Pts',(-10.0777747071064,-12.3512228749223,
118.046788440826)) ;
#157740=CARTESIAN_POINT('Ctrl Pts',(-10.0039708340854,-12.3512229164656,
118.071019392351)) ;
#157741=CARTESIAN_POINT('Ctrl Pts',(-10.0135422022618,-12.4206416986158,
118.100172237485)) ;
#157742=CARTESIAN_POINT('Ctrl Pts',(-10.1114862816905,-12.3408954926335,
118.363002383417)) ;
#157743=CARTESIAN_POINT('Ctrl Pts',(-10.114968062946,-12.4159838825569,
118.373607329397)) ;
#157744=CARTESIAN_POINT('Ctrl Pts',(-10.1887719392433,-12.4159838672949,
118.34937638785)) ;
#157745=CARTESIAN_POINT('Ctrl Pts',(-10.2625758155405,-12.4159838520328,
118.325145446303)) ;
#157746=CARTESIAN_POINT('Ctrl Pts',(-10.259094034285,-12.3408954621094,
118.314540500324)) ;
#157747=CARTESIAN_POINT('Ctrl Pts',(-10.2556122530295,-12.265807072186,
118.303935554344)) ;
#157748=CARTESIAN_POINT('Ctrl Pts',(-10.1818083767322,-12.265807087448,
118.32816649589)) ;
#157749=CARTESIAN_POINT('Ctrl Pts',(-10.1080045004349,-12.26580710271,118.352397437437)) ;
#157750=CARTESIAN_POINT('Ctrl Pts',(-10.1114862816905,-12.3408954926335,
118.363002383417)) ;
#157751=CARTESIAN_POINT('Ctrl Pts',(-10.2131168846024,-12.3388375024718,
118.636985267721)) ;
#157752=CARTESIAN_POINT('Ctrl Pts',(-10.2102443248058,-12.4141806587766,
118.628235916156)) ;
#157753=CARTESIAN_POINT('Ctrl Pts',(-10.2840482016702,-12.414180672439,
118.604004976337)) ;
#157754=CARTESIAN_POINT('Ctrl Pts',(-10.3578520785346,-12.4141806861015,
118.579774036517)) ;
#157755=CARTESIAN_POINT('Ctrl Pts',(-10.3607246383311,-12.3388375297967,
118.588523388082)) ;
#157756=CARTESIAN_POINT('Ctrl Pts',(-10.3635971981277,-12.263494373492,
118.597272739647)) ;
#157757=CARTESIAN_POINT('Ctrl Pts',(-10.2897933212633,-12.2634943598295,
118.621503679467)) ;
#157758=CARTESIAN_POINT('Ctrl Pts',(-10.2159894443989,-12.2634943461671,
118.645734619286)) ;
#157759=CARTESIAN_POINT('Ctrl Pts',(-10.2131168846024,-12.3388375024718,
118.636985267721)) ;
#157760=CARTESIAN_POINT('Ctrl Pts',(-10.3111631418804,-12.413706142133,
118.900239883285)) ;
#157761=CARTESIAN_POINT('Ctrl Pts',(-10.3021731424948,-12.4839334398815,
118.872857797784)) ;
#157762=CARTESIAN_POINT('Ctrl Pts',(-10.3759770171298,-12.4839334817003,
118.848626851174)) ;
#157763=CARTESIAN_POINT('Ctrl Pts',(-10.4497808917647,-12.4839335235192,
118.824395904564)) ;
#157764=CARTESIAN_POINT('Ctrl Pts',(-10.4587708911503,-12.4137062257707,
118.851777990065)) ;
#157765=CARTESIAN_POINT('Ctrl Pts',(-10.4677608905359,-12.3434789280223,
118.879160075566)) ;
#157766=CARTESIAN_POINT('Ctrl Pts',(-10.3939570159009,-12.3434788862035,
118.903391022176)) ;
#157767=CARTESIAN_POINT('Ctrl Pts',(-10.3201531412659,-12.3434788443846,
118.927621968785)) ;
#157768=CARTESIAN_POINT('Ctrl Pts',(-10.3111631418804,-12.413706142133,
118.900239883285)) ;
#157769=CARTESIAN_POINT('Ctrl Pts',(-10.4005037459975,-12.5617183582742,
119.136700846574)) ;
#157770=CARTESIAN_POINT('Ctrl Pts',(-10.3860007082531,-12.6217168854957,
119.092526935736)) ;
#157771=CARTESIAN_POINT('Ctrl Pts',(-10.4598045779934,-12.6217169518503,
119.068295974218)) ;
#157772=CARTESIAN_POINT('Ctrl Pts',(-10.5336084477337,-12.6217170182048,
119.044065012699)) ;
#157773=CARTESIAN_POINT('Ctrl Pts',(-10.5481114854781,-12.5617184909834,
119.088238923537)) ;
#157774=CARTESIAN_POINT('Ctrl Pts',(-10.5626145232225,-12.501719963762,
119.132412834375)) ;
#157775=CARTESIAN_POINT('Ctrl Pts',(-10.4888106534822,-12.5017198974074,
119.156643795893)) ;
#157776=CARTESIAN_POINT('Ctrl Pts',(-10.4150067837419,-12.5017198310528,
119.180874757412)) ;
#157777=CARTESIAN_POINT('Ctrl Pts',(-10.4005037459975,-12.5617183582742,
119.136700846574)) ;
#157778=CARTESIAN_POINT('Ctrl Pts',(-10.4738998219897,-12.7688407831079,
119.325034793762)) ;
#157779=CARTESIAN_POINT('Ctrl Pts',(-10.4549797292597,-12.8144672602671,
119.267407246099)) ;
#157780=CARTESIAN_POINT('Ctrl Pts',(-10.5287835923174,-12.8144673453734,
119.243176264227)) ;
#157781=CARTESIAN_POINT('Ctrl Pts',(-10.6025874553752,-12.8144674304797,
119.218945282355)) ;
#157782=CARTESIAN_POINT('Ctrl Pts',(-10.6215075481052,-12.7688409533206,
119.276572830018)) ;
#157783=CARTESIAN_POINT('Ctrl Pts',(-10.6404276408353,-12.7232144761614,
119.334200377682)) ;
#157784=CARTESIAN_POINT('Ctrl Pts',(-10.5666237777775,-12.7232143910551,
119.358431359554)) ;
#157785=CARTESIAN_POINT('Ctrl Pts',(-10.4928199147197,-12.7232143059487,
119.382662341426)) ;
#157786=CARTESIAN_POINT('Ctrl Pts',(-10.4738998219897,-12.7688407831079,
119.325034793762)) ;
#157787=CARTESIAN_POINT('Ctrl Pts',(-10.528497781938,-13.0241117816514,
119.455791678547)) ;
#157788=CARTESIAN_POINT('Ctrl Pts',(-10.5064729183125,-13.0519843902153,
119.388707499628)) ;
#157789=CARTESIAN_POINT('Ctrl Pts',(-10.580276773221,-13.0519844861314,
119.364476492934)) ;
#157790=CARTESIAN_POINT('Ctrl Pts',(-10.6540806281294,-13.0519845820475,
119.34024548624)) ;
#157791=CARTESIAN_POINT('Ctrl Pts',(-10.6761054917549,-13.0241119734836,
119.407329665159)) ;
#157792=CARTESIAN_POINT('Ctrl Pts',(-10.6981303553804,-12.9962393649197,
119.474413844078)) ;
#157793=CARTESIAN_POINT('Ctrl Pts',(-10.624326500472,-12.9962392690036,
119.498644850772)) ;
#157794=CARTESIAN_POINT('Ctrl Pts',(-10.5505226455635,-12.9962391730874,
119.522875857466)) ;
#157795=CARTESIAN_POINT('Ctrl Pts',(-10.528497781938,-13.0241117816514,
119.455791678547)) ;
#157796=CARTESIAN_POINT('Ctrl Pts',(-10.5602307777131,-13.3070010234793,
119.517011250028)) ;
#157797=CARTESIAN_POINT('Ctrl Pts',(-10.5366906221351,-13.31516473517,119.445311736237)) ;
#157798=CARTESIAN_POINT('Ctrl Pts',(-10.6104944685515,-13.3151648334865,
119.421080703678)) ;
#157799=CARTESIAN_POINT('Ctrl Pts',(-10.684298314968,-13.315164931803,119.396849671119)) ;
#157800=CARTESIAN_POINT('Ctrl Pts',(-10.7078384705459,-13.3070012201123,
119.46854918491)) ;
#157801=CARTESIAN_POINT('Ctrl Pts',(-10.7313786261238,-13.2988375084216,
119.540248698701)) ;
#157802=CARTESIAN_POINT('Ctrl Pts',(-10.6575747797074,-13.2988374101051,
119.56447973126)) ;
#157803=CARTESIAN_POINT('Ctrl Pts',(-10.583770933291,-13.2988373117886,
119.588710763819)) ;
#157804=CARTESIAN_POINT('Ctrl Pts',(-10.5602307777131,-13.3070010234793,
119.517011250028)) ;
#157805=CARTESIAN_POINT('Ctrl Pts',(-10.5678547390295,-13.5985554109386,
119.504704332823)) ;
#157806=CARTESIAN_POINT('Ctrl Pts',(-10.5444820245611,-13.5863758262572,
119.43351481753)) ;
#157807=CARTESIAN_POINT('Ctrl Pts',(-10.6182858629544,-13.5863759182584,
119.409283760534)) ;
#157808=CARTESIAN_POINT('Ctrl Pts',(-10.6920897013477,-13.5863760102596,
119.385052703538)) ;
#157809=CARTESIAN_POINT('Ctrl Pts',(-10.7154624158161,-13.5985555949411,
119.45624221883)) ;
#157810=CARTESIAN_POINT('Ctrl Pts',(-10.7388351302845,-13.6107351796225,
119.527431734122)) ;
#157811=CARTESIAN_POINT('Ctrl Pts',(-10.6650312918912,-13.6107350876213,
119.551662791119)) ;
#157812=CARTESIAN_POINT('Ctrl Pts',(-10.5912274534979,-13.6107349956201,
119.575893848115)) ;
#157813=CARTESIAN_POINT('Ctrl Pts',(-10.5678547390295,-13.5985554109386,
119.504704332823)) ;
#157814=CARTESIAN_POINT('Ctrl Pts',(-10.5513598758863,-13.8770852609277,
119.418937728725)) ;
#157815=CARTESIAN_POINT('Ctrl Pts',(-10.5298386410176,-13.8454408144546,
119.353387521432)) ;
#157816=CARTESIAN_POINT('Ctrl Pts',(-10.6036424728301,-13.8454408929621,
119.329156444392)) ;
#157817=CARTESIAN_POINT('Ctrl Pts',(-10.6774463046426,-13.8454409714697,
119.304925367352)) ;
#157818=CARTESIAN_POINT('Ctrl Pts',(-10.6989675395113,-13.8770854179428,
119.370475574645)) ;
#157819=CARTESIAN_POINT('Ctrl Pts',(-10.72048877438,-13.9087298644159,119.436025781938)) ;
#157820=CARTESIAN_POINT('Ctrl Pts',(-10.6466849425675,-13.9087297859083,
119.460256858978)) ;
#157821=CARTESIAN_POINT('Ctrl Pts',(-10.572881110755,-13.9087297074008,
119.484487936018)) ;
#157822=CARTESIAN_POINT('Ctrl Pts',(-10.5513598758863,-13.8770852609277,
119.418937728725)) ;
#157823=CARTESIAN_POINT('Ctrl Pts',(-10.5130330103292,-14.1214182763711,
119.266862919213)) ;
#157824=CARTESIAN_POINT('Ctrl Pts',(-10.4948865671328,-14.0726671201406,
119.21159178272)) ;
#157825=CARTESIAN_POINT('Ctrl Pts',(-10.5686903940646,-14.0726671815673,
119.187360690814)) ;
#157826=CARTESIAN_POINT('Ctrl Pts',(-10.6424942209963,-14.072667242994,
119.163129598908)) ;
#157827=CARTESIAN_POINT('Ctrl Pts',(-10.6606406641927,-14.1214183992245,
119.2184007354)) ;
#157828=CARTESIAN_POINT('Ctrl Pts',(-10.6787871073891,-14.170169555455,
119.273671871893)) ;
#157829=CARTESIAN_POINT('Ctrl Pts',(-10.6049832804574,-14.1701694940283,
119.297902963799)) ;
#157830=CARTESIAN_POINT('Ctrl Pts',(-10.5311794535256,-14.1701694326015,
119.322134055705)) ;
#157831=CARTESIAN_POINT('Ctrl Pts',(-10.5130330103292,-14.1214182763711,
119.266862919213)) ;
#157832=CARTESIAN_POINT('Ctrl Pts',(-10.4561208615973,-14.3164119676812,
119.058063869766)) ;
#157833=CARTESIAN_POINT('Ctrl Pts',(-10.4426541691121,-14.2539728440819,
119.017046498723)) ;
#157834=CARTESIAN_POINT('Ctrl Pts',(-10.5164579934008,-14.2539728850066,
118.992815398767)) ;
#157835=CARTESIAN_POINT('Ctrl Pts',(-10.5902618176896,-14.2539729259314,
118.968584298811)) ;
#157836=CARTESIAN_POINT('Ctrl Pts',(-10.6037285101748,-14.3164120495308,
119.009601669854)) ;
#157837=CARTESIAN_POINT('Ctrl Pts',(-10.6171952026601,-14.3788511731302,
119.050619040897)) ;
#157838=CARTESIAN_POINT('Ctrl Pts',(-10.5433913783713,-14.3788511322054,
119.074850140853)) ;
#157839=CARTESIAN_POINT('Ctrl Pts',(-10.4695875540826,-14.3788510912806,
119.099081240809)) ;
#157840=CARTESIAN_POINT('Ctrl Pts',(-10.4561208615973,-14.3164119676812,
119.058063869766)) ;
#157841=CARTESIAN_POINT('Ctrl Pts',(-10.3852189870946,-14.4472714989735,
118.806537992562)) ;
#157842=CARTESIAN_POINT('Ctrl Pts',(-10.3774182459339,-14.3756009231922,
118.782778194882)) ;
#157843=CARTESIAN_POINT('Ctrl Pts',(-10.4512220701755,-14.3756009434077,
118.758547094782)) ;
#157844=CARTESIAN_POINT('Ctrl Pts',(-10.525025894417,-14.3756009636232,
118.734315994681)) ;
#157845=CARTESIAN_POINT('Ctrl Pts',(-10.5328266355777,-14.4472715394045,
118.758075792362)) ;
#157846=CARTESIAN_POINT('Ctrl Pts',(-10.5406273767383,-14.5189421151858,
118.781835590042)) ;
#157847=CARTESIAN_POINT('Ctrl Pts',(-10.4668235524968,-14.5189420949703,
118.806066690143)) ;
#157848=CARTESIAN_POINT('Ctrl Pts',(-10.3930197282553,-14.5189420747548,
118.830297790243)) ;
#157849=CARTESIAN_POINT('Ctrl Pts',(-10.3852189870946,-14.4472714989735,
118.806537992562)) ;
#157850=CARTESIAN_POINT('Ctrl Pts',(-10.3066385089528,-14.5039655219921,
118.531734459687)) ;
#157851=CARTESIAN_POINT('Ctrl Pts',(-10.305046250753,-14.4282278620231,
118.526884699208)) ;
#157852=CARTESIAN_POINT('Ctrl Pts',(-10.37885007664,-14.4282278646451,118.502653604119)) ;
#157853=CARTESIAN_POINT('Ctrl Pts',(-10.4526539025269,-14.4282278672671,
118.47842250903)) ;
#157854=CARTESIAN_POINT('Ctrl Pts',(-10.4542461607266,-14.5039655272361,
118.48327226951)) ;
#157855=CARTESIAN_POINT('Ctrl Pts',(-10.4558384189264,-14.5797031872051,
118.48812202999)) ;
#157856=CARTESIAN_POINT('Ctrl Pts',(-10.3820345930394,-14.5797031845831,
118.512353125078)) ;
#157857=CARTESIAN_POINT('Ctrl Pts',(-10.3082307671525,-14.5797031819611,
118.536584220167)) ;
#157858=CARTESIAN_POINT('Ctrl Pts',(-10.3066385089528,-14.5039655219921,
118.531734459687)) ;
#157859=CARTESIAN_POINT('Ctrl Pts',(-10.2263549450695,-14.4826373105238,
118.251644902637)) ;
#157860=CARTESIAN_POINT('Ctrl Pts',(-10.2311016200229,-14.4082736216989,
118.266102509573)) ;
#157861=CARTESIAN_POINT('Ctrl Pts',(-10.3049054492475,-14.4082736113454,
118.24187142465)) ;
#157862=CARTESIAN_POINT('Ctrl Pts',(-10.378709278472,-14.4082736009919,
118.217640339728)) ;
#157863=CARTESIAN_POINT('Ctrl Pts',(-10.3739626035186,-14.4826372898169,
118.203182732792)) ;
#157864=CARTESIAN_POINT('Ctrl Pts',(-10.3692159285652,-14.5570009786418,
118.188725125855)) ;
#157865=CARTESIAN_POINT('Ctrl Pts',(-10.2954120993406,-14.5570009889953,
118.212956210778)) ;
#157866=CARTESIAN_POINT('Ctrl Pts',(-10.2216082701161,-14.5570009993487,
118.237187295701)) ;
#157867=CARTESIAN_POINT('Ctrl Pts',(-10.2263549450695,-14.4826373105238,
118.251644902637)) ;
#157868=CARTESIAN_POINT('Ctrl Pts',(-10.1515928117172,-14.3855815012644,
117.988618093193)) ;
#157869=CARTESIAN_POINT('Ctrl Pts',(-10.1622974516462,-14.3178820902551,
118.021222699991)) ;
#157870=CARTESIAN_POINT('Ctrl Pts',(-10.2361012842216,-14.3178820716342,
117.996991625275)) ;
#157871=CARTESIAN_POINT('Ctrl Pts',(-10.309905116797,-14.3178820530132,
117.972760550558)) ;
#157872=CARTESIAN_POINT('Ctrl Pts',(-10.299200476868,-14.3855814640225,
117.94015594376)) ;
#157873=CARTESIAN_POINT('Ctrl Pts',(-10.288495836939,-14.4532808750318,
117.907551336961)) ;
#157874=CARTESIAN_POINT('Ctrl Pts',(-10.2146920043635,-14.4532808936528,
117.931782411678)) ;
#157875=CARTESIAN_POINT('Ctrl Pts',(-10.1408881717881,-14.4532809122737,
117.956013486395)) ;
#157876=CARTESIAN_POINT('Ctrl Pts',(-10.1515928117172,-14.3855815012644,
117.988618093193)) ;
#157877=CARTESIAN_POINT('Ctrl Pts',(-10.0875742094217,-14.2190969785884,
117.758158308275)) ;
#157878=CARTESIAN_POINT('Ctrl Pts',(-10.1034990260791,-14.1629192872983,
117.806662730949)) ;
#157879=CARTESIAN_POINT('Ctrl Pts',(-10.1773028625826,-14.1629192658567,
117.782431668197)) ;
#157880=CARTESIAN_POINT('Ctrl Pts',(-10.2511066990861,-14.1629192444152,
117.758200605445)) ;
#157881=CARTESIAN_POINT('Ctrl Pts',(-10.2351818824287,-14.2190969357053,
117.709696182771)) ;
#157882=CARTESIAN_POINT('Ctrl Pts',(-10.2192570657713,-14.2752746269954,
117.661191760097)) ;
#157883=CARTESIAN_POINT('Ctrl Pts',(-10.1454532292678,-14.275274648437,
117.685422822849)) ;
#157884=CARTESIAN_POINT('Ctrl Pts',(-10.0716493927643,-14.2752746698786,
117.709653885601)) ;
#157885=CARTESIAN_POINT('Ctrl Pts',(-10.0875742094217,-14.2190969785884,
117.758158308275)) ;
#157886=CARTESIAN_POINT('Ctrl Pts',(-10.0400271797391,-13.9949296481822,
117.577849034879)) ;
#157887=CARTESIAN_POINT('Ctrl Pts',(-10.0600304577515,-13.9543190677503,
117.638775792622)) ;
#157888=CARTESIAN_POINT('Ctrl Pts',(-10.1338342976265,-13.9543190483412,
117.614544740138)) ;
#157889=CARTESIAN_POINT('Ctrl Pts',(-10.2076381375015,-13.9543190289321,
117.590313687655)) ;
#157890=CARTESIAN_POINT('Ctrl Pts',(-10.1876348594891,-13.9949296093639,
117.529386929912)) ;
#157891=CARTESIAN_POINT('Ctrl Pts',(-10.1676315814767,-14.0355401897957,
117.468460172169)) ;
#157892=CARTESIAN_POINT('Ctrl Pts',(-10.0938277416017,-14.0355402092049,
117.492691224653)) ;
#157893=CARTESIAN_POINT('Ctrl Pts',(-10.0200239017268,-14.035540228614,
117.516922277136)) ;
#157894=CARTESIAN_POINT('Ctrl Pts',(-10.0400271797391,-13.9949296481822,
117.577849034879)) ;
#157895=CARTESIAN_POINT('Ctrl Pts',(-10.013089520595,-13.7298783707897,
117.46036854867)) ;
#157896=CARTESIAN_POINT('Ctrl Pts',(-10.0357371803655,-13.7077134495774,
117.529349666438)) ;
#157897=CARTESIAN_POINT('Ctrl Pts',(-10.1095410226297,-13.7077134348718,
117.505118621232)) ;
#157898=CARTESIAN_POINT('Ctrl Pts',(-10.1833448648939,-13.7077134201661,
117.480887576025)) ;
#157899=CARTESIAN_POINT('Ctrl Pts',(-10.1606972051234,-13.7298783413784,
117.411906458258)) ;
#157900=CARTESIAN_POINT('Ctrl Pts',(-10.138049545353,-13.7520432625907,
117.342925340491)) ;
#157901=CARTESIAN_POINT('Ctrl Pts',(-10.0642457030888,-13.7520432772964,
117.367156385697)) ;
#157902=CARTESIAN_POINT('Ctrl Pts',(-9.99044186082453,-13.752043292002,
117.391387430903)) ;
#157903=CARTESIAN_POINT('Ctrl Pts',(-10.013089520595,-13.7298783707897,
117.46036854867)) ;
#157904=CARTESIAN_POINT('Ctrl Pts',(-10.0095205229371,-13.4411780607526,
117.413901364897)) ;
#157905=CARTESIAN_POINT('Ctrl Pts',(-10.033188325731,-13.4391385958436,
117.485989673571)) ;
#157906=CARTESIAN_POINT('Ctrl Pts',(-10.1069921692462,-13.4391385881017,
117.461758632175)) ;
#157907=CARTESIAN_POINT('Ctrl Pts',(-10.1807960127614,-13.4391385803598,
117.437527590779)) ;
#157908=CARTESIAN_POINT('Ctrl Pts',(-10.1571282099675,-13.4411780452688,
117.365439282106)) ;
#157909=CARTESIAN_POINT('Ctrl Pts',(-10.1334604071736,-13.4432175101778,
117.293350973432)) ;
#157910=CARTESIAN_POINT('Ctrl Pts',(-10.0596565636584,-13.4432175179197,
117.317582014828)) ;
#157911=CARTESIAN_POINT('Ctrl Pts',(-9.98585272014315,-13.4432175256616,
117.341813056224)) ;
#157912=CARTESIAN_POINT('Ctrl Pts',(-10.0095205229371,-13.4411780607526,
117.413901364897)) ;
#157913=CARTESIAN_POINT('Ctrl Pts',(-10.0300438994439,-13.1535366585443,
117.441164670617)) ;
#157914=CARTESIAN_POINT('Ctrl Pts',(-10.0530434647087,-13.1715786657878,
117.511217635516)) ;
#157915=CARTESIAN_POINT('Ctrl Pts',(-10.1268473085128,-13.1715786624699,
117.486986595)) ;
#157916=CARTESIAN_POINT('Ctrl Pts',(-10.2006511523169,-13.1715786591521,
117.462755554485)) ;
#157917=CARTESIAN_POINT('Ctrl Pts',(-10.1776515870522,-13.1535366519086,
117.392702589586)) ;
#157918=CARTESIAN_POINT('Ctrl Pts',(-10.1546520217874,-13.1354946446651,
117.322649624687)) ;
#157919=CARTESIAN_POINT('Ctrl Pts',(-10.0808481779833,-13.1354946479829,
117.346880665203)) ;
#157920=CARTESIAN_POINT('Ctrl Pts',(-10.0070443341792,-13.1354946513008,
117.371111705719)) ;
#157921=CARTESIAN_POINT('Ctrl Pts',(-10.0300438994439,-13.1535366585443,
117.441164670617)) ;
#157922=CARTESIAN_POINT('Ctrl Pts',(-10.0745982760158,-12.8812078446008,
117.541146052817)) ;
#157923=CARTESIAN_POINT('Ctrl Pts',(-10.0952606474382,-12.9182937200929,
117.604080302277)) ;
#157924=CARTESIAN_POINT('Ctrl Pts',(-10.1690644906924,-12.9182937216163,
117.579849260086)) ;
#157925=CARTESIAN_POINT('Ctrl Pts',(-10.2428683339466,-12.9182937231397,
117.555618217895)) ;
#157926=CARTESIAN_POINT('Ctrl Pts',(-10.2222059625242,-12.8812078476476,
117.492683968435)) ;
#157927=CARTESIAN_POINT('Ctrl Pts',(-10.2015435911017,-12.8441219721555,
117.429749718974)) ;
#157928=CARTESIAN_POINT('Ctrl Pts',(-10.1277397478476,-12.8441219706321,
117.453980761165)) ;
#157929=CARTESIAN_POINT('Ctrl Pts',(-10.0539359045934,-12.8441219691087,
117.478211803356)) ;
#157930=CARTESIAN_POINT('Ctrl Pts',(-10.0745982760158,-12.8812078446008,
117.541146052817)) ;
#157931=CARTESIAN_POINT('Ctrl Pts',(-10.1399166575301,-12.6502697095916,
117.704747539768)) ;
#157932=CARTESIAN_POINT('Ctrl Pts',(-10.1567801601785,-12.7035365652379,
117.756111047861)) ;
#157933=CARTESIAN_POINT('Ctrl Pts',(-10.2305840029382,-12.7035365674139,
117.731880004164)) ;
#157934=CARTESIAN_POINT('Ctrl Pts',(-10.304387845698,-12.7035365695899,
117.707648960467)) ;
#157935=CARTESIAN_POINT('Ctrl Pts',(-10.2875243430495,-12.6502697139436,
117.656285452374)) ;
#157936=CARTESIAN_POINT('Ctrl Pts',(-10.2706608404011,-12.5970028582972,
117.604921944281)) ;
#157937=CARTESIAN_POINT('Ctrl Pts',(-10.1968569976414,-12.5970028561212,
117.629152987977)) ;
#157938=CARTESIAN_POINT('Ctrl Pts',(-10.1230531548816,-12.5970028539452,
117.653384031674)) ;
#157939=CARTESIAN_POINT('Ctrl Pts',(-10.1399166575301,-12.6502697095916,
117.704747539768)) ;
#157940=CARTESIAN_POINT('Ctrl Pts',(-10.2222158366404,-12.4736381112203,
117.920071829275)) ;
#157941=CARTESIAN_POINT('Ctrl Pts',(-10.2340889281916,-12.5393175291298,
117.95623535036)) ;
#157942=CARTESIAN_POINT('Ctrl Pts',(-10.3078927706903,-12.5393175306857,
117.932004305868)) ;
#157943=CARTESIAN_POINT('Ctrl Pts',(-10.381696613189,-12.5393175322416,
117.907773261376)) ;
#157944=CARTESIAN_POINT('Ctrl Pts',(-10.3698235216379,-12.473638114332,
117.871609740292)) ;
#157945=CARTESIAN_POINT('Ctrl Pts',(-10.3579504300867,-12.4079586964224,
117.835446219207)) ;
#157946=CARTESIAN_POINT('Ctrl Pts',(-10.284146587588,-12.4079586948666,
117.859677263699)) ;
#157947=CARTESIAN_POINT('Ctrl Pts',(-10.2103427450893,-12.4079586933107,
117.883908308191)) ;
#157948=CARTESIAN_POINT('Ctrl Pts',(-10.2222158366404,-12.4736381112203,
117.920071829275)) ;
#157949=CARTESIAN_POINT('Ctrl Pts',(-10.3174784950143,-12.3636957343507,
118.174552893488)) ;
#157950=CARTESIAN_POINT('Ctrl Pts',(-10.3234552555865,-12.4371496799271,
118.192757141833)) ;
#157951=CARTESIAN_POINT('Ctrl Pts',(-10.397259098797,-12.4371496797509,
118.168526099509)) ;
#157952=CARTESIAN_POINT('Ctrl Pts',(-10.4710629420074,-12.4371496795748,
118.144295057185)) ;
#157953=CARTESIAN_POINT('Ctrl Pts',(-10.4650861814352,-12.3636957339984,
118.126090808839)) ;
#157954=CARTESIAN_POINT('Ctrl Pts',(-10.459109420863,-12.290241788422,118.107886560494)) ;
#157955=CARTESIAN_POINT('Ctrl Pts',(-10.3853055776525,-12.2902417885981,
118.132117602818)) ;
#157956=CARTESIAN_POINT('Ctrl Pts',(-10.3115017344421,-12.2902417887743,
118.156348645142)) ;
#157957=CARTESIAN_POINT('Ctrl Pts',(-10.3174784950143,-12.3636957343507,
118.174552893488)) ;
#157958=CARTESIAN_POINT('Ctrl Pts',(-10.4179636590566,-12.3303161657527,
118.445239950958)) ;
#157959=CARTESIAN_POINT('Ctrl Pts',(-10.4176647566625,-12.4062080741742,
118.444329542558)) ;
#157960=CARTESIAN_POINT('Ctrl Pts',(-10.4914686010974,-12.4062080738796,
118.420098503963)) ;
#157961=CARTESIAN_POINT('Ctrl Pts',(-10.5652724455322,-12.406208073585,
118.395867465368)) ;
#157962=CARTESIAN_POINT('Ctrl Pts',(-10.5655713479262,-12.3303161651636,
118.396777873769)) ;
#157963=CARTESIAN_POINT('Ctrl Pts',(-10.5658702503203,-12.2544242567421,
118.39768828217)) ;
#157964=CARTESIAN_POINT('Ctrl Pts',(-10.4920664058854,-12.2544242570367,
118.421919320765)) ;
#157965=CARTESIAN_POINT('Ctrl Pts',(-10.4182625614506,-12.2544242573313,
118.446150359359)) ;
#157966=CARTESIAN_POINT('Ctrl Pts',(-10.4179636590566,-12.3303161657527,
118.445239950958)) ;
#157967=CARTESIAN_POINT('Ctrl Pts',(-10.5180970410555,-12.3741418831008,
118.71482587813)) ;
#157968=CARTESIAN_POINT('Ctrl Pts',(-10.511538602985,-12.4470842325009,
118.694849934126)) ;
#157969=CARTESIAN_POINT('Ctrl Pts',(-10.5853424489065,-12.447084234237,
118.67061890006)) ;
#157970=CARTESIAN_POINT('Ctrl Pts',(-10.6591462948279,-12.4470842359731,
118.646387865993)) ;
#157971=CARTESIAN_POINT('Ctrl Pts',(-10.6657047328985,-12.374141886573,
118.666363809997)) ;
#157972=CARTESIAN_POINT('Ctrl Pts',(-10.672263170969,-12.3011995371729,
118.686339754001)) ;
#157973=CARTESIAN_POINT('Ctrl Pts',(-10.5984593250475,-12.3011995354367,
118.710570788068)) ;
#157974=CARTESIAN_POINT('Ctrl Pts',(-10.524655479126,-12.3011995337006,
118.734801822134)) ;
#157975=CARTESIAN_POINT('Ctrl Pts',(-10.5180970410555,-12.3741418831008,
118.71482587813)) ;
#157976=CARTESIAN_POINT('Ctrl Pts',(-10.611946558723,-12.4937241519796,
118.965043678186)) ;
#157977=CARTESIAN_POINT('Ctrl Pts',(-10.5995629169345,-12.5584232360499,
118.927325103705)) ;
#157978=CARTESIAN_POINT('Ctrl Pts',(-10.6733667647407,-12.5584232440279,
118.903094075379)) ;
#157979=CARTESIAN_POINT('Ctrl Pts',(-10.7471706125469,-12.558423252006,
118.878863047052)) ;
#157980=CARTESIAN_POINT('Ctrl Pts',(-10.7595542543354,-12.4937241679357,
118.916581621534)) ;
#157981=CARTESIAN_POINT('Ctrl Pts',(-10.7719378961239,-12.4290250838654,
118.954300196015)) ;
#157982=CARTESIAN_POINT('Ctrl Pts',(-10.6981340483176,-12.4290250758873,
118.978531224342)) ;
#157983=CARTESIAN_POINT('Ctrl Pts',(-10.6243302005114,-12.4290250679093,
119.002762252668)) ;
#157984=CARTESIAN_POINT('Ctrl Pts',(-10.611946558723,-12.4937241519796,
118.965043678186)) ;
#157985=CARTESIAN_POINT('Ctrl Pts',(-10.6922395149728,-12.6783961032596,
119.174263610413)) ;
#157986=CARTESIAN_POINT('Ctrl Pts',(-10.6749630709864,-12.7302945007164,
119.121642350014)) ;
#157987=CARTESIAN_POINT('Ctrl Pts',(-10.7487669193606,-12.7302945169849,
119.097411323418)) ;
#157988=CARTESIAN_POINT('Ctrl Pts',(-10.8225707677349,-12.7302945332533,
119.073180296822)) ;
#157989=CARTESIAN_POINT('Ctrl Pts',(-10.8398472117212,-12.6783961357965,
119.125801557221)) ;
#157990=CARTESIAN_POINT('Ctrl Pts',(-10.8571236557076,-12.6264977383397,
119.17842281762)) ;
#157991=CARTESIAN_POINT('Ctrl Pts',(-10.7833198073334,-12.6264977220713,
119.202653844216)) ;
#157992=CARTESIAN_POINT('Ctrl Pts',(-10.7095159589592,-12.6264977058028,
119.226884870812)) ;
#157993=CARTESIAN_POINT('Ctrl Pts',(-10.6922395149728,-12.6783961032596,
119.174263610413)) ;
#157994=CARTESIAN_POINT('Ctrl Pts',(-10.7550368562695,-12.9163766433386,
119.330077430903)) ;
#157995=CARTESIAN_POINT('Ctrl Pts',(-10.7340845279254,-12.951734042377,
119.266260020007)) ;
#157996=CARTESIAN_POINT('Ctrl Pts',(-10.8078883759639,-12.9517340693484,
119.242028992389)) ;
#157997=CARTESIAN_POINT('Ctrl Pts',(-10.8816922240024,-12.9517340963197,
119.21779796477)) ;
#157998=CARTESIAN_POINT('Ctrl Pts',(-10.9026445523466,-12.9163766972813,
119.281615375666)) ;
#157999=CARTESIAN_POINT('Ctrl Pts',(-10.9235968806907,-12.8810192982428,
119.345432786561)) ;
#158000=CARTESIAN_POINT('Ctrl Pts',(-10.8497930326522,-12.8810192712715,
119.36966381418)) ;
#158001=CARTESIAN_POINT('Ctrl Pts',(-10.7759891846136,-12.8810192443002,
119.393894841798)) ;
#158002=CARTESIAN_POINT('Ctrl Pts',(-10.7550368562695,-12.9163766433386,
119.330077430903)) ;
#158003=CARTESIAN_POINT('Ctrl Pts',(-10.7962673301715,-13.1903758945546,
119.420199225543)) ;
#158004=CARTESIAN_POINT('Ctrl Pts',(-10.7731397430985,-13.2066536724704,
119.3497563277)) ;
#158005=CARTESIAN_POINT('Ctrl Pts',(-10.8469435893136,-13.206653710727,
119.325525294528)) ;
#158006=CARTESIAN_POINT('Ctrl Pts',(-10.9207474355287,-13.2066537489837,
119.301294261356)) ;
#158007=CARTESIAN_POINT('Ctrl Pts',(-10.9438750226017,-13.1903759710679,
119.371737159198)) ;
#158008=CARTESIAN_POINT('Ctrl Pts',(-10.9670026096747,-13.1740981931521,
119.442180057041)) ;
#158009=CARTESIAN_POINT('Ctrl Pts',(-10.8931987634596,-13.1740981548955,
119.466411090213)) ;
#158010=CARTESIAN_POINT('Ctrl Pts',(-10.8193949172445,-13.1740981166388,
119.490642123386)) ;
#158011=CARTESIAN_POINT('Ctrl Pts',(-10.7962673301715,-13.1903758945546,
119.420199225543)) ;
#158012=CARTESIAN_POINT('Ctrl Pts',(-10.8137492360295,-13.481432819081,
119.437894714578)) ;
#158013=CARTESIAN_POINT('Ctrl Pts',(-10.7901032169059,-13.4774126955136,
119.365872756543)) ;
#158014=CARTESIAN_POINT('Ctrl Pts',(-10.8639070596865,-13.4774127443564,
119.34164171291)) ;
#158015=CARTESIAN_POINT('Ctrl Pts',(-10.9377109024671,-13.4774127931991,
119.317410669277)) ;
#158016=CARTESIAN_POINT('Ctrl Pts',(-10.9613569215908,-13.4814329167664,
119.389432627311)) ;
#158017=CARTESIAN_POINT('Ctrl Pts',(-10.9850029407144,-13.4854530403338,
119.461454585346)) ;
#158018=CARTESIAN_POINT('Ctrl Pts',(-10.9111990979337,-13.4854529914911,
119.48568562898)) ;
#158019=CARTESIAN_POINT('Ctrl Pts',(-10.8373952551531,-13.4854529426483,
119.509916672613)) ;
#158020=CARTESIAN_POINT('Ctrl Pts',(-10.8137492360295,-13.481432819081,
119.437894714578)) ;
#158021=CARTESIAN_POINT('Ctrl Pts',(-10.8068277964098,-13.7673558416161,
119.38132985396)) ;
#158022=CARTESIAN_POINT('Ctrl Pts',(-10.7843650610985,-13.7433670881258,
119.312911987666)) ;
#158023=CARTESIAN_POINT('Ctrl Pts',(-10.8581688989208,-13.7433671429839,
119.288680928931)) ;
#158024=CARTESIAN_POINT('Ctrl Pts',(-10.9319727367432,-13.7433671978421,
119.264449870195)) ;
#158025=CARTESIAN_POINT('Ctrl Pts',(-10.9544354720545,-13.7673559513324,
119.332867736489)) ;
#158026=CARTESIAN_POINT('Ctrl Pts',(-10.9768982073658,-13.7913447048227,
119.401285602783)) ;
#158027=CARTESIAN_POINT('Ctrl Pts',(-10.9030943695434,-13.7913446499646,
119.425516661519)) ;
#158028=CARTESIAN_POINT('Ctrl Pts',(-10.8292905317211,-13.7913445951064,
119.449747720254)) ;
#158029=CARTESIAN_POINT('Ctrl Pts',(-10.8068277964098,-13.7673558416161,
119.38132985396)) ;
#158030=CARTESIAN_POINT('Ctrl Pts',(-10.7770884508321,-14.0271101613543,
119.255429248926)) ;
#158031=CARTESIAN_POINT('Ctrl Pts',(-10.7574005437931,-13.9849513065541,
119.195463061969)) ;
#158032=CARTESIAN_POINT('Ctrl Pts',(-10.8312043760563,-13.9849513605373,
119.171231986301)) ;
#158033=CARTESIAN_POINT('Ctrl Pts',(-10.9050082083194,-13.9849514145205,
119.147000910633)) ;
#158034=CARTESIAN_POINT('Ctrl Pts',(-10.9246961153584,-14.0271102693206,
119.206967097591)) ;
#158035=CARTESIAN_POINT('Ctrl Pts',(-10.9443840223974,-14.0692691241208,
119.266933284548)) ;
#158036=CARTESIAN_POINT('Ctrl Pts',(-10.8705801901342,-14.0692690701376,
119.291164360216)) ;
#158037=CARTESIAN_POINT('Ctrl Pts',(-10.7967763578711,-14.0692690161544,
119.315395435884)) ;
#158038=CARTESIAN_POINT('Ctrl Pts',(-10.7770884508321,-14.0271101613543,
119.255429248926)) ;
#158039=CARTESIAN_POINT('Ctrl Pts',(-10.7271574214564,-14.2445027860115,
119.067879150203)) ;
#158040=CARTESIAN_POINT('Ctrl Pts',(-10.7116609736876,-14.187105106811,
119.02067947205)) ;
#158041=CARTESIAN_POINT('Ctrl Pts',(-10.785464799976,-14.1871051547693,
118.996448378184)) ;
#158042=CARTESIAN_POINT('Ctrl Pts',(-10.8592686262643,-14.1871052027276,
118.972217284318)) ;
#158043=CARTESIAN_POINT('Ctrl Pts',(-10.8747650740332,-14.244502881928,
119.019416962471)) ;
#158044=CARTESIAN_POINT('Ctrl Pts',(-10.890261521802,-14.3019005611285,
119.066616640624)) ;
#158045=CARTESIAN_POINT('Ctrl Pts',(-10.8164576955137,-14.3019005131702,
119.09084773449)) ;
#158046=CARTESIAN_POINT('Ctrl Pts',(-10.7426538692253,-14.3019004652119,
119.115078828355)) ;
#158047=CARTESIAN_POINT('Ctrl Pts',(-10.7271574214564,-14.2445027860115,
119.067879150203)) ;
#158048=CARTESIAN_POINT('Ctrl Pts',(-10.6612093802085,-14.4028029107363,
118.831466877353)) ;
#158049=CARTESIAN_POINT('Ctrl Pts',(-10.651030199486,-14.3342697574314,
118.800462736843)) ;
#158050=CARTESIAN_POINT('Ctrl Pts',(-10.7248340200921,-14.3342697924112,
118.77623162567)) ;
#158051=CARTESIAN_POINT('Ctrl Pts',(-10.7986378406982,-14.334269827391,
118.752000514496)) ;
#158052=CARTESIAN_POINT('Ctrl Pts',(-10.8088170214206,-14.402802980696,
118.783004655006)) ;
#158053=CARTESIAN_POINT('Ctrl Pts',(-10.8189962021431,-14.471336134001,
118.814008795516)) ;
#158054=CARTESIAN_POINT('Ctrl Pts',(-10.7451923815371,-14.4713360990211,
118.838239906689)) ;
#158055=CARTESIAN_POINT('Ctrl Pts',(-10.671388560931,-14.4713360640413,
118.862471017863)) ;
#158056=CARTESIAN_POINT('Ctrl Pts',(-10.6612093802085,-14.4028029107363,
118.831466877353)) ;
#158057=CARTESIAN_POINT('Ctrl Pts',(-10.5852730928227,-14.4900131921161,
118.564801583323)) ;
#158058=CARTESIAN_POINT('Ctrl Pts',(-10.5811127826548,-14.4152919696491,
118.552129951499)) ;
#158059=CARTESIAN_POINT('Ctrl Pts',(-10.6549165993077,-14.4152919849729,
118.527898828285)) ;
#158060=CARTESIAN_POINT('Ctrl Pts',(-10.7287204159607,-14.4152920002968,
118.503667705072)) ;
#158061=CARTESIAN_POINT('Ctrl Pts',(-10.7328807261286,-14.4900132227638,
118.516339336896)) ;
#158062=CARTESIAN_POINT('Ctrl Pts',(-10.7370410362966,-14.5647344452309,
118.52901096872)) ;
#158063=CARTESIAN_POINT('Ctrl Pts',(-10.6632372196436,-14.5647344299071,
118.553242091933)) ;
#158064=CARTESIAN_POINT('Ctrl Pts',(-10.5894334029907,-14.5647344145832,
118.577473215147)) ;
#158065=CARTESIAN_POINT('Ctrl Pts',(-10.5852730928227,-14.4900131921161,
118.564801583323)) ;
#158066=CARTESIAN_POINT('Ctrl Pts',(-10.5049910429359,-14.5009049303826,
118.284799184651)) ;
#158067=CARTESIAN_POINT('Ctrl Pts',(-10.5071637236144,-14.4253144760394,
118.29141682124)) ;
#158068=CARTESIAN_POINT('Ctrl Pts',(-10.5809675380395,-14.4253144674804,
118.267185691241)) ;
#158069=CARTESIAN_POINT('Ctrl Pts',(-10.6547713524647,-14.4253144589214,
118.242954561242)) ;
#158070=CARTESIAN_POINT('Ctrl Pts',(-10.6525986717862,-14.5009049132646,
118.236336924653)) ;
#158071=CARTESIAN_POINT('Ctrl Pts',(-10.6504259911078,-14.5764953676079,
118.229719288063)) ;
#158072=CARTESIAN_POINT('Ctrl Pts',(-10.5766221766826,-14.5764953761669,
118.253950418063)) ;
#158073=CARTESIAN_POINT('Ctrl Pts',(-10.5028183622575,-14.5764953847259,
118.278181548062)) ;
#158074=CARTESIAN_POINT('Ctrl Pts',(-10.5049910429359,-14.5009049303826,
118.284799184651)) ;
#158075=CARTESIAN_POINT('Ctrl Pts',(-10.4268806844919,-14.4337694493022,
118.011321719883)) ;
#158076=CARTESIAN_POINT('Ctrl Pts',(-10.4352458048887,-14.3627554397417,
118.036800528817)) ;
#158077=CARTESIAN_POINT('Ctrl Pts',(-10.5090496194382,-14.3627554046461,
118.012569399197)) ;
#158078=CARTESIAN_POINT('Ctrl Pts',(-10.5828534339877,-14.3627553695504,
117.988338269576)) ;
#158079=CARTESIAN_POINT('Ctrl Pts',(-10.5744883135909,-14.4337693791109,
117.962859460643)) ;
#158080=CARTESIAN_POINT('Ctrl Pts',(-10.566123193194,-14.5047833886713,
117.937380651709)) ;
#158081=CARTESIAN_POINT('Ctrl Pts',(-10.4923193786445,-14.504783423767,
117.961611781329)) ;
#158082=CARTESIAN_POINT('Ctrl Pts',(-10.418515564095,-14.5047834588626,
117.98584291095)) ;
#158083=CARTESIAN_POINT('Ctrl Pts',(-10.4268806844919,-14.4337694493022,
118.011321719883)) ;
#158084=CARTESIAN_POINT('Ctrl Pts',(-10.3576955154029,-14.2939322119372,
117.765123850201)) ;
#158085=CARTESIAN_POINT('Ctrl Pts',(-10.3716370706473,-14.232577073239,
117.807587580005)) ;
#158086=CARTESIAN_POINT('Ctrl Pts',(-10.4454408881443,-14.2325770123608,
117.783356459362)) ;
#158087=CARTESIAN_POINT('Ctrl Pts',(-10.5192447056414,-14.2325769514826,
117.759125338719)) ;
#158088=CARTESIAN_POINT('Ctrl Pts',(-10.505303150397,-14.2939320901808,
117.716661608916)) ;
#158089=CARTESIAN_POINT('Ctrl Pts',(-10.4913615951525,-14.3552872288789,
117.674197879113)) ;
#158090=CARTESIAN_POINT('Ctrl Pts',(-10.4175577776555,-14.3552872897571,
117.698428999756)) ;
#158091=CARTESIAN_POINT('Ctrl Pts',(-10.3437539601585,-14.3552873506354,
117.722660120398)) ;
#158092=CARTESIAN_POINT('Ctrl Pts',(-10.3576955154029,-14.2939322119372,
117.765123850201)) ;
#158093=CARTESIAN_POINT('Ctrl Pts',(-10.3029320432203,-14.0911613446941,
117.562827612356)) ;
#158094=CARTESIAN_POINT('Ctrl Pts',(-10.3214519189372,-14.0438726639187,
117.619236167666)) ;
#158095=CARTESIAN_POINT('Ctrl Pts',(-10.3952557418565,-14.0438725807802,
117.595005063539)) ;
#158096=CARTESIAN_POINT('Ctrl Pts',(-10.4690595647757,-14.0438724976418,
117.570773959411)) ;
#158097=CARTESIAN_POINT('Ctrl Pts',(-10.4505396890587,-14.0911611784172,
117.5143654041)) ;
#158098=CARTESIAN_POINT('Ctrl Pts',(-10.4320198133418,-14.1384498591927,
117.45795684879)) ;
#158099=CARTESIAN_POINT('Ctrl Pts',(-10.3582159904226,-14.1384499423311,
117.482187952917)) ;
#158100=CARTESIAN_POINT('Ctrl Pts',(-10.2844121675033,-14.1384500254695,
117.506419057045)) ;
#158101=CARTESIAN_POINT('Ctrl Pts',(-10.3029320432203,-14.0911613446941,
117.562827612356)) ;
#158102=CARTESIAN_POINT('Ctrl Pts',(-10.2673499177128,-13.8412394795533,
117.419099337292)) ;
#158103=CARTESIAN_POINT('Ctrl Pts',(-10.289112664957,-13.8113299936379,
117.485385156072)) ;
#158104=CARTESIAN_POINT('Ctrl Pts',(-10.3629164952868,-13.8113298944944,
117.461154074516)) ;
#158105=CARTESIAN_POINT('Ctrl Pts',(-10.4367203256165,-13.8113297953509,
117.436922992959)) ;
#158106=CARTESIAN_POINT('Ctrl Pts',(-10.4149575783723,-13.8412392812663,
117.370637174179)) ;
#158107=CARTESIAN_POINT('Ctrl Pts',(-10.393194831128,-13.8711487671817,
117.304351355399)) ;
#158108=CARTESIAN_POINT('Ctrl Pts',(-10.3193910007983,-13.8711488663252,
117.328582436956)) ;
#158109=CARTESIAN_POINT('Ctrl Pts',(-10.2455871704685,-13.8711489654687,
117.352813518512)) ;
#158110=CARTESIAN_POINT('Ctrl Pts',(-10.2673499177128,-13.8412394795533,
117.419099337292)) ;
#158111=CARTESIAN_POINT('Ctrl Pts',(-10.254056072628,-13.5592605313859,
117.343020397243)) ;
#158112=CARTESIAN_POINT('Ctrl Pts',(-10.2775155822903,-13.5489932748768,
117.414474280592)) ;
#158113=CARTESIAN_POINT('Ctrl Pts',(-10.3513194213136,-13.5489931673576,
117.390243225514)) ;
#158114=CARTESIAN_POINT('Ctrl Pts',(-10.4251232603369,-13.5489930598384,
117.366012170437)) ;
#158115=CARTESIAN_POINT('Ctrl Pts',(-10.4016637506746,-13.5592603163474,
117.294558287088)) ;
#158116=CARTESIAN_POINT('Ctrl Pts',(-10.3782042410124,-13.5695275728564,
117.223104403739)) ;
#158117=CARTESIAN_POINT('Ctrl Pts',(-10.3044004019891,-13.5695276803756,
117.247335458816)) ;
#158118=CARTESIAN_POINT('Ctrl Pts',(-10.2305965629658,-13.5695277878949,
117.271566513894)) ;
#158119=CARTESIAN_POINT('Ctrl Pts',(-10.254056072628,-13.5592605313859,
117.343020397243)) ;
#158120=CARTESIAN_POINT('Ctrl Pts',(-10.2648180246204,-13.2696223387077,
117.34052655831)) ;
#158121=CARTESIAN_POINT('Ctrl Pts',(-10.2882906220838,-13.279561631404,
117.412020304983)) ;
#158122=CARTESIAN_POINT('Ctrl Pts',(-10.3620944701325,-13.2795615243136,
117.387789277396)) ;
#158123=CARTESIAN_POINT('Ctrl Pts',(-10.4358983181812,-13.2795614172232,
117.363558249809)) ;
#158124=CARTESIAN_POINT('Ctrl Pts',(-10.4124257207178,-13.2696221245269,
117.292064503135)) ;
#158125=CARTESIAN_POINT('Ctrl Pts',(-10.3889531232543,-13.2596828318306,
117.220570756461)) ;
#158126=CARTESIAN_POINT('Ctrl Pts',(-10.3151492752056,-13.259682938921,
117.244801784049)) ;
#158127=CARTESIAN_POINT('Ctrl Pts',(-10.2413454271569,-13.2596830460114,
117.269032811636)) ;
#158128=CARTESIAN_POINT('Ctrl Pts',(-10.2648180246204,-13.2696223387077,
117.34052655831)) ;
#158129=CARTESIAN_POINT('Ctrl Pts',(-10.2997358790123,-12.9883139496615,
117.411316976137)) ;
#158130=CARTESIAN_POINT('Ctrl Pts',(-10.321541507602,-13.0179078909162,
117.477733404555)) ;
#158131=CARTESIAN_POINT('Ctrl Pts',(-10.3953453642065,-13.0179077930937,
117.453502403027)) ;
#158132=CARTESIAN_POINT('Ctrl Pts',(-10.469149220811,-13.0179076952712,
117.4292714015)) ;
#158133=CARTESIAN_POINT('Ctrl Pts',(-10.4473435922213,-12.9883137540165,
117.362854973081)) ;
#158134=CARTESIAN_POINT('Ctrl Pts',(-10.4255379636317,-12.9587198127618,
117.296438544663)) ;
#158135=CARTESIAN_POINT('Ctrl Pts',(-10.3517341070272,-12.9587199105843,
117.32066954619)) ;
#158136=CARTESIAN_POINT('Ctrl Pts',(-10.2779302504227,-12.9587200084068,
117.344900547718)) ;
#158137=CARTESIAN_POINT('Ctrl Pts',(-10.2997358790123,-12.9883139496615,
117.411316976137)) ;
#158138=CARTESIAN_POINT('Ctrl Pts',(-10.3569669367904,-12.7386910562247,
117.550180832731)) ;
#158139=CARTESIAN_POINT('Ctrl Pts',(-10.3755429712197,-12.7857570655332,
117.606760438379)) ;
#158140=CARTESIAN_POINT('Ctrl Pts',(-10.4493468349472,-12.7857569845681,
117.582529458547)) ;
#158141=CARTESIAN_POINT('Ctrl Pts',(-10.5231506986747,-12.785756903603,
117.558298478715)) ;
#158142=CARTESIAN_POINT('Ctrl Pts',(-10.5045746642454,-12.7386908942945,
117.501718873067)) ;
#158143=CARTESIAN_POINT('Ctrl Pts',(-10.4859986298161,-12.691624884986,
117.445139267419)) ;
#158144=CARTESIAN_POINT('Ctrl Pts',(-10.4121947660886,-12.6916249659511,
117.469370247251)) ;
#158145=CARTESIAN_POINT('Ctrl Pts',(-10.3383909023611,-12.6916250469162,
117.493601227083)) ;
#158146=CARTESIAN_POINT('Ctrl Pts',(-10.3569669367904,-12.7386910562247,
117.550180832731)) ;
#158147=CARTESIAN_POINT('Ctrl Pts',(-10.4331834431151,-12.5375785963018,
117.746852091262)) ;
#158148=CARTESIAN_POINT('Ctrl Pts',(-10.4472000358455,-12.5987561417494,
117.789544373086)) ;
#158149=CARTESIAN_POINT('Ctrl Pts',(-10.521003904621,-12.5987560832211,
117.76531340863)) ;
#158150=CARTESIAN_POINT('Ctrl Pts',(-10.5948077733966,-12.5987560246928,
117.741082444173)) ;
#158151=CARTESIAN_POINT('Ctrl Pts',(-10.5807911806663,-12.5375784792451,
117.698390162349)) ;
#158152=CARTESIAN_POINT('Ctrl Pts',(-10.566774587936,-12.4764009337975,
117.655697880525)) ;
#158153=CARTESIAN_POINT('Ctrl Pts',(-10.4929707191604,-12.4764009923258,
117.679928844982)) ;
#158154=CARTESIAN_POINT('Ctrl Pts',(-10.4191668503848,-12.4764010508541,
117.704159809438)) ;
#158155=CARTESIAN_POINT('Ctrl Pts',(-10.4331834431151,-12.5375785963018,
117.746852091262)) ;
#158156=CARTESIAN_POINT('Ctrl Pts',(-10.5236752561247,-12.3995778757378,
117.98701193378)) ;
#158157=CARTESIAN_POINT('Ctrl Pts',(-10.5321287714972,-12.4704821067912,
118.01275997948)) ;
#158158=CARTESIAN_POINT('Ctrl Pts',(-10.6059326428365,-12.4704820736808,
117.988529022832)) ;
#158159=CARTESIAN_POINT('Ctrl Pts',(-10.6797365141757,-12.4704820405704,
117.964298066184)) ;
#158160=CARTESIAN_POINT('Ctrl Pts',(-10.6712829988032,-12.399577809517,
117.938550020484)) ;
#158161=CARTESIAN_POINT('Ctrl Pts',(-10.6628294834308,-12.3286735784636,
117.912801974784)) ;
#158162=CARTESIAN_POINT('Ctrl Pts',(-10.5890256120915,-12.328673611574,
117.937032931432)) ;
#158163=CARTESIAN_POINT('Ctrl Pts',(-10.5152217407523,-12.3286736446844,
117.96126388808)) ;
#158164=CARTESIAN_POINT('Ctrl Pts',(-10.5236752561247,-12.3995778757378,
117.98701193378)) ;
#158165=CARTESIAN_POINT('Ctrl Pts',(-10.6227835579732,-12.3345174279643,
118.253393687995)) ;
#158166=CARTESIAN_POINT('Ctrl Pts',(-10.6250645346301,-12.4100708039264,
118.26034117659)) ;
#158167=CARTESIAN_POINT('Ctrl Pts',(-10.6988684058985,-12.4100707963706,
118.236110219726)) ;
#158168=CARTESIAN_POINT('Ctrl Pts',(-10.7726722771668,-12.4100707888147,
118.211879262862)) ;
#158169=CARTESIAN_POINT('Ctrl Pts',(-10.7703913005099,-12.3345174128525,
118.204931774267)) ;
#158170=CARTESIAN_POINT('Ctrl Pts',(-10.7681103238529,-12.2589640368904,
118.197984285672)) ;
#158171=CARTESIAN_POINT('Ctrl Pts',(-10.6943064525846,-12.2589640444462,
118.222215242536)) ;
#158172=CARTESIAN_POINT('Ctrl Pts',(-10.6205025813162,-12.2589640520021,
118.2464461994)) ;
#158173=CARTESIAN_POINT('Ctrl Pts',(-10.6227835579732,-12.3345174279643,
118.253393687995)) ;
#158174=CARTESIAN_POINT('Ctrl Pts',(-10.7239238622889,-12.3471393395654,
118.526024465767)) ;
#158175=CARTESIAN_POINT('Ctrl Pts',(-10.7198798307175,-12.4219252940087,
118.513706999714)) ;
#158176=CARTESIAN_POINT('Ctrl Pts',(-10.7936836996938,-12.4219253092695,
118.489476035868)) ;
#158177=CARTESIAN_POINT('Ctrl Pts',(-10.86748756867,-12.4219253245303,118.465245072023)) ;
#158178=CARTESIAN_POINT('Ctrl Pts',(-10.8715316002415,-12.347139370087,
118.477562538076)) ;
#158179=CARTESIAN_POINT('Ctrl Pts',(-10.8755756318129,-12.2723534156437,
118.48988000413)) ;
#158180=CARTESIAN_POINT('Ctrl Pts',(-10.8017717628366,-12.272353400383,
118.514110967975)) ;
#158181=CARTESIAN_POINT('Ctrl Pts',(-10.7279678938604,-12.2723533851222,
118.538341931821)) ;
#158182=CARTESIAN_POINT('Ctrl Pts',(-10.7239238622889,-12.3471393395654,
118.526024465767)) ;
#158183=CARTESIAN_POINT('Ctrl Pts',(-10.8207516399519,-12.4360428670471,
118.785542422515)) ;
#158184=CARTESIAN_POINT('Ctrl Pts',(-10.8106736759998,-12.5047344738789,
118.754846571873)) ;
#158185=CARTESIAN_POINT('Ctrl Pts',(-10.8844775408933,-12.5047345075886,
118.730615595592)) ;
#158186=CARTESIAN_POINT('Ctrl Pts',(-10.9582814057869,-12.5047345412984,
118.706384619311)) ;
#158187=CARTESIAN_POINT('Ctrl Pts',(-10.9683593697391,-12.4360429344666,
118.737080469954)) ;
#158188=CARTESIAN_POINT('Ctrl Pts',(-10.9784373336912,-12.3673513276347,
118.767776320597)) ;
#158189=CARTESIAN_POINT('Ctrl Pts',(-10.9046334687976,-12.367351293925,
118.792007296877)) ;
#158190=CARTESIAN_POINT('Ctrl Pts',(-10.830829603904,-12.3673512602152,
118.816238273158)) ;
#158191=CARTESIAN_POINT('Ctrl Pts',(-10.8207516399519,-12.4360428670471,
118.785542422515)) ;
#158192=CARTESIAN_POINT('Ctrl Pts',(-10.9075644967453,-12.5962612233629,
119.014358156929)) ;
#158193=CARTESIAN_POINT('Ctrl Pts',(-10.892146670105,-12.6538708074165,
118.967397945946)) ;
#158194=CARTESIAN_POINT('Ctrl Pts',(-10.965950529285,-12.6538708522854,
118.943166952263)) ;
#158195=CARTESIAN_POINT('Ctrl Pts',(-11.039754388465,-12.6538708971542,
118.918935958579)) ;
#158196=CARTESIAN_POINT('Ctrl Pts',(-11.0551722151052,-12.5962613131006,
118.965896169562)) ;
#158197=CARTESIAN_POINT('Ctrl Pts',(-11.0705900417455,-12.538651729047,
119.012856380545)) ;
#158198=CARTESIAN_POINT('Ctrl Pts',(-10.9967861825655,-12.5386516841781,
119.037087374229)) ;
#158199=CARTESIAN_POINT('Ctrl Pts',(-10.9229823233856,-12.5386516393093,
119.061318367912)) ;
#158200=CARTESIAN_POINT('Ctrl Pts',(-10.9075644967453,-12.5962612233629,
119.014358156929)) ;
#158201=CARTESIAN_POINT('Ctrl Pts',(-10.9778413211601,-12.8139558923281,
119.19307998567)) ;
#158202=CARTESIAN_POINT('Ctrl Pts',(-10.9582245183943,-12.8564528958473,
119.133330370774)) ;
#158203=CARTESIAN_POINT('Ctrl Pts',(-11.0320283721088,-12.8564529465473,
119.109099360444)) ;
#158204=CARTESIAN_POINT('Ctrl Pts',(-11.1058322258233,-12.8564529972473,
119.084868350113)) ;
#158205=CARTESIAN_POINT('Ctrl Pts',(-11.125449028589,-12.8139559937281,
119.144617965009)) ;
#158206=CARTESIAN_POINT('Ctrl Pts',(-11.1450658313548,-12.7714589902089,
119.204367579904)) ;
#158207=CARTESIAN_POINT('Ctrl Pts',(-11.0712619776403,-12.7714589395089,
119.228598590235)) ;
#158208=CARTESIAN_POINT('Ctrl Pts',(-10.9974581239259,-12.7714588888089,
119.252829600565)) ;
#158209=CARTESIAN_POINT('Ctrl Pts',(-10.9778413211601,-12.8139558923281,
119.19307998567)) ;
#158210=CARTESIAN_POINT('Ctrl Pts',(-11.0282836106079,-13.0756188660845,
119.311240887642)) ;
#158211=CARTESIAN_POINT('Ctrl Pts',(-11.0058492656937,-13.0999108300579,
119.242909493803)) ;
#158212=CARTESIAN_POINT('Ctrl Pts',(-11.0796531139265,-13.0999108795098,
119.218678466776)) ;
#158213=CARTESIAN_POINT('Ctrl Pts',(-11.1534569621592,-13.0999109289618,
119.194447439749)) ;
#158214=CARTESIAN_POINT('Ctrl Pts',(-11.1758913070734,-13.0756189649884,
119.262778833588)) ;
#158215=CARTESIAN_POINT('Ctrl Pts',(-11.1983256519876,-13.051327001015,
119.331110227428)) ;
#158216=CARTESIAN_POINT('Ctrl Pts',(-11.1245218037548,-13.0513269515631,
119.355341254455)) ;
#158217=CARTESIAN_POINT('Ctrl Pts',(-11.0507179555221,-13.0513269021111,
119.379572281481)) ;
#158218=CARTESIAN_POINT('Ctrl Pts',(-11.0282836106079,-13.0756188660845,
119.311240887642)) ;
#158219=CARTESIAN_POINT('Ctrl Pts',(-11.0555791922085,-13.3624251132735,
119.358838014228)) ;
#158220=CARTESIAN_POINT('Ctrl Pts',(-11.0319403546085,-13.3667285784785,
119.286837929828)) ;
#158221=CARTESIAN_POINT('Ctrl Pts',(-11.1057441984597,-13.3667286208057,
119.262606889456)) ;
#158222=CARTESIAN_POINT('Ctrl Pts',(-11.1795480423108,-13.3667286631328,
119.238375849083)) ;
#158223=CARTESIAN_POINT('Ctrl Pts',(-11.2031868799108,-13.3624251979278,
119.310375933482)) ;
#158224=CARTESIAN_POINT('Ctrl Pts',(-11.2268257175108,-13.3581217327227,
119.382376017881)) ;
#158225=CARTESIAN_POINT('Ctrl Pts',(-11.1530218736597,-13.3581216903956,
119.406607058254)) ;
#158226=CARTESIAN_POINT('Ctrl Pts',(-11.0792180298085,-13.3581216480684,
119.430838098627)) ;
#158227=CARTESIAN_POINT('Ctrl Pts',(-11.0555791922085,-13.3624251132735,
119.358838014228)) ;
#158228=CARTESIAN_POINT('Ctrl Pts',(-11.0586048593759,-13.651982180129,
119.332672404455)) ;
#158229=CARTESIAN_POINT('Ctrl Pts',(-11.0354511320318,-13.6360746304586,
119.262149887471)) ;
#158230=CARTESIAN_POINT('Ctrl Pts',(-11.1092549728687,-13.6360746639262,
119.237918837918)) ;
#158231=CARTESIAN_POINT('Ctrl Pts',(-11.1830588137057,-13.6360746973937,
119.213687788364)) ;
#158232=CARTESIAN_POINT('Ctrl Pts',(-11.2062125410498,-13.651982247064,
119.284210305348)) ;
#158233=CARTESIAN_POINT('Ctrl Pts',(-11.2293662683938,-13.6678897967344,
119.354732822331)) ;
#158234=CARTESIAN_POINT('Ctrl Pts',(-11.1555624275569,-13.6678897632668,
119.378963871885)) ;
#158235=CARTESIAN_POINT('Ctrl Pts',(-11.0817585867199,-13.6678897297993,
119.403194921438)) ;
#158236=CARTESIAN_POINT('Ctrl Pts',(-11.0586048593759,-13.651982180129,
119.332672404455)) ;
#158237=CARTESIAN_POINT('Ctrl Pts',(-11.0376843527776,-13.9268736432231,
119.23328044909)) ;
#158238=CARTESIAN_POINT('Ctrl Pts',(-11.0166942808238,-13.8917477253801,
119.169348077124)) ;
#158239=CARTESIAN_POINT('Ctrl Pts',(-11.0904981204884,-13.8917477464933,
119.145117023999)) ;
#158240=CARTESIAN_POINT('Ctrl Pts',(-11.1643019601529,-13.8917477676065,
119.120885970875)) ;
#158241=CARTESIAN_POINT('Ctrl Pts',(-11.1852920321068,-13.9268736854496,
119.184818342842)) ;
#158242=CARTESIAN_POINT('Ctrl Pts',(-11.2062821040606,-13.9619996032926,
119.248750714809)) ;
#158243=CARTESIAN_POINT('Ctrl Pts',(-11.132478264396,-13.9619995821794,
119.272981767933)) ;
#158244=CARTESIAN_POINT('Ctrl Pts',(-11.0586744247314,-13.9619995610662,
119.297212821057)) ;
#158245=CARTESIAN_POINT('Ctrl Pts',(-11.0376843527776,-13.9268736432231,
119.23328044909)) ;
#158246=CARTESIAN_POINT('Ctrl Pts',(-10.9956210330096,-14.1624927779437,
119.069898286994)) ;
#158247=CARTESIAN_POINT('Ctrl Pts',(-10.9782661256245,-14.1108622061885,
119.017038039656)) ;
#158248=CARTESIAN_POINT('Ctrl Pts',(-11.052069965002,-14.1108622190925,
118.992806985658)) ;
#158249=CARTESIAN_POINT('Ctrl Pts',(-11.1258738043794,-14.1108622319965,
118.968575931659)) ;
#158250=CARTESIAN_POINT('Ctrl Pts',(-11.1432287117646,-14.1624928037518,
119.021436178997)) ;
#158251=CARTESIAN_POINT('Ctrl Pts',(-11.1605836191497,-14.214123375507,
119.074296426334)) ;
#158252=CARTESIAN_POINT('Ctrl Pts',(-11.0867797797722,-14.214123362603,
119.098527480333)) ;
#158253=CARTESIAN_POINT('Ctrl Pts',(-11.0129759403947,-14.214123349699,
119.122758534332)) ;
#158254=CARTESIAN_POINT('Ctrl Pts',(-10.9956210330096,-14.1624927779437,
119.069898286994)) ;
#158255=CARTESIAN_POINT('Ctrl Pts',(-10.9354933314548,-14.3467872124729,
118.851183898762)) ;
#158256=CARTESIAN_POINT('Ctrl Pts',(-10.9230467944216,-14.28220994504,118.813273755401)) ;
#158257=CARTESIAN_POINT('Ctrl Pts',(-10.9968506349554,-14.2822099499131,
118.789042704924)) ;
#158258=CARTESIAN_POINT('Ctrl Pts',(-11.0706544754893,-14.2822099547862,
118.764811654447)) ;
#158259=CARTESIAN_POINT('Ctrl Pts',(-11.0831010125224,-14.346787222219,
118.802721797808)) ;
#158260=CARTESIAN_POINT('Ctrl Pts',(-11.0955475495556,-14.4113644896518,
118.840631941169)) ;
#158261=CARTESIAN_POINT('Ctrl Pts',(-11.0217437090218,-14.4113644847787,
118.864862991646)) ;
#158262=CARTESIAN_POINT('Ctrl Pts',(-10.9479398684879,-14.4113644799057,
118.889094042122)) ;
#158263=CARTESIAN_POINT('Ctrl Pts',(-10.9354933314548,-14.3467872124729,
118.851183898762)) ;
#158264=CARTESIAN_POINT('Ctrl Pts',(-10.8629481065443,-14.4636106389172,
118.594821165369)) ;
#158265=CARTESIAN_POINT('Ctrl Pts',(-10.8562810213142,-14.3907789878482,
118.574514299585)) ;
#158266=CARTESIAN_POINT('Ctrl Pts',(-10.930084863199,-14.3907789888133,
118.550283253223)) ;
#158267=CARTESIAN_POINT('Ctrl Pts',(-11.0038887050839,-14.3907789897784,
118.526052206862)) ;
#158268=CARTESIAN_POINT('Ctrl Pts',(-11.0105557903141,-14.4636106408474,
118.546359072646)) ;
#158269=CARTESIAN_POINT('Ctrl Pts',(-11.0172228755442,-14.5364422919164,
118.566665938431)) ;
#158270=CARTESIAN_POINT('Ctrl Pts',(-10.9434190336593,-14.5364422909513,
118.590896984792)) ;
#158271=CARTESIAN_POINT('Ctrl Pts',(-10.8696151917745,-14.5364422899862,
118.615128031154)) ;
#158272=CARTESIAN_POINT('Ctrl Pts',(-10.8629481065443,-14.4636106389172,
118.594821165369)) ;
#158273=CARTESIAN_POINT('Ctrl Pts',(-10.7836225816458,-14.505904926533,
118.317753204467)) ;
#158274=CARTESIAN_POINT('Ctrl Pts',(-10.7832182997654,-14.4300107624531,
118.316521827099)) ;
#158275=CARTESIAN_POINT('Ctrl Pts',(-10.8570221430318,-14.430010762108,
118.292290784945)) ;
#158276=CARTESIAN_POINT('Ctrl Pts',(-10.9308259862981,-14.430010761763,
118.268059742791)) ;
#158277=CARTESIAN_POINT('Ctrl Pts',(-10.9312302681785,-14.5059049258428,
118.26929112016)) ;
#158278=CARTESIAN_POINT('Ctrl Pts',(-10.9316345500589,-14.5817990899227,
118.270522497528)) ;
#158279=CARTESIAN_POINT('Ctrl Pts',(-10.8578307067925,-14.5817990902678,
118.294753539682)) ;
#158280=CARTESIAN_POINT('Ctrl Pts',(-10.7840268635262,-14.5817990906128,
118.318984581835)) ;
#158281=CARTESIAN_POINT('Ctrl Pts',(-10.7836225816458,-14.505904926533,
118.317753204467)) ;
#158282=CARTESIAN_POINT('Ctrl Pts',(-10.7040268941245,-14.4703681622542,
118.039876785396)) ;
#158283=CARTESIAN_POINT('Ctrl Pts',(-10.7099134458307,-14.3968421199682,
118.057806272054)) ;
#158284=CARTESIAN_POINT('Ctrl Pts',(-10.7837172900055,-14.3968421204311,
118.033575232667)) ;
#158285=CARTESIAN_POINT('Ctrl Pts',(-10.8575211341802,-14.3968421208941,
118.00934419328)) ;
#158286=CARTESIAN_POINT('Ctrl Pts',(-10.851634582474,-14.4703681631801,
117.991414706622)) ;
#158287=CARTESIAN_POINT('Ctrl Pts',(-10.8457480307678,-14.5438942054661,
117.973485219964)) ;
#158288=CARTESIAN_POINT('Ctrl Pts',(-10.771944186593,-14.5438942050032,
117.997716259351)) ;
#158289=CARTESIAN_POINT('Ctrl Pts',(-10.6981403424182,-14.5438942045402,
118.021947298738)) ;
#158290=CARTESIAN_POINT('Ctrl Pts',(-10.7040268941245,-14.4703681622542,
118.039876785396)) ;
#158291=CARTESIAN_POINT('Ctrl Pts',(-10.6303958446743,-14.359008640194,
117.780055371545)) ;
#158292=CARTESIAN_POINT('Ctrl Pts',(-10.642168662501,-14.2931494608221,
117.815913475043)) ;
#158293=CARTESIAN_POINT('Ctrl Pts',(-10.7159725068258,-14.293149462549,
117.791682436113)) ;
#158294=CARTESIAN_POINT('Ctrl Pts',(-10.7897763511506,-14.2931494642759,
117.767451397183)) ;
#158295=CARTESIAN_POINT('Ctrl Pts',(-10.7780035333239,-14.3590086436478,
117.731593293686)) ;
#158296=CARTESIAN_POINT('Ctrl Pts',(-10.7662307154971,-14.4248678230197,
117.695735190188)) ;
#158297=CARTESIAN_POINT('Ctrl Pts',(-10.6924268711723,-14.4248678212928,
117.719966229118)) ;
#158298=CARTESIAN_POINT('Ctrl Pts',(-10.6186230268475,-14.4248678195659,
117.744197268048)) ;
#158299=CARTESIAN_POINT('Ctrl Pts',(-10.6303958446743,-14.359008640194,
117.780055371545)) ;
#158300=CARTESIAN_POINT('Ctrl Pts',(-10.5692768535784,-14.1808823670753,
117.558510542006)) ;
#158301=CARTESIAN_POINT('Ctrl Pts',(-10.5860671303228,-14.1273644575797,
117.609651015829)) ;
#158302=CARTESIAN_POINT('Ctrl Pts',(-10.6598709741343,-14.1273644591981,
117.585419975335)) ;
#158303=CARTESIAN_POINT('Ctrl Pts',(-10.7336748179457,-14.1273644608165,
117.561188934842)) ;
#158304=CARTESIAN_POINT('Ctrl Pts',(-10.7168845412014,-14.1808823703121,
117.510048461019)) ;
#158305=CARTESIAN_POINT('Ctrl Pts',(-10.700094264457,-14.2344002798077,
117.458907987196)) ;
#158306=CARTESIAN_POINT('Ctrl Pts',(-10.6262904206455,-14.2344002781893,
117.48313902769)) ;
#158307=CARTESIAN_POINT('Ctrl Pts',(-10.552486576834,-14.2344002765709,
117.507370068183)) ;
#158308=CARTESIAN_POINT('Ctrl Pts',(-10.5692768535784,-14.1808823670753,
117.558510542006)) ;
#158309=CARTESIAN_POINT('Ctrl Pts',(-10.525296106505,-13.9476582149858,
117.389059170047)) ;
#158310=CARTESIAN_POINT('Ctrl Pts',(-10.5459166163672,-13.9103470808531,
117.451865916005)) ;
#158311=CARTESIAN_POINT('Ctrl Pts',(-10.6197204594822,-13.9103470799281,
117.42763487339)) ;
#158312=CARTESIAN_POINT('Ctrl Pts',(-10.6935243025973,-13.910347079003,
117.403403830775)) ;
#158313=CARTESIAN_POINT('Ctrl Pts',(-10.6729037927351,-13.9476582131357,
117.340597084818)) ;
#158314=CARTESIAN_POINT('Ctrl Pts',(-10.6522832828729,-13.9849693472685,
117.27779033886)) ;
#158315=CARTESIAN_POINT('Ctrl Pts',(-10.5784794397578,-13.9849693481935,
117.302021381474)) ;
#158316=CARTESIAN_POINT('Ctrl Pts',(-10.5046755966428,-13.9849693491186,
117.326252424089)) ;
#158317=CARTESIAN_POINT('Ctrl Pts',(-10.525296106505,-13.9476582149858,
117.389059170047)) ;
#158318=CARTESIAN_POINT('Ctrl Pts',(-10.5026217165176,-13.6767014389998,
117.284544765499)) ;
#158319=CARTESIAN_POINT('Ctrl Pts',(-10.52558923415,-13.6582555044241,117.35450011853)) ;
#158320=CARTESIAN_POINT('Ctrl Pts',(-10.5993930769601,-13.6582554985914,
117.330269074987)) ;
#158321=CARTESIAN_POINT('Ctrl Pts',(-10.6731969197703,-13.6582554927588,
117.306038031443)) ;
#158322=CARTESIAN_POINT('Ctrl Pts',(-10.6502294021379,-13.6767014273345,
117.236082678412)) ;
#158323=CARTESIAN_POINT('Ctrl Pts',(-10.6272618845055,-13.6951473619102,
117.16612732538)) ;
#158324=CARTESIAN_POINT('Ctrl Pts',(-10.5534580416954,-13.6951473677429,
117.190358368924)) ;
#158325=CARTESIAN_POINT('Ctrl Pts',(-10.4796541988852,-13.6951473735755,
117.214589412467)) ;
#158326=CARTESIAN_POINT('Ctrl Pts',(-10.5026217165176,-13.6767014389998,
117.284544765499)) ;
#158327=CARTESIAN_POINT('Ctrl Pts',(-10.503514877856,-13.3872299120028,
117.251810399679)) ;
#158328=CARTESIAN_POINT('Ctrl Pts',(-10.5271871489125,-13.3889692104813,
117.323912318046)) ;
#158329=CARTESIAN_POINT('Ctrl Pts',(-10.6009909922353,-13.388969198278,
117.299681276064)) ;
#158330=CARTESIAN_POINT('Ctrl Pts',(-10.674794835558,-13.3889691860747,
117.275450234082)) ;
#158331=CARTESIAN_POINT('Ctrl Pts',(-10.6511225645015,-13.3872298875961,
117.203348315715)) ;
#158332=CARTESIAN_POINT('Ctrl Pts',(-10.627450293445,-13.3854905891176,
117.131246397348)) ;
#158333=CARTESIAN_POINT('Ctrl Pts',(-10.5536464501223,-13.385490601321,
117.15547743933)) ;
#158334=CARTESIAN_POINT('Ctrl Pts',(-10.4798426067995,-13.3854906135243,
117.179708481312)) ;
#158335=CARTESIAN_POINT('Ctrl Pts',(-10.503514877856,-13.3872299120028,
117.251810399679)) ;
#158336=CARTESIAN_POINT('Ctrl Pts',(-10.5287931159004,-13.0993467868879,
117.2932723904)) ;
#158337=CARTESIAN_POINT('Ctrl Pts',(-10.5514700704768,-13.1211895488815,
117.362342735512)) ;
#158338=CARTESIAN_POINT('Ctrl Pts',(-10.6252739154986,-13.1211895296054,
117.338111698705)) ;
#158339=CARTESIAN_POINT('Ctrl Pts',(-10.6990777605203,-13.1211895103292,
117.313880661898)) ;
#158340=CARTESIAN_POINT('Ctrl Pts',(-10.6764008059439,-13.0993467483356,
117.244810316786)) ;
#158341=CARTESIAN_POINT('Ctrl Pts',(-10.6537238513675,-13.077503986342,
117.175739971674)) ;
#158342=CARTESIAN_POINT('Ctrl Pts',(-10.5799200063458,-13.0775040056182,
117.199971008481)) ;
#158343=CARTESIAN_POINT('Ctrl Pts',(-10.506116161324,-13.0775040248944,
117.224202045288)) ;
#158344=CARTESIAN_POINT('Ctrl Pts',(-10.5287931159004,-13.0993467868879,
117.2932723904)) ;
#158345=CARTESIAN_POINT('Ctrl Pts',(-10.5772819647789,-12.8349662721153,
117.405511188278)) ;
#158346=CARTESIAN_POINT('Ctrl Pts',(-10.5973397474272,-12.8753001510476,
117.466603958451)) ;
#158347=CARTESIAN_POINT('Ctrl Pts',(-10.6711435953011,-12.8753001272113,
117.442372930331)) ;
#158348=CARTESIAN_POINT('Ctrl Pts',(-10.744947443175,-12.875300103375,117.418141902211)) ;
#158349=CARTESIAN_POINT('Ctrl Pts',(-10.7248896605266,-12.8349662244428,
117.357049132038)) ;
#158350=CARTESIAN_POINT('Ctrl Pts',(-10.7048318778782,-12.7946323455105,
117.295956361865)) ;
#158351=CARTESIAN_POINT('Ctrl Pts',(-10.6310280300044,-12.7946323693468,
117.320187389985)) ;
#158352=CARTESIAN_POINT('Ctrl Pts',(-10.5572241821305,-12.7946323931831,
117.344418418105)) ;
#158353=CARTESIAN_POINT('Ctrl Pts',(-10.5772819647789,-12.8349662721153,
117.405511188278)) ;
#158354=CARTESIAN_POINT('Ctrl Pts',(-10.6462390061054,-12.6123125745559,
117.580099001699)) ;
#158355=CARTESIAN_POINT('Ctrl Pts',(-10.6622445927396,-12.6682505751424,
117.628849436791)) ;
#158356=CARTESIAN_POINT('Ctrl Pts',(-10.7360484443089,-12.6682505503797,
117.604618419927)) ;
#158357=CARTESIAN_POINT('Ctrl Pts',(-10.8098522958782,-12.6682505256169,
117.580387403062)) ;
#158358=CARTESIAN_POINT('Ctrl Pts',(-10.793846709244,-12.6123125250304,
117.53163696797)) ;
#158359=CARTESIAN_POINT('Ctrl Pts',(-10.7778411226098,-12.5563745244438,
117.482886532878)) ;
#158360=CARTESIAN_POINT('Ctrl Pts',(-10.7040372710405,-12.5563745492066,
117.507117549743)) ;
#158361=CARTESIAN_POINT('Ctrl Pts',(-10.6302334194712,-12.5563745739693,
117.531348566607)) ;
#158362=CARTESIAN_POINT('Ctrl Pts',(-10.6462390061054,-12.6123125745559,
117.580099001699)) ;
#158363=CARTESIAN_POINT('Ctrl Pts',(-10.7316789245276,-12.447065748415,
117.804830116923)) ;
#158364=CARTESIAN_POINT('Ctrl Pts',(-10.7424769532379,-12.5146221963664,
117.83771917099)) ;
#158365=CARTESIAN_POINT('Ctrl Pts',(-10.8162808090886,-12.5146221752964,
117.813488167166)) ;
#158366=CARTESIAN_POINT('Ctrl Pts',(-10.8900846649393,-12.5146221542264,
117.789257163342)) ;
#158367=CARTESIAN_POINT('Ctrl Pts',(-10.8792866362291,-12.4470657062751,
117.756368109275)) ;
#158368=CARTESIAN_POINT('Ctrl Pts',(-10.8684886075188,-12.3795092583237,
117.723479055207)) ;
#158369=CARTESIAN_POINT('Ctrl Pts',(-10.7946847516681,-12.3795092793937,
117.747710059031)) ;
#158370=CARTESIAN_POINT('Ctrl Pts',(-10.7208808958174,-12.3795093004636,
117.771941062855)) ;
#158371=CARTESIAN_POINT('Ctrl Pts',(-10.7316789245276,-12.447065748415,
117.804830116923)) ;
#158372=CARTESIAN_POINT('Ctrl Pts',(-10.8280555786512,-12.3516677675638,
118.062896940008)) ;
#158373=CARTESIAN_POINT('Ctrl Pts',(-10.8328744678437,-12.4259824807609,
118.077574500006)) ;
#158374=CARTESIAN_POINT('Ctrl Pts',(-10.9066783277089,-12.4259824693785,
118.05334350841)) ;
#158375=CARTESIAN_POINT('Ctrl Pts',(-10.980482187574,-12.425982457996,118.029112516813)) ;
#158376=CARTESIAN_POINT('Ctrl Pts',(-10.9756632983816,-12.3516677447989,
118.014434956815)) ;
#158377=CARTESIAN_POINT('Ctrl Pts',(-10.9708444091891,-12.2773530316018,
117.999757396817)) ;
#158378=CARTESIAN_POINT('Ctrl Pts',(-10.897040549324,-12.2773530429843,
118.023988388413)) ;
#158379=CARTESIAN_POINT('Ctrl Pts',(-10.8232366894588,-12.2773530543667,
118.048219380009)) ;
#158380=CARTESIAN_POINT('Ctrl Pts',(-10.8280555786512,-12.3516677675638,
118.062896940008)) ;
#158381=CARTESIAN_POINT('Ctrl Pts',(-10.9289420861559,-12.3325934792249,
118.334805693187)) ;
#158382=CARTESIAN_POINT('Ctrl Pts',(-10.9274561838145,-12.4083470766961,
118.330279875596)) ;
#158383=CARTESIAN_POINT('Ctrl Pts',(-11.00126004642,-12.4083470802209,118.306048892346)) ;
#158384=CARTESIAN_POINT('Ctrl Pts',(-11.0750639090255,-12.4083470837456,
118.281817909096)) ;
#158385=CARTESIAN_POINT('Ctrl Pts',(-11.0765498113669,-12.3325934862743,
118.286343726687)) ;
#158386=CARTESIAN_POINT('Ctrl Pts',(-11.0780357137083,-12.256839888803,
118.290869544278)) ;
#158387=CARTESIAN_POINT('Ctrl Pts',(-11.0042318511028,-12.2568398852783,
118.315100527528)) ;
#158388=CARTESIAN_POINT('Ctrl Pts',(-10.9304279884973,-12.2568398817536,
118.339331510778)) ;
#158389=CARTESIAN_POINT('Ctrl Pts',(-10.9289420861559,-12.3325934792249,
118.334805693187)) ;
#158390=CARTESIAN_POINT('Ctrl Pts',(-11.0285549216706,-12.3910918553195,
118.602705295816)) ;
#158391=CARTESIAN_POINT('Ctrl Pts',(-11.0208468030654,-12.4628709667284,
118.579227611603)) ;
#158392=CARTESIAN_POINT('Ctrl Pts',(-11.0946506672526,-12.4628709892207,
118.554996633171)) ;
#158393=CARTESIAN_POINT('Ctrl Pts',(-11.1684545314399,-12.4628710117129,
118.530765654739)) ;
#158394=CARTESIAN_POINT('Ctrl Pts',(-11.176162650045,-12.3910919003041,
118.554243338952)) ;
#158395=CARTESIAN_POINT('Ctrl Pts',(-11.1838707686502,-12.3193127888952,
118.577721023164)) ;
#158396=CARTESIAN_POINT('Ctrl Pts',(-11.110066904463,-12.319312766403,118.601952001596)) ;
#158397=CARTESIAN_POINT('Ctrl Pts',(-11.0362630402758,-12.3193127439107,
118.626182980028)) ;
#158398=CARTESIAN_POINT('Ctrl Pts',(-11.0285549216706,-12.3910918553195,
118.602705295816)) ;
#158399=CARTESIAN_POINT('Ctrl Pts',(-11.1202575355664,-12.5239274893633,
118.846436016608)) ;
#158400=CARTESIAN_POINT('Ctrl Pts',(-11.1068720088082,-12.5865367592055,
118.805665863374)) ;
#158401=CARTESIAN_POINT('Ctrl Pts',(-11.1806758725532,-12.5865368036991,
118.781434883595)) ;
#158402=CARTESIAN_POINT('Ctrl Pts',(-11.2544797362982,-12.5865368481928,
118.757203903816)) ;
#158403=CARTESIAN_POINT('Ctrl Pts',(-11.2678652630564,-12.5239275783507,
118.797974057049)) ;
#158404=CARTESIAN_POINT('Ctrl Pts',(-11.2812507898146,-12.4613183085085,
118.838744210283)) ;
#158405=CARTESIAN_POINT('Ctrl Pts',(-11.2074469260696,-12.4613182640148,
118.862975190062)) ;
#158406=CARTESIAN_POINT('Ctrl Pts',(-11.1336430623246,-12.4613182195212,
118.887206169841)) ;
#158407=CARTESIAN_POINT('Ctrl Pts',(-11.1202575355664,-12.5239274893633,
118.846436016608)) ;
#158408=CARTESIAN_POINT('Ctrl Pts',(-11.1974790053523,-12.7192927751428,
119.046348283817)) ;
#158409=CARTESIAN_POINT('Ctrl Pts',(-11.1794130086027,-12.7683526424801,
118.991322174291)) ;
#158410=CARTESIAN_POINT('Ctrl Pts',(-11.2532168690804,-12.7683527070147,
118.96709118456)) ;
#158411=CARTESIAN_POINT('Ctrl Pts',(-11.3270207295581,-12.7683527715494,
118.942860194829)) ;
#158412=CARTESIAN_POINT('Ctrl Pts',(-11.3450867263076,-12.719292904212,
118.997886304356)) ;
#158413=CARTESIAN_POINT('Ctrl Pts',(-11.3631527230572,-12.6702330368747,
119.052912413882)) ;
#158414=CARTESIAN_POINT('Ctrl Pts',(-11.2893488625795,-12.67023297234,119.077143403613)) ;
#158415=CARTESIAN_POINT('Ctrl Pts',(-11.2155450021019,-12.6702329078054,
119.101374393344)) ;
#158416=CARTESIAN_POINT('Ctrl Pts',(-11.1974790053523,-12.7192927751428,
119.046348283817)) ;
#158417=CARTESIAN_POINT('Ctrl Pts',(-11.256570149613,-12.9658343070978,
119.190811409268)) ;
#158418=CARTESIAN_POINT('Ctrl Pts',(-11.2350872471003,-12.9977530103242,
119.125377956234)) ;
#158419=CARTESIAN_POINT('Ctrl Pts',(-11.3088911024947,-12.9977530931819,
119.10114695102)) ;
#158420=CARTESIAN_POINT('Ctrl Pts',(-11.3826949578891,-12.9977531760396,
119.076915945806)) ;
#158421=CARTESIAN_POINT('Ctrl Pts',(-11.4041778604018,-12.9658344728131,
119.142349398841)) ;
#158422=CARTESIAN_POINT('Ctrl Pts',(-11.4256607629145,-12.9339157695866,
119.207782851876)) ;
#158423=CARTESIAN_POINT('Ctrl Pts',(-11.3518569075202,-12.9339156867289,
119.23201385709)) ;
#158424=CARTESIAN_POINT('Ctrl Pts',(-11.2780530521258,-12.9339156038712,
119.256244862303)) ;
#158425=CARTESIAN_POINT('Ctrl Pts',(-11.256570149613,-12.9658343070978,
119.190811409268)) ;
#158426=CARTESIAN_POINT('Ctrl Pts',(-11.2934413311918,-13.2443245338218,
119.267674974483)) ;
#158427=CARTESIAN_POINT('Ctrl Pts',(-11.2700862207604,-13.2568466102088,
119.196539078311)) ;
#158428=CARTESIAN_POINT('Ctrl Pts',(-11.3438900691195,-13.2568467056125,
119.172308051669)) ;
#158429=CARTESIAN_POINT('Ctrl Pts',(-11.4176939174786,-13.2568468010161,
119.148077025028)) ;
#158430=CARTESIAN_POINT('Ctrl Pts',(-11.4410490279101,-13.2443247246291,
119.2192129212)) ;
#158431=CARTESIAN_POINT('Ctrl Pts',(-11.4644041383415,-13.2318026482422,
119.290348817372)) ;
#158432=CARTESIAN_POINT('Ctrl Pts',(-11.3906002899824,-13.2318025528385,
119.314579844014)) ;
#158433=CARTESIAN_POINT('Ctrl Pts',(-11.3167964416232,-13.2318024574349,
119.338810870656)) ;
#158434=CARTESIAN_POINT('Ctrl Pts',(-11.2934413311918,-13.2443245338218,
119.267674974483)) ;
#158435=CARTESIAN_POINT('Ctrl Pts',(-11.3062978123674,-13.5367809605308,
119.271198329631)) ;
#158436=CARTESIAN_POINT('Ctrl Pts',(-11.2827481298824,-13.5289033830346,
119.199469798479)) ;
#158437=CARTESIAN_POINT('Ctrl Pts',(-11.356551969916,-13.5289034843527,
119.175238746478)) ;
#158438=CARTESIAN_POINT('Ctrl Pts',(-11.4303558099495,-13.5289035856708,
119.151007694478)) ;
#158439=CARTESIAN_POINT('Ctrl Pts',(-11.4539054924344,-13.536781163167,
119.222736225631)) ;
#158440=CARTESIAN_POINT('Ctrl Pts',(-11.4774551749194,-13.5446587406632,
119.294464756783)) ;
#158441=CARTESIAN_POINT('Ctrl Pts',(-11.4036513348859,-13.5446586393451,
119.318695808783)) ;
#158442=CARTESIAN_POINT('Ctrl Pts',(-11.3298474948524,-13.544658538027,
119.342926860784)) ;
#158443=CARTESIAN_POINT('Ctrl Pts',(-11.3062978123674,-13.5367809605308,
119.271198329631)) ;
#158444=CARTESIAN_POINT('Ctrl Pts',(-11.2949986489025,-13.8179726435299,
119.201501210985)) ;
#158445=CARTESIAN_POINT('Ctrl Pts',(-11.2729334999951,-13.790451684124,
119.134294329632)) ;
#158446=CARTESIAN_POINT('Ctrl Pts',(-11.3467373314644,-13.7904517814122,
119.110063251546)) ;
#158447=CARTESIAN_POINT('Ctrl Pts',(-11.4205411629338,-13.7904518787005,
119.085832173461)) ;
#158448=CARTESIAN_POINT('Ctrl Pts',(-11.4426063118413,-13.8179728381065,
119.153039054814)) ;
#158449=CARTESIAN_POINT('Ctrl Pts',(-11.4646714607487,-13.8454937975124,
119.220245936167)) ;
#158450=CARTESIAN_POINT('Ctrl Pts',(-11.3908676292793,-13.8454937002241,
119.244477014252)) ;
#158451=CARTESIAN_POINT('Ctrl Pts',(-11.3170637978099,-13.8454936029358,
119.268708092337)) ;
#158452=CARTESIAN_POINT('Ctrl Pts',(-11.2949986489025,-13.8179726435299,
119.201501210985)) ;
#158453=CARTESIAN_POINT('Ctrl Pts',(-11.2610571461274,-14.0724753431544,
119.062587049155)) ;
#158454=CARTESIAN_POINT('Ctrl Pts',(-11.2420643680726,-14.0271455372004,
119.004738113744)) ;
#158455=CARTESIAN_POINT('Ctrl Pts',(-11.315868191413,-14.0271456228523,
118.980507010899)) ;
#158456=CARTESIAN_POINT('Ctrl Pts',(-11.3896720147534,-14.0271457085042,
118.956275908055)) ;
#158457=CARTESIAN_POINT('Ctrl Pts',(-11.4086647928082,-14.0724755144583,
119.014124843466)) ;
#158458=CARTESIAN_POINT('Ctrl Pts',(-11.4276575708631,-14.1178053204124,
119.071973778877)) ;
#158459=CARTESIAN_POINT('Ctrl Pts',(-11.3538537475226,-14.1178052347605,
119.096204881721)) ;
#158460=CARTESIAN_POINT('Ctrl Pts',(-11.2800499241822,-14.1178051491085,
119.120435984566)) ;
#158461=CARTESIAN_POINT('Ctrl Pts',(-11.2610571461274,-14.0724753431544,
119.062587049155)) ;
#158462=CARTESIAN_POINT('Ctrl Pts',(-11.2078251507878,-14.279096140685,
118.865063933435)) ;
#158463=CARTESIAN_POINT('Ctrl Pts',(-11.193253085461,-14.2192740208291,
118.820679775734)) ;
#158464=CARTESIAN_POINT('Ctrl Pts',(-11.2670569021607,-14.219274086963,
118.796448652663)) ;
#158465=CARTESIAN_POINT('Ctrl Pts',(-11.3408607188604,-14.219274153097,
118.772217529592)) ;
#158466=CARTESIAN_POINT('Ctrl Pts',(-11.3554327841873,-14.2790962729529,
118.816601687293)) ;
#158467=CARTESIAN_POINT('Ctrl Pts',(-11.3700048495141,-14.3389183928089,
118.860985844993)) ;
#158468=CARTESIAN_POINT('Ctrl Pts',(-11.2962010328144,-14.3389183266749,
118.885216968064)) ;
#158469=CARTESIAN_POINT('Ctrl Pts',(-11.2223972161146,-14.3389182605409,
118.909448091136)) ;
#158470=CARTESIAN_POINT('Ctrl Pts',(-11.2078251507878,-14.279096140685,
118.865063933435)) ;
#158471=CARTESIAN_POINT('Ctrl Pts',(-11.1396467770328,-14.4248617955916,
118.621919734993)) ;
#158472=CARTESIAN_POINT('Ctrl Pts',(-11.1305472737529,-14.3547743304939,
118.594204118298)) ;
#158473=CARTESIAN_POINT('Ctrl Pts',(-11.2043510858454,-14.3547743715158,
118.569972981194)) ;
#158474=CARTESIAN_POINT('Ctrl Pts',(-11.2781548979379,-14.3547744125376,
118.545741844089)) ;
#158475=CARTESIAN_POINT('Ctrl Pts',(-11.2872544012177,-14.4248618776352,
118.573457460785)) ;
#158476=CARTESIAN_POINT('Ctrl Pts',(-11.2963539044976,-14.4949493427329,
118.60117307748)) ;
#158477=CARTESIAN_POINT('Ctrl Pts',(-11.2225500924051,-14.494949301711,
118.625404214584)) ;
#158478=CARTESIAN_POINT('Ctrl Pts',(-11.1487462803127,-14.4949492606892,
118.649635351688)) ;
#158479=CARTESIAN_POINT('Ctrl Pts',(-11.1396467770328,-14.4248617955916,
118.621919734993)) ;
#158480=CARTESIAN_POINT('Ctrl Pts',(-11.0618371790876,-14.4982152843021,
118.349277506824)) ;
#158481=CARTESIAN_POINT('Ctrl Pts',(-11.0588940278122,-14.4229018669145,
118.340313144982)) ;
#158482=CARTESIAN_POINT('Ctrl Pts',(-11.132697838093,-14.4229018794509,
118.31608200236)) ;
#158483=CARTESIAN_POINT('Ctrl Pts',(-11.2065016483738,-14.4229018919873,
118.291850859737)) ;
#158484=CARTESIAN_POINT('Ctrl Pts',(-11.2094447996491,-14.4982153093749,
118.300815221579)) ;
#158485=CARTESIAN_POINT('Ctrl Pts',(-11.2123879509244,-14.5735287267625,
118.309779583422)) ;
#158486=CARTESIAN_POINT('Ctrl Pts',(-11.1385841406437,-14.5735287142261,
118.334010726044)) ;
#158487=CARTESIAN_POINT('Ctrl Pts',(-11.0647803303629,-14.5735287016897,
118.358241868666)) ;
#158488=CARTESIAN_POINT('Ctrl Pts',(-11.0618371790876,-14.4982152843021,
118.349277506824)) ;
#158489=CARTESIAN_POINT('Ctrl Pts',(-10.9820685755435,-14.4941260357652,
118.071094122751)) ;
#158490=CARTESIAN_POINT('Ctrl Pts',(-10.9854191081343,-14.4189866403318,
118.081299306452)) ;
#158491=CARTESIAN_POINT('Ctrl Pts',(-11.0592229190619,-14.4189866245763,
118.0570681658)) ;
#158492=CARTESIAN_POINT('Ctrl Pts',(-11.1330267299894,-14.4189866088209,
118.032837025147)) ;
#158493=CARTESIAN_POINT('Ctrl Pts',(-11.1296761973986,-14.4941260042543,
118.022631841447)) ;
#158494=CARTESIAN_POINT('Ctrl Pts',(-11.1263256648078,-14.5692653996877,
118.012426657746)) ;
#158495=CARTESIAN_POINT('Ctrl Pts',(-11.0525218538802,-14.5692654154432,
118.036657798398)) ;
#158496=CARTESIAN_POINT('Ctrl Pts',(-10.9787180429527,-14.5692654311986,
118.060888939051)) ;
#158497=CARTESIAN_POINT('Ctrl Pts',(-10.9820685755435,-14.4941260357652,
118.071094122751)) ;
#158498=CARTESIAN_POINT('Ctrl Pts',(-10.9049115286395,-14.4126782343137,
117.800421801026)) ;
#158499=CARTESIAN_POINT('Ctrl Pts',(-10.9143918514831,-14.3431123024057,
117.829297336722)) ;
#158500=CARTESIAN_POINT('Ctrl Pts',(-10.9881956660435,-14.3431122609052,
117.805066207135)) ;
#158501=CARTESIAN_POINT('Ctrl Pts',(-11.061999480604,-14.3431122194047,
117.780835077547)) ;
#158502=CARTESIAN_POINT('Ctrl Pts',(-11.0525191577604,-14.4126781513128,
117.751959541852)) ;
#158503=CARTESIAN_POINT('Ctrl Pts',(-11.0430388349169,-14.4822440832209,
117.723084006156)) ;
#158504=CARTESIAN_POINT('Ctrl Pts',(-10.9692350203564,-14.4822441247213,
117.747315135743)) ;
#158505=CARTESIAN_POINT('Ctrl Pts',(-10.8954312057959,-14.4822441662218,
117.77154626533)) ;
#158506=CARTESIAN_POINT('Ctrl Pts',(-10.9049115286395,-14.4126782343137,
117.800421801026)) ;
#158507=CARTESIAN_POINT('Ctrl Pts',(-10.8381211251888,-14.2599648668114,
117.561542528994)) ;
#158508=CARTESIAN_POINT('Ctrl Pts',(-10.8530122817742,-14.2009567428221,
117.606898591146)) ;
#158509=CARTESIAN_POINT('Ctrl Pts',(-10.9268161018888,-14.2009566811552,
117.582667478476)) ;
#158510=CARTESIAN_POINT('Ctrl Pts',(-11.0006199220034,-14.2009566194882,
117.558436365806)) ;
#158511=CARTESIAN_POINT('Ctrl Pts',(-10.9857287654181,-14.2599647434775,
117.513080303654)) ;
#158512=CARTESIAN_POINT('Ctrl Pts',(-10.9708376088328,-14.3189728674668,
117.467724241502)) ;
#158513=CARTESIAN_POINT('Ctrl Pts',(-10.8970337887181,-14.3189729291337,
117.491955354172)) ;
#158514=CARTESIAN_POINT('Ctrl Pts',(-10.8232299686035,-14.3189729908007,
117.516186466842)) ;
#158515=CARTESIAN_POINT('Ctrl Pts',(-10.8381211251888,-14.2599648668114,
117.561542528994)) ;
#158516=CARTESIAN_POINT('Ctrl Pts',(-10.7868067530969,-14.0478524029628,
117.369893536837)) ;
#158517=CARTESIAN_POINT('Ctrl Pts',(-10.8060344417783,-14.0035651769701,
117.428457975966)) ;
#158518=CARTESIAN_POINT('Ctrl Pts',(-10.8798382686568,-14.0035651015323,
117.404226883898)) ;
#158519=CARTESIAN_POINT('Ctrl Pts',(-10.9536420955354,-14.0035650260945,
117.37999579183)) ;
#158520=CARTESIAN_POINT('Ctrl Pts',(-10.934414406854,-14.0478522520872,
117.321431352701)) ;
#158521=CARTESIAN_POINT('Ctrl Pts',(-10.9151867181727,-14.0921394780799,
117.262866913572)) ;
#158522=CARTESIAN_POINT('Ctrl Pts',(-10.8413828912941,-14.0921395535177,
117.28709800564)) ;
#158523=CARTESIAN_POINT('Ctrl Pts',(-10.7675790644156,-14.0921396289556,
117.311329097708)) ;
#158524=CARTESIAN_POINT('Ctrl Pts',(-10.7868067530969,-14.0478524029628,
117.369893536837)) ;
#158525=CARTESIAN_POINT('Ctrl Pts',(-10.7550957653846,-13.7904112840523,
117.237886359139)) ;
#158526=CARTESIAN_POINT('Ctrl Pts',(-10.7772993131729,-13.764031497392,
117.305514784843)) ;
#158527=CARTESIAN_POINT('Ctrl Pts',(-10.8511031475577,-13.7640314159743,
117.281283715637)) ;
#158528=CARTESIAN_POINT('Ctrl Pts',(-10.9249069819425,-13.7640313345566,
117.257052646432)) ;
#158529=CARTESIAN_POINT('Ctrl Pts',(-10.9027034341542,-13.7904111212169,
117.189424220728)) ;
#158530=CARTESIAN_POINT('Ctrl Pts',(-10.8804998863659,-13.8167909078772,
117.121795795024)) ;
#158531=CARTESIAN_POINT('Ctrl Pts',(-10.8066960519811,-13.8167909892949,
117.14602686423)) ;
#158532=CARTESIAN_POINT('Ctrl Pts',(-10.7328922175963,-13.8167910707126,
117.170257933435)) ;
#158533=CARTESIAN_POINT('Ctrl Pts',(-10.7550957653846,-13.7904112840523,
117.237886359139)) ;
#158534=CARTESIAN_POINT('Ctrl Pts',(-10.7462257200646,-13.5044552055669,
117.175225916484)) ;
#158535=CARTESIAN_POINT('Ctrl Pts',(-10.7698198062168,-13.4980004286212,
117.247089697519)) ;
#158536=CARTESIAN_POINT('Ctrl Pts',(-10.8436236479381,-13.498000350832,
117.222858650659)) ;
#158537=CARTESIAN_POINT('Ctrl Pts',(-10.9174274896593,-13.4980002730428,
117.198627603799)) ;
#158538=CARTESIAN_POINT('Ctrl Pts',(-10.893833403507,-13.5044550499884,
117.126763822765)) ;
#158539=CARTESIAN_POINT('Ctrl Pts',(-10.8702393173548,-13.5109098269341,
117.05490004173)) ;
#158540=CARTESIAN_POINT('Ctrl Pts',(-10.7964354756336,-13.5109099047233,
117.07913108859)) ;
#158541=CARTESIAN_POINT('Ctrl Pts',(-10.7226316339123,-13.5109099825126,
117.10336213545)) ;
#158542=CARTESIAN_POINT('Ctrl Pts',(-10.7462257200646,-13.5044552055669,
117.175225916484)) ;
#158543=CARTESIAN_POINT('Ctrl Pts',(-10.7617483985087,-13.2137879040768,
117.187050717025)) ;
#158544=CARTESIAN_POINT('Ctrl Pts',(-10.7850280399954,-13.227617723032,
117.257956750195)) ;
#158545=CARTESIAN_POINT('Ctrl Pts',(-10.8588318877171,-13.2276176541368,
117.233725721612)) ;
#158546=CARTESIAN_POINT('Ctrl Pts',(-10.9326357354387,-13.2276175852417,
117.209494693028)) ;
#158547=CARTESIAN_POINT('Ctrl Pts',(-10.909356093952,-13.2137877662865,
117.138588659857)) ;
#158548=CARTESIAN_POINT('Ctrl Pts',(-10.8860764524653,-13.1999579473313,
117.067682626687)) ;
#158549=CARTESIAN_POINT('Ctrl Pts',(-10.8122726047436,-13.1999580162265,
117.091913655271)) ;
#158550=CARTESIAN_POINT('Ctrl Pts',(-10.738468757022,-13.1999580851216,
117.116144683854)) ;
#158551=CARTESIAN_POINT('Ctrl Pts',(-10.7617483985087,-13.2137879040768,
117.187050717025)) ;
#158552=CARTESIAN_POINT('Ctrl Pts',(-10.8009076226651,-12.9385963486889,
117.270982185733)) ;
#158553=CARTESIAN_POINT('Ctrl Pts',(-10.8222196074267,-12.9716609792406,
117.335895053863)) ;
#158554=CARTESIAN_POINT('Ctrl Pts',(-10.8960234597266,-12.9716609227663,
117.311664039224)) ;
#158555=CARTESIAN_POINT('Ctrl Pts',(-10.9698273120265,-12.9716608662921,
117.287433024585)) ;
#158556=CARTESIAN_POINT('Ctrl Pts',(-10.9485153272649,-12.9385962357404,
117.222520156455)) ;
#158557=CARTESIAN_POINT('Ctrl Pts',(-10.9272033425033,-12.9055316051888,
117.157607288325)) ;
#158558=CARTESIAN_POINT('Ctrl Pts',(-10.8533994902034,-12.905531661663,
117.181838302964)) ;
#158559=CARTESIAN_POINT('Ctrl Pts',(-10.7795956379035,-12.9055317181373,
117.206069317603)) ;
#158560=CARTESIAN_POINT('Ctrl Pts',(-10.8009076226651,-12.9385963486889,
117.270982185733)) ;
#158561=CARTESIAN_POINT('Ctrl Pts',(-10.8619688891867,-12.6966955833364,
117.421502681034)) ;
#158562=CARTESIAN_POINT('Ctrl Pts',(-10.8797836635334,-12.746700030026,
117.475763610349)) ;
#158563=CARTESIAN_POINT('Ctrl Pts',(-10.9535875184615,-12.7466999895666,
117.451532603715)) ;
#158564=CARTESIAN_POINT('Ctrl Pts',(-11.0273913733895,-12.7466999491071,
117.427301597081)) ;
#158565=CARTESIAN_POINT('Ctrl Pts',(-11.0095765990428,-12.6966955024176,
117.373040667766)) ;
#158566=CARTESIAN_POINT('Ctrl Pts',(-10.991761824696,-12.646691055728,117.31877973845)) ;
#158567=CARTESIAN_POINT('Ctrl Pts',(-10.9179579697679,-12.6466910961874,
117.343010745084)) ;
#158568=CARTESIAN_POINT('Ctrl Pts',(-10.8441541148399,-12.6466911366469,
117.367241751718)) ;
#158569=CARTESIAN_POINT('Ctrl Pts',(-10.8619688891867,-12.6966955833364,
117.421502681034)) ;
#158570=CARTESIAN_POINT('Ctrl Pts',(-10.9413222714456,-12.5064217313258,
117.627710657807)) ;
#158571=CARTESIAN_POINT('Ctrl Pts',(-10.9543578954928,-12.5697873341699,
117.667415066251)) ;
#158572=CARTESIAN_POINT('Ctrl Pts',(-11.0281617510148,-12.5697873098007,
117.643184061426)) ;
#158573=CARTESIAN_POINT('Ctrl Pts',(-11.1019656065368,-12.5697872854314,
117.618953056601)) ;
#158574=CARTESIAN_POINT('Ctrl Pts',(-11.0889299824896,-12.5064216825873,
117.579248648158)) ;
#158575=CARTESIAN_POINT('Ctrl Pts',(-11.0758943584425,-12.4430560797432,
117.539544239714)) ;
#158576=CARTESIAN_POINT('Ctrl Pts',(-11.0020905029204,-12.4430561041124,
117.563775244539)) ;
#158577=CARTESIAN_POINT('Ctrl Pts',(-10.9282866473984,-12.4430561284817,
117.588006249364)) ;
#158578=CARTESIAN_POINT('Ctrl Pts',(-10.9413222714456,-12.5064217313258,
117.627710657807)) ;
#158579=CARTESIAN_POINT('Ctrl Pts',(-11.0338914556794,-12.3814205030376,
117.874194374824)) ;
#158580=CARTESIAN_POINT('Ctrl Pts',(-11.0412174109701,-12.45361013115,117.896508053317)) ;
#158581=CARTESIAN_POINT('Ctrl Pts',(-11.1150212654786,-12.4536101207451,
117.872277045405)) ;
#158582=CARTESIAN_POINT('Ctrl Pts',(-11.1888251199871,-12.4536101103402,
117.848046037493)) ;
#158583=CARTESIAN_POINT('Ctrl Pts',(-11.1814991646964,-12.3814204822278,
117.825732359)) ;
#158584=CARTESIAN_POINT('Ctrl Pts',(-11.1741732094057,-12.3092308541153,
117.803418680506)) ;
#158585=CARTESIAN_POINT('Ctrl Pts',(-11.1003693548972,-12.3092308645202,
117.827649688418)) ;
#158586=CARTESIAN_POINT('Ctrl Pts',(-11.0265655003887,-12.3092308749251,
117.85188069633)) ;
#158587=CARTESIAN_POINT('Ctrl Pts',(-11.0338914556794,-12.3814205030376,
117.874194374824)) ;
#158588=CARTESIAN_POINT('Ctrl Pts',(-11.1342884555144,-12.3309490204366,
118.144369386401)) ;
#158589=CARTESIAN_POINT('Ctrl Pts',(-11.1353525093658,-12.4067726596542,
118.147610323274)) ;
#158590=CARTESIAN_POINT('Ctrl Pts',(-11.2091563612748,-12.4067726592374,
118.123379307444)) ;
#158591=CARTESIAN_POINT('Ctrl Pts',(-11.2829602131838,-12.4067726588207,
118.099148291614)) ;
#158592=CARTESIAN_POINT('Ctrl Pts',(-11.2818961593323,-12.330949019603,
118.095907354741)) ;
#158593=CARTESIAN_POINT('Ctrl Pts',(-11.2808321054809,-12.2551253803854,
118.092666417868)) ;
#158594=CARTESIAN_POINT('Ctrl Pts',(-11.2070282535719,-12.2551253808022,
118.116897433698)) ;
#158595=CARTESIAN_POINT('Ctrl Pts',(-11.133224401663,-12.255125381219,118.141128449528)) ;
#158596=CARTESIAN_POINT('Ctrl Pts',(-11.1342884555144,-12.3309490204366,
118.144369386401)) ;
#158597=CARTESIAN_POINT('Ctrl Pts',(-11.2344352101216,-12.3579787522632,
118.414220057428)) ;
#158598=CARTESIAN_POINT('Ctrl Pts',(-11.2292363302067,-12.4320290416833,
118.398385108464)) ;
#158599=CARTESIAN_POINT('Ctrl Pts',(-11.303040180183,-12.4320290471933,
118.374154086748)) ;
#158600=CARTESIAN_POINT('Ctrl Pts',(-11.3768440301593,-12.4320290527033,
118.349923065032)) ;
#158601=CARTESIAN_POINT('Ctrl Pts',(-11.3820429100743,-12.3579787632832,
118.365758013996)) ;
#158602=CARTESIAN_POINT('Ctrl Pts',(-11.3872417899893,-12.2839284738631,
118.38159296296)) ;
#158603=CARTESIAN_POINT('Ctrl Pts',(-11.3134379400129,-12.2839284683531,
118.405823984676)) ;
#158604=CARTESIAN_POINT('Ctrl Pts',(-11.2396340900366,-12.2839284628431,
118.430055006392)) ;
#158605=CARTESIAN_POINT('Ctrl Pts',(-11.2344352101216,-12.3579787522632,
118.414220057428)) ;
#158606=CARTESIAN_POINT('Ctrl Pts',(-11.3303750050126,-12.461461206882,
118.670792503069)) ;
#158607=CARTESIAN_POINT('Ctrl Pts',(-11.3192068132449,-12.5283982631063,
118.636775993175)) ;
#158608=CARTESIAN_POINT('Ctrl Pts',(-11.3930106600982,-12.5283982698858,
118.612544961947)) ;
#158609=CARTESIAN_POINT('Ctrl Pts',(-11.4668145069516,-12.5283982766654,
118.588313930718)) ;
#158610=CARTESIAN_POINT('Ctrl Pts',(-11.4779826987193,-12.4614612204411,
118.622330440612)) ;
#158611=CARTESIAN_POINT('Ctrl Pts',(-11.4891508904871,-12.3945241642168,
118.656346950506)) ;
#158612=CARTESIAN_POINT('Ctrl Pts',(-11.4153470436337,-12.3945241574372,
118.680577981735)) ;
#158613=CARTESIAN_POINT('Ctrl Pts',(-11.3415431967804,-12.3945241506577,
118.704809012963)) ;
#158614=CARTESIAN_POINT('Ctrl Pts',(-11.3303750050126,-12.461461206882,
118.670792503069)) ;
#158615=CARTESIAN_POINT('Ctrl Pts',(-11.4139998494669,-12.6327579824641,
118.890139759141)) ;
#158616=CARTESIAN_POINT('Ctrl Pts',(-11.3977074845766,-12.6878348099754,
118.840515844591)) ;
#158617=CARTESIAN_POINT('Ctrl Pts',(-11.4715113295313,-12.6878348153818,
118.816284807579)) ;
#158618=CARTESIAN_POINT('Ctrl Pts',(-11.5453151744861,-12.6878348207882,
118.792053770568)) ;
#158619=CARTESIAN_POINT('Ctrl Pts',(-11.5616075393764,-12.632757993277,
118.841677685119)) ;
#158620=CARTESIAN_POINT('Ctrl Pts',(-11.5778999042667,-12.5776811657657,
118.891301599669)) ;
#158621=CARTESIAN_POINT('Ctrl Pts',(-11.5040960593119,-12.5776811603593,
118.91553263668)) ;
#158622=CARTESIAN_POINT('Ctrl Pts',(-11.4302922143571,-12.5776811549529,
118.939763673692)) ;
#158623=CARTESIAN_POINT('Ctrl Pts',(-11.4139998494669,-12.6327579824641,
118.890139759141)) ;
#158624=CARTESIAN_POINT('Ctrl Pts',(-11.4811854191605,-12.8610649262646,
119.059239036713)) ;
#158625=CARTESIAN_POINT('Ctrl Pts',(-11.4609125728297,-12.9002826126032,
118.997491217836)) ;
#158626=CARTESIAN_POINT('Ctrl Pts',(-11.5347164164161,-12.9002826143644,
118.973260176657)) ;
#158627=CARTESIAN_POINT('Ctrl Pts',(-11.6085202600025,-12.9002826161256,
118.949029135478)) ;
#158628=CARTESIAN_POINT('Ctrl Pts',(-11.6287931063334,-12.861064929787,
119.010776954355)) ;
#158629=CARTESIAN_POINT('Ctrl Pts',(-11.6490659526642,-12.8218472434483,
119.072524773233)) ;
#158630=CARTESIAN_POINT('Ctrl Pts',(-11.5752621090778,-12.8218472416871,
119.096755814412)) ;
#158631=CARTESIAN_POINT('Ctrl Pts',(-11.5014582654913,-12.8218472399259,
119.120986855591)) ;
#158632=CARTESIAN_POINT('Ctrl Pts',(-11.4811854191605,-12.8610649262646,
119.059239036713)) ;
#158633=CARTESIAN_POINT('Ctrl Pts',(-11.5272358980316,-13.1282120035714,
119.164129227647)) ;
#158634=CARTESIAN_POINT('Ctrl Pts',(-11.5044492380184,-13.1488341330094,
119.094724737833)) ;
#158635=CARTESIAN_POINT('Ctrl Pts',(-11.578253081244,-13.1488341316972,
119.070493695555)) ;
#158636=CARTESIAN_POINT('Ctrl Pts',(-11.6520569244697,-13.148834130385,
119.046262653278)) ;
#158637=CARTESIAN_POINT('Ctrl Pts',(-11.6748435844829,-13.1282120009471,
119.115667143091)) ;
#158638=CARTESIAN_POINT('Ctrl Pts',(-11.6976302444961,-13.1075898715092,
119.185071632905)) ;
#158639=CARTESIAN_POINT('Ctrl Pts',(-11.6238264012704,-13.1075898728214,
119.209302675182)) ;
#158640=CARTESIAN_POINT('Ctrl Pts',(-11.5500225580448,-13.1075898741335,
119.23353371746)) ;
#158641=CARTESIAN_POINT('Ctrl Pts',(-11.5272358980316,-13.1282120035714,
119.164129227647)) ;
#158642=CARTESIAN_POINT('Ctrl Pts',(-11.550031999704,-13.4170777357306,
119.198051643061)) ;
#158643=CARTESIAN_POINT('Ctrl Pts',(-11.5263544375705,-13.4175593372615,
119.125933609099)) ;
#158644=CARTESIAN_POINT('Ctrl Pts',(-11.6001582809506,-13.4175593339228,
119.101702567291)) ;
#158645=CARTESIAN_POINT('Ctrl Pts',(-11.6739621243306,-13.4175593305841,
119.077471525484)) ;
#158646=CARTESIAN_POINT('Ctrl Pts',(-11.697639686464,-13.4170777290533,
119.149589559446)) ;
#158647=CARTESIAN_POINT('Ctrl Pts',(-11.7213172485975,-13.4165961275224,
119.221707593408)) ;
#158648=CARTESIAN_POINT('Ctrl Pts',(-11.6475134052175,-13.4165961308611,
119.245938635216)) ;
#158649=CARTESIAN_POINT('Ctrl Pts',(-11.5737095618374,-13.4165961341998,
119.270169677024)) ;
#158650=CARTESIAN_POINT('Ctrl Pts',(-11.550031999704,-13.4170777357306,
119.198051643061)) ;
#158651=CARTESIAN_POINT('Ctrl Pts',(-11.5484863559817,-13.7056413839055,
119.157890620187)) ;
#158652=CARTESIAN_POINT('Ctrl Pts',(-11.5256154218655,-13.6859734009019,
119.088229445024)) ;
#158653=CARTESIAN_POINT('Ctrl Pts',(-11.5994192655733,-13.6859733981245,
119.063998404215)) ;
#158654=CARTESIAN_POINT('Ctrl Pts',(-11.6732231092811,-13.6859733953471,
119.039767363405)) ;
#158655=CARTESIAN_POINT('Ctrl Pts',(-11.6960940433973,-13.7056413783507,
119.109428538568)) ;
#158656=CARTESIAN_POINT('Ctrl Pts',(-11.7189649775135,-13.7253093613543,
119.179089713731)) ;
#158657=CARTESIAN_POINT('Ctrl Pts',(-11.6451611338057,-13.7253093641317,
119.20332075454)) ;
#158658=CARTESIAN_POINT('Ctrl Pts',(-11.5713572900979,-13.725309366909,
119.22755179535)) ;
#158659=CARTESIAN_POINT('Ctrl Pts',(-11.5484863559817,-13.7056413839055,
119.157890620187)) ;
#158660=CARTESIAN_POINT('Ctrl Pts',(-11.5233022878553,-13.9747406301587,
119.04555969316)) ;
#158661=CARTESIAN_POINT('Ctrl Pts',(-11.5028934277546,-13.9362526969778,
118.983397598257)) ;
#158662=CARTESIAN_POINT('Ctrl Pts',(-11.5766972711998,-13.9362526974253,
118.959166556648)) ;
#158663=CARTESIAN_POINT('Ctrl Pts',(-11.650501114645,-13.9362526978728,
118.934935515039)) ;
#158664=CARTESIAN_POINT('Ctrl Pts',(-11.6709099747456,-13.9747406310537,
118.997097609941)) ;
#158665=CARTESIAN_POINT('Ctrl Pts',(-11.6913188348462,-14.0132285642346,
119.059259704844)) ;
#158666=CARTESIAN_POINT('Ctrl Pts',(-11.6175149914011,-14.0132285637871,
119.083490746453)) ;
#158667=CARTESIAN_POINT('Ctrl Pts',(-11.5437111479559,-14.0132285633396,
119.107721788062)) ;
#158668=CARTESIAN_POINT('Ctrl Pts',(-11.5233022878553,-13.9747406301587,
119.04555969316)) ;
#158669=CARTESIAN_POINT('Ctrl Pts',(-11.4774772491034,-14.201974810105,
118.870644857214)) ;
#158670=CARTESIAN_POINT('Ctrl Pts',(-11.4609696918761,-14.1475641696475,
118.820365501466)) ;
#158671=CARTESIAN_POINT('Ctrl Pts',(-11.5347735344237,-14.1475641728961,
118.796134457123)) ;
#158672=CARTESIAN_POINT('Ctrl Pts',(-11.6085773769713,-14.1475641761448,
118.77190341278)) ;
#158673=CARTESIAN_POINT('Ctrl Pts',(-11.6250849341986,-14.2019748166024,
118.822182768528)) ;
#158674=CARTESIAN_POINT('Ctrl Pts',(-11.6415924914259,-14.2563854570598,
118.872462124276)) ;
#158675=CARTESIAN_POINT('Ctrl Pts',(-11.5677886488783,-14.2563854538112,
118.896693168619)) ;
#158676=CARTESIAN_POINT('Ctrl Pts',(-11.4939848063307,-14.2563854505624,
118.920924212962)) ;
#158677=CARTESIAN_POINT('Ctrl Pts',(-11.4774772491034,-14.201974810105,
118.870644857214)) ;
#158678=CARTESIAN_POINT('Ctrl Pts',(-11.4147391200156,-14.3739130003505,
118.644102382187)) ;
#158679=CARTESIAN_POINT('Ctrl Pts',(-11.4033218176889,-14.3074175885929,
118.609327121665)) ;
#158680=CARTESIAN_POINT('Ctrl Pts',(-11.4771256584836,-14.3074175937146,
118.585096071983)) ;
#158681=CARTESIAN_POINT('Ctrl Pts',(-11.5509294992783,-14.3074175988363,
118.560865022301)) ;
#158682=CARTESIAN_POINT('Ctrl Pts',(-11.5623468016051,-14.3739130105938,
118.595640282823)) ;
#158683=CARTESIAN_POINT('Ctrl Pts',(-11.5737641039319,-14.4404084223513,
118.630415543346)) ;
#158684=CARTESIAN_POINT('Ctrl Pts',(-11.4999602631372,-14.4404084172297,
118.654646593028)) ;
#158685=CARTESIAN_POINT('Ctrl Pts',(-11.4261564223424,-14.440408412108,
118.67887764271)) ;
#158686=CARTESIAN_POINT('Ctrl Pts',(-11.4147391200156,-14.3739130003505,
118.644102382187)) ;
#158687=CARTESIAN_POINT('Ctrl Pts',(-11.3404625025784,-14.4775305035498,
118.382452018192)) ;
#158688=CARTESIAN_POINT('Ctrl Pts',(-11.3349477261256,-14.4037037065639,
118.365654899236)) ;
#158689=CARTESIAN_POINT('Ctrl Pts',(-11.4087515646572,-14.403703711016,
118.341423842661)) ;
#158690=CARTESIAN_POINT('Ctrl Pts',(-11.4825554031887,-14.4037037154681,
118.317192786086)) ;
#158691=CARTESIAN_POINT('Ctrl Pts',(-11.4880701796416,-14.477530512454,
118.333989905042)) ;
#158692=CARTESIAN_POINT('Ctrl Pts',(-11.4935849560945,-14.5513573094398,
118.350787023998)) ;
#158693=CARTESIAN_POINT('Ctrl Pts',(-11.4197811175629,-14.5513573049878,
118.375018080573)) ;
#158694=CARTESIAN_POINT('Ctrl Pts',(-11.3459772790313,-14.5513573005357,
118.399249137148)) ;
#158695=CARTESIAN_POINT('Ctrl Pts',(-11.3404625025784,-14.4775305035498,
118.382452018192)) ;
#158696=CARTESIAN_POINT('Ctrl Pts',(-11.2600762837107,-14.5050608269986,
118.101928838668)) ;
#158697=CARTESIAN_POINT('Ctrl Pts',(-11.2609046322842,-14.4292041443238,
118.104451855268)) ;
#158698=CARTESIAN_POINT('Ctrl Pts',(-11.334708467639,-14.4292041439296,
118.080220789018)) ;
#158699=CARTESIAN_POINT('Ctrl Pts',(-11.4085123029939,-14.4292041435354,
118.055989722767)) ;
#158700=CARTESIAN_POINT('Ctrl Pts',(-11.4076839544204,-14.5050608262101,
118.053466706166)) ;
#158701=CARTESIAN_POINT('Ctrl Pts',(-11.4068556058469,-14.5809175088849,
118.050943689565)) ;
#158702=CARTESIAN_POINT('Ctrl Pts',(-11.333051770492,-14.5809175092791,
118.075174755816)) ;
#158703=CARTESIAN_POINT('Ctrl Pts',(-11.2592479351372,-14.5809175096733,
118.099405822067)) ;
#158704=CARTESIAN_POINT('Ctrl Pts',(-11.2600762837107,-14.5050608269986,
118.101928838668)) ;
#158705=CARTESIAN_POINT('Ctrl Pts',(-11.1816706187826,-14.4551363613954,
117.827909095909)) ;
#158706=CARTESIAN_POINT('Ctrl Pts',(-11.1887030165374,-14.3826564737513,
117.84932864541)) ;
#158707=CARTESIAN_POINT('Ctrl Pts',(-11.2625068504305,-14.3826564648488,
117.825097574707)) ;
#158708=CARTESIAN_POINT('Ctrl Pts',(-11.3363106843237,-14.3826564559462,
117.800866504004)) ;
#158709=CARTESIAN_POINT('Ctrl Pts',(-11.3292782865689,-14.4551363435903,
117.779446954503)) ;
#158710=CARTESIAN_POINT('Ctrl Pts',(-11.3222458888142,-14.5276162312344,
117.758027405002)) ;
#158711=CARTESIAN_POINT('Ctrl Pts',(-11.248442054921,-14.5276162401369,
117.782258475705)) ;
#158712=CARTESIAN_POINT('Ctrl Pts',(-11.1746382210279,-14.5276162490395,
117.806489546408)) ;
#158713=CARTESIAN_POINT('Ctrl Pts',(-11.1816706187826,-14.4551363613954,
117.827909095909)) ;
#158714=CARTESIAN_POINT('Ctrl Pts',(-11.1096219883487,-14.3298705824412,
117.57276605832)) ;
#158715=CARTESIAN_POINT('Ctrl Pts',(-11.122433722577,-14.2660313750253,
117.611788534437)) ;
#158716=CARTESIAN_POINT('Ctrl Pts',(-11.1962375547277,-14.2660313525063,
117.587557458426)) ;
#158717=CARTESIAN_POINT('Ctrl Pts',(-11.2700413868783,-14.2660313299873,
117.563326382416)) ;
#158718=CARTESIAN_POINT('Ctrl Pts',(-11.25722965265,-14.3298705374032,117.524303906299)) ;
#158719=CARTESIAN_POINT('Ctrl Pts',(-11.2444179184216,-14.3937097448191,
117.485281430183)) ;
#158720=CARTESIAN_POINT('Ctrl Pts',(-11.1706140862709,-14.3937097673381,
117.509512506193)) ;
#158721=CARTESIAN_POINT('Ctrl Pts',(-11.0968102541203,-14.3937097898571,
117.533743582204)) ;
#158722=CARTESIAN_POINT('Ctrl Pts',(-11.1096219883487,-14.3298705824412,
117.57276605832)) ;
#158723=CARTESIAN_POINT('Ctrl Pts',(-11.0516186729526,-14.1407879039854,
117.36082074906)) ;
#158724=CARTESIAN_POINT('Ctrl Pts',(-11.0692285186037,-14.0900585571138,
117.41445749853)) ;
#158725=CARTESIAN_POINT('Ctrl Pts',(-11.1430323516223,-14.090058520559,
117.390226425163)) ;
#158726=CARTESIAN_POINT('Ctrl Pts',(-11.2168361846408,-14.0900584840042,
117.365995351797)) ;
#158727=CARTESIAN_POINT('Ctrl Pts',(-11.1992263389897,-14.1407878308758,
117.312358602326)) ;
#158728=CARTESIAN_POINT('Ctrl Pts',(-11.1816164933386,-14.1915171777474,
117.258721852855)) ;
#158729=CARTESIAN_POINT('Ctrl Pts',(-11.10781266032,-14.1915172143022,117.282952926222)) ;
#158730=CARTESIAN_POINT('Ctrl Pts',(-11.0340088273015,-14.191517250857,
117.307183999589)) ;
#158731=CARTESIAN_POINT('Ctrl Pts',(-11.0516186729526,-14.1407879039854,
117.36082074906)) ;
#158732=CARTESIAN_POINT('Ctrl Pts',(-11.01133249899,-13.8991517087972,117.202620381188)) ;
#158733=CARTESIAN_POINT('Ctrl Pts',(-11.0325150051225,-13.8652196589451,
117.267138878212)) ;
#158734=CARTESIAN_POINT('Ctrl Pts',(-11.1063188402424,-13.8652196069501,
117.242907811245)) ;
#158735=CARTESIAN_POINT('Ctrl Pts',(-11.1801226753623,-13.865219554955,
117.218676744278)) ;
#158736=CARTESIAN_POINT('Ctrl Pts',(-11.1589401692297,-13.8991516048072,
117.154158247255)) ;
#158737=CARTESIAN_POINT('Ctrl Pts',(-11.1377576630972,-13.9330836546593,
117.089639750231)) ;
#158738=CARTESIAN_POINT('Ctrl Pts',(-11.0639538279773,-13.9330837066543,
117.113870817198)) ;
#158739=CARTESIAN_POINT('Ctrl Pts',(-10.9901499928574,-13.9330837586493,
117.138101884165)) ;
#158740=CARTESIAN_POINT('Ctrl Pts',(-11.01133249899,-13.8991517087972,117.202620381188)) ;
#158741=CARTESIAN_POINT('Ctrl Pts',(-10.9929531483878,-13.622377664187,
117.111093121158)) ;
#158742=CARTESIAN_POINT('Ctrl Pts',(-11.0161851111488,-13.6077202458349,
117.18185393257)) ;
#158743=CARTESIAN_POINT('Ctrl Pts',(-11.0899889503916,-13.6077201796241,
117.157622878161)) ;
#158744=CARTESIAN_POINT('Ctrl Pts',(-11.1637927896344,-13.6077201134133,
117.133391823752)) ;
#158745=CARTESIAN_POINT('Ctrl Pts',(-11.1405608268735,-13.6223775317654,
117.062631012341)) ;
#158746=CARTESIAN_POINT('Ctrl Pts',(-11.1173288641125,-13.6370349501174,
116.991870200929)) ;
#158747=CARTESIAN_POINT('Ctrl Pts',(-11.0435250248697,-13.6370350163283,
117.016101255338)) ;
#158748=CARTESIAN_POINT('Ctrl Pts',(-10.9697211856269,-13.6370350825391,
117.040332309746)) ;
#158749=CARTESIAN_POINT('Ctrl Pts',(-10.9929531483878,-13.622377664187,
117.111093121158)) ;
#158750=CARTESIAN_POINT('Ctrl Pts',(-10.9984700935864,-13.3324243748073,
117.092526186947)) ;
#158751=CARTESIAN_POINT('Ctrl Pts',(-11.0220823143521,-13.3379896350766,
117.164445203023)) ;
#158752=CARTESIAN_POINT('Ctrl Pts',(-11.0958861594165,-13.3379895606869,
117.140214166346)) ;
#158753=CARTESIAN_POINT('Ctrl Pts',(-11.1696900044808,-13.3379894862972,
117.115983129668)) ;
#158754=CARTESIAN_POINT('Ctrl Pts',(-11.1460777837151,-13.3324242260279,
117.044064113592)) ;
#158755=CARTESIAN_POINT('Ctrl Pts',(-11.1224655629494,-13.3268589657586,
116.972145097516)) ;
#158756=CARTESIAN_POINT('Ctrl Pts',(-11.0486617178851,-13.3268590401483,
116.996376134193)) ;
#158757=CARTESIAN_POINT('Ctrl Pts',(-10.9748578728207,-13.326859114538,
117.020607170871)) ;
#158758=CARTESIAN_POINT('Ctrl Pts',(-10.9984700935864,-13.3324243748073,
117.092526186947)) ;
#158759=CARTESIAN_POINT('Ctrl Pts',(-11.0281068838988,-13.0478498918573,
117.147341996027)) ;
#158760=CARTESIAN_POINT('Ctrl Pts',(-11.0504177704374,-13.0732913047775,
117.215297358159)) ;
#158761=CARTESIAN_POINT('Ctrl Pts',(-11.1242216223397,-13.073291227464,
117.191066342309)) ;
#158762=CARTESIAN_POINT('Ctrl Pts',(-11.198025474242,-13.0732911501505,
117.166835326459)) ;
#158763=CARTESIAN_POINT('Ctrl Pts',(-11.1757145877034,-13.0478497372302,
117.098879964327)) ;
#158764=CARTESIAN_POINT('Ctrl Pts',(-11.1534037011648,-13.02240832431,117.030924602195)) ;
#158765=CARTESIAN_POINT('Ctrl Pts',(-11.0795998492625,-13.0224084016235,
117.055155618045)) ;
#158766=CARTESIAN_POINT('Ctrl Pts',(-11.0057959973602,-13.022408478937,
117.079386633895)) ;
#158767=CARTESIAN_POINT('Ctrl Pts',(-11.0281068838988,-13.0478498918573,
117.147341996027)) ;
#158768=CARTESIAN_POINT('Ctrl Pts',(-11.081052628238,-12.7884262570381,
117.272939564718)) ;
#158769=CARTESIAN_POINT('Ctrl Pts',(-11.1004376583258,-12.8320168743516,
117.331983240342)) ;
#158770=CARTESIAN_POINT('Ctrl Pts',(-11.1742415178474,-12.8320168006288,
117.3077522477)) ;
#158771=CARTESIAN_POINT('Ctrl Pts',(-11.248045377369,-12.8320167269059,
117.283521255057)) ;
#158772=CARTESIAN_POINT('Ctrl Pts',(-11.2286603472812,-12.7884261095925,
117.224477579433)) ;
#158773=CARTESIAN_POINT('Ctrl Pts',(-11.2092753171935,-12.744835492279,
117.165433903809)) ;
#158774=CARTESIAN_POINT('Ctrl Pts',(-11.1354714576718,-12.7448355660018,
117.189664896451)) ;
#158775=CARTESIAN_POINT('Ctrl Pts',(-11.0616675981502,-12.7448356397246,
117.213895889094)) ;
#158776=CARTESIAN_POINT('Ctrl Pts',(-11.081052628238,-12.7884262570381,
117.272939564718)) ;
#158777=CARTESIAN_POINT('Ctrl Pts',(-11.1532846644103,-12.5764203972658,
117.457617573228)) ;
#158778=CARTESIAN_POINT('Ctrl Pts',(-11.1683858439302,-12.6348758868913,
117.503613331312)) ;
#158779=CARTESIAN_POINT('Ctrl Pts',(-11.2421897101441,-12.6348758265582,
117.479382359053)) ;
#158780=CARTESIAN_POINT('Ctrl Pts',(-11.315993576358,-12.6348757662251,
117.455151386793)) ;
#158781=CARTESIAN_POINT('Ctrl Pts',(-11.300892396838,-12.5764202765996,
117.40915562871)) ;
#158782=CARTESIAN_POINT('Ctrl Pts',(-11.285791217318,-12.517964786974,117.363159870627)) ;
#158783=CARTESIAN_POINT('Ctrl Pts',(-11.2119873511042,-12.5179648473072,
117.387390842886)) ;
#158784=CARTESIAN_POINT('Ctrl Pts',(-11.1381834848903,-12.5179649076403,
117.411621815145)) ;
#158785=CARTESIAN_POINT('Ctrl Pts',(-11.1532846644103,-12.5764203972658,
117.457617573228)) ;
#158786=CARTESIAN_POINT('Ctrl Pts',(-11.2410864798589,-12.4236100991773,
117.689588048581)) ;
#158787=CARTESIAN_POINT('Ctrl Pts',(-11.2508134478998,-12.4928195575656,
117.71921482572)) ;
#158788=CARTESIAN_POINT('Ctrl Pts',(-11.3246173196788,-12.4928195167555,
117.694983870411)) ;
#158789=CARTESIAN_POINT('Ctrl Pts',(-11.3984211914579,-12.4928194759453,
117.670752915103)) ;
#158790=CARTESIAN_POINT('Ctrl Pts',(-11.3886942234171,-12.423610017557,
117.641126137964)) ;
#158791=CARTESIAN_POINT('Ctrl Pts',(-11.3789672553762,-12.3544005591686,
117.611499360826)) ;
#158792=CARTESIAN_POINT('Ctrl Pts',(-11.3051633835971,-12.3544005999788,
117.635730316134)) ;
#158793=CARTESIAN_POINT('Ctrl Pts',(-11.2313595118181,-12.354400640789,
117.659961271443)) ;
#158794=CARTESIAN_POINT('Ctrl Pts',(-11.2410864798589,-12.4236100991773,
117.689588048581)) ;
#158795=CARTESIAN_POINT('Ctrl Pts',(-11.3390837070061,-12.3419562515338,
117.95250976013)) ;
#158796=CARTESIAN_POINT('Ctrl Pts',(-11.3427190480782,-12.4169681280718,
117.963582424484)) ;
#158797=CARTESIAN_POINT('Ctrl Pts',(-11.4165229235351,-12.4169681124147,
117.939351480377)) ;
#158798=CARTESIAN_POINT('Ctrl Pts',(-11.4903267989919,-12.4169680967576,
117.915120536271)) ;
#158799=CARTESIAN_POINT('Ctrl Pts',(-11.4866914579199,-12.3419562202195,
117.904047871917)) ;
#158800=CARTESIAN_POINT('Ctrl Pts',(-11.4830561168478,-12.2669443436815,
117.892975207564)) ;
#158801=CARTESIAN_POINT('Ctrl Pts',(-11.4092522413909,-12.2669443593386,
117.91720615167)) ;
#158802=CARTESIAN_POINT('Ctrl Pts',(-11.3354483659341,-12.2669443749958,
117.941437095777)) ;
#158803=CARTESIAN_POINT('Ctrl Pts',(-11.3390837070061,-12.3419562515338,
117.95250976013)) ;
#158804=CARTESIAN_POINT('Ctrl Pts',(-11.440496530574,-12.3379525743983,
118.225901103267)) ;
#158805=CARTESIAN_POINT('Ctrl Pts',(-11.4377914229972,-12.4133543694812,
118.217661784115)) ;
#158806=CARTESIAN_POINT('Ctrl Pts',(-11.5115952994,-12.4133543821139,118.193430842889)) ;
#158807=CARTESIAN_POINT('Ctrl Pts',(-11.5853991758027,-12.4133543947465,
118.169199901664)) ;
#158808=CARTESIAN_POINT('Ctrl Pts',(-11.5881042833795,-12.3379525996635,
118.177439220816)) ;
#158809=CARTESIAN_POINT('Ctrl Pts',(-11.5908093909563,-12.2625508045805,
118.185678539969)) ;
#158810=CARTESIAN_POINT('Ctrl Pts',(-11.5170055145535,-12.2625507919479,
118.209909481194)) ;
#158811=CARTESIAN_POINT('Ctrl Pts',(-11.4432016381508,-12.2625507793153,
118.23414042242)) ;
#158812=CARTESIAN_POINT('Ctrl Pts',(-11.440496530574,-12.3379525743983,
118.225901103267)) ;
#158813=CARTESIAN_POINT('Ctrl Pts',(-11.5383739159563,-12.4104778611719,
118.488760855449)) ;
#158814=CARTESIAN_POINT('Ctrl Pts',(-11.529560927282,-12.4809266819483,
118.461917916001)) ;
#158815=CARTESIAN_POINT('Ctrl Pts',(-11.6033648018396,-12.4809267225878,
118.437686969155)) ;
#158816=CARTESIAN_POINT('Ctrl Pts',(-11.6771686763971,-12.4809267632273,
118.413456022309)) ;
#158817=CARTESIAN_POINT('Ctrl Pts',(-11.6859816650714,-12.4104779424509,
118.440298961757)) ;
#158818=CARTESIAN_POINT('Ctrl Pts',(-11.6947946537456,-12.3400291216744,
118.467141901205)) ;
#158819=CARTESIAN_POINT('Ctrl Pts',(-11.6209907791881,-12.3400290810349,
118.491372848051)) ;
#158820=CARTESIAN_POINT('Ctrl Pts',(-11.5471869046306,-12.3400290403954,
118.515603794896)) ;
#158821=CARTESIAN_POINT('Ctrl Pts',(-11.5383739159563,-12.4104778611719,
118.488760855449)) ;
#158822=CARTESIAN_POINT('Ctrl Pts',(-11.6278480336845,-12.5557718304403,
118.725738663281)) ;
#158823=CARTESIAN_POINT('Ctrl Pts',(-11.6135107689349,-12.6161812209366,
118.682069670258)) ;
#158824=CARTESIAN_POINT('Ctrl Pts',(-11.6873146391511,-12.6161812871028,
118.65783871019)) ;
#158825=CARTESIAN_POINT('Ctrl Pts',(-11.7611185093674,-12.6161813532691,
118.633607750121)) ;
#158826=CARTESIAN_POINT('Ctrl Pts',(-11.7754557741171,-12.5557719627728,
118.677276743144)) ;
#158827=CARTESIAN_POINT('Ctrl Pts',(-11.7897930388667,-12.4953625722765,
118.720945736166)) ;
#158828=CARTESIAN_POINT('Ctrl Pts',(-11.7159891686504,-12.4953625061102,
118.745176696234)) ;
#158829=CARTESIAN_POINT('Ctrl Pts',(-11.6421852984342,-12.495362439944,
118.769407656303)) ;
#158830=CARTESIAN_POINT('Ctrl Pts',(-11.6278480336845,-12.5557718304403,
118.725738663281)) ;
#158831=CARTESIAN_POINT('Ctrl Pts',(-11.7021593126348,-12.7621800376528,
118.916687014316)) ;
#158832=CARTESIAN_POINT('Ctrl Pts',(-11.6833449736774,-12.8082681507132,
118.85938157562)) ;
#158833=CARTESIAN_POINT('Ctrl Pts',(-11.7571488373388,-12.8082682369313,
118.835150595586)) ;
#158834=CARTESIAN_POINT('Ctrl Pts',(-11.8309527010001,-12.8082683231495,
118.810919615553)) ;
#158835=CARTESIAN_POINT('Ctrl Pts',(-11.8497670399575,-12.7621802100891,
118.868225054249)) ;
#158836=CARTESIAN_POINT('Ctrl Pts',(-11.8685813789148,-12.7160920970287,
118.925530492945)) ;
#158837=CARTESIAN_POINT('Ctrl Pts',(-11.7947775152535,-12.7160920108106,
118.949761472978)) ;
#158838=CARTESIAN_POINT('Ctrl Pts',(-11.7209736515922,-12.7160919245924,
118.973992453012)) ;
#158839=CARTESIAN_POINT('Ctrl Pts',(-11.7021593126348,-12.7621800376528,
118.916687014316)) ;
#158840=CARTESIAN_POINT('Ctrl Pts',(-11.7573807659036,-13.0168738808962,
119.049290511668)) ;
#158841=CARTESIAN_POINT('Ctrl Pts',(-11.735419427469,-13.0452490763117,
118.982399820292)) ;
#158842=CARTESIAN_POINT('Ctrl Pts',(-11.8092232829879,-13.0452491748441,
118.958168815457)) ;
#158843=CARTESIAN_POINT('Ctrl Pts',(-11.8830271385067,-13.0452492733765,
118.933937810623)) ;
#158844=CARTESIAN_POINT('Ctrl Pts',(-11.9049884769414,-13.0168740779611,
119.000828501999)) ;
#158845=CARTESIAN_POINT('Ctrl Pts',(-11.926949815376,-12.9884988825456,
119.067719193375)) ;
#158846=CARTESIAN_POINT('Ctrl Pts',(-11.8531459598571,-12.9884987840132,
119.09195019821)) ;
#158847=CARTESIAN_POINT('Ctrl Pts',(-11.7793421043382,-12.9884986854807,
119.116181203044)) ;
#158848=CARTESIAN_POINT('Ctrl Pts',(-11.7573807659036,-13.0168738808962,
119.049290511668)) ;
#158849=CARTESIAN_POINT('Ctrl Pts',(-11.7896803869344,-13.2984278863564,
119.112337306604)) ;
#158850=CARTESIAN_POINT('Ctrl Pts',(-11.7661623960868,-13.3071879031459,
119.040705303094)) ;
#158851=CARTESIAN_POINT('Ctrl Pts',(-11.8399662429446,-13.3071880059568,
119.01647427188)) ;
#158852=CARTESIAN_POINT('Ctrl Pts',(-11.9137700898025,-13.3071881087676,
118.992243240665)) ;
#158853=CARTESIAN_POINT('Ctrl Pts',(-11.9372880806501,-13.2984280919781,
119.063875244175)) ;
#158854=CARTESIAN_POINT('Ctrl Pts',(-11.9608060714977,-13.2896680751886,
119.135507247684)) ;
#158855=CARTESIAN_POINT('Ctrl Pts',(-11.8870022246399,-13.2896679723777,
119.159738278899)) ;
#158856=CARTESIAN_POINT('Ctrl Pts',(-11.8131983777821,-13.2896678695669,
119.183969310113)) ;
#158857=CARTESIAN_POINT('Ctrl Pts',(-11.7896803869344,-13.2984278863564,
119.112337306604)) ;
#158858=CARTESIAN_POINT('Ctrl Pts',(-11.7980400482597,-13.5897265030932,
119.102308017698)) ;
#158859=CARTESIAN_POINT('Ctrl Pts',(-11.7746375625407,-13.5781620490211,
119.031027824098)) ;
#158860=CARTESIAN_POINT('Ctrl Pts',(-11.8484414009126,-13.5781621471943,
119.006796767037)) ;
#158861=CARTESIAN_POINT('Ctrl Pts',(-11.9222452392845,-13.5781622453675,
118.982565709975)) ;
#158862=CARTESIAN_POINT('Ctrl Pts',(-11.9456477250035,-13.5897266994396,
119.053845903575)) ;
#158863=CARTESIAN_POINT('Ctrl Pts',(-11.9690502107225,-13.6012911535118,
119.125126097176)) ;
#158864=CARTESIAN_POINT('Ctrl Pts',(-11.8952463723506,-13.6012910553386,
119.149357154237)) ;
#158865=CARTESIAN_POINT('Ctrl Pts',(-11.8214425339787,-13.6012909571654,
119.173588211298)) ;
#158866=CARTESIAN_POINT('Ctrl Pts',(-11.7980400482597,-13.5897265030932,
119.102308017698)) ;
#158867=CARTESIAN_POINT('Ctrl Pts',(-11.7822956103083,-13.8688372211758,
119.018847493834)) ;
#158868=CARTESIAN_POINT('Ctrl Pts',(-11.7606918569279,-13.8377685346258,
118.953045948613)) ;
#158869=CARTESIAN_POINT('Ctrl Pts',(-11.8344956879977,-13.8377686202372,
118.928814869311)) ;
#158870=CARTESIAN_POINT('Ctrl Pts',(-11.9082995190675,-13.8377687058487,
118.904583790008)) ;
#158871=CARTESIAN_POINT('Ctrl Pts',(-11.9299032724479,-13.8688373923986,
118.97038533523)) ;
#158872=CARTESIAN_POINT('Ctrl Pts',(-11.9515070258284,-13.8999060789486,
119.036186880451)) ;
#158873=CARTESIAN_POINT('Ctrl Pts',(-11.8777031947586,-13.8999059933372,
119.060417959753)) ;
#158874=CARTESIAN_POINT('Ctrl Pts',(-11.8038993636888,-13.8999059077257,
119.084649039056)) ;
#158875=CARTESIAN_POINT('Ctrl Pts',(-11.7822956103083,-13.8688372211758,
119.018847493834)) ;
#158876=CARTESIAN_POINT('Ctrl Pts',(-11.7444566994981,-14.1152016754008,
118.868145849198)) ;
#158877=CARTESIAN_POINT('Ctrl Pts',(-11.7261958261659,-14.0668854985442,
118.81252617712)) ;
#158878=CARTESIAN_POINT('Ctrl Pts',(-11.7999996517436,-14.0668855661399,
118.78829508109)) ;
#158879=CARTESIAN_POINT('Ctrl Pts',(-11.8738034773214,-14.0668856337355,
118.764063985059)) ;
#158880=CARTESIAN_POINT('Ctrl Pts',(-11.8920643506536,-14.1152018105922,
118.819683657137)) ;
#158881=CARTESIAN_POINT('Ctrl Pts',(-11.9103252239859,-14.1635179874488,
118.875303329215)) ;
#158882=CARTESIAN_POINT('Ctrl Pts',(-11.8365213984081,-14.1635179198531,
118.899534425246)) ;
#158883=CARTESIAN_POINT('Ctrl Pts',(-11.7627175728303,-14.1635178522575,
118.923765521276)) ;
#158884=CARTESIAN_POINT('Ctrl Pts',(-11.7444566994981,-14.1152016754008,
118.868145849198)) ;
#158885=CARTESIAN_POINT('Ctrl Pts',(-11.6880197549201,-14.3116011164225,
118.660817745576)) ;
#158886=CARTESIAN_POINT('Ctrl Pts',(-11.6744048444867,-14.2494997572639,
118.61934892674)) ;
#158887=CARTESIAN_POINT('Ctrl Pts',(-11.7482086667398,-14.249499803588,
118.595117820584)) ;
#158888=CARTESIAN_POINT('Ctrl Pts',(-11.8220124889928,-14.249499849912,
118.570886714427)) ;
#158889=CARTESIAN_POINT('Ctrl Pts',(-11.8356273994263,-14.3116012090706,
118.612355533262)) ;
#158890=CARTESIAN_POINT('Ctrl Pts',(-11.8492423098597,-14.3737025682292,
118.653824352097)) ;
#158891=CARTESIAN_POINT('Ctrl Pts',(-11.7754384876066,-14.3737025219051,
118.678055458254)) ;
#158892=CARTESIAN_POINT('Ctrl Pts',(-11.7016346653535,-14.3737024755811,
118.702286564411)) ;
#158893=CARTESIAN_POINT('Ctrl Pts',(-11.6880197549201,-14.3116011164225,
118.660817745576)) ;
#158894=CARTESIAN_POINT('Ctrl Pts',(-11.6176369249549,-14.4442909382302,
118.410962690409)) ;
#158895=CARTESIAN_POINT('Ctrl Pts',(-11.6096496641421,-14.3728313741273,
118.386634784156)) ;
#158896=CARTESIAN_POINT('Ctrl Pts',(-11.6834534855113,-14.3728313982058,
118.362403675307)) ;
#158897=CARTESIAN_POINT('Ctrl Pts',(-11.7572573068805,-14.3728314222843,
118.338172566458)) ;
#158898=CARTESIAN_POINT('Ctrl Pts',(-11.7652445676933,-14.4442909863872,
118.362500472711)) ;
#158899=CARTESIAN_POINT('Ctrl Pts',(-11.7732318285061,-14.5157505504901,
118.386828378965)) ;
#158900=CARTESIAN_POINT('Ctrl Pts',(-11.6994280071369,-14.5157505264116,
118.411059487814)) ;
#158901=CARTESIAN_POINT('Ctrl Pts',(-11.6256241857677,-14.5157505023331,
118.435290596663)) ;
#158902=CARTESIAN_POINT('Ctrl Pts',(-11.6176369249549,-14.4442909382302,
118.410962690409)) ;
#158903=CARTESIAN_POINT('Ctrl Pts',(-11.5390960272606,-14.5033545209173,
118.136228492371)) ;
#158904=CARTESIAN_POINT('Ctrl Pts',(-11.5373151934807,-14.4276627971391,
118.130804361294)) ;
#158905=CARTESIAN_POINT('Ctrl Pts',(-11.6111190162617,-14.4276628009884,
118.106573256745)) ;
#158906=CARTESIAN_POINT('Ctrl Pts',(-11.6849228390427,-14.4276628048377,
118.082342152196)) ;
#158907=CARTESIAN_POINT('Ctrl Pts',(-11.6867036728227,-14.5033545286159,
118.087766283273)) ;
#158908=CARTESIAN_POINT('Ctrl Pts',(-11.6884845066026,-14.5790462523942,
118.09319041435)) ;
#158909=CARTESIAN_POINT('Ctrl Pts',(-11.6146806838216,-14.5790462485448,
118.117421518899)) ;
#158910=CARTESIAN_POINT('Ctrl Pts',(-11.5408768610406,-14.5790462446955,
118.141652623448)) ;
#158911=CARTESIAN_POINT('Ctrl Pts',(-11.5390960272606,-14.5033545209173,
118.136228492371)) ;
#158912=CARTESIAN_POINT('Ctrl Pts',(-11.4590251392824,-14.4845849990311,
117.856907062077)) ;
#158913=CARTESIAN_POINT('Ctrl Pts',(-11.4635655267513,-14.4100891125331,
117.870736350841)) ;
#158914=CARTESIAN_POINT('Ctrl Pts',(-11.5373693524449,-14.4100891003362,
117.846505255164)) ;
#158915=CARTESIAN_POINT('Ctrl Pts',(-11.6111731781385,-14.4100890881394,
117.822274159486)) ;
#158916=CARTESIAN_POINT('Ctrl Pts',(-11.6066327906697,-14.4845849746373,
117.808444870722)) ;
#158917=CARTESIAN_POINT('Ctrl Pts',(-11.6020924032008,-14.5590808611353,
117.794615581958)) ;
#158918=CARTESIAN_POINT('Ctrl Pts',(-11.5282885775072,-14.5590808733321,
117.818846677636)) ;
#158919=CARTESIAN_POINT('Ctrl Pts',(-11.4544847518136,-14.559080885529,
117.843077773313)) ;
#158920=CARTESIAN_POINT('Ctrl Pts',(-11.4590251392824,-14.4845849990311,
117.856907062077)) ;
#158921=CARTESIAN_POINT('Ctrl Pts',(-11.383664627329,-14.3894948595566,
117.591898604544)) ;
#158922=CARTESIAN_POINT('Ctrl Pts',(-11.3942076932912,-14.3215252408879,
117.624011083301)) ;
#158923=CARTESIAN_POINT('Ctrl Pts',(-11.4680115230728,-14.3215252179033,
117.599780000075)) ;
#158924=CARTESIAN_POINT('Ctrl Pts',(-11.5418153528544,-14.3215251949188,
117.575548916849)) ;
#158925=CARTESIAN_POINT('Ctrl Pts',(-11.5312722868923,-14.3894948135875,
117.543436438092)) ;
#158926=CARTESIAN_POINT('Ctrl Pts',(-11.52072922093,-14.4574644322562,117.511323959334)) ;
#158927=CARTESIAN_POINT('Ctrl Pts',(-11.4469253911484,-14.4574644552408,
117.53555504256)) ;
#158928=CARTESIAN_POINT('Ctrl Pts',(-11.3731215613668,-14.4574644782253,
117.559786125786)) ;
#158929=CARTESIAN_POINT('Ctrl Pts',(-11.383664627329,-14.3894948595566,
117.591898604544)) ;
#158930=CARTESIAN_POINT('Ctrl Pts',(-11.3191676650949,-14.2243477865837,
117.359917217915)) ;
#158931=CARTESIAN_POINT('Ctrl Pts',(-11.3349653990732,-14.1678057740267,
117.40803456743)) ;
#158932=CARTESIAN_POINT('Ctrl Pts',(-11.4087692334159,-14.1678057466232,
117.383803498096)) ;
#158933=CARTESIAN_POINT('Ctrl Pts',(-11.4825730677585,-14.1678057192196,
117.359572428762)) ;
#158934=CARTESIAN_POINT('Ctrl Pts',(-11.4667753337802,-14.2243477317766,
117.311455079247)) ;
#158935=CARTESIAN_POINT('Ctrl Pts',(-11.4509775998019,-14.2808897443336,
117.263337729732)) ;
#158936=CARTESIAN_POINT('Ctrl Pts',(-11.3771737654593,-14.2808897717371,
117.287568799066)) ;
#158937=CARTESIAN_POINT('Ctrl Pts',(-11.3033699311166,-14.2808897991407,
117.3117998684)) ;
#158938=CARTESIAN_POINT('Ctrl Pts',(-11.3191676650949,-14.2243477865837,
117.359917217915)) ;
#158939=CARTESIAN_POINT('Ctrl Pts',(-11.2712397649004,-14.0022176408066,
117.178548503574)) ;
#158940=CARTESIAN_POINT('Ctrl Pts',(-11.2911401693373,-13.9610998254784,
117.239161925192)) ;
#158941=CARTESIAN_POINT('Ctrl Pts',(-11.3649440075334,-13.9610997980143,
117.214930867595)) ;
#158942=CARTESIAN_POINT('Ctrl Pts',(-11.4387478457295,-13.9610997705502,
117.190699809998)) ;
#158943=CARTESIAN_POINT('Ctrl Pts',(-11.4188474412926,-14.0022175858784,
117.13008638838)) ;
#158944=CARTESIAN_POINT('Ctrl Pts',(-11.3989470368558,-14.0433354012065,
117.069472966763)) ;
#158945=CARTESIAN_POINT('Ctrl Pts',(-11.3251431986597,-14.0433354286706,
117.093704024359)) ;
#158946=CARTESIAN_POINT('Ctrl Pts',(-11.2513393604635,-14.0433354561347,
117.117935081956)) ;
#158947=CARTESIAN_POINT('Ctrl Pts',(-11.2712397649004,-14.0022176408066,
117.178548503574)) ;
#158948=CARTESIAN_POINT('Ctrl Pts',(-11.2436435716615,-13.738467096939,
117.059098820409)) ;
#158949=CARTESIAN_POINT('Ctrl Pts',(-11.2662334036352,-13.7157029540504,
117.127903804218)) ;
#158950=CARTESIAN_POINT('Ctrl Pts',(-11.3400372450378,-13.7157029304284,
117.103672756388)) ;
#158951=CARTESIAN_POINT('Ctrl Pts',(-11.4138410864404,-13.7157029068064,
117.079441708557)) ;
#158952=CARTESIAN_POINT('Ctrl Pts',(-11.3912512544667,-13.7384670496951,
117.010636724748)) ;
#158953=CARTESIAN_POINT('Ctrl Pts',(-11.3686614224929,-13.7612311925838,
116.941831740939)) ;
#158954=CARTESIAN_POINT('Ctrl Pts',(-11.2948575810903,-13.7612312162057,
116.966062788769)) ;
#158955=CARTESIAN_POINT('Ctrl Pts',(-11.2210537396878,-13.7612312398277,
116.9902938366)) ;
#158956=CARTESIAN_POINT('Ctrl Pts',(-11.2436435716615,-13.738467096939,
117.059098820409)) ;
#158957=CARTESIAN_POINT('Ctrl Pts',(-11.2393171495216,-13.4497089979361,
117.010273305457)) ;
#158958=CARTESIAN_POINT('Ctrl Pts',(-11.2629811286976,-13.4470729422015,
117.082349968154)) ;
#158959=CARTESIAN_POINT('Ctrl Pts',(-11.336784972178,-13.4470729268746,
117.058118926652)) ;
#158960=CARTESIAN_POINT('Ctrl Pts',(-11.4105888156583,-13.4470729115476,
117.03388788515)) ;
#158961=CARTESIAN_POINT('Ctrl Pts',(-11.3869248364822,-13.4497089672822,
116.961811222453)) ;
#158962=CARTESIAN_POINT('Ctrl Pts',(-11.3632608573062,-13.4523450230167,
116.889734559756)) ;
#158963=CARTESIAN_POINT('Ctrl Pts',(-11.2894570138259,-13.4523450383437,
116.913965601258)) ;
#158964=CARTESIAN_POINT('Ctrl Pts',(-11.2156531703456,-13.4523450536706,
116.93819664276)) ;
#158965=CARTESIAN_POINT('Ctrl Pts',(-11.2393171495216,-13.4497089979361,
117.010273305457)) ;
#158966=CARTESIAN_POINT('Ctrl Pts',(-11.2592549423813,-13.1612741016994,
117.035679695456)) ;
#158967=CARTESIAN_POINT('Ctrl Pts',(-11.2822932686128,-13.1787740076572,
117.105850720125)) ;
#158968=CARTESIAN_POINT('Ctrl Pts',(-11.3560971128853,-13.1787739983459,
117.081619681036)) ;
#158969=CARTESIAN_POINT('Ctrl Pts',(-11.4299009571579,-13.1787739890347,
117.057388641947)) ;
#158970=CARTESIAN_POINT('Ctrl Pts',(-11.4068626309263,-13.161274083077,
116.987217617278)) ;
#158971=CARTESIAN_POINT('Ctrl Pts',(-11.3838243046947,-13.1437741771192,
116.917046592609)) ;
#158972=CARTESIAN_POINT('Ctrl Pts',(-11.3100204604222,-13.1437741864305,
116.941277631698)) ;
#158973=CARTESIAN_POINT('Ctrl Pts',(-11.2362166161497,-13.1437741957417,
116.965508670787)) ;
#158974=CARTESIAN_POINT('Ctrl Pts',(-11.2592549423813,-13.1612741016994,
117.035679695456)) ;
#158975=CARTESIAN_POINT('Ctrl Pts',(-11.3028442445725,-12.8897094409154,
117.132937982061)) ;
#158976=CARTESIAN_POINT('Ctrl Pts',(-11.3236084130691,-12.9261981229531,
117.196182289087)) ;
#158977=CARTESIAN_POINT('Ctrl Pts',(-11.3974122571748,-12.9261981199508,
117.171951249489)) ;
#158978=CARTESIAN_POINT('Ctrl Pts',(-11.4712161012806,-12.9261981169484,
117.147720209892)) ;
#158979=CARTESIAN_POINT('Ctrl Pts',(-11.450451932784,-12.8897094349106,
117.084475902866)) ;
#158980=CARTESIAN_POINT('Ctrl Pts',(-11.4296877642875,-12.8532207528728,
117.02123159584)) ;
#158981=CARTESIAN_POINT('Ctrl Pts',(-11.3558839201817,-12.8532207558752,
117.045462635438)) ;
#158982=CARTESIAN_POINT('Ctrl Pts',(-11.282080076076,-12.8532207588776,
117.069693675035)) ;
#158983=CARTESIAN_POINT('Ctrl Pts',(-11.3028442445725,-12.8897094409154,
117.132937982061)) ;
#158984=CARTESIAN_POINT('Ctrl Pts',(-11.3677649574765,-12.6562456914582,
117.295185497117)) ;
#158985=CARTESIAN_POINT('Ctrl Pts',(-11.3847614632271,-12.7090913672215,
117.346954111247)) ;
#158986=CARTESIAN_POINT('Ctrl Pts',(-11.4585653065822,-12.7090913678115,
117.322723069363)) ;
#158987=CARTESIAN_POINT('Ctrl Pts',(-11.5323691499374,-12.7090913684014,
117.29849202748)) ;
#158988=CARTESIAN_POINT('Ctrl Pts',(-11.5153726441868,-12.6562456926381,
117.24672341335)) ;
#158989=CARTESIAN_POINT('Ctrl Pts',(-11.4983761384362,-12.6034000168748,
117.19495479922)) ;
#158990=CARTESIAN_POINT('Ctrl Pts',(-11.4245722950811,-12.6034000162848,
117.219185841103)) ;
#158991=CARTESIAN_POINT('Ctrl Pts',(-11.3507684517259,-12.6034000156949,
117.243416882987)) ;
#158992=CARTESIAN_POINT('Ctrl Pts',(-11.3677649574765,-12.6562456914582,
117.295185497117)) ;
#158993=CARTESIAN_POINT('Ctrl Pts',(-11.4498623668221,-12.4776727385034,
117.509821759606)) ;
#158994=CARTESIAN_POINT('Ctrl Pts',(-11.4618845034565,-12.5430665367951,
117.546439247975)) ;
#158995=CARTESIAN_POINT('Ctrl Pts',(-11.5356883461067,-12.5430665383516,
117.522208203944)) ;
#158996=CARTESIAN_POINT('Ctrl Pts',(-11.609492188757,-12.543066539908,117.497977159914)) ;
#158997=CARTESIAN_POINT('Ctrl Pts',(-11.5974700521225,-12.4776727416163,
117.461359671545)) ;
#158998=CARTESIAN_POINT('Ctrl Pts',(-11.585447915488,-12.4122789433245,
117.424742183177)) ;
#158999=CARTESIAN_POINT('Ctrl Pts',(-11.5116440728378,-12.4122789417681,
117.448973227207)) ;
#159000=CARTESIAN_POINT('Ctrl Pts',(-11.4378402301876,-12.4122789402116,
117.473204271238)) ;
#159001=CARTESIAN_POINT('Ctrl Pts',(-11.4498623668221,-12.4776727385034,
117.509821759606)) ;
#159002=CARTESIAN_POINT('Ctrl Pts',(-11.5443175113425,-12.3662041520314,
117.762040087288)) ;
#159003=CARTESIAN_POINT('Ctrl Pts',(-11.5504958939717,-12.439478800866,
117.780858443836)) ;
#159004=CARTESIAN_POINT('Ctrl Pts',(-11.6242997363917,-12.4394788016548,
117.756627399104)) ;
#159005=CARTESIAN_POINT('Ctrl Pts',(-11.6981035788117,-12.4394788024435,
117.732396354372)) ;
#159006=CARTESIAN_POINT('Ctrl Pts',(-11.6919251961824,-12.3662041536089,
117.713577997825)) ;
#159007=CARTESIAN_POINT('Ctrl Pts',(-11.6857468135531,-12.2929295047743,
117.694759641277)) ;
#159008=CARTESIAN_POINT('Ctrl Pts',(-11.6119429711331,-12.2929295039855,
117.718990686009)) ;
#159009=CARTESIAN_POINT('Ctrl Pts',(-11.5381391287132,-12.2929295031968,
117.743221730741)) ;
#159010=CARTESIAN_POINT('Ctrl Pts',(-11.5443175113425,-12.3662041520314,
117.762040087288)) ;
#159011=CARTESIAN_POINT('Ctrl Pts',(-11.6448025118947,-12.3300379060018,
118.032692201155)) ;
#159012=CARTESIAN_POINT('Ctrl Pts',(-11.6447061301734,-12.4059457816004,
118.032398637951)) ;
#159013=CARTESIAN_POINT('Ctrl Pts',(-11.7185099730727,-12.405945781314,
118.008167594679)) ;
#159014=CARTESIAN_POINT('Ctrl Pts',(-11.792313815972,-12.4059457810276,
117.983936551407)) ;
#159015=CARTESIAN_POINT('Ctrl Pts',(-11.7924101976934,-12.330037905429,
117.984230114611)) ;
#159016=CARTESIAN_POINT('Ctrl Pts',(-11.7925065794147,-12.2541300298303,
117.984523677815)) ;
#159017=CARTESIAN_POINT('Ctrl Pts',(-11.7187027365154,-12.2541300301167,
118.008754721086)) ;
#159018=CARTESIAN_POINT('Ctrl Pts',(-11.6448988936161,-12.2541300304032,
118.032985764358)) ;
#159019=CARTESIAN_POINT('Ctrl Pts',(-11.6448025118947,-12.3300379060018,
118.032692201155)) ;
#159020=CARTESIAN_POINT('Ctrl Pts',(-11.7455128333517,-12.3719948524369,
118.303864829156)) ;
#159021=CARTESIAN_POINT('Ctrl Pts',(-11.7391201622597,-12.4450845928375,
118.284393784512)) ;
#159022=CARTESIAN_POINT('Ctrl Pts',(-11.8129240064551,-12.4450845931213,
118.260162745188)) ;
#159023=CARTESIAN_POINT('Ctrl Pts',(-11.8867278506504,-12.4450845934052,
118.235931705864)) ;
#159024=CARTESIAN_POINT('Ctrl Pts',(-11.8931205217425,-12.3719948530046,
118.255402750508)) ;
#159025=CARTESIAN_POINT('Ctrl Pts',(-11.8995131928345,-12.298905112604,
118.274873795152)) ;
#159026=CARTESIAN_POINT('Ctrl Pts',(-11.8257093486391,-12.2989051123201,
118.299104834476)) ;
#159027=CARTESIAN_POINT('Ctrl Pts',(-11.7519055044438,-12.2989051120363,
118.323335873801)) ;
#159028=CARTESIAN_POINT('Ctrl Pts',(-11.7455128333517,-12.3719948524369,
118.303864829156)) ;
#159029=CARTESIAN_POINT('Ctrl Pts',(-11.8390028851572,-12.4886302946211,
118.553235459183)) ;
#159030=CARTESIAN_POINT('Ctrl Pts',(-11.8268052546836,-12.5536824070631,
118.516083444983)) ;
#159031=CARTESIAN_POINT('Ctrl Pts',(-11.900609100121,-12.5536824104958,
118.491852409442)) ;
#159032=CARTESIAN_POINT('Ctrl Pts',(-11.9744129455585,-12.5536824139286,
118.467621373901)) ;
#159033=CARTESIAN_POINT('Ctrl Pts',(-11.9866105760321,-12.4886303014866,
118.504773388101)) ;
#159034=CARTESIAN_POINT('Ctrl Pts',(-11.9988082065056,-12.4235781890446,
118.541925402301)) ;
#159035=CARTESIAN_POINT('Ctrl Pts',(-11.9250043610682,-12.4235781856119,
118.566156437842)) ;
#159036=CARTESIAN_POINT('Ctrl Pts',(-11.8512005156307,-12.4235781821791,
118.590387473383)) ;
#159037=CARTESIAN_POINT('Ctrl Pts',(-11.8390028851572,-12.4886302946211,
118.553235459183)) ;
#159038=CARTESIAN_POINT('Ctrl Pts',(-11.9200724717719,-12.6716133926028,
118.764723942327)) ;
#159039=CARTESIAN_POINT('Ctrl Pts',(-11.902929845151,-12.7239835426952,
118.712510267852)) ;
#159040=CARTESIAN_POINT('Ctrl Pts',(-11.9767336915948,-12.7239835519862,
118.688279235376)) ;
#159041=CARTESIAN_POINT('Ctrl Pts',(-12.0505375380386,-12.7239835612772,
118.6640482029)) ;
#159042=CARTESIAN_POINT('Ctrl Pts',(-12.0676801646595,-12.6716134111847,
118.716261877375)) ;
#159043=CARTESIAN_POINT('Ctrl Pts',(-12.0848227912804,-12.6192432610923,
118.768475551851)) ;
#159044=CARTESIAN_POINT('Ctrl Pts',(-12.0110189448367,-12.6192432518013,
118.792706584326)) ;
#159045=CARTESIAN_POINT('Ctrl Pts',(-11.9372150983929,-12.6192432425104,
118.816937616802)) ;
#159046=CARTESIAN_POINT('Ctrl Pts',(-11.9200724717719,-12.6716133926028,
118.764723942327)) ;
#159047=CARTESIAN_POINT('Ctrl Pts',(-11.983729776495,-12.9096205473869,
118.922975846097)) ;
#159048=CARTESIAN_POINT('Ctrl Pts',(-11.9628548652098,-12.9454485292725,
118.859394234908)) ;
#159049=CARTESIAN_POINT('Ctrl Pts',(-12.0366587120697,-12.9454485486713,
118.835163203699)) ;
#159050=CARTESIAN_POINT('Ctrl Pts',(-12.1104625589295,-12.9454485680701,
118.810932172491)) ;
#159051=CARTESIAN_POINT('Ctrl Pts',(-12.1313374702147,-12.9096205861845,
118.874513783679)) ;
#159052=CARTESIAN_POINT('Ctrl Pts',(-12.1522123814999,-12.8737926042989,
118.938095394868)) ;
#159053=CARTESIAN_POINT('Ctrl Pts',(-12.07840853464,-12.8737925849001,118.962326426077)) ;
#159054=CARTESIAN_POINT('Ctrl Pts',(-12.0046046877801,-12.8737925655013,
118.986557457285)) ;
#159055=CARTESIAN_POINT('Ctrl Pts',(-11.983729776495,-12.9096205473869,
118.922975846097)) ;
#159056=CARTESIAN_POINT('Ctrl Pts',(-12.0254107822208,-13.1819739695916,
119.014592567458)) ;
#159057=CARTESIAN_POINT('Ctrl Pts',(-12.0023267784959,-13.1988376121803,
118.944282417269)) ;
#159058=CARTESIAN_POINT('Ctrl Pts',(-12.0761306240772,-13.1988376406376,
118.920051382166)) ;
#159059=CARTESIAN_POINT('Ctrl Pts',(-12.1499344696585,-13.198837669095,
118.895820347063)) ;
#159060=CARTESIAN_POINT('Ctrl Pts',(-12.1730184733834,-13.1819740265063,
118.966130497253)) ;
#159061=CARTESIAN_POINT('Ctrl Pts',(-12.1961024771082,-13.1651103839176,
119.036440647442)) ;
#159062=CARTESIAN_POINT('Ctrl Pts',(-12.122298631527,-13.1651103554602,
119.060671682545)) ;
#159063=CARTESIAN_POINT('Ctrl Pts',(-12.0484947859457,-13.1651103270029,
119.084902717648)) ;
#159064=CARTESIAN_POINT('Ctrl Pts',(-12.0254107822208,-13.1819739695916,
119.014592567458)) ;
#159065=CARTESIAN_POINT('Ctrl Pts',(-12.0436296355972,-13.4720244815185,
119.034627026831)) ;
#159066=CARTESIAN_POINT('Ctrl Pts',(-12.0199739180033,-13.4686610544737,
118.962575528604)) ;
#159067=CARTESIAN_POINT('Ctrl Pts',(-12.0937777610834,-13.4686610921263,
118.938344485883)) ;
#159068=CARTESIAN_POINT('Ctrl Pts',(-12.1675816041635,-13.4686611297789,
118.914113443162)) ;
#159069=CARTESIAN_POINT('Ctrl Pts',(-12.1912373217574,-13.4720245568238,
118.986164941389)) ;
#159070=CARTESIAN_POINT('Ctrl Pts',(-12.2148930393512,-13.4753879838686,
119.058216439616)) ;
#159071=CARTESIAN_POINT('Ctrl Pts',(-12.1410891962711,-13.475387946216,
119.082447482337)) ;
#159072=CARTESIAN_POINT('Ctrl Pts',(-12.067285353191,-13.4753879085634,
119.106678525058)) ;
#159073=CARTESIAN_POINT('Ctrl Pts',(-12.0436296355972,-13.4720244815185,
119.034627026831)) ;
#159074=CARTESIAN_POINT('Ctrl Pts',(-12.0374852966316,-13.7591219512168,
118.980348270067)) ;
#159075=CARTESIAN_POINT('Ctrl Pts',(-12.01496020499,-13.7357085596368,118.911740476252)) ;
#159076=CARTESIAN_POINT('Ctrl Pts',(-12.0887640440176,-13.7357086049052,
118.887509421188)) ;
#159077=CARTESIAN_POINT('Ctrl Pts',(-12.1625678830453,-13.7357086501736,
118.863278366124)) ;
#159078=CARTESIAN_POINT('Ctrl Pts',(-12.1850929746868,-13.7591220417536,
118.931886159939)) ;
#159079=CARTESIAN_POINT('Ctrl Pts',(-12.2076180663284,-13.7825354333337,
119.000493953753)) ;
#159080=CARTESIAN_POINT('Ctrl Pts',(-12.1338142273008,-13.7825353880653,
119.024725008817)) ;
#159081=CARTESIAN_POINT('Ctrl Pts',(-12.0600103882731,-13.7825353427969,
119.048956063881)) ;
#159082=CARTESIAN_POINT('Ctrl Pts',(-12.0374852966316,-13.7591219512168,
118.980348270067)) ;
#159083=CARTESIAN_POINT('Ctrl Pts',(-12.0081585226799,-14.0209982570872,
118.855533677512)) ;
#159084=CARTESIAN_POINT('Ctrl Pts',(-11.9883827926061,-13.9792670582561,
118.795299995598)) ;
#159085=CARTESIAN_POINT('Ctrl Pts',(-12.0621866264462,-13.9792671054372,
118.771068924733)) ;
#159086=CARTESIAN_POINT('Ctrl Pts',(-12.1359904602863,-13.9792671526183,
118.746837853868)) ;
#159087=CARTESIAN_POINT('Ctrl Pts',(-12.1557661903601,-14.0209983514494,
118.807071535783)) ;
#159088=CARTESIAN_POINT('Ctrl Pts',(-12.1755419204339,-14.0627295502805,
118.867305217698)) ;
#159089=CARTESIAN_POINT('Ctrl Pts',(-12.1017380865938,-14.0627295030994,
118.891536288562)) ;
#159090=CARTESIAN_POINT('Ctrl Pts',(-12.0279342527537,-14.0627294559183,
118.915767359427)) ;
#159091=CARTESIAN_POINT('Ctrl Pts',(-12.0081585226799,-14.0209982570872,
118.855533677512)) ;
#159092=CARTESIAN_POINT('Ctrl Pts',(-11.9589803424424,-14.2386408615737,
118.670464829268)) ;
#159093=CARTESIAN_POINT('Ctrl Pts',(-11.9433397158785,-14.1816542557546,
118.622826005578)) ;
#159094=CARTESIAN_POINT('Ctrl Pts',(-12.0171435445993,-14.1816542976557,
118.598594919121)) ;
#159095=CARTESIAN_POINT('Ctrl Pts',(-12.0909473733201,-14.1816543395568,
118.574363832664)) ;
#159096=CARTESIAN_POINT('Ctrl Pts',(-12.1065879998839,-14.2386409453758,
118.622002656354)) ;
#159097=CARTESIAN_POINT('Ctrl Pts',(-12.1222286264478,-14.2956275511949,
118.669641480044)) ;
#159098=CARTESIAN_POINT('Ctrl Pts',(-12.0484247977271,-14.2956275092938,
118.693872566501)) ;
#159099=CARTESIAN_POINT('Ctrl Pts',(-11.9746209690063,-14.2956274673927,
118.718103652958)) ;
#159100=CARTESIAN_POINT('Ctrl Pts',(-11.9589803424424,-14.2386408615737,
118.670464829268)) ;
#159101=CARTESIAN_POINT('Ctrl Pts',(-11.8933789786321,-14.3991847031552,
118.435064542878)) ;
#159102=CARTESIAN_POINT('Ctrl Pts',(-11.8830321664254,-14.3309065513588,
118.403549823745)) ;
#159103=CARTESIAN_POINT('Ctrl Pts',(-11.956835989594,-14.330906583244,118.379318720377)) ;
#159104=CARTESIAN_POINT('Ctrl Pts',(-12.0306398127626,-14.3309066151293,
118.355087617009)) ;
#159105=CARTESIAN_POINT('Ctrl Pts',(-12.0409866249693,-14.3991847669257,
118.386602336141)) ;
#159106=CARTESIAN_POINT('Ctrl Pts',(-12.051333437176,-14.4674629187221,
118.418117055273)) ;
#159107=CARTESIAN_POINT('Ctrl Pts',(-11.9775296140074,-14.4674628868368,
118.442348158641)) ;
#159108=CARTESIAN_POINT('Ctrl Pts',(-11.9037257908388,-14.4674628549516,
118.46657926201)) ;
#159109=CARTESIAN_POINT('Ctrl Pts',(-11.8933789786321,-14.3991847031552,
118.435064542878)) ;
#159110=CARTESIAN_POINT('Ctrl Pts',(-11.8176447978217,-14.4885294284138,
118.169014818533)) ;
#159111=CARTESIAN_POINT('Ctrl Pts',(-11.8133025721141,-14.4139147342441,
118.155789101172)) ;
#159112=CARTESIAN_POINT('Ctrl Pts',(-11.8871063912677,-14.4139147488746,
118.131557985575)) ;
#159113=CARTESIAN_POINT('Ctrl Pts',(-11.9609102104214,-14.4139147635052,
118.107326869978)) ;
#159114=CARTESIAN_POINT('Ctrl Pts',(-11.9652524361289,-14.4885294576749,
118.120552587339)) ;
#159115=CARTESIAN_POINT('Ctrl Pts',(-11.9695946618365,-14.5631441518446,
118.1337783047)) ;
#159116=CARTESIAN_POINT('Ctrl Pts',(-11.8957908426829,-14.563144137214,
118.158009420297)) ;
#159117=CARTESIAN_POINT('Ctrl Pts',(-11.8219870235292,-14.5631441225835,
118.182240535894)) ;
#159118=CARTESIAN_POINT('Ctrl Pts',(-11.8176447978217,-14.4885294284138,
118.169014818533)) ;
#159119=CARTESIAN_POINT('Ctrl Pts',(-11.7374057481524,-14.5016597743674,
117.889145533914)) ;
#159120=CARTESIAN_POINT('Ctrl Pts',(-11.7393932576882,-14.4260199965907,
117.895199168941)) ;
#159121=CARTESIAN_POINT('Ctrl Pts',(-11.8131970743123,-14.4260199894703,
117.87096804564)) ;
#159122=CARTESIAN_POINT('Ctrl Pts',(-11.8870008909365,-14.4260199823499,
117.846736922338)) ;
#159123=CARTESIAN_POINT('Ctrl Pts',(-11.8850133814006,-14.5016597601266,
117.84068328731)) ;
#159124=CARTESIAN_POINT('Ctrl Pts',(-11.8830258718648,-14.5772995379034,
117.834629652282)) ;
#159125=CARTESIAN_POINT('Ctrl Pts',(-11.8092220552407,-14.5772995450237,
117.858860775584)) ;
#159126=CARTESIAN_POINT('Ctrl Pts',(-11.7354182386166,-14.5772995521441,
117.883091898886)) ;
#159127=CARTESIAN_POINT('Ctrl Pts',(-11.7374057481524,-14.5016597743674,
117.889145533914)) ;
#159128=CARTESIAN_POINT('Ctrl Pts',(-11.6592539148603,-14.437009415365,
117.615605436135)) ;
#159129=CARTESIAN_POINT('Ctrl Pts',(-11.6674351874113,-14.3657730764766,
117.640524274072)) ;
#159130=CARTESIAN_POINT('Ctrl Pts',(-11.7412390037029,-14.3657730444813,
117.616293149758)) ;
#159131=CARTESIAN_POINT('Ctrl Pts',(-11.8150428199945,-14.365773012486,
117.592062025443)) ;
#159132=CARTESIAN_POINT('Ctrl Pts',(-11.8068615474435,-14.4370093513744,
117.567143187506)) ;
#159133=CARTESIAN_POINT('Ctrl Pts',(-11.7986802748926,-14.5082456902627,
117.54222434957)) ;
#159134=CARTESIAN_POINT('Ctrl Pts',(-11.724876458601,-14.508245722258,117.566455473884)) ;
#159135=CARTESIAN_POINT('Ctrl Pts',(-11.6510726423094,-14.5082457542533,
117.590686598198)) ;
#159136=CARTESIAN_POINT('Ctrl Pts',(-11.6592539148603,-14.437009415365,
117.615605436135)) ;
#159137=CARTESIAN_POINT('Ctrl Pts',(-11.5896054471436,-14.2988734246617,
117.367922624978)) ;
#159138=CARTESIAN_POINT('Ctrl Pts',(-11.6033967533199,-14.2371769971241,
117.40992872027)) ;
#159139=CARTESIAN_POINT('Ctrl Pts',(-11.6772005718606,-14.237176939765,
117.385697602806)) ;
#159140=CARTESIAN_POINT('Ctrl Pts',(-11.7510043904013,-14.2371768824059,
117.361466485342)) ;
#159141=CARTESIAN_POINT('Ctrl Pts',(-11.7372130842249,-14.2988733099436,
117.31946039005)) ;
#159142=CARTESIAN_POINT('Ctrl Pts',(-11.7234217780486,-14.3605697374812,
117.277454294757)) ;
#159143=CARTESIAN_POINT('Ctrl Pts',(-11.649617959508,-14.3605697948403,
117.301685412221)) ;
#159144=CARTESIAN_POINT('Ctrl Pts',(-11.5758141409673,-14.3605698521993,
117.325916529686)) ;
#159145=CARTESIAN_POINT('Ctrl Pts',(-11.5896054471436,-14.2988734246617,
117.367922624978)) ;
#159146=CARTESIAN_POINT('Ctrl Pts',(-11.5345577224684,-14.0989764690058,
117.164944532834)) ;
#159147=CARTESIAN_POINT('Ctrl Pts',(-11.5529430146087,-14.0511462695814,
117.220943168205)) ;
#159148=CARTESIAN_POINT('Ctrl Pts',(-11.6267468380803,-14.0511461903864,
117.19671206576)) ;
#159149=CARTESIAN_POINT('Ctrl Pts',(-11.700550661552,-14.0511461111915,
117.172480963314)) ;
#159150=CARTESIAN_POINT('Ctrl Pts',(-11.6821653694116,-14.0989763106159,
117.116482327944)) ;
#159151=CARTESIAN_POINT('Ctrl Pts',(-11.6637800772713,-14.1468065100403,
117.060483692574)) ;
#159152=CARTESIAN_POINT('Ctrl Pts',(-11.5899762537996,-14.1468065892353,
117.084714795019)) ;
#159153=CARTESIAN_POINT('Ctrl Pts',(-11.516172430328,-14.1468066684302,
117.108945897464)) ;
#159154=CARTESIAN_POINT('Ctrl Pts',(-11.5345577224684,-14.0989764690058,
117.164944532834)) ;
#159155=CARTESIAN_POINT('Ctrl Pts',(-11.4980687401448,-13.8484694868484,
117.018190484838)) ;
#159156=CARTESIAN_POINT('Ctrl Pts',(-11.5197655262105,-13.8180580458534,
117.084275396472)) ;
#159157=CARTESIAN_POINT('Ctrl Pts',(-11.5935693565242,-13.8180579489714,
117.060044314866)) ;
#159158=CARTESIAN_POINT('Ctrl Pts',(-11.6673731868378,-13.8180578520894,
117.035813233261)) ;
#159159=CARTESIAN_POINT('Ctrl Pts',(-11.645676400772,-13.8484692930843,
116.969728321627)) ;
#159160=CARTESIAN_POINT('Ctrl Pts',(-11.6239796147063,-13.8788807340793,
116.903643409994)) ;
#159161=CARTESIAN_POINT('Ctrl Pts',(-11.5501757843926,-13.8788808309613,
116.9278744916)) ;
#159162=CARTESIAN_POINT('Ctrl Pts',(-11.476371954079,-13.8788809278433,
116.952105573205)) ;
#159163=CARTESIAN_POINT('Ctrl Pts',(-11.4980687401448,-13.8484694868484,
117.018190484838)) ;
#159164=CARTESIAN_POINT('Ctrl Pts',(-11.484185252244,-13.5679794956402,
116.940440639052)) ;
#159165=CARTESIAN_POINT('Ctrl Pts',(-11.5076170750098,-13.5571060309524,
117.011810192564)) ;
#159166=CARTESIAN_POINT('Ctrl Pts',(-11.5814209137794,-13.5571059245038,
116.987579136714)) ;
#159167=CARTESIAN_POINT('Ctrl Pts',(-11.6552247525489,-13.5571058180553,
116.963348080864)) ;
#159168=CARTESIAN_POINT('Ctrl Pts',(-11.6317929297832,-13.567979282743,
116.891978527352)) ;
#159169=CARTESIAN_POINT('Ctrl Pts',(-11.6083611070174,-13.5788527474308,
116.820608973841)) ;
#159170=CARTESIAN_POINT('Ctrl Pts',(-11.5345572682478,-13.5788528538794,
116.844840029691)) ;
#159171=CARTESIAN_POINT('Ctrl Pts',(-11.4607534294783,-13.578852960328,
116.869071085541)) ;
#159172=CARTESIAN_POINT('Ctrl Pts',(-11.484185252244,-13.5679794956402,
116.940440639052)) ;
#159173=CARTESIAN_POINT('Ctrl Pts',(-11.4942413352023,-13.2778704302602,
116.935732247541)) ;
#159174=CARTESIAN_POINT('Ctrl Pts',(-11.5177367482968,-13.2872353982741,
117.007295486949)) ;
#159175=CARTESIAN_POINT('Ctrl Pts',(-11.5915405960583,-13.2872352908657,
116.983064458487)) ;
#159176=CARTESIAN_POINT('Ctrl Pts',(-11.6653444438198,-13.2872351834573,
116.958833430025)) ;
#159177=CARTESIAN_POINT('Ctrl Pts',(-11.6418490307253,-13.2778702154433,
116.887270190616)) ;
#159178=CARTESIAN_POINT('Ctrl Pts',(-11.6183536176309,-13.2685052474294,
116.815706951208)) ;
#159179=CARTESIAN_POINT('Ctrl Pts',(-11.5445497698694,-13.2685053548378,
116.83993797967)) ;
#159180=CARTESIAN_POINT('Ctrl Pts',(-11.4707459221079,-13.2685054622462,
116.864169008132)) ;
#159181=CARTESIAN_POINT('Ctrl Pts',(-11.4942413352023,-13.2778704302602,
116.935732247541)) ;
#159182=CARTESIAN_POINT('Ctrl Pts',(-11.5283649580948,-12.9966579805532,
117.004198786349)) ;
#159183=CARTESIAN_POINT('Ctrl Pts',(-11.5502466916195,-13.0256699682594,
117.070847018154)) ;
#159184=CARTESIAN_POINT('Ctrl Pts',(-11.6240505481439,-13.025669868452,
117.046616016382)) ;
#159185=CARTESIAN_POINT('Ctrl Pts',(-11.6978544046683,-13.0256697686447,
117.02238501461)) ;
#159186=CARTESIAN_POINT('Ctrl Pts',(-11.6759726711435,-12.9966577809386,
116.955736782806)) ;
#159187=CARTESIAN_POINT('Ctrl Pts',(-11.6540909376187,-12.9676457932324,
116.889088551001)) ;
#159188=CARTESIAN_POINT('Ctrl Pts',(-11.5802870810944,-12.9676458930398,
116.913319552772)) ;
#159189=CARTESIAN_POINT('Ctrl Pts',(-11.50648322457,-12.9676459928471,116.937550554544)) ;
#159190=CARTESIAN_POINT('Ctrl Pts',(-11.5283649580948,-12.9966579805532,
117.004198786349)) ;
#159191=CARTESIAN_POINT('Ctrl Pts',(-11.5851655684408,-12.7449733317735,
117.141625652285)) ;
#159192=CARTESIAN_POINT('Ctrl Pts',(-11.6038505096671,-12.7916002389954,
117.19853697052)) ;
#159193=CARTESIAN_POINT('Ctrl Pts',(-11.6776543737352,-12.7916001552318,
117.174305991725)) ;
#159194=CARTESIAN_POINT('Ctrl Pts',(-11.7514582378032,-12.7916000714681,
117.15007501293)) ;
#159195=CARTESIAN_POINT('Ctrl Pts',(-11.7327732965769,-12.7449731642463,
117.093163694695)) ;
#159196=CARTESIAN_POINT('Ctrl Pts',(-11.7140883553506,-12.6983462570244,
117.03625237646)) ;
#159197=CARTESIAN_POINT('Ctrl Pts',(-11.6402844912826,-12.698346340788,
117.060483355255)) ;
#159198=CARTESIAN_POINT('Ctrl Pts',(-11.5664806272145,-12.6983464245516,
117.08471433405)) ;
#159199=CARTESIAN_POINT('Ctrl Pts',(-11.5851655684408,-12.7449733317735,
117.141625652285)) ;
#159200=CARTESIAN_POINT('Ctrl Pts',(-11.6608769322514,-12.5424420519023,
117.336783089927)) ;
#159201=CARTESIAN_POINT('Ctrl Pts',(-11.6750372583365,-12.6032785791417,
117.379913160438)) ;
#159202=CARTESIAN_POINT('Ctrl Pts',(-11.7488411279863,-12.6032785174952,
117.355682198644)) ;
#159203=CARTESIAN_POINT('Ctrl Pts',(-11.8226449976362,-12.6032784558487,
117.33145123685)) ;
#159204=CARTESIAN_POINT('Ctrl Pts',(-11.8084846715511,-12.5424419286094,
117.28832116634)) ;
#159205=CARTESIAN_POINT('Ctrl Pts',(-11.794324345466,-12.48160540137,117.245191095829)) ;
#159206=CARTESIAN_POINT('Ctrl Pts',(-11.7205204758162,-12.4816054630165,
117.269422057623)) ;
#159207=CARTESIAN_POINT('Ctrl Pts',(-11.6467166061663,-12.481605524663,
117.293653019416)) ;
#159208=CARTESIAN_POINT('Ctrl Pts',(-11.6608769322514,-12.5424420519023,
117.336783089927)) ;
#159209=CARTESIAN_POINT('Ctrl Pts',(-11.751128641274,-12.4024494998622,
117.576178163021)) ;
#159210=CARTESIAN_POINT('Ctrl Pts',(-11.7597435525524,-12.4731509953254,
117.602417794707)) ;
#159211=CARTESIAN_POINT('Ctrl Pts',(-11.8335474252807,-12.4731509596195,
117.57818684229)) ;
#159212=CARTESIAN_POINT('Ctrl Pts',(-11.9073512980089,-12.4731509239136,
117.553955889872)) ;
#159213=CARTESIAN_POINT('Ctrl Pts',(-11.8987363867305,-12.4024494284505,
117.527716258186)) ;
#159214=CARTESIAN_POINT('Ctrl Pts',(-11.8901214754521,-12.3317479329873,
117.5014766265)) ;
#159215=CARTESIAN_POINT('Ctrl Pts',(-11.8163176027239,-12.3317479686932,
117.525707578917)) ;
#159216=CARTESIAN_POINT('Ctrl Pts',(-11.7425137299956,-12.331748004399,
117.549938531335)) ;
#159217=CARTESIAN_POINT('Ctrl Pts',(-11.751128641274,-12.4024494998622,
117.576178163021)) ;
#159218=CARTESIAN_POINT('Ctrl Pts',(-11.849749431196,-12.33540698977,117.841192600071)) ;
#159219=CARTESIAN_POINT('Ctrl Pts',(-11.8522235854152,-12.4108950254445,
117.848728476483)) ;
#159220=CARTESIAN_POINT('Ctrl Pts',(-11.9260274587751,-12.4108950163572,
117.824497525989)) ;
#159221=CARTESIAN_POINT('Ctrl Pts',(-11.999831332135,-12.4108950072698,
117.800266575496)) ;
#159222=CARTESIAN_POINT('Ctrl Pts',(-11.9973571779159,-12.3354069715953,
117.792730699084)) ;
#159223=CARTESIAN_POINT('Ctrl Pts',(-11.9948830236967,-12.2599189359207,
117.785194822671)) ;
#159224=CARTESIAN_POINT('Ctrl Pts',(-11.9210791503368,-12.2599189450081,
117.809425773165)) ;
#159225=CARTESIAN_POINT('Ctrl Pts',(-11.8472752769769,-12.2599189540954,
117.833656723658)) ;
#159226=CARTESIAN_POINT('Ctrl Pts',(-11.849749431196,-12.33540698977,117.841192600071)) ;
#159227=CARTESIAN_POINT('Ctrl Pts',(-11.9511794851965,-12.3455818235887,
118.114616538353)) ;
#159228=CARTESIAN_POINT('Ctrl Pts',(-11.9473106410994,-12.4204731523851,
118.102832665221)) ;
#159229=CARTESIAN_POINT('Ctrl Pts',(-12.0211145123507,-12.4204731683141,
118.078601708306)) ;
#159230=CARTESIAN_POINT('Ctrl Pts',(-12.0949183836021,-12.4204731842432,
118.05437075139)) ;
#159231=CARTESIAN_POINT('Ctrl Pts',(-12.0987872276992,-12.3455818554468,
118.066154624522)) ;
#159232=CARTESIAN_POINT('Ctrl Pts',(-12.1026560717964,-12.2706905266504,
118.077938497654)) ;
#159233=CARTESIAN_POINT('Ctrl Pts',(-12.028852200545,-12.2706905107213,
118.10216945457)) ;
#159234=CARTESIAN_POINT('Ctrl Pts',(-11.9550483292936,-12.2706904947923,
118.126400411485)) ;
#159235=CARTESIAN_POINT('Ctrl Pts',(-11.9511794851965,-12.3455818235887,
118.114616538353)) ;
#159236=CARTESIAN_POINT('Ctrl Pts',(-12.048568512048,-12.433061741337,118.375702938129)) ;
#159237=CARTESIAN_POINT('Ctrl Pts',(-12.0386297693431,-12.5019585481824,
118.345431133076)) ;
#159238=CARTESIAN_POINT('Ctrl Pts',(-12.1124336362693,-12.5019585842902,
118.321200162986)) ;
#159239=CARTESIAN_POINT('Ctrl Pts',(-12.1862375031954,-12.501958620398,
118.296969192897)) ;
#159240=CARTESIAN_POINT('Ctrl Pts',(-12.1961762459003,-12.4330618135526,
118.32724099795)) ;
#159241=CARTESIAN_POINT('Ctrl Pts',(-12.2061149886052,-12.3641650067072,
118.357512803003)) ;
#159242=CARTESIAN_POINT('Ctrl Pts',(-12.132311121679,-12.3641649705994,
118.381743773093)) ;
#159243=CARTESIAN_POINT('Ctrl Pts',(-12.0585072547529,-12.3641649344917,
118.405974743183)) ;
#159244=CARTESIAN_POINT('Ctrl Pts',(-12.048568512048,-12.433061741337,118.375702938129)) ;
#159245=CARTESIAN_POINT('Ctrl Pts',(-12.1352985452608,-12.5907670484714,
118.604444245422)) ;
#159246=CARTESIAN_POINT('Ctrl Pts',(-12.1200223854668,-12.6487569748398,
118.557915528971)) ;
#159247=CARTESIAN_POINT('Ctrl Pts',(-12.193826246934,-12.6487570251188,
118.533684542254)) ;
#159248=CARTESIAN_POINT('Ctrl Pts',(-12.2676301084012,-12.6487570753977,
118.509453555537)) ;
#159249=CARTESIAN_POINT('Ctrl Pts',(-12.2829062681952,-12.5907671490293,
118.555982271988)) ;
#159250=CARTESIAN_POINT('Ctrl Pts',(-12.2981824279892,-12.5327772226608,
118.60251098844)) ;
#159251=CARTESIAN_POINT('Ctrl Pts',(-12.224378566522,-12.5327771723819,
118.626741975157)) ;
#159252=CARTESIAN_POINT('Ctrl Pts',(-12.1505747050549,-12.5327771221029,
118.650972961874)) ;
#159253=CARTESIAN_POINT('Ctrl Pts',(-12.1352985452608,-12.5907670484714,
118.604444245422)) ;
#159254=CARTESIAN_POINT('Ctrl Pts',(-12.2062338243243,-12.8072730343164,
118.785110454359)) ;
#159255=CARTESIAN_POINT('Ctrl Pts',(-12.1867142471291,-12.8502341493777,
118.725656973039)) ;
#159256=CARTESIAN_POINT('Ctrl Pts',(-12.2605181025395,-12.8502342073388,
118.701425967874)) ;
#159257=CARTESIAN_POINT('Ctrl Pts',(-12.33432195795,-12.8502342652999,118.677194962709)) ;
#159258=CARTESIAN_POINT('Ctrl Pts',(-12.3538415351452,-12.8072731502386,
118.73664844403)) ;
#159259=CARTESIAN_POINT('Ctrl Pts',(-12.3733611123405,-12.7643120351774,
118.79610192535)) ;
#159260=CARTESIAN_POINT('Ctrl Pts',(-12.29955725693,-12.7643119772163,118.820332930515)) ;
#159261=CARTESIAN_POINT('Ctrl Pts',(-12.2257534015195,-12.7643119192552,
118.844563935679)) ;
#159262=CARTESIAN_POINT('Ctrl Pts',(-12.2062338243243,-12.8072730343164,
118.785110454359)) ;
#159263=CARTESIAN_POINT('Ctrl Pts',(-12.2572961681927,-13.0681776762317,
118.90514030015)) ;
#159264=CARTESIAN_POINT('Ctrl Pts',(-12.2349163490449,-13.0929875781858,
118.836974983176)) ;
#159265=CARTESIAN_POINT('Ctrl Pts',(-12.308720198304,-13.0929876362341,
118.812743959275)) ;
#159266=CARTESIAN_POINT('Ctrl Pts',(-12.3825240475632,-13.0929876942824,
118.788512935374)) ;
#159267=CARTESIAN_POINT('Ctrl Pts',(-12.4049038667109,-13.0681777923284,
118.856678252349)) ;
#159268=CARTESIAN_POINT('Ctrl Pts',(-12.4272836858587,-13.0433678903743,
118.924843569323)) ;
#159269=CARTESIAN_POINT('Ctrl Pts',(-12.3534798365995,-13.043367832326,
118.949074593224)) ;
#159270=CARTESIAN_POINT('Ctrl Pts',(-12.2796759873404,-13.0433677742776,
118.973305617125)) ;
#159271=CARTESIAN_POINT('Ctrl Pts',(-12.2572961681927,-13.0681776762317,
118.90514030015)) ;
#159272=CARTESIAN_POINT('Ctrl Pts',(-12.2852469770119,-13.3550287065478,
118.954680417514)) ;
#159273=CARTESIAN_POINT('Ctrl Pts',(-12.2616180631814,-13.3598480286535,
118.882710559486)) ;
#159274=CARTESIAN_POINT('Ctrl Pts',(-12.3354219072866,-13.3598480797462,
118.858479519887)) ;
#159275=CARTESIAN_POINT('Ctrl Pts',(-12.4092257513917,-13.3598481308389,
118.834248480288)) ;
#159276=CARTESIAN_POINT('Ctrl Pts',(-12.4328546652223,-13.3550288087332,
118.906218338317)) ;
#159277=CARTESIAN_POINT('Ctrl Pts',(-12.4564835790527,-13.3502094866275,
118.978188196345)) ;
#159278=CARTESIAN_POINT('Ctrl Pts',(-12.3826797349476,-13.3502094355348,
119.002419235944)) ;
#159279=CARTESIAN_POINT('Ctrl Pts',(-12.3088758908424,-13.3502093844422,
119.026650275543)) ;
#159280=CARTESIAN_POINT('Ctrl Pts',(-12.2852469770119,-13.3550287065478,
118.954680417514)) ;
#159281=CARTESIAN_POINT('Ctrl Pts',(-12.288870726614,-13.6436167217993,
118.930470264435)) ;
#159282=CARTESIAN_POINT('Ctrl Pts',(-12.2656825372451,-13.6282936387258,
118.859842781879)) ;
#159283=CARTESIAN_POINT('Ctrl Pts',(-12.3394863775681,-13.6282936821549,
118.83561173076)) ;
#159284=CARTESIAN_POINT('Ctrl Pts',(-12.413290217891,-13.6282937255841,
118.811380679642)) ;
#159285=CARTESIAN_POINT('Ctrl Pts',(-12.43647840726,-13.6436168086577,118.882008162198)) ;
#159286=CARTESIAN_POINT('Ctrl Pts',(-12.459666596629,-13.6589398917312,
118.952635644754)) ;
#159287=CARTESIAN_POINT('Ctrl Pts',(-12.385862756306,-13.6589398483021,
118.976866695873)) ;
#159288=CARTESIAN_POINT('Ctrl Pts',(-12.312058915983,-13.6589398048729,
119.001097746991)) ;
#159289=CARTESIAN_POINT('Ctrl Pts',(-12.288870726614,-13.6436167217993,
118.930470264435)) ;
#159290=CARTESIAN_POINT('Ctrl Pts',(-12.2688371151345,-13.9180811572707,
118.833953017997)) ;
#159291=CARTESIAN_POINT('Ctrl Pts',(-12.2477470847811,-13.8835710604602,
118.769716189091)) ;
#159292=CARTESIAN_POINT('Ctrl Pts',(-12.3215509228609,-13.8835710916854,
118.74548513114)) ;
#159293=CARTESIAN_POINT('Ctrl Pts',(-12.3953547609406,-13.8835711229105,
118.721254073189)) ;
#159294=CARTESIAN_POINT('Ctrl Pts',(-12.416444791294,-13.918081219721,118.785490902094)) ;
#159295=CARTESIAN_POINT('Ctrl Pts',(-12.4375348216475,-13.9525913165315,
118.849727730999)) ;
#159296=CARTESIAN_POINT('Ctrl Pts',(-12.3637309835677,-13.9525912853064,
118.873958788951)) ;
#159297=CARTESIAN_POINT('Ctrl Pts',(-12.289927145488,-13.9525912540812,
118.898189846902)) ;
#159298=CARTESIAN_POINT('Ctrl Pts',(-12.2688371151345,-13.9180811572707,
118.833953017997)) ;
#159299=CARTESIAN_POINT('Ctrl Pts',(-12.2271646134758,-14.156549136634,
118.671552459278)) ;
#159300=CARTESIAN_POINT('Ctrl Pts',(-12.2096863684391,-14.1053360637856,
118.618316545524)) ;
#159301=CARTESIAN_POINT('Ctrl Pts',(-12.2834902059413,-14.1053360831036,
118.594085485813)) ;
#159302=CARTESIAN_POINT('Ctrl Pts',(-12.3572940434434,-14.1053361024216,
118.569854426102)) ;
#159303=CARTESIAN_POINT('Ctrl Pts',(-12.3747722884801,-14.1565491752701,
118.623090339857)) ;
#159304=CARTESIAN_POINT('Ctrl Pts',(-12.3922505335167,-14.2077622481185,
118.676326253611)) ;
#159305=CARTESIAN_POINT('Ctrl Pts',(-12.3184466960146,-14.2077622288005,
118.700557313322)) ;
#159306=CARTESIAN_POINT('Ctrl Pts',(-12.2446428585124,-14.2077622094825,
118.724788373032)) ;
#159307=CARTESIAN_POINT('Ctrl Pts',(-12.2271646134758,-14.156549136634,
118.671552459278)) ;
#159308=CARTESIAN_POINT('Ctrl Pts',(-12.1674566622439,-14.3423727651068,
118.454127809899)) ;
#159309=CARTESIAN_POINT('Ctrl Pts',(-12.1548569449561,-14.2781068691163,
118.415751104352)) ;
#159310=CARTESIAN_POINT('Ctrl Pts',(-12.2286607833888,-14.2781068782219,
118.391520047475)) ;
#159311=CARTESIAN_POINT('Ctrl Pts',(-12.3024646218214,-14.2781068873274,
118.367288990599)) ;
#159312=CARTESIAN_POINT('Ctrl Pts',(-12.3150643391092,-14.342372783318,
118.405665696146)) ;
#159313=CARTESIAN_POINT('Ctrl Pts',(-12.327664056397,-14.4066386793085,
118.444042401693)) ;
#159314=CARTESIAN_POINT('Ctrl Pts',(-12.2538602179643,-14.406638670203,
118.468273458569)) ;
#159315=CARTESIAN_POINT('Ctrl Pts',(-12.1800563795317,-14.4066386610974,
118.492504515446)) ;
#159316=CARTESIAN_POINT('Ctrl Pts',(-12.1674566622439,-14.3423727651068,
118.454127809899)) ;
#159317=CARTESIAN_POINT('Ctrl Pts',(-12.0952414310603,-14.4613427108393,
118.198784751216)) ;
#159318=CARTESIAN_POINT('Ctrl Pts',(-12.0883974197828,-14.3886728717829,
118.177938997371)) ;
#159319=CARTESIAN_POINT('Ctrl Pts',(-12.1622012596057,-14.3886728745372,
118.153707944729)) ;
#159320=CARTESIAN_POINT('Ctrl Pts',(-12.2360050994286,-14.3886728772916,
118.129476892087)) ;
#159321=CARTESIAN_POINT('Ctrl Pts',(-12.242849110706,-14.461342716348,118.150322645932)) ;
#159322=CARTESIAN_POINT('Ctrl Pts',(-12.2496931219834,-14.5340125554044,
118.171168399777)) ;
#159323=CARTESIAN_POINT('Ctrl Pts',(-12.1758892821606,-14.5340125526501,
118.195399452419)) ;
#159324=CARTESIAN_POINT('Ctrl Pts',(-12.1020854423377,-14.5340125498957,
118.219630505062)) ;
#159325=CARTESIAN_POINT('Ctrl Pts',(-12.0952414310603,-14.4613427108393,
118.198784751216)) ;
#159326=CARTESIAN_POINT('Ctrl Pts',(-12.0156536366213,-14.5057889124528,
117.920757945584)) ;
#159327=CARTESIAN_POINT('Ctrl Pts',(-12.0150937248393,-14.4299056340327,
117.919052544731)) ;
#159328=CARTESIAN_POINT('Ctrl Pts',(-12.088897566724,-14.4299056336396,
117.894821498369)) ;
#159329=CARTESIAN_POINT('Ctrl Pts',(-12.1627014086088,-14.4299056332465,
117.870590452007)) ;
#159330=CARTESIAN_POINT('Ctrl Pts',(-12.1632613203908,-14.5057889116665,
117.87229585286)) ;
#159331=CARTESIAN_POINT('Ctrl Pts',(-12.1638212321729,-14.5816721900866,
117.874001253712)) ;
#159332=CARTESIAN_POINT('Ctrl Pts',(-12.0900173902881,-14.5816721904797,
117.898232300074)) ;
#159333=CARTESIAN_POINT('Ctrl Pts',(-12.0162135484033,-14.5816721908728,
117.922463346436)) ;
#159334=CARTESIAN_POINT('Ctrl Pts',(-12.0156536366213,-14.5057889124528,
117.920757945584)) ;
#159335=CARTESIAN_POINT('Ctrl Pts',(-11.9363592364177,-14.4724226584541,
117.643968542152)) ;
#159336=CARTESIAN_POINT('Ctrl Pts',(-11.9420651845438,-14.3987559090156,
117.661347939515)) ;
#159337=CARTESIAN_POINT('Ctrl Pts',(-12.0158690276237,-14.3987559084173,
117.637116896794)) ;
#159338=CARTESIAN_POINT('Ctrl Pts',(-12.0896728707036,-14.3987559078189,
117.612885854072)) ;
#159339=CARTESIAN_POINT('Ctrl Pts',(-12.0839669225775,-14.4724226572574,
117.595506456708)) ;
#159340=CARTESIAN_POINT('Ctrl Pts',(-12.0782609744514,-14.5460894066958,
117.578127059344)) ;
#159341=CARTESIAN_POINT('Ctrl Pts',(-12.0044571313715,-14.5460894072942,
117.602358102066)) ;
#159342=CARTESIAN_POINT('Ctrl Pts',(-11.9306532882916,-14.5460894078926,
117.626589144788)) ;
#159343=CARTESIAN_POINT('Ctrl Pts',(-11.9363592364177,-14.4724226584541,
117.643968542152)) ;
#159344=CARTESIAN_POINT('Ctrl Pts',(-11.8623371282566,-14.3630839653471,
117.382899183667)) ;
#159345=CARTESIAN_POINT('Ctrl Pts',(-11.8739575043683,-14.2969416918189,
117.418292974314)) ;
#159346=CARTESIAN_POINT('Ctrl Pts',(-11.9477613484913,-14.2969416928651,
117.394061934769)) ;
#159347=CARTESIAN_POINT('Ctrl Pts',(-12.0215651926142,-14.2969416939113,
117.369830895225)) ;
#159348=CARTESIAN_POINT('Ctrl Pts',(-12.0099448165026,-14.3630839674395,
117.334437104578)) ;
#159349=CARTESIAN_POINT('Ctrl Pts',(-11.9983244403909,-14.4292262409677,
117.299043313931)) ;
#159350=CARTESIAN_POINT('Ctrl Pts',(-11.9245205962679,-14.4292262399216,
117.323274353476)) ;
#159351=CARTESIAN_POINT('Ctrl Pts',(-11.850716752145,-14.4292262388754,
117.34750539302)) ;
#159352=CARTESIAN_POINT('Ctrl Pts',(-11.8623371282566,-14.3630839653471,
117.382899183667)) ;
#159353=CARTESIAN_POINT('Ctrl Pts',(-11.8008173863079,-14.1865023299291,
117.160124591948)) ;
#159354=CARTESIAN_POINT('Ctrl Pts',(-11.8174833681576,-14.132592518795,
117.210886483552)) ;
#159355=CARTESIAN_POINT('Ctrl Pts',(-11.8912872123,-14.1325925211688,117.186655444066)) ;
#159356=CARTESIAN_POINT('Ctrl Pts',(-11.9650910564424,-14.1325925235426,
117.162424404581)) ;
#159357=CARTESIAN_POINT('Ctrl Pts',(-11.9484250745928,-14.1865023346767,
117.111662512977)) ;
#159358=CARTESIAN_POINT('Ctrl Pts',(-11.9317590927431,-14.2404121458108,
117.060900621374)) ;
#159359=CARTESIAN_POINT('Ctrl Pts',(-11.8579552486006,-14.240412143437,
117.085131660859)) ;
#159360=CARTESIAN_POINT('Ctrl Pts',(-11.7841514044582,-14.2404121410632,
117.109362700344)) ;
#159361=CARTESIAN_POINT('Ctrl Pts',(-11.8008173863079,-14.1865023299291,
117.160124591948)) ;
#159362=CARTESIAN_POINT('Ctrl Pts',(-11.7563748042704,-13.9552367476643,
116.989354134913)) ;
#159363=CARTESIAN_POINT('Ctrl Pts',(-11.7769014328037,-13.91739633188,117.051874933419)) ;
#159364=CARTESIAN_POINT('Ctrl Pts',(-11.8507052765402,-13.917396334111,
117.027643892697)) ;
#159365=CARTESIAN_POINT('Ctrl Pts',(-11.9245091202767,-13.9173963363419,
117.003412851975)) ;
#159366=CARTESIAN_POINT('Ctrl Pts',(-11.9039824917435,-13.9552367521262,
116.94089205347)) ;
#159367=CARTESIAN_POINT('Ctrl Pts',(-11.8834558632103,-13.9930771679105,
116.878371254964)) ;
#159368=CARTESIAN_POINT('Ctrl Pts',(-11.8096520194738,-13.9930771656796,
116.902602295686)) ;
#159369=CARTESIAN_POINT('Ctrl Pts',(-11.7358481757372,-13.9930771634486,
116.926833336408)) ;
#159370=CARTESIAN_POINT('Ctrl Pts',(-11.7563748042704,-13.9552367476643,
116.989354134913)) ;
#159371=CARTESIAN_POINT('Ctrl Pts',(-11.7329833978953,-13.6844063432408,
116.882563304078)) ;
#159372=CARTESIAN_POINT('Ctrl Pts',(-11.7559091967072,-13.6654217630373,
116.952391588213)) ;
#159373=CARTESIAN_POINT('Ctrl Pts',(-11.8297130399375,-13.6654217622708,
116.928160545949)) ;
#159374=CARTESIAN_POINT('Ctrl Pts',(-11.9035168831679,-13.6654217615044,
116.903929503685)) ;
#159375=CARTESIAN_POINT('Ctrl Pts',(-11.8805910843559,-13.6844063417079,
116.834101219551)) ;
#159376=CARTESIAN_POINT('Ctrl Pts',(-11.857665285544,-13.7033909219114,
116.764272935417)) ;
#159377=CARTESIAN_POINT('Ctrl Pts',(-11.7838614423137,-13.7033909226779,
116.78850397768)) ;
#159378=CARTESIAN_POINT('Ctrl Pts',(-11.7100575990833,-13.7033909234443,
116.812735019944)) ;
#159379=CARTESIAN_POINT('Ctrl Pts',(-11.7329833978953,-13.6844063432408,
116.882563304078)) ;
#159380=CARTESIAN_POINT('Ctrl Pts',(-11.7332475390205,-13.395616216205,
116.847967590773)) ;
#159381=CARTESIAN_POINT('Ctrl Pts',(-11.7569209111697,-13.3967687826649,
116.920072862757)) ;
#159382=CARTESIAN_POINT('Ctrl Pts',(-11.8307247544843,-13.3967687773501,
116.89584182075)) ;
#159383=CARTESIAN_POINT('Ctrl Pts',(-11.9045285977989,-13.3967687720353,
116.871610778744)) ;
#159384=CARTESIAN_POINT('Ctrl Pts',(-11.8808552256497,-13.3956162055754,
116.799505506759)) ;
#159385=CARTESIAN_POINT('Ctrl Pts',(-11.8571818535005,-13.3944636391155,
116.727400234774)) ;
#159386=CARTESIAN_POINT('Ctrl Pts',(-11.7833780101859,-13.3944636444303,
116.751631276781)) ;
#159387=CARTESIAN_POINT('Ctrl Pts',(-11.7095741668713,-13.3944636497451,
116.775862318788)) ;
#159388=CARTESIAN_POINT('Ctrl Pts',(-11.7332475390205,-13.395616216205,
116.847967590773)) ;
#159389=CARTESIAN_POINT('Ctrl Pts',(-11.7576801957441,-13.1080920804484,
116.886949996486)) ;
#159390=CARTESIAN_POINT('Ctrl Pts',(-11.7804153341548,-13.1293224287734,
116.956197559996)) ;
#159391=CARTESIAN_POINT('Ctrl Pts',(-11.8542191783384,-13.1293224180304,
116.931966520636)) ;
#159392=CARTESIAN_POINT('Ctrl Pts',(-11.9280230225219,-13.1293224072874,
116.907735481276)) ;
#159393=CARTESIAN_POINT('Ctrl Pts',(-11.9052878841112,-13.1080920589624,
116.838487917765)) ;
#159394=CARTESIAN_POINT('Ctrl Pts',(-11.8825527457004,-13.0868617106374,
116.769240354255)) ;
#159395=CARTESIAN_POINT('Ctrl Pts',(-11.8087489015169,-13.0868617213805,
116.793471393615)) ;
#159396=CARTESIAN_POINT('Ctrl Pts',(-11.7349450573333,-13.0868617321235,
116.817702432975)) ;
#159397=CARTESIAN_POINT('Ctrl Pts',(-11.7576801957441,-13.1080920804484,
116.886949996486)) ;
#159398=CARTESIAN_POINT('Ctrl Pts',(-11.8057887216514,-12.8414911099526,
116.997851240026)) ;
#159399=CARTESIAN_POINT('Ctrl Pts',(-11.8259351949678,-12.8813675737048,
117.059214147502)) ;
#159400=CARTESIAN_POINT('Ctrl Pts',(-11.8997390414271,-12.8813675568765,
117.034983115074)) ;
#159401=CARTESIAN_POINT('Ctrl Pts',(-11.9735428878864,-12.8813675400482,
117.010752082645)) ;
#159402=CARTESIAN_POINT('Ctrl Pts',(-11.95339641457,-12.8414910762961,116.949389175168)) ;
#159403=CARTESIAN_POINT('Ctrl Pts',(-11.9332499412537,-12.8016146125439,
116.888026267692)) ;
#159404=CARTESIAN_POINT('Ctrl Pts',(-11.8594460947944,-12.8016146293722,
116.912257300121)) ;
#159405=CARTESIAN_POINT('Ctrl Pts',(-11.7856422483351,-12.8016146462005,
116.936488332549)) ;
#159406=CARTESIAN_POINT('Ctrl Pts',(-11.8057887216514,-12.8414911099526,
116.997851240026)) ;
#159407=CARTESIAN_POINT('Ctrl Pts',(-11.8738646701692,-12.6185827250958,
117.169942474425)) ;
#159408=CARTESIAN_POINT('Ctrl Pts',(-11.8900165906483,-12.6740802978787,
117.219138618594)) ;
#159409=CARTESIAN_POINT('Ctrl Pts',(-11.9638204397661,-12.6740802801009,
117.194907594263)) ;
#159410=CARTESIAN_POINT('Ctrl Pts',(-12.037624288884,-12.674080262323,117.170676569932)) ;
#159411=CARTESIAN_POINT('Ctrl Pts',(-12.0214723684048,-12.6185826895401,
117.121480425762)) ;
#159412=CARTESIAN_POINT('Ctrl Pts',(-12.0053204479257,-12.5630851167572,
117.072284281593)) ;
#159413=CARTESIAN_POINT('Ctrl Pts',(-11.9315165988079,-12.563085134535,
117.096515305924)) ;
#159414=CARTESIAN_POINT('Ctrl Pts',(-11.85771274969,-12.5630851523128,117.120746330255)) ;
#159415=CARTESIAN_POINT('Ctrl Pts',(-11.8738646701692,-12.6185827250958,
117.169942474425)) ;
#159416=CARTESIAN_POINT('Ctrl Pts',(-11.959020038101,-12.4509854490646,
117.393736018184)) ;
#159417=CARTESIAN_POINT('Ctrl Pts',(-11.969985920216,-12.518265407944,117.427136326441)) ;
#159418=CARTESIAN_POINT('Ctrl Pts',(-12.0437897731662,-12.5182653912533,
117.402905313782)) ;
#159419=CARTESIAN_POINT('Ctrl Pts',(-12.1175936261163,-12.5182653745627,
117.378674301124)) ;
#159420=CARTESIAN_POINT('Ctrl Pts',(-12.1066277440013,-12.4509854156833,
117.345273992867)) ;
#159421=CARTESIAN_POINT('Ctrl Pts',(-12.0956618618863,-12.383705456804,
117.311873684609)) ;
#159422=CARTESIAN_POINT('Ctrl Pts',(-12.0218580089361,-12.3837054734946,
117.336104697268)) ;
#159423=CARTESIAN_POINT('Ctrl Pts',(-11.948054155986,-12.3837054901852,
117.360335709926)) ;
#159424=CARTESIAN_POINT('Ctrl Pts',(-11.959020038101,-12.4509854490646,
117.393736018184)) ;
#159425=CARTESIAN_POINT('Ctrl Pts',(-12.0550313167262,-12.3534810644787,
117.650738776618)) ;
#159426=CARTESIAN_POINT('Ctrl Pts',(-12.0600427070521,-12.427665920119,
117.666002663801)) ;
#159427=CARTESIAN_POINT('Ctrl Pts',(-12.1338465636051,-12.4276659104835,
117.641771662116)) ;
#159428=CARTESIAN_POINT('Ctrl Pts',(-12.2076504201582,-12.4276659008479,
117.617540660431)) ;
#159429=CARTESIAN_POINT('Ctrl Pts',(-12.2026390298322,-12.3534810452076,
117.602276773248)) ;
#159430=CARTESIAN_POINT('Ctrl Pts',(-12.1976276395063,-12.2792961895673,
117.587012886065)) ;
#159431=CARTESIAN_POINT('Ctrl Pts',(-12.1238237829533,-12.2792961992029,
117.61124388775)) ;
#159432=CARTESIAN_POINT('Ctrl Pts',(-12.0500199264003,-12.2792962088384,
117.635474889435)) ;
#159433=CARTESIAN_POINT('Ctrl Pts',(-12.0550313167262,-12.3534810644787,
117.650738776618)) ;
#159434=CARTESIAN_POINT('Ctrl Pts',(-12.1561839108002,-12.3320089256095,
117.923345972253)) ;
#159435=CARTESIAN_POINT('Ctrl Pts',(-12.1548744716883,-12.407800207037,
117.919357633003)) ;
#159436=CARTESIAN_POINT('Ctrl Pts',(-12.2286783313457,-12.407800209429,
117.895126640774)) ;
#159437=CARTESIAN_POINT('Ctrl Pts',(-12.302482191003,-12.4078002118209,
117.870895648545)) ;
#159438=CARTESIAN_POINT('Ctrl Pts',(-12.303791630115,-12.3320089303934,
117.874883987795)) ;
#159439=CARTESIAN_POINT('Ctrl Pts',(-12.305101069227,-12.2562176489658,
117.878872327045)) ;
#159440=CARTESIAN_POINT('Ctrl Pts',(-12.2312972095696,-12.2562176465738,
117.903103319274)) ;
#159441=CARTESIAN_POINT('Ctrl Pts',(-12.1574933499122,-12.2562176441819,
117.927334311503)) ;
#159442=CARTESIAN_POINT('Ctrl Pts',(-12.1561839108002,-12.3320089256095,
117.923345972253)) ;
#159443=CARTESIAN_POINT('Ctrl Pts',(-12.2558122040571,-12.3884256006082,
118.1913322941)) ;
#159444=CARTESIAN_POINT('Ctrl Pts',(-12.2482788311864,-12.4603875127443,
118.168386857015)) ;
#159445=CARTESIAN_POINT('Ctrl Pts',(-12.3220826926037,-12.4603875316984,
118.144155870146)) ;
#159446=CARTESIAN_POINT('Ctrl Pts',(-12.3958865540209,-12.4603875506525,
118.119924883277)) ;
#159447=CARTESIAN_POINT('Ctrl Pts',(-12.4034199268916,-12.3884256385165,
118.142870320362)) ;
#159448=CARTESIAN_POINT('Ctrl Pts',(-12.4109532997624,-12.3164637263805,
118.165815757446)) ;
#159449=CARTESIAN_POINT('Ctrl Pts',(-12.3371494383451,-12.3164637074263,
118.190046744315)) ;
#159450=CARTESIAN_POINT('Ctrl Pts',(-12.2633455769279,-12.3164636884722,
118.214277731184)) ;
#159451=CARTESIAN_POINT('Ctrl Pts',(-12.2558122040571,-12.3884256006082,
118.1913322941)) ;
#159452=CARTESIAN_POINT('Ctrl Pts',(-12.3475394657345,-12.5185566369419,
118.43526353432)) ;
#159453=CARTESIAN_POINT('Ctrl Pts',(-12.3343246291813,-12.5815371501028,
118.395013275716)) ;
#159454=CARTESIAN_POINT('Ctrl Pts',(-12.4081284904738,-12.5815371883386,
118.370782288467)) ;
#159455=CARTESIAN_POINT('Ctrl Pts',(-12.4819323517663,-12.5815372265744,
118.346551301219)) ;
#159456=CARTESIAN_POINT('Ctrl Pts',(-12.4951471883196,-12.5185567134136,
118.386801559822)) ;
#159457=CARTESIAN_POINT('Ctrl Pts',(-12.5083620248728,-12.4555762002527,
118.427051818425)) ;
#159458=CARTESIAN_POINT('Ctrl Pts',(-12.4345581635803,-12.4555761620169,
118.451282805674)) ;
#159459=CARTESIAN_POINT('Ctrl Pts',(-12.3607543022878,-12.4555761237811,
118.475513792923)) ;
#159460=CARTESIAN_POINT('Ctrl Pts',(-12.3475394657345,-12.5185566369419,
118.43526353432)) ;
#159461=CARTESIAN_POINT('Ctrl Pts',(-12.4255960408986,-12.7128146761132,
118.637581654736)) ;
#159462=CARTESIAN_POINT('Ctrl Pts',(-12.4076454894822,-12.7623237651114,
118.582907172911)) ;
#159463=CARTESIAN_POINT('Ctrl Pts',(-12.4814493485287,-12.7623238229043,
118.558676178821)) ;
#159464=CARTESIAN_POINT('Ctrl Pts',(-12.5552532075751,-12.7623238806971,
118.534445184731)) ;
#159465=CARTESIAN_POINT('Ctrl Pts',(-12.5732037589916,-12.7128147916989,
118.589119666556)) ;
#159466=CARTESIAN_POINT('Ctrl Pts',(-12.591154310408,-12.6633057027007,
118.643794148382)) ;
#159467=CARTESIAN_POINT('Ctrl Pts',(-12.5173504513616,-12.6633056449079,
118.668025142472)) ;
#159468=CARTESIAN_POINT('Ctrl Pts',(-12.4435465923151,-12.663305587115,
118.692256136562)) ;
#159469=CARTESIAN_POINT('Ctrl Pts',(-12.4255960408986,-12.7128146761132,
118.637581654736)) ;
#159470=CARTESIAN_POINT('Ctrl Pts',(-12.4854118400066,-12.9591843124397,
118.784128401409)) ;
#159471=CARTESIAN_POINT('Ctrl Pts',(-12.4639964600509,-12.9915649142031,
118.718900611066)) ;
#159472=CARTESIAN_POINT('Ctrl Pts',(-12.537800314808,-12.9915649910661,
118.694669603911)) ;
#159473=CARTESIAN_POINT('Ctrl Pts',(-12.6116041695651,-12.9915650679292,
118.670438596757)) ;
#159474=CARTESIAN_POINT('Ctrl Pts',(-12.6330195495208,-12.9591844661657,
118.735666387099)) ;
#159475=CARTESIAN_POINT('Ctrl Pts',(-12.6544349294764,-12.9268038644023,
118.800894177441)) ;
#159476=CARTESIAN_POINT('Ctrl Pts',(-12.5806310747193,-12.9268037875393,
118.825125184596)) ;
#159477=CARTESIAN_POINT('Ctrl Pts',(-12.5068272199622,-12.9268037106763,
118.849356191751)) ;
#159478=CARTESIAN_POINT('Ctrl Pts',(-12.4854118400066,-12.9591843124397,
118.784128401409)) ;
#159479=CARTESIAN_POINT('Ctrl Pts',(-12.5227062774273,-13.2359003760254,
118.862430198041)) ;
#159480=CARTESIAN_POINT('Ctrl Pts',(-12.4993863439673,-13.2490083473187,
118.791401445121)) ;
#159481=CARTESIAN_POINT('Ctrl Pts',(-12.5731901922074,-13.24900843612,118.767170418116)) ;
#159482=CARTESIAN_POINT('Ctrl Pts',(-12.6469940404474,-13.2490085249213,
118.742939391112)) ;
#159483=CARTESIAN_POINT('Ctrl Pts',(-12.6703139739074,-13.235900553628,
118.813968144031)) ;
#159484=CARTESIAN_POINT('Ctrl Pts',(-12.6936339073674,-13.2227925823347,
118.884996896951)) ;
#159485=CARTESIAN_POINT('Ctrl Pts',(-12.6198300591273,-13.2227924935334,
118.909227923956)) ;
#159486=CARTESIAN_POINT('Ctrl Pts',(-12.5460262108872,-13.2227924047321,
118.93345895096)) ;
#159487=CARTESIAN_POINT('Ctrl Pts',(-12.5227062774273,-13.2359003760254,
118.862430198041)) ;
#159488=CARTESIAN_POINT('Ctrl Pts',(-12.5363357220994,-13.5269168879405,
118.86847314923)) ;
#159489=CARTESIAN_POINT('Ctrl Pts',(-12.5127641692558,-13.5197262961672,
118.796678004376)) ;
#159490=CARTESIAN_POINT('Ctrl Pts',(-12.5865680098084,-13.5197263915446,
118.772446953957)) ;
#159491=CARTESIAN_POINT('Ctrl Pts',(-12.6603718503611,-13.5197264869221,
118.748215903538)) ;
#159492=CARTESIAN_POINT('Ctrl Pts',(-12.6839434032046,-13.5269170786954,
118.820011048392)) ;
#159493=CARTESIAN_POINT('Ctrl Pts',(-12.7075149560482,-13.5341076704686,
118.891806193245)) ;
#159494=CARTESIAN_POINT('Ctrl Pts',(-12.6337111154956,-13.5341075750912,
118.916037243664)) ;
#159495=CARTESIAN_POINT('Ctrl Pts',(-12.559907274943,-13.5341074797137,
118.940268294084)) ;
#159496=CARTESIAN_POINT('Ctrl Pts',(-12.5363357220994,-13.5269168879405,
118.86847314923)) ;
#159497=CARTESIAN_POINT('Ctrl Pts',(-12.5257513802662,-13.8100818853549,
118.80078051953)) ;
#159498=CARTESIAN_POINT('Ctrl Pts',(-12.5036179456418,-13.7831112951298,
118.733365650822)) ;
#159499=CARTESIAN_POINT('Ctrl Pts',(-12.5774217778562,-13.7831113889682,
118.709134575006)) ;
#159500=CARTESIAN_POINT('Ctrl Pts',(-12.6512256100705,-13.7831114828066,
118.68490349919)) ;
#159501=CARTESIAN_POINT('Ctrl Pts',(-12.6733590446949,-13.8100820730318,
118.752318367897)) ;
#159502=CARTESIAN_POINT('Ctrl Pts',(-12.6954924793192,-13.837052663257,
118.819733236605)) ;
#159503=CARTESIAN_POINT('Ctrl Pts',(-12.6216886471049,-13.8370525694185,
118.843964312421)) ;
#159504=CARTESIAN_POINT('Ctrl Pts',(-12.5478848148905,-13.8370524755801,
118.868195388238)) ;
#159505=CARTESIAN_POINT('Ctrl Pts',(-12.5257513802662,-13.8100818853549,
118.80078051953)) ;
#159506=CARTESIAN_POINT('Ctrl Pts',(-12.4923757936398,-14.0658493622321,
118.663565106864)) ;
#159507=CARTESIAN_POINT('Ctrl Pts',(-12.4732757223142,-14.0209825335161,
118.60538937341)) ;
#159508=CARTESIAN_POINT('Ctrl Pts',(-12.5470795463847,-14.0209826175788,
118.581158272789)) ;
#159509=CARTESIAN_POINT('Ctrl Pts',(-12.6208833704551,-14.0209827016415,
118.556927172168)) ;
#159510=CARTESIAN_POINT('Ctrl Pts',(-12.6399834417808,-14.0658495303575,
118.615102905622)) ;
#159511=CARTESIAN_POINT('Ctrl Pts',(-12.6590835131064,-14.1107163590735,
118.673278639076)) ;
#159512=CARTESIAN_POINT('Ctrl Pts',(-12.5852796890359,-14.1107162750108,
118.697509739697)) ;
#159513=CARTESIAN_POINT('Ctrl Pts',(-12.5114758649654,-14.1107161909481,
118.721740840318)) ;
#159514=CARTESIAN_POINT('Ctrl Pts',(-12.4923757936398,-14.0658493622321,
118.663565106864)) ;
#159515=CARTESIAN_POINT('Ctrl Pts',(-12.4395119409733,-14.2744004374724,
118.467090668042)) ;
#159516=CARTESIAN_POINT('Ctrl Pts',(-12.4248082411244,-14.2149073780421,
118.4223055728)) ;
#159517=CARTESIAN_POINT('Ctrl Pts',(-12.4986120583206,-14.2149074440193,
118.398074451241)) ;
#159518=CARTESIAN_POINT('Ctrl Pts',(-12.5724158755168,-14.2149075099964,
118.373843329682)) ;
#159519=CARTESIAN_POINT('Ctrl Pts',(-12.5871195753657,-14.2744005694268,
118.418628424924)) ;
#159520=CARTESIAN_POINT('Ctrl Pts',(-12.6018232752146,-14.3338936288571,
118.463413520166)) ;
#159521=CARTESIAN_POINT('Ctrl Pts',(-12.5280194580184,-14.3338935628799,
118.487644641725)) ;
#159522=CARTESIAN_POINT('Ctrl Pts',(-12.4542156408222,-14.3338934969028,
118.511875763284)) ;
#159523=CARTESIAN_POINT('Ctrl Pts',(-12.4395119409733,-14.2744004374724,
118.467090668042)) ;
#159524=CARTESIAN_POINT('Ctrl Pts',(-12.371795140951,-14.4215076088756,
118.225429654782)) ;
#159525=CARTESIAN_POINT('Ctrl Pts',(-12.362530137544,-14.3516564443396,
118.197209951397)) ;
#159526=CARTESIAN_POINT('Ctrl Pts',(-12.4363339498473,-14.3516564861261,
118.172978814935)) ;
#159527=CARTESIAN_POINT('Ctrl Pts',(-12.5101377621506,-14.3516565279127,
118.148747678473)) ;
#159528=CARTESIAN_POINT('Ctrl Pts',(-12.5194027655576,-14.4215076924487,
118.176967381858)) ;
#159529=CARTESIAN_POINT('Ctrl Pts',(-12.5286677689646,-14.4913588569847,
118.205187085244)) ;
#159530=CARTESIAN_POINT('Ctrl Pts',(-12.4548639566613,-14.4913588151982,
118.229418221706)) ;
#159531=CARTESIAN_POINT('Ctrl Pts',(-12.381060144358,-14.4913587734116,
118.253649358168)) ;
#159532=CARTESIAN_POINT('Ctrl Pts',(-12.371795140951,-14.4215076088756,
118.225429654782)) ;
#159533=CARTESIAN_POINT('Ctrl Pts',(-12.2946403903294,-14.4970287487176,
117.954986337942)) ;
#159534=CARTESIAN_POINT('Ctrl Pts',(-12.2914816993358,-14.421801684016,
117.945365476924)) ;
#159535=CARTESIAN_POINT('Ctrl Pts',(-12.3652855092019,-14.42180169783,117.921134333039)) ;
#159536=CARTESIAN_POINT('Ctrl Pts',(-12.4390893190681,-14.421801711644,
117.896903189154)) ;
#159537=CARTESIAN_POINT('Ctrl Pts',(-12.4422480100617,-14.4970287763456,
117.906524050172)) ;
#159538=CARTESIAN_POINT('Ctrl Pts',(-12.4454067010553,-14.5722558410471,
117.91614491119)) ;
#159539=CARTESIAN_POINT('Ctrl Pts',(-12.3716028911892,-14.5722558272332,
117.940376055076)) ;
#159540=CARTESIAN_POINT('Ctrl Pts',(-12.297799081323,-14.5722558134192,
117.964607198961)) ;
#159541=CARTESIAN_POINT('Ctrl Pts',(-12.2946403903294,-14.4970287487176,
117.954986337942)) ;
#159542=CARTESIAN_POINT('Ctrl Pts',(-12.2142494904348,-14.495364180026,
117.674634887753)) ;
#159543=CARTESIAN_POINT('Ctrl Pts',(-12.2174331076008,-14.420141562785,
117.684331674045)) ;
#159544=CARTESIAN_POINT('Ctrl Pts',(-12.2912369177925,-14.4201415475385,
117.660100531151)) ;
#159545=CARTESIAN_POINT('Ctrl Pts',(-12.3650407279842,-14.420141532292,
117.635869388258)) ;
#159546=CARTESIAN_POINT('Ctrl Pts',(-12.3618571108181,-14.495364149533,
117.626172601966)) ;
#159547=CARTESIAN_POINT('Ctrl Pts',(-12.3586734936521,-14.570586766774,
117.616475815674)) ;
#159548=CARTESIAN_POINT('Ctrl Pts',(-12.2848696834604,-14.5705867820204,
117.640706958568)) ;
#159549=CARTESIAN_POINT('Ctrl Pts',(-12.2110658732687,-14.5705867972669,
117.664938101461)) ;
#159550=CARTESIAN_POINT('Ctrl Pts',(-12.2142494904348,-14.495364180026,
117.674634887753)) ;
#159551=CARTESIAN_POINT('Ctrl Pts',(-12.1371207254048,-14.4159600881982,
117.404140731358)) ;
#159552=CARTESIAN_POINT('Ctrl Pts',(-12.1464300057665,-14.3461687677575,
117.432495299325)) ;
#159553=CARTESIAN_POINT('Ctrl Pts',(-12.2202338191202,-14.346168725633,
117.408264166062)) ;
#159554=CARTESIAN_POINT('Ctrl Pts',(-12.294037632474,-14.3461686835086,
117.3840330328)) ;
#159555=CARTESIAN_POINT('Ctrl Pts',(-12.2847283521122,-14.4159600039494,
117.355678464832)) ;
#159556=CARTESIAN_POINT('Ctrl Pts',(-12.2754190717505,-14.4857513243901,
117.327323896865)) ;
#159557=CARTESIAN_POINT('Ctrl Pts',(-12.2016152583968,-14.4857513665145,
117.351555030128)) ;
#159558=CARTESIAN_POINT('Ctrl Pts',(-12.1278114450431,-14.485751408639,
117.37578616339)) ;
#159559=CARTESIAN_POINT('Ctrl Pts',(-12.1371207254048,-14.4159600881982,
117.404140731358)) ;
#159560=CARTESIAN_POINT('Ctrl Pts',(-12.0701819932153,-14.2660479877099,
117.164946413806)) ;
#159561=CARTESIAN_POINT('Ctrl Pts',(-12.0849092529423,-14.2066193411526,
117.209803272681)) ;
#159562=CARTESIAN_POINT('Ctrl Pts',(-12.1587130714868,-14.206619276698,
117.185572155228)) ;
#159563=CARTESIAN_POINT('Ctrl Pts',(-12.2325168900312,-14.2066192122434,
117.161341037776)) ;
#159564=CARTESIAN_POINT('Ctrl Pts',(-12.2177896303041,-14.2660478588008,
117.1164841789)) ;
#159565=CARTESIAN_POINT('Ctrl Pts',(-12.2030623705771,-14.3254765053581,
117.071627320025)) ;
#159566=CARTESIAN_POINT('Ctrl Pts',(-12.1292585520327,-14.3254765698126,
117.095858437478)) ;
#159567=CARTESIAN_POINT('Ctrl Pts',(-12.0554547334883,-14.3254766342672,
117.12008955493)) ;
#159568=CARTESIAN_POINT('Ctrl Pts',(-12.0701819932153,-14.2660479877099,
117.164946413806)) ;
#159569=CARTESIAN_POINT('Ctrl Pts',(-12.0180738968896,-14.0549162780305,
116.970748910434)) ;
#159570=CARTESIAN_POINT('Ctrl Pts',(-12.0371954975587,-14.010139153776,
117.028990222714)) ;
#159571=CARTESIAN_POINT('Ctrl Pts',(-12.1109993231329,-14.0101390737133,
117.004759126673)) ;
#159572=CARTESIAN_POINT('Ctrl Pts',(-12.184803148707,-14.0101389936507,
116.980528030632)) ;
#159573=CARTESIAN_POINT('Ctrl Pts',(-12.1656815480379,-14.0549161179053,
116.922286718351)) ;
#159574=CARTESIAN_POINT('Ctrl Pts',(-12.1465599473688,-14.0996932421598,
116.864045406071)) ;
#159575=CARTESIAN_POINT('Ctrl Pts',(-12.0727561217947,-14.0996933222224,
116.888276502112)) ;
#159576=CARTESIAN_POINT('Ctrl Pts',(-11.9989522962205,-14.0996934022851,
116.912507598153)) ;
#159577=CARTESIAN_POINT('Ctrl Pts',(-12.0180738968896,-14.0549162780305,
116.970748910434)) ;
#159578=CARTESIAN_POINT('Ctrl Pts',(-11.9857272141969,-13.7973888984154,
116.836670452939)) ;
#159579=CARTESIAN_POINT('Ctrl Pts',(-12.0078717114481,-13.7705242930268,
116.904119020354)) ;
#159580=CARTESIAN_POINT('Ctrl Pts',(-12.0816755449335,-13.7705242060614,
116.87988794841)) ;
#159581=CARTESIAN_POINT('Ctrl Pts',(-12.155479378419,-13.770524119096,116.855656876465)) ;
#159582=CARTESIAN_POINT('Ctrl Pts',(-12.1333348811679,-13.7973887244846,
116.78820830905)) ;
#159583=CARTESIAN_POINT('Ctrl Pts',(-12.1111903839167,-13.8242533298732,
116.720759741635)) ;
#159584=CARTESIAN_POINT('Ctrl Pts',(-12.0373865504313,-13.8242534168386,
116.744990813579)) ;
#159585=CARTESIAN_POINT('Ctrl Pts',(-11.9635827169458,-13.824253503804,
116.769221885524)) ;
#159586=CARTESIAN_POINT('Ctrl Pts',(-11.9857272141969,-13.7973888984154,
116.836670452939)) ;
#159587=CARTESIAN_POINT('Ctrl Pts',(-11.9762272551923,-13.5143192821472,
116.772389751235)) ;
#159588=CARTESIAN_POINT('Ctrl Pts',(-11.999799643485,-13.5071778533561,
116.844187444272)) ;
#159589=CARTESIAN_POINT('Ctrl Pts',(-12.0736034846683,-13.507177766311,
116.819956395774)) ;
#159590=CARTESIAN_POINT('Ctrl Pts',(-12.1474073258517,-13.5071776792659,
116.795725347276)) ;
#159591=CARTESIAN_POINT('Ctrl Pts',(-12.1238349375591,-13.514319108057,
116.723927654239)) ;
#159592=CARTESIAN_POINT('Ctrl Pts',(-12.1002625492664,-13.5214605368481,
116.652129961202)) ;
#159593=CARTESIAN_POINT('Ctrl Pts',(-12.0264587080831,-13.5214606238932,
116.6763610097)) ;
#159594=CARTESIAN_POINT('Ctrl Pts',(-11.9526548668997,-13.5214607109383,
116.700592058198)) ;
#159595=CARTESIAN_POINT('Ctrl Pts',(-11.9762272551923,-13.5143192821472,
116.772389751235)) ;
#159596=CARTESIAN_POINT('Ctrl Pts',(-11.9909277151902,-13.2228141005811,
116.78161966851)) ;
#159597=CARTESIAN_POINT('Ctrl Pts',(-12.0142449048521,-13.236014362639,
116.85264006755)) ;
#159598=CARTESIAN_POINT('Ctrl Pts',(-12.0880487529386,-13.2360142841561,
116.828409040078)) ;
#159599=CARTESIAN_POINT('Ctrl Pts',(-12.1618526010251,-13.2360142056732,
116.804178012605)) ;
#159600=CARTESIAN_POINT('Ctrl Pts',(-12.1385354113632,-13.2228139436153,
116.733157613566)) ;
#159601=CARTESIAN_POINT('Ctrl Pts',(-12.1152182217013,-13.2096136815574,
116.662137214526)) ;
#159602=CARTESIAN_POINT('Ctrl Pts',(-12.0414143736148,-13.2096137600403,
116.686368241999)) ;
#159603=CARTESIAN_POINT('Ctrl Pts',(-11.9676105255282,-13.2096138385232,
116.710599269471)) ;
#159604=CARTESIAN_POINT('Ctrl Pts',(-11.9909277151902,-13.2228141005811,
116.78161966851)) ;
#159605=CARTESIAN_POINT('Ctrl Pts',(-12.0294614824962,-12.9463122499942,
116.863581031885)) ;
#159606=CARTESIAN_POINT('Ctrl Pts',(-12.0508561203109,-12.9788376519378,
116.928745648064)) ;
#159607=CARTESIAN_POINT('Ctrl Pts',(-12.1246599737822,-12.978837586653,
116.904514636993)) ;
#159608=CARTESIAN_POINT('Ctrl Pts',(-12.1984638272535,-12.9788375213682,
116.880283625922)) ;
#159609=CARTESIAN_POINT('Ctrl Pts',(-12.1770691894388,-12.9463121194246,
116.815119009743)) ;
#159610=CARTESIAN_POINT('Ctrl Pts',(-12.1556745516242,-12.913786717481,
116.749954393564)) ;
#159611=CARTESIAN_POINT('Ctrl Pts',(-12.0818706981529,-12.9137867827658,
116.774185404635)) ;
#159612=CARTESIAN_POINT('Ctrl Pts',(-12.0080668446816,-12.9137868480506,
116.798416415706)) ;
#159613=CARTESIAN_POINT('Ctrl Pts',(-12.0294614824962,-12.9463122499942,
116.863581031885)) ;
#159614=CARTESIAN_POINT('Ctrl Pts',(-12.0901776028958,-12.7025112775513,
117.012934916738)) ;
#159615=CARTESIAN_POINT('Ctrl Pts',(-12.1081017353665,-12.7521082971811,
117.067528933426)) ;
#159616=CARTESIAN_POINT('Ctrl Pts',(-12.1819055920202,-12.7521082496802,
117.043297932048)) ;
#159617=CARTESIAN_POINT('Ctrl Pts',(-12.255709448674,-12.7521082021794,
117.01906693067)) ;
#159618=CARTESIAN_POINT('Ctrl Pts',(-12.2377853162033,-12.7025111825496,
116.964472913982)) ;
#159619=CARTESIAN_POINT('Ctrl Pts',(-12.2198611837327,-12.6529141629198,
116.909878897294)) ;
#159620=CARTESIAN_POINT('Ctrl Pts',(-12.1460573270789,-12.6529142104206,
116.934109898672)) ;
#159621=CARTESIAN_POINT('Ctrl Pts',(-12.0722534704252,-12.6529142579215,
116.958340900049)) ;
#159622=CARTESIAN_POINT('Ctrl Pts',(-12.0901776028958,-12.7025112775513,
117.012934916738)) ;
#159623=CARTESIAN_POINT('Ctrl Pts',(-12.1687375174296,-12.5113386435153,
117.216879767183)) ;
#159624=CARTESIAN_POINT('Ctrl Pts',(-12.1819348220533,-12.5743584257443,
117.25707662878)) ;
#159625=CARTESIAN_POINT('Ctrl Pts',(-12.2557386802607,-12.5743583951879,
117.232845632134)) ;
#159626=CARTESIAN_POINT('Ctrl Pts',(-12.3295425384681,-12.5743583646314,
117.208614635489)) ;
#159627=CARTESIAN_POINT('Ctrl Pts',(-12.3163452338444,-12.5113385824024,
117.168417773891)) ;
#159628=CARTESIAN_POINT('Ctrl Pts',(-12.3031479292207,-12.4483188001733,
117.128220912294)) ;
#159629=CARTESIAN_POINT('Ctrl Pts',(-12.2293440710133,-12.4483188307298,
117.15245190894)) ;
#159630=CARTESIAN_POINT('Ctrl Pts',(-12.1555402128059,-12.4483188612862,
117.176682905585)) ;
#159631=CARTESIAN_POINT('Ctrl Pts',(-12.1687375174296,-12.5113386435153,
117.216879767183)) ;
#159632=CARTESIAN_POINT('Ctrl Pts',(-12.2612290461381,-12.3839986409936,
117.463033125205)) ;
#159633=CARTESIAN_POINT('Ctrl Pts',(-12.2687243980064,-12.45600534241,117.48586275853)) ;
#159634=CARTESIAN_POINT('Ctrl Pts',(-12.3425282553788,-12.4560053286552,
117.461631759341)) ;
#159635=CARTESIAN_POINT('Ctrl Pts',(-12.4163321127512,-12.4560053149005,
117.437400760152)) ;
#159636=CARTESIAN_POINT('Ctrl Pts',(-12.408836760883,-12.3839986134842,
117.414571126827)) ;
#159637=CARTESIAN_POINT('Ctrl Pts',(-12.4013414090147,-12.3119919120679,
117.391741493502)) ;
#159638=CARTESIAN_POINT('Ctrl Pts',(-12.3275375516422,-12.3119919258226,
117.415972492691)) ;
#159639=CARTESIAN_POINT('Ctrl Pts',(-12.2537336942698,-12.3119919395773,
117.44020349188)) ;
#159640=CARTESIAN_POINT('Ctrl Pts',(-12.2612290461381,-12.3839986409936,
117.463033125205)) ;
#159641=CARTESIAN_POINT('Ctrl Pts',(-12.3609719875208,-12.3313598679509,
117.731405074504)) ;
#159642=CARTESIAN_POINT('Ctrl Pts',(-12.3622475504806,-12.4071510797427,
117.735290234212)) ;
#159643=CARTESIAN_POINT('Ctrl Pts',(-12.4360514058846,-12.4071510785913,
117.711059229027)) ;
#159644=CARTESIAN_POINT('Ctrl Pts',(-12.5098552612885,-12.4071510774399,
117.686828223842)) ;
#159645=CARTESIAN_POINT('Ctrl Pts',(-12.5085796983286,-12.3313598656482,
117.682943064135)) ;
#159646=CARTESIAN_POINT('Ctrl Pts',(-12.5073041353688,-12.2555686538564,
117.679057904427)) ;
#159647=CARTESIAN_POINT('Ctrl Pts',(-12.4335002799649,-12.2555686550078,
117.703288909611)) ;
#159648=CARTESIAN_POINT('Ctrl Pts',(-12.3596964245609,-12.2555686561592,
117.727519914796)) ;
#159649=CARTESIAN_POINT('Ctrl Pts',(-12.3609719875208,-12.3313598679509,
117.731405074504)) ;
#159650=CARTESIAN_POINT('Ctrl Pts',(-12.4619148744611,-12.3561484752169,
118.003421771831)) ;
#159651=CARTESIAN_POINT('Ctrl Pts',(-12.4568776202729,-12.4303237529548,
117.988079108915)) ;
#159652=CARTESIAN_POINT('Ctrl Pts',(-12.5306814728019,-12.4303237603732,
117.963848094974)) ;
#159653=CARTESIAN_POINT('Ctrl Pts',(-12.6044853253309,-12.4303237677915,
117.939617081032)) ;
#159654=CARTESIAN_POINT('Ctrl Pts',(-12.6095225795191,-12.3561484900536,
117.954959743949)) ;
#159655=CARTESIAN_POINT('Ctrl Pts',(-12.6145598337073,-12.2819732123158,
117.970302406865)) ;
#159656=CARTESIAN_POINT('Ctrl Pts',(-12.5407559811783,-12.2819732048974,
117.994533420806)) ;
#159657=CARTESIAN_POINT('Ctrl Pts',(-12.4669521286493,-12.2819731974791,
118.018764434748)) ;
#159658=CARTESIAN_POINT('Ctrl Pts',(-12.4619148744611,-12.3561484752169,
118.003421771831)) ;
#159659=CARTESIAN_POINT('Ctrl Pts',(-12.558035703025,-12.4578681360596,
118.260559283857)) ;
#159660=CARTESIAN_POINT('Ctrl Pts',(-12.5470165166241,-12.5250537220818,
118.226996620417)) ;
#159661=CARTESIAN_POINT('Ctrl Pts',(-12.6208203656014,-12.5250537323896,
118.202765595658)) ;
#159662=CARTESIAN_POINT('Ctrl Pts',(-12.6946242145786,-12.5250537426973,
118.178534570898)) ;
#159663=CARTESIAN_POINT('Ctrl Pts',(-12.7056434009795,-12.4578681566752,
118.212097234338)) ;
#159664=CARTESIAN_POINT('Ctrl Pts',(-12.7166625873804,-12.390682570653,
118.245659897778)) ;
#159665=CARTESIAN_POINT('Ctrl Pts',(-12.6428587384032,-12.3906825603452,
118.269890922537)) ;
#159666=CARTESIAN_POINT('Ctrl Pts',(-12.5690548894259,-12.3906825500374,
118.294121947297)) ;
#159667=CARTESIAN_POINT('Ctrl Pts',(-12.558035703025,-12.4578681360596,
118.260559283857)) ;
#159668=CARTESIAN_POINT('Ctrl Pts',(-12.6418650591551,-12.6270814220524,
118.480600547495)) ;
#159669=CARTESIAN_POINT('Ctrl Pts',(-12.6257062539618,-12.6825528988753,
118.431383434374)) ;
#159670=CARTESIAN_POINT('Ctrl Pts',(-12.6995101005983,-12.6825529093536,
118.407152402485)) ;
#159671=CARTESIAN_POINT('Ctrl Pts',(-12.7733139472347,-12.6825529198319,
118.382921370596)) ;
#159672=CARTESIAN_POINT('Ctrl Pts',(-12.7894727524281,-12.627081443009,
118.432138483717)) ;
#159673=CARTESIAN_POINT('Ctrl Pts',(-12.8056315576213,-12.5716099661861,
118.481355596837)) ;
#159674=CARTESIAN_POINT('Ctrl Pts',(-12.7318277109849,-12.5716099557078,
118.505586628726)) ;
#159675=CARTESIAN_POINT('Ctrl Pts',(-12.6580238643484,-12.5716099452296,
118.529817660615)) ;
#159676=CARTESIAN_POINT('Ctrl Pts',(-12.6418650591551,-12.6270814220524,
118.480600547495)) ;
#159677=CARTESIAN_POINT('Ctrl Pts',(-12.709500616301,-12.8533401319523,
118.65115248197)) ;
#159678=CARTESIAN_POINT('Ctrl Pts',(-12.68932847821,-12.8930967028274,118.589711404264)) ;
#159679=CARTESIAN_POINT('Ctrl Pts',(-12.763132322778,-12.8930967101103,
118.565480366075)) ;
#159680=CARTESIAN_POINT('Ctrl Pts',(-12.8369361673461,-12.8930967173931,
118.541249327886)) ;
#159681=CARTESIAN_POINT('Ctrl Pts',(-12.8571083054371,-12.853340146518,
118.602690405592)) ;
#159682=CARTESIAN_POINT('Ctrl Pts',(-12.8772804435281,-12.8135835756429,
118.664131483297)) ;
#159683=CARTESIAN_POINT('Ctrl Pts',(-12.80347659896,-12.8135835683601,118.688362521486)) ;
#159684=CARTESIAN_POINT('Ctrl Pts',(-12.729672754392,-12.8135835610772,
118.712593559675)) ;
#159685=CARTESIAN_POINT('Ctrl Pts',(-12.709500616301,-12.8533401319523,
118.65115248197)) ;
#159686=CARTESIAN_POINT('Ctrl Pts',(-12.7564269379405,-13.1210491167834,
118.758518890216)) ;
#159687=CARTESIAN_POINT('Ctrl Pts',(-12.7336836205255,-13.1421721692445,
118.689246415035)) ;
#159688=CARTESIAN_POINT('Ctrl Pts',(-12.8074874639998,-13.1421721715333,
118.665015373515)) ;
#159689=CARTESIAN_POINT('Ctrl Pts',(-12.8812913074742,-13.1421721738222,
118.640784331994)) ;
#159690=CARTESIAN_POINT('Ctrl Pts',(-12.9040346248891,-13.121049121361,
118.710056807176)) ;
#159691=CARTESIAN_POINT('Ctrl Pts',(-12.926777942304,-13.0999260688999,
118.779329282357)) ;
#159692=CARTESIAN_POINT('Ctrl Pts',(-12.8529740988297,-13.0999260666111,
118.803560323877)) ;
#159693=CARTESIAN_POINT('Ctrl Pts',(-12.7791702553554,-13.0999260643223,
118.827791365398)) ;
#159694=CARTESIAN_POINT('Ctrl Pts',(-12.7564269379405,-13.1210491167834,
118.758518890216)) ;
#159695=CARTESIAN_POINT('Ctrl Pts',(-12.7797729830741,-13.40900770729,118.794199282391)) ;
#159696=CARTESIAN_POINT('Ctrl Pts',(-12.756098640465,-13.410054885097,118.722091054621)) ;
#159697=CARTESIAN_POINT('Ctrl Pts',(-12.8299024838005,-13.4100548838608,
118.697860012678)) ;
#159698=CARTESIAN_POINT('Ctrl Pts',(-12.903706327136,-13.4100548826247,
118.673628970735)) ;
#159699=CARTESIAN_POINT('Ctrl Pts',(-12.9273806697451,-13.4090077048177,
118.745737198505)) ;
#159700=CARTESIAN_POINT('Ctrl Pts',(-12.9510550123542,-13.4079605270107,
118.817845426275)) ;
#159701=CARTESIAN_POINT('Ctrl Pts',(-12.8772511690187,-13.4079605282469,
118.842076468218)) ;
#159702=CARTESIAN_POINT('Ctrl Pts',(-12.8034473256832,-13.407960529483,
118.866307510161)) ;
#159703=CARTESIAN_POINT('Ctrl Pts',(-12.7797729830741,-13.40900770729,118.794199282391)) ;
#159704=CARTESIAN_POINT('Ctrl Pts',(-12.7789054138412,-13.6972694862933,
118.756166722536)) ;
#159705=CARTESIAN_POINT('Ctrl Pts',(-12.7559888438116,-13.6781895282422,
118.686366547741)) ;
#159706=CARTESIAN_POINT('Ctrl Pts',(-12.8297926874375,-13.6781895252059,
118.662135506682)) ;
#159707=CARTESIAN_POINT('Ctrl Pts',(-12.9035965310634,-13.6781895221696,
118.637904465624)) ;
#159708=CARTESIAN_POINT('Ctrl Pts',(-12.926513101093,-13.6972694802207,
118.707704640419)) ;
#159709=CARTESIAN_POINT('Ctrl Pts',(-12.9494296711225,-13.7163494382719,
118.777504815214)) ;
#159710=CARTESIAN_POINT('Ctrl Pts',(-12.8756258274966,-13.7163494413082,
118.801735856273)) ;
#159711=CARTESIAN_POINT('Ctrl Pts',(-12.8018219838707,-13.7163494443445,
118.825966897331)) ;
#159712=CARTESIAN_POINT('Ctrl Pts',(-12.7789054138412,-13.6972694862933,
118.756166722536)) ;
#159713=CARTESIAN_POINT('Ctrl Pts',(-12.7545947470765,-13.9663054532962,
118.646647736907)) ;
#159714=CARTESIAN_POINT('Ctrl Pts',(-12.7340759482531,-13.9284104742122,
118.584150786325)) ;
#159715=CARTESIAN_POINT('Ctrl Pts',(-12.8078797922052,-13.9284104715145,
118.55991974626)) ;
#159716=CARTESIAN_POINT('Ctrl Pts',(-12.8816836361573,-13.9284104688168,
118.535688706195)) ;
#159717=CARTESIAN_POINT('Ctrl Pts',(-12.9022024349807,-13.9663054479008,
118.598185656777)) ;
#159718=CARTESIAN_POINT('Ctrl Pts',(-12.9227212338041,-14.0042004269848,
118.660682607359)) ;
#159719=CARTESIAN_POINT('Ctrl Pts',(-12.848917389852,-14.0042004296825,
118.684913647424)) ;
#159720=CARTESIAN_POINT('Ctrl Pts',(-12.7751135458999,-14.0042004323802,
118.709144687489)) ;
#159721=CARTESIAN_POINT('Ctrl Pts',(-12.7545947470765,-13.9663054532962,
118.646647736907)) ;
#159722=CARTESIAN_POINT('Ctrl Pts',(-12.708953623995,-14.1969043333081,
118.471990317947)) ;
#159723=CARTESIAN_POINT('Ctrl Pts',(-12.692329221625,-14.1428507400375,
118.421355070661)) ;
#159724=CARTESIAN_POINT('Ctrl Pts',(-12.7661330651514,-14.1428507401224,
118.3971240293)) ;
#159725=CARTESIAN_POINT('Ctrl Pts',(-12.8399369086778,-14.1428507402074,
118.372892987938)) ;
#159726=CARTESIAN_POINT('Ctrl Pts',(-12.8565613110478,-14.196904333478,
118.423528235223)) ;
#159727=CARTESIAN_POINT('Ctrl Pts',(-12.8731857134178,-14.2509579267487,
118.474163482509)) ;
#159728=CARTESIAN_POINT('Ctrl Pts',(-12.7993818698914,-14.2509579266637,
118.498394523871)) ;
#159729=CARTESIAN_POINT('Ctrl Pts',(-12.725578026365,-14.2509579265788,
118.522625565232)) ;
#159730=CARTESIAN_POINT('Ctrl Pts',(-12.708953623995,-14.1969043333081,
118.471990317947)) ;
#159731=CARTESIAN_POINT('Ctrl Pts',(-12.6467531532713,-14.3698914257013,
118.24719675644)) ;
#159732=CARTESIAN_POINT('Ctrl Pts',(-12.6351790212959,-14.3036801668695,
118.211943817991)) ;
#159733=CARTESIAN_POINT('Ctrl Pts',(-12.7089828637962,-14.3036801689092,
118.187712773504)) ;
#159734=CARTESIAN_POINT('Ctrl Pts',(-12.7827867062965,-14.303680170949,
118.163481729016)) ;
#159735=CARTESIAN_POINT('Ctrl Pts',(-12.7943608382718,-14.3698914297808,
118.198734667466)) ;
#159736=CARTESIAN_POINT('Ctrl Pts',(-12.8059349702472,-14.4361026886127,
118.233987605915)) ;
#159737=CARTESIAN_POINT('Ctrl Pts',(-12.7321311277469,-14.4361026865729,
118.258218650402)) ;
#159738=CARTESIAN_POINT('Ctrl Pts',(-12.6583272852466,-14.4361026845332,
118.282449694889)) ;
#159739=CARTESIAN_POINT('Ctrl Pts',(-12.6467531532713,-14.3698914257013,
118.24719675644)) ;
#159740=CARTESIAN_POINT('Ctrl Pts',(-12.5727418641631,-14.4755193866787,
117.986353001203)) ;
#159741=CARTESIAN_POINT('Ctrl Pts',(-12.5670515910477,-14.4018362726686,
117.969021347583)) ;
#159742=CARTESIAN_POINT('Ctrl Pts',(-12.6408554318707,-14.4018362752404,
117.944790297987)) ;
#159743=CARTESIAN_POINT('Ctrl Pts',(-12.7146592726937,-14.4018362778122,
117.920559248391)) ;
#159744=CARTESIAN_POINT('Ctrl Pts',(-12.7203495458091,-14.4755193918222,
117.937890902011)) ;
#159745=CARTESIAN_POINT('Ctrl Pts',(-12.7260398189245,-14.5492025058322,
117.955222555631)) ;
#159746=CARTESIAN_POINT('Ctrl Pts',(-12.6522359781016,-14.5492025032605,
117.979453605227)) ;
#159747=CARTESIAN_POINT('Ctrl Pts',(-12.5784321372786,-14.5492025006887,
118.003684654823)) ;
#159748=CARTESIAN_POINT('Ctrl Pts',(-12.5727418641631,-14.4755193866787,
117.986353001203)) ;
#159749=CARTESIAN_POINT('Ctrl Pts',(-12.4928027634597,-14.5054697818126,
117.707363787146)) ;
#159750=CARTESIAN_POINT('Ctrl Pts',(-12.4934206488961,-14.4295881889502,
117.709245766793)) ;
#159751=CARTESIAN_POINT('Ctrl Pts',(-12.5672244874137,-14.4295881891086,
117.685014710175)) ;
#159752=CARTESIAN_POINT('Ctrl Pts',(-12.6410283259312,-14.429588189267,
117.660783653557)) ;
#159753=CARTESIAN_POINT('Ctrl Pts',(-12.6404104404947,-14.5054697821294,
117.65890167391)) ;
#159754=CARTESIAN_POINT('Ctrl Pts',(-12.6397925550582,-14.5813513749918,
117.657019694263)) ;
#159755=CARTESIAN_POINT('Ctrl Pts',(-12.5659887165407,-14.5813513748333,
117.681250750881)) ;
#159756=CARTESIAN_POINT('Ctrl Pts',(-12.4921848780232,-14.5813513746749,
117.705481807498)) ;
#159757=CARTESIAN_POINT('Ctrl Pts',(-12.4928027634597,-14.5054697818126,
117.707363787146)) ;
#159758=CARTESIAN_POINT('Ctrl Pts',(-12.4137352350169,-14.4574393177702,
117.431077181479)) ;
#159759=CARTESIAN_POINT('Ctrl Pts',(-12.4206084727546,-14.384801335134,
117.452011955084)) ;
#159760=CARTESIAN_POINT('Ctrl Pts',(-12.4944123091801,-14.384801328945,
117.427780892094)) ;
#159761=CARTESIAN_POINT('Ctrl Pts',(-12.5682161456056,-14.384801322756,
117.403549829104)) ;
#159762=CARTESIAN_POINT('Ctrl Pts',(-12.5613429078678,-14.4574393053923,
117.382615055499)) ;
#159763=CARTESIAN_POINT('Ctrl Pts',(-12.5544696701301,-14.5300772880285,
117.361680281894)) ;
#159764=CARTESIAN_POINT('Ctrl Pts',(-12.4806658337047,-14.5300772942175,
117.385911344884)) ;
#159765=CARTESIAN_POINT('Ctrl Pts',(-12.4068619972792,-14.5300773004065,
117.410142407874)) ;
#159766=CARTESIAN_POINT('Ctrl Pts',(-12.4137352350169,-14.4574393177702,
117.431077181479)) ;
#159767=CARTESIAN_POINT('Ctrl Pts',(-12.3418324266654,-14.3349211938034,
117.176601530105)) ;
#159768=CARTESIAN_POINT('Ctrl Pts',(-12.3544699690229,-14.2707324518497,
117.215093445674)) ;
#159769=CARTESIAN_POINT('Ctrl Pts',(-12.4282738040413,-14.2707324355109,
117.190862378399)) ;
#159770=CARTESIAN_POINT('Ctrl Pts',(-12.5020776390596,-14.2707324191721,
117.166631311123)) ;
#159771=CARTESIAN_POINT('Ctrl Pts',(-12.4894400967021,-14.3349211611258,
117.128139395553)) ;
#159772=CARTESIAN_POINT('Ctrl Pts',(-12.4768025543446,-14.3991099030794,
117.089647479984)) ;
#159773=CARTESIAN_POINT('Ctrl Pts',(-12.4029987193263,-14.3991099194182,
117.11387854726)) ;
#159774=CARTESIAN_POINT('Ctrl Pts',(-12.3291948843079,-14.399109935757,
117.138109614536)) ;
#159775=CARTESIAN_POINT('Ctrl Pts',(-12.3418324266654,-14.3349211938034,
117.176601530105)) ;
#159776=CARTESIAN_POINT('Ctrl Pts',(-12.2830970975097,-14.1470800055845,
116.962290261975)) ;
#159777=CARTESIAN_POINT('Ctrl Pts',(-12.3005865815552,-14.0959137214437,
117.015560409224)) ;
#159778=CARTESIAN_POINT('Ctrl Pts',(-12.3743904165327,-14.0959136926008,
116.991329341823)) ;
#159779=CARTESIAN_POINT('Ctrl Pts',(-12.4481942515102,-14.095913663758,
116.967098274423)) ;
#159780=CARTESIAN_POINT('Ctrl Pts',(-12.4307047674647,-14.1470799478988,
116.913828127174)) ;
#159781=CARTESIAN_POINT('Ctrl Pts',(-12.4132152834192,-14.1982462320397,
116.860557979926)) ;
#159782=CARTESIAN_POINT('Ctrl Pts',(-12.3394114484417,-14.1982462608825,
116.884789047326)) ;
#159783=CARTESIAN_POINT('Ctrl Pts',(-12.2656076134642,-14.1982462897254,
116.909020114726)) ;
#159784=CARTESIAN_POINT('Ctrl Pts',(-12.2830970975097,-14.1470800055845,
116.962290261975)) ;
#159785=CARTESIAN_POINT('Ctrl Pts',(-12.2422554856577,-13.9065331674936,
116.80239048803)) ;
#159786=CARTESIAN_POINT('Ctrl Pts',(-12.2633564495242,-13.8720877275132,
116.866660620279)) ;
#159787=CARTESIAN_POINT('Ctrl Pts',(-12.3371602858923,-13.8720876844338,
116.842429557115)) ;
#159788=CARTESIAN_POINT('Ctrl Pts',(-12.4109641222604,-13.8720876413544,
116.81819849395)) ;
#159789=CARTESIAN_POINT('Ctrl Pts',(-12.3898631583939,-13.9065330813348,
116.753928361701)) ;
#159790=CARTESIAN_POINT('Ctrl Pts',(-12.3687621945274,-13.9409785213152,
116.689658229452)) ;
#159791=CARTESIAN_POINT('Ctrl Pts',(-12.2949583581593,-13.9409785643945,
116.713889292616)) ;
#159792=CARTESIAN_POINT('Ctrl Pts',(-12.2211545217912,-13.9409786074739,
116.738120355781)) ;
#159793=CARTESIAN_POINT('Ctrl Pts',(-12.2422554856577,-13.9065331674936,
116.80239048803)) ;
#159794=CARTESIAN_POINT('Ctrl Pts',(-12.2232261811748,-13.630738678715,
116.708912567899)) ;
#159795=CARTESIAN_POINT('Ctrl Pts',(-12.2464212316731,-13.6154990346672,
116.779560950327)) ;
#159796=CARTESIAN_POINT('Ctrl Pts',(-12.3202250713423,-13.6154989781254,
116.755329897217)) ;
#159797=CARTESIAN_POINT('Ctrl Pts',(-12.3940289110116,-13.6154989215836,
116.731098844107)) ;
#159798=CARTESIAN_POINT('Ctrl Pts',(-12.3708338605132,-13.6307385656315,
116.660450461679)) ;
#159799=CARTESIAN_POINT('Ctrl Pts',(-12.3476388100149,-13.6459782096793,
116.589802079252)) ;
#159800=CARTESIAN_POINT('Ctrl Pts',(-12.2738349703457,-13.6459782662211,
116.614033132362)) ;
#159801=CARTESIAN_POINT('Ctrl Pts',(-12.2000311306764,-13.6459783227629,
116.638264185472)) ;
#159802=CARTESIAN_POINT('Ctrl Pts',(-12.2232261811748,-13.630738678715,
116.708912567899)) ;
#159803=CARTESIAN_POINT('Ctrl Pts',(-12.2280126456687,-13.3408270196336,
116.688112612688)) ;
#159804=CARTESIAN_POINT('Ctrl Pts',(-12.2516390316777,-13.3458064636332,
116.760074773632)) ;
#159805=CARTESIAN_POINT('Ctrl Pts',(-12.3254428763228,-13.3458063983403,
116.735843735678)) ;
#159806=CARTESIAN_POINT('Ctrl Pts',(-12.3992467209678,-13.3458063330474,
116.711612697724)) ;
#159807=CARTESIAN_POINT('Ctrl Pts',(-12.3756203349588,-13.3408268890478,
116.639650536779)) ;
#159808=CARTESIAN_POINT('Ctrl Pts',(-12.3519939489498,-13.3358474450482,
116.567688375835)) ;
#159809=CARTESIAN_POINT('Ctrl Pts',(-12.2781901043047,-13.3358475103411,
116.591919413789)) ;
#159810=CARTESIAN_POINT('Ctrl Pts',(-12.2043862596596,-13.335847575634,
116.616150451744)) ;
#159811=CARTESIAN_POINT('Ctrl Pts',(-12.2280126456687,-13.3408270196336,
116.688112612688)) ;
#159812=CARTESIAN_POINT('Ctrl Pts',(-12.2570791816381,-13.0553492265632,
116.741127681574)) ;
#159813=CARTESIAN_POINT('Ctrl Pts',(-12.2794453818278,-13.0802672240232,
116.809251520007)) ;
#159814=CARTESIAN_POINT('Ctrl Pts',(-12.3532492327196,-13.0802671541192,
116.785020501079)) ;
#159815=CARTESIAN_POINT('Ctrl Pts',(-12.4270530836114,-13.0802670842153,
116.760789482151)) ;
#159816=CARTESIAN_POINT('Ctrl Pts',(-12.4046868834218,-13.0553490867554,
116.692665643718)) ;
#159817=CARTESIAN_POINT('Ctrl Pts',(-12.3823206832321,-13.0304310892955,
116.624541805285)) ;
#159818=CARTESIAN_POINT('Ctrl Pts',(-12.3085168323402,-13.0304311591994,
116.648772824213)) ;
#159819=CARTESIAN_POINT('Ctrl Pts',(-12.2347129814484,-13.0304312291033,
116.673003843141)) ;
#159820=CARTESIAN_POINT('Ctrl Pts',(-12.2570791816381,-13.0553492265632,
116.741127681574)) ;
#159821=CARTESIAN_POINT('Ctrl Pts',(-12.3090343418545,-12.7963986353394,
116.863927628217)) ;
#159822=CARTESIAN_POINT('Ctrl Pts',(-12.3285390631052,-12.8394319369363,
116.923335863641)) ;
#159823=CARTESIAN_POINT('Ctrl Pts',(-12.4023429208373,-12.8394318699613,
116.899104865548)) ;
#159824=CARTESIAN_POINT('Ctrl Pts',(-12.4761467785694,-12.8394318029862,
116.874873867454)) ;
#159825=CARTESIAN_POINT('Ctrl Pts',(-12.4566420573186,-12.7963985013893,
116.815465632031)) ;
#159826=CARTESIAN_POINT('Ctrl Pts',(-12.4371373360679,-12.7533651997924,
116.756057396607)) ;
#159827=CARTESIAN_POINT('Ctrl Pts',(-12.3633334783358,-12.7533652667675,
116.7802883947)) ;
#159828=CARTESIAN_POINT('Ctrl Pts',(-12.2895296206037,-12.7533653337425,
116.804519392794)) ;
#159829=CARTESIAN_POINT('Ctrl Pts',(-12.3090343418545,-12.7963986353394,
116.863927628217)) ;
#159830=CARTESIAN_POINT('Ctrl Pts',(-12.3809755753915,-12.581755675213,
117.047570548939)) ;
#159831=CARTESIAN_POINT('Ctrl Pts',(-12.3962200578774,-12.6398371824031,
117.094002784605)) ;
#159832=CARTESIAN_POINT('Ctrl Pts',(-12.4700239222921,-12.6398371256695,
117.069771806866)) ;
#159833=CARTESIAN_POINT('Ctrl Pts',(-12.5438277867068,-12.639837068936,
117.045540829126)) ;
#159834=CARTESIAN_POINT('Ctrl Pts',(-12.5285833042209,-12.581755561746,
116.999108593461)) ;
#159835=CARTESIAN_POINT('Ctrl Pts',(-12.5133388217349,-12.5236740545559,
116.952676357795)) ;
#159836=CARTESIAN_POINT('Ctrl Pts',(-12.4395349573202,-12.5236741112895,
116.976907335534)) ;
#159837=CARTESIAN_POINT('Ctrl Pts',(-12.3657310929056,-12.523674168023,
117.001138313273)) ;
#159838=CARTESIAN_POINT('Ctrl Pts',(-12.3809755753915,-12.581755675213,
117.047570548939)) ;
#159839=CARTESIAN_POINT('Ctrl Pts',(-12.4684134110327,-12.4271874700909,
117.278442488482)) ;
#159840=CARTESIAN_POINT('Ctrl Pts',(-12.478308991434,-12.4961449438695,
117.308582831552)) ;
#159841=CARTESIAN_POINT('Ctrl Pts',(-12.5521128614542,-12.4961449047111,
117.284351870886)) ;
#159842=CARTESIAN_POINT('Ctrl Pts',(-12.6259167314744,-12.4961448655528,
117.26012091022)) ;
#159843=CARTESIAN_POINT('Ctrl Pts',(-12.6160211510731,-12.4271873917741,
117.22998056715)) ;
#159844=CARTESIAN_POINT('Ctrl Pts',(-12.6061255706718,-12.3582299179955,
117.199840224079)) ;
#159845=CARTESIAN_POINT('Ctrl Pts',(-12.5323217006516,-12.3582299571538,
117.224071184745)) ;
#159846=CARTESIAN_POINT('Ctrl Pts',(-12.4585178306314,-12.3582299963122,
117.248302145411)) ;
#159847=CARTESIAN_POINT('Ctrl Pts',(-12.4684134110327,-12.4271874700909,
117.278442488482)) ;
#159848=CARTESIAN_POINT('Ctrl Pts',(-12.5658597005341,-12.3434882644401,
117.539803720469)) ;
#159849=CARTESIAN_POINT('Ctrl Pts',(-12.5696997847096,-12.4183899253302,
117.551499999181)) ;
#159850=CARTESIAN_POINT('Ctrl Pts',(-12.6435036585378,-12.4183899094731,
117.527269050114)) ;
#159851=CARTESIAN_POINT('Ctrl Pts',(-12.717307532366,-12.418389893616,117.503038101047)) ;
#159852=CARTESIAN_POINT('Ctrl Pts',(-12.7134674481905,-12.3434882327259,
117.491341822334)) ;
#159853=CARTESIAN_POINT('Ctrl Pts',(-12.709627364015,-12.2685865718357,
117.479645543622)) ;
#159854=CARTESIAN_POINT('Ctrl Pts',(-12.6358234901868,-12.2685865876929,
117.503876492689)) ;
#159855=CARTESIAN_POINT('Ctrl Pts',(-12.5620196163586,-12.26858660355,117.528107441756)) ;
#159856=CARTESIAN_POINT('Ctrl Pts',(-12.5658597005341,-12.3434882644401,
117.539803720469)) ;
#159857=CARTESIAN_POINT('Ctrl Pts',(-12.6672936908425,-12.3367187774922,
117.813250325772)) ;
#159858=CARTESIAN_POINT('Ctrl Pts',(-12.6647923438579,-12.412202858538,
117.805631628438)) ;
#159859=CARTESIAN_POINT('Ctrl Pts',(-12.7385962192158,-12.4122028696992,
117.781400684031)) ;
#159860=CARTESIAN_POINT('Ctrl Pts',(-12.8124000945738,-12.4122028808603,
117.757169739623)) ;
#159861=CARTESIAN_POINT('Ctrl Pts',(-12.8149014415584,-12.3367187998145,
117.764788436956)) ;
#159862=CARTESIAN_POINT('Ctrl Pts',(-12.8174027885431,-12.2612347187686,
117.772407134289)) ;
#159863=CARTESIAN_POINT('Ctrl Pts',(-12.7435989131851,-12.2612347076075,
117.796638078697)) ;
#159864=CARTESIAN_POINT('Ctrl Pts',(-12.6697950378272,-12.2612346964463,
117.820869023105)) ;
#159865=CARTESIAN_POINT('Ctrl Pts',(-12.6672936908425,-12.3367187774922,
117.813250325772)) ;
#159866=CARTESIAN_POINT('Ctrl Pts',(-12.765948884936,-12.4076100218016,
118.078256939231)) ;
#159867=CARTESIAN_POINT('Ctrl Pts',(-12.7572902976169,-12.478255694811,
118.051884281362)) ;
#159868=CARTESIAN_POINT('Ctrl Pts',(-12.8310941717384,-12.4782557339545,
118.027653333189)) ;
#159869=CARTESIAN_POINT('Ctrl Pts',(-12.90489804586,-12.4782557730979,118.003422385015)) ;
#159870=CARTESIAN_POINT('Ctrl Pts',(-12.9135566331791,-12.4076101000885,
118.029795042883)) ;
#159871=CARTESIAN_POINT('Ctrl Pts',(-12.9222152204983,-12.3369644270791,
118.056167700752)) ;
#159872=CARTESIAN_POINT('Ctrl Pts',(-12.8484113463767,-12.3369643879356,
118.080398648925)) ;
#159873=CARTESIAN_POINT('Ctrl Pts',(-12.7746074722552,-12.3369643487922,
118.104629597099)) ;
#159874=CARTESIAN_POINT('Ctrl Pts',(-12.765948884936,-12.4076100218016,
118.078256939231)) ;
#159875=CARTESIAN_POINT('Ctrl Pts',(-12.8553355026567,-12.5503272886106,
118.315139856333)) ;
#159876=CARTESIAN_POINT('Ctrl Pts',(-12.8411554877371,-12.6111127645847,
118.271949820905)) ;
#159877=CARTESIAN_POINT('Ctrl Pts',(-12.9149593579354,-12.6111128294537,
118.247718860782)) ;
#159878=CARTESIAN_POINT('Ctrl Pts',(-12.9887632281337,-12.6111128943226,
118.223487900658)) ;
#159879=CARTESIAN_POINT('Ctrl Pts',(-13.0029432430532,-12.5503274183485,
118.266677936086)) ;
#159880=CARTESIAN_POINT('Ctrl Pts',(-13.0171232579728,-12.4895419423743,
118.309867971514)) ;
#159881=CARTESIAN_POINT('Ctrl Pts',(-12.9433193877745,-12.4895418775054,
118.334098931637)) ;
#159882=CARTESIAN_POINT('Ctrl Pts',(-12.8695155175762,-12.4895418126364,
118.358329891761)) ;
#159883=CARTESIAN_POINT('Ctrl Pts',(-12.8553355026567,-12.5503272886106,
118.315139856333)) ;
#159884=CARTESIAN_POINT('Ctrl Pts',(-12.9304176070875,-12.7556871760659,
118.508319195545)) ;
#159885=CARTESIAN_POINT('Ctrl Pts',(-12.9117094172772,-12.8022252144536,
118.451337070035)) ;
#159886=CARTESIAN_POINT('Ctrl Pts',(-12.9855132812814,-12.8022253005655,
118.427106091045)) ;
#159887=CARTESIAN_POINT('Ctrl Pts',(-13.0593171452855,-12.8022253866775,
118.402875112056)) ;
#159888=CARTESIAN_POINT('Ctrl Pts',(-13.0780253350958,-12.7556873482899,
118.459857237566)) ;
#159889=CARTESIAN_POINT('Ctrl Pts',(-13.0967335249062,-12.7091493099022,
118.516839363076)) ;
#159890=CARTESIAN_POINT('Ctrl Pts',(-13.022929660902,-12.7091492237902,
118.541070342065)) ;
#159891=CARTESIAN_POINT('Ctrl Pts',(-12.9491257968979,-12.7091491376783,
118.565301321055)) ;
#159892=CARTESIAN_POINT('Ctrl Pts',(-12.9304176070875,-12.7556871760659,
118.508319195545)) ;
#159893=CARTESIAN_POINT('Ctrl Pts',(-12.9861723417227,-13.0091921750313,
118.642571963292)) ;
#159894=CARTESIAN_POINT('Ctrl Pts',(-12.964279676432,-13.038100701856,118.575890439269)) ;
#159895=CARTESIAN_POINT('Ctrl Pts',(-13.0380835324484,-13.03810080188,118.551659435951)) ;
#159896=CARTESIAN_POINT('Ctrl Pts',(-13.1118873884648,-13.038100901904,
118.527428432632)) ;
#159897=CARTESIAN_POINT('Ctrl Pts',(-13.1337800537556,-13.0091923750794,
118.594109956654)) ;
#159898=CARTESIAN_POINT('Ctrl Pts',(-13.1556727190464,-12.9802838482547,
118.660791480676)) ;
#159899=CARTESIAN_POINT('Ctrl Pts',(-13.08186886303,-12.9802837482307,118.685022483995)) ;
#159900=CARTESIAN_POINT('Ctrl Pts',(-13.0080650070135,-12.9802836482067,
118.709253487314)) ;
#159901=CARTESIAN_POINT('Ctrl Pts',(-12.9861723417227,-13.0091921750313,
118.642571963292)) ;
#159902=CARTESIAN_POINT('Ctrl Pts',(-13.0191734609878,-13.2902503547293,
118.707745845769)) ;
#159903=CARTESIAN_POINT('Ctrl Pts',(-12.9956755887425,-13.2995791016308,
118.636175120335)) ;
#159904=CARTESIAN_POINT('Ctrl Pts',(-13.0694794359814,-13.2995792074157,
118.611944090282)) ;
#159905=CARTESIAN_POINT('Ctrl Pts',(-13.1432832832204,-13.2995793132006,
118.587713060228)) ;
#159906=CARTESIAN_POINT('Ctrl Pts',(-13.1667811554657,-13.2902505662991,
118.659283785661)) ;
#159907=CARTESIAN_POINT('Ctrl Pts',(-13.190279027711,-13.2809218193976,
118.730854511095)) ;
#159908=CARTESIAN_POINT('Ctrl Pts',(-13.1164751804721,-13.2809217136127,
118.755085541148)) ;
#159909=CARTESIAN_POINT('Ctrl Pts',(-13.0426713332331,-13.2809216078278,
118.779316571202)) ;
#159910=CARTESIAN_POINT('Ctrl Pts',(-13.0191734609878,-13.2902503547293,
118.707745845769)) ;
#159911=CARTESIAN_POINT('Ctrl Pts',(-13.028209715569,-13.5823834440121,
118.699683255514)) ;
#159912=CARTESIAN_POINT('Ctrl Pts',(-13.0047821035049,-13.5713305139235,
118.628326531197)) ;
#159913=CARTESIAN_POINT('Ctrl Pts',(-13.0785859419211,-13.5713306161393,
118.604095474271)) ;
#159914=CARTESIAN_POINT('Ctrl Pts',(-13.1523897803373,-13.5713307183552,
118.579864417345)) ;
#159915=CARTESIAN_POINT('Ctrl Pts',(-13.1758173924015,-13.5823836484438,
118.651221141661)) ;
#159916=CARTESIAN_POINT('Ctrl Pts',(-13.1992450044656,-13.5934365785324,
118.722577865978)) ;
#159917=CARTESIAN_POINT('Ctrl Pts',(-13.1254411660494,-13.5934364763166,
118.746808922905)) ;
#159918=CARTESIAN_POINT('Ctrl Pts',(-13.0516373276332,-13.5934363741007,
118.771039979831)) ;
#159919=CARTESIAN_POINT('Ctrl Pts',(-13.028209715569,-13.5823834440121,
118.699683255514)) ;
#159920=CARTESIAN_POINT('Ctrl Pts',(-13.0130366717192,-13.8618181146796,
118.617988137292)) ;
#159921=CARTESIAN_POINT('Ctrl Pts',(-12.9913674586558,-13.8312391943693,
118.551987212537)) ;
#159922=CARTESIAN_POINT('Ctrl Pts',(-13.0651712893114,-13.8312392849538,
118.527756131973)) ;
#159923=CARTESIAN_POINT('Ctrl Pts',(-13.138975119967,-13.8312393755383,
118.503525051408)) ;
#159924=CARTESIAN_POINT('Ctrl Pts',(-13.1606443330303,-13.8618182958485,
118.569525976164)) ;
#159925=CARTESIAN_POINT('Ctrl Pts',(-13.1823135460937,-13.8923972161587,
118.635526900919)) ;
#159926=CARTESIAN_POINT('Ctrl Pts',(-13.1085097154381,-13.8923971255743,
118.659757981483)) ;
#159927=CARTESIAN_POINT('Ctrl Pts',(-13.0347058847825,-13.8923970349898,
118.683989062047)) ;
#159928=CARTESIAN_POINT('Ctrl Pts',(-13.0130366717192,-13.8618181146796,
118.617988137292)) ;
#159929=CARTESIAN_POINT('Ctrl Pts',(-12.9759659852745,-14.1083106024044,
118.469780251358)) ;
#159930=CARTESIAN_POINT('Ctrl Pts',(-12.957582964321,-14.0604763693046,
118.413788537469)) ;
#159931=CARTESIAN_POINT('Ctrl Pts',(-13.0313867887157,-14.0604764428427,
118.389557437835)) ;
#159932=CARTESIAN_POINT('Ctrl Pts',(-13.1051906131104,-14.0604765163808,
118.365326338202)) ;
#159933=CARTESIAN_POINT('Ctrl Pts',(-13.1235736340638,-14.1083107494807,
118.42131805209)) ;
#159934=CARTESIAN_POINT('Ctrl Pts',(-13.1419566550173,-14.1561449825805,
118.477309765979)) ;
#159935=CARTESIAN_POINT('Ctrl Pts',(-13.0681528306226,-14.1561449090424,
118.501540865613)) ;
#159936=CARTESIAN_POINT('Ctrl Pts',(-12.994349006228,-14.1561448355042,
118.525771965247)) ;
#159937=CARTESIAN_POINT('Ctrl Pts',(-12.9759659852745,-14.1083106024044,
118.469780251358)) ;
#159938=CARTESIAN_POINT('Ctrl Pts',(-12.9198792403032,-14.3070623418306,
118.263416505571)) ;
#159939=CARTESIAN_POINT('Ctrl Pts',(-12.906119592085,-14.2452796350311,
118.221506838939)) ;
#159940=CARTESIAN_POINT('Ctrl Pts',(-12.9799234125691,-14.2452796860699,
118.197275727394)) ;
#159941=CARTESIAN_POINT('Ctrl Pts',(-13.0537272330532,-14.2452797371086,
118.173044615849)) ;
#159942=CARTESIAN_POINT('Ctrl Pts',(-13.0674868812713,-14.3070624439081,
118.214954282482)) ;
#159943=CARTESIAN_POINT('Ctrl Pts',(-13.0812465294895,-14.3688451507076,
118.256863949114)) ;
#159944=CARTESIAN_POINT('Ctrl Pts',(-13.0074427090054,-14.3688450996689,
118.281095060659)) ;
#159945=CARTESIAN_POINT('Ctrl Pts',(-12.9336388885213,-14.3688450486301,
118.305326172203)) ;
#159946=CARTESIAN_POINT('Ctrl Pts',(-12.9198792403032,-14.3070623418306,
118.263416505571)) ;
#159947=CARTESIAN_POINT('Ctrl Pts',(-12.849560606782,-14.4418892785907,
118.013651989613)) ;
#159948=CARTESIAN_POINT('Ctrl Pts',(-12.8414260041814,-14.370599628049,
117.988875304187)) ;
#159949=CARTESIAN_POINT('Ctrl Pts',(-12.9152298234765,-14.3705996550827,
117.964644189021)) ;
#159950=CARTESIAN_POINT('Ctrl Pts',(-12.9890336427715,-14.3705996821164,
117.940413073854)) ;
#159951=CARTESIAN_POINT('Ctrl Pts',(-12.9971682453721,-14.4418893326581,
117.96518975928)) ;
#159952=CARTESIAN_POINT('Ctrl Pts',(-13.0053028479727,-14.5131789831999,
117.989966444705)) ;
#159953=CARTESIAN_POINT('Ctrl Pts',(-12.9314990286777,-14.5131789561661,
118.014197559872)) ;
#159954=CARTESIAN_POINT('Ctrl Pts',(-12.8576952093826,-14.5131789291324,
118.038428675038)) ;
#159955=CARTESIAN_POINT('Ctrl Pts',(-12.849560606782,-14.4418892785907,
118.013651989613)) ;
#159956=CARTESIAN_POINT('Ctrl Pts',(-12.7712938037721,-14.502692884587,
117.739819479159)) ;
#159957=CARTESIAN_POINT('Ctrl Pts',(-12.7693448921635,-14.4270502382033,
117.733883410297)) ;
#159958=CARTESIAN_POINT('Ctrl Pts',(-12.8431487123452,-14.4270502433144,
117.709652297831)) ;
#159959=CARTESIAN_POINT('Ctrl Pts',(-12.9169525325268,-14.4270502484255,
117.685421185365)) ;
#159960=CARTESIAN_POINT('Ctrl Pts',(-12.9189014441354,-14.5026928948091,
117.691357254227)) ;
#159961=CARTESIAN_POINT('Ctrl Pts',(-12.920850355744,-14.5783355411928,
117.697293323088)) ;
#159962=CARTESIAN_POINT('Ctrl Pts',(-12.8470465355624,-14.5783355360817,
117.721524435554)) ;
#159963=CARTESIAN_POINT('Ctrl Pts',(-12.7732427153807,-14.5783355309706,
117.74575554802)) ;
#159964=CARTESIAN_POINT('Ctrl Pts',(-12.7712938037721,-14.502692884587,
117.739819479159)) ;
#159965=CARTESIAN_POINT('Ctrl Pts',(-12.691443150556,-14.4862255258319,
117.461283982672)) ;
#159966=CARTESIAN_POINT('Ctrl Pts',(-12.6957973956779,-14.4116185668452,
117.474546312073)) ;
#159967=CARTESIAN_POINT('Ctrl Pts',(-12.7696012182988,-14.4116185533067,
117.450315207036)) ;
#159968=CARTESIAN_POINT('Ctrl Pts',(-12.8434050409197,-14.4116185397681,
117.426084102)) ;
#159969=CARTESIAN_POINT('Ctrl Pts',(-12.8390507957978,-14.4862254987549,
117.412821772599)) ;
#159970=CARTESIAN_POINT('Ctrl Pts',(-12.8346965506758,-14.5608324577416,
117.399559443198)) ;
#159971=CARTESIAN_POINT('Ctrl Pts',(-12.7608927280549,-14.5608324712802,
117.423790548234)) ;
#159972=CARTESIAN_POINT('Ctrl Pts',(-12.687088905434,-14.5608324848187,
117.448021653271)) ;
#159973=CARTESIAN_POINT('Ctrl Pts',(-12.691443150556,-14.4862255258319,
117.461283982672)) ;
#159974=CARTESIAN_POINT('Ctrl Pts',(-12.6158746315244,-14.3934141564473,
117.195652815533)) ;
#159975=CARTESIAN_POINT('Ctrl Pts',(-12.6262454854695,-14.3251742595679,
117.227240764473)) ;
#159976=CARTESIAN_POINT('Ctrl Pts',(-12.700049312281,-14.325174232371,117.203009672201)) ;
#159977=CARTESIAN_POINT('Ctrl Pts',(-12.7738531390925,-14.3251742051741,
117.178778579928)) ;
#159978=CARTESIAN_POINT('Ctrl Pts',(-12.7634822851474,-14.3934141020535,
117.147190630988)) ;
#159979=CARTESIAN_POINT('Ctrl Pts',(-12.7531114312024,-14.4616539989329,
117.115602682048)) ;
#159980=CARTESIAN_POINT('Ctrl Pts',(-12.6793076043909,-14.4616540261298,
117.139833774321)) ;
#159981=CARTESIAN_POINT('Ctrl Pts',(-12.6055037775794,-14.4616540533267,
117.164064866593)) ;
#159982=CARTESIAN_POINT('Ctrl Pts',(-12.6158746315244,-14.3934141564473,
117.195652815533)) ;
#159983=CARTESIAN_POINT('Ctrl Pts',(-12.5509163096876,-14.2302607448999,
116.962257398382)) ;
#159984=CARTESIAN_POINT('Ctrl Pts',(-12.5665738753727,-14.1733086335148,
117.009947818093)) ;
#159985=CARTESIAN_POINT('Ctrl Pts',(-12.6403777072618,-14.1733085993244,
116.985716741286)) ;
#159986=CARTESIAN_POINT('Ctrl Pts',(-12.7141815391508,-14.173308565134,
116.961485664479)) ;
#159987=CARTESIAN_POINT('Ctrl Pts',(-12.6985239734657,-14.2302606765191,
116.913795244768)) ;
#159988=CARTESIAN_POINT('Ctrl Pts',(-12.6828664077805,-14.2872127879042,
116.866104825057)) ;
#159989=CARTESIAN_POINT('Ctrl Pts',(-12.6090625758915,-14.2872128220946,
116.890335901864)) ;
#159990=CARTESIAN_POINT('Ctrl Pts',(-12.5352587440024,-14.287212856285,
116.914566978671)) ;
#159991=CARTESIAN_POINT('Ctrl Pts',(-12.5509163096876,-14.2302607448999,
116.962257398382)) ;
#159992=CARTESIAN_POINT('Ctrl Pts',(-12.5022332898898,-14.0081666908763,
116.778385267356)) ;
#159993=CARTESIAN_POINT('Ctrl Pts',(-12.5220503757503,-13.9666350467411,
116.838744914192)) ;
#159994=CARTESIAN_POINT('Ctrl Pts',(-12.5958542125087,-13.9666350124539,
116.814513852216)) ;
#159995=CARTESIAN_POINT('Ctrl Pts',(-12.6696580492672,-13.9666349781666,
116.790282790241)) ;
#159996=CARTESIAN_POINT('Ctrl Pts',(-12.6498409634067,-14.0081666223018,
116.729923143405)) ;
#159997=CARTESIAN_POINT('Ctrl Pts',(-12.6300238775463,-14.0496982664369,
116.669563496569)) ;
#159998=CARTESIAN_POINT('Ctrl Pts',(-12.5562200407878,-14.0496983007242,
116.693794558544)) ;
#159999=CARTESIAN_POINT('Ctrl Pts',(-12.4824162040293,-14.0496983350115,
116.71802562052)) ;
#160000=CARTESIAN_POINT('Ctrl Pts',(-12.5022332898898,-14.0081666908763,
116.778385267356)) ;
#160001=CARTESIAN_POINT('Ctrl Pts',(-12.4742506823548,-13.7466548362381,
116.657950049822)) ;
#160002=CARTESIAN_POINT('Ctrl Pts',(-12.4967799149851,-13.7233199580348,
116.726570457999)) ;
#160003=CARTESIAN_POINT('Ctrl Pts',(-12.5705837553633,-13.7233199251522,
116.702339407048)) ;
#160004=CARTESIAN_POINT('Ctrl Pts',(-12.6443875957415,-13.7233198922696,
116.678108356097)) ;
#160005=CARTESIAN_POINT('Ctrl Pts',(-12.6218583631112,-13.7466547704729,
116.609487947921)) ;
#160006=CARTESIAN_POINT('Ctrl Pts',(-12.5993291304809,-13.7699896486762,
116.540867539744)) ;
#160007=CARTESIAN_POINT('Ctrl Pts',(-12.5255252901027,-13.7699896815587,
116.565098590695)) ;
#160008=CARTESIAN_POINT('Ctrl Pts',(-12.4517214497245,-13.7699897144413,
116.589329641646)) ;
#160009=CARTESIAN_POINT('Ctrl Pts',(-12.4742506823548,-13.7466548362381,
116.657950049822)) ;
#160010=CARTESIAN_POINT('Ctrl Pts',(-12.4691100549571,-13.4587847124533,
116.606699386214)) ;
#160011=CARTESIAN_POINT('Ctrl Pts',(-12.4927690498238,-13.4555144548359,
116.678760867692)) ;
#160012=CARTESIAN_POINT('Ctrl Pts',(-12.5665728932212,-13.4555144300918,
116.654529825937)) ;
#160013=CARTESIAN_POINT('Ctrl Pts',(-12.6403767366186,-13.4555144053477,
116.630298784182)) ;
#160014=CARTESIAN_POINT('Ctrl Pts',(-12.6167177417518,-13.4587846629652,
116.558237302705)) ;
#160015=CARTESIAN_POINT('Ctrl Pts',(-12.5930587468851,-13.4620549205826,
116.486175821228)) ;
#160016=CARTESIAN_POINT('Ctrl Pts',(-12.5192549034877,-13.4620549453267,
116.510406862983)) ;
#160017=CARTESIAN_POINT('Ctrl Pts',(-12.4454510600903,-13.4620549700708,
116.534637904737)) ;
#160018=CARTESIAN_POINT('Ctrl Pts',(-12.4691100549571,-13.4587847124533,
116.606699386214)) ;
#160019=CARTESIAN_POINT('Ctrl Pts',(-12.4885192361608,-13.1685102080527,
116.630294437279)) ;
#160020=CARTESIAN_POINT('Ctrl Pts',(-12.5115939319546,-13.1855034690251,
116.700576237899)) ;
#160021=CARTESIAN_POINT('Ctrl Pts',(-12.5853977767225,-13.1855034529917,
116.676345200319)) ;
#160022=CARTESIAN_POINT('Ctrl Pts',(-12.6592016214903,-13.1855034369582,
116.652114162738)) ;
#160023=CARTESIAN_POINT('Ctrl Pts',(-12.6361269256965,-13.1685101759858,
116.581832362118)) ;
#160024=CARTESIAN_POINT('Ctrl Pts',(-12.6130522299027,-13.1515169150133,
116.511550561497)) ;
#160025=CARTESIAN_POINT('Ctrl Pts',(-12.5392483851348,-13.1515169310468,
116.535781599078)) ;
#160026=CARTESIAN_POINT('Ctrl Pts',(-12.465444540367,-13.1515169470802,
116.560012636658)) ;
#160027=CARTESIAN_POINT('Ctrl Pts',(-12.4885192361608,-13.1685102080527,
116.630294437279)) ;
#160028=CARTESIAN_POINT('Ctrl Pts',(-12.5312093541707,-12.8978336872395,
116.725034238603)) ;
#160029=CARTESIAN_POINT('Ctrl Pts',(-12.5520681509441,-12.9337522455578,
116.788566768234)) ;
#160030=CARTESIAN_POINT('Ctrl Pts',(-12.6258719961565,-12.9337522361366,
116.764335732008)) ;
#160031=CARTESIAN_POINT('Ctrl Pts',(-12.6996758413689,-12.9337522267154,
116.740104695781)) ;
#160032=CARTESIAN_POINT('Ctrl Pts',(-12.6788170445955,-12.897833668397,
116.67657216615)) ;
#160033=CARTESIAN_POINT('Ctrl Pts',(-12.657958247822,-12.8619151100786,
116.613039636519)) ;
#160034=CARTESIAN_POINT('Ctrl Pts',(-12.5841544026096,-12.8619151194999,
116.637270672746)) ;
#160035=CARTESIAN_POINT('Ctrl Pts',(-12.5103505573972,-12.8619151289211,
116.661501708972)) ;
#160036=CARTESIAN_POINT('Ctrl Pts',(-12.5312093541707,-12.8978336872395,
116.725034238603)) ;
#160037=CARTESIAN_POINT('Ctrl Pts',(-12.5957395733222,-12.6619537350285,
116.885954892402)) ;
#160038=CARTESIAN_POINT('Ctrl Pts',(-12.612861275193,-12.7143974709413,
116.938104833802)) ;
#160039=CARTESIAN_POINT('Ctrl Pts',(-12.6866651195987,-12.714397468419,
116.913873795118)) ;
#160040=CARTESIAN_POINT('Ctrl Pts',(-12.7604689640043,-12.7143974658967,
116.889642756435)) ;
#160041=CARTESIAN_POINT('Ctrl Pts',(-12.7433472621335,-12.6619537299839,
116.837492815035)) ;
#160042=CARTESIAN_POINT('Ctrl Pts',(-12.7262255602627,-12.6095099940711,
116.785342873635)) ;
#160043=CARTESIAN_POINT('Ctrl Pts',(-12.652421715857,-12.6095099965934,
116.809573912318)) ;
#160044=CARTESIAN_POINT('Ctrl Pts',(-12.5786178714514,-12.6095099991157,
116.833804951002)) ;
#160045=CARTESIAN_POINT('Ctrl Pts',(-12.5957395733222,-12.6619537350285,
116.885954892402)) ;
#160046=CARTESIAN_POINT('Ctrl Pts',(-12.6776143419512,-12.4816257056073,
117.099854766256)) ;
#160047=CARTESIAN_POINT('Ctrl Pts',(-12.6897787676254,-12.5467399887244,
117.136905644134)) ;
#160048=CARTESIAN_POINT('Ctrl Pts',(-12.7635826110348,-12.5467399890346,
117.112674602415)) ;
#160049=CARTESIAN_POINT('Ctrl Pts',(-12.8373864544442,-12.5467399893448,
117.088443560697)) ;
#160050=CARTESIAN_POINT('Ctrl Pts',(-12.8252220287701,-12.4816257062277,
117.051392682819)) ;
#160051=CARTESIAN_POINT('Ctrl Pts',(-12.8130576030959,-12.4165114231106,
117.014341804942)) ;
#160052=CARTESIAN_POINT('Ctrl Pts',(-12.7392537596865,-12.4165114228005,
117.03857284666)) ;
#160053=CARTESIAN_POINT('Ctrl Pts',(-12.6654499162771,-12.4165114224903,
117.062803888378)) ;
#160054=CARTESIAN_POINT('Ctrl Pts',(-12.6776143419512,-12.4816257056073,
117.099854766256)) ;
#160055=CARTESIAN_POINT('Ctrl Pts',(-12.7713529617644,-12.3684889471066,
117.350055385643)) ;
#160056=CARTESIAN_POINT('Ctrl Pts',(-12.7777208023874,-12.441600008621,
117.369450800684)) ;
#160057=CARTESIAN_POINT('Ctrl Pts',(-12.8515246450419,-12.441600009445,
117.345219756667)) ;
#160058=CARTESIAN_POINT('Ctrl Pts',(-12.9253284876963,-12.4416000102689,
117.320988712649)) ;
#160059=CARTESIAN_POINT('Ctrl Pts',(-12.9189606470733,-12.3684889487544,
117.301593297608)) ;
#160060=CARTESIAN_POINT('Ctrl Pts',(-12.9125928064503,-12.2953778872399,
117.282197882567)) ;
#160061=CARTESIAN_POINT('Ctrl Pts',(-12.8387889637959,-12.295377886416,
117.306428926584)) ;
#160062=CARTESIAN_POINT('Ctrl Pts',(-12.7649851211414,-12.2953778855921,
117.330659970602)) ;
#160063=CARTESIAN_POINT('Ctrl Pts',(-12.7713529617644,-12.3684889471066,
117.350055385643)) ;
#160064=CARTESIAN_POINT('Ctrl Pts',(-12.8723202400041,-12.3299903879882,
117.621972650026)) ;
#160065=CARTESIAN_POINT('Ctrl Pts',(-12.8723839341267,-12.4058988295515,
117.622166651981)) ;
#160066=CARTESIAN_POINT('Ctrl Pts',(-12.9461877764825,-12.4058988295036,
117.597935607054)) ;
#160067=CARTESIAN_POINT('Ctrl Pts',(-13.0199916188383,-12.4058988294557,
117.573704562126)) ;
#160068=CARTESIAN_POINT('Ctrl Pts',(-13.0199279247158,-12.3299903878923,
117.573510560171)) ;
#160069=CARTESIAN_POINT('Ctrl Pts',(-13.0198642305932,-12.254081946329,
117.573316558216)) ;
#160070=CARTESIAN_POINT('Ctrl Pts',(-12.9460603882374,-12.2540819463769,
117.597547603144)) ;
#160071=CARTESIAN_POINT('Ctrl Pts',(-12.8722565458816,-12.2540819464249,
117.621778648071)) ;
#160072=CARTESIAN_POINT('Ctrl Pts',(-12.8723202400041,-12.3299903879882,
117.621972650026)) ;
#160073=CARTESIAN_POINT('Ctrl Pts',(-12.9724385289638,-12.3696139932957,
117.891584408557)) ;
#160074=CARTESIAN_POINT('Ctrl Pts',(-12.9662425210927,-12.4428670872802,
117.872712368267)) ;
#160075=CARTESIAN_POINT('Ctrl Pts',(-13.040046363953,-12.4428670865975,
117.848481324877)) ;
#160076=CARTESIAN_POINT('Ctrl Pts',(-13.1138502068133,-12.4428670859149,
117.824250281486)) ;
#160077=CARTESIAN_POINT('Ctrl Pts',(-13.1200462146844,-12.3696139919303,
117.843122321775)) ;
#160078=CARTESIAN_POINT('Ctrl Pts',(-13.1262422225556,-12.2963608979458,
117.861994362065)) ;
#160079=CARTESIAN_POINT('Ctrl Pts',(-13.0524383796953,-12.2963608986285,
117.886225405455)) ;
#160080=CARTESIAN_POINT('Ctrl Pts',(-12.978634536835,-12.2963608993112,
117.910456448846)) ;
#160081=CARTESIAN_POINT('Ctrl Pts',(-12.9724385289638,-12.3696139932957,
117.891584408557)) ;
#160082=CARTESIAN_POINT('Ctrl Pts',(-13.0664515487238,-12.4839372794238,
118.142479880966)) ;
#160083=CARTESIAN_POINT('Ctrl Pts',(-13.0544155149314,-12.5493150647165,
118.105820064064)) ;
#160084=CARTESIAN_POINT('Ctrl Pts',(-13.1282193587287,-12.5493150649477,
118.081589023527)) ;
#160085=CARTESIAN_POINT('Ctrl Pts',(-13.2020232025261,-12.549315065179,
118.057357982991)) ;
#160086=CARTESIAN_POINT('Ctrl Pts',(-13.2140592363185,-12.4839372798862,
118.094017799893)) ;
#160087=CARTESIAN_POINT('Ctrl Pts',(-13.2260952701109,-12.4185594945934,
118.130677616795)) ;
#160088=CARTESIAN_POINT('Ctrl Pts',(-13.1522914263136,-12.4185594943622,
118.154908657331)) ;
#160089=CARTESIAN_POINT('Ctrl Pts',(-13.0784875825162,-12.418559494131,
118.179139697867)) ;
#160090=CARTESIAN_POINT('Ctrl Pts',(-13.0664515487238,-12.4839372794238,
118.142479880966)) ;
#160091=CARTESIAN_POINT('Ctrl Pts',(-13.1484405032608,-12.6667316342934,
118.356525775525)) ;
#160092=CARTESIAN_POINT('Ctrl Pts',(-13.1314001129427,-12.7194414647668,
118.304623496218)) ;
#160093=CARTESIAN_POINT('Ctrl Pts',(-13.2052039581057,-12.7194414698136,
118.280392459841)) ;
#160094=CARTESIAN_POINT('Ctrl Pts',(-13.2790078032687,-12.7194414748605,
118.256161423465)) ;
#160095=CARTESIAN_POINT('Ctrl Pts',(-13.2960481935868,-12.6667316443871,
118.308063702771)) ;
#160096=CARTESIAN_POINT('Ctrl Pts',(-13.3130885839048,-12.6140218139138,
118.359965982077)) ;
#160097=CARTESIAN_POINT('Ctrl Pts',(-13.2392847387418,-12.6140218088669,
118.384197018454)) ;
#160098=CARTESIAN_POINT('Ctrl Pts',(-13.1654808935788,-12.6140218038201,
118.408428054831)) ;
#160099=CARTESIAN_POINT('Ctrl Pts',(-13.1484405032608,-12.6667316342934,
118.356525775525)) ;
#160100=CARTESIAN_POINT('Ctrl Pts',(-13.2121850011556,-12.9020313562946,
118.515277498017)) ;
#160101=CARTESIAN_POINT('Ctrl Pts',(-13.191401639139,-12.9383882322268,
118.45197473096)) ;
#160102=CARTESIAN_POINT('Ctrl Pts',(-13.265205484716,-12.9383882439588,
118.427743695844)) ;
#160103=CARTESIAN_POINT('Ctrl Pts',(-13.3390093302929,-12.9383882556908,
118.403512660728)) ;
#160104=CARTESIAN_POINT('Ctrl Pts',(-13.3597926923095,-12.9020313797586,
118.466815427784)) ;
#160105=CARTESIAN_POINT('Ctrl Pts',(-13.3805760543261,-12.8656745038264,
118.530118194841)) ;
#160106=CARTESIAN_POINT('Ctrl Pts',(-13.3067722087492,-12.8656744920944,
118.554349229957)) ;
#160107=CARTESIAN_POINT('Ctrl Pts',(-13.2329683631722,-12.8656744803624,
118.578580265073)) ;
#160108=CARTESIAN_POINT('Ctrl Pts',(-13.2121850011556,-12.9020313562946,
118.515277498017)) ;
#160109=CARTESIAN_POINT('Ctrl Pts',(-13.2546371352095,-13.1740426154344,
118.609174623203)) ;
#160110=CARTESIAN_POINT('Ctrl Pts',(-13.2315922119599,-13.1914596717363,
118.538983505663)) ;
#160111=CARTESIAN_POINT('Ctrl Pts',(-13.3053960569823,-13.1914596914773,
118.514752468858)) ;
#160112=CARTESIAN_POINT('Ctrl Pts',(-13.3791999020048,-13.1914597112182,
118.490521432053)) ;
#160113=CARTESIAN_POINT('Ctrl Pts',(-13.4022448252544,-13.1740426549163,
118.560712549593)) ;
#160114=CARTESIAN_POINT('Ctrl Pts',(-13.4252897485041,-13.1566255986144,
118.630903667132)) ;
#160115=CARTESIAN_POINT('Ctrl Pts',(-13.3514859034817,-13.1566255788734,
118.655134703937)) ;
#160116=CARTESIAN_POINT('Ctrl Pts',(-13.2776820584592,-13.1566255591325,
118.679365740742)) ;
#160117=CARTESIAN_POINT('Ctrl Pts',(-13.2546371352095,-13.1740426154344,
118.609174623203)) ;
#160118=CARTESIAN_POINT('Ctrl Pts',(-13.2734900958146,-13.4634545824485,
118.631199247328)) ;
#160119=CARTESIAN_POINT('Ctrl Pts',(-13.2498280242855,-13.4606896668886,
118.559128395849)) ;
#160120=CARTESIAN_POINT('Ctrl Pts',(-13.3236318675582,-13.4606896946661,
118.534897353714)) ;
#160121=CARTESIAN_POINT('Ctrl Pts',(-13.3974357108309,-13.4606897224437,
118.51066631158)) ;
#160122=CARTESIAN_POINT('Ctrl Pts',(-13.42109778236,-13.4634546380036,118.58273716306)) ;
#160123=CARTESIAN_POINT('Ctrl Pts',(-13.4447598538892,-13.4662195535635,
118.654808014539)) ;
#160124=CARTESIAN_POINT('Ctrl Pts',(-13.3709560106164,-13.466219525786,
118.679039056674)) ;
#160125=CARTESIAN_POINT('Ctrl Pts',(-13.2971521673437,-13.4662194980085,
118.703270098808)) ;
#160126=CARTESIAN_POINT('Ctrl Pts',(-13.2734900958146,-13.4634545824485,
118.631199247328)) ;
#160127=CARTESIAN_POINT('Ctrl Pts',(-13.2680796257058,-13.7505708131454,
118.579201045788)) ;
#160128=CARTESIAN_POINT('Ctrl Pts',(-13.245496029926,-13.7277551955946,
118.510415057603)) ;
#160129=CARTESIAN_POINT('Ctrl Pts',(-13.3192998700676,-13.7277552307989,
118.486184005931)) ;
#160130=CARTESIAN_POINT('Ctrl Pts',(-13.3931037102092,-13.7277552660031,
118.46195295426)) ;
#160131=CARTESIAN_POINT('Ctrl Pts',(-13.415687305989,-13.7505708835539,
118.530738942446)) ;
#160132=CARTESIAN_POINT('Ctrl Pts',(-13.4382709017688,-13.7733865011047,
118.599524930632)) ;
#160133=CARTESIAN_POINT('Ctrl Pts',(-13.3644670616272,-13.7733864659004,
118.623755982303)) ;
#160134=CARTESIAN_POINT('Ctrl Pts',(-13.2906632214856,-13.7733864306961,
118.647987033974)) ;
#160135=CARTESIAN_POINT('Ctrl Pts',(-13.2680796257058,-13.7505708131454,
118.579201045788)) ;
#160136=CARTESIAN_POINT('Ctrl Pts',(-13.2394962360415,-14.0133363300327,
118.456684613439)) ;
#160137=CARTESIAN_POINT('Ctrl Pts',(-13.2196093760611,-13.9721415095329,
118.396112447548)) ;
#160138=CARTESIAN_POINT('Ctrl Pts',(-13.2934132119228,-13.9721415478717,
118.371881382841)) ;
#160139=CARTESIAN_POINT('Ctrl Pts',(-13.3672170477845,-13.9721415862106,
118.347650318134)) ;
#160140=CARTESIAN_POINT('Ctrl Pts',(-13.3871039077648,-14.0133364067105,
118.408222484025)) ;
#160141=CARTESIAN_POINT('Ctrl Pts',(-13.4069907677452,-14.0545312272103,
118.468794649916)) ;
#160142=CARTESIAN_POINT('Ctrl Pts',(-13.3331869318835,-14.0545311888715,
118.493025714623)) ;
#160143=CARTESIAN_POINT('Ctrl Pts',(-13.2593830960218,-14.0545311505326,
118.51725677933)) ;
#160144=CARTESIAN_POINT('Ctrl Pts',(-13.2394962360415,-14.0133363300327,
118.456684613439)) ;
#160145=CARTESIAN_POINT('Ctrl Pts',(-13.1905999974754,-14.2335678065818,
118.272293478368)) ;
#160146=CARTESIAN_POINT('Ctrl Pts',(-13.1748320592631,-14.1769371406859,
118.224266883765)) ;
#160147=CARTESIAN_POINT('Ctrl Pts',(-13.2486358902102,-14.1769371770333,
118.200035804088)) ;
#160148=CARTESIAN_POINT('Ctrl Pts',(-13.3224397211572,-14.1769372133807,
118.175804724412)) ;
#160149=CARTESIAN_POINT('Ctrl Pts',(-13.3382076593695,-14.2335678792767,
118.223831319015)) ;
#160150=CARTESIAN_POINT('Ctrl Pts',(-13.3539755975818,-14.2901985451726,
118.271857913619)) ;
#160151=CARTESIAN_POINT('Ctrl Pts',(-13.2801717666348,-14.2901985088252,
118.296088993295)) ;
#160152=CARTESIAN_POINT('Ctrl Pts',(-13.2063679356877,-14.2901984724778,
118.320320072971)) ;
#160153=CARTESIAN_POINT('Ctrl Pts',(-13.1905999974754,-14.2335678065818,
118.272293478368)) ;
#160154=CARTESIAN_POINT('Ctrl Pts',(-13.1253712311633,-14.3958087768564,
118.038043104771)) ;
#160155=CARTESIAN_POINT('Ctrl Pts',(-13.114870684948,-14.3277685970779,
118.006060136485)) ;
#160156=CARTESIAN_POINT('Ctrl Pts',(-13.1886745106335,-14.3277686257104,
117.981829040783)) ;
#160157=CARTESIAN_POINT('Ctrl Pts',(-13.2624783363189,-14.327768654343,
117.957597945081)) ;
#160158=CARTESIAN_POINT('Ctrl Pts',(-13.2729788825342,-14.3958088341215,
117.989580913366)) ;
#160159=CARTESIAN_POINT('Ctrl Pts',(-13.2834794287496,-14.4638490139001,
118.021563881652)) ;
#160160=CARTESIAN_POINT('Ctrl Pts',(-13.2096756030641,-14.4638489852675,
118.045794977354)) ;
#160161=CARTESIAN_POINT('Ctrl Pts',(-13.1358717773787,-14.463848956635,
118.070026073057)) ;
#160162=CARTESIAN_POINT('Ctrl Pts',(-13.1253712311633,-14.3958087768564,
118.038043104771)) ;
#160163=CARTESIAN_POINT('Ctrl Pts',(-13.0496091296525,-14.4872051600084,
117.771802663667)) ;
#160164=CARTESIAN_POINT('Ctrl Pts',(-13.0451171023842,-14.4126853477426,
117.758120674782)) ;
#160165=CARTESIAN_POINT('Ctrl Pts',(-13.1189209238047,-14.4126853615341,
117.73388956609)) ;
#160166=CARTESIAN_POINT('Ctrl Pts',(-13.1927247452252,-14.4126853753255,
117.709658457397)) ;
#160167=CARTESIAN_POINT('Ctrl Pts',(-13.1972167724935,-14.4872051875913,
117.723340446282)) ;
#160168=CARTESIAN_POINT('Ctrl Pts',(-13.2017087997618,-14.561724999857,
117.737022435167)) ;
#160169=CARTESIAN_POINT('Ctrl Pts',(-13.1279049783413,-14.5617249860656,
117.761253543859)) ;
#160170=CARTESIAN_POINT('Ctrl Pts',(-13.0541011569208,-14.5617249722742,
117.785484652552)) ;
#160171=CARTESIAN_POINT('Ctrl Pts',(-13.0496091296525,-14.4872051600084,
117.771802663667)) ;
#160172=CARTESIAN_POINT('Ctrl Pts',(-12.9697977471393,-14.5023836342265,
117.493417412762)) ;
#160173=CARTESIAN_POINT('Ctrl Pts',(-12.9716017236427,-14.4266966491582,
117.498912035629)) ;
#160174=CARTESIAN_POINT('Ctrl Pts',(-13.0454055427674,-14.4266966434283,
117.474680919943)) ;
#160175=CARTESIAN_POINT('Ctrl Pts',(-13.119209361892,-14.4266966376984,
117.450449804258)) ;
#160176=CARTESIAN_POINT('Ctrl Pts',(-13.1174053853887,-14.5023836227667,
117.444955181391)) ;
#160177=CARTESIAN_POINT('Ctrl Pts',(-13.1156014088854,-14.5780706078349,
117.439460558524)) ;
#160178=CARTESIAN_POINT('Ctrl Pts',(-13.0417975897607,-14.5780706135648,
117.463691674209)) ;
#160179=CARTESIAN_POINT('Ctrl Pts',(-12.967993770636,-14.5780706192947,
117.487922789895)) ;
#160180=CARTESIAN_POINT('Ctrl Pts',(-12.9697977471393,-14.5023836342265,
117.493417412762)) ;
#160181=CARTESIAN_POINT('Ctrl Pts',(-12.8911729784752,-14.4395233841403,
117.218279983479)) ;
#160182=CARTESIAN_POINT('Ctrl Pts',(-12.8992067287691,-14.3681145695168,
117.242749492307)) ;
#160183=CARTESIAN_POINT('Ctrl Pts',(-12.9730105467516,-14.3681145402781,
117.218518373143)) ;
#160184=CARTESIAN_POINT('Ctrl Pts',(-13.046814364734,-14.3681145110395,
117.194287253978)) ;
#160185=CARTESIAN_POINT('Ctrl Pts',(-13.0387806144401,-14.4395233256629,
117.16981774515)) ;
#160186=CARTESIAN_POINT('Ctrl Pts',(-13.0307468641462,-14.5109321402864,
117.145348236322)) ;
#160187=CARTESIAN_POINT('Ctrl Pts',(-12.9569430461637,-14.510932169525,
117.169579355486)) ;
#160188=CARTESIAN_POINT('Ctrl Pts',(-12.8831392281813,-14.5109321987637,
117.193810474651)) ;
#160189=CARTESIAN_POINT('Ctrl Pts',(-12.8911729784752,-14.4395233841403,
117.218279983479)) ;
#160190=CARTESIAN_POINT('Ctrl Pts',(-12.8215722521092,-14.3038981389521,
116.970926660863)) ;
#160191=CARTESIAN_POINT('Ctrl Pts',(-12.8352086467856,-14.2418546197311,
117.0124609206)) ;
#160192=CARTESIAN_POINT('Ctrl Pts',(-12.9090124667695,-14.2418545666607,
116.988229807532)) ;
#160193=CARTESIAN_POINT('Ctrl Pts',(-12.9828162867534,-14.2418545135903,
116.963998694464)) ;
#160194=CARTESIAN_POINT('Ctrl Pts',(-12.969179892077,-14.3038980328113,
116.922464434726)) ;
#160195=CARTESIAN_POINT('Ctrl Pts',(-12.9555434974006,-14.3659415520323,
116.880930174989)) ;
#160196=CARTESIAN_POINT('Ctrl Pts',(-12.8817396774167,-14.3659416051027,
116.905161288057)) ;
#160197=CARTESIAN_POINT('Ctrl Pts',(-12.8079358574328,-14.3659416581731,
116.929392401125)) ;
#160198=CARTESIAN_POINT('Ctrl Pts',(-12.8215722521092,-14.3038981389521,
116.970926660863)) ;
#160199=CARTESIAN_POINT('Ctrl Pts',(-12.765908924504,-14.1052991872385,
116.765996341192)) ;
#160200=CARTESIAN_POINT('Ctrl Pts',(-12.7841836185283,-14.057030828904,
116.821658112453)) ;
#160201=CARTESIAN_POINT('Ctrl Pts',(-12.8579874427366,-14.0570307540221,
116.797427012251)) ;
#160202=CARTESIAN_POINT('Ctrl Pts',(-12.9317912669448,-14.0570306791401,
116.77319591205)) ;
#160203=CARTESIAN_POINT('Ctrl Pts',(-12.9135165729205,-14.1052990374745,
116.717534140789)) ;
#160204=CARTESIAN_POINT('Ctrl Pts',(-12.8952418788962,-14.1535673958089,
116.661872369529)) ;
#160205=CARTESIAN_POINT('Ctrl Pts',(-12.821438054688,-14.1535674706909,
116.68610346973)) ;
#160206=CARTESIAN_POINT('Ctrl Pts',(-12.7476342304797,-14.1535675455729,
116.710334569932)) ;
#160207=CARTESIAN_POINT('Ctrl Pts',(-12.765908924504,-14.1052991872385,
116.765996341192)) ;
#160208=CARTESIAN_POINT('Ctrl Pts',(-12.7289194558588,-13.8563431079666,
116.617783489361)) ;
#160209=CARTESIAN_POINT('Ctrl Pts',(-12.7505389533844,-13.8253850611036,
116.683632992497)) ;
#160210=CARTESIAN_POINT('Ctrl Pts',(-12.8243427839167,-13.8253849680989,
116.659401911558)) ;
#160211=CARTESIAN_POINT('Ctrl Pts',(-12.8981466144491,-13.8253848750942,
116.635170830618)) ;
#160212=CARTESIAN_POINT('Ctrl Pts',(-12.8765271169234,-13.8563429219572,
116.569321327482)) ;
#160213=CARTESIAN_POINT('Ctrl Pts',(-12.8549076193978,-13.8873009688202,
116.503471824345)) ;
#160214=CARTESIAN_POINT('Ctrl Pts',(-12.7811037888655,-13.8873010618249,
116.527702905285)) ;
#160215=CARTESIAN_POINT('Ctrl Pts',(-12.7072999583332,-13.8873011548297,
116.551933986224)) ;
#160216=CARTESIAN_POINT('Ctrl Pts',(-12.7289194558588,-13.8563431079666,
116.617783489361)) ;
#160217=CARTESIAN_POINT('Ctrl Pts',(-12.7143046569284,-13.5768529523028,
116.537845772707)) ;
#160218=CARTESIAN_POINT('Ctrl Pts',(-12.7377091514829,-13.5653624857166,
116.609132088846)) ;
#160219=CARTESIAN_POINT('Ctrl Pts',(-12.8115129900551,-13.56536238196,116.584901032395)) ;
#160220=CARTESIAN_POINT('Ctrl Pts',(-12.8853168286273,-13.5653622782034,
116.560669975944)) ;
#160221=CARTESIAN_POINT('Ctrl Pts',(-12.8619123340728,-13.5768527447896,
116.489383659805)) ;
#160222=CARTESIAN_POINT('Ctrl Pts',(-12.8385078395183,-13.5883432113757,
116.418097343665)) ;
#160223=CARTESIAN_POINT('Ctrl Pts',(-12.7647040009461,-13.5883433151323,
116.442328400117)) ;
#160224=CARTESIAN_POINT('Ctrl Pts',(-12.6909001623739,-13.5883434188889,
116.466559456568)) ;
#160225=CARTESIAN_POINT('Ctrl Pts',(-12.7143046569284,-13.5768529523028,
116.537845772707)) ;
#160226=CARTESIAN_POINT('Ctrl Pts',(-12.7237017190187,-13.2855121533732,
116.530980294664)) ;
#160227=CARTESIAN_POINT('Ctrl Pts',(-12.7472188965232,-13.2943449974089,
116.602609824933)) ;
#160228=CARTESIAN_POINT('Ctrl Pts',(-12.8210227439731,-13.2943448909631,
116.578378795522)) ;
#160229=CARTESIAN_POINT('Ctrl Pts',(-12.894826591423,-13.2943447845173,
116.554147766111)) ;
#160230=CARTESIAN_POINT('Ctrl Pts',(-12.8713094139185,-13.2855119404815,
116.482518235842)) ;
#160231=CARTESIAN_POINT('Ctrl Pts',(-12.847792236414,-13.2766790964458,
116.410888705573)) ;
#160232=CARTESIAN_POINT('Ctrl Pts',(-12.7739883889641,-13.2766792028916,
116.435119734985)) ;
#160233=CARTESIAN_POINT('Ctrl Pts',(-12.7001845415141,-13.2766793093374,
116.459350764396)) ;
#160234=CARTESIAN_POINT('Ctrl Pts',(-12.7237017190187,-13.2855121533732,
116.530980294664)) ;
#160235=CARTESIAN_POINT('Ctrl Pts',(-12.7572168622974,-13.0041275578471,
116.597631042541)) ;
#160236=CARTESIAN_POINT('Ctrl Pts',(-12.7791619438715,-13.0326186796293,
116.664472222282)) ;
#160237=CARTESIAN_POINT('Ctrl Pts',(-12.8529658001272,-13.0326185795002,
116.640241219692)) ;
#160238=CARTESIAN_POINT('Ctrl Pts',(-12.9267696563828,-13.0326184793711,
116.616010217102)) ;
#160239=CARTESIAN_POINT('Ctrl Pts',(-12.9048245748087,-13.0041273575889,
116.54916903736)) ;
#160240=CARTESIAN_POINT('Ctrl Pts',(-12.8828794932346,-12.9756362358068,
116.482327857619)) ;
#160241=CARTESIAN_POINT('Ctrl Pts',(-12.809075636979,-12.9756363359359,
116.506558860209)) ;
#160242=CARTESIAN_POINT('Ctrl Pts',(-12.7352717807234,-12.975636436065,
116.5307898628)) ;
#160243=CARTESIAN_POINT('Ctrl Pts',(-12.7572168622974,-13.0041275578471,
116.597631042541)) ;
#160244=CARTESIAN_POINT('Ctrl Pts',(-12.8130794083186,-12.7524010633512,
116.732371814801)) ;
#160245=CARTESIAN_POINT('Ctrl Pts',(-12.8318894471127,-12.798508919761,
116.789664160074)) ;
#160246=CARTESIAN_POINT('Ctrl Pts',(-12.9056933112272,-12.798508834093,
116.765433181421)) ;
#160247=CARTESIAN_POINT('Ctrl Pts',(-12.9794971753417,-12.7985087484251,
116.741202202767)) ;
#160248=CARTESIAN_POINT('Ctrl Pts',(-12.9606871365476,-12.7524008920153,
116.683909857494)) ;
#160249=CARTESIAN_POINT('Ctrl Pts',(-12.9418770977535,-12.7062930356055,
116.626617512222)) ;
#160250=CARTESIAN_POINT('Ctrl Pts',(-12.868073233639,-12.7062931212734,
116.650848490875)) ;
#160251=CARTESIAN_POINT('Ctrl Pts',(-12.7942693695245,-12.7062932069414,
116.675079469529)) ;
#160252=CARTESIAN_POINT('Ctrl Pts',(-12.8130794083186,-12.7524010633512,
116.732371814801)) ;
#160253=CARTESIAN_POINT('Ctrl Pts',(-12.88854761512,-12.5474082659178,116.92665451824)) ;
#160254=CARTESIAN_POINT('Ctrl Pts',(-12.9028530268849,-12.6078966446447,
116.970226496376)) ;
#160255=CARTESIAN_POINT('Ctrl Pts',(-12.9766568970565,-12.6078965805878,
116.945995536171)) ;
#160256=CARTESIAN_POINT('Ctrl Pts',(-13.050460767228,-12.6078965165309,
116.921764575967)) ;
#160257=CARTESIAN_POINT('Ctrl Pts',(-13.036155355463,-12.5474081378039,
116.878192597831)) ;
#160258=CARTESIAN_POINT('Ctrl Pts',(-13.0218499436981,-12.4869197590769,
116.834620619695)) ;
#160259=CARTESIAN_POINT('Ctrl Pts',(-12.9480460735266,-12.4869198231338,
116.8588515799)) ;
#160260=CARTESIAN_POINT('Ctrl Pts',(-12.874242203355,-12.4869198871908,
116.883082540105)) ;
#160261=CARTESIAN_POINT('Ctrl Pts',(-12.88854761512,-12.5474082659178,116.92665451824)) ;
#160262=CARTESIAN_POINT('Ctrl Pts',(-12.9782123177536,-12.4057612857423,
117.164359360981)) ;
#160263=CARTESIAN_POINT('Ctrl Pts',(-12.9870113646885,-12.4762290506085,
117.191159840251)) ;
#160264=CARTESIAN_POINT('Ctrl Pts',(-13.0608152385725,-12.4762290124344,
117.166928891354)) ;
#160265=CARTESIAN_POINT('Ctrl Pts',(-13.1346191124565,-12.4762289742604,
117.142697942457)) ;
#160266=CARTESIAN_POINT('Ctrl Pts',(-13.1258200655216,-12.4057612093942,
117.115897463187)) ;
#160267=CARTESIAN_POINT('Ctrl Pts',(-13.1170210185867,-12.3352934445281,
117.089096983917)) ;
#160268=CARTESIAN_POINT('Ctrl Pts',(-13.0432171447027,-12.3352934827021,
117.113327932814)) ;
#160269=CARTESIAN_POINT('Ctrl Pts',(-12.9694132708188,-12.3352935208762,
117.137558881711)) ;
#160270=CARTESIAN_POINT('Ctrl Pts',(-12.9782123177536,-12.4057612857423,
117.164359360981)) ;
#160271=CARTESIAN_POINT('Ctrl Pts',(-13.0770064791105,-12.3361751661113,
117.429775138385)) ;
#160272=CARTESIAN_POINT('Ctrl Pts',(-13.0796556464204,-12.4116066467127,
117.43784407653)) ;
#160273=CARTESIAN_POINT('Ctrl Pts',(-13.1534595213048,-12.4116066363173,
117.41361313068)) ;
#160274=CARTESIAN_POINT('Ctrl Pts',(-13.2272633961891,-12.4116066259219,
117.38938218483)) ;
#160275=CARTESIAN_POINT('Ctrl Pts',(-13.2246142288792,-12.3361751453206,
117.381313246685)) ;
#160276=CARTESIAN_POINT('Ctrl Pts',(-13.2219650615692,-12.2607436647193,
117.37324430854)) ;
#160277=CARTESIAN_POINT('Ctrl Pts',(-13.1481611866849,-12.2607436751146,
117.39747525439)) ;
#160278=CARTESIAN_POINT('Ctrl Pts',(-13.0743573118005,-12.26074368551,117.42170620024)) ;
#160279=CARTESIAN_POINT('Ctrl Pts',(-13.0770064791105,-12.3361751661113,
117.429775138385)) ;
#160280=CARTESIAN_POINT('Ctrl Pts',(-13.1783190413846,-12.3442704255669,
117.702890794258)) ;
#160281=CARTESIAN_POINT('Ctrl Pts',(-13.1746326472494,-12.4192498359007,
117.691662634393)) ;
#160282=CARTESIAN_POINT('Ctrl Pts',(-13.2484365204859,-12.4192498519891,
117.667431683524)) ;
#160283=CARTESIAN_POINT('Ctrl Pts',(-13.3222403937224,-12.4192498680774,
117.643200732654)) ;
#160284=CARTESIAN_POINT('Ctrl Pts',(-13.3259267878576,-12.3442704577436,
117.654428892519)) ;
#160285=CARTESIAN_POINT('Ctrl Pts',(-13.3296131819927,-12.2692910474097,
117.665657052383)) ;
#160286=CARTESIAN_POINT('Ctrl Pts',(-13.2558093087563,-12.2692910313214,
117.689888003252)) ;
#160287=CARTESIAN_POINT('Ctrl Pts',(-13.1820054355198,-12.269291015233,
117.714118954122)) ;
#160288=CARTESIAN_POINT('Ctrl Pts',(-13.1783190413846,-12.3442704255669,
117.702890794258)) ;
#160289=CARTESIAN_POINT('Ctrl Pts',(-13.2756527267231,-12.4291570429794,
117.963909021848)) ;
#160290=CARTESIAN_POINT('Ctrl Pts',(-13.2658985708581,-12.4983225025168,
117.934199438683)) ;
#160291=CARTESIAN_POINT('Ctrl Pts',(-13.3397024401949,-12.4983225412537,
117.909968475935)) ;
#160292=CARTESIAN_POINT('Ctrl Pts',(-13.4135063095318,-12.4983225799905,
117.885737513188)) ;
#160293=CARTESIAN_POINT('Ctrl Pts',(-13.4232604653967,-12.429157120453,
117.915447096353)) ;
#160294=CARTESIAN_POINT('Ctrl Pts',(-13.4330146212616,-12.3599916609156,
117.945156679518)) ;
#160295=CARTESIAN_POINT('Ctrl Pts',(-13.3592107519248,-12.3599916221787,
117.969387642266)) ;
#160296=CARTESIAN_POINT('Ctrl Pts',(-13.285406882588,-12.3599915834419,
117.993618605013)) ;
#160297=CARTESIAN_POINT('Ctrl Pts',(-13.2756527267231,-12.4291570429794,
117.963909021848)) ;
#160298=CARTESIAN_POINT('Ctrl Pts',(-13.36292678935,-12.5849331529663,118.194259899517)) ;
#160299=CARTESIAN_POINT('Ctrl Pts',(-13.3477985856065,-12.6433268351206,
118.148181833491)) ;
#160300=CARTESIAN_POINT('Ctrl Pts',(-13.4216024492848,-12.6433268905322,
118.123950853509)) ;
#160301=CARTESIAN_POINT('Ctrl Pts',(-13.495406312963,-12.6433269459438,
118.099719873526)) ;
#160302=CARTESIAN_POINT('Ctrl Pts',(-13.5105345167065,-12.5849332637895,
118.145797939552)) ;
#160303=CARTESIAN_POINT('Ctrl Pts',(-13.52566272045,-12.5265395816352,118.191876005578)) ;
#160304=CARTESIAN_POINT('Ctrl Pts',(-13.4518588567717,-12.5265395262236,
118.21610698556)) ;
#160305=CARTESIAN_POINT('Ctrl Pts',(-13.3780549930935,-12.526539470812,
118.240337965542)) ;
#160306=CARTESIAN_POINT('Ctrl Pts',(-13.36292678935,-12.5849331529663,118.194259899517)) ;
#160307=CARTESIAN_POINT('Ctrl Pts',(-13.4345794652228,-12.8005108515807,
118.377018028647)) ;
#160308=CARTESIAN_POINT('Ctrl Pts',(-13.4151599387072,-12.8439413739947,
118.317869285721)) ;
#160309=CARTESIAN_POINT('Ctrl Pts',(-13.4889637957772,-12.8439414387627,
118.293638285611)) ;
#160310=CARTESIAN_POINT('Ctrl Pts',(-13.5627676528473,-12.8439415035308,
118.269407285501)) ;
#160311=CARTESIAN_POINT('Ctrl Pts',(-13.5821871793629,-12.8005109811168,
118.328556028427)) ;
#160312=CARTESIAN_POINT('Ctrl Pts',(-13.6016067058785,-12.7570804587029,
118.387704771354)) ;
#160313=CARTESIAN_POINT('Ctrl Pts',(-13.5278028488085,-12.7570803939349,
118.411935771464)) ;
#160314=CARTESIAN_POINT('Ctrl Pts',(-13.4539989917384,-12.7570803291668,
118.436166771574)) ;
#160315=CARTESIAN_POINT('Ctrl Pts',(-13.4345794652228,-12.8005108515807,
118.377018028647)) ;
#160316=CARTESIAN_POINT('Ctrl Pts',(-13.4861674949149,-13.060269126664,
118.498676029101)) ;
#160317=CARTESIAN_POINT('Ctrl Pts',(-13.4638507023729,-13.0856291470037,
118.43070268118)) ;
#160318=CARTESIAN_POINT('Ctrl Pts',(-13.537654552795,-13.0856292137402,
118.406471660822)) ;
#160319=CARTESIAN_POINT('Ctrl Pts',(-13.6114584032172,-13.0856292804768,
118.382240640464)) ;
#160320=CARTESIAN_POINT('Ctrl Pts',(-13.6337751957592,-13.0602692601371,
118.450213988385)) ;
#160321=CARTESIAN_POINT('Ctrl Pts',(-13.6560919883012,-13.0349092397974,
118.518187336306)) ;
#160322=CARTESIAN_POINT('Ctrl Pts',(-13.582288137879,-13.0349091730608,
118.542418356664)) ;
#160323=CARTESIAN_POINT('Ctrl Pts',(-13.5084842874569,-13.0349091063243,
118.566649377022)) ;
#160324=CARTESIAN_POINT('Ctrl Pts',(-13.4861674949149,-13.060269126664,
118.498676029101)) ;
#160325=CARTESIAN_POINT('Ctrl Pts',(-13.5147933718825,-13.3453693583979,
118.550429429881)) ;
#160326=CARTESIAN_POINT('Ctrl Pts',(-13.4911774012882,-13.3508620232142,
118.478498995081)) ;
#160327=CARTESIAN_POINT('Ctrl Pts',(-13.5649812457546,-13.3508620856039,
118.454267956582)) ;
#160328=CARTESIAN_POINT('Ctrl Pts',(-13.638785090221,-13.3508621479936,
118.430036918084)) ;
#160329=CARTESIAN_POINT('Ctrl Pts',(-13.6624010608153,-13.3453694831773,
118.501967352883)) ;
#160330=CARTESIAN_POINT('Ctrl Pts',(-13.6860170314095,-13.3398768183609,
118.573897787683)) ;
#160331=CARTESIAN_POINT('Ctrl Pts',(-13.6122131869431,-13.3398767559712,
118.598128826182)) ;
#160332=CARTESIAN_POINT('Ctrl Pts',(-13.5384093424767,-13.3398766935815,
118.62235986468)) ;
#160333=CARTESIAN_POINT('Ctrl Pts',(-13.5147933718825,-13.3453693583979,
118.550429429881)) ;
#160334=CARTESIAN_POINT('Ctrl Pts',(-13.5191703640909,-13.6361640667827,
118.528261672456)) ;
#160335=CARTESIAN_POINT('Ctrl Pts',(-13.4959475223528,-13.6213614987656,
118.457528644549)) ;
#160336=CARTESIAN_POINT('Ctrl Pts',(-13.5697513621746,-13.6213615511211,
118.433297591904)) ;
#160337=CARTESIAN_POINT('Ctrl Pts',(-13.6435552019965,-13.6213616034766,
118.409066539259)) ;
#160338=CARTESIAN_POINT('Ctrl Pts',(-13.6667780437346,-13.6361641714938,
118.479799567165)) ;
#160339=CARTESIAN_POINT('Ctrl Pts',(-13.6900008854728,-13.6509667395109,
118.550532595072)) ;
#160340=CARTESIAN_POINT('Ctrl Pts',(-13.6161970456509,-13.6509666871554,
118.574763647717)) ;
#160341=CARTESIAN_POINT('Ctrl Pts',(-13.542393205829,-13.6509666347999,
118.598994700362)) ;
#160342=CARTESIAN_POINT('Ctrl Pts',(-13.5191703640909,-13.6361640667827,
118.528261672456)) ;
#160343=CARTESIAN_POINT('Ctrl Pts',(-13.4997846887976,-13.9104324089111,
118.433833737107)) ;
#160344=CARTESIAN_POINT('Ctrl Pts',(-13.478612399891,-13.8764575771015,
118.369346362117)) ;
#160345=CARTESIAN_POINT('Ctrl Pts',(-13.5524162366454,-13.8764576175232,
118.345115300128)) ;
#160346=CARTESIAN_POINT('Ctrl Pts',(-13.6262200733997,-13.8764576579448,
118.32088423814)) ;
#160347=CARTESIAN_POINT('Ctrl Pts',(-13.6473923623063,-13.9104324897545,
118.38537161313)) ;
#160348=CARTESIAN_POINT('Ctrl Pts',(-13.6685646512129,-13.9444073215641,
118.44985898812)) ;
#160349=CARTESIAN_POINT('Ctrl Pts',(-13.5947608144585,-13.9444072811424,
118.474090050108)) ;
#160350=CARTESIAN_POINT('Ctrl Pts',(-13.5209569777042,-13.9444072407208,
118.498321112097)) ;
#160351=CARTESIAN_POINT('Ctrl Pts',(-13.4997846887976,-13.9104324089111,
118.433833737107)) ;
#160352=CARTESIAN_POINT('Ctrl Pts',(-13.4587413574297,-14.1501784561149,
118.27335686083)) ;
#160353=CARTESIAN_POINT('Ctrl Pts',(-13.4411365754914,-14.0994124816197,
118.219735536282)) ;
#160354=CARTESIAN_POINT('Ctrl Pts',(-13.5149404109386,-14.0994125084155,
118.195504470312)) ;
#160355=CARTESIAN_POINT('Ctrl Pts',(-13.5887442463858,-14.0994125352114,
118.171273404342)) ;
#160356=CARTESIAN_POINT('Ctrl Pts',(-13.6063490283242,-14.1501785097066,
118.22489472889)) ;
#160357=CARTESIAN_POINT('Ctrl Pts',(-13.6239538102625,-14.2009444842018,
118.278516053439)) ;
#160358=CARTESIAN_POINT('Ctrl Pts',(-13.5501499748153,-14.200944457406,
118.302747119408)) ;
#160359=CARTESIAN_POINT('Ctrl Pts',(-13.4763461393681,-14.2009444306102,
118.326978185378)) ;
#160360=CARTESIAN_POINT('Ctrl Pts',(-13.4587413574297,-14.1501784561149,
118.27335686083)) ;
#160361=CARTESIAN_POINT('Ctrl Pts',(-13.39950930923,-14.3377944456025,118.057390334685)) ;
#160362=CARTESIAN_POINT('Ctrl Pts',(-13.3867493283457,-14.273851283079,
118.018525492262)) ;
#160363=CARTESIAN_POINT('Ctrl Pts',(-13.4605531643258,-14.2738512972119,
117.994294427915)) ;
#160364=CARTESIAN_POINT('Ctrl Pts',(-13.5343570003059,-14.2738513113447,
117.970063363569)) ;
#160365=CARTESIAN_POINT('Ctrl Pts',(-13.5471169811902,-14.3377944738682,
118.008928205992)) ;
#160366=CARTESIAN_POINT('Ctrl Pts',(-13.5598769620745,-14.4017376363917,
118.047793048415)) ;
#160367=CARTESIAN_POINT('Ctrl Pts',(-13.4860731260944,-14.4017376222589,
118.072024112762)) ;
#160368=CARTESIAN_POINT('Ctrl Pts',(-13.4122692901143,-14.4017376081261,
118.096255177108)) ;
#160369=CARTESIAN_POINT('Ctrl Pts',(-13.39950930923,-14.3377944456025,118.057390334685)) ;
#160370=CARTESIAN_POINT('Ctrl Pts',(-13.32749153125,-14.4588735568458,117.802602901111)) ;
#160371=CARTESIAN_POINT('Ctrl Pts',(-13.3204740636633,-14.3863794182977,
117.781228827494)) ;
#160372=CARTESIAN_POINT('Ctrl Pts',(-13.3942779010377,-14.3863794234914,
117.756997767394)) ;
#160373=CARTESIAN_POINT('Ctrl Pts',(-13.468081738412,-14.3863794286851,
117.732766707294)) ;
#160374=CARTESIAN_POINT('Ctrl Pts',(-13.4750992059987,-14.4588735672332,
117.754140780912)) ;
#160375=CARTESIAN_POINT('Ctrl Pts',(-13.4821166735854,-14.5313677057812,
117.775514854529)) ;
#160376=CARTESIAN_POINT('Ctrl Pts',(-13.408312836211,-14.5313677005875,
117.799745914629)) ;
#160377=CARTESIAN_POINT('Ctrl Pts',(-13.3345089988367,-14.5313676953939,
117.823976974729)) ;
#160378=CARTESIAN_POINT('Ctrl Pts',(-13.32749153125,-14.4588735568458,117.802602901111)) ;
#160379=CARTESIAN_POINT('Ctrl Pts',(-13.2483458924945,-14.5056122473976,
117.526071610546)) ;
#160380=CARTESIAN_POINT('Ctrl Pts',(-13.2475781043464,-14.4297450127553,
117.523733051975)) ;
#160381=CARTESIAN_POINT('Ctrl Pts',(-13.3213819437732,-14.4297450124761,
117.499501998127)) ;
#160382=CARTESIAN_POINT('Ctrl Pts',(-13.3951857832,-14.4297450121969,117.475270944278)) ;
#160383=CARTESIAN_POINT('Ctrl Pts',(-13.3959535713481,-14.5056122468393,
117.477609502849)) ;
#160384=CARTESIAN_POINT('Ctrl Pts',(-13.3967213594963,-14.5814794814817,
117.479948061419)) ;
#160385=CARTESIAN_POINT('Ctrl Pts',(-13.3229175200695,-14.5814794817608,
117.504179115268)) ;
#160386=CARTESIAN_POINT('Ctrl Pts',(-13.2491136806427,-14.58147948204,117.528410169116)) ;
#160387=CARTESIAN_POINT('Ctrl Pts',(-13.2483458924945,-14.5056122473976,
117.526071610546)) ;
#160388=CARTESIAN_POINT('Ctrl Pts',(-13.1685437749415,-14.4743736272664,
117.247539732196)) ;
#160389=CARTESIAN_POINT('Ctrl Pts',(-13.1740810712629,-14.4005733067483,
117.264405443477)) ;
#160390=CARTESIAN_POINT('Ctrl Pts',(-13.2478849127416,-14.4005733047048,
117.240174395878)) ;
#160391=CARTESIAN_POINT('Ctrl Pts',(-13.3216887542203,-14.4005733026613,
117.21594334828)) ;
#160392=CARTESIAN_POINT('Ctrl Pts',(-13.3161514578989,-14.4743736231794,
117.199077636998)) ;
#160393=CARTESIAN_POINT('Ctrl Pts',(-13.3106141615776,-14.5481739436975,
117.182211925717)) ;
#160394=CARTESIAN_POINT('Ctrl Pts',(-13.2368103200988,-14.548173945741,
117.206442973316)) ;
#160395=CARTESIAN_POINT('Ctrl Pts',(-13.1630064786201,-14.5481739477846,
117.230674020914)) ;
#160396=CARTESIAN_POINT('Ctrl Pts',(-13.1685437749415,-14.4743736272664,
117.247539732196)) ;
#160397=CARTESIAN_POINT('Ctrl Pts',(-13.0946020226361,-14.3676054099568,
116.986884001878)) ;
#160398=CARTESIAN_POINT('Ctrl Pts',(-13.1060441801812,-14.3011495694392,
117.021734967606)) ;
#160399=CARTESIAN_POINT('Ctrl Pts',(-13.1798480232085,-14.3011495683314,
116.997503924724)) ;
#160400=CARTESIAN_POINT('Ctrl Pts',(-13.2536518662359,-14.3011495672236,
116.973272881842)) ;
#160401=CARTESIAN_POINT('Ctrl Pts',(-13.2422097086908,-14.3676054077411,
116.938421916114)) ;
#160402=CARTESIAN_POINT('Ctrl Pts',(-13.2307675511457,-14.4340612482587,
116.903570950386)) ;
#160403=CARTESIAN_POINT('Ctrl Pts',(-13.1569637081184,-14.4340612493665,
116.927801993268)) ;
#160404=CARTESIAN_POINT('Ctrl Pts',(-13.0831598650911,-14.4340612504743,
116.95203303615)) ;
#160405=CARTESIAN_POINT('Ctrl Pts',(-13.0946020226361,-14.3676054099568,
116.986884001878)) ;
#160406=CARTESIAN_POINT('Ctrl Pts',(-13.0324910029511,-14.1926642104704,
116.762231273457)) ;
#160407=CARTESIAN_POINT('Ctrl Pts',(-13.0490214672177,-14.1383247775165,
116.812580400398)) ;
#160408=CARTESIAN_POINT('Ctrl Pts',(-13.1228253110723,-14.1383247785838,
116.788349360036)) ;
#160409=CARTESIAN_POINT('Ctrl Pts',(-13.1966291549269,-14.1383247796511,
116.764118319674)) ;
#160410=CARTESIAN_POINT('Ctrl Pts',(-13.1800986906603,-14.192664212605,
116.713769192732)) ;
#160411=CARTESIAN_POINT('Ctrl Pts',(-13.1635682263937,-14.2470036455589,
116.663420065791)) ;
#160412=CARTESIAN_POINT('Ctrl Pts',(-13.0897643825391,-14.2470036444916,
116.687651106153)) ;
#160413=CARTESIAN_POINT('Ctrl Pts',(-13.0159605386845,-14.2470036434243,
116.711882146515)) ;
#160414=CARTESIAN_POINT('Ctrl Pts',(-13.0324910029511,-14.1926642104704,
116.762231273457)) ;
#160415=CARTESIAN_POINT('Ctrl Pts',(-12.9874746142067,-13.9629645552833,
116.589736773677)) ;
#160416=CARTESIAN_POINT('Ctrl Pts',(-13.0079052715445,-13.9245838600997,
116.651965259386)) ;
#160417=CARTESIAN_POINT('Ctrl Pts',(-13.0817091155005,-13.9245838630912,
116.627734219333)) ;
#160418=CARTESIAN_POINT('Ctrl Pts',(-13.1555129594564,-13.9245838660827,
116.603503179279)) ;
#160419=CARTESIAN_POINT('Ctrl Pts',(-13.1350823021187,-13.9629645612662,
116.54127469357)) ;
#160420=CARTESIAN_POINT('Ctrl Pts',(-13.1146516447809,-14.0013452564497,
116.47904620786)) ;
#160421=CARTESIAN_POINT('Ctrl Pts',(-13.040847800825,-14.0013452534583,
116.503277247914)) ;
#160422=CARTESIAN_POINT('Ctrl Pts',(-12.967043956869,-14.0013452504668,
116.527508287967)) ;
#160423=CARTESIAN_POINT('Ctrl Pts',(-12.9874746142067,-13.9629645552833,
116.589736773677)) ;
#160424=CARTESIAN_POINT('Ctrl Pts',(-12.9633562559811,-13.6916669453695,
116.48056065792)) ;
#160425=CARTESIAN_POINT('Ctrl Pts',(-12.9862407299605,-13.6721744570857,
116.55026307322)) ;
#160426=CARTESIAN_POINT('Ctrl Pts',(-13.0600445735023,-13.6721744593942,
116.526032031905)) ;
#160427=CARTESIAN_POINT('Ctrl Pts',(-13.1338484170441,-13.6721744617026,
116.50180099059)) ;
#160428=CARTESIAN_POINT('Ctrl Pts',(-13.1109639430647,-13.6916669499864,
116.43209857529)) ;
#160429=CARTESIAN_POINT('Ctrl Pts',(-13.0880794690853,-13.7111594382702,
116.36239615999)) ;
#160430=CARTESIAN_POINT('Ctrl Pts',(-13.0142756255436,-13.7111594359618,
116.386627201305)) ;
#160431=CARTESIAN_POINT('Ctrl Pts',(-12.9404717820018,-13.7111594336534,
116.41085824262)) ;
#160432=CARTESIAN_POINT('Ctrl Pts',(-12.9633562559811,-13.6916669453695,
116.48056065792)) ;
#160433=CARTESIAN_POINT('Ctrl Pts',(-12.9629691653421,-13.4042886281479,
116.444129256868)) ;
#160434=CARTESIAN_POINT('Ctrl Pts',(-12.9866435826147,-13.4048339669214,
116.516237712028)) ;
#160435=CARTESIAN_POINT('Ctrl Pts',(-13.0604474259364,-13.4048339668837,
116.492006670043)) ;
#160436=CARTESIAN_POINT('Ctrl Pts',(-13.1342512692581,-13.404833966846,
116.467775628057)) ;
#160437=CARTESIAN_POINT('Ctrl Pts',(-13.1105768519855,-13.4042886280725,
116.395667172897)) ;
#160438=CARTESIAN_POINT('Ctrl Pts',(-13.0869024347129,-13.403743289299,
116.323558717737)) ;
#160439=CARTESIAN_POINT('Ctrl Pts',(-13.0130985913912,-13.4037432893367,
116.347789759722)) ;
#160440=CARTESIAN_POINT('Ctrl Pts',(-12.9392947480694,-13.4037432893744,
116.372020801708)) ;
#160441=CARTESIAN_POINT('Ctrl Pts',(-12.9629691653421,-13.4042886281479,
116.444129256868)) ;
#160442=CARTESIAN_POINT('Ctrl Pts',(-12.9867239596031,-13.1160881842174,
116.481000353099)) ;
#160443=CARTESIAN_POINT('Ctrl Pts',(-13.0095086248234,-13.1367582104912,
116.550398767152)) ;
#160444=CARTESIAN_POINT('Ctrl Pts',(-13.08331246846,-13.1367582061789,116.526167726126)) ;
#160445=CARTESIAN_POINT('Ctrl Pts',(-13.1571163120967,-13.1367582018666,
116.5019366851)) ;
#160446=CARTESIAN_POINT('Ctrl Pts',(-13.1343316468764,-13.1160881755929,
116.432538271047)) ;
#160447=CARTESIAN_POINT('Ctrl Pts',(-13.1115469816561,-13.0954181493191,
116.363139856994)) ;
#160448=CARTESIAN_POINT('Ctrl Pts',(-13.0377431380194,-13.0954181536314,
116.38737089802)) ;
#160449=CARTESIAN_POINT('Ctrl Pts',(-12.9639392943828,-13.0954181579436,
116.411601939046)) ;
#160450=CARTESIAN_POINT('Ctrl Pts',(-12.9867239596031,-13.1160881842174,
116.481000353099)) ;
#160451=CARTESIAN_POINT('Ctrl Pts',(-13.0339690435015,-12.8495738757798,
116.589413701142)) ;
#160452=CARTESIAN_POINT('Ctrl Pts',(-13.0542224194139,-12.8888833461409,
116.651102216502)) ;
#160453=CARTESIAN_POINT('Ctrl Pts',(-13.1280262643834,-12.8888833370438,
116.626871179536)) ;
#160454=CARTESIAN_POINT('Ctrl Pts',(-13.2018301093529,-12.8888833279467,
116.602640142569)) ;
#160455=CARTESIAN_POINT('Ctrl Pts',(-13.1815767334405,-12.8495738575856,
116.540951627209)) ;
#160456=CARTESIAN_POINT('Ctrl Pts',(-13.1613233575281,-12.8102643872246,
116.479263111849)) ;
#160457=CARTESIAN_POINT('Ctrl Pts',(-13.0875195125586,-12.8102643963217,
116.503494148816)) ;
#160458=CARTESIAN_POINT('Ctrl Pts',(-13.0137156675891,-12.8102644054188,
116.527725185782)) ;
#160459=CARTESIAN_POINT('Ctrl Pts',(-13.0339690435015,-12.8495738757798,
116.589413701142)) ;
#160460=CARTESIAN_POINT('Ctrl Pts',(-13.1016362988514,-12.6242652876755,
116.76014561289)) ;
#160461=CARTESIAN_POINT('Ctrl Pts',(-13.1179262753709,-12.6793633695142,
116.809762253308)) ;
#160462=CARTESIAN_POINT('Ctrl Pts',(-13.1917301223629,-12.6793633576824,
116.785531222502)) ;
#160463=CARTESIAN_POINT('Ctrl Pts',(-13.2655339693549,-12.6793633458506,
116.761300191696)) ;
#160464=CARTESIAN_POINT('Ctrl Pts',(-13.2492439928354,-12.6242652640119,
116.711683551278)) ;
#160465=CARTESIAN_POINT('Ctrl Pts',(-13.2329540163159,-12.5691671821732,
116.66206691086)) ;
#160466=CARTESIAN_POINT('Ctrl Pts',(-13.1591501693239,-12.569167194005,
116.686297941666)) ;
#160467=CARTESIAN_POINT('Ctrl Pts',(-13.0853463223319,-12.5691672058369,
116.710528972472)) ;
#160468=CARTESIAN_POINT('Ctrl Pts',(-13.1016362988514,-12.6242652876755,
116.76014561289)) ;
#160469=CARTESIAN_POINT('Ctrl Pts',(-13.1868381515301,-12.4543477917217,
116.98391806025)) ;
#160470=CARTESIAN_POINT('Ctrl Pts',(-13.1979423963532,-12.5213905408383,
117.017739798833)) ;
#160471=CARTESIAN_POINT('Ctrl Pts',(-13.2717462470113,-12.5213905278412,
116.993508779193)) ;
#160472=CARTESIAN_POINT('Ctrl Pts',(-13.3455500976693,-12.521390514844,
116.969277759554)) ;
#160473=CARTESIAN_POINT('Ctrl Pts',(-13.3344458528461,-12.4543477657274,
116.93545602097)) ;
#160474=CARTESIAN_POINT('Ctrl Pts',(-13.323341608023,-12.3873050166108,
116.901634282387)) ;
#160475=CARTESIAN_POINT('Ctrl Pts',(-13.2495377573649,-12.387305029608,
116.925865302027)) ;
#160476=CARTESIAN_POINT('Ctrl Pts',(-13.1757339067069,-12.3873050426051,
116.950096321667)) ;
#160477=CARTESIAN_POINT('Ctrl Pts',(-13.1868381515301,-12.4543477917217,
116.98391806025)) ;
#160478=CARTESIAN_POINT('Ctrl Pts',(-13.282130994495,-12.3553371823295,
117.238917231087)) ;
#160479=CARTESIAN_POINT('Ctrl Pts',(-13.2873271899244,-12.4293892510952,
117.254744004599)) ;
#160480=CARTESIAN_POINT('Ctrl Pts',(-13.3611310433399,-12.4293892433542,
117.230512993358)) ;
#160481=CARTESIAN_POINT('Ctrl Pts',(-13.4349348967555,-12.4293892356132,
117.206281982117)) ;
#160482=CARTESIAN_POINT('Ctrl Pts',(-13.4297387013261,-12.3553371668475,
117.190455208605)) ;
#160483=CARTESIAN_POINT('Ctrl Pts',(-13.4245425058967,-12.2812850980819,
117.174628435093)) ;
#160484=CARTESIAN_POINT('Ctrl Pts',(-13.3507386524812,-12.2812851058229,
117.198859446334)) ;
#160485=CARTESIAN_POINT('Ctrl Pts',(-13.2769347990657,-12.2812851135639,
117.223090457575)) ;
#160486=CARTESIAN_POINT('Ctrl Pts',(-13.282130994495,-12.3553371823295,
117.238917231087)) ;
#160487=CARTESIAN_POINT('Ctrl Pts',(-13.3835527278556,-12.3315537600446,
117.512226746283)) ;
#160488=CARTESIAN_POINT('Ctrl Pts',(-13.3824119200247,-12.4073738615737,
117.508752030529)) ;
#160489=CARTESIAN_POINT('Ctrl Pts',(-13.456215776812,-12.4073738630853,
117.484521029558)) ;
#160490=CARTESIAN_POINT('Ctrl Pts',(-13.5300196335994,-12.4073738645969,
117.460290028587)) ;
#160491=CARTESIAN_POINT('Ctrl Pts',(-13.5311604414304,-12.3315537630678,
117.463764744342)) ;
#160492=CARTESIAN_POINT('Ctrl Pts',(-13.5323012492613,-12.2557336615386,
117.467239460096)) ;
#160493=CARTESIAN_POINT('Ctrl Pts',(-13.4584973924739,-12.255733660027,
117.491470461067)) ;
#160494=CARTESIAN_POINT('Ctrl Pts',(-13.3846935356866,-12.2557336585155,
117.515701462038)) ;
#160495=CARTESIAN_POINT('Ctrl Pts',(-13.3835527278556,-12.3315537600446,
117.512226746283)) ;
#160496=CARTESIAN_POINT('Ctrl Pts',(-13.4828912406925,-12.3856473127391,
117.779479511165)) ;
#160497=CARTESIAN_POINT('Ctrl Pts',(-13.4755438357451,-12.4577997306566,
117.757100502165)) ;
#160498=CARTESIAN_POINT('Ctrl Pts',(-13.549347694077,-12.4577997458788,
117.732869505898)) ;
#160499=CARTESIAN_POINT('Ctrl Pts',(-13.6231515524089,-12.457799761101,
117.708638509632)) ;
#160500=CARTESIAN_POINT('Ctrl Pts',(-13.6304989573563,-12.3856473431835,
117.731017518632)) ;
#160501=CARTESIAN_POINT('Ctrl Pts',(-13.6378463623037,-12.3134949252661,
117.753396527632)) ;
#160502=CARTESIAN_POINT('Ctrl Pts',(-13.5640425039718,-12.3134949100439,
117.777627523899)) ;
#160503=CARTESIAN_POINT('Ctrl Pts',(-13.4902386456399,-12.3134948948217,
117.801858520165)) ;
#160504=CARTESIAN_POINT('Ctrl Pts',(-13.4828912406925,-12.3856473127391,
117.779479511165)) ;
#160505=CARTESIAN_POINT('Ctrl Pts',(-13.5751280064643,-12.513656004823,
118.024906933845)) ;
#160506=CARTESIAN_POINT('Ctrl Pts',(-13.5620649402894,-12.5769754722421,
117.98511894314)) ;
#160507=CARTESIAN_POINT('Ctrl Pts',(-13.6358687992258,-12.5769755044901,
117.960887948714)) ;
#160508=CARTESIAN_POINT('Ctrl Pts',(-13.7096726581622,-12.576975536738,
117.936656954289)) ;
#160509=CARTESIAN_POINT('Ctrl Pts',(-13.7227357243371,-12.5136560693188,
117.976444944994)) ;
#160510=CARTESIAN_POINT('Ctrl Pts',(-13.7357987905121,-12.4503366018996,
118.016232935699)) ;
#160511=CARTESIAN_POINT('Ctrl Pts',(-13.6619949315757,-12.4503365696517,
118.040463930124)) ;
#160512=CARTESIAN_POINT('Ctrl Pts',(-13.5881910726393,-12.4503365374038,
118.06469492455)) ;
#160513=CARTESIAN_POINT('Ctrl Pts',(-13.5751280064643,-12.513656004823,
118.024906933845)) ;
#160514=CARTESIAN_POINT('Ctrl Pts',(-13.6539134068514,-12.707439556573,
118.229281918463)) ;
#160515=CARTESIAN_POINT('Ctrl Pts',(-13.6360672125102,-12.7573213774984,
118.174925291302)) ;
#160516=CARTESIAN_POINT('Ctrl Pts',(-13.7098710700878,-12.7573214291752,
118.150694292738)) ;
#160517=CARTESIAN_POINT('Ctrl Pts',(-13.7836749276654,-12.7573214808521,
118.126463294174)) ;
#160518=CARTESIAN_POINT('Ctrl Pts',(-13.8015211220067,-12.7074396599266,
118.180819921335)) ;
#160519=CARTESIAN_POINT('Ctrl Pts',(-13.8193673163479,-12.6575578390012,
118.235176548496)) ;
#160520=CARTESIAN_POINT('Ctrl Pts',(-13.7455634587703,-12.6575577873243,
118.25940754706)) ;
#160521=CARTESIAN_POINT('Ctrl Pts',(-13.6717596011927,-12.6575577356475,
118.283638545624)) ;
#160522=CARTESIAN_POINT('Ctrl Pts',(-13.6539134068514,-12.707439556573,
118.229281918463)) ;
#160523=CARTESIAN_POINT('Ctrl Pts',(-13.7137234776106,-12.9500051005904,
118.376179984501)) ;
#160524=CARTESIAN_POINT('Ctrl Pts',(-13.6924056592633,-12.9830234168188,
118.31124935088)) ;
#160525=CARTESIAN_POINT('Ctrl Pts',(-13.7662095128799,-12.9830234842415,
118.287018340252)) ;
#160526=CARTESIAN_POINT('Ctrl Pts',(-13.8400133664964,-12.9830235516642,
118.262787329623)) ;
#160527=CARTESIAN_POINT('Ctrl Pts',(-13.8613311848437,-12.9500052354358,
118.327717963243)) ;
#160528=CARTESIAN_POINT('Ctrl Pts',(-13.8826490031911,-12.9169869192073,
118.392648596863)) ;
#160529=CARTESIAN_POINT('Ctrl Pts',(-13.8088451495745,-12.9169868517846,
118.416879607492)) ;
#160530=CARTESIAN_POINT('Ctrl Pts',(-13.735041295958,-12.9169867843619,
118.441110618121)) ;
#160531=CARTESIAN_POINT('Ctrl Pts',(-13.7137234776106,-12.9500051005904,
118.376179984501)) ;
#160532=CARTESIAN_POINT('Ctrl Pts',(-13.7520689708624,-13.2274462581565,
118.457479335507)) ;
#160533=CARTESIAN_POINT('Ctrl Pts',(-13.7287774968662,-13.2411424706592,
118.386537265376)) ;
#160534=CARTESIAN_POINT('Ctrl Pts',(-13.8025813449987,-13.2411425518727,
118.362306238044)) ;
#160535=CARTESIAN_POINT('Ctrl Pts',(-13.8763851931311,-13.2411426330862,
118.338075210711)) ;
#160536=CARTESIAN_POINT('Ctrl Pts',(-13.8996766671273,-13.2274464205834,
118.409017280842)) ;
#160537=CARTESIAN_POINT('Ctrl Pts',(-13.9229681411235,-13.2137502080807,
118.479959350972)) ;
#160538=CARTESIAN_POINT('Ctrl Pts',(-13.8491642929911,-13.2137501268672,
118.504190378305)) ;
#160539=CARTESIAN_POINT('Ctrl Pts',(-13.7753604448586,-13.2137500456537,
118.528421405637)) ;
#160540=CARTESIAN_POINT('Ctrl Pts',(-13.7520689708624,-13.2274462581565,
118.457479335507)) ;
#160541=CARTESIAN_POINT('Ctrl Pts',(-13.7663393260749,-13.5192262317475,
118.465377287378)) ;
#160542=CARTESIAN_POINT('Ctrl Pts',(-13.7427535201405,-13.5125713400262,
118.393538729794)) ;
#160543=CARTESIAN_POINT('Ctrl Pts',(-13.8165573610894,-13.5125714295465,
118.369307680582)) ;
#160544=CARTESIAN_POINT('Ctrl Pts',(-13.8903612020383,-13.5125715190667,
118.34507663137)) ;
#160545=CARTESIAN_POINT('Ctrl Pts',(-13.9139470079727,-13.519226410788,
118.416915188953)) ;
#160546=CARTESIAN_POINT('Ctrl Pts',(-13.9375328139072,-13.5258813025093,
118.488753746537)) ;
#160547=CARTESIAN_POINT('Ctrl Pts',(-13.8637289729583,-13.525881212989,
118.512984795749)) ;
#160548=CARTESIAN_POINT('Ctrl Pts',(-13.7899251320094,-13.5258811234688,
118.537215844962)) ;
#160549=CARTESIAN_POINT('Ctrl Pts',(-13.7663393260749,-13.5192262317475,
118.465377287378)) ;
#160550=CARTESIAN_POINT('Ctrl Pts',(-13.7564573176797,-13.8018769048648,
118.399949096535)) ;
#160551=CARTESIAN_POINT('Ctrl Pts',(-13.7342582218036,-13.7754786172954,
118.332334234138)) ;
#160552=CARTESIAN_POINT('Ctrl Pts',(-13.8080620549042,-13.7754787060709,
118.308103161021)) ;
#160553=CARTESIAN_POINT('Ctrl Pts',(-13.8818658880047,-13.7754787948464,
118.283872087904)) ;
#160554=CARTESIAN_POINT('Ctrl Pts',(-13.9040649838808,-13.8018770824157,
118.351486950301)) ;
#160555=CARTESIAN_POINT('Ctrl Pts',(-13.9262640797569,-13.8282753699851,
118.419101812698)) ;
#160556=CARTESIAN_POINT('Ctrl Pts',(-13.8524602466564,-13.8282752812096,
118.443332885815)) ;
#160557=CARTESIAN_POINT('Ctrl Pts',(-13.7786564135558,-13.8282751924341,
118.467563958932)) ;
#160558=CARTESIAN_POINT('Ctrl Pts',(-13.7564573176797,-13.8018769048648,
118.399949096535)) ;
#160559=CARTESIAN_POINT('Ctrl Pts',(-13.7237468055255,-14.058784271986,
118.264759363062)) ;
#160560=CARTESIAN_POINT('Ctrl Pts',(-13.7045346643817,-14.0144111213973,
118.20624228294)) ;
#160561=CARTESIAN_POINT('Ctrl Pts',(-13.7783384894998,-14.0144112025132,
118.18201118551)) ;
#160562=CARTESIAN_POINT('Ctrl Pts',(-13.8521423146179,-14.014411283629,
118.157780088079)) ;
#160563=CARTESIAN_POINT('Ctrl Pts',(-13.8713544557617,-14.0587844342176,
118.216297168201)) ;
#160564=CARTESIAN_POINT('Ctrl Pts',(-13.8905665969056,-14.1031575848063,
118.274814248324)) ;
#160565=CARTESIAN_POINT('Ctrl Pts',(-13.8167627717875,-14.1031575036904,
118.299045345754)) ;
#160566=CARTESIAN_POINT('Ctrl Pts',(-13.7429589466694,-14.1031574225746,
118.323276443184)) ;
#160567=CARTESIAN_POINT('Ctrl Pts',(-13.7237468055255,-14.058784271986,
118.264759363062)) ;
#160568=CARTESIAN_POINT('Ctrl Pts',(-13.6714025576082,-14.2690401451517,
118.069862285334)) ;
#160569=CARTESIAN_POINT('Ctrl Pts',(-13.6565505498238,-14.2099227100526,
118.024625467992)) ;
#160570=CARTESIAN_POINT('Ctrl Pts',(-13.7303543679443,-14.2099227749143,
118.000394349248)) ;
#160571=CARTESIAN_POINT('Ctrl Pts',(-13.8041581860649,-14.209922839776,
117.976163230505)) ;
#160572=CARTESIAN_POINT('Ctrl Pts',(-13.8190101938493,-14.2690402748751,
118.021400047847)) ;
#160573=CARTESIAN_POINT('Ctrl Pts',(-13.8338622016338,-14.3281577099741,
118.066636865189)) ;
#160574=CARTESIAN_POINT('Ctrl Pts',(-13.7600583835132,-14.3281576451124,
118.090867983933)) ;
#160575=CARTESIAN_POINT('Ctrl Pts',(-13.6862545653926,-14.3281575802507,
118.115099102677)) ;
#160576=CARTESIAN_POINT('Ctrl Pts',(-13.6714025576082,-14.2690401451517,
118.069862285334)) ;
#160577=CARTESIAN_POINT('Ctrl Pts',(-13.6038901489006,-14.418345814643,
117.828744781992)) ;
#160578=CARTESIAN_POINT('Ctrl Pts',(-13.5944639944471,-14.3487174926443,
117.80003423849)) ;
#160579=CARTESIAN_POINT('Ctrl Pts',(-13.6682678073288,-14.3487175346435,
117.77580310379)) ;
#160580=CARTESIAN_POINT('Ctrl Pts',(-13.7420716202107,-14.3487175766427,
117.751571969089)) ;
#160581=CARTESIAN_POINT('Ctrl Pts',(-13.7514977746642,-14.4183458986414,
117.780282512592)) ;
#160582=CARTESIAN_POINT('Ctrl Pts',(-13.7609239291177,-14.48797422064,117.808993056095)) ;
#160583=CARTESIAN_POINT('Ctrl Pts',(-13.6871201162359,-14.4879741786408,
117.833224190795)) ;
#160584=CARTESIAN_POINT('Ctrl Pts',(-13.6133163033541,-14.4879741366417,
117.857455325495)) ;
#160585=CARTESIAN_POINT('Ctrl Pts',(-13.6038901489006,-14.418345814643,
117.828744781992)) ;
#160586=CARTESIAN_POINT('Ctrl Pts',(-13.5270066699605,-14.4960013207205,
117.559173432525)) ;
#160587=CARTESIAN_POINT('Ctrl Pts',(-13.5236667615923,-14.4208489309484,
117.549000612615)) ;
#160588=CARTESIAN_POINT('Ctrl Pts',(-13.5974705716151,-14.4208489456351,
117.524769469207)) ;
#160589=CARTESIAN_POINT('Ctrl Pts',(-13.6712743816379,-14.4208489603219,
117.500538325799)) ;
#160590=CARTESIAN_POINT('Ctrl Pts',(-13.6746142900061,-14.496001350094,
117.510711145709)) ;
#160591=CARTESIAN_POINT('Ctrl Pts',(-13.6779541983743,-14.5711537398661,
117.520883965618)) ;
#160592=CARTESIAN_POINT('Ctrl Pts',(-13.6041503883515,-14.5711537251794,
117.545115109027)) ;
#160593=CARTESIAN_POINT('Ctrl Pts',(-13.5303465783287,-14.5711537104926,
117.569346252435)) ;
#160594=CARTESIAN_POINT('Ctrl Pts',(-13.5270066699605,-14.4960013207205,
117.559173432525)) ;
#160595=CARTESIAN_POINT('Ctrl Pts',(-13.4463172125483,-14.4962457299704,
117.277772265082)) ;
#160596=CARTESIAN_POINT('Ctrl Pts',(-13.4493430518799,-14.4209645456079,
117.286988485564)) ;
#160597=CARTESIAN_POINT('Ctrl Pts',(-13.5231468617819,-14.4209645311187,
117.262757341788)) ;
#160598=CARTESIAN_POINT('Ctrl Pts',(-13.5969506716839,-14.4209645166296,
117.238526198012)) ;
#160599=CARTESIAN_POINT('Ctrl Pts',(-13.5939248323523,-14.4962457009921,
117.22930997753)) ;
#160600=CARTESIAN_POINT('Ctrl Pts',(-13.5908989930207,-14.5715268853546,
117.220093757049)) ;
#160601=CARTESIAN_POINT('Ctrl Pts',(-13.5170951831187,-14.5715268998438,
117.244324900825)) ;
#160602=CARTESIAN_POINT('Ctrl Pts',(-13.4432913732167,-14.5715269143329,
117.268556044601)) ;
#160603=CARTESIAN_POINT('Ctrl Pts',(-13.4463172125483,-14.4962457299704,
117.277772265082)) ;
#160604=CARTESIAN_POINT('Ctrl Pts',(-13.3696988473351,-14.4198799151553,
117.009166760654)) ;
#160605=CARTESIAN_POINT('Ctrl Pts',(-13.3788075758718,-14.3498193552219,
117.036910480173)) ;
#160606=CARTESIAN_POINT('Ctrl Pts',(-13.4526113883286,-14.3498193130492,
117.012679344178)) ;
#160607=CARTESIAN_POINT('Ctrl Pts',(-13.5264152007854,-14.3498192708765,
116.988448208184)) ;
#160608=CARTESIAN_POINT('Ctrl Pts',(-13.5173064722488,-14.4198798308098,
116.960704488665)) ;
#160609=CARTESIAN_POINT('Ctrl Pts',(-13.5081977437121,-14.4899403907432,
116.932960769146)) ;
#160610=CARTESIAN_POINT('Ctrl Pts',(-13.4343939312553,-14.4899404329159,
116.957191905141)) ;
#160611=CARTESIAN_POINT('Ctrl Pts',(-13.3605901187985,-14.4899404750886,
116.981423041135)) ;
#160612=CARTESIAN_POINT('Ctrl Pts',(-13.3696988473351,-14.4198799151553,
117.009166760654)) ;
#160613=CARTESIAN_POINT('Ctrl Pts',(-13.3017866089322,-14.2709014086462,
116.76670550127)) ;
#160614=CARTESIAN_POINT('Ctrl Pts',(-13.3163871564839,-14.2111372247694,
116.811176415367)) ;
#160615=CARTESIAN_POINT('Ctrl Pts',(-13.390190974086,-14.2111371588843,
116.786945295044)) ;
#160616=CARTESIAN_POINT('Ctrl Pts',(-13.4639947916881,-14.2111370929992,
116.762714174722)) ;
#160617=CARTESIAN_POINT('Ctrl Pts',(-13.4493942441364,-14.270901276876,
116.718243260625)) ;
#160618=CARTESIAN_POINT('Ctrl Pts',(-13.4347936965847,-14.3306654607528,
116.673772346528)) ;
#160619=CARTESIAN_POINT('Ctrl Pts',(-13.3609898789826,-14.3306655266379,
116.698003466851)) ;
#160620=CARTESIAN_POINT('Ctrl Pts',(-13.2871860613805,-14.330665592523,
116.722234587174)) ;
#160621=CARTESIAN_POINT('Ctrl Pts',(-13.3017866089322,-14.2709014086462,
116.76670550127)) ;
#160622=CARTESIAN_POINT('Ctrl Pts',(-13.2493889815294,-14.0614284920593,
116.571702252918)) ;
#160623=CARTESIAN_POINT('Ctrl Pts',(-13.2684022387902,-14.016200017183,
116.629613568744)) ;
#160624=CARTESIAN_POINT('Ctrl Pts',(-13.342206063304,-14.01619993407,116.605382469473)) ;
#160625=CARTESIAN_POINT('Ctrl Pts',(-13.4160098878178,-14.016199850957,
116.581151370202)) ;
#160626=CARTESIAN_POINT('Ctrl Pts',(-13.396996630557,-14.0614283258333,
116.523240054376)) ;
#160627=CARTESIAN_POINT('Ctrl Pts',(-13.3779833732962,-14.1066568007097,
116.46532873855)) ;
#160628=CARTESIAN_POINT('Ctrl Pts',(-13.3041795487824,-14.1066568838226,
116.48955983782)) ;
#160629=CARTESIAN_POINT('Ctrl Pts',(-13.2303757242686,-14.1066569669356,
116.513790937091)) ;
#160630=CARTESIAN_POINT('Ctrl Pts',(-13.2493889815294,-14.0614284920593,
116.571702252918)) ;
#160631=CARTESIAN_POINT('Ctrl Pts',(-13.2164243628667,-13.8059370930909,
116.435853274894)) ;
#160632=CARTESIAN_POINT('Ctrl Pts',(-13.23850096586,-13.778478597832,116.503095047478)) ;
#160633=CARTESIAN_POINT('Ctrl Pts',(-13.3123047984058,-13.7784785051367,
116.478863972672)) ;
#160634=CARTESIAN_POINT('Ctrl Pts',(-13.3861086309516,-13.7784784124414,
116.454632897865)) ;
#160635=CARTESIAN_POINT('Ctrl Pts',(-13.3640320279583,-13.8059369077003,
116.38739112528)) ;
#160636=CARTESIAN_POINT('Ctrl Pts',(-13.3419554249649,-13.8333954029592,
116.320149352695)) ;
#160637=CARTESIAN_POINT('Ctrl Pts',(-13.2681515924191,-13.8333954956545,
116.344380427502)) ;
#160638=CARTESIAN_POINT('Ctrl Pts',(-13.1943477598733,-13.8333955883498,
116.368611502309)) ;
#160639=CARTESIAN_POINT('Ctrl Pts',(-13.2164243628667,-13.8059370930909,
116.435853274894)) ;
#160640=CARTESIAN_POINT('Ctrl Pts',(-13.2062477246467,-13.5211628984478,
116.369237660814)) ;
#160641=CARTESIAN_POINT('Ctrl Pts',(-13.2298051727491,-13.5135452087457,
116.44098984855)) ;
#160642=CARTESIAN_POINT('Ctrl Pts',(-13.3036090135613,-13.5135451161284,
116.416758798922)) ;
#160643=CARTESIAN_POINT('Ctrl Pts',(-13.3774128543735,-13.513545023511,
116.392527749293)) ;
#160644=CARTESIAN_POINT('Ctrl Pts',(-13.3538554062711,-13.5211627132132,
116.320775561557)) ;
#160645=CARTESIAN_POINT('Ctrl Pts',(-13.3302979581687,-13.5287804029153,
116.24902337382)) ;
#160646=CARTESIAN_POINT('Ctrl Pts',(-13.2564941173566,-13.5287804955326,
116.273254423449)) ;
#160647=CARTESIAN_POINT('Ctrl Pts',(-13.1826902765444,-13.52878058815,116.297485473077)) ;
#160648=CARTESIAN_POINT('Ctrl Pts',(-13.2062477246467,-13.5211628984478,
116.369237660814)) ;
#160649=CARTESIAN_POINT('Ctrl Pts',(-13.2201829843462,-13.2317212421624,
116.376408413708)) ;
#160650=CARTESIAN_POINT('Ctrl Pts',(-13.2435326740826,-13.244300576159,
116.447527802893)) ;
#160651=CARTESIAN_POINT('Ctrl Pts',(-13.3173365223856,-13.2443004892996,
116.42329677608)) ;
#160652=CARTESIAN_POINT('Ctrl Pts',(-13.3911403706885,-13.2443004024403,
116.399065749266)) ;
#160653=CARTESIAN_POINT('Ctrl Pts',(-13.367790680952,-13.2317210684437,
116.327946360081)) ;
#160654=CARTESIAN_POINT('Ctrl Pts',(-13.3444409912156,-13.2191417344471,
116.256826970896)) ;
#160655=CARTESIAN_POINT('Ctrl Pts',(-13.2706371429126,-13.2191418213064,
116.281057997709)) ;
#160656=CARTESIAN_POINT('Ctrl Pts',(-13.1968332946097,-13.2191419081658,
116.305289024523)) ;
#160657=CARTESIAN_POINT('Ctrl Pts',(-13.2201829843462,-13.2317212421624,
116.376408413708)) ;
#160658=CARTESIAN_POINT('Ctrl Pts',(-13.2582351273943,-12.953209842425,
116.456720631326)) ;
#160659=CARTESIAN_POINT('Ctrl Pts',(-13.2796998255669,-12.9852534588735,
116.522098640202)) ;
#160660=CARTESIAN_POINT('Ctrl Pts',(-13.3535036799056,-12.9852533862488,
116.497867631773)) ;
#160661=CARTESIAN_POINT('Ctrl Pts',(-13.4273075342443,-12.9852533136241,
116.473636623344)) ;
#160662=CARTESIAN_POINT('Ctrl Pts',(-13.4058428360717,-12.9532096971755,
116.408258614468)) ;
#160663=CARTESIAN_POINT('Ctrl Pts',(-13.384378137899,-12.921166080727,116.342880605593)) ;
#160664=CARTESIAN_POINT('Ctrl Pts',(-13.3105742835603,-12.9211661533517,
116.367111614022)) ;
#160665=CARTESIAN_POINT('Ctrl Pts',(-13.2367704292216,-12.9211662259765,
116.391342622451)) ;
#160666=CARTESIAN_POINT('Ctrl Pts',(-13.2582351273943,-12.953209842425,
116.456720631326)) ;
#160667=CARTESIAN_POINT('Ctrl Pts',(-13.3179987777289,-12.7094642616823,
116.60338316649)) ;
#160668=CARTESIAN_POINT('Ctrl Pts',(-13.336055040414,-12.7585743721417,
116.658379630691)) ;
#160669=CARTESIAN_POINT('Ctrl Pts',(-13.4098588990292,-12.7585743165694,
116.634148635288)) ;
#160670=CARTESIAN_POINT('Ctrl Pts',(-13.4836627576445,-12.7585742609971,
116.609917639884)) ;
#160671=CARTESIAN_POINT('Ctrl Pts',(-13.4656064949594,-12.7094641505378,
116.554921175684)) ;
#160672=CARTESIAN_POINT('Ctrl Pts',(-13.4475502322743,-12.6603540400784,
116.499924711483)) ;
#160673=CARTESIAN_POINT('Ctrl Pts',(-13.3737463736591,-12.6603540956507,
116.524155706886)) ;
#160674=CARTESIAN_POINT('Ctrl Pts',(-13.2999425150438,-12.660354151223,
116.54838670229)) ;
#160675=CARTESIAN_POINT('Ctrl Pts',(-13.3179987777289,-12.7094642616823,
116.60338316649)) ;
#160676=CARTESIAN_POINT('Ctrl Pts',(-13.3968395702768,-12.5150572905195,
116.807856696789)) ;
#160677=CARTESIAN_POINT('Ctrl Pts',(-13.4101566106701,-12.5778156836835,
116.848418254369)) ;
#160678=CARTESIAN_POINT('Ctrl Pts',(-13.4839604707963,-12.5778156484991,
116.824187263567)) ;
#160679=CARTESIAN_POINT('Ctrl Pts',(-13.5577643309226,-12.5778156133148,
116.799956272766)) ;
#160680=CARTESIAN_POINT('Ctrl Pts',(-13.5444472905293,-12.5150572201508,
116.759394715186)) ;
#160681=CARTESIAN_POINT('Ctrl Pts',(-13.531130250136,-12.4522988269869,
116.718833157607)) ;
#160682=CARTESIAN_POINT('Ctrl Pts',(-13.4573263900098,-12.4522988621712,
116.743064148408)) ;
#160683=CARTESIAN_POINT('Ctrl Pts',(-13.3835225298836,-12.4522988973556,
116.767295139209)) ;
#160684=CARTESIAN_POINT('Ctrl Pts',(-13.3968395702768,-12.5150572905195,
116.807856696789)) ;
#160685=CARTESIAN_POINT('Ctrl Pts',(-13.4880657336334,-12.3871819681861,
117.050541251165)) ;
#160686=CARTESIAN_POINT('Ctrl Pts',(-13.4957612186245,-12.4589631112732,
117.073980457915)) ;
#160687=CARTESIAN_POINT('Ctrl Pts',(-13.5695650793503,-12.4589630933021,
117.049749468939)) ;
#160688=CARTESIAN_POINT('Ctrl Pts',(-13.6433689400761,-12.458963075331,
117.025518479964)) ;
#160689=CARTESIAN_POINT('Ctrl Pts',(-13.635673455085,-12.3871819322439,
117.002079273215)) ;
#160690=CARTESIAN_POINT('Ctrl Pts',(-13.6279779700939,-12.3154007891568,
116.978640066466)) ;
#160691=CARTESIAN_POINT('Ctrl Pts',(-13.5541741093681,-12.3154008071279,
117.002871055441)) ;
#160692=CARTESIAN_POINT('Ctrl Pts',(-13.4803702486423,-12.315400825099,
117.027102044416)) ;
#160693=CARTESIAN_POINT('Ctrl Pts',(-13.4880657336334,-12.3871819681861,
117.050541251165)) ;
#160694=CARTESIAN_POINT('Ctrl Pts',(-13.5882207279045,-12.3316884564228,
117.319958997263)) ;
#160695=CARTESIAN_POINT('Ctrl Pts',(-13.5896724457049,-12.4074536121107,
117.324380696378)) ;
#160696=CARTESIAN_POINT('Ctrl Pts',(-13.663476304107,-12.4074536102533,
117.300149700326)) ;
#160697=CARTESIAN_POINT('Ctrl Pts',(-13.7372801625091,-12.407453608396,
117.275918704273)) ;
#160698=CARTESIAN_POINT('Ctrl Pts',(-13.7358284447087,-12.3316884527082,
117.271497005158)) ;
#160699=CARTESIAN_POINT('Ctrl Pts',(-13.7343767269083,-12.2559232970203,
117.267075306043)) ;
#160700=CARTESIAN_POINT('Ctrl Pts',(-13.6605728685062,-12.2559232988777,
117.291306302096)) ;
#160701=CARTESIAN_POINT('Ctrl Pts',(-13.5867690101041,-12.255923300735,
117.315537298149)) ;
#160702=CARTESIAN_POINT('Ctrl Pts',(-13.5882207279045,-12.3316884564228,
117.319958997263)) ;
#160703=CARTESIAN_POINT('Ctrl Pts',(-13.6888941607603,-12.3542922095437,
117.591275254107)) ;
#160704=CARTESIAN_POINT('Ctrl Pts',(-13.6840497212975,-12.4285936621951,
117.576519873938)) ;
#160705=CARTESIAN_POINT('Ctrl Pts',(-13.7578535770702,-12.428593671534,
117.552288869877)) ;
#160706=CARTESIAN_POINT('Ctrl Pts',(-13.831657432843,-12.428593680873,117.528057865815)) ;
#160707=CARTESIAN_POINT('Ctrl Pts',(-13.8365018723058,-12.3542922282216,
117.542813245984)) ;
#160708=CARTESIAN_POINT('Ctrl Pts',(-13.8413463117686,-12.2799907755701,
117.557568626153)) ;
#160709=CARTESIAN_POINT('Ctrl Pts',(-13.7675424559959,-12.2799907662312,
117.581799630214)) ;
#160710=CARTESIAN_POINT('Ctrl Pts',(-13.6937386002231,-12.2799907568923,
117.606030634276)) ;
#160711=CARTESIAN_POINT('Ctrl Pts',(-13.6888941607603,-12.3542922095437,
117.591275254107)) ;
#160712=CARTESIAN_POINT('Ctrl Pts',(-13.7853698113562,-12.4537268763868,
117.849457635997)) ;
#160713=CARTESIAN_POINT('Ctrl Pts',(-13.774519802585,-12.5211987643482,
117.816410260506)) ;
#160714=CARTESIAN_POINT('Ctrl Pts',(-13.8483236542404,-12.5211987790939,
117.792179243904)) ;
#160715=CARTESIAN_POINT('Ctrl Pts',(-13.9221275058957,-12.5211987938395,
117.767948227302)) ;
#160716=CARTESIAN_POINT('Ctrl Pts',(-13.932977514667,-12.4537269058781,
117.800995602792)) ;
#160717=CARTESIAN_POINT('Ctrl Pts',(-13.9438275234382,-12.3862550179166,
117.834042978283)) ;
#160718=CARTESIAN_POINT('Ctrl Pts',(-13.8700236717828,-12.386255003171,
117.858273994885)) ;
#160719=CARTESIAN_POINT('Ctrl Pts',(-13.7962198201275,-12.3862549884253,
117.882505011487)) ;
#160720=CARTESIAN_POINT('Ctrl Pts',(-13.7853698113562,-12.4537268763868,
117.849457635997)) ;
#160721=CARTESIAN_POINT('Ctrl Pts',(-13.8696982601704,-12.6212675456056,
118.070986029358)) ;
#160722=CARTESIAN_POINT('Ctrl Pts',(-13.8536747152405,-12.6771429779521,
118.022180897344)) ;
#160723=CARTESIAN_POINT('Ctrl Pts',(-13.9274785638659,-12.6771429943205,
117.997949871512)) ;
#160724=CARTESIAN_POINT('Ctrl Pts',(-14.0012824124912,-12.6771430106889,
117.973718845681)) ;
#160725=CARTESIAN_POINT('Ctrl Pts',(-14.017305957421,-12.6212675783423,
118.022523977695)) ;
#160726=CARTESIAN_POINT('Ctrl Pts',(-14.0333295023509,-12.5653921459958,
118.07132910971)) ;
#160727=CARTESIAN_POINT('Ctrl Pts',(-13.9595256537255,-12.5653921296274,
118.095560135541)) ;
#160728=CARTESIAN_POINT('Ctrl Pts',(-13.8857218051002,-12.565392113259,
118.119791161372)) ;
#160729=CARTESIAN_POINT('Ctrl Pts',(-13.8696982601704,-12.6212675456056,
118.070986029358)) ;
#160730=CARTESIAN_POINT('Ctrl Pts',(-13.9378798134609,-12.846192059173,
118.243189707452)) ;
#160731=CARTESIAN_POINT('Ctrl Pts',(-13.917805231475,-12.8864467914097,
118.18204577005)) ;
#160732=CARTESIAN_POINT('Ctrl Pts',(-13.9916090772929,-12.8864468052169,
118.157814735668)) ;
#160733=CARTESIAN_POINT('Ctrl Pts',(-14.0654129231109,-12.8864468190241,
118.133583701286)) ;
#160734=CARTESIAN_POINT('Ctrl Pts',(-14.0854875050968,-12.8461920867874,
118.194727638688)) ;
#160735=CARTESIAN_POINT('Ctrl Pts',(-14.1055620870827,-12.8059373545508,
118.25587157609)) ;
#160736=CARTESIAN_POINT('Ctrl Pts',(-14.0317582412647,-12.8059373407436,
118.280102610472)) ;
#160737=CARTESIAN_POINT('Ctrl Pts',(-13.9579543954468,-12.8059373269364,
118.304333644854)) ;
#160738=CARTESIAN_POINT('Ctrl Pts',(-13.9378798134609,-12.846192059173,
118.243189707452)) ;
#160739=CARTESIAN_POINT('Ctrl Pts',(-13.9854016724836,-13.1124184461725,
118.352441492381)) ;
#160740=CARTESIAN_POINT('Ctrl Pts',(-13.9627130007129,-13.1341445509028,
118.283335459142)) ;
#160741=CARTESIAN_POINT('Ctrl Pts',(-14.0365168447199,-13.1341445595333,
118.259104419244)) ;
#160742=CARTESIAN_POINT('Ctrl Pts',(-14.1103206887269,-13.1341445681639,
118.234873379346)) ;
#160743=CARTESIAN_POINT('Ctrl Pts',(-14.1330093604975,-13.1124184634336,
118.303979412585)) ;
#160744=CARTESIAN_POINT('Ctrl Pts',(-14.1556980322682,-13.0906923587033,
118.373085445824)) ;
#160745=CARTESIAN_POINT('Ctrl Pts',(-14.0818941882612,-13.0906923500727,
118.397316485722)) ;
#160746=CARTESIAN_POINT('Ctrl Pts',(-14.0080903442542,-13.0906923414422,
118.42154752562)) ;
#160747=CARTESIAN_POINT('Ctrl Pts',(-13.9854016724836,-13.1124184461725,
118.352441492381)) ;
#160748=CARTESIAN_POINT('Ctrl Pts',(-14.0095130072085,-13.400879749144,
118.390345126407)) ;
#160749=CARTESIAN_POINT('Ctrl Pts',(-13.9858419287106,-13.4024961126535,
118.318246840676)) ;
#160750=CARTESIAN_POINT('Ctrl Pts',(-14.059645772004,-13.4024961156936,
118.294015798605)) ;
#160751=CARTESIAN_POINT('Ctrl Pts',(-14.1334496152975,-13.4024961187337,
118.269784756533)) ;
#160752=CARTESIAN_POINT('Ctrl Pts',(-14.1571206937954,-13.4008797552242,
118.341883042265)) ;
#160753=CARTESIAN_POINT('Ctrl Pts',(-14.1807917722932,-13.3992633917147,
118.413981327996)) ;
#160754=CARTESIAN_POINT('Ctrl Pts',(-14.1069879289998,-13.3992633886746,
118.438212370068)) ;
#160755=CARTESIAN_POINT('Ctrl Pts',(-14.0331840857064,-13.3992633856344,
118.462443412139)) ;
#160756=CARTESIAN_POINT('Ctrl Pts',(-14.0095130072085,-13.400879749144,
118.390345126407)) ;
#160757=CARTESIAN_POINT('Ctrl Pts',(-14.0093724892591,-13.6891262166377,
118.354574264124)) ;
#160758=CARTESIAN_POINT('Ctrl Pts',(-13.9864072579121,-13.6706178186388,
118.284625874855)) ;
#160759=CARTESIAN_POINT('Ctrl Pts',(-14.0602111012856,-13.6706178179427,
118.260394833028)) ;
#160760=CARTESIAN_POINT('Ctrl Pts',(-14.1340149446592,-13.6706178172465,
118.236163791201)) ;
#160761=CARTESIAN_POINT('Ctrl Pts',(-14.1569801760062,-13.6891262152454,
118.30611218047)) ;
#160762=CARTESIAN_POINT('Ctrl Pts',(-14.1799454073532,-13.7076346132443,
118.376060569739)) ;
#160763=CARTESIAN_POINT('Ctrl Pts',(-14.1061415639797,-13.7076346139405,
118.400291611566)) ;
#160764=CARTESIAN_POINT('Ctrl Pts',(-14.0323377206061,-13.7076346146366,
118.424522653393)) ;
#160765=CARTESIAN_POINT('Ctrl Pts',(-14.0093724892591,-13.6891262166377,
118.354574264124)) ;
#160766=CARTESIAN_POINT('Ctrl Pts',(-13.985414910218,-13.9605413879786,
118.245894494186)) ;
#160767=CARTESIAN_POINT('Ctrl Pts',(-13.9648272415158,-13.9230519796462,
118.183187777064)) ;
#160768=CARTESIAN_POINT('Ctrl Pts',(-14.0386310853959,-13.9230519767635,
118.15895673678)) ;
#160769=CARTESIAN_POINT('Ctrl Pts',(-14.1124349292761,-13.9230519738809,
118.134725696495)) ;
#160770=CARTESIAN_POINT('Ctrl Pts',(-14.1330225979783,-13.9605413822133,
118.197432413617)) ;
#160771=CARTESIAN_POINT('Ctrl Pts',(-14.1536102666806,-13.9980307905457,
118.260139130739)) ;
#160772=CARTESIAN_POINT('Ctrl Pts',(-14.0798064228004,-13.9980307934284,
118.284370171023)) ;
#160773=CARTESIAN_POINT('Ctrl Pts',(-14.0060025789203,-13.9980307963111,
118.308601211307)) ;
#160774=CARTESIAN_POINT('Ctrl Pts',(-13.985414910218,-13.9605413879786,
118.245894494186)) ;
#160775=CARTESIAN_POINT('Ctrl Pts',(-13.9409451108123,-14.1894540736428,
118.075288407443)) ;
#160776=CARTESIAN_POINT('Ctrl Pts',(-13.9241599655485,-14.1359254038344,
118.02416356318)) ;
#160777=CARTESIAN_POINT('Ctrl Pts',(-13.9979638096976,-14.1359254016367,
117.999932523715)) ;
#160778=CARTESIAN_POINT('Ctrl Pts',(-14.0717676538467,-14.135925399439,
117.97570148425)) ;
#160779=CARTESIAN_POINT('Ctrl Pts',(-14.0885527991105,-14.1894540692474,
118.026826328513)) ;
#160780=CARTESIAN_POINT('Ctrl Pts',(-14.1053379443743,-14.2429827390558,
118.077951172775)) ;
#160781=CARTESIAN_POINT('Ctrl Pts',(-14.0315341002252,-14.2429827412535,
118.10218221224)) ;
#160782=CARTESIAN_POINT('Ctrl Pts',(-13.9577302560761,-14.2429827434512,
118.126413251706)) ;
#160783=CARTESIAN_POINT('Ctrl Pts',(-13.9409451108123,-14.1894540736428,
118.075288407443)) ;
#160784=CARTESIAN_POINT('Ctrl Pts',(-13.8788030525502,-14.3660067048925,
117.850395877402)) ;
#160785=CARTESIAN_POINT('Ctrl Pts',(-13.8670695405437,-14.3000702425711,
117.814657493004)) ;
#160786=CARTESIAN_POINT('Ctrl Pts',(-13.9408733842996,-14.3000702422313,
117.790426452341)) ;
#160787=CARTESIAN_POINT('Ctrl Pts',(-14.0146772280555,-14.3000702418915,
117.766195411678)) ;
#160788=CARTESIAN_POINT('Ctrl Pts',(-14.026410740062,-14.3660067042129,
117.801933796077)) ;
#160789=CARTESIAN_POINT('Ctrl Pts',(-14.0381442520685,-14.4319431665342,
117.837672180475)) ;
#160790=CARTESIAN_POINT('Ctrl Pts',(-13.9643404083126,-14.431943166874,
117.861903221138)) ;
#160791=CARTESIAN_POINT('Ctrl Pts',(-13.8905365645568,-14.4319431672138,
117.886134261801)) ;
#160792=CARTESIAN_POINT('Ctrl Pts',(-13.8788030525502,-14.3660067048925,
117.850395877402)) ;
#160793=CARTESIAN_POINT('Ctrl Pts',(-13.805049295041,-14.4734792612079,
117.590360278057)) ;
#160794=CARTESIAN_POINT('Ctrl Pts',(-13.7991810058367,-14.3999420243742,
117.572486416034)) ;
#160795=CARTESIAN_POINT('Ctrl Pts',(-13.8729848485188,-14.3999420254069,
117.548255372101)) ;
#160796=CARTESIAN_POINT('Ctrl Pts',(-13.9467886912009,-14.3999420264397,
117.524024328167)) ;
#160797=CARTESIAN_POINT('Ctrl Pts',(-13.9526569804052,-14.4734792632734,
117.54189819019)) ;
#160798=CARTESIAN_POINT('Ctrl Pts',(-13.9585252696096,-14.5470165001072,
117.559772052213)) ;
#160799=CARTESIAN_POINT('Ctrl Pts',(-13.8847214269275,-14.5470164990744,
117.584003096146)) ;
#160800=CARTESIAN_POINT('Ctrl Pts',(-13.8109175842454,-14.5470164980416,
117.60823414008)) ;
#160801=CARTESIAN_POINT('Ctrl Pts',(-13.805049295041,-14.4734792612079,
117.590360278057)) ;
#160802=CARTESIAN_POINT('Ctrl Pts',(-13.7251059804211,-14.5056975632985,
117.311316857951)) ;
#160803=CARTESIAN_POINT('Ctrl Pts',(-13.7255468602542,-14.4298031115965,
117.312659706948)) ;
#160804=CARTESIAN_POINT('Ctrl Pts',(-13.7993507010675,-14.4298031119292,
117.288428657322)) ;
#160805=CARTESIAN_POINT('Ctrl Pts',(-13.8731545418808,-14.4298031122619,
117.264197607697)) ;
#160806=CARTESIAN_POINT('Ctrl Pts',(-13.8727136620476,-14.5056975639639,
117.2628547587)) ;
#160807=CARTESIAN_POINT('Ctrl Pts',(-13.8722727822144,-14.5815920156659,
117.261511909703)) ;
#160808=CARTESIAN_POINT('Ctrl Pts',(-13.7984689414012,-14.5815920153332,
117.285742959328)) ;
#160809=CARTESIAN_POINT('Ctrl Pts',(-13.7246651005879,-14.5815920150005,
117.309974008954)) ;
#160810=CARTESIAN_POINT('Ctrl Pts',(-13.7251059804211,-14.5056975632985,
117.311316857951)) ;
#160811=CARTESIAN_POINT('Ctrl Pts',(-13.6460687434891,-14.4599236721213,
117.035189019244)) ;
#160812=CARTESIAN_POINT('Ctrl Pts',(-13.6527613166628,-14.387115192455,
117.055573517566)) ;
#160813=CARTESIAN_POINT('Ctrl Pts',(-13.7265651557173,-14.3871151888849,
117.031342462584)) ;
#160814=CARTESIAN_POINT('Ctrl Pts',(-13.8003689947718,-14.3871151853148,
117.007111407601)) ;
#160815=CARTESIAN_POINT('Ctrl Pts',(-13.7936764215981,-14.4599236649811,
116.986726909279)) ;
#160816=CARTESIAN_POINT('Ctrl Pts',(-13.7869838484244,-14.5327321446473,
116.966342410956)) ;
#160817=CARTESIAN_POINT('Ctrl Pts',(-13.7131800093699,-14.5327321482174,
116.990573465939)) ;
#160818=CARTESIAN_POINT('Ctrl Pts',(-13.6393761703155,-14.5327321517875,
117.014804520921)) ;
#160819=CARTESIAN_POINT('Ctrl Pts',(-13.6460687434891,-14.4599236721213,
117.035189019244)) ;
#160820=CARTESIAN_POINT('Ctrl Pts',(-13.5738853047407,-14.3395761921465,
116.779866121718)) ;
#160821=CARTESIAN_POINT('Ctrl Pts',(-13.5863614796708,-14.27506508821,116.817866537953)) ;
#160822=CARTESIAN_POINT('Ctrl Pts',(-13.660165317222,-14.2750650771765,
116.793635478392)) ;
#160823=CARTESIAN_POINT('Ctrl Pts',(-13.7339691547732,-14.2750650661431,
116.76940441883)) ;
#160824=CARTESIAN_POINT('Ctrl Pts',(-13.7214929798432,-14.3395761700796,
116.731404002596)) ;
#160825=CARTESIAN_POINT('Ctrl Pts',(-13.7090168049131,-14.4040872740161,
116.693403586361)) ;
#160826=CARTESIAN_POINT('Ctrl Pts',(-13.6352129673619,-14.4040872850496,
116.717634645922)) ;
#160827=CARTESIAN_POINT('Ctrl Pts',(-13.5614091298106,-14.404087296083,
116.741865705483)) ;
#160828=CARTESIAN_POINT('Ctrl Pts',(-13.5738853047407,-14.3395761921465,
116.779866121718)) ;
#160829=CARTESIAN_POINT('Ctrl Pts',(-13.5146382184193,-14.1535350418836,
116.563988746602)) ;
#160830=CARTESIAN_POINT('Ctrl Pts',(-13.5320020882261,-14.101920284912,
116.616876292952)) ;
#160831=CARTESIAN_POINT('Ctrl Pts',(-13.6058059252282,-14.1019202637606,
116.592645231719)) ;
#160832=CARTESIAN_POINT('Ctrl Pts',(-13.6796097622303,-14.1019202426092,
116.568414170485)) ;
#160833=CARTESIAN_POINT('Ctrl Pts',(-13.6622458924235,-14.1535349995808,
116.515526624135)) ;
#160834=CARTESIAN_POINT('Ctrl Pts',(-13.6448820226168,-14.2051497565524,
116.462639077784)) ;
#160835=CARTESIAN_POINT('Ctrl Pts',(-13.5710781856146,-14.2051497777038,
116.486870139018)) ;
#160836=CARTESIAN_POINT('Ctrl Pts',(-13.4972743486125,-14.2051497988552,
116.511101200251)) ;
#160837=CARTESIAN_POINT('Ctrl Pts',(-13.5146382184193,-14.1535350418836,
116.563988746602)) ;
#160838=CARTESIAN_POINT('Ctrl Pts',(-13.4731069605417,-13.9130985111844,
116.401832242531)) ;
#160839=CARTESIAN_POINT('Ctrl Pts',(-13.4941337169664,-13.8781962453412,
116.465876350717)) ;
#160840=CARTESIAN_POINT('Ctrl Pts',(-13.5679375545039,-13.8781962102056,
116.441645291114)) ;
#160841=CARTESIAN_POINT('Ctrl Pts',(-13.6417413920414,-13.87819617507,116.417414231511)) ;
#160842=CARTESIAN_POINT('Ctrl Pts',(-13.6207146356167,-13.9130984409133,
116.353370123325)) ;
#160843=CARTESIAN_POINT('Ctrl Pts',(-13.5996878791919,-13.9480007067565,
116.28932601514)) ;
#160844=CARTESIAN_POINT('Ctrl Pts',(-13.5258840416544,-13.9480007418921,
116.313557074743)) ;
#160845=CARTESIAN_POINT('Ctrl Pts',(-13.452080204117,-13.9480007770277,
116.337788134346)) ;
#160846=CARTESIAN_POINT('Ctrl Pts',(-13.4731069605417,-13.9130985111844,
116.401832242531)) ;
#160847=CARTESIAN_POINT('Ctrl Pts',(-13.4535360973529,-13.6395736822347,
116.306908957539)) ;
#160848=CARTESIAN_POINT('Ctrl Pts',(-13.4766902515202,-13.6237185301076,
116.377432776133)) ;
#160849=CARTESIAN_POINT('Ctrl Pts',(-13.5504940917278,-13.6237184841126,
116.353201724663)) ;
#160850=CARTESIAN_POINT('Ctrl Pts',(-13.6242979319354,-13.6237184381175,
116.328970673193)) ;
#160851=CARTESIAN_POINT('Ctrl Pts',(-13.6011437777682,-13.6395735902447,
116.258446854598)) ;
#160852=CARTESIAN_POINT('Ctrl Pts',(-13.577989623601,-13.6554287423718,
116.187923036004)) ;
#160853=CARTESIAN_POINT('Ctrl Pts',(-13.5041857833933,-13.6554287883668,
116.212154087474)) ;
#160854=CARTESIAN_POINT('Ctrl Pts',(-13.4303819431857,-13.6554288343619,
116.236385138944)) ;
#160855=CARTESIAN_POINT('Ctrl Pts',(-13.4535360973529,-13.6395736822347,
116.306908957539)) ;
#160856=CARTESIAN_POINT('Ctrl Pts',(-13.4576157743933,-13.3487006076146,
116.283814176628)) ;
#160857=CARTESIAN_POINT('Ctrl Pts',(-13.4812536077164,-13.3531309210736,
116.355811204069)) ;
#160858=CARTESIAN_POINT('Ctrl Pts',(-13.5550574520074,-13.3531308648212,
116.331580165036)) ;
#160859=CARTESIAN_POINT('Ctrl Pts',(-13.6288612962983,-13.3531308085687,
116.307349126003)) ;
#160860=CARTESIAN_POINT('Ctrl Pts',(-13.6052234629752,-13.3487004951098,
116.235352098562)) ;
#160861=CARTESIAN_POINT('Ctrl Pts',(-13.5815856296521,-13.3442701816508,
116.163355071121)) ;
#160862=CARTESIAN_POINT('Ctrl Pts',(-13.5077817853611,-13.3442702379032,
116.187586110155)) ;
#160863=CARTESIAN_POINT('Ctrl Pts',(-13.4339779410702,-13.3442702941557,
116.211817149188)) ;
#160864=CARTESIAN_POINT('Ctrl Pts',(-13.4576157743933,-13.3487006076146,
116.283814176628)) ;
#160865=CARTESIAN_POINT('Ctrl Pts',(-13.4859406302875,-13.0636371844073,
116.334679965118)) ;
#160866=CARTESIAN_POINT('Ctrl Pts',(-13.5083676426488,-13.0879765100876,
116.402989027427)) ;
#160867=CARTESIAN_POINT('Ctrl Pts',(-13.5821714923869,-13.0879764491053,
116.378758004986)) ;
#160868=CARTESIAN_POINT('Ctrl Pts',(-13.655975342125,-13.0879763881229,
116.354526982544)) ;
#160869=CARTESIAN_POINT('Ctrl Pts',(-13.6335483297638,-13.0636370624426,
116.286217920235)) ;
#160870=CARTESIAN_POINT('Ctrl Pts',(-13.6111213174025,-13.0392977367622,
116.217908857925)) ;
#160871=CARTESIAN_POINT('Ctrl Pts',(-13.5373174676644,-13.0392977977446,
116.242139880367)) ;
#160872=CARTESIAN_POINT('Ctrl Pts',(-13.4635136179263,-13.0392978587269,
116.266370902809)) ;
#160873=CARTESIAN_POINT('Ctrl Pts',(-13.4859406302875,-13.0636371844073,
116.334679965118)) ;
#160874=CARTESIAN_POINT('Ctrl Pts',(-13.537302484578,-12.803286823163,116.455624512449)) ;
#160875=CARTESIAN_POINT('Ctrl Pts',(-13.5569104932401,-12.8458384350668,
116.515347344498)) ;
#160876=CARTESIAN_POINT('Ctrl Pts',(-13.6307143492738,-12.8458383747554,
116.491116341231)) ;
#160877=CARTESIAN_POINT('Ctrl Pts',(-13.7045182053075,-12.8458383144439,
116.466885337965)) ;
#160878=CARTESIAN_POINT('Ctrl Pts',(-13.6849101966454,-12.8032867025401,
116.407162505917)) ;
#160879=CARTESIAN_POINT('Ctrl Pts',(-13.6653021879832,-12.7607350906363,
116.347439673868)) ;
#160880=CARTESIAN_POINT('Ctrl Pts',(-13.5914983319496,-12.7607351509478,
116.371670677135)) ;
#160881=CARTESIAN_POINT('Ctrl Pts',(-13.5176944759159,-12.7607352112592,
116.395901680401)) ;
#160882=CARTESIAN_POINT('Ctrl Pts',(-13.537302484578,-12.803286823163,116.455624512449)) ;
#160883=CARTESIAN_POINT('Ctrl Pts',(-13.6086911430819,-12.5872505028287,
116.637604570861)) ;
#160884=CARTESIAN_POINT('Ctrl Pts',(-13.6240771137081,-12.644946835435,
116.68446775642)) ;
#160885=CARTESIAN_POINT('Ctrl Pts',(-13.697880976079,-12.6449467832351,
116.660236772456)) ;
#160886=CARTESIAN_POINT('Ctrl Pts',(-13.7716848384499,-12.6449467310352,
116.636005788491)) ;
#160887=CARTESIAN_POINT('Ctrl Pts',(-13.7562988678237,-12.5872503984288,
116.589142602933)) ;
#160888=CARTESIAN_POINT('Ctrl Pts',(-13.7409128971974,-12.5295540658224,
116.542279417374)) ;
#160889=CARTESIAN_POINT('Ctrl Pts',(-13.6671090348266,-12.5295541180224,
116.566510401338)) ;
#160890=CARTESIAN_POINT('Ctrl Pts',(-13.5933051724557,-12.5295541702223,
116.590741385303)) ;
#160891=CARTESIAN_POINT('Ctrl Pts',(-13.6086911430819,-12.5872505028287,
116.637604570861)) ;
#160892=CARTESIAN_POINT('Ctrl Pts',(-13.6958832608641,-12.4304809457012,
116.867672531912)) ;
#160893=CARTESIAN_POINT('Ctrl Pts',(-13.705938807208,-12.4992062995871,
116.898300105306)) ;
#160894=CARTESIAN_POINT('Ctrl Pts',(-13.7797426752621,-12.4992062624081,
116.874069138652)) ;
#160895=CARTESIAN_POINT('Ctrl Pts',(-13.8535465433162,-12.4992062252292,
116.849838171998)) ;
#160896=CARTESIAN_POINT('Ctrl Pts',(-13.8434909969723,-12.4304808713433,
116.819210598604)) ;
#160897=CARTESIAN_POINT('Ctrl Pts',(-13.8334354506284,-12.3617555174574,
116.788583025209)) ;
#160898=CARTESIAN_POINT('Ctrl Pts',(-13.7596315825743,-12.3617555546364,
116.812813991863)) ;
#160899=CARTESIAN_POINT('Ctrl Pts',(-13.6858277145202,-12.3617555918153,
116.837044958517)) ;
#160900=CARTESIAN_POINT('Ctrl Pts',(-13.6958832608641,-12.4304809457012,
116.867672531912)) ;
#160901=CARTESIAN_POINT('Ctrl Pts',(-13.7933144950255,-12.3447676693836,
117.128927982332)) ;
#160902=CARTESIAN_POINT('Ctrl Pts',(-13.7973170359522,-12.4195774199376,
117.141119077995)) ;
#160903=CARTESIAN_POINT('Ctrl Pts',(-13.8711209081213,-12.4195774042201,
117.116888123875)) ;
#160904=CARTESIAN_POINT('Ctrl Pts',(-13.9449247802904,-12.4195773885026,
117.092657169754)) ;
#160905=CARTESIAN_POINT('Ctrl Pts',(-13.9409222393638,-12.3447676379485,
117.080466074092)) ;
#160906=CARTESIAN_POINT('Ctrl Pts',(-13.9369196984371,-12.2699578873945,
117.068274978429)) ;
#160907=CARTESIAN_POINT('Ctrl Pts',(-13.863115826268,-12.269957903112,117.092505932549)) ;
#160908=CARTESIAN_POINT('Ctrl Pts',(-13.7893119540988,-12.2699579188295,
117.11673688667)) ;
#160909=CARTESIAN_POINT('Ctrl Pts',(-13.7933144950255,-12.3447676693836,
117.128927982332)) ;
#160910=CARTESIAN_POINT('Ctrl Pts',(-13.8942106173158,-12.3358385329225,
117.400917482378)) ;
#160911=CARTESIAN_POINT('Ctrl Pts',(-13.8919056550011,-12.4113804397121,
117.393896940963)) ;
#160912=CARTESIAN_POINT('Ctrl Pts',(-13.965709528786,-12.4113804494303,
117.369665991764)) ;
#160913=CARTESIAN_POINT('Ctrl Pts',(-14.039513402571,-12.4113804591485,
117.345435042565)) ;
#160914=CARTESIAN_POINT('Ctrl Pts',(-14.0418183648857,-12.335838552359,
117.35245558398)) ;
#160915=CARTESIAN_POINT('Ctrl Pts',(-14.0441233272004,-12.2602966455695,
117.359476125395)) ;
#160916=CARTESIAN_POINT('Ctrl Pts',(-13.9703194534154,-12.2602966358513,
117.383707074594)) ;
#160917=CARTESIAN_POINT('Ctrl Pts',(-13.8965155796305,-12.260296626133,
117.407938023793)) ;
#160918=CARTESIAN_POINT('Ctrl Pts',(-13.8942106173158,-12.3358385329225,
117.400917482378)) ;
#160919=CARTESIAN_POINT('Ctrl Pts',(-13.9931058830893,-12.4042599768703,
117.666636589428)) ;
#160920=CARTESIAN_POINT('Ctrl Pts',(-13.9846276244577,-12.4751356263476,
117.640813183575)) ;
#160921=CARTESIAN_POINT('Ctrl Pts',(-14.0584314976336,-12.4751356632063,
117.616582232521)) ;
#160922=CARTESIAN_POINT('Ctrl Pts',(-14.1322353708096,-12.4751357000651,
117.592351281467)) ;
#160923=CARTESIAN_POINT('Ctrl Pts',(-14.1407136294413,-12.4042600505878,
117.61817468732)) ;
#160924=CARTESIAN_POINT('Ctrl Pts',(-14.1491918880729,-12.3333844011106,
117.643998093173)) ;
#160925=CARTESIAN_POINT('Ctrl Pts',(-14.0753880148969,-12.3333843642518,
117.668229044227)) ;
#160926=CARTESIAN_POINT('Ctrl Pts',(-14.0015841417209,-12.3333843273931,
117.692459995281)) ;
#160927=CARTESIAN_POINT('Ctrl Pts',(-13.9931058830893,-12.4042599768703,
117.666636589428)) ;
#160928=CARTESIAN_POINT('Ctrl Pts',(-14.0830802598219,-12.5454038835963,
117.905215825566)) ;
#160929=CARTESIAN_POINT('Ctrl Pts',(-14.0690417835344,-12.6065294802411,
117.862456893932)) ;
#160930=CARTESIAN_POINT('Ctrl Pts',(-14.1428456533588,-12.6065295430782,
117.83822593267)) ;
#160931=CARTESIAN_POINT('Ctrl Pts',(-14.2166495231833,-12.6065296059152,
117.813994971409)) ;
#160932=CARTESIAN_POINT('Ctrl Pts',(-14.2306879994708,-12.5454040092703,
117.856753903043)) ;
#160933=CARTESIAN_POINT('Ctrl Pts',(-14.2447264757583,-12.4842784126255,
117.899512834677)) ;
#160934=CARTESIAN_POINT('Ctrl Pts',(-14.1709226059339,-12.4842783497885,
117.923743795939)) ;
#160935=CARTESIAN_POINT('Ctrl Pts',(-14.0971187361094,-12.4842782869515,
117.9479747572)) ;
#160936=CARTESIAN_POINT('Ctrl Pts',(-14.0830802598219,-12.5454038835963,
117.905215825566)) ;
#160937=CARTESIAN_POINT('Ctrl Pts',(-14.1585388443987,-12.7490645526663,
118.099576579279)) ;
#160938=CARTESIAN_POINT('Ctrl Pts',(-14.1399454760981,-12.796061398436,
118.042944181542)) ;
#160939=CARTESIAN_POINT('Ctrl Pts',(-14.2137493401466,-12.7960614831609,
118.018713202688)) ;
#160940=CARTESIAN_POINT('Ctrl Pts',(-14.2875532041952,-12.7960615678859,
117.994482223833)) ;
#160941=CARTESIAN_POINT('Ctrl Pts',(-14.3061465724958,-12.7490647221162,
118.05111462157)) ;
#160942=CARTESIAN_POINT('Ctrl Pts',(-14.3247399407963,-12.7020678763465,
118.107747019307)) ;
#160943=CARTESIAN_POINT('Ctrl Pts',(-14.2509360767478,-12.7020677916216,
118.131977998162)) ;
#160944=CARTESIAN_POINT('Ctrl Pts',(-14.1771322126992,-12.7020677068967,
118.156208977016)) ;
#160945=CARTESIAN_POINT('Ctrl Pts',(-14.1585388443987,-12.7490645526663,
118.099576579279)) ;
#160946=CARTESIAN_POINT('Ctrl Pts',(-14.2147792241185,-13.0004109945635,
118.235435558541)) ;
#160947=CARTESIAN_POINT('Ctrl Pts',(-14.1929652259204,-13.0299291555683,
118.168993641801)) ;
#160948=CARTESIAN_POINT('Ctrl Pts',(-14.2667690823032,-13.0299292556675,
118.144762639597)) ;
#160949=CARTESIAN_POINT('Ctrl Pts',(-14.340572938686,-13.0299293557667,
118.120531637394)) ;
#160950=CARTESIAN_POINT('Ctrl Pts',(-14.362386936884,-13.0004111947619,
118.186973554135)) ;
#160951=CARTESIAN_POINT('Ctrl Pts',(-14.384200935082,-12.9708930337571,
118.253415470876)) ;
#160952=CARTESIAN_POINT('Ctrl Pts',(-14.3103970786992,-12.9708929336578,
118.277646473079)) ;
#160953=CARTESIAN_POINT('Ctrl Pts',(-14.2365932223165,-12.9708928335586,
118.301877475282)) ;
#160954=CARTESIAN_POINT('Ctrl Pts',(-14.2147792241185,-13.0004109945635,
118.235435558541)) ;
#160955=CARTESIAN_POINT('Ctrl Pts',(-14.2486273894212,-13.281956740539,
118.303050309436)) ;
#160956=CARTESIAN_POINT('Ctrl Pts',(-14.2251520583296,-13.2918622013087,
118.231548240752)) ;
#160957=CARTESIAN_POINT('Ctrl Pts',(-14.2989559059233,-13.2918623086419,
118.207317211779)) ;
#160958=CARTESIAN_POINT('Ctrl Pts',(-14.372759753517,-13.2918624159751,
118.183086182806)) ;
#160959=CARTESIAN_POINT('Ctrl Pts',(-14.3962350846086,-13.2819569552054,
118.25458825149)) ;
#160960=CARTESIAN_POINT('Ctrl Pts',(-14.4197104157001,-13.2720514944356,
118.326090320173)) ;
#160961=CARTESIAN_POINT('Ctrl Pts',(-14.3459065681064,-13.2720513871025,
118.350321349146)) ;
#160962=CARTESIAN_POINT('Ctrl Pts',(-14.2721027205127,-13.2720512797693,
118.37455237812)) ;
#160963=CARTESIAN_POINT('Ctrl Pts',(-14.2486273894212,-13.281956740539,
118.303050309436)) ;
#160964=CARTESIAN_POINT('Ctrl Pts',(-14.2583346166308,-13.573019683806,
118.297166121252)) ;
#160965=CARTESIAN_POINT('Ctrl Pts',(-14.234880205577,-13.5626188486144,
118.225727771601)) ;
#160966=CARTESIAN_POINT('Ctrl Pts',(-14.3086840441726,-13.5626189543087,
118.201496715222)) ;
#160967=CARTESIAN_POINT('Ctrl Pts',(-14.3824878827682,-13.5626190600031,
118.177265658842)) ;
#160968=CARTESIAN_POINT('Ctrl Pts',(-14.405942293822,-13.5730198951947,
118.248704008492)) ;
#160969=CARTESIAN_POINT('Ctrl Pts',(-14.4293967048758,-13.5834207303863,
118.320142358142)) ;
#160970=CARTESIAN_POINT('Ctrl Pts',(-14.3555928662802,-13.583420624692,
118.344373414522)) ;
#160971=CARTESIAN_POINT('Ctrl Pts',(-14.2817890276846,-13.5834205189976,
118.368604470902)) ;
#160972=CARTESIAN_POINT('Ctrl Pts',(-14.2583346166308,-13.573019683806,
118.297166121252)) ;
#160973=CARTESIAN_POINT('Ctrl Pts',(-14.2439797697,-13.8532505028034,118.217957846964)) ;
#160974=CARTESIAN_POINT('Ctrl Pts',(-14.222226824094,-13.823269355178,118.151701886488)) ;
#160975=CARTESIAN_POINT('Ctrl Pts',(-14.2960306544012,-13.823269450611,
118.127470804863)) ;
#160976=CARTESIAN_POINT('Ctrl Pts',(-14.3698344847084,-13.8232695460439,
118.103239723238)) ;
#160977=CARTESIAN_POINT('Ctrl Pts',(-14.3915874303144,-13.8532506936693,
118.169495683714)) ;
#160978=CARTESIAN_POINT('Ctrl Pts',(-14.4133403759204,-13.8832318412947,
118.23575164419)) ;
#160979=CARTESIAN_POINT('Ctrl Pts',(-14.3395365456132,-13.8832317458617,
118.259982725815)) ;
#160980=CARTESIAN_POINT('Ctrl Pts',(-14.265732715306,-13.8832316504288,
118.28421380744)) ;
#160981=CARTESIAN_POINT('Ctrl Pts',(-14.2439797697,-13.8532505028034,118.217957846964)) ;
#160982=CARTESIAN_POINT('Ctrl Pts',(-14.2073259241701,-14.1021597581384,
118.070845549194)) ;
#160983=CARTESIAN_POINT('Ctrl Pts',(-14.1888334456528,-14.0547556097992,
118.014520445326)) ;
#160984=CARTESIAN_POINT('Ctrl Pts',(-14.262637269227,-14.0547556877835,
117.990289343193)) ;
#160985=CARTESIAN_POINT('Ctrl Pts',(-14.3364410928012,-14.0547557657678,
117.96605824106)) ;
#160986=CARTESIAN_POINT('Ctrl Pts',(-14.3549335713185,-14.102159914107,
118.022383344929)) ;
#160987=CARTESIAN_POINT('Ctrl Pts',(-14.3734260498358,-14.1495640624461,
118.078708448797)) ;
#160988=CARTESIAN_POINT('Ctrl Pts',(-14.2996222262616,-14.1495639844619,
118.10293955093)) ;
#160989=CARTESIAN_POINT('Ctrl Pts',(-14.2258184026873,-14.1495639064776,
118.127170653063)) ;
#160990=CARTESIAN_POINT('Ctrl Pts',(-14.2073259241701,-14.1021597581384,
118.070845549194)) ;
#160991=CARTESIAN_POINT('Ctrl Pts',(-14.1518319080389,-14.3018608409922,
117.866383830764)) ;
#160992=CARTESIAN_POINT('Ctrl Pts',(-14.1379194094146,-14.240442969134,
117.824008606587)) ;
#160993=CARTESIAN_POINT('Ctrl Pts',(-14.2117232283738,-14.2404430248273,
117.799777490397)) ;
#160994=CARTESIAN_POINT('Ctrl Pts',(-14.285527047333,-14.2404430805207,
117.775546374208)) ;
#160995=CARTESIAN_POINT('Ctrl Pts',(-14.2994395459573,-14.3018609523788,
117.817921598386)) ;
#160996=CARTESIAN_POINT('Ctrl Pts',(-14.3133520445816,-14.3632788242369,
117.860296822564)) ;
#160997=CARTESIAN_POINT('Ctrl Pts',(-14.2395482256223,-14.3632787685436,
117.884527938753)) ;
#160998=CARTESIAN_POINT('Ctrl Pts',(-14.1657444066631,-14.3632787128503,
117.908759054942)) ;
#160999=CARTESIAN_POINT('Ctrl Pts',(-14.1518319080389,-14.3018608409922,
117.866383830764)) ;
#161000=CARTESIAN_POINT('Ctrl Pts',(-14.0821691837154,-14.4384983198451,
117.618753194085)) ;
#161001=CARTESIAN_POINT('Ctrl Pts',(-14.0738329886517,-14.3674483770308,
117.593362490715)) ;
#161002=CARTESIAN_POINT('Ctrl Pts',(-14.147636805446,-14.3674484079295,
117.569131367932)) ;
#161003=CARTESIAN_POINT('Ctrl Pts',(-14.2214406222404,-14.3674484388281,
117.544900245149)) ;
#161004=CARTESIAN_POINT('Ctrl Pts',(-14.2297768173042,-14.4384983816424,
117.570290948519)) ;
#161005=CARTESIAN_POINT('Ctrl Pts',(-14.2381130123679,-14.5095483244567,
117.59568165189)) ;
#161006=CARTESIAN_POINT('Ctrl Pts',(-14.1643091955736,-14.509548293558,
117.619912774673)) ;
#161007=CARTESIAN_POINT('Ctrl Pts',(-14.0905053787792,-14.5095482626594,
117.644143897456)) ;
#161008=CARTESIAN_POINT('Ctrl Pts',(-14.0821691837154,-14.4384983198451,
117.618753194085)) ;
#161009=CARTESIAN_POINT('Ctrl Pts',(-14.0038053646086,-14.5020770602936,
117.344502812886)) ;
#161010=CARTESIAN_POINT('Ctrl Pts',(-14.0016637496419,-14.4264807176174,
117.33797980086)) ;
#161011=CARTESIAN_POINT('Ctrl Pts',(-14.0754675670679,-14.4264807240547,
117.313748680001)) ;
#161012=CARTESIAN_POINT('Ctrl Pts',(-14.1492713844939,-14.426480730492,
117.289517559142)) ;
#161013=CARTESIAN_POINT('Ctrl Pts',(-14.1514129994607,-14.5020770731682,
117.296040571168)) ;
#161014=CARTESIAN_POINT('Ctrl Pts',(-14.1535546144274,-14.5776734158445,
117.302563583194)) ;
#161015=CARTESIAN_POINT('Ctrl Pts',(-14.0797507970014,-14.5776734094072,
117.326794704053)) ;
#161016=CARTESIAN_POINT('Ctrl Pts',(-14.0059469795754,-14.5776734029699,
117.351025824912)) ;
#161017=CARTESIAN_POINT('Ctrl Pts',(-14.0038053646086,-14.5020770602936,
117.344502812886)) ;
#161018=CARTESIAN_POINT('Ctrl Pts',(-13.9237302084394,-14.48777877411,117.065203884427)) ;
#161019=CARTESIAN_POINT('Ctrl Pts',(-13.927908724164,-14.4130666847603,
117.077930970607)) ;
#161020=CARTESIAN_POINT('Ctrl Pts',(-14.0017125440559,-14.413066670136,
117.053699857259)) ;
#161021=CARTESIAN_POINT('Ctrl Pts',(-14.0755163639479,-14.4130666555116,
117.029468743911)) ;
#161022=CARTESIAN_POINT('Ctrl Pts',(-14.0713378482233,-14.4877787448612,
117.01674165773)) ;
#161023=CARTESIAN_POINT('Ctrl Pts',(-14.0671593324987,-14.5624908342109,
117.004014571549)) ;
#161024=CARTESIAN_POINT('Ctrl Pts',(-13.9933555126067,-14.5624908488352,
117.028245684898)) ;
#161025=CARTESIAN_POINT('Ctrl Pts',(-13.9195516927148,-14.5624908634596,
117.052476798246)) ;
#161026=CARTESIAN_POINT('Ctrl Pts',(-13.9237302084394,-14.48777877411,117.065203884427)) ;
#161027=CARTESIAN_POINT('Ctrl Pts',(-13.8479693987333,-14.3970097456745,
116.798993617263)) ;
#161028=CARTESIAN_POINT('Ctrl Pts',(-13.8581774849074,-14.3285220925645,
116.830085802016)) ;
#161029=CARTESIAN_POINT('Ctrl Pts',(-13.9319813090122,-14.3285220617789,
116.805854701499)) ;
#161030=CARTESIAN_POINT('Ctrl Pts',(-14.005785133117,-14.3285220309933,
116.781623600983)) ;
#161031=CARTESIAN_POINT('Ctrl Pts',(-13.995577046943,-14.3970096841033,
116.75053141623)) ;
#161032=CARTESIAN_POINT('Ctrl Pts',(-13.9853689607689,-14.4654973372134,
116.719439231476)) ;
#161033=CARTESIAN_POINT('Ctrl Pts',(-13.9115651366641,-14.465497367999,
116.743670331993)) ;
#161034=CARTESIAN_POINT('Ctrl Pts',(-13.8377613125592,-14.4654973987846,
116.76790143251)) ;
#161035=CARTESIAN_POINT('Ctrl Pts',(-13.8479693987333,-14.3970097456745,
116.798993617263)) ;
#161036=CARTESIAN_POINT('Ctrl Pts',(-13.782799826033,-14.2362612997962,
116.5650573821)) ;
#161037=CARTESIAN_POINT('Ctrl Pts',(-13.7983068769087,-14.1788934065685,
116.612289358194)) ;
#161038=CARTESIAN_POINT('Ctrl Pts',(-13.8721107061698,-14.1788933656858,
116.588058273383)) ;
#161039=CARTESIAN_POINT('Ctrl Pts',(-13.9459145354309,-14.178893324803,
116.563827188572)) ;
#161040=CARTESIAN_POINT('Ctrl Pts',(-13.9304074845553,-14.2362612180308,
116.516595212478)) ;
#161041=CARTESIAN_POINT('Ctrl Pts',(-13.9149004336796,-14.2936291112585,
116.469363236383)) ;
#161042=CARTESIAN_POINT('Ctrl Pts',(-13.8410966044185,-14.2936291521412,
116.493594321195)) ;
#161043=CARTESIAN_POINT('Ctrl Pts',(-13.7672927751574,-14.293629193024,
116.517825406006)) ;
#161044=CARTESIAN_POINT('Ctrl Pts',(-13.782799826033,-14.2362612997962,
116.5650573821)) ;
#161045=CARTESIAN_POINT('Ctrl Pts',(-13.733518100292,-14.0159101115065,
116.379369583749)) ;
#161046=CARTESIAN_POINT('Ctrl Pts',(-13.7532259903904,-13.973840125215,
116.439396638124)) ;
#161047=CARTESIAN_POINT('Ctrl Pts',(-13.8270298252004,-13.97384008191,116.415165570213)) ;
#161048=CARTESIAN_POINT('Ctrl Pts',(-13.9008336600105,-13.973840038605,
116.390934502303)) ;
#161049=CARTESIAN_POINT('Ctrl Pts',(-13.8811257699121,-14.0159100248966,
116.330907447928)) ;
#161050=CARTESIAN_POINT('Ctrl Pts',(-13.8614178798137,-14.0579800111881,
116.270880393553)) ;
#161051=CARTESIAN_POINT('Ctrl Pts',(-13.7876140450037,-14.0579800544931,
116.295111461463)) ;
#161052=CARTESIAN_POINT('Ctrl Pts',(-13.7138102101937,-14.0579800977981,
116.319342529374)) ;
#161053=CARTESIAN_POINT('Ctrl Pts',(-13.733518100292,-14.0159101115065,
116.379369583749)) ;
#161054=CARTESIAN_POINT('Ctrl Pts',(-13.7047590259111,-13.7543350935969,
116.256429298379)) ;
#161055=CARTESIAN_POINT('Ctrl Pts',(-13.7272361212088,-13.7304650573216,
116.324890904835)) ;
#161056=CARTESIAN_POINT('Ctrl Pts',(-13.8010399606436,-13.730465015473,
116.300659851011)) ;
#161057=CARTESIAN_POINT('Ctrl Pts',(-13.8748438000783,-13.7304649736245,
116.276428797187)) ;
#161058=CARTESIAN_POINT('Ctrl Pts',(-13.8523667047806,-13.7543350098997,
116.20796719073)) ;
#161059=CARTESIAN_POINT('Ctrl Pts',(-13.8298896094828,-13.778205046175,
116.139505584273)) ;
#161060=CARTESIAN_POINT('Ctrl Pts',(-13.7560857700481,-13.7782050880236,
116.163736638098)) ;
#161061=CARTESIAN_POINT('Ctrl Pts',(-13.6822819306134,-13.7782051298721,
116.187967691922)) ;
#161062=CARTESIAN_POINT('Ctrl Pts',(-13.7047590259111,-13.7543350935969,
116.256429298379)) ;
#161063=CARTESIAN_POINT('Ctrl Pts',(-13.699032750653,-13.4665595551094,
116.203361929234)) ;
#161064=CARTESIAN_POINT('Ctrl Pts',(-13.7226811442359,-13.4627465020412,
116.275391121082)) ;
#161065=CARTESIAN_POINT('Ctrl Pts',(-13.7964849874278,-13.4627464684725,
116.251160078701)) ;
#161066=CARTESIAN_POINT('Ctrl Pts',(-13.8702888306197,-13.4627464349037,
116.22692903632)) ;
#161067=CARTESIAN_POINT('Ctrl Pts',(-13.8466404370368,-13.4665594879718,
116.154899844473)) ;
#161068=CARTESIAN_POINT('Ctrl Pts',(-13.822992043454,-13.4703725410399,
116.082870652625)) ;
#161069=CARTESIAN_POINT('Ctrl Pts',(-13.749188200262,-13.4703725746087,
116.107101695006)) ;
#161070=CARTESIAN_POINT('Ctrl Pts',(-13.6753843570701,-13.4703726081775,
116.131332737386)) ;
#161071=CARTESIAN_POINT('Ctrl Pts',(-13.699032750653,-13.4665595551094,
116.203361929234)) ;
#161072=CARTESIAN_POINT('Ctrl Pts',(-13.7175768117472,-13.1776643244991,
116.224521765399)) ;
#161073=CARTESIAN_POINT('Ctrl Pts',(-13.7406970529322,-13.1940170948714,
116.294942290125)) ;
#161074=CARTESIAN_POINT('Ctrl Pts',(-13.8145008983678,-13.1940170691323,
116.270711254578)) ;
#161075=CARTESIAN_POINT('Ctrl Pts',(-13.8883047438033,-13.1940170433932,
116.246480219032)) ;
#161076=CARTESIAN_POINT('Ctrl Pts',(-13.8651845026183,-13.1776642730209,
116.176059694306)) ;
#161077=CARTESIAN_POINT('Ctrl Pts',(-13.8420642614332,-13.1613115026485,
116.10563916958)) ;
#161078=CARTESIAN_POINT('Ctrl Pts',(-13.7682604159977,-13.1613115283877,
116.129870205127)) ;
#161079=CARTESIAN_POINT('Ctrl Pts',(-13.6944565705621,-13.1613115541268,
116.154101240673)) ;
#161080=CARTESIAN_POINT('Ctrl Pts',(-13.7175768117472,-13.1776643244991,
116.224521765399)) ;
#161081=CARTESIAN_POINT('Ctrl Pts',(-13.7598364090687,-12.90467088677,116.317749177515)) ;
#161082=CARTESIAN_POINT('Ctrl Pts',(-13.7807753175707,-12.9401099840166,
116.381525714689)) ;
#161083=CARTESIAN_POINT('Ctrl Pts',(-13.8545791638935,-12.9401099680248,
116.357294681845)) ;
#161084=CARTESIAN_POINT('Ctrl Pts',(-13.9283830102164,-12.9401099520331,
116.333063649001)) ;
#161085=CARTESIAN_POINT('Ctrl Pts',(-13.9074441017143,-12.9046708547865,
116.269287111826)) ;
#161086=CARTESIAN_POINT('Ctrl Pts',(-13.8865051932123,-12.86923175754,116.205510574652)) ;
#161087=CARTESIAN_POINT('Ctrl Pts',(-13.8127013468894,-12.8692317735317,
116.229741607496)) ;
#161088=CARTESIAN_POINT('Ctrl Pts',(-13.7388975005666,-12.8692317895235,
116.253972640341)) ;
#161089=CARTESIAN_POINT('Ctrl Pts',(-13.7598364090687,-12.90467088677,116.317749177515)) ;
#161090=CARTESIAN_POINT('Ctrl Pts',(-13.8234518415385,-12.6688603640825,
116.476089051097)) ;
#161091=CARTESIAN_POINT('Ctrl Pts',(-13.8407134383904,-12.7208184006723,
116.528665090186)) ;
#161092=CARTESIAN_POINT('Ctrl Pts',(-13.9145172844529,-12.7208183925847,
116.504434056549)) ;
#161093=CARTESIAN_POINT('Ctrl Pts',(-13.9883211305155,-12.7208183844972,
116.480203022912)) ;
#161094=CARTESIAN_POINT('Ctrl Pts',(-13.9710595336636,-12.6688603479075,
116.427626983823)) ;
#161095=CARTESIAN_POINT('Ctrl Pts',(-13.9537979368117,-12.6169023113178,
116.375050944734)) ;
#161096=CARTESIAN_POINT('Ctrl Pts',(-13.8799940907491,-12.6169023194053,
116.399281978371)) ;
#161097=CARTESIAN_POINT('Ctrl Pts',(-13.8061902446866,-12.6169023274928,
116.423513012008)) ;
#161098=CARTESIAN_POINT('Ctrl Pts',(-13.8234518415385,-12.6688603640825,
116.476089051097)) ;
#161099=CARTESIAN_POINT('Ctrl Pts',(-13.9049557333608,-12.48602188738,116.688787580776)) ;
#161100=CARTESIAN_POINT('Ctrl Pts',(-13.9172879290513,-12.5508253721629,
116.726349459155)) ;
#161101=CARTESIAN_POINT('Ctrl Pts',(-13.9910917739091,-12.5508253699932,
116.702118421849)) ;
#161102=CARTESIAN_POINT('Ctrl Pts',(-14.0648956187668,-12.5508253678235,
116.677887384542)) ;
#161103=CARTESIAN_POINT('Ctrl Pts',(-14.0525634230762,-12.4860218830405,
116.640325506162)) ;
#161104=CARTESIAN_POINT('Ctrl Pts',(-14.0402312273857,-12.4212183982575,
116.602763627783)) ;
#161105=CARTESIAN_POINT('Ctrl Pts',(-13.966427382528,-12.4212184004273,
116.62699466509)) ;
#161106=CARTESIAN_POINT('Ctrl Pts',(-13.8926235376703,-12.421218402597,
116.651225702396)) ;
#161107=CARTESIAN_POINT('Ctrl Pts',(-13.9049557333608,-12.48602188738,116.688787580776)) ;
#161108=CARTESIAN_POINT('Ctrl Pts',(-13.9989576689692,-12.3704601308902,
116.939602004027)) ;
#161109=CARTESIAN_POINT('Ctrl Pts',(-14.0054791232532,-12.4434303508523,
116.95946530155)) ;
#161110=CARTESIAN_POINT('Ctrl Pts',(-14.0792829667969,-12.4434303510562,
116.935234260241)) ;
#161111=CARTESIAN_POINT('Ctrl Pts',(-14.1530868103407,-12.4434303512601,
116.911003218932)) ;
#161112=CARTESIAN_POINT('Ctrl Pts',(-14.1465653560567,-12.370460131298,
116.891139921409)) ;
#161113=CARTESIAN_POINT('Ctrl Pts',(-14.1400439017728,-12.297489911336,
116.871276623886)) ;
#161114=CARTESIAN_POINT('Ctrl Pts',(-14.066240058229,-12.2974899111321,
116.895507665195)) ;
#161115=CARTESIAN_POINT('Ctrl Pts',(-13.9924362146853,-12.2974899109282,
116.919738706504)) ;
#161116=CARTESIAN_POINT('Ctrl Pts',(-13.9989576689692,-12.3704601308902,
116.939602004027)) ;
#161117=CARTESIAN_POINT('Ctrl Pts',(-14.0992273955684,-12.3301504850153,
117.209607062401)) ;
#161118=CARTESIAN_POINT('Ctrl Pts',(-14.0994895791475,-12.406044193393,
117.210405631236)) ;
#161119=CARTESIAN_POINT('Ctrl Pts',(-14.1732934218532,-12.4060441935951,
117.186174587374)) ;
#161120=CARTESIAN_POINT('Ctrl Pts',(-14.2470972645588,-12.4060441937972,
117.161943543513)) ;
#161121=CARTESIAN_POINT('Ctrl Pts',(-14.2468350809797,-12.3301504854195,
117.161144974677)) ;
#161122=CARTESIAN_POINT('Ctrl Pts',(-14.2465728974006,-12.2542567770418,
117.160346405842)) ;
#161123=CARTESIAN_POINT('Ctrl Pts',(-14.1727690546949,-12.2542567768397,
117.184577449703)) ;
#161124=CARTESIAN_POINT('Ctrl Pts',(-14.0989652119893,-12.2542567766376,
117.208808493565)) ;
#161125=CARTESIAN_POINT('Ctrl Pts',(-14.0992273955684,-12.3301504850153,
117.209607062401)) ;
#161126=CARTESIAN_POINT('Ctrl Pts',(-14.1995620772837,-12.3670848663884,
117.479845083354)) ;
#161127=CARTESIAN_POINT('Ctrl Pts',(-14.1935503460574,-12.440512077599,
117.461534319959)) ;
#161128=CARTESIAN_POINT('Ctrl Pts',(-14.2673541883964,-12.4405120766493,
117.43730327498)) ;
#161129=CARTESIAN_POINT('Ctrl Pts',(-14.3411580307353,-12.4405120756996,
117.413072230002)) ;
#161130=CARTESIAN_POINT('Ctrl Pts',(-14.3471697619617,-12.367084864489,
117.431382993397)) ;
#161131=CARTESIAN_POINT('Ctrl Pts',(-14.353181493188,-12.2936576532783,
117.449693756792)) ;
#161132=CARTESIAN_POINT('Ctrl Pts',(-14.279377650849,-12.293657654228,117.47392480177)) ;
#161133=CARTESIAN_POINT('Ctrl Pts',(-14.2055738085101,-12.2936576551777,
117.498155846749)) ;
#161134=CARTESIAN_POINT('Ctrl Pts',(-14.1995620772837,-12.3670848663884,
117.479845083354)) ;
#161135=CARTESIAN_POINT('Ctrl Pts',(-14.2945308343906,-12.4806961242678,
117.733368848111)) ;
#161136=CARTESIAN_POINT('Ctrl Pts',(-14.2826179068284,-12.5462988180666,
117.697083992866)) ;
#161137=CARTESIAN_POINT('Ctrl Pts',(-14.3564217497902,-12.5462988169735,
117.672852949784)) ;
#161138=CARTESIAN_POINT('Ctrl Pts',(-14.4302255927519,-12.5462988158804,
117.648621906703)) ;
#161139=CARTESIAN_POINT('Ctrl Pts',(-14.4421385203141,-12.4806961220815,
117.684906761948)) ;
#161140=CARTESIAN_POINT('Ctrl Pts',(-14.4540514478763,-12.4150934282827,
117.721191617193)) ;
#161141=CARTESIAN_POINT('Ctrl Pts',(-14.3802476049145,-12.4150934293758,
117.745422660274)) ;
#161142=CARTESIAN_POINT('Ctrl Pts',(-14.3064437619527,-12.415093430469,
117.769653703356)) ;
#161143=CARTESIAN_POINT('Ctrl Pts',(-14.2945308343906,-12.4806961242678,
117.733368848111)) ;
#161144=CARTESIAN_POINT('Ctrl Pts',(-14.3760228392886,-12.659847054779,
117.946296624332)) ;
#161145=CARTESIAN_POINT('Ctrl Pts',(-14.3591324954954,-12.7130362017687,
117.894851362404)) ;
#161146=CARTESIAN_POINT('Ctrl Pts',(-14.4329363392067,-12.7130362022566,
117.870620321606)) ;
#161147=CARTESIAN_POINT('Ctrl Pts',(-14.5067401829181,-12.7130362027444,
117.846389280807)) ;
#161148=CARTESIAN_POINT('Ctrl Pts',(-14.5236305267113,-12.6598470557547,
117.897834542735)) ;
#161149=CARTESIAN_POINT('Ctrl Pts',(-14.5405208705045,-12.606657908765,
117.949279804662)) ;
#161150=CARTESIAN_POINT('Ctrl Pts',(-14.4667170267932,-12.6066579082772,
117.973510845461)) ;
#161151=CARTESIAN_POINT('Ctrl Pts',(-14.3929131830819,-12.6066579077893,
117.997741886259)) ;
#161152=CARTESIAN_POINT('Ctrl Pts',(-14.3760228392886,-12.659847054779,
117.946296624332)) ;
#161153=CARTESIAN_POINT('Ctrl Pts',(-14.4406901314542,-12.8944266812495,
118.107719161995)) ;
#161154=CARTESIAN_POINT('Ctrl Pts',(-14.4199951352374,-12.9313139586903,
118.044685542764)) ;
#161155=CARTESIAN_POINT('Ctrl Pts',(-14.4937989797123,-12.9313139638645,
118.020454504291)) ;
#161156=CARTESIAN_POINT('Ctrl Pts',(-14.5676028241872,-12.9313139690387,
117.996223465819)) ;
#161157=CARTESIAN_POINT('Ctrl Pts',(-14.5882978204039,-12.8944266915978,
118.05925708505)) ;
#161158=CARTESIAN_POINT('Ctrl Pts',(-14.6089928166207,-12.8575394141569,
118.122290704281)) ;
#161159=CARTESIAN_POINT('Ctrl Pts',(-14.5351889721458,-12.8575394089827,
118.146521742754)) ;
#161160=CARTESIAN_POINT('Ctrl Pts',(-14.4613851276709,-12.8575394038086,
118.170752781227)) ;
#161161=CARTESIAN_POINT('Ctrl Pts',(-14.4406901314542,-12.8944266812495,
118.107719161995)) ;
#161162=CARTESIAN_POINT('Ctrl Pts',(-14.4837690484985,-13.1656332510844,
118.203535687924)) ;
#161163=CARTESIAN_POINT('Ctrl Pts',(-14.4607685127247,-13.183637429578,
118.13347976731)) ;
#161164=CARTESIAN_POINT('Ctrl Pts',(-14.5345723571586,-13.1836374410536,
118.109248728713)) ;
#161165=CARTESIAN_POINT('Ctrl Pts',(-14.6083762015924,-13.1836374525291,
118.085017690115)) ;
#161166=CARTESIAN_POINT('Ctrl Pts',(-14.6313767373662,-13.1656332740355,
118.155073610728)) ;
#161167=CARTESIAN_POINT('Ctrl Pts',(-14.65437727314,-13.1476290955419,118.225129531342)) ;
#161168=CARTESIAN_POINT('Ctrl Pts',(-14.5805734287061,-13.1476290840664,
118.24936056994)) ;
#161169=CARTESIAN_POINT('Ctrl Pts',(-14.5067695842722,-13.1476290725908,
118.273591608538)) ;
#161170=CARTESIAN_POINT('Ctrl Pts',(-14.4837690484985,-13.1656332510844,
118.203535687924)) ;
#161171=CARTESIAN_POINT('Ctrl Pts',(-14.5033674776862,-13.455130793988,
118.227791066086)) ;
#161172=CARTESIAN_POINT('Ctrl Pts',(-14.479698496056,-13.4529475727115,
118.155699167379)) ;
#161173=CARTESIAN_POINT('Ctrl Pts',(-14.5535023394862,-13.452947591497,
118.131468125724)) ;
#161174=CARTESIAN_POINT('Ctrl Pts',(-14.6273061829163,-13.4529476102826,
118.107237084069)) ;
#161175=CARTESIAN_POINT('Ctrl Pts',(-14.6509751645465,-13.4551308315591,
118.179328982776)) ;
#161176=CARTESIAN_POINT('Ctrl Pts',(-14.6746441461766,-13.4573140528355,
118.251420881482)) ;
#161177=CARTESIAN_POINT('Ctrl Pts',(-14.6008403027464,-13.45731403405,118.275651923137)) ;
#161178=CARTESIAN_POINT('Ctrl Pts',(-14.5270364593163,-13.4573140152645,
118.299882964792)) ;
#161179=CARTESIAN_POINT('Ctrl Pts',(-14.5033674776862,-13.455130793988,
118.227791066086)) ;
#161180=CARTESIAN_POINT('Ctrl Pts',(-14.4986092754277,-13.7427936624919,
118.177758141915)) ;
#161181=CARTESIAN_POINT('Ctrl Pts',(-14.4759736082191,-13.7205220170914,
118.108813552378)) ;
#161182=CARTESIAN_POINT('Ctrl Pts',(-14.549777449295,-13.7205220434154,
118.084582503552)) ;
#161183=CARTESIAN_POINT('Ctrl Pts',(-14.6235812903709,-13.7205220697394,
118.060351454727)) ;
#161184=CARTESIAN_POINT('Ctrl Pts',(-14.6462169575795,-13.7427937151399,
118.129296044264)) ;
#161185=CARTESIAN_POINT('Ctrl Pts',(-14.6688526247881,-13.7650653605404,
118.198240633801)) ;
#161186=CARTESIAN_POINT('Ctrl Pts',(-14.5950487837123,-13.7650653342164,
118.222471682627)) ;
#161187=CARTESIAN_POINT('Ctrl Pts',(-14.5212449426364,-13.7650653078924,
118.246702731452)) ;
#161188=CARTESIAN_POINT('Ctrl Pts',(-14.4986092754277,-13.7427936624919,
118.177758141915)) ;
#161189=CARTESIAN_POINT('Ctrl Pts',(-14.4707221810934,-14.0059776158613,
118.057435006683)) ;
#161190=CARTESIAN_POINT('Ctrl Pts',(-14.4507331312598,-13.9652981717702,
117.996551586788)) ;
#161191=CARTESIAN_POINT('Ctrl Pts',(-14.5245369689501,-13.9652982015733,
117.97232052765)) ;
#161192=CARTESIAN_POINT('Ctrl Pts',(-14.5983408066405,-13.9652982313764,
117.948089468513)) ;
#161193=CARTESIAN_POINT('Ctrl Pts',(-14.6183298564741,-14.0059776754674,
118.008972888409)) ;
#161194=CARTESIAN_POINT('Ctrl Pts',(-14.6383189063077,-14.0466571195585,
118.069856308304)) ;
#161195=CARTESIAN_POINT('Ctrl Pts',(-14.5645150686173,-14.0466570897554,
118.094087367441)) ;
#161196=CARTESIAN_POINT('Ctrl Pts',(-14.4907112309269,-14.0466570599524,
118.118318426579)) ;
#161197=CARTESIAN_POINT('Ctrl Pts',(-14.4707221810934,-14.0059776158613,
118.057435006683)) ;
#161198=CARTESIAN_POINT('Ctrl Pts',(-14.422360755841,-14.2279037819529,
117.874652010575)) ;
#161199=CARTESIAN_POINT('Ctrl Pts',(-14.4064536010254,-14.1716706622332,
117.826201384463)) ;
#161200=CARTESIAN_POINT('Ctrl Pts',(-14.4802574344402,-14.1716706921349,
117.801970312303)) ;
#161201=CARTESIAN_POINT('Ctrl Pts',(-14.5540612678551,-14.1716707220365,
117.777739240143)) ;
#161202=CARTESIAN_POINT('Ctrl Pts',(-14.5699684226707,-14.2279038417561,
117.826189866255)) ;
#161203=CARTESIAN_POINT('Ctrl Pts',(-14.5858755774864,-14.2841369614758,
117.874640492367)) ;
#161204=CARTESIAN_POINT('Ctrl Pts',(-14.5120717440715,-14.2841369315741,
117.898871564527)) ;
#161205=CARTESIAN_POINT('Ctrl Pts',(-14.4382679106566,-14.2841369016725,
117.923102636686)) ;
#161206=CARTESIAN_POINT('Ctrl Pts',(-14.422360755841,-14.2279037819529,
117.874652010575)) ;
#161207=CARTESIAN_POINT('Ctrl Pts',(-14.3575106947756,-14.3919406672911,
117.641551257708)) ;
#161208=CARTESIAN_POINT('Ctrl Pts',(-14.3468444592662,-14.3241730854154,
117.609063626374)) ;
#161209=CARTESIAN_POINT('Ctrl Pts',(-14.4206482878016,-14.3241731099825,
117.584832539352)) ;
#161210=CARTESIAN_POINT('Ctrl Pts',(-14.494452116337,-14.3241731345496,
117.560601452331)) ;
#161211=CARTESIAN_POINT('Ctrl Pts',(-14.5051183518464,-14.3919407164252,
117.593089083665)) ;
#161212=CARTESIAN_POINT('Ctrl Pts',(-14.5157845873559,-14.4597082983009,
117.625576714999)) ;
#161213=CARTESIAN_POINT('Ctrl Pts',(-14.4419807588204,-14.4597082737338,
117.649807802021)) ;
#161214=CARTESIAN_POINT('Ctrl Pts',(-14.368176930285,-14.4597082491667,
117.674038889043)) ;
#161215=CARTESIAN_POINT('Ctrl Pts',(-14.3575106947756,-14.3919406672911,
117.641551257708)) ;
#161216=CARTESIAN_POINT('Ctrl Pts',(-14.2822303298045,-14.4855253459423,
117.376890300863)) ;
#161217=CARTESIAN_POINT('Ctrl Pts',(-14.2775365285705,-14.4111261442654,
117.36259374083)) ;
#161218=CARTESIAN_POINT('Ctrl Pts',(-14.3513403532585,-14.4111261567896,
117.33836264209)) ;
#161219=CARTESIAN_POINT('Ctrl Pts',(-14.4251441779466,-14.4111261693137,
117.31413154335)) ;
#161220=CARTESIAN_POINT('Ctrl Pts',(-14.4298379791805,-14.4855253709906,
117.328428103382)) ;
#161221=CARTESIAN_POINT('Ctrl Pts',(-14.4345317804145,-14.5599245726675,
117.342724663414)) ;
#161222=CARTESIAN_POINT('Ctrl Pts',(-14.3607279557265,-14.5599245601434,
117.366955762154)) ;
#161223=CARTESIAN_POINT('Ctrl Pts',(-14.2869241310384,-14.5599245476192,
117.391186860895)) ;
#161224=CARTESIAN_POINT('Ctrl Pts',(-14.2822303298045,-14.4855253459423,
117.376890300863)) ;
#161225=CARTESIAN_POINT('Ctrl Pts',(-14.2019505143216,-14.5029122651219,
117.09684616291)) ;
#161226=CARTESIAN_POINT('Ctrl Pts',(-14.203589948758,-14.4271913157213,
117.101839617036)) ;
#161227=CARTESIAN_POINT('Ctrl Pts',(-14.2773937703637,-14.4271913111352,
117.077608508907)) ;
#161228=CARTESIAN_POINT('Ctrl Pts',(-14.3511975919692,-14.427191306549,
117.053377400778)) ;
#161229=CARTESIAN_POINT('Ctrl Pts',(-14.3495581575327,-14.5029122559496,
117.048383946652)) ;
#161230=CARTESIAN_POINT('Ctrl Pts',(-14.3479187230963,-14.5786332053501,
117.043390492526)) ;
#161231=CARTESIAN_POINT('Ctrl Pts',(-14.2741149014907,-14.5786332099363,
117.067621600655)) ;
#161232=CARTESIAN_POINT('Ctrl Pts',(-14.2003110798851,-14.5786332145224,
117.091852708784)) ;
#161233=CARTESIAN_POINT('Ctrl Pts',(-14.2019505143216,-14.5029122651219,
117.09684616291)) ;
#161234=CARTESIAN_POINT('Ctrl Pts',(-14.1238906002577,-14.4429567945224,
116.823764513881)) ;
#161235=CARTESIAN_POINT('Ctrl Pts',(-14.131713252239,-14.3713125211074,
116.847591051117)) ;
#161236=CARTESIAN_POINT('Ctrl Pts',(-14.2055170730593,-14.3713124959872,
116.823359940596)) ;
#161237=CARTESIAN_POINT('Ctrl Pts',(-14.2793208938797,-14.371312470867,
116.799128830075)) ;
#161238=CARTESIAN_POINT('Ctrl Pts',(-14.2714982418984,-14.4429567442819,
116.77530229284)) ;
#161239=CARTESIAN_POINT('Ctrl Pts',(-14.2636755899171,-14.5146010176969,
116.751475755604)) ;
#161240=CARTESIAN_POINT('Ctrl Pts',(-14.1898717690967,-14.5146010428171,
116.775706866125)) ;
#161241=CARTESIAN_POINT('Ctrl Pts',(-14.1160679482764,-14.5146010679373,
116.799937976645)) ;
#161242=CARTESIAN_POINT('Ctrl Pts',(-14.1238906002577,-14.4429567945224,
116.823764513881)) ;
#161243=CARTESIAN_POINT('Ctrl Pts',(-14.0534400115056,-14.3088313127917,
116.573580387455)) ;
#161244=CARTESIAN_POINT('Ctrl Pts',(-14.0669293704049,-14.2464468463962,
116.614666799803)) ;
#161245=CARTESIAN_POINT('Ctrl Pts',(-14.1407331920325,-14.2464467981566,
116.590435691741)) ;
#161246=CARTESIAN_POINT('Ctrl Pts',(-14.2145370136601,-14.2464467499169,
116.566204583679)) ;
#161247=CARTESIAN_POINT('Ctrl Pts',(-14.2010476547608,-14.3088312163124,
116.525118171332)) ;
#161248=CARTESIAN_POINT('Ctrl Pts',(-14.1875582958615,-14.3712156827079,
116.484031758984)) ;
#161249=CARTESIAN_POINT('Ctrl Pts',(-14.1137544742339,-14.3712157309476,
116.508262867046)) ;
#161250=CARTESIAN_POINT('Ctrl Pts',(-14.0399506526063,-14.3712157791872,
116.532493975107)) ;
#161251=CARTESIAN_POINT('Ctrl Pts',(-14.0534400115056,-14.3088313127917,
116.573580387455)) ;
#161252=CARTESIAN_POINT('Ctrl Pts',(-13.9973344587926,-14.1118280044828,
116.36732016952)) ;
#161253=CARTESIAN_POINT('Ctrl Pts',(-14.0154923901431,-14.0631071534286,
116.422626300394)) ;
#161254=CARTESIAN_POINT('Ctrl Pts',(-14.0892962154004,-14.0631070839309,
116.398395203387)) ;
#161255=CARTESIAN_POINT('Ctrl Pts',(-14.1631000406576,-14.0631070144332,
116.374164106381)) ;
#161256=CARTESIAN_POINT('Ctrl Pts',(-14.1449421093071,-14.1118278654874,
116.318857975507)) ;
#161257=CARTESIAN_POINT('Ctrl Pts',(-14.1267841779565,-14.1605487165416,
116.263551844633)) ;
#161258=CARTESIAN_POINT('Ctrl Pts',(-14.0529803526993,-14.1605487860393,
116.28778294164)) ;
#161259=CARTESIAN_POINT('Ctrl Pts',(-13.979176527442,-14.160548855537,116.312014038646)) ;
#161260=CARTESIAN_POINT('Ctrl Pts',(-13.9973344587926,-14.1118280044828,
116.36732016952)) ;
#161261=CARTESIAN_POINT('Ctrl Pts',(-13.9596840563562,-13.8633524569287,
116.216996890361)) ;
#161262=CARTESIAN_POINT('Ctrl Pts',(-13.9812347707687,-13.8319077248758,
116.282636891145)) ;
#161263=CARTESIAN_POINT('Ctrl Pts',(-14.055038601653,-13.8319076363894,
116.258405811277)) ;
#161264=CARTESIAN_POINT('Ctrl Pts',(-14.1288424325373,-13.8319075479029,
116.23417473141)) ;
#161265=CARTESIAN_POINT('Ctrl Pts',(-14.1072917181249,-13.8633522799557,
116.168534730626)) ;
#161266=CARTESIAN_POINT('Ctrl Pts',(-14.0857410037124,-13.8947970120086,
116.102894729843)) ;
#161267=CARTESIAN_POINT('Ctrl Pts',(-14.0119371728281,-13.894797100495,
116.12712580971)) ;
#161268=CARTESIAN_POINT('Ctrl Pts',(-13.9381333419438,-13.8947971889815,
116.151356889577)) ;
#161269=CARTESIAN_POINT('Ctrl Pts',(-13.9596840563562,-13.8633524569287,
116.216996890361)) ;
#161270=CARTESIAN_POINT('Ctrl Pts',(-13.9444872281656,-13.5856086171591,
116.135434675017)) ;
#161271=CARTESIAN_POINT('Ctrl Pts',(-13.967860187308,-13.5735093381459,
116.206624939297)) ;
#161272=CARTESIAN_POINT('Ctrl Pts',(-14.0416640258029,-13.5735092387167,
116.18239388261)) ;
#161273=CARTESIAN_POINT('Ctrl Pts',(-14.1154678642979,-13.5735091392875,
116.158162825924)) ;
#161274=CARTESIAN_POINT('Ctrl Pts',(-14.0920949051554,-13.5856084183006,
116.086972561643)) ;
#161275=CARTESIAN_POINT('Ctrl Pts',(-14.068721946013,-13.5977076973138,
116.015782297363)) ;
#161276=CARTESIAN_POINT('Ctrl Pts',(-13.9949181075181,-13.597707796743,
116.04001335405)) ;
#161277=CARTESIAN_POINT('Ctrl Pts',(-13.9211142690232,-13.5977078961722,
116.064244410736)) ;
#161278=CARTESIAN_POINT('Ctrl Pts',(-13.9444872281656,-13.5856086171591,
116.135434675017)) ;
#161279=CARTESIAN_POINT('Ctrl Pts',(-13.9531206776375,-13.29429050433,116.126236655127)) ;
#161280=CARTESIAN_POINT('Ctrl Pts',(-13.9766595960887,-13.3025120940468,
116.197932404757)) ;
#161281=CARTESIAN_POINT('Ctrl Pts',(-14.0504634431248,-13.3025119902988,
116.173701374085)) ;
#161282=CARTESIAN_POINT('Ctrl Pts',(-14.1242672901609,-13.3025118865508,
116.149470343414)) ;
#161283=CARTESIAN_POINT('Ctrl Pts',(-14.1007283717097,-13.294290296834,
116.077774593784)) ;
#161284=CARTESIAN_POINT('Ctrl Pts',(-14.0771894532585,-13.2860687071171,
116.006078844155)) ;
#161285=CARTESIAN_POINT('Ctrl Pts',(-14.0033856062224,-13.2860688108651,
116.030309874826)) ;
#161286=CARTESIAN_POINT('Ctrl Pts',(-13.9295817591863,-13.2860689146131,
116.054540905498)) ;
#161287=CARTESIAN_POINT('Ctrl Pts',(-13.9531206776375,-13.29429050433,116.126236655127)) ;
#161288=CARTESIAN_POINT('Ctrl Pts',(-13.9859156053883,-13.0122145331766,
116.19068657179)) ;
#161289=CARTESIAN_POINT('Ctrl Pts',(-14.0079327694877,-13.0401416634717,
116.257747303244)) ;
#161290=CARTESIAN_POINT('Ctrl Pts',(-14.0817366252876,-13.0401415643198,
116.233516299266)) ;
#161291=CARTESIAN_POINT('Ctrl Pts',(-14.1555404810876,-13.0401414651678,
116.209285295287)) ;
#161292=CARTESIAN_POINT('Ctrl Pts',(-14.1335233169882,-13.0122143348728,
116.142224563833)) ;
#161293=CARTESIAN_POINT('Ctrl Pts',(-14.1115061528888,-12.9842872045777,
116.075163832378)) ;
#161294=CARTESIAN_POINT('Ctrl Pts',(-14.0377022970889,-12.9842873037296,
116.099394836357)) ;
#161295=CARTESIAN_POINT('Ctrl Pts',(-13.963898441289,-12.9842874028816,
116.123625840335)) ;
#161296=CARTESIAN_POINT('Ctrl Pts',(-13.9859156053883,-13.0122145331766,
116.19068657179)) ;
#161297=CARTESIAN_POINT('Ctrl Pts',(-14.0414265852797,-12.7583429519339,
116.324206721183)) ;
#161298=CARTESIAN_POINT('Ctrl Pts',(-14.0603365111948,-12.8040356004971,
116.381803306508)) ;
#161299=CARTESIAN_POINT('Ctrl Pts',(-14.1341403750837,-12.8040355143443,
116.357572327168)) ;
#161300=CARTESIAN_POINT('Ctrl Pts',(-14.2079442389726,-12.8040354281915,
116.333341347827)) ;
#161301=CARTESIAN_POINT('Ctrl Pts',(-14.1890343130574,-12.7583427796283,
116.275744762501)) ;
#161302=CARTESIAN_POINT('Ctrl Pts',(-14.1701243871423,-12.7126501310651,
116.218148177176)) ;
#161303=CARTESIAN_POINT('Ctrl Pts',(-14.0963205232534,-12.7126502172179,
116.242379156517)) ;
#161304=CARTESIAN_POINT('Ctrl Pts',(-14.0225166593645,-12.7126503033707,
116.266610135857)) ;
#161305=CARTESIAN_POINT('Ctrl Pts',(-14.0414265852797,-12.7583429519339,
116.324206721183)) ;
#161306=CARTESIAN_POINT('Ctrl Pts',(-14.1163566701285,-12.5522896132778,
116.516904433369)) ;
#161307=CARTESIAN_POINT('Ctrl Pts',(-14.1307984259442,-12.6124359304363,
116.560891693508)) ;
#161308=CARTESIAN_POINT('Ctrl Pts',(-14.2046022962474,-12.6124358649261,
116.536660733704)) ;
#161309=CARTESIAN_POINT('Ctrl Pts',(-14.2784061665505,-12.6124357994159,
116.5124297739)) ;
#161310=CARTESIAN_POINT('Ctrl Pts',(-14.2639644107349,-12.5522894822574,
116.468442513761)) ;
#161311=CARTESIAN_POINT('Ctrl Pts',(-14.2495226549191,-12.4921431650989,
116.424455253623)) ;
#161312=CARTESIAN_POINT('Ctrl Pts',(-14.175718784616,-12.4921432306091,
116.448686213427)) ;
#161313=CARTESIAN_POINT('Ctrl Pts',(-14.1019149143128,-12.4921432961193,
116.47291717323)) ;
#161314=CARTESIAN_POINT('Ctrl Pts',(-14.1163566701285,-12.5522896132778,
116.516904433369)) ;
#161315=CARTESIAN_POINT('Ctrl Pts',(-14.2054208500919,-12.4090180636989,
116.75287655481)) ;
#161316=CARTESIAN_POINT('Ctrl Pts',(-14.2143962414437,-12.4792560944464,
116.78021415077)) ;
#161317=CARTESIAN_POINT('Ctrl Pts',(-14.2882001159623,-12.4792560544209,
116.755983203806)) ;
#161318=CARTESIAN_POINT('Ctrl Pts',(-14.3620039904809,-12.4792560143955,
116.731752256842)) ;
#161319=CARTESIAN_POINT('Ctrl Pts',(-14.3530285991291,-12.409017983648,
116.704414660881)) ;
#161320=CARTESIAN_POINT('Ctrl Pts',(-14.3440532077773,-12.3387799529005,
116.67707706492)) ;
#161321=CARTESIAN_POINT('Ctrl Pts',(-14.2702493332587,-12.3387799929259,
116.701308011885)) ;
#161322=CARTESIAN_POINT('Ctrl Pts',(-14.1964454587401,-12.3387800329514,
116.725538958849)) ;
#161323=CARTESIAN_POINT('Ctrl Pts',(-14.2054208500919,-12.4090180636989,
116.75287655481)) ;
#161324=CARTESIAN_POINT('Ctrl Pts',(-14.3041315741692,-12.3371174607651,
117.018003366661)) ;
#161325=CARTESIAN_POINT('Ctrl Pts',(-14.306963905046,-12.4124801362831,
117.026630191551)) ;
#161326=CARTESIAN_POINT('Ctrl Pts',(-14.3807677810887,-12.4124801245382,
117.002399249229)) ;
#161327=CARTESIAN_POINT('Ctrl Pts',(-14.4545716571313,-12.4124801127933,
116.978168306907)) ;
#161328=CARTESIAN_POINT('Ctrl Pts',(-14.4517393262545,-12.3371174372753,
116.969541482016)) ;
#161329=CARTESIAN_POINT('Ctrl Pts',(-14.4489069953776,-12.2617547617574,
116.960914657126)) ;
#161330=CARTESIAN_POINT('Ctrl Pts',(-14.375103119335,-12.2617547735023,
116.985145599448)) ;
#161331=CARTESIAN_POINT('Ctrl Pts',(-14.3012992432923,-12.2617547852472,
117.009376541771)) ;
#161332=CARTESIAN_POINT('Ctrl Pts',(-14.3041315741692,-12.3371174607651,
117.018003366661)) ;
#161333=CARTESIAN_POINT('Ctrl Pts',(-14.4053499510961,-12.3428658905722,
117.290874128105)) ;
#161334=CARTESIAN_POINT('Ctrl Pts',(-14.40185271617,-12.4179397314328,117.280222116772)) ;
#161335=CARTESIAN_POINT('Ctrl Pts',(-14.4756565910603,-12.4179397474679,
117.25599117094)) ;
#161336=CARTESIAN_POINT('Ctrl Pts',(-14.5494604659506,-12.4179397635031,
117.231760225108)) ;
#161337=CARTESIAN_POINT('Ctrl Pts',(-14.5529577008767,-12.3428659226425,
117.242412236441)) ;
#161338=CARTESIAN_POINT('Ctrl Pts',(-14.5564549358029,-12.267792081782,
117.253064247774)) ;
#161339=CARTESIAN_POINT('Ctrl Pts',(-14.4826510609126,-12.2677920657468,
117.277295193606)) ;
#161340=CARTESIAN_POINT('Ctrl Pts',(-14.4088471860223,-12.2677920497116,
117.301526139438)) ;
#161341=CARTESIAN_POINT('Ctrl Pts',(-14.4053499510961,-12.3428658905722,
117.290874128105)) ;
#161342=CARTESIAN_POINT('Ctrl Pts',(-14.5030362331871,-12.4257351119528,
117.55290734156)) ;
#161343=CARTESIAN_POINT('Ctrl Pts',(-14.4934481825595,-12.4951358678153,
117.523703688264)) ;
#161344=CARTESIAN_POINT('Ctrl Pts',(-14.5672520537253,-12.4951359082695,
117.499472731088)) ;
#161345=CARTESIAN_POINT('Ctrl Pts',(-14.6410559248911,-12.4951359487237,
117.475241773911)) ;
#161346=CARTESIAN_POINT('Ctrl Pts',(-14.6506439755188,-12.4257351928613,
117.504445427208)) ;
#161347=CARTESIAN_POINT('Ctrl Pts',(-14.6602320261464,-12.3563344369988,
117.533649080504)) ;
#161348=CARTESIAN_POINT('Ctrl Pts',(-14.5864281549806,-12.3563343965446,
117.557880037681)) ;
#161349=CARTESIAN_POINT('Ctrl Pts',(-14.5126242838148,-12.3563343560904,
117.582110994857)) ;
#161350=CARTESIAN_POINT('Ctrl Pts',(-14.5030362331871,-12.4257351119528,
117.55290734156)) ;
#161351=CARTESIAN_POINT('Ctrl Pts',(-14.5904621270827,-12.5790185234623,
117.783826332769)) ;
#161352=CARTESIAN_POINT('Ctrl Pts',(-14.5754876103016,-12.6378213476739,
117.738216372584)) ;
#161353=CARTESIAN_POINT('Ctrl Pts',(-14.6492914760003,-12.6378214074388,
117.713985398756)) ;
#161354=CARTESIAN_POINT('Ctrl Pts',(-14.7230953416989,-12.6378214672038,
117.689754424927)) ;
#161355=CARTESIAN_POINT('Ctrl Pts',(-14.7380698584799,-12.5790186429921,
117.735364385112)) ;
#161356=CARTESIAN_POINT('Ctrl Pts',(-14.753044375261,-12.5202158187805,
117.780974345297)) ;
#161357=CARTESIAN_POINT('Ctrl Pts',(-14.6792405095624,-12.5202157590156,
117.805205319126)) ;
#161358=CARTESIAN_POINT('Ctrl Pts',(-14.6054366438637,-12.5202156992507,
117.829436292955)) ;
#161359=CARTESIAN_POINT('Ctrl Pts',(-14.5904621270827,-12.5790185234623,
117.783826332769)) ;
#161360=CARTESIAN_POINT('Ctrl Pts',(-14.6629652552051,-12.7940406828703,
117.969008479269)) ;
#161361=CARTESIAN_POINT('Ctrl Pts',(-14.6436437278103,-12.837920143464,
117.910158225998)) ;
#161362=CARTESIAN_POINT('Ctrl Pts',(-14.717447586395,-12.8379202140664,
117.885927230502)) ;
#161363=CARTESIAN_POINT('Ctrl Pts',(-14.7912514449796,-12.8379202846688,
117.861696235005)) ;
#161364=CARTESIAN_POINT('Ctrl Pts',(-14.8105729723744,-12.7940408240752,
117.920546488276)) ;
#161365=CARTESIAN_POINT('Ctrl Pts',(-14.8298944997692,-12.7501613634815,
117.979396741547)) ;
#161366=CARTESIAN_POINT('Ctrl Pts',(-14.7560906411845,-12.7501612928791,
118.003627737044)) ;
#161367=CARTESIAN_POINT('Ctrl Pts',(-14.6822867825999,-12.7501612222767,
118.02785873254)) ;
#161368=CARTESIAN_POINT('Ctrl Pts',(-14.6629652552051,-12.7940406828703,
117.969008479269)) ;
#161369=CARTESIAN_POINT('Ctrl Pts',(-14.7149782729242,-13.0518842131347,
118.092091883262)) ;
#161370=CARTESIAN_POINT('Ctrl Pts',(-14.6927274213406,-13.0778272755866,
118.02431938104)) ;
#161371=CARTESIAN_POINT('Ctrl Pts',(-14.7665312729268,-13.0778273508396,
118.000088364228)) ;
#161372=CARTESIAN_POINT('Ctrl Pts',(-14.840335124513,-13.0778274260925,
117.975857347415)) ;
#161373=CARTESIAN_POINT('Ctrl Pts',(-14.8625859760966,-13.0518843636406,
118.043629849637)) ;
#161374=CARTESIAN_POINT('Ctrl Pts',(-14.8848368276802,-13.0259413011886,
118.111402351858)) ;
#161375=CARTESIAN_POINT('Ctrl Pts',(-14.811032976094,-13.0259412259357,
118.135633368671)) ;
#161376=CARTESIAN_POINT('Ctrl Pts',(-14.7372291245078,-13.0259411506828,
118.159864385484)) ;
#161377=CARTESIAN_POINT('Ctrl Pts',(-14.7149782729242,-13.0518842131347,
118.092091883262)) ;
#161378=CARTESIAN_POINT('Ctrl Pts',(-14.7443671066665,-13.3370763555055,
118.146092536195)) ;
#161379=CARTESIAN_POINT('Ctrl Pts',(-14.7207654994872,-13.343146769627,
118.074205850219)) ;
#161380=CARTESIAN_POINT('Ctrl Pts',(-14.7945693443435,-13.3431468412151,
118.049974812908)) ;
#161381=CARTESIAN_POINT('Ctrl Pts',(-14.8683731891997,-13.3431469128033,
118.025743775596)) ;
#161382=CARTESIAN_POINT('Ctrl Pts',(-14.891974796379,-13.3370764986818,
118.097630461573)) ;
#161383=CARTESIAN_POINT('Ctrl Pts',(-14.9155764035582,-13.3310060845603,
118.16951714755)) ;
#161384=CARTESIAN_POINT('Ctrl Pts',(-14.8417725587019,-13.3310060129721,
118.193748184861)) ;
#161385=CARTESIAN_POINT('Ctrl Pts',(-14.7679687138457,-13.3310059413839,
118.217979222172)) ;
#161386=CARTESIAN_POINT('Ctrl Pts',(-14.7443671066665,-13.3370763555055,
118.146092536195)) ;
#161387=CARTESIAN_POINT('Ctrl Pts',(-14.7494764883566,-13.6270297095458,
118.126281327732)) ;
#161388=CARTESIAN_POINT('Ctrl Pts',(-14.7262144515455,-13.6128647269904,
118.055428918166)) ;
#161389=CARTESIAN_POINT('Ctrl Pts',(-14.8000182908552,-13.6128647900771,
118.031197863962)) ;
#161390=CARTESIAN_POINT('Ctrl Pts',(-14.8738221301649,-13.6128648531639,
118.006966809757)) ;
#161391=CARTESIAN_POINT('Ctrl Pts',(-14.897084166976,-13.6270298357193,
118.077819219322)) ;
#161392=CARTESIAN_POINT('Ctrl Pts',(-14.9203462037872,-13.6411948182747,
118.148671628887)) ;
#161393=CARTESIAN_POINT('Ctrl Pts',(-14.8465423644775,-13.6411947551879,
118.172902683092)) ;
#161394=CARTESIAN_POINT('Ctrl Pts',(-14.7727385251678,-13.6411946921012,
118.197133737297)) ;
#161395=CARTESIAN_POINT('Ctrl Pts',(-14.7494764883566,-13.6270297095458,
118.126281327732)) ;
#161396=CARTESIAN_POINT('Ctrl Pts',(-14.7306708206297,-13.9038567932623,
118.033390708072)) ;
#161397=CARTESIAN_POINT('Ctrl Pts',(-14.7094232936479,-13.8703419963818,
117.968674170216)) ;
#161398=CARTESIAN_POINT('Ctrl Pts',(-14.7832271292031,-13.8703420447739,
117.944443104575)) ;
#161399=CARTESIAN_POINT('Ctrl Pts',(-14.8570309647582,-13.8703420931661,
117.920212038934)) ;
#161400=CARTESIAN_POINT('Ctrl Pts',(-14.87827849174,-13.9038568900467,117.98492857679)) ;
#161401=CARTESIAN_POINT('Ctrl Pts',(-14.8995260187217,-13.9373716869272,
118.049645114647)) ;
#161402=CARTESIAN_POINT('Ctrl Pts',(-14.8257221831665,-13.9373716385351,
118.073876180288)) ;
#161403=CARTESIAN_POINT('Ctrl Pts',(-14.7519183476114,-13.9373715901429,
118.098107245928)) ;
#161404=CARTESIAN_POINT('Ctrl Pts',(-14.7306708206297,-13.9038567932623,
118.033390708072)) ;
#161405=CARTESIAN_POINT('Ctrl Pts',(-14.690027558541,-14.1447030861545,
117.874109045323)) ;
#161406=CARTESIAN_POINT('Ctrl Pts',(-14.6723199395305,-14.0943210410225,
117.820174495812)) ;
#161407=CARTESIAN_POINT('Ctrl Pts',(-14.7461237732829,-14.0943210744769,
117.79594342468)) ;
#161408=CARTESIAN_POINT('Ctrl Pts',(-14.8199276070354,-14.0943211079313,
117.771712353549)) ;
#161409=CARTESIAN_POINT('Ctrl Pts',(-14.8376352260459,-14.1447031530633,
117.82564690306)) ;
#161410=CARTESIAN_POINT('Ctrl Pts',(-14.8553428450565,-14.1950851981953,
117.879581452572)) ;
#161411=CARTESIAN_POINT('Ctrl Pts',(-14.781539011304,-14.1950851647409,
117.903812523703)) ;
#161412=CARTESIAN_POINT('Ctrl Pts',(-14.7077351775515,-14.1950851312865,
117.928043594835)) ;
#161413=CARTESIAN_POINT('Ctrl Pts',(-14.690027558541,-14.1447030861545,
117.874109045323)) ;
#161414=CARTESIAN_POINT('Ctrl Pts',(-14.6316472186503,-14.332817774621,
117.660971076182)) ;
#161415=CARTESIAN_POINT('Ctrl Pts',(-14.6187199695823,-14.2692250612684,
117.621596762065)) ;
#161416=CARTESIAN_POINT('Ctrl Pts',(-14.6925238028212,-14.2692250813647,
117.597365689369)) ;
#161417=CARTESIAN_POINT('Ctrl Pts',(-14.76632763606,-14.269225101461,117.573134616673)) ;
#161418=CARTESIAN_POINT('Ctrl Pts',(-14.7792548851279,-14.3328178148136,
117.61250893079)) ;
#161419=CARTESIAN_POINT('Ctrl Pts',(-14.7921821341959,-14.3964105281663,
117.651883244906)) ;
#161420=CARTESIAN_POINT('Ctrl Pts',(-14.718378300957,-14.3964105080699,
117.676114317602)) ;
#161421=CARTESIAN_POINT('Ctrl Pts',(-14.6445744677182,-14.3964104879736,
117.700345390298)) ;
#161422=CARTESIAN_POINT('Ctrl Pts',(-14.6316472186503,-14.332817774621,
117.660971076182)) ;
#161423=CARTESIAN_POINT('Ctrl Pts',(-14.5597455784243,-14.45646682902,117.406433016193)) ;
#161424=CARTESIAN_POINT('Ctrl Pts',(-14.5525544833958,-14.3841439170352,
117.384530101578)) ;
#161425=CARTESIAN_POINT('Ctrl Pts',(-14.6263583180638,-14.3841439249686,
117.360299033234)) ;
#161426=CARTESIAN_POINT('Ctrl Pts',(-14.7001621527318,-14.3841439329019,
117.336067964891)) ;
#161427=CARTESIAN_POINT('Ctrl Pts',(-14.7073532477603,-14.4564668448866,
117.357970879507)) ;
#161428=CARTESIAN_POINT('Ctrl Pts',(-14.7145443427888,-14.5287897568713,
117.379873794122)) ;
#161429=CARTESIAN_POINT('Ctrl Pts',(-14.6407405081208,-14.528789748938,
117.404104862465)) ;
#161430=CARTESIAN_POINT('Ctrl Pts',(-14.5669366734528,-14.5287897410047,
117.428335930808)) ;
#161431=CARTESIAN_POINT('Ctrl Pts',(-14.5597455784243,-14.45646682902,117.406433016193)) ;
#161432=CARTESIAN_POINT('Ctrl Pts',(-14.4807629365922,-14.5053560860543,
117.130424369544)) ;
#161433=CARTESIAN_POINT('Ctrl Pts',(-14.4798092245676,-14.4295100560536,
117.127519517009)) ;
#161434=CARTESIAN_POINT('Ctrl Pts',(-14.5536130613439,-14.4295100560703,
117.103288455087)) ;
#161435=CARTESIAN_POINT('Ctrl Pts',(-14.6274168981201,-14.429510056087,
117.079057393166)) ;
#161436=CARTESIAN_POINT('Ctrl Pts',(-14.6283706101447,-14.5053560860877,
117.081962245701)) ;
#161437=CARTESIAN_POINT('Ctrl Pts',(-14.6293243221693,-14.5812021160883,
117.084867098236)) ;
#161438=CARTESIAN_POINT('Ctrl Pts',(-14.5555204853931,-14.5812021160717,
117.109098160158)) ;
#161439=CARTESIAN_POINT('Ctrl Pts',(-14.4817166486168,-14.581202116055,
117.133329222079)) ;
#161440=CARTESIAN_POINT('Ctrl Pts',(-14.4807629365922,-14.5053560860543,
117.130424369544)) ;
#161441=CARTESIAN_POINT('Ctrl Pts',(-14.4006764355962,-14.4762759602464,
116.850932976369)) ;
#161442=CARTESIAN_POINT('Ctrl Pts',(-14.4060492486959,-14.4023454887856,
116.867297698424)) ;
#161443=CARTESIAN_POINT('Ctrl Pts',(-14.4798530881773,-14.4023454850915,
116.843066644742)) ;
#161444=CARTESIAN_POINT('Ctrl Pts',(-14.5536569276586,-14.4023454813974,
116.818835591059)) ;
#161445=CARTESIAN_POINT('Ctrl Pts',(-14.5482841145589,-14.4762759528582,
116.802470869005)) ;
#161446=CARTESIAN_POINT('Ctrl Pts',(-14.5429113014591,-14.5502064243191,
116.78610614695)) ;
#161447=CARTESIAN_POINT('Ctrl Pts',(-14.4691074619778,-14.5502064280132,
116.810337200632)) ;
#161448=CARTESIAN_POINT('Ctrl Pts',(-14.3953036224965,-14.5502064317073,
116.834568254315)) ;
#161449=CARTESIAN_POINT('Ctrl Pts',(-14.4006764355962,-14.4762759602464,
116.850932976369)) ;
#161450=CARTESIAN_POINT('Ctrl Pts',(-14.3265390078925,-14.3712943997113,
116.589686458049)) ;
#161451=CARTESIAN_POINT('Ctrl Pts',(-14.3378299538683,-14.3045830394382,
116.624076857841)) ;
#161452=CARTESIAN_POINT('Ctrl Pts',(-14.4116337954084,-14.3045830356426,
116.599845810429)) ;
#161453=CARTESIAN_POINT('Ctrl Pts',(-14.4854376369484,-14.3045830318471,
116.575614763017)) ;
#161454=CARTESIAN_POINT('Ctrl Pts',(-14.4741466909726,-14.3712943921201,
116.541224363225)) ;
#161455=CARTESIAN_POINT('Ctrl Pts',(-14.4628557449968,-14.4380057523932,
116.506833963433)) ;
#161456=CARTESIAN_POINT('Ctrl Pts',(-14.3890519034567,-14.4380057561888,
116.531065010845)) ;
#161457=CARTESIAN_POINT('Ctrl Pts',(-14.3152480619167,-14.4380057599843,
116.555296058257)) ;
#161458=CARTESIAN_POINT('Ctrl Pts',(-14.3265390078925,-14.3712943997113,
116.589686458049)) ;
#161459=CARTESIAN_POINT('Ctrl Pts',(-14.2642291252365,-14.1990455522355,
116.364581017991)) ;
#161460=CARTESIAN_POINT('Ctrl Pts',(-14.2806187025119,-14.1442616573657,
116.414501025975)) ;
#161461=CARTESIAN_POINT('Ctrl Pts',(-14.3544225454209,-14.1442616552479,
116.390269982733)) ;
#161462=CARTESIAN_POINT('Ctrl Pts',(-14.4282263883299,-14.1442616531301,
116.36603893949)) ;
#161463=CARTESIAN_POINT('Ctrl Pts',(-14.4118368110544,-14.1990455479999,
116.316118931507)) ;
#161464=CARTESIAN_POINT('Ctrl Pts',(-14.3954472337789,-14.2538294428697,
116.266198923523)) ;
#161465=CARTESIAN_POINT('Ctrl Pts',(-14.3216433908699,-14.2538294449875,
116.290429966766)) ;
#161466=CARTESIAN_POINT('Ctrl Pts',(-14.247839547961,-14.2538294471053,
116.314661010008)) ;
#161467=CARTESIAN_POINT('Ctrl Pts',(-14.2642291252365,-14.1990455522355,
116.364581017991)) ;
#161468=CARTESIAN_POINT('Ctrl Pts',(-14.2184481514674,-13.969268231171,
116.189542795207)) ;
#161469=CARTESIAN_POINT('Ctrl Pts',(-14.2387958666726,-13.9304471194496,
116.251518652599)) ;
#161470=CARTESIAN_POINT('Ctrl Pts',(-14.312599710417,-13.9304471207081,
116.227287611902)) ;
#161471=CARTESIAN_POINT('Ctrl Pts',(-14.3864035541614,-13.9304471219666,
116.203056571204)) ;
#161472=CARTESIAN_POINT('Ctrl Pts',(-14.3660558389563,-13.9692682336881,
116.141080713812)) ;
#161473=CARTESIAN_POINT('Ctrl Pts',(-14.3457081237511,-14.0080893454095,
116.07910485642)) ;
#161474=CARTESIAN_POINT('Ctrl Pts',(-14.2719042800067,-14.008089344151,
116.103335897118)) ;
#161475=CARTESIAN_POINT('Ctrl Pts',(-14.1981004362623,-14.0080893428925,
116.127566937816)) ;
#161476=CARTESIAN_POINT('Ctrl Pts',(-14.2184481514674,-13.969268231171,
116.189542795207)) ;
#161477=CARTESIAN_POINT('Ctrl Pts',(-14.1938561787033,-13.7012052922517,
116.079239578809)) ;
#161478=CARTESIAN_POINT('Ctrl Pts',(-14.2166839653933,-13.6810448607135,
116.148769333753)) ;
#161479=CARTESIAN_POINT('Ctrl Pts',(-14.2904878090818,-13.6810448639026,
116.124538292885)) ;
#161480=CARTESIAN_POINT('Ctrl Pts',(-14.3642916527704,-13.6810448670916,
116.100307252017)) ;
#161481=CARTESIAN_POINT('Ctrl Pts',(-14.3414638660804,-13.7012052986298,
116.030777497073)) ;
#161482=CARTESIAN_POINT('Ctrl Pts',(-14.3186360793905,-13.7213657301679,
115.961247742129)) ;
#161483=CARTESIAN_POINT('Ctrl Pts',(-14.2448322357019,-13.7213657269789,
115.985478782997)) ;
#161484=CARTESIAN_POINT('Ctrl Pts',(-14.1710283920134,-13.7213657237898,
116.009709823865)) ;
#161485=CARTESIAN_POINT('Ctrl Pts',(-14.1938561787033,-13.7012052922517,
116.079239578809)) ;
#161486=CARTESIAN_POINT('Ctrl Pts',(-14.1927076708075,-13.4115854195081,
116.040169663763)) ;
#161487=CARTESIAN_POINT('Ctrl Pts',(-14.2163857118218,-13.4116194662379,
116.112289156201)) ;
#161488=CARTESIAN_POINT('Ctrl Pts',(-14.2901895551865,-13.4116194689939,
116.088058114347)) ;
#161489=CARTESIAN_POINT('Ctrl Pts',(-14.3639933985512,-13.41161947175,116.063827072493)) ;
#161490=CARTESIAN_POINT('Ctrl Pts',(-14.3403153575369,-13.4115854250202,
115.991707580054)) ;
#161491=CARTESIAN_POINT('Ctrl Pts',(-14.3166373165225,-13.4115513782904,
115.919588087615)) ;
#161492=CARTESIAN_POINT('Ctrl Pts',(-14.2428334731578,-13.4115513755344,
115.94381912947)) ;
#161493=CARTESIAN_POINT('Ctrl Pts',(-14.1690296297931,-13.4115513727784,
115.968050171324)) ;
#161494=CARTESIAN_POINT('Ctrl Pts',(-14.1927076708075,-13.4115854195081,
116.040169663763)) ;
#161495=CARTESIAN_POINT('Ctrl Pts',(-14.2158186831131,-13.1240520278943,
116.075200920001)) ;
#161496=CARTESIAN_POINT('Ctrl Pts',(-14.238649448497,-13.1441635924048,
116.144739747623)) ;
#161497=CARTESIAN_POINT('Ctrl Pts',(-14.3124532917785,-13.144163592711,
116.120508705515)) ;
#161498=CARTESIAN_POINT('Ctrl Pts',(-14.38625713506,-13.1441635930171,116.096277663407)) ;
#161499=CARTESIAN_POINT('Ctrl Pts',(-14.3634263696761,-13.1240520285066,
116.026738835786)) ;
#161500=CARTESIAN_POINT('Ctrl Pts',(-14.3405956042921,-13.103940463996,
115.957200008165)) ;
#161501=CARTESIAN_POINT('Ctrl Pts',(-14.2667917610107,-13.1039404636899,
115.981431050272)) ;
#161502=CARTESIAN_POINT('Ctrl Pts',(-14.1929879177292,-13.1039404633837,
116.00566209238)) ;
#161503=CARTESIAN_POINT('Ctrl Pts',(-14.2158186831131,-13.1240520278943,
116.075200920001)) ;
#161504=CARTESIAN_POINT('Ctrl Pts',(-14.2623847117566,-12.8565945311091,
116.181543563239)) ;
#161505=CARTESIAN_POINT('Ctrl Pts',(-14.2827318296291,-12.895411134357,
116.243517601359)) ;
#161506=CARTESIAN_POINT('Ctrl Pts',(-14.3565356735563,-12.8954111308149,
116.219286561218)) ;
#161507=CARTESIAN_POINT('Ctrl Pts',(-14.4303395174835,-12.8954111272728,
116.195055521077)) ;
#161508=CARTESIAN_POINT('Ctrl Pts',(-14.409992399611,-12.8565945240249,
116.133081482957)) ;
#161509=CARTESIAN_POINT('Ctrl Pts',(-14.3896452817385,-12.817777920777,
116.071107444837)) ;
#161510=CARTESIAN_POINT('Ctrl Pts',(-14.3158414378113,-12.8177779243191,
116.095338484978)) ;
#161511=CARTESIAN_POINT('Ctrl Pts',(-14.2420375938841,-12.8177779278612,
116.119569525119)) ;
#161512=CARTESIAN_POINT('Ctrl Pts',(-14.2623847117566,-12.8565945311091,
116.181543563239)) ;
#161513=CARTESIAN_POINT('Ctrl Pts',(-14.3295805648497,-12.6299321000607,
116.350826699486)) ;
#161514=CARTESIAN_POINT('Ctrl Pts',(-14.345997626373,-12.6846316848106,
116.400830420177)) ;
#161515=CARTESIAN_POINT('Ctrl Pts',(-14.4198014716913,-12.6846316781894,
116.376599384273)) ;
#161516=CARTESIAN_POINT('Ctrl Pts',(-14.4936053170096,-12.6846316715683,
116.352368348369)) ;
#161517=CARTESIAN_POINT('Ctrl Pts',(-14.4771882554863,-12.6299320868185,
116.302364627678)) ;
#161518=CARTESIAN_POINT('Ctrl Pts',(-14.460771193963,-12.5752325020687,
116.252360906988)) ;
#161519=CARTESIAN_POINT('Ctrl Pts',(-14.3869673486447,-12.5752325086898,
116.276591942892)) ;
#161520=CARTESIAN_POINT('Ctrl Pts',(-14.3131635033265,-12.5752325153109,
116.300822978795)) ;
#161521=CARTESIAN_POINT('Ctrl Pts',(-14.3295805648497,-12.6299321000607,
116.350826699486)) ;
#161522=CARTESIAN_POINT('Ctrl Pts',(-14.4139535876279,-12.458754218581,
116.572235100756)) ;
#161523=CARTESIAN_POINT('Ctrl Pts',(-14.425239560756,-12.5254858902144,
116.60661035424)) ;
#161524=CARTESIAN_POINT('Ctrl Pts',(-14.4990434086302,-12.5254858817945,
116.582379326121)) ;
#161525=CARTESIAN_POINT('Ctrl Pts',(-14.5728472565044,-12.5254858733746,
116.558148298002)) ;
#161526=CARTESIAN_POINT('Ctrl Pts',(-14.5615612833762,-12.4587542017412,
116.523773044517)) ;
#161527=CARTESIAN_POINT('Ctrl Pts',(-14.550275310248,-12.3920225301078,
116.489397791033)) ;
#161528=CARTESIAN_POINT('Ctrl Pts',(-14.4764714623738,-12.3920225385277,
116.513628819152)) ;
#161529=CARTESIAN_POINT('Ctrl Pts',(-14.4026676144997,-12.3920225469476,
116.537859847271)) ;
#161530=CARTESIAN_POINT('Ctrl Pts',(-14.4139535876279,-12.458754218581,
116.572235100756)) ;
#161531=CARTESIAN_POINT('Ctrl Pts',(-14.5094836498744,-12.3569969390507,
116.827772100287)) ;
#161532=CARTESIAN_POINT('Ctrl Pts',(-14.5148490608815,-12.4309301429408,
116.844114276972)) ;
#161533=CARTESIAN_POINT('Ctrl Pts',(-14.5886529115489,-12.4309301369064,
116.819883257361)) ;
#161534=CARTESIAN_POINT('Ctrl Pts',(-14.6624567622163,-12.430930130872,
116.795652237749)) ;
#161535=CARTESIAN_POINT('Ctrl Pts',(-14.6570913512092,-12.356996926982,
116.779310061064)) ;
#161536=CARTESIAN_POINT('Ctrl Pts',(-14.6517259402021,-12.283063723092,
116.762967884378)) ;
#161537=CARTESIAN_POINT('Ctrl Pts',(-14.5779220895347,-12.2830637291264,
116.787198903989)) ;
#161538=CARTESIAN_POINT('Ctrl Pts',(-14.5041182388673,-12.2830637351607,
116.811429923601)) ;
#161539=CARTESIAN_POINT('Ctrl Pts',(-14.5094836498744,-12.3569969390507,
116.827772100287)) ;
#161540=CARTESIAN_POINT('Ctrl Pts',(-14.6106904064239,-12.3311725454961,
117.10048536176)) ;
#161541=CARTESIAN_POINT('Ctrl Pts',(-14.6097327538528,-12.4070160661621,
117.097568507183)) ;
#161542=CARTESIAN_POINT('Ctrl Pts',(-14.6835366075574,-12.4070160669481,
117.073337496822)) ;
#161543=CARTESIAN_POINT('Ctrl Pts',(-14.7573404612619,-12.4070160677341,
117.049106486462)) ;
#161544=CARTESIAN_POINT('Ctrl Pts',(-14.7582981138329,-12.3311725470681,
117.052023341038)) ;
#161545=CARTESIAN_POINT('Ctrl Pts',(-14.759255766404,-12.2553290264021,
117.054940195615)) ;
#161546=CARTESIAN_POINT('Ctrl Pts',(-14.6854519126995,-12.2553290256161,
117.079171205975)) ;
#161547=CARTESIAN_POINT('Ctrl Pts',(-14.611648058995,-12.2553290248301,
117.103402216336)) ;
#161548=CARTESIAN_POINT('Ctrl Pts',(-14.6106904064239,-12.3311725454961,
117.10048536176)) ;
#161549=CARTESIAN_POINT('Ctrl Pts',(-14.7103650458112,-12.3830921654557,
117.368691273652)) ;
#161550=CARTESIAN_POINT('Ctrl Pts',(-14.7031789791306,-12.4554200435771,
117.3468036748)) ;
#161551=CARTESIAN_POINT('Ctrl Pts',(-14.7769828347535,-12.4554200554495,
117.322572670283)) ;
#161552=CARTESIAN_POINT('Ctrl Pts',(-14.8507866903763,-12.4554200673219,
117.298341665765)) ;
#161553=CARTESIAN_POINT('Ctrl Pts',(-14.8579727570569,-12.3830921892004,
117.320229264616)) ;
#161554=CARTESIAN_POINT('Ctrl Pts',(-14.8651588237375,-12.310764311079,
117.342116863467)) ;
#161555=CARTESIAN_POINT('Ctrl Pts',(-14.7913549681146,-12.3107642992066,
117.366347867985)) ;
#161556=CARTESIAN_POINT('Ctrl Pts',(-14.7175511124917,-12.3107642873342,
117.390578872503)) ;
#161557=CARTESIAN_POINT('Ctrl Pts',(-14.7103650458112,-12.3830921654557,
117.368691273652)) ;
#161558=CARTESIAN_POINT('Ctrl Pts',(-14.8029787361383,-12.5097082549453,
117.615209351864)) ;
#161559=CARTESIAN_POINT('Ctrl Pts',(-14.790052001847,-12.5733006688363,
117.575836605912)) ;
#161560=CARTESIAN_POINT('Ctrl Pts',(-14.8638558585522,-12.5733006960963,
117.55160560469)) ;
#161561=CARTESIAN_POINT('Ctrl Pts',(-14.9376597152575,-12.5733007233563,
117.527374603469)) ;
#161562=CARTESIAN_POINT('Ctrl Pts',(-14.9505864495488,-12.5097083094653,
117.566747349422)) ;
#161563=CARTESIAN_POINT('Ctrl Pts',(-14.9635131838401,-12.4461158955744,
117.606120095374)) ;
#161564=CARTESIAN_POINT('Ctrl Pts',(-14.8897093271349,-12.4461158683144,
117.630351096595)) ;
#161565=CARTESIAN_POINT('Ctrl Pts',(-14.8159054704297,-12.4461158410544,
117.654582097816)) ;
#161566=CARTESIAN_POINT('Ctrl Pts',(-14.8029787361383,-12.5097082549453,
117.615209351864)) ;
#161567=CARTESIAN_POINT('Ctrl Pts',(-14.8815949767115,-12.6999655173835,
117.819379893254)) ;
#161568=CARTESIAN_POINT('Ctrl Pts',(-14.8638908473129,-12.7503658770991,
117.765455972768)) ;
#161569=CARTESIAN_POINT('Ctrl Pts',(-14.9376947027237,-12.7503659198469,
117.741224967604)) ;
#161570=CARTESIAN_POINT('Ctrl Pts',(-15.0114985581344,-12.7503659625947,
117.71699396244)) ;
#161571=CARTESIAN_POINT('Ctrl Pts',(-15.029202687533,-12.699965602879,117.770917882926)) ;
#161572=CARTESIAN_POINT('Ctrl Pts',(-15.0469068169316,-12.6495652431633,
117.824841803413)) ;
#161573=CARTESIAN_POINT('Ctrl Pts',(-14.9731029615209,-12.6495652004156,
117.849072808577)) ;
#161574=CARTESIAN_POINT('Ctrl Pts',(-14.8992991061101,-12.6495651576678,
117.873303813741)) ;
#161575=CARTESIAN_POINT('Ctrl Pts',(-14.8815949767115,-12.6999655173835,
117.819379893254)) ;
#161576=CARTESIAN_POINT('Ctrl Pts',(-14.9425172204992,-12.9431519741363,
117.969375033027)) ;
#161577=CARTESIAN_POINT('Ctrl Pts',(-14.9212698376286,-12.9766466266446,
117.904658934347)) ;
#161578=CARTESIAN_POINT('Ctrl Pts',(-14.9950736903222,-12.9766466864281,
117.880427920907)) ;
#161579=CARTESIAN_POINT('Ctrl Pts',(-15.0688775430157,-12.9766467462115,
117.856196907467)) ;
#161580=CARTESIAN_POINT('Ctrl Pts',(-15.0901249258863,-12.9431520937032,
117.920913006147)) ;
#161581=CARTESIAN_POINT('Ctrl Pts',(-15.1113723087568,-12.9096574411949,
117.985629104826)) ;
#161582=CARTESIAN_POINT('Ctrl Pts',(-15.0375684560633,-12.9096573814114,
118.009860118267)) ;
#161583=CARTESIAN_POINT('Ctrl Pts',(-14.9637646033697,-12.9096573216279,
118.034091131707)) ;
#161584=CARTESIAN_POINT('Ctrl Pts',(-14.9425172204992,-12.9431519741363,
117.969375033027)) ;
#161585=CARTESIAN_POINT('Ctrl Pts',(-14.9812992054159,-13.2187420743147,
118.052168315938)) ;
#161586=CARTESIAN_POINT('Ctrl Pts',(-14.9580445655685,-13.233044020348,
117.981338436508)) ;
#161587=CARTESIAN_POINT('Ctrl Pts',(-15.0318484133956,-13.2330440926295,
117.957107408245)) ;
#161588=CARTESIAN_POINT('Ctrl Pts',(-15.1056522612227,-13.2330441649111,
117.932876379983)) ;
#161589=CARTESIAN_POINT('Ctrl Pts',(-15.1289069010701,-13.2187422188778,
118.003706259413)) ;
#161590=CARTESIAN_POINT('Ctrl Pts',(-15.1521615409175,-13.2044402728445,
118.074536138843)) ;
#161591=CARTESIAN_POINT('Ctrl Pts',(-15.0783576930904,-13.204440200563,
118.098767167106)) ;
#161592=CARTESIAN_POINT('Ctrl Pts',(-15.0045538452633,-13.2044401282814,
118.122998195368)) ;
#161593=CARTESIAN_POINT('Ctrl Pts',(-14.9812992054159,-13.2187420743147,
118.052168315938)) ;
#161594=CARTESIAN_POINT('Ctrl Pts',(-14.9963500333539,-13.5111774969548,
118.062342681364)) ;
#161595=CARTESIAN_POINT('Ctrl Pts',(-14.9727486985028,-13.505083397222,
117.990456825067)) ;
#161596=CARTESIAN_POINT('Ctrl Pts',(-15.046552539892,-13.5050834796266,
117.966225777196)) ;
#161597=CARTESIAN_POINT('Ctrl Pts',(-15.1203563812812,-13.5050835620312,
117.941994729324)) ;
#161598=CARTESIAN_POINT('Ctrl Pts',(-15.1439577161323,-13.511177661764,
118.013880585621)) ;
#161599=CARTESIAN_POINT('Ctrl Pts',(-15.1675590509834,-13.5172717614969,
118.085766441919)) ;
#161600=CARTESIAN_POINT('Ctrl Pts',(-15.0937552095942,-13.5172716790923,
118.10999748979)) ;
#161601=CARTESIAN_POINT('Ctrl Pts',(-15.019951368205,-13.5172715966877,
118.134228537661)) ;
#161602=CARTESIAN_POINT('Ctrl Pts',(-14.9963500333539,-13.5111774969548,
118.062342681364)) ;
#161603=CARTESIAN_POINT('Ctrl Pts',(-14.9871457345053,-13.7940494918521,
117.999019373326)) ;
#161604=CARTESIAN_POINT('Ctrl Pts',(-14.9648830646108,-13.7681973144643,
117.931210874597)) ;
#161605=CARTESIAN_POINT('Ctrl Pts',(-15.0386868986759,-13.7681973972875,
117.906979804418)) ;
#161606=CARTESIAN_POINT('Ctrl Pts',(-15.112490732741,-13.7681974801107,
117.882748734239)) ;
#161607=CARTESIAN_POINT('Ctrl Pts',(-15.1347534026356,-13.7940496574985,
117.950557232967)) ;
#161608=CARTESIAN_POINT('Ctrl Pts',(-15.1570160725302,-13.8199018348862,
118.018365731696)) ;
#161609=CARTESIAN_POINT('Ctrl Pts',(-15.0832122384651,-13.819901752063,
118.042596801875)) ;
#161610=CARTESIAN_POINT('Ctrl Pts',(-15.0094084043999,-13.8199016692398,
118.066827872054)) ;
#161611=CARTESIAN_POINT('Ctrl Pts',(-14.9871457345053,-13.7940494918521,
117.999019373326)) ;
#161612=CARTESIAN_POINT('Ctrl Pts',(-14.9548742901699,-14.0529110285333,
117.865026253004)) ;
#161613=CARTESIAN_POINT('Ctrl Pts',(-14.9355706975565,-14.0089483158053,
117.806230626371)) ;
#161614=CARTESIAN_POINT('Ctrl Pts',(-15.0093745237244,-14.0089483935527,
117.781999532138)) ;
#161615=CARTESIAN_POINT('Ctrl Pts',(-15.0831783498923,-14.0089484713001,
117.757768437906)) ;
#161616=CARTESIAN_POINT('Ctrl Pts',(-15.1024819425057,-14.0529111840282,
117.816564064539)) ;
#161617=CARTESIAN_POINT('Ctrl Pts',(-15.1217855351191,-14.0968738967562,
117.875359691172)) ;
#161618=CARTESIAN_POINT('Ctrl Pts',(-15.0479817089512,-14.0968738190088,
117.899590785405)) ;
#161619=CARTESIAN_POINT('Ctrl Pts',(-14.9741778827833,-14.0968737412614,
117.923821879638)) ;
#161620=CARTESIAN_POINT('Ctrl Pts',(-14.9548742901699,-14.0529110285333,
117.865026253004)) ;
#161621=CARTESIAN_POINT('Ctrl Pts',(-14.9032500009219,-14.2634870650102,
117.672503574574)) ;
#161622=CARTESIAN_POINT('Ctrl Pts',(-14.8882526660298,-14.2047586746315,
117.62682411422)) ;
#161623=CARTESIAN_POINT('Ctrl Pts',(-14.9620564854445,-14.2047587372463,
117.602592999418)) ;
#161624=CARTESIAN_POINT('Ctrl Pts',(-15.0358603048591,-14.204758799861,
117.578361884616)) ;
#161625=CARTESIAN_POINT('Ctrl Pts',(-15.0508576397512,-14.2634871902397,
117.62404134497)) ;
#161626=CARTESIAN_POINT('Ctrl Pts',(-15.0658549746433,-14.3222155806184,
117.669720805323)) ;
#161627=CARTESIAN_POINT('Ctrl Pts',(-14.9920511552287,-14.3222155180036,
117.693951920125)) ;
#161628=CARTESIAN_POINT('Ctrl Pts',(-14.918247335814,-14.3222154553889,
117.718183034927)) ;
#161629=CARTESIAN_POINT('Ctrl Pts',(-14.9032500009219,-14.2634870650102,
117.672503574574)) ;
#161630=CARTESIAN_POINT('Ctrl Pts',(-14.8361924144871,-14.4148461022599,
117.432794192959)) ;
#161631=CARTESIAN_POINT('Ctrl Pts',(-14.8265885875091,-14.3454644446965,
117.40354248755)) ;
#161632=CARTESIAN_POINT('Ctrl Pts',(-14.9003924014718,-14.3454644862781,
117.379311356142)) ;
#161633=CARTESIAN_POINT('Ctrl Pts',(-14.9741962154345,-14.3454645278597,
117.355080224734)) ;
#161634=CARTESIAN_POINT('Ctrl Pts',(-14.9838000424125,-14.414846185423,
117.384331930144)) ;
#161635=CARTESIAN_POINT('Ctrl Pts',(-14.9934038693905,-14.4842278429864,
117.413583635553)) ;
#161636=CARTESIAN_POINT('Ctrl Pts',(-14.9196000554278,-14.4842278014048,
117.437814766961)) ;
#161637=CARTESIAN_POINT('Ctrl Pts',(-14.8457962414651,-14.4842277598232,
117.462045898369)) ;
#161638=CARTESIAN_POINT('Ctrl Pts',(-14.8361924144871,-14.4148461022599,
117.432794192959)) ;
#161639=CARTESIAN_POINT('Ctrl Pts',(-14.7594134311292,-14.494780073978,
117.16350011444)) ;
#161640=CARTESIAN_POINT('Ctrl Pts',(-14.7558891680831,-14.4197159016166,
117.152765779888)) ;
#161641=CARTESIAN_POINT('Ctrl Pts',(-14.8296929787699,-14.4197159169921,
117.128534638503)) ;
#161642=CARTESIAN_POINT('Ctrl Pts',(-14.9034967894568,-14.4197159323676,
117.104303497117)) ;
#161643=CARTESIAN_POINT('Ctrl Pts',(-14.9070210525029,-14.4947801047291,
117.115037831669)) ;
#161644=CARTESIAN_POINT('Ctrl Pts',(-14.910545315549,-14.5698442770905,
117.125772166221)) ;
#161645=CARTESIAN_POINT('Ctrl Pts',(-14.8367415048621,-14.5698442617149,
117.150003307607)) ;
#161646=CARTESIAN_POINT('Ctrl Pts',(-14.7629376941752,-14.5698442463394,
117.174234448992)) ;
#161647=CARTESIAN_POINT('Ctrl Pts',(-14.7594134311292,-14.494780073978,
117.16350011444)) ;
#161648=CARTESIAN_POINT('Ctrl Pts',(-14.6788165394104,-14.4974507314962,
116.882424493313)) ;
#161649=CARTESIAN_POINT('Ctrl Pts',(-14.6816504035553,-14.4220890720825,
116.891055988342)) ;
#161650=CARTESIAN_POINT('Ctrl Pts',(-14.7554542135507,-14.4220890586317,
116.866824844851)) ;
#161651=CARTESIAN_POINT('Ctrl Pts',(-14.8292580235462,-14.4220890451809,
116.842593701359)) ;
#161652=CARTESIAN_POINT('Ctrl Pts',(-14.8264241594014,-14.4974507045946,
116.83396220633)) ;
#161653=CARTESIAN_POINT('Ctrl Pts',(-14.8235902952566,-14.5728123640084,
116.825330711301)) ;
#161654=CARTESIAN_POINT('Ctrl Pts',(-14.7497864852611,-14.5728123774592,
116.849561854792)) ;
#161655=CARTESIAN_POINT('Ctrl Pts',(-14.6759826752656,-14.57281239091,116.873792998283)) ;
#161656=CARTESIAN_POINT('Ctrl Pts',(-14.6788165394104,-14.4974507314962,
116.882424493313)) ;
#161657=CARTESIAN_POINT('Ctrl Pts',(-14.6018098242213,-14.4229495346006,
116.612531368624)) ;
#161658=CARTESIAN_POINT('Ctrl Pts',(-14.6107555369899,-14.3526782474262,
116.639778568426)) ;
#161659=CARTESIAN_POINT('Ctrl Pts',(-14.6845593491738,-14.3526782058987,
116.615547431601)) ;
#161660=CARTESIAN_POINT('Ctrl Pts',(-14.7583631613577,-14.3526781643712,
116.591316294775)) ;
#161661=CARTESIAN_POINT('Ctrl Pts',(-14.7494174485891,-14.4229494515456,
116.564069094973)) ;
#161662=CARTESIAN_POINT('Ctrl Pts',(-14.7404717358206,-14.49322073872,116.53682189517)) ;
#161663=CARTESIAN_POINT('Ctrl Pts',(-14.6666679236366,-14.4932207802475,
116.561053031996)) ;
#161664=CARTESIAN_POINT('Ctrl Pts',(-14.5928641114527,-14.493220821775,
116.585284168822)) ;
#161665=CARTESIAN_POINT('Ctrl Pts',(-14.6018098242213,-14.4229495346006,
116.612531368624)) ;
#161666=CARTESIAN_POINT('Ctrl Pts',(-14.5338249366433,-14.2768020033666,
116.370022693878)) ;
#161667=CARTESIAN_POINT('Ctrl Pts',(-14.5482635939486,-14.2166300695752,
116.414000516451)) ;
#161668=CARTESIAN_POINT('Ctrl Pts',(-14.6220674107796,-14.2166300030693,
116.389769393779)) ;
#161669=CARTESIAN_POINT('Ctrl Pts',(-14.6958712276106,-14.2166299365633,
116.365538271108)) ;
#161670=CARTESIAN_POINT('Ctrl Pts',(-14.6814325703052,-14.2768018703547,
116.321560448536)) ;
#161671=CARTESIAN_POINT('Ctrl Pts',(-14.6669939129999,-14.336973804146,
116.277582625963)) ;
#161672=CARTESIAN_POINT('Ctrl Pts',(-14.5931900961689,-14.336973870652,
116.301813748635)) ;
#161673=CARTESIAN_POINT('Ctrl Pts',(-14.5193862793379,-14.3369739371579,
116.326044871306)) ;
#161674=CARTESIAN_POINT('Ctrl Pts',(-14.5338249366433,-14.2768020033666,
116.370022693878)) ;
#161675=CARTESIAN_POINT('Ctrl Pts',(-14.4805103340185,-14.0672719747909,
116.171945276152)) ;
#161676=CARTESIAN_POINT('Ctrl Pts',(-14.4994313031301,-14.0216384576254,
116.229575497223)) ;
#161677=CARTESIAN_POINT('Ctrl Pts',(-14.5732351268998,-14.0216383725684,
116.205344395686)) ;
#161678=CARTESIAN_POINT('Ctrl Pts',(-14.6470389506695,-14.0216382875114,
116.181113294149)) ;
#161679=CARTESIAN_POINT('Ctrl Pts',(-14.628117981558,-14.067271804677,116.123483073077)) ;
#161680=CARTESIAN_POINT('Ctrl Pts',(-14.6091970124464,-14.1129053218425,
116.065852852006)) ;
#161681=CARTESIAN_POINT('Ctrl Pts',(-14.5353931886767,-14.1129054068995,
116.090083953543)) ;
#161682=CARTESIAN_POINT('Ctrl Pts',(-14.4615893649069,-14.1129054919565,
116.11431505508)) ;
#161683=CARTESIAN_POINT('Ctrl Pts',(-14.4805103340185,-14.0672719747909,
116.171945276152)) ;
#161684=CARTESIAN_POINT('Ctrl Pts',(-14.4472092133991,-13.8140437794069,
116.035263380737)) ;
#161685=CARTESIAN_POINT('Ctrl Pts',(-14.4692127086449,-13.786022349902,
116.102282479007)) ;
#161686=CARTESIAN_POINT('Ctrl Pts',(-14.5430165403838,-13.7860222533108,
116.078051401742)) ;
#161687=CARTESIAN_POINT('Ctrl Pts',(-14.6168203721226,-13.7860221567197,
116.053820324478)) ;
#161688=CARTESIAN_POINT('Ctrl Pts',(-14.5948168768768,-13.8140435862246,
115.986801226207)) ;
#161689=CARTESIAN_POINT('Ctrl Pts',(-14.5728133816309,-13.8420650157295,
115.919782127937)) ;
#161690=CARTESIAN_POINT('Ctrl Pts',(-14.4990095498921,-13.8420651123206,
115.944013205202)) ;
#161691=CARTESIAN_POINT('Ctrl Pts',(-14.4252057181532,-13.8420652089118,
115.968244282466)) ;
#161692=CARTESIAN_POINT('Ctrl Pts',(-14.4472092133991,-13.8140437794069,
116.035263380737)) ;
#161693=CARTESIAN_POINT('Ctrl Pts',(-14.4362486432515,-13.5305545368903,
115.96633944488)) ;
#161694=CARTESIAN_POINT('Ctrl Pts',(-14.4597857472441,-13.5222834200997,
116.038029667866)) ;
#161695=CARTESIAN_POINT('Ctrl Pts',(-14.5335895875712,-13.5222833210965,
116.01379861676)) ;
#161696=CARTESIAN_POINT('Ctrl Pts',(-14.6073934278984,-13.5222832220932,
115.989567565655)) ;
#161697=CARTESIAN_POINT('Ctrl Pts',(-14.5838563239058,-13.5305543388838,
115.917877342668)) ;
#161698=CARTESIAN_POINT('Ctrl Pts',(-14.5603192199132,-13.5388254556744,
115.846187119682)) ;
#161699=CARTESIAN_POINT('Ctrl Pts',(-14.486515379586,-13.5388255546776,
115.870418170788)) ;
#161700=CARTESIAN_POINT('Ctrl Pts',(-14.4127115392589,-13.5388256536809,
115.894649221894)) ;
#161701=CARTESIAN_POINT('Ctrl Pts',(-14.4362486432515,-13.5305545368903,
115.96633944488)) ;
#161702=CARTESIAN_POINT('Ctrl Pts',(-14.449486240473,-13.2400469135056,
115.971266296655)) ;
#161703=CARTESIAN_POINT('Ctrl Pts',(-14.4728667368979,-13.2520460162367,
116.042479518172)) ;
#161704=CARTESIAN_POINT('Ctrl Pts',(-14.5466705853202,-13.2520459225966,
116.018248491723)) ;
#161705=CARTESIAN_POINT('Ctrl Pts',(-14.6204744337425,-13.2520458289565,
115.994017465274)) ;
#161706=CARTESIAN_POINT('Ctrl Pts',(-14.5970939373175,-13.2400467262255,
115.922804243756)) ;
#161707=CARTESIAN_POINT('Ctrl Pts',(-14.5737134408926,-13.2280476234944,
115.851591022239)) ;
#161708=CARTESIAN_POINT('Ctrl Pts',(-14.4999095924703,-13.2280477171344,
115.875822048688)) ;
#161709=CARTESIAN_POINT('Ctrl Pts',(-14.426105744048,-13.2280478107745,
115.900053075137)) ;
#161710=CARTESIAN_POINT('Ctrl Pts',(-14.449486240473,-13.2400469135056,
115.971266296655)) ;
#161711=CARTESIAN_POINT('Ctrl Pts',(-14.4868824566312,-12.9607801917685,
116.04957346963)) ;
#161712=CARTESIAN_POINT('Ctrl Pts',(-14.5084238912217,-12.9922952069383,
116.115185205403)) ;
#161713=CARTESIAN_POINT('Ctrl Pts',(-14.5822277463875,-12.9922951270176,
116.090954199492)) ;
#161714=CARTESIAN_POINT('Ctrl Pts',(-14.6560316015532,-12.9922950470968,
116.066723193582)) ;
#161715=CARTESIAN_POINT('Ctrl Pts',(-14.6344901669627,-12.960780031927,
116.00111145781)) ;
#161716=CARTESIAN_POINT('Ctrl Pts',(-14.6129487323722,-12.9292650167572,
115.935499722038)) ;
#161717=CARTESIAN_POINT('Ctrl Pts',(-14.5391448772065,-12.929265096678,
115.959730727948)) ;
#161718=CARTESIAN_POINT('Ctrl Pts',(-14.4653410220408,-12.9292651765987,
115.983961733858)) ;
#161719=CARTESIAN_POINT('Ctrl Pts',(-14.4868824566312,-12.9607801917685,
116.04957346963)) ;
#161720=CARTESIAN_POINT('Ctrl Pts',(-14.5461400633249,-12.7157522020321,
116.194666581357)) ;
#161721=CARTESIAN_POINT('Ctrl Pts',(-14.5643090647105,-12.7644222769748,
116.250006429608)) ;
#161722=CARTESIAN_POINT('Ctrl Pts',(-14.6381129248079,-12.7644222146516,
116.225775438719)) ;
#161723=CARTESIAN_POINT('Ctrl Pts',(-14.7119167849052,-12.7644221523283,
116.20154444783)) ;
#161724=CARTESIAN_POINT('Ctrl Pts',(-14.6937477835196,-12.7157520773856,
116.146204599579)) ;
#161725=CARTESIAN_POINT('Ctrl Pts',(-14.675578782134,-12.6670820024428,
116.090864751328)) ;
#161726=CARTESIAN_POINT('Ctrl Pts',(-14.6017749220366,-12.6670820647661,
116.115095742217)) ;
#161727=CARTESIAN_POINT('Ctrl Pts',(-14.5279710619392,-12.6670821270893,
116.139326733106)) ;
#161728=CARTESIAN_POINT('Ctrl Pts',(-14.5461400633249,-12.7157522020321,
116.194666581357)) ;
#161729=CARTESIAN_POINT('Ctrl Pts',(-14.6240444846692,-12.5205021117526,
116.396478689841)) ;
#161730=CARTESIAN_POINT('Ctrl Pts',(-14.6375357271718,-12.5828779756765,
116.437570839145)) ;
#161731=CARTESIAN_POINT('Ctrl Pts',(-14.7113395899329,-12.5828779339693,
116.413339856369)) ;
#161732=CARTESIAN_POINT('Ctrl Pts',(-14.785143452694,-12.582877892262,116.389108873593)) ;
#161733=CARTESIAN_POINT('Ctrl Pts',(-14.7716522101914,-12.5205020283381,
116.348016724289)) ;
#161734=CARTESIAN_POINT('Ctrl Pts',(-14.7581609676887,-12.4581261644142,
116.306924574986)) ;
#161735=CARTESIAN_POINT('Ctrl Pts',(-14.6843571049276,-12.4581262061215,
116.331155557762)) ;
#161736=CARTESIAN_POINT('Ctrl Pts',(-14.6105532421665,-12.4581262478287,
116.355386540537)) ;
#161737=CARTESIAN_POINT('Ctrl Pts',(-14.6240444846692,-12.5205021117526,
116.396478689841)) ;
#161738=CARTESIAN_POINT('Ctrl Pts',(-14.7155078962198,-12.3896091910669,
116.639659815513)) ;
#161739=CARTESIAN_POINT('Ctrl Pts',(-14.7233661315669,-12.4612182427459,
116.663594733761)) ;
#161740=CARTESIAN_POINT('Ctrl Pts',(-14.7971699949239,-12.4612182215385,
116.6393637528)) ;
#161741=CARTESIAN_POINT('Ctrl Pts',(-14.8709738582809,-12.461218200331,
116.615132771839)) ;
#161742=CARTESIAN_POINT('Ctrl Pts',(-14.8631156229337,-12.389609148652,
116.591197853591)) ;
#161743=CARTESIAN_POINT('Ctrl Pts',(-14.8552573875865,-12.318000096973,
116.567262935343)) ;
#161744=CARTESIAN_POINT('Ctrl Pts',(-14.7814535242296,-12.3180001181804,
116.591493916304)) ;
#161745=CARTESIAN_POINT('Ctrl Pts',(-14.7076496608726,-12.3180001393879,
116.615724897265)) ;
#161746=CARTESIAN_POINT('Ctrl Pts',(-14.7155078962198,-12.3896091910669,
116.639659815513)) ;
#161747=CARTESIAN_POINT('Ctrl Pts',(-14.8155283401331,-12.3322116649338,
116.908678402663)) ;
#161748=CARTESIAN_POINT('Ctrl Pts',(-14.817152276422,-12.4079372852091,
116.913624651688)) ;
#161749=CARTESIAN_POINT('Ctrl Pts',(-14.8909561377333,-12.4079372823359,
116.889393664496)) ;
#161750=CARTESIAN_POINT('Ctrl Pts',(-14.9647599990446,-12.4079372794628,
116.865162677304)) ;
#161751=CARTESIAN_POINT('Ctrl Pts',(-14.9631360627557,-12.3322116591875,
116.860216428279)) ;
#161752=CARTESIAN_POINT('Ctrl Pts',(-14.9615121264668,-12.2564860389122,
116.855270179255)) ;
#161753=CARTESIAN_POINT('Ctrl Pts',(-14.8877082651555,-12.2564860417854,
116.879501166446)) ;
#161754=CARTESIAN_POINT('Ctrl Pts',(-14.8139044038442,-12.2564860446585,
116.903732153638)) ;
#161755=CARTESIAN_POINT('Ctrl Pts',(-14.8155283401331,-12.3322116649338,
116.908678402663)) ;
#161756=CARTESIAN_POINT('Ctrl Pts',(-14.9160696924354,-12.3526193896652,
117.179651593861)) ;
#161757=CARTESIAN_POINT('Ctrl Pts',(-14.9114057877124,-12.4270343562084,
117.165446093574)) ;
#161758=CARTESIAN_POINT('Ctrl Pts',(-14.9852096465855,-12.4270343671983,
117.141215098956)) ;
#161759=CARTESIAN_POINT('Ctrl Pts',(-15.0590135054586,-12.4270343781882,
117.116984104338)) ;
#161760=CARTESIAN_POINT('Ctrl Pts',(-15.0636774101816,-12.352619411645,
117.131189604624)) ;
#161761=CARTESIAN_POINT('Ctrl Pts',(-15.0683413149046,-12.2782044451017,
117.145395104911)) ;
#161762=CARTESIAN_POINT('Ctrl Pts',(-14.9945374560315,-12.2782044341118,
117.169626099529)) ;
#161763=CARTESIAN_POINT('Ctrl Pts',(-14.9207335971584,-12.2782044231219,
117.193857094147)) ;
#161764=CARTESIAN_POINT('Ctrl Pts',(-14.9160696924354,-12.3526193896652,
117.179651593861)) ;
#161765=CARTESIAN_POINT('Ctrl Pts',(-15.0126074976825,-12.4495335034968,
117.438097138294)) ;
#161766=CARTESIAN_POINT('Ctrl Pts',(-15.0019325703686,-12.5172950398371,
117.405583032877)) ;
#161767=CARTESIAN_POINT('Ctrl Pts',(-15.075736424986,-12.517295059255,117.381352025297)) ;
#161768=CARTESIAN_POINT('Ctrl Pts',(-15.1495402796035,-12.5172950786729,
117.357121017717)) ;
#161769=CARTESIAN_POINT('Ctrl Pts',(-15.1602152069174,-12.4495335423326,
117.389635123133)) ;
#161770=CARTESIAN_POINT('Ctrl Pts',(-15.1708901342314,-12.3817720059923,
117.42214922855)) ;
#161771=CARTESIAN_POINT('Ctrl Pts',(-15.0970862796139,-12.3817719865744,
117.44638023613)) ;
#161772=CARTESIAN_POINT('Ctrl Pts',(-15.0232824249965,-12.3817719671566,
117.47061124371)) ;
#161773=CARTESIAN_POINT('Ctrl Pts',(-15.0126074976825,-12.4495335034968,
117.438097138294)) ;
#161774=CARTESIAN_POINT('Ctrl Pts',(-15.0977303726993,-12.6159519111974,
117.661885772396)) ;
#161775=CARTESIAN_POINT('Ctrl Pts',(-15.0818299469695,-12.6721964554001,
117.613455641767)) ;
#161776=CARTESIAN_POINT('Ctrl Pts',(-15.1556337975825,-12.6721964775936,
117.58922462199)) ;
#161777=CARTESIAN_POINT('Ctrl Pts',(-15.2294376481955,-12.6721964997871,
117.564993602213)) ;
#161778=CARTESIAN_POINT('Ctrl Pts',(-15.2453380739253,-12.6159519555843,
117.613423732842)) ;
#161779=CARTESIAN_POINT('Ctrl Pts',(-15.2612384996551,-12.5597074113816,
117.661853863472)) ;
#161780=CARTESIAN_POINT('Ctrl Pts',(-15.1874346490421,-12.5597073891882,
117.686084883249)) ;
#161781=CARTESIAN_POINT('Ctrl Pts',(-15.1136307984291,-12.5597073669947,
117.710315903026)) ;
#161782=CARTESIAN_POINT('Ctrl Pts',(-15.0977303726993,-12.6159519111974,
117.661885772396)) ;
#161783=CARTESIAN_POINT('Ctrl Pts',(-15.1663307990368,-12.8395609374739,
117.835382986547)) ;
#161784=CARTESIAN_POINT('Ctrl Pts',(-15.1463499196944,-12.8802774256323,
117.774524452437)) ;
#161785=CARTESIAN_POINT('Ctrl Pts',(-15.2201537669202,-12.8802774463099,
117.750293422343)) ;
#161786=CARTESIAN_POINT('Ctrl Pts',(-15.293957614146,-12.8802774669874,
117.726062392249)) ;
#161787=CARTESIAN_POINT('Ctrl Pts',(-15.3139384934884,-12.839560978829,
117.786920926359)) ;
#161788=CARTESIAN_POINT('Ctrl Pts',(-15.3339193728309,-12.7988444906705,
117.847779460469)) ;
#161789=CARTESIAN_POINT('Ctrl Pts',(-15.260115525605,-12.798844469993,117.872010490563)) ;
#161790=CARTESIAN_POINT('Ctrl Pts',(-15.1863116783792,-12.7988444493154,
117.896241520657)) ;
#161791=CARTESIAN_POINT('Ctrl Pts',(-15.1663307990368,-12.8395609374739,
117.835382986547)) ;
#161792=CARTESIAN_POINT('Ctrl Pts',(-15.2143261495517,-13.1036924153161,
117.946224932861)) ;
#161793=CARTESIAN_POINT('Ctrl Pts',(-15.1916953168761,-13.126027690226,
117.877295068337)) ;
#161794=CARTESIAN_POINT('Ctrl Pts',(-15.265499161631,-13.1260277069746,
117.853064030717)) ;
#161795=CARTESIAN_POINT('Ctrl Pts',(-15.3393030063859,-13.1260277237232,
117.828832993097)) ;
#161796=CARTESIAN_POINT('Ctrl Pts',(-15.3619338390615,-13.1036924488133,
117.897762857621)) ;
#161797=CARTESIAN_POINT('Ctrl Pts',(-15.3845646717372,-13.0813571739034,
117.966692722145)) ;
#161798=CARTESIAN_POINT('Ctrl Pts',(-15.3107608269823,-13.0813571571548,
117.990923759765)) ;
#161799=CARTESIAN_POINT('Ctrl Pts',(-15.2369569822274,-13.0813571404062,
118.015154797385)) ;
#161800=CARTESIAN_POINT('Ctrl Pts',(-15.2143261495517,-13.1036924153161,
117.946224932861)) ;
#161801=CARTESIAN_POINT('Ctrl Pts',(-15.2392646854199,-13.3927905140901,
117.986526462558)) ;
#161802=CARTESIAN_POINT('Ctrl Pts',(-15.2155960469045,-13.3949729390862,
117.914435608735)) ;
#161803=CARTESIAN_POINT('Ctrl Pts',(-15.2893998901954,-13.3949729481192,
117.890204566656)) ;
#161804=CARTESIAN_POINT('Ctrl Pts',(-15.3632037334863,-13.3949729571521,
117.865973524577)) ;
#161805=CARTESIAN_POINT('Ctrl Pts',(-15.3868723720017,-13.392790532156,
117.9380643784)) ;
#161806=CARTESIAN_POINT('Ctrl Pts',(-15.4105410105172,-13.3906081071599,
118.010155232223)) ;
#161807=CARTESIAN_POINT('Ctrl Pts',(-15.3367371672263,-13.390608098127,
118.034386274302)) ;
#161808=CARTESIAN_POINT('Ctrl Pts',(-15.2629333239354,-13.3906080890941,
118.058617316381)) ;
#161809=CARTESIAN_POINT('Ctrl Pts',(-15.2392646854199,-13.3927905140901,
117.986526462558)) ;
#161810=CARTESIAN_POINT('Ctrl Pts',(-15.2397192982517,-13.6807940128297,
117.9526185938)) ;
#161811=CARTESIAN_POINT('Ctrl Pts',(-15.2167138279062,-13.6628697332101,
117.882547643134)) ;
#161812=CARTESIAN_POINT('Ctrl Pts',(-15.2905176708599,-13.6628697375112,
117.858316600028)) ;
#161813=CARTESIAN_POINT('Ctrl Pts',(-15.3643215138137,-13.6628697418123,
117.834085556922)) ;
#161814=CARTESIAN_POINT('Ctrl Pts',(-15.3873269841592,-13.680794021432,
117.904156507587)) ;
#161815=CARTESIAN_POINT('Ctrl Pts',(-15.4103324545046,-13.6987183010517,
117.974227458253)) ;
#161816=CARTESIAN_POINT('Ctrl Pts',(-15.3365286115509,-13.6987182967505,
117.998458501359)) ;
#161817=CARTESIAN_POINT('Ctrl Pts',(-15.2627247685972,-13.6987182924494,
118.022689544465)) ;
#161818=CARTESIAN_POINT('Ctrl Pts',(-15.2397192982517,-13.6807940128297,
117.9526185938)) ;
#161819=CARTESIAN_POINT('Ctrl Pts',(-15.2167475033035,-13.9516407801447,
117.847166620473)) ;
#161820=CARTESIAN_POINT('Ctrl Pts',(-15.1960458684568,-13.9147771638665,
117.784112780923)) ;
#161821=CARTESIAN_POINT('Ctrl Pts',(-15.2698497117907,-13.9147771635359,
117.759881738975)) ;
#161822=CARTESIAN_POINT('Ctrl Pts',(-15.3436535551245,-13.9147771632054,
117.735650697027)) ;
#161823=CARTESIAN_POINT('Ctrl Pts',(-15.3643551899713,-13.9516407794836,
117.798704536577)) ;
#161824=CARTESIAN_POINT('Ctrl Pts',(-15.3850568248181,-13.9885043957617,
117.861758376127)) ;
#161825=CARTESIAN_POINT('Ctrl Pts',(-15.3112529814842,-13.9885043960923,
117.885989418075)) ;
#161826=CARTESIAN_POINT('Ctrl Pts',(-15.2374491381503,-13.9885043964229,
117.910220460023)) ;
#161827=CARTESIAN_POINT('Ctrl Pts',(-15.2167475033035,-13.9516407801447,
117.847166620473)) ;
#161828=CARTESIAN_POINT('Ctrl Pts',(-15.1722328786369,-14.1848191645832,
117.675959254401)) ;
#161829=CARTESIAN_POINT('Ctrl Pts',(-15.1553459389584,-14.1316174193291,
117.62452436078)) ;
#161830=CARTESIAN_POINT('Ctrl Pts',(-15.2291497829877,-14.1316174171336,
117.600293320951)) ;
#161831=CARTESIAN_POINT('Ctrl Pts',(-15.3029536270171,-14.1316174149382,
117.576062281121)) ;
#161832=CARTESIAN_POINT('Ctrl Pts',(-15.3198405666957,-14.1848191601922,
117.627497174741)) ;
#161833=CARTESIAN_POINT('Ctrl Pts',(-15.3367275063742,-14.2380209054463,
117.678932068361)) ;
#161834=CARTESIAN_POINT('Ctrl Pts',(-15.2629236623449,-14.2380209076418,
117.703163108191)) ;
#161835=CARTESIAN_POINT('Ctrl Pts',(-15.1891198183155,-14.2380209098372,
117.727394148021)) ;
#161836=CARTESIAN_POINT('Ctrl Pts',(-15.1722328786369,-14.1848191645832,
117.675959254401)) ;
#161837=CARTESIAN_POINT('Ctrl Pts',(-15.1111116959615,-14.3611535147467,
117.45455531879)) ;
#161838=CARTESIAN_POINT('Ctrl Pts',(-15.0991970488396,-14.2955603830771,
117.418265226013)) ;
#161839=CARTESIAN_POINT('Ctrl Pts',(-15.173000893171,-14.2955603814556,
117.394034187103)) ;
#161840=CARTESIAN_POINT('Ctrl Pts',(-15.2468047375024,-14.2955603798341,
117.369803148193)) ;
#161841=CARTESIAN_POINT('Ctrl Pts',(-15.2587193846242,-14.3611535115037,
117.40609324097)) ;
#161842=CARTESIAN_POINT('Ctrl Pts',(-15.2706340317462,-14.4267466431733,
117.442383333747)) ;
#161843=CARTESIAN_POINT('Ctrl Pts',(-15.1968301874148,-14.4267466447948,
117.466614372657)) ;
#161844=CARTESIAN_POINT('Ctrl Pts',(-15.1230263430834,-14.4267466464163,
117.490845411567)) ;
#161845=CARTESIAN_POINT('Ctrl Pts',(-15.1111116959615,-14.3611535147467,
117.45455531879)) ;
#161846=CARTESIAN_POINT('Ctrl Pts',(-15.03716340119,-14.4717132500286,117.193678534081)) ;
#161847=CARTESIAN_POINT('Ctrl Pts',(-15.0311325532717,-14.3983025037114,
117.175309544367)) ;
#161848=CARTESIAN_POINT('Ctrl Pts',(-15.1049363971596,-14.3983025035885,
117.151078504106)) ;
#161849=CARTESIAN_POINT('Ctrl Pts',(-15.1787402410475,-14.3983025034657,
117.126847463845)) ;
#161850=CARTESIAN_POINT('Ctrl Pts',(-15.1847710889657,-14.4717132497829,
117.14521645356)) ;
#161851=CARTESIAN_POINT('Ctrl Pts',(-15.190801936884,-14.5451239961002,
117.163585443274)) ;
#161852=CARTESIAN_POINT('Ctrl Pts',(-15.1169980929961,-14.545123996223,
117.187816483535)) ;
#161853=CARTESIAN_POINT('Ctrl Pts',(-15.0431942491082,-14.5451239963458,
117.212047523796)) ;
#161854=CARTESIAN_POINT('Ctrl Pts',(-15.03716340119,-14.4717132500286,117.193678534081)) ;
#161855=CARTESIAN_POINT('Ctrl Pts',(-14.9574931202988,-14.5058049610956,
116.91556782578)) ;
#161856=CARTESIAN_POINT('Ctrl Pts',(-14.9577501226259,-14.4299061959812,
116.916350613445)) ;
#161857=CARTESIAN_POINT('Ctrl Pts',(-15.031553965324,-14.4299061963414,
116.892119569561)) ;
#161858=CARTESIAN_POINT('Ctrl Pts',(-15.105357808022,-14.4299061967016,
116.867888525676)) ;
#161859=CARTESIAN_POINT('Ctrl Pts',(-15.1051008056949,-14.505804961816,
116.86710573801)) ;
#161860=CARTESIAN_POINT('Ctrl Pts',(-15.1048438033677,-14.5817037269304,
116.866322950345)) ;
#161861=CARTESIAN_POINT('Ctrl Pts',(-15.0310399606696,-14.5817037265702,
116.89055399423)) ;
#161862=CARTESIAN_POINT('Ctrl Pts',(-14.9572361179716,-14.58170372621,116.914785038115)) ;
#161863=CARTESIAN_POINT('Ctrl Pts',(-14.9574931202988,-14.5058049610956,
116.91556782578)) ;
#161864=CARTESIAN_POINT('Ctrl Pts',(-14.8782558620267,-14.4622432474708,
116.638782637704)) ;
#161865=CARTESIAN_POINT('Ctrl Pts',(-14.8847794043709,-14.389275462024,
116.658652295255)) ;
#161866=CARTESIAN_POINT('Ctrl Pts',(-14.9585832455578,-14.3892754604599,
116.634421246768)) ;
#161867=CARTESIAN_POINT('Ctrl Pts',(-15.0323870867446,-14.3892754588959,
116.61019019828)) ;
#161868=CARTESIAN_POINT('Ctrl Pts',(-15.0258635444004,-14.4622432443427,
116.590320540728)) ;
#161869=CARTESIAN_POINT('Ctrl Pts',(-15.0193400020562,-14.5352110297894,
116.570450883177)) ;
#161870=CARTESIAN_POINT('Ctrl Pts',(-14.9455361608693,-14.5352110313535,
116.594681931664)) ;
#161871=CARTESIAN_POINT('Ctrl Pts',(-14.8717323196825,-14.5352110329176,
116.618912980152)) ;
#161872=CARTESIAN_POINT('Ctrl Pts',(-14.8782558620267,-14.4622432474708,
116.638782637704)) ;
#161873=CARTESIAN_POINT('Ctrl Pts',(-14.8058079691528,-14.343914063795,
116.382668771781)) ;
#161874=CARTESIAN_POINT('Ctrl Pts',(-14.8181331615164,-14.2791023763225,
116.42020931932)) ;
#161875=CARTESIAN_POINT('Ctrl Pts',(-14.8919370012243,-14.2791023697226,
116.395978266328)) ;
#161876=CARTESIAN_POINT('Ctrl Pts',(-14.9657408409322,-14.2791023631227,
116.371747213336)) ;
#161877=CARTESIAN_POINT('Ctrl Pts',(-14.9534156485687,-14.3439140505953,
116.334206665797)) ;
#161878=CARTESIAN_POINT('Ctrl Pts',(-14.9410904562051,-14.4087257380679,
116.296666118258)) ;
#161879=CARTESIAN_POINT('Ctrl Pts',(-14.8672866164972,-14.4087257446678,
116.32089717125)) ;
#161880=CARTESIAN_POINT('Ctrl Pts',(-14.7934827767893,-14.4087257512676,
116.345128224242)) ;
#161881=CARTESIAN_POINT('Ctrl Pts',(-14.8058079691528,-14.343914063795,
116.382668771781)) ;
#161882=CARTESIAN_POINT('Ctrl Pts',(-14.7461096383968,-14.1592285094383,
116.165376277947)) ;
#161883=CARTESIAN_POINT('Ctrl Pts',(-14.7633548151318,-14.1072180552491,
116.217902304186)) ;
#161884=CARTESIAN_POINT('Ctrl Pts',(-14.8371586539576,-14.1072180404113,
116.193671248507)) ;
#161885=CARTESIAN_POINT('Ctrl Pts',(-14.9109624927834,-14.1072180255735,
116.169440192828)) ;
#161886=CARTESIAN_POINT('Ctrl Pts',(-14.8937173160483,-14.1592284797627,
116.116914166588)) ;
#161887=CARTESIAN_POINT('Ctrl Pts',(-14.8764721393133,-14.2112389339519,
116.064388140349)) ;
#161888=CARTESIAN_POINT('Ctrl Pts',(-14.8026683004875,-14.2112389487897,
116.088619196028)) ;
#161889=CARTESIAN_POINT('Ctrl Pts',(-14.7288644616617,-14.2112389636275,
116.112850251707)) ;
#161890=CARTESIAN_POINT('Ctrl Pts',(-14.7461096383968,-14.1592285094383,
116.165376277947)) ;
#161891=CARTESIAN_POINT('Ctrl Pts',(-14.7042341925757,-13.9218383285055,
116.002418128098)) ;
#161892=CARTESIAN_POINT('Ctrl Pts',(-14.725160890206,-13.8863275964736,
116.066157473119)) ;
#161893=CARTESIAN_POINT('Ctrl Pts',(-14.7989647293144,-13.8863275716233,
116.0419264183)) ;
#161894=CARTESIAN_POINT('Ctrl Pts',(-14.8727685684227,-13.886327546773,
116.017695363482)) ;
#161895=CARTESIAN_POINT('Ctrl Pts',(-14.8518418707924,-13.9218382788049,
115.953956018461)) ;
#161896=CARTESIAN_POINT('Ctrl Pts',(-14.8309151731621,-13.9573490108368,
115.89021667344)) ;
#161897=CARTESIAN_POINT('Ctrl Pts',(-14.7571113340538,-13.9573490356871,
115.914447728259)) ;
#161898=CARTESIAN_POINT('Ctrl Pts',(-14.6833074949454,-13.9573490605374,
115.938678783077)) ;
#161899=CARTESIAN_POINT('Ctrl Pts',(-14.7042341925757,-13.9218383285055,
116.002418128098)) ;
#161900=CARTESIAN_POINT('Ctrl Pts',(-14.6838147453501,-13.6477929587425,
115.904727451076)) ;
#161901=CARTESIAN_POINT('Ctrl Pts',(-14.7069319501639,-13.6313648712608,
115.97513872771)) ;
#161902=CARTESIAN_POINT('Ctrl Pts',(-14.7807357908862,-13.6313648350965,
115.950907677807)) ;
#161903=CARTESIAN_POINT('Ctrl Pts',(-14.8545396316085,-13.6313647989322,
115.926676627904)) ;
#161904=CARTESIAN_POINT('Ctrl Pts',(-14.8314224267947,-13.6477928864138,
115.85626535127)) ;
#161905=CARTESIAN_POINT('Ctrl Pts',(-14.8083052219809,-13.6642209738955,
115.785854074636)) ;
#161906=CARTESIAN_POINT('Ctrl Pts',(-14.7345013812586,-13.6642210100599,
115.810085124539)) ;
#161907=CARTESIAN_POINT('Ctrl Pts',(-14.6606975405363,-13.6642210462242,
115.834316174442)) ;
#161908=CARTESIAN_POINT('Ctrl Pts',(-14.6838147453501,-13.6477929587425,
115.904727451076)) ;
#161909=CARTESIAN_POINT('Ctrl Pts',(-14.6872087463539,-13.3573882946602,
115.879587299227)) ;
#161910=CARTESIAN_POINT('Ctrl Pts',(-14.7108565242422,-13.3612124494826,
115.951614616009)) ;
#161911=CARTESIAN_POINT('Ctrl Pts',(-14.7846603682144,-13.3612124035114,
115.927383576005)) ;
#161912=CARTESIAN_POINT('Ctrl Pts',(-14.8584642121865,-13.3612123575402,
115.903152536001)) ;
#161913=CARTESIAN_POINT('Ctrl Pts',(-14.8348164342983,-13.3573882027177,
115.83112521922)) ;
#161914=CARTESIAN_POINT('Ctrl Pts',(-14.81116865641,-13.3535640478952,115.759097902438)) ;
#161915=CARTESIAN_POINT('Ctrl Pts',(-14.7373648124378,-13.3535640938664,
115.783328942442)) ;
#161916=CARTESIAN_POINT('Ctrl Pts',(-14.6635609684656,-13.3535641398377,
115.807559982446)) ;
#161917=CARTESIAN_POINT('Ctrl Pts',(-14.6872087463539,-13.3573882946602,
115.879587299227)) ;
#161918=CARTESIAN_POINT('Ctrl Pts',(-14.7148769500706,-13.0713760146383,
115.928387341854)) ;
#161919=CARTESIAN_POINT('Ctrl Pts',(-14.7373611554509,-13.0951747720227,
115.996870604688)) ;
#161920=CARTESIAN_POINT('Ctrl Pts',(-14.8111650040805,-13.0951747198527,
115.97263957887)) ;
#161921=CARTESIAN_POINT('Ctrl Pts',(-14.8849688527101,-13.0951746676827,
115.948408553052)) ;
#161922=CARTESIAN_POINT('Ctrl Pts',(-14.8624846473298,-13.0713759102982,
115.879925290218)) ;
#161923=CARTESIAN_POINT('Ctrl Pts',(-14.8400004419496,-13.0475771529138,
115.811442027384)) ;
#161924=CARTESIAN_POINT('Ctrl Pts',(-14.76619659332,-13.0475772050838,115.835673053202)) ;
#161925=CARTESIAN_POINT('Ctrl Pts',(-14.6923927446904,-13.0475772572539,
115.859904079021)) ;
#161926=CARTESIAN_POINT('Ctrl Pts',(-14.7148769500706,-13.0713760146383,
115.928387341854)) ;
#161927=CARTESIAN_POINT('Ctrl Pts',(-14.7656221631295,-12.8101300373193,
116.047465559082)) ;
#161928=CARTESIAN_POINT('Ctrl Pts',(-14.785330177933,-12.852202961782,116.107492993524)) ;
#161929=CARTESIAN_POINT('Ctrl Pts',(-14.8591340322195,-12.8522029087301,
116.083261984936)) ;
#161930=CARTESIAN_POINT('Ctrl Pts',(-14.9329378865061,-12.8522028556782,
116.059030976348)) ;
#161931=CARTESIAN_POINT('Ctrl Pts',(-14.9132298717026,-12.8101299312156,
115.999003541906)) ;
#161932=CARTESIAN_POINT('Ctrl Pts',(-14.8935218568992,-12.7680570067529,
115.938976107465)) ;
#161933=CARTESIAN_POINT('Ctrl Pts',(-14.8197180026126,-12.7680570598048,
115.963207116053)) ;
#161934=CARTESIAN_POINT('Ctrl Pts',(-14.745914148326,-12.7680571128567,
115.987438124641)) ;
#161935=CARTESIAN_POINT('Ctrl Pts',(-14.7656221631295,-12.8101300373193,
116.047465559082)) ;
#161936=CARTESIAN_POINT('Ctrl Pts',(-14.836499389826,-12.5926203368979,
116.227885615043)) ;
#161937=CARTESIAN_POINT('Ctrl Pts',(-14.8520211846851,-12.6499401722223,
116.275162499135)) ;
#161938=CARTESIAN_POINT('Ctrl Pts',(-14.9258250448979,-12.6499401250942,
116.250931508597)) ;
#161939=CARTESIAN_POINT('Ctrl Pts',(-14.9996289051108,-12.6499400779661,
116.22670051806)) ;
#161940=CARTESIAN_POINT('Ctrl Pts',(-14.9841071102517,-12.5926202426416,
116.179423633968)) ;
#161941=CARTESIAN_POINT('Ctrl Pts',(-14.9685853153926,-12.5353004073172,
116.132146749876)) ;
#161942=CARTESIAN_POINT('Ctrl Pts',(-14.8947814551798,-12.5353004544453,
116.156377740414)) ;
#161943=CARTESIAN_POINT('Ctrl Pts',(-14.820977594967,-12.5353005015734,
116.180608730951)) ;
#161944=CARTESIAN_POINT('Ctrl Pts',(-14.836499389826,-12.5926203368979,
116.227885615043)) ;
#161945=CARTESIAN_POINT('Ctrl Pts',(-14.9232190242914,-12.4341144288436,
116.456553356206)) ;
#161946=CARTESIAN_POINT('Ctrl Pts',(-14.9334426620929,-12.5025837722115,
116.487692908903)) ;
#161947=CARTESIAN_POINT('Ctrl Pts',(-15.0072465277716,-12.5025837377898,
116.463461935014)) ;
#161948=CARTESIAN_POINT('Ctrl Pts',(-15.0810503934502,-12.502583703368,
116.439230961124)) ;
#161949=CARTESIAN_POINT('Ctrl Pts',(-15.0708267556487,-12.4341143600001,
116.408091408427)) ;
#161950=CARTESIAN_POINT('Ctrl Pts',(-15.0606031178471,-12.3656450166321,
116.37695185573)) ;
#161951=CARTESIAN_POINT('Ctrl Pts',(-14.9867992521685,-12.3656450510539,
116.40118282962)) ;
#161952=CARTESIAN_POINT('Ctrl Pts',(-14.9129953864899,-12.3656450854756,
116.425413803509)) ;
#161953=CARTESIAN_POINT('Ctrl Pts',(-14.9232190242914,-12.4341144288436,
116.456553356206)) ;
#161954=CARTESIAN_POINT('Ctrl Pts',(-15.0204191933641,-12.346259851331,
116.717108536912)) ;
#161955=CARTESIAN_POINT('Ctrl Pts',(-15.0246060505222,-12.4209624752005,
116.729861029938)) ;
#161956=CARTESIAN_POINT('Ctrl Pts',(-15.0984099204493,-12.4209624599237,
116.705630068989)) ;
#161957=CARTESIAN_POINT('Ctrl Pts',(-15.1722137903763,-12.4209624446469,
116.681399108039)) ;
#161958=CARTESIAN_POINT('Ctrl Pts',(-15.1680269332182,-12.3462598207773,
116.668646615013)) ;
#161959=CARTESIAN_POINT('Ctrl Pts',(-15.1638400760601,-12.2715571969078,
116.655894121986)) ;
#161960=CARTESIAN_POINT('Ctrl Pts',(-15.090036206133,-12.2715572121846,
116.680125082936)) ;
#161961=CARTESIAN_POINT('Ctrl Pts',(-15.016232336206,-12.2715572274614,
116.704356043885)) ;
#161962=CARTESIAN_POINT('Ctrl Pts',(-15.0204191933641,-12.346259851331,
116.717108536912)) ;
#161963=CARTESIAN_POINT('Ctrl Pts',(-15.1212516203235,-12.3348158852733,
116.98892332195)) ;
#161964=CARTESIAN_POINT('Ctrl Pts',(-15.1191352709603,-12.4104256805368,
116.982477265032)) ;
#161965=CARTESIAN_POINT('Ctrl Pts',(-15.1929391428361,-12.4104256886821,
116.958246310018)) ;
#161966=CARTESIAN_POINT('Ctrl Pts',(-15.266743014712,-12.4104256968275,
116.934015355004)) ;
#161967=CARTESIAN_POINT('Ctrl Pts',(-15.2688593640751,-12.334815901564,
116.940461411923)) ;
#161968=CARTESIAN_POINT('Ctrl Pts',(-15.2709757134383,-12.2592061063006,
116.946907468841)) ;
#161969=CARTESIAN_POINT('Ctrl Pts',(-15.1971718415625,-12.2592060981552,
116.971138423855)) ;
#161970=CARTESIAN_POINT('Ctrl Pts',(-15.1233679696867,-12.2592060900098,
116.995369378869)) ;
#161971=CARTESIAN_POINT('Ctrl Pts',(-15.1212516203235,-12.3348158852733,
116.98892332195)) ;
#161972=CARTESIAN_POINT('Ctrl Pts',(-15.2210253617375,-12.4019396871859,
117.257046128186)) ;
#161973=CARTESIAN_POINT('Ctrl Pts',(-15.2126803008155,-12.4729745049504,
117.231628420995)) ;
#161974=CARTESIAN_POINT('Ctrl Pts',(-15.2864841729896,-12.4729745398318,
117.207397466889)) ;
#161975=CARTESIAN_POINT('Ctrl Pts',(-15.3602880451638,-12.4729745747131,
117.183166512784)) ;
#161976=CARTESIAN_POINT('Ctrl Pts',(-15.3686331060857,-12.4019397569486,
117.208584219976)) ;
#161977=CARTESIAN_POINT('Ctrl Pts',(-15.3769781670076,-12.330904939184,
117.234001927168)) ;
#161978=CARTESIAN_POINT('Ctrl Pts',(-15.3031742948335,-12.3309049043027,
117.258232881273)) ;
#161979=CARTESIAN_POINT('Ctrl Pts',(-15.2293704226594,-12.3309048694214,
117.282463835378)) ;
#161980=CARTESIAN_POINT('Ctrl Pts',(-15.2210253617375,-12.4019396871859,
117.257046128186)) ;
#161981=CARTESIAN_POINT('Ctrl Pts',(-15.3104774186011,-12.5400212389952,
117.494364772624)) ;
#161982=CARTESIAN_POINT('Ctrl Pts',(-15.2966020261323,-12.6015185806479,
117.452102567907)) ;
#161983=CARTESIAN_POINT('Ctrl Pts',(-15.3704058950722,-12.6015186402617,
117.427871603951)) ;
#161984=CARTESIAN_POINT('Ctrl Pts',(-15.4442097640122,-12.6015186998755,
117.403640639995)) ;
#161985=CARTESIAN_POINT('Ctrl Pts',(-15.458085156481,-12.5400213582228,
117.445902844712)) ;
#161986=CARTESIAN_POINT('Ctrl Pts',(-15.4719605489497,-12.4785240165702,
117.488165049428)) ;
#161987=CARTESIAN_POINT('Ctrl Pts',(-15.3981566800098,-12.4785239569564,
117.512396013384)) ;
#161988=CARTESIAN_POINT('Ctrl Pts',(-15.3243528110698,-12.4785238973426,
117.53662697734)) ;
#161989=CARTESIAN_POINT('Ctrl Pts',(-15.3104774186011,-12.5400212389952,
117.494364772624)) ;
#161990=CARTESIAN_POINT('Ctrl Pts',(-15.386781464252,-12.7426569389483,
117.691155444074)) ;
#161991=CARTESIAN_POINT('Ctrl Pts',(-15.368295445562,-12.790097789664,117.634850015886)) ;
#161992=CARTESIAN_POINT('Ctrl Pts',(-15.4420993094136,-12.7900978720305,
117.610619036432)) ;
#161993=CARTESIAN_POINT('Ctrl Pts',(-15.5159031732653,-12.790097954397,
117.586388056978)) ;
#161994=CARTESIAN_POINT('Ctrl Pts',(-15.5343891919552,-12.7426571036813,
117.642693485165)) ;
#161995=CARTESIAN_POINT('Ctrl Pts',(-15.5528752106452,-12.6952162529655,
117.698998913352)) ;
#161996=CARTESIAN_POINT('Ctrl Pts',(-15.4790713467936,-12.695216170599,
117.723229892807)) ;
#161997=CARTESIAN_POINT('Ctrl Pts',(-15.405267482942,-12.6952160882325,
117.747460872261)) ;
#161998=CARTESIAN_POINT('Ctrl Pts',(-15.386781464252,-12.7426569389483,
117.691155444074)) ;
#161999=CARTESIAN_POINT('Ctrl Pts',(-15.4435452552671,-12.9928209893326,
117.828633943598)) ;
#162000=CARTESIAN_POINT('Ctrl Pts',(-15.4218018018575,-13.0228660525859,
117.762406894878)) ;
#162001=CARTESIAN_POINT('Ctrl Pts',(-15.4956056583648,-13.0228661512881,
117.738175893054)) ;
#162002=CARTESIAN_POINT('Ctrl Pts',(-15.569409514872,-13.0228662499903,
117.71394489123)) ;
#162003=CARTESIAN_POINT('Ctrl Pts',(-15.5911529682816,-12.992821186737,
117.78017193995)) ;
#162004=CARTESIAN_POINT('Ctrl Pts',(-15.6128964216912,-12.9627761234838,
117.846398988669)) ;
#162005=CARTESIAN_POINT('Ctrl Pts',(-15.5390925651839,-12.9627760247816,
117.870629990493)) ;
#162006=CARTESIAN_POINT('Ctrl Pts',(-15.4652887086767,-12.9627759260794,
117.894860992317)) ;
#162007=CARTESIAN_POINT('Ctrl Pts',(-15.4435452552671,-12.9928209893326,
117.828633943598)) ;
#162008=CARTESIAN_POINT('Ctrl Pts',(-15.4780991318046,-13.274121349933,
117.89835399274)) ;
#162009=CARTESIAN_POINT('Ctrl Pts',(-15.454646181204,-13.2845716251807,
117.826920091425)) ;
#162010=CARTESIAN_POINT('Ctrl Pts',(-15.5284500290858,-13.2845717326201,
117.80268906333)) ;
#162011=CARTESIAN_POINT('Ctrl Pts',(-15.6022538769677,-13.2845718400594,
117.778458035234)) ;
#162012=CARTESIAN_POINT('Ctrl Pts',(-15.6257068275682,-13.2741215648117,
117.849891936549)) ;
#162013=CARTESIAN_POINT('Ctrl Pts',(-15.6491597781688,-13.263671289564,
117.921325837863)) ;
#162014=CARTESIAN_POINT('Ctrl Pts',(-15.5753559302869,-13.2636711821247,
117.945556865959)) ;
#162015=CARTESIAN_POINT('Ctrl Pts',(-15.5015520824051,-13.2636710746853,
117.969787894055)) ;
#162016=CARTESIAN_POINT('Ctrl Pts',(-15.4780991318046,-13.274121349933,
117.89835399274)) ;
#162017=CARTESIAN_POINT('Ctrl Pts',(-15.4884434105682,-13.5650423075934,
117.894429498399)) ;
#162018=CARTESIAN_POINT('Ctrl Pts',(-15.4649666718816,-13.5551969668732,
117.822923142409)) ;
#162019=CARTESIAN_POINT('Ctrl Pts',(-15.5387705106964,-13.555197074088,
117.798692086697)) ;
#162020=CARTESIAN_POINT('Ctrl Pts',(-15.6125743495112,-13.5551971813029,
117.774461030985)) ;
#162021=CARTESIAN_POINT('Ctrl Pts',(-15.6360510881978,-13.5650425220231,
117.845967386975)) ;
#162022=CARTESIAN_POINT('Ctrl Pts',(-15.6595278268843,-13.5748878627432,
117.917473742965)) ;
#162023=CARTESIAN_POINT('Ctrl Pts',(-15.5857239880695,-13.5748877555284,
117.941704798677)) ;
#162024=CARTESIAN_POINT('Ctrl Pts',(-15.5119201492547,-13.5748876483136,
117.965935854389)) ;
#162025=CARTESIAN_POINT('Ctrl Pts',(-15.4884434105682,-13.5650423075934,
117.894429498399)) ;
#162026=CARTESIAN_POINT('Ctrl Pts',(-15.4747873042015,-13.8454220244642,
117.817406765733)) ;
#162027=CARTESIAN_POINT('Ctrl Pts',(-15.4529622075996,-13.8159869229919,
117.750931045019)) ;
#162028=CARTESIAN_POINT('Ctrl Pts',(-15.5267660378298,-13.8159870213789,
117.72669996316)) ;
#162029=CARTESIAN_POINT('Ctrl Pts',(-15.60056986806,-13.8159871197658,117.7024688813)) ;
#162030=CARTESIAN_POINT('Ctrl Pts',(-15.622394964662,-13.8454222212381,
117.768944602014)) ;
#162031=CARTESIAN_POINT('Ctrl Pts',(-15.644220061264,-13.8748573227103,
117.835420322728)) ;
#162032=CARTESIAN_POINT('Ctrl Pts',(-15.5704162310338,-13.8748572243234,
117.859651404588)) ;
#162033=CARTESIAN_POINT('Ctrl Pts',(-15.4966124008035,-13.8748571259364,
117.883882486447)) ;
#162034=CARTESIAN_POINT('Ctrl Pts',(-15.4747873042015,-13.8454220244642,
117.817406765733)) ;
#162035=CARTESIAN_POINT('Ctrl Pts',(-15.4387248228193,-14.095635489283,
117.672076552588)) ;
#162036=CARTESIAN_POINT('Ctrl Pts',(-15.4201192687897,-14.0486874017416,
117.615407039032)) ;
#162037=CARTESIAN_POINT('Ctrl Pts',(-15.4939230917936,-14.0486874834364,
117.591175935163)) ;
#162038=CARTESIAN_POINT('Ctrl Pts',(-15.5677269147975,-14.0486875651311,
117.566944831293)) ;
#162039=CARTESIAN_POINT('Ctrl Pts',(-15.5863324688271,-14.0956356526725,
117.623614344849)) ;
#162040=CARTESIAN_POINT('Ctrl Pts',(-15.6049380228566,-14.1425837402138,
117.680283858405)) ;
#162041=CARTESIAN_POINT('Ctrl Pts',(-15.5311341998527,-14.1425836585191,
117.704514962275)) ;
#162042=CARTESIAN_POINT('Ctrl Pts',(-15.4573303768488,-14.1425835768243,
117.728746066145)) ;
#162043=CARTESIAN_POINT('Ctrl Pts',(-15.4387248228193,-14.095635489283,
117.672076552588)) ;
#162044=CARTESIAN_POINT('Ctrl Pts',(-15.3836965141025,-14.2970558104585,
117.469021551389)) ;
#162045=CARTESIAN_POINT('Ctrl Pts',(-15.3696385446302,-14.2359749683573,
117.426203246579)) ;
#162046=CARTESIAN_POINT('Ctrl Pts',(-15.4434423624372,-14.2359750277231,
117.40197212688)) ;
#162047=CARTESIAN_POINT('Ctrl Pts',(-15.5172461802443,-14.2359750870889,
117.377741007182)) ;
#162048=CARTESIAN_POINT('Ctrl Pts',(-15.5313041497167,-14.2970559291901,
117.420559311992)) ;
#162049=CARTESIAN_POINT('Ctrl Pts',(-15.545362119189,-14.3581367712912,
117.463377616802)) ;
#162050=CARTESIAN_POINT('Ctrl Pts',(-15.471558301382,-14.3581367119255,
117.487608736501)) ;
#162051=CARTESIAN_POINT('Ctrl Pts',(-15.3977544835749,-14.3581366525597,
117.511839856199)) ;
#162052=CARTESIAN_POINT('Ctrl Pts',(-15.3836965141025,-14.2970558104585,
117.469021551389)) ;
#162053=CARTESIAN_POINT('Ctrl Pts',(-15.3141371945857,-14.4359480747077,
117.221601988843)) ;
#162054=CARTESIAN_POINT('Ctrl Pts',(-15.3056501747108,-14.3650783452255,
117.195751897542)) ;
#162055=CARTESIAN_POINT('Ctrl Pts',(-15.3794539899394,-14.3650783787337,
117.17152076999)) ;
#162056=CARTESIAN_POINT('Ctrl Pts',(-15.453257805168,-14.3650784122419,
117.147289642437)) ;
#162057=CARTESIAN_POINT('Ctrl Pts',(-15.4617448250429,-14.4359481417242,
117.173139733739)) ;
#162058=CARTESIAN_POINT('Ctrl Pts',(-15.4702318449178,-14.5068178712064,
117.19898982504)) ;
#162059=CARTESIAN_POINT('Ctrl Pts',(-15.3964280296892,-14.5068178376981,
117.223220952592)) ;
#162060=CARTESIAN_POINT('Ctrl Pts',(-15.3226242144606,-14.5068178041899,
117.247452080144)) ;
#162061=CARTESIAN_POINT('Ctrl Pts',(-15.3141371945857,-14.4359480747077,
117.221601988843)) ;
#162062=CARTESIAN_POINT('Ctrl Pts',(-15.2359817859273,-14.501304829004,
116.948020668741)) ;
#162063=CARTESIAN_POINT('Ctrl Pts',(-15.2336738762587,-14.4257651981435,
116.940991150015)) ;
#162064=CARTESIAN_POINT('Ctrl Pts',(-15.3074776916091,-14.4257652059426,
116.916760022834)) ;
#162065=CARTESIAN_POINT('Ctrl Pts',(-15.3812815069595,-14.4257652137418,
116.892528895653)) ;
#162066=CARTESIAN_POINT('Ctrl Pts',(-15.3835894166281,-14.5013048446024,
116.899558414379)) ;
#162067=CARTESIAN_POINT('Ctrl Pts',(-15.3858973262967,-14.576844475463,
116.906587933104)) ;
#162068=CARTESIAN_POINT('Ctrl Pts',(-15.3120935109463,-14.5768444676638,
116.930819060286)) ;
#162069=CARTESIAN_POINT('Ctrl Pts',(-15.2382896955959,-14.5768444598646,
116.955050187467)) ;
#162070=CARTESIAN_POINT('Ctrl Pts',(-15.2359817859273,-14.501304829004,
116.948020668741)) ;
#162071=CARTESIAN_POINT('Ctrl Pts',(-15.1561240539043,-14.4893139259723,
116.669494222094)) ;
#162072=CARTESIAN_POINT('Ctrl Pts',(-15.1601185367574,-14.4144981524163,
116.681660774003)) ;
#162073=CARTESIAN_POINT('Ctrl Pts',(-15.2339223540431,-14.4144981369881,
116.657429652717)) ;
#162074=CARTESIAN_POINT('Ctrl Pts',(-15.3077261713288,-14.4144981215599,
116.63319853143)) ;
#162075=CARTESIAN_POINT('Ctrl Pts',(-15.3037316884757,-14.4893138951159,
116.621031979521)) ;
#162076=CARTESIAN_POINT('Ctrl Pts',(-15.2997372056226,-14.564129668672,
116.608865427612)) ;
#162077=CARTESIAN_POINT('Ctrl Pts',(-15.2259333883369,-14.5641296841002,
116.633096548898)) ;
#162078=CARTESIAN_POINT('Ctrl Pts',(-15.1521295710511,-14.5641296995284,
116.657327670185)) ;
#162079=CARTESIAN_POINT('Ctrl Pts',(-15.1561240539043,-14.4893139259723,
116.669494222094)) ;
#162080=CARTESIAN_POINT('Ctrl Pts',(-15.0799694117837,-14.4004454436412,
116.401998946719)) ;
#162081=CARTESIAN_POINT('Ctrl Pts',(-15.090022382406,-14.3317211347541,
116.432618674691)) ;
#162082=CARTESIAN_POINT('Ctrl Pts',(-15.1638262040758,-14.331721100851,
116.408387566758)) ;
#162083=CARTESIAN_POINT('Ctrl Pts',(-15.2376300257455,-14.331721066948,
116.384156458824)) ;
#162084=CARTESIAN_POINT('Ctrl Pts',(-15.2275770551231,-14.4004453758351,
116.353536730852)) ;
#162085=CARTESIAN_POINT('Ctrl Pts',(-15.2175240845008,-14.4691696847222,
116.322917002879)) ;
#162086=CARTESIAN_POINT('Ctrl Pts',(-15.143720262831,-14.4691697186253,
116.347148110813)) ;
#162087=CARTESIAN_POINT('Ctrl Pts',(-15.0699164411613,-14.4691697525284,
116.371379218746)) ;
#162088=CARTESIAN_POINT('Ctrl Pts',(-15.0799694117837,-14.4004454436412,
116.401998946719)) ;
#162089=CARTESIAN_POINT('Ctrl Pts',(-15.0146075791838,-14.2418718140722,
116.167568446909)) ;
#162090=CARTESIAN_POINT('Ctrl Pts',(-15.0299707183661,-14.1841154082224,
116.214362091392)) ;
#162091=CARTESIAN_POINT('Ctrl Pts',(-15.1037745452079,-14.1841153614757,
116.190130999212)) ;
#162092=CARTESIAN_POINT('Ctrl Pts',(-15.1775783720496,-14.1841153147289,
116.165899907032)) ;
#162093=CARTESIAN_POINT('Ctrl Pts',(-15.1622152328674,-14.2418717205788,
116.119106262548)) ;
#162094=CARTESIAN_POINT('Ctrl Pts',(-15.1468520936851,-14.2996281264286,
116.072312618065)) ;
#162095=CARTESIAN_POINT('Ctrl Pts',(-15.0730482668433,-14.2996281731753,
116.096543710245)) ;
#162096=CARTESIAN_POINT('Ctrl Pts',(-14.9992444400016,-14.299628219922,
116.120774802425)) ;
#162097=CARTESIAN_POINT('Ctrl Pts',(-15.0146075791838,-14.2418718140722,
116.167568446909)) ;
#162098=CARTESIAN_POINT('Ctrl Pts',(-14.9647824826636,-14.0233785235775,
115.98025836275)) ;
#162099=CARTESIAN_POINT('Ctrl Pts',(-14.9843833842169,-13.9807896305814,
116.039959547481)) ;
#162100=CARTESIAN_POINT('Ctrl Pts',(-15.0581872171145,-13.9807895787785,
116.015728473746)) ;
#162101=CARTESIAN_POINT('Ctrl Pts',(-15.1319910500122,-13.9807895269757,
115.991497400011)) ;
#162102=CARTESIAN_POINT('Ctrl Pts',(-15.1123901484589,-14.0233784199718,
115.93179621528)) ;
#162103=CARTESIAN_POINT('Ctrl Pts',(-15.0927892469056,-14.0659673129679,
115.872095030548)) ;
#162104=CARTESIAN_POINT('Ctrl Pts',(-15.018985414008,-14.0659673647708,
115.896326104283)) ;
#162105=CARTESIAN_POINT('Ctrl Pts',(-14.9451815811103,-14.0659674165736,
115.920557178019)) ;
#162106=CARTESIAN_POINT('Ctrl Pts',(-14.9647824826636,-14.0233785235775,
115.98025836275)) ;
#162107=CARTESIAN_POINT('Ctrl Pts',(-14.9353130383132,-13.7618917263419,
115.855036424513)) ;
#162108=CARTESIAN_POINT('Ctrl Pts',(-14.9577350844152,-13.7374955038548,
115.923330360184)) ;
#162109=CARTESIAN_POINT('Ctrl Pts',(-15.0315389228224,-13.7374954531261,
115.89909930323)) ;
#162110=CARTESIAN_POINT('Ctrl Pts',(-15.1053427612296,-13.7374954023974,
115.874868246276)) ;
#162111=CARTESIAN_POINT('Ctrl Pts',(-15.0829207151276,-13.7618916248845,
115.806574310605)) ;
#162112=CARTESIAN_POINT('Ctrl Pts',(-15.0604986690256,-13.7862878473716,
115.738280374933)) ;
#162113=CARTESIAN_POINT('Ctrl Pts',(-14.9866948306184,-13.7862878981003,
115.762511431887)) ;
#162114=CARTESIAN_POINT('Ctrl Pts',(-14.9128909922112,-13.786287948829,
115.786742488841)) ;
#162115=CARTESIAN_POINT('Ctrl Pts',(-14.9353130383132,-13.7618917263419,
115.855036424513)) ;
#162116=CARTESIAN_POINT('Ctrl Pts',(-14.9289325059808,-13.4754623735639,
115.800094097423)) ;
#162117=CARTESIAN_POINT('Ctrl Pts',(-14.9525688879762,-13.471028133492,
115.872086704117)) ;
#162118=CARTESIAN_POINT('Ctrl Pts',(-15.0263727308896,-13.4710280894286,
115.847855660888)) ;
#162119=CARTESIAN_POINT('Ctrl Pts',(-15.100176573803,-13.4710280453652,
115.823624617659)) ;
#162120=CARTESIAN_POINT('Ctrl Pts',(-15.0765401918076,-13.4754622854371,
115.751632010965)) ;
#162121=CARTESIAN_POINT('Ctrl Pts',(-15.0529038098122,-13.479896525509,
115.679639404272)) ;
#162122=CARTESIAN_POINT('Ctrl Pts',(-14.9790999668988,-13.4798965695724,
115.703870447501)) ;
#162123=CARTESIAN_POINT('Ctrl Pts',(-14.9052961239854,-13.4798966136358,
115.728101490729)) ;
#162124=CARTESIAN_POINT('Ctrl Pts',(-14.9289325059808,-13.4754623735639,
115.800094097423)) ;
#162125=CARTESIAN_POINT('Ctrl Pts',(-14.9467156400316,-13.1862230579374,
115.818918808621)) ;
#162126=CARTESIAN_POINT('Ctrl Pts',(-14.9698774007745,-13.2019774295457,
115.889465795415)) ;
#162127=CARTESIAN_POINT('Ctrl Pts',(-15.0436812468443,-13.2019773939464,
115.8652347618)) ;
#162128=CARTESIAN_POINT('Ctrl Pts',(-15.1174850929142,-13.2019773583471,
115.841003728185)) ;
#162129=CARTESIAN_POINT('Ctrl Pts',(-15.0943233321713,-13.1862229867387,
115.770456741391)) ;
#162130=CARTESIAN_POINT('Ctrl Pts',(-15.0711615714284,-13.1704686151304,
115.699909754597)) ;
#162131=CARTESIAN_POINT('Ctrl Pts',(-14.9973577253585,-13.1704686507297,
115.724140788212)) ;
#162132=CARTESIAN_POINT('Ctrl Pts',(-14.9235538792887,-13.170468686329,
115.748371821826)) ;
#162133=CARTESIAN_POINT('Ctrl Pts',(-14.9467156400316,-13.1862230579374,
115.818918808621)) ;
#162134=CARTESIAN_POINT('Ctrl Pts',(-14.9883696704994,-12.9121173454345,
115.910257352319)) ;
#162135=CARTESIAN_POINT('Ctrl Pts',(-15.0093934840061,-12.9470346448942,
115.974292496613)) ;
#162136=CARTESIAN_POINT('Ctrl Pts',(-15.0831973316234,-12.947034620835,
115.950061467711)) ;
#162137=CARTESIAN_POINT('Ctrl Pts',(-15.1570011792406,-12.9470345967758,
115.925830438809)) ;
#162138=CARTESIAN_POINT('Ctrl Pts',(-15.1359773657339,-12.9121172973162,
115.861795294515)) ;
#162139=CARTESIAN_POINT('Ctrl Pts',(-15.1149535522271,-12.8771999978565,
115.797760150221)) ;
#162140=CARTESIAN_POINT('Ctrl Pts',(-15.0411497046099,-12.8772000219157,
115.821991179123)) ;
#162141=CARTESIAN_POINT('Ctrl Pts',(-14.9673458569927,-12.8772000459749,
115.846222208024)) ;
#162142=CARTESIAN_POINT('Ctrl Pts',(-14.9883696704994,-12.9121173454345,
115.910257352319)) ;
#162143=CARTESIAN_POINT('Ctrl Pts',(-15.0514075082548,-12.6748571224349,
116.066831542999)) ;
#162144=CARTESIAN_POINT('Ctrl Pts',(-15.0687947514386,-12.7263936809792,
116.119790280699)) ;
#162145=CARTESIAN_POINT('Ctrl Pts',(-15.1425985992495,-12.7263936670357,
116.095559252388)) ;
#162146=CARTESIAN_POINT('Ctrl Pts',(-15.2164024470604,-12.7263936530922,
116.071328224076)) ;
#162147=CARTESIAN_POINT('Ctrl Pts',(-15.1990152038766,-12.6748570945479,
116.018369486375)) ;
#162148=CARTESIAN_POINT('Ctrl Pts',(-15.1816279606928,-12.6233205360036,
115.965410748675)) ;
#162149=CARTESIAN_POINT('Ctrl Pts',(-15.1078241128819,-12.6233205499471,
115.989641776987)) ;
#162150=CARTESIAN_POINT('Ctrl Pts',(-15.034020265071,-12.6233205638906,
116.013872805299)) ;
#162151=CARTESIAN_POINT('Ctrl Pts',(-15.0514075082548,-12.6748571224349,
116.066831542999)) ;
#162152=CARTESIAN_POINT('Ctrl Pts',(-15.1328444729729,-12.4898752939566,
116.279188009529)) ;
#162153=CARTESIAN_POINT('Ctrl Pts',(-15.1453102034931,-12.5544068109691,
116.317156613569)) ;
#162154=CARTESIAN_POINT('Ctrl Pts',(-15.2191140499375,-12.5544068057079,
116.292925581095)) ;
#162155=CARTESIAN_POINT('Ctrl Pts',(-15.2929178963818,-12.5544068004467,
116.26869454862)) ;
#162156=CARTESIAN_POINT('Ctrl Pts',(-15.2804521658616,-12.4898752834342,
116.230725944581)) ;
#162157=CARTESIAN_POINT('Ctrl Pts',(-15.2679864353413,-12.4253437664217,
116.192757340541)) ;
#162158=CARTESIAN_POINT('Ctrl Pts',(-15.194182588897,-12.4253437716829,
116.216988373016)) ;
#162159=CARTESIAN_POINT('Ctrl Pts',(-15.1203787424527,-12.4253437769441,
116.24121940549)) ;
#162160=CARTESIAN_POINT('Ctrl Pts',(-15.1328444729729,-12.4898752939566,
116.279188009529)) ;
#162161=CARTESIAN_POINT('Ctrl Pts',(-15.2258152326025,-12.3730682967797,
116.527146434279)) ;
#162162=CARTESIAN_POINT('Ctrl Pts',(-15.2325367436392,-12.4458523869168,
116.547619072512)) ;
#162163=CARTESIAN_POINT('Ctrl Pts',(-15.3063405890483,-12.4458523855329,
116.523388036884)) ;
#162164=CARTESIAN_POINT('Ctrl Pts',(-15.3801444344574,-12.445852384149,
116.499157001257)) ;
#162165=CARTESIAN_POINT('Ctrl Pts',(-15.3734229234207,-12.3730682940119,
116.478684363024)) ;
#162166=CARTESIAN_POINT('Ctrl Pts',(-15.366701412384,-12.3002842038747,
116.458211724791)) ;
#162167=CARTESIAN_POINT('Ctrl Pts',(-15.2928975669749,-12.3002842052586,
116.482442760418)) ;
#162168=CARTESIAN_POINT('Ctrl Pts',(-15.2190937215657,-12.3002842066425,
116.506673796046)) ;
#162169=CARTESIAN_POINT('Ctrl Pts',(-15.2258152326025,-12.3730682967797,
116.527146434279)) ;
#162170=CARTESIAN_POINT('Ctrl Pts',(-15.3267957548085,-12.330125354393,
116.799022433184)) ;
#162171=CARTESIAN_POINT('Ctrl Pts',(-15.327214765721,-12.4060180175289,
116.800298672828)) ;
#162172=CARTESIAN_POINT('Ctrl Pts',(-15.4010186093175,-12.4060180179283,
116.77606763168)) ;
#162173=CARTESIAN_POINT('Ctrl Pts',(-15.474822452914,-12.4060180183277,
116.751836590531)) ;
#162174=CARTESIAN_POINT('Ctrl Pts',(-15.4744034420016,-12.3301253551918,
116.750560350888)) ;
#162175=CARTESIAN_POINT('Ctrl Pts',(-15.4739844310891,-12.2542326920559,
116.749284111245)) ;
#162176=CARTESIAN_POINT('Ctrl Pts',(-15.4001805874926,-12.2542326916565,
116.773515152393)) ;
#162177=CARTESIAN_POINT('Ctrl Pts',(-15.326376743896,-12.2542326912571,
116.797746193541)) ;
#162178=CARTESIAN_POINT('Ctrl Pts',(-15.3267957548085,-12.330125354393,
116.799022433184)) ;
#162179=CARTESIAN_POINT('Ctrl Pts',(-15.4267371080215,-12.3650026478225,
117.068234016832)) ;
#162180=CARTESIAN_POINT('Ctrl Pts',(-15.4209065945382,-12.4385726507877,
117.050475213478)) ;
#162181=CARTESIAN_POINT('Ctrl Pts',(-15.4947104373962,-12.4385726504867,
117.02624417008)) ;
#162182=CARTESIAN_POINT('Ctrl Pts',(-15.5685142802541,-12.4385726501857,
117.002013126682)) ;
#162183=CARTESIAN_POINT('Ctrl Pts',(-15.5743447937374,-12.3650026472205,
117.019771930036)) ;
#162184=CARTESIAN_POINT('Ctrl Pts',(-15.5801753072207,-12.2914326442552,
117.037530733391)) ;
#162185=CARTESIAN_POINT('Ctrl Pts',(-15.5063714643627,-12.2914326445563,
117.061761776789)) ;
#162186=CARTESIAN_POINT('Ctrl Pts',(-15.4325676215048,-12.2914326448573,
117.085992820186)) ;
#162187=CARTESIAN_POINT('Ctrl Pts',(-15.4267371080215,-12.3650026478225,
117.068234016832)) ;
#162188=CARTESIAN_POINT('Ctrl Pts',(-15.5220396277674,-12.4764750890778,
117.322748096145)) ;
#162189=CARTESIAN_POINT('Ctrl Pts',(-15.5102853182541,-12.5423709931459,
117.286946365851)) ;
#162190=CARTESIAN_POINT('Ctrl Pts',(-15.5840891607112,-12.5423709914641,
117.262715321232)) ;
#162191=CARTESIAN_POINT('Ctrl Pts',(-15.6578930031683,-12.5423709897823,
117.238484276613)) ;
#162192=CARTESIAN_POINT('Ctrl Pts',(-15.6696473126816,-12.4764750857142,
117.274286006907)) ;
#162193=CARTESIAN_POINT('Ctrl Pts',(-15.6814016221949,-12.410579181646,
117.310087737201)) ;
#162194=CARTESIAN_POINT('Ctrl Pts',(-15.6075977797378,-12.4105791833278,
117.33431878182)) ;
#162195=CARTESIAN_POINT('Ctrl Pts',(-15.5337939372807,-12.4105791850096,
117.358549826438)) ;
#162196=CARTESIAN_POINT('Ctrl Pts',(-15.5220396277674,-12.4764750890778,
117.322748096145)) ;
#162197=CARTESIAN_POINT('Ctrl Pts',(-15.6038717305927,-12.6535586984017,
117.536764515105)) ;
#162198=CARTESIAN_POINT('Ctrl Pts',(-15.5871151861937,-12.7071860625279,
117.485726784475)) ;
#162199=CARTESIAN_POINT('Ctrl Pts',(-15.6609190290941,-12.7071860605199,
117.461495741206)) ;
#162200=CARTESIAN_POINT('Ctrl Pts',(-15.7347228719945,-12.7071860585118,
117.437264697938)) ;
#162201=CARTESIAN_POINT('Ctrl Pts',(-15.7514794163935,-12.6535586943856,
117.488302428568)) ;
#162202=CARTESIAN_POINT('Ctrl Pts',(-15.7682359607925,-12.5999313302593,
117.539340159199)) ;
#162203=CARTESIAN_POINT('Ctrl Pts',(-15.6944321178921,-12.5999313322674,
117.563571202468)) ;
#162204=CARTESIAN_POINT('Ctrl Pts',(-15.6206282749917,-12.5999313342754,
117.587802245736)) ;
#162205=CARTESIAN_POINT('Ctrl Pts',(-15.6038717305927,-12.6535586984017,
117.536764515105)) ;
#162206=CARTESIAN_POINT('Ctrl Pts',(-15.6692705920402,-12.8875907025722,
117.700299247988)) ;
#162207=CARTESIAN_POINT('Ctrl Pts',(-15.648660558624,-12.9249550568961,
117.637524411639)) ;
#162208=CARTESIAN_POINT('Ctrl Pts',(-15.7224644022642,-12.9249550576415,
117.613293370624)) ;
#162209=CARTESIAN_POINT('Ctrl Pts',(-15.7962682459044,-12.9249550583868,
117.589062329609)) ;
#162210=CARTESIAN_POINT('Ctrl Pts',(-15.8168782793206,-12.887590704063,
117.651837165958)) ;
#162211=CARTESIAN_POINT('Ctrl Pts',(-15.8374883127368,-12.8502263497391,
117.714612002307)) ;
#162212=CARTESIAN_POINT('Ctrl Pts',(-15.7636844690966,-12.8502263489938,
117.738843043322)) ;
#162213=CARTESIAN_POINT('Ctrl Pts',(-15.6898806254564,-12.8502263482484,
117.763074084338)) ;
#162214=CARTESIAN_POINT('Ctrl Pts',(-15.6692705920402,-12.8875907025722,
117.700299247988)) ;
#162215=CARTESIAN_POINT('Ctrl Pts',(-15.7128057696858,-13.1564738506933,
117.797702690961)) ;
#162216=CARTESIAN_POINT('Ctrl Pts',(-15.6898544161461,-13.1751180004759,
117.727796571349)) ;
#162217=CARTESIAN_POINT('Ctrl Pts',(-15.7636582600179,-13.1751180045343,
117.703565531039)) ;
#162218=CARTESIAN_POINT('Ctrl Pts',(-15.8374621038898,-13.1751180085928,
117.67933449073)) ;
#162219=CARTESIAN_POINT('Ctrl Pts',(-15.8604134574295,-13.1564738588101,
117.749240610342)) ;
#162220=CARTESIAN_POINT('Ctrl Pts',(-15.8833648109692,-13.1378297090275,
117.819146729954)) ;
#162221=CARTESIAN_POINT('Ctrl Pts',(-15.8095609670974,-13.1378297049691,
117.843377770263)) ;
#162222=CARTESIAN_POINT('Ctrl Pts',(-15.7357571232256,-13.1378297009107,
117.867608810573)) ;
#162223=CARTESIAN_POINT('Ctrl Pts',(-15.7128057696858,-13.1564738506933,
117.797702690961)) ;
#162224=CARTESIAN_POINT('Ctrl Pts',(-15.7332548587096,-13.4476180482474,
117.824312090504)) ;
#162225=CARTESIAN_POINT('Ctrl Pts',(-15.709580261815,-13.4459601626287,
117.752203088467)) ;
#162226=CARTESIAN_POINT('Ctrl Pts',(-15.7833841053314,-13.4459601740975,
117.727972047075)) ;
#162227=CARTESIAN_POINT('Ctrl Pts',(-15.8571879488478,-13.4459601855664,
117.703741005682)) ;
#162228=CARTESIAN_POINT('Ctrl Pts',(-15.8808625457424,-13.4476180711851,
117.77585000772)) ;
#162229=CARTESIAN_POINT('Ctrl Pts',(-15.904537142637,-13.4492759568038,
117.847959009757)) ;
#162230=CARTESIAN_POINT('Ctrl Pts',(-15.8307332991206,-13.4492759453349,
117.872190051149)) ;
#162231=CARTESIAN_POINT('Ctrl Pts',(-15.7569294556042,-13.4492759338661,
117.896421092541)) ;
#162232=CARTESIAN_POINT('Ctrl Pts',(-15.7332548587096,-13.4476180482474,
117.824312090504)) ;
#162233=CARTESIAN_POINT('Ctrl Pts',(-15.7291353924876,-13.7346448783816,
117.776350799521)) ;
#162234=CARTESIAN_POINT('Ctrl Pts',(-15.7064469536668,-13.7129435340765,
117.707245475991)) ;
#162235=CARTESIAN_POINT('Ctrl Pts',(-15.7802507956075,-13.7129435517169,
117.6830144298)) ;
#162236=CARTESIAN_POINT('Ctrl Pts',(-15.8540546375481,-13.7129435693573,
117.658783383608)) ;
#162237=CARTESIAN_POINT('Ctrl Pts',(-15.8767430763689,-13.7346449136625,
117.727888707137)) ;
#162238=CARTESIAN_POINT('Ctrl Pts',(-15.8994315151896,-13.7563462579677,
117.796994030667)) ;
#162239=CARTESIAN_POINT('Ctrl Pts',(-15.8256276732489,-13.7563462403272,
117.821225076858)) ;
#162240=CARTESIAN_POINT('Ctrl Pts',(-15.7518238313083,-13.7563462226868,
117.84545612305)) ;
#162241=CARTESIAN_POINT('Ctrl Pts',(-15.7291353924876,-13.7346448783816,
117.776350799521)) ;
#162242=CARTESIAN_POINT('Ctrl Pts',(-15.7018297830167,-13.9993799399049,
117.657715317448)) ;
#162243=CARTESIAN_POINT('Ctrl Pts',(-15.6817489265485,-13.9591628378215,
117.596552269184)) ;
#162244=CARTESIAN_POINT('Ctrl Pts',(-15.7555527657976,-13.9591628601971,
117.572321214794)) ;
#162245=CARTESIAN_POINT('Ctrl Pts',(-15.8293566050468,-13.9591628825727,
117.548090160405)) ;
#162246=CARTESIAN_POINT('Ctrl Pts',(-15.849437461515,-13.9993799846561,
117.609253208669)) ;
#162247=CARTESIAN_POINT('Ctrl Pts',(-15.8695183179831,-14.0395970867396,
117.670416256934)) ;
#162248=CARTESIAN_POINT('Ctrl Pts',(-15.795714478734,-14.0395970643639,
117.694647311323)) ;
#162249=CARTESIAN_POINT('Ctrl Pts',(-15.7219106394849,-14.0395970419883,
117.718878365713)) ;
#162250=CARTESIAN_POINT('Ctrl Pts',(-15.7018297830167,-13.9993799399049,
117.657715317448)) ;
#162251=CARTESIAN_POINT('Ctrl Pts',(-15.6540905337258,-14.2219559568416,
117.476929036007)) ;
#162252=CARTESIAN_POINT('Ctrl Pts',(-15.6380460071677,-14.1661403968853,
117.428059997535)) ;
#162253=CARTESIAN_POINT('Ctrl Pts',(-15.7118498429771,-14.1661404199882,
117.403828932668)) ;
#162254=CARTESIAN_POINT('Ctrl Pts',(-15.7856536787865,-14.166140443091,
117.379597867802)) ;
#162255=CARTESIAN_POINT('Ctrl Pts',(-15.8016982053447,-14.2219560030472,
117.428466906274)) ;
#162256=CARTESIAN_POINT('Ctrl Pts',(-15.8177427319028,-14.2777715630035,
117.477335944747)) ;
#162257=CARTESIAN_POINT('Ctrl Pts',(-15.7439388960934,-14.2777715399007,
117.501567009613)) ;
#162258=CARTESIAN_POINT('Ctrl Pts',(-15.6701350602839,-14.2777715167979,
117.525798074479)) ;
#162259=CARTESIAN_POINT('Ctrl Pts',(-15.6540905337258,-14.2219559568416,
117.476929036007)) ;
#162260=CARTESIAN_POINT('Ctrl Pts',(-15.5899295337492,-14.3877271051732,
117.246044868715)) ;
#162261=CARTESIAN_POINT('Ctrl Pts',(-15.5790752953713,-14.3202567503196,
117.212984610756)) ;
#162262=CARTESIAN_POINT('Ctrl Pts',(-15.652879127185,-14.3202567702551,
117.188753533719)) ;
#162263=CARTESIAN_POINT('Ctrl Pts',(-15.7266829589986,-14.3202567901906,
117.164522456682)) ;
#162264=CARTESIAN_POINT('Ctrl Pts',(-15.7375371973765,-14.3877271450442,
117.197582714642)) ;
#162265=CARTESIAN_POINT('Ctrl Pts',(-15.7483914357544,-14.4551974998978,
117.230642972601)) ;
#162266=CARTESIAN_POINT('Ctrl Pts',(-15.6745876039407,-14.4551974799623,
117.254874049638)) ;
#162267=CARTESIAN_POINT('Ctrl Pts',(-15.6007837721271,-14.4551974600268,
117.279105126675)) ;
#162268=CARTESIAN_POINT('Ctrl Pts',(-15.5899295337492,-14.3877271051732,
117.246044868715)) ;
#162269=CARTESIAN_POINT('Ctrl Pts',(-15.5142887883934,-14.4840522417127,
116.980008252819)) ;
#162270=CARTESIAN_POINT('Ctrl Pts',(-15.5094376169318,-14.4097585017527,
116.965232368298)) ;
#162271=CARTESIAN_POINT('Ctrl Pts',(-15.583241444289,-14.4097585129656,
116.941001277688)) ;
#162272=CARTESIAN_POINT('Ctrl Pts',(-15.6570452716462,-14.4097585241785,
116.916770187077)) ;
#162273=CARTESIAN_POINT('Ctrl Pts',(-15.6618964431078,-14.4840522641385,
116.931546071598)) ;
#162274=CARTESIAN_POINT('Ctrl Pts',(-15.6667476145694,-14.5583460040984,
116.946321956118)) ;
#162275=CARTESIAN_POINT('Ctrl Pts',(-15.5929437872122,-14.5583459928856,
116.970553046728)) ;
#162276=CARTESIAN_POINT('Ctrl Pts',(-15.519139959855,-14.5583459816727,
116.994784137339)) ;
#162277=CARTESIAN_POINT('Ctrl Pts',(-15.5142887883934,-14.4840522417127,
116.980008252819)) ;
#162278=CARTESIAN_POINT('Ctrl Pts',(-15.4346677192972,-14.5035551456864,
116.702251625481)) ;
#162279=CARTESIAN_POINT('Ctrl Pts',(-15.4360978653644,-14.4277930448145,
116.706607620791)) ;
#162280=CARTESIAN_POINT('Ctrl Pts',(-15.5099016903547,-14.4277930415592,
116.682376522971)) ;
#162281=CARTESIAN_POINT('Ctrl Pts',(-15.583705515345,-14.427793038304,116.658145425152)) ;
#162282=CARTESIAN_POINT('Ctrl Pts',(-15.5822753692777,-14.503555139176,
116.653789429841)) ;
#162283=CARTESIAN_POINT('Ctrl Pts',(-15.5808452232104,-14.579317240048,
116.649433434531)) ;
#162284=CARTESIAN_POINT('Ctrl Pts',(-15.5070413982202,-14.5793172433032,
116.673664532351)) ;
#162285=CARTESIAN_POINT('Ctrl Pts',(-15.4332375732299,-14.5793172465584,
116.69789563017)) ;
#162286=CARTESIAN_POINT('Ctrl Pts',(-15.4346677192972,-14.5035551456864,
116.702251625481)) ;
#162287=CARTESIAN_POINT('Ctrl Pts',(-15.3559292275796,-14.4455933724693,
116.426856756554)) ;
#162288=CARTESIAN_POINT('Ctrl Pts',(-15.3635948048506,-14.3737681183539,
116.450204869409)) ;
#162289=CARTESIAN_POINT('Ctrl Pts',(-15.4373986280072,-14.3737680965987,
116.425973766004)) ;
#162290=CARTESIAN_POINT('Ctrl Pts',(-15.5112024511638,-14.3737680748436,
116.4017426626)) ;
#162291=CARTESIAN_POINT('Ctrl Pts',(-15.5035368738929,-14.445593328959,
116.378394549745)) ;
#162292=CARTESIAN_POINT('Ctrl Pts',(-15.4958712966219,-14.5174185830743,
116.355046436891)) ;
#162293=CARTESIAN_POINT('Ctrl Pts',(-15.4220674734653,-14.5174186048295,
116.379277540295)) ;
#162294=CARTESIAN_POINT('Ctrl Pts',(-15.3482636503086,-14.5174186265847,
116.4035086437)) ;
#162295=CARTESIAN_POINT('Ctrl Pts',(-15.3559292275796,-14.4455933724693,
116.426856756554)) ;
#162296=CARTESIAN_POINT('Ctrl Pts',(-15.285414304366,-14.3137077173971,
116.176599635695)) ;
#162297=CARTESIAN_POINT('Ctrl Pts',(-15.2987483150693,-14.2509862906075,
116.21721288234)) ;
#162298=CARTESIAN_POINT('Ctrl Pts',(-15.3725521387493,-14.2509862477117,
116.192981780529)) ;
#162299=CARTESIAN_POINT('Ctrl Pts',(-15.4463559624294,-14.2509862048158,
116.168750678719)) ;
#162300=CARTESIAN_POINT('Ctrl Pts',(-15.4330219517261,-14.3137076316054,
116.128137432075)) ;
#162301=CARTESIAN_POINT('Ctrl Pts',(-15.4196879410228,-14.3764290583951,
116.08752418543)) ;
#162302=CARTESIAN_POINT('Ctrl Pts',(-15.3458841173428,-14.3764291012909,
116.111755287241)) ;
#162303=CARTESIAN_POINT('Ctrl Pts',(-15.2720802936627,-14.3764291441867,
116.135986389051)) ;
#162304=CARTESIAN_POINT('Ctrl Pts',(-15.285414304366,-14.3137077173971,
116.176599635695)) ;
#162305=CARTESIAN_POINT('Ctrl Pts',(-15.2287932761951,-14.118290994482,
115.968741900664)) ;
#162306=CARTESIAN_POINT('Ctrl Pts',(-15.2468321761194,-14.0691221426053,
116.023685480875)) ;
#162307=CARTESIAN_POINT('Ctrl Pts',(-15.3206360026981,-14.0691220793387,
115.999454387893)) ;
#162308=CARTESIAN_POINT('Ctrl Pts',(-15.3944398292768,-14.0691220160722,
115.975223294912)) ;
#162309=CARTESIAN_POINT('Ctrl Pts',(-15.3764009293525,-14.1182908679489,
115.920279714701)) ;
#162310=CARTESIAN_POINT('Ctrl Pts',(-15.3583620294282,-14.1674597198256,
115.865336134491)) ;
#162311=CARTESIAN_POINT('Ctrl Pts',(-15.2845582028495,-14.1674597830921,
115.889567227472)) ;
#162312=CARTESIAN_POINT('Ctrl Pts',(-15.2107543762708,-14.1674598463587,
115.913798320454)) ;
#162313=CARTESIAN_POINT('Ctrl Pts',(-15.2287932761951,-14.118290994482,
115.968741900664)) ;
#162314=CARTESIAN_POINT('Ctrl Pts',(-15.190662017011,-13.8721339097932,
115.817104400349)) ;
#162315=CARTESIAN_POINT('Ctrl Pts',(-15.2121238291066,-13.840079359465,
115.882473618878)) ;
#162316=CARTESIAN_POINT('Ctrl Pts',(-15.2859276606813,-13.8400792780125,
115.858242541114)) ;
#162317=CARTESIAN_POINT('Ctrl Pts',(-15.3597314922561,-13.8400791965599,
115.83401146335)) ;
#162318=CARTESIAN_POINT('Ctrl Pts',(-15.3382696801605,-13.872133746888,
115.76864224482)) ;
#162319=CARTESIAN_POINT('Ctrl Pts',(-15.316807868065,-13.9041882972162,
115.703273026291)) ;
#162320=CARTESIAN_POINT('Ctrl Pts',(-15.2430040364902,-13.9041883786687,
115.727504104055)) ;
#162321=CARTESIAN_POINT('Ctrl Pts',(-15.1692002049154,-13.9041884601213,
115.75173518182)) ;
#162322=CARTESIAN_POINT('Ctrl Pts',(-15.190662017011,-13.8721339097932,
115.817104400349)) ;
#162323=CARTESIAN_POINT('Ctrl Pts',(-15.1746169230128,-13.5943341067766,
115.732853741077)) ;
#162324=CARTESIAN_POINT('Ctrl Pts',(-15.1979622079392,-13.5816279445403,
115.803959714053)) ;
#162325=CARTESIAN_POINT('Ctrl Pts',(-15.2717660463982,-13.5816278507647,
115.779728657256)) ;
#162326=CARTESIAN_POINT('Ctrl Pts',(-15.3455698848571,-13.5816277569891,
115.75549760046)) ;
#162327=CARTESIAN_POINT('Ctrl Pts',(-15.3222245999306,-13.5943339192254,
115.684391627484)) ;
#162328=CARTESIAN_POINT('Ctrl Pts',(-15.2988793150042,-13.6070400814617,
115.613285654508)) ;
#162329=CARTESIAN_POINT('Ctrl Pts',(-15.2250754765453,-13.6070401752373,
115.637516711305)) ;
#162330=CARTESIAN_POINT('Ctrl Pts',(-15.1512716380863,-13.6070402690129,
115.661747768101)) ;
#162331=CARTESIAN_POINT('Ctrl Pts',(-15.1746169230128,-13.5943341067766,
115.732853741077)) ;
#162332=CARTESIAN_POINT('Ctrl Pts',(-15.1826673766295,-13.3016132059809,
115.721705106696)) ;
#162333=CARTESIAN_POINT('Ctrl Pts',(-15.2062229726213,-13.309324862532,
115.793451653354)) ;
#162334=CARTESIAN_POINT('Ctrl Pts',(-15.2800268192901,-13.3093247622356,
115.769220621564)) ;
#162335=CARTESIAN_POINT('Ctrl Pts',(-15.3538306659589,-13.3093246619392,
115.744989589774)) ;
#162336=CARTESIAN_POINT('Ctrl Pts',(-15.3302750699671,-13.3016130053881,
115.673243043115)) ;
#162337=CARTESIAN_POINT('Ctrl Pts',(-15.3067194739753,-13.293901348837,
115.601496496456)) ;
#162338=CARTESIAN_POINT('Ctrl Pts',(-15.2329156273065,-13.2939014491334,
115.625727528247)) ;
#162339=CARTESIAN_POINT('Ctrl Pts',(-15.1591117806377,-13.2939015494298,
115.649958560037)) ;
#162340=CARTESIAN_POINT('Ctrl Pts',(-15.1826673766295,-13.3016132059809,
115.721705106696)) ;
#162341=CARTESIAN_POINT('Ctrl Pts',(-15.2146933752457,-13.0203974601351,
115.783981898111)) ;
#162342=CARTESIAN_POINT('Ctrl Pts',(-15.2367771372747,-13.0477539673653,
115.851245476052)) ;
#162343=CARTESIAN_POINT('Ctrl Pts',(-15.3105809924454,-13.0477538708474,
115.827014470158)) ;
#162344=CARTESIAN_POINT('Ctrl Pts',(-15.3843848476162,-13.0477537743296,
115.802783464263)) ;
#162345=CARTESIAN_POINT('Ctrl Pts',(-15.3623010855873,-13.0203972670994,
115.735519886322)) ;
#162346=CARTESIAN_POINT('Ctrl Pts',(-15.3402173235583,-12.9930407598692,
115.668256308381)) ;
#162347=CARTESIAN_POINT('Ctrl Pts',(-15.2664134683876,-12.9930408563871,
115.692487314276)) ;
#162348=CARTESIAN_POINT('Ctrl Pts',(-15.1926096132168,-12.9930409529049,
115.71671832017)) ;
#162349=CARTESIAN_POINT('Ctrl Pts',(-15.2146933752457,-13.0203974601351,
115.783981898111)) ;
#162350=CARTESIAN_POINT('Ctrl Pts',(-15.269404025713,-12.7657619407627,
115.915129891759)) ;
#162351=CARTESIAN_POINT('Ctrl Pts',(-15.2884349716493,-12.8109362194434,
115.973095084508)) ;
#162352=CARTESIAN_POINT('Ctrl Pts',(-15.362238834935,-12.8109361340697,
115.948864103331)) ;
#162353=CARTESIAN_POINT('Ctrl Pts',(-15.4360426982208,-12.810936048696,
115.924633122153)) ;
#162354=CARTESIAN_POINT('Ctrl Pts',(-15.4170117522845,-12.7657617700153,
115.866667929404)) ;
#162355=CARTESIAN_POINT('Ctrl Pts',(-15.3979808063481,-12.7205874913346,
115.808702736655)) ;
#162356=CARTESIAN_POINT('Ctrl Pts',(-15.3241769430624,-12.7205875767083,
115.832933717832)) ;
#162357=CARTESIAN_POINT('Ctrl Pts',(-15.2503730797767,-12.720587662082,
115.85716469901)) ;
#162358=CARTESIAN_POINT('Ctrl Pts',(-15.269404025713,-12.7657619407627,
115.915129891759)) ;
#162359=CARTESIAN_POINT('Ctrl Pts',(-15.3438708491905,-12.5577255499837,
116.10637631446)) ;
#162360=CARTESIAN_POINT('Ctrl Pts',(-15.3584669209644,-12.6174909098253,
116.150833596105)) ;
#162361=CARTESIAN_POINT('Ctrl Pts',(-15.4322707910339,-12.6174908436088,
116.12660263559)) ;
#162362=CARTESIAN_POINT('Ctrl Pts',(-15.5060746611033,-12.6174907773923,
116.102371675074)) ;
#162363=CARTESIAN_POINT('Ctrl Pts',(-15.4914785893295,-12.5577254175507,
116.057914393429)) ;
#162364=CARTESIAN_POINT('Ctrl Pts',(-15.4768825175556,-12.497960057709,
116.013457111784)) ;
#162365=CARTESIAN_POINT('Ctrl Pts',(-15.4030786474862,-12.4979601239256,
116.0376880723)) ;
#162366=CARTESIAN_POINT('Ctrl Pts',(-15.3292747774167,-12.4979601901421,
116.061919032815)) ;
#162367=CARTESIAN_POINT('Ctrl Pts',(-15.3438708491905,-12.5577255499837,
116.10637631446)) ;
#162368=CARTESIAN_POINT('Ctrl Pts',(-15.4327636159981,-12.4120606642955,
116.34175086754)) ;
#162369=CARTESIAN_POINT('Ctrl Pts',(-15.4419070935897,-12.4820840248362,
116.369600427087)) ;
#162370=CARTESIAN_POINT('Ctrl Pts',(-15.5157109682969,-12.482083983576,
116.345369480697)) ;
#162371=CARTESIAN_POINT('Ctrl Pts',(-15.5895148430041,-12.4820839423157,
116.321138534307)) ;
#162372=CARTESIAN_POINT('Ctrl Pts',(-15.5803713654125,-12.412060581775,
116.293288974761)) ;
#162373=CARTESIAN_POINT('Ctrl Pts',(-15.5712278878209,-12.3420372212343,
116.265439415215)) ;
#162374=CARTESIAN_POINT('Ctrl Pts',(-15.4974240131137,-12.3420372624946,
116.289670361605)) ;
#162375=CARTESIAN_POINT('Ctrl Pts',(-15.4236201384065,-12.3420373037548,
116.313901307994)) ;
#162376=CARTESIAN_POINT('Ctrl Pts',(-15.4327636159981,-12.4120606642955,
116.34175086754)) ;
#162377=CARTESIAN_POINT('Ctrl Pts',(-15.5316685213714,-12.3380220880362,
116.60734315125)) ;
#162378=CARTESIAN_POINT('Ctrl Pts',(-15.5346582890961,-12.4133190427032,
116.616449503417)) ;
#162379=CARTESIAN_POINT('Ctrl Pts',(-15.6084621657583,-12.4133190298849,
116.592218562982)) ;
#162380=CARTESIAN_POINT('Ctrl Pts',(-15.6822660424204,-12.4133190170666,
116.567987622547)) ;
#162381=CARTESIAN_POINT('Ctrl Pts',(-15.6792762746957,-12.3380220623996,
116.558881270379)) ;
#162382=CARTESIAN_POINT('Ctrl Pts',(-15.676286506971,-12.2627251077326,
116.549774918212)) ;
#162383=CARTESIAN_POINT('Ctrl Pts',(-15.6024826303088,-12.2627251205509,
116.574005858647)) ;
#162384=CARTESIAN_POINT('Ctrl Pts',(-15.5286787536467,-12.2627251333692,
116.598236799083)) ;
#162385=CARTESIAN_POINT('Ctrl Pts',(-15.5316685213714,-12.3380220880362,
116.60734315125)) ;
#162386=CARTESIAN_POINT('Ctrl Pts',(-15.6323103361434,-12.3416277493325,
116.878663222145)) ;
#162387=CARTESIAN_POINT('Ctrl Pts',(-15.629006691363,-12.4167843477481,
116.868600855232)) ;
#162388=CARTESIAN_POINT('Ctrl Pts',(-15.7028105674402,-12.4167843633384,
116.844369913015)) ;
#162389=CARTESIAN_POINT('Ctrl Pts',(-15.7766144435173,-12.4167843789286,
116.820138970798)) ;
#162390=CARTESIAN_POINT('Ctrl Pts',(-15.7799180882977,-12.3416277805131,
116.830201337711)) ;
#162391=CARTESIAN_POINT('Ctrl Pts',(-15.7832217330782,-12.2664711820975,
116.840263704625)) ;
#162392=CARTESIAN_POINT('Ctrl Pts',(-15.709417857001,-12.2664711665072,
116.864494646842)) ;
#162393=CARTESIAN_POINT('Ctrl Pts',(-15.6356139809238,-12.266471150917,
116.888725589059)) ;
#162394=CARTESIAN_POINT('Ctrl Pts',(-15.6323103361434,-12.3416277493325,
116.878663222145)) ;
#162395=CARTESIAN_POINT('Ctrl Pts',(-15.7303191792415,-12.4221117178776,
117.141642652826)) ;
#162396=CARTESIAN_POINT('Ctrl Pts',(-15.7209033300313,-12.4917616411482,
117.112963497359)) ;
#162397=CARTESIAN_POINT('Ctrl Pts',(-15.7947072027341,-12.4917616828604,
117.088732544865)) ;
#162398=CARTESIAN_POINT('Ctrl Pts',(-15.868511075437,-12.4917617245726,
117.06450159237)) ;
#162399=CARTESIAN_POINT('Ctrl Pts',(-15.8779269246473,-12.422111801302,
117.093180747837)) ;
#162400=CARTESIAN_POINT('Ctrl Pts',(-15.8873427738576,-12.3524618780314,
117.121859903304)) ;
#162401=CARTESIAN_POINT('Ctrl Pts',(-15.8135389011547,-12.3524618363192,
117.146090855799)) ;
#162402=CARTESIAN_POINT('Ctrl Pts',(-15.7397350284518,-12.3524617946069,
117.170321808294)) ;
#162403=CARTESIAN_POINT('Ctrl Pts',(-15.7303191792415,-12.4221117178776,
117.141642652826)) ;
#162404=CARTESIAN_POINT('Ctrl Pts',(-15.818253094992,-12.5739000669618,
117.37404115853)) ;
#162405=CARTESIAN_POINT('Ctrl Pts',(-15.8034170204807,-12.6330567654726,
117.32885287127)) ;
#162406=CARTESIAN_POINT('Ctrl Pts',(-15.8772208877114,-12.6330568281404,
117.304621902107)) ;
#162407=CARTESIAN_POINT('Ctrl Pts',(-15.951024754942,-12.6330568908083,
117.280390932945)) ;
#162408=CARTESIAN_POINT('Ctrl Pts',(-15.9658608294533,-12.5739001922976,
117.325579220205)) ;
#162409=CARTESIAN_POINT('Ctrl Pts',(-15.9806969039645,-12.5147434937868,
117.370767507466)) ;
#162410=CARTESIAN_POINT('Ctrl Pts',(-15.9068930367339,-12.5147434311189,
117.394998476628)) ;
#162411=CARTESIAN_POINT('Ctrl Pts',(-15.8330891695033,-12.5147433684511,
117.41922944579)) ;
#162412=CARTESIAN_POINT('Ctrl Pts',(-15.818253094992,-12.5739000669618,
117.37404115853)) ;
#162413=CARTESIAN_POINT('Ctrl Pts',(-15.8910677122169,-12.7865530350162,
117.560294460758)) ;
#162414=CARTESIAN_POINT('Ctrl Pts',(-15.8718607305365,-12.830951855475,
117.5017930954)) ;
#162415=CARTESIAN_POINT('Ctrl Pts',(-15.9456645907029,-12.8309519318751,
117.477562104721)) ;
#162416=CARTESIAN_POINT('Ctrl Pts',(-16.0194684508694,-12.8309520082752,
117.453331114042)) ;
#162417=CARTESIAN_POINT('Ctrl Pts',(-16.0386754325498,-12.7865531878164,
117.511832479401)) ;
#162418=CARTESIAN_POINT('Ctrl Pts',(-16.0578824142302,-12.7421543673576,
117.57033384476)) ;
#162419=CARTESIAN_POINT('Ctrl Pts',(-15.9840785540637,-12.7421542909575,
117.594564835438)) ;
#162420=CARTESIAN_POINT('Ctrl Pts',(-15.9102746938973,-12.7421542145574,
117.618795826117)) ;
#162421=CARTESIAN_POINT('Ctrl Pts',(-15.8910677122169,-12.7865530350162,
117.560294460758)) ;
#162422=CARTESIAN_POINT('Ctrl Pts',(-15.943961350988,-13.044698151263,117.685874037695)) ;
#162423=CARTESIAN_POINT('Ctrl Pts',(-15.921767547098,-13.071140713464,117.618275293682)) ;
#162424=CARTESIAN_POINT('Ctrl Pts',(-15.9955713996357,-13.0711407952517,
117.594044279767)) ;
#162425=CARTESIAN_POINT('Ctrl Pts',(-16.0693752521733,-13.0711408770393,
117.569813265852)) ;
#162426=CARTESIAN_POINT('Ctrl Pts',(-16.0915690560633,-13.0446983148383,
117.637412009865)) ;
#162427=CARTESIAN_POINT('Ctrl Pts',(-16.1137628599533,-13.0182557526373,
117.705010753878)) ;
#162428=CARTESIAN_POINT('Ctrl Pts',(-16.0399590074156,-13.0182556708497,
117.729241767793)) ;
#162429=CARTESIAN_POINT('Ctrl Pts',(-15.966155154878,-13.018255589062,117.753472781708)) ;
#162430=CARTESIAN_POINT('Ctrl Pts',(-15.943961350988,-13.044698151263,117.685874037695)) ;
#162431=CARTESIAN_POINT('Ctrl Pts',(-15.973861910085,-13.328059924083,117.741608955228)) ;
#162432=CARTESIAN_POINT('Ctrl Pts',(-15.9502783076643,-13.33475818736,117.669777109021)) ;
#162433=CARTESIAN_POINT('Ctrl Pts',(-16.024082152983,-13.3347582681445,
117.645546073119)) ;
#162434=CARTESIAN_POINT('Ctrl Pts',(-16.0978859983017,-13.334758348929,
117.621315037216)) ;
#162435=CARTESIAN_POINT('Ctrl Pts',(-16.1214696007224,-13.328060085652,
117.693146883423)) ;
#162436=CARTESIAN_POINT('Ctrl Pts',(-16.145053203143,-13.321361822375,117.764978729631)) ;
#162437=CARTESIAN_POINT('Ctrl Pts',(-16.0712493578243,-13.3213617415905,
117.789209765533)) ;
#162438=CARTESIAN_POINT('Ctrl Pts',(-15.9974455125056,-13.321361660806,
117.813440801436)) ;
#162439=CARTESIAN_POINT('Ctrl Pts',(-15.973861910085,-13.328059924083,117.741608955228)) ;
#162440=CARTESIAN_POINT('Ctrl Pts',(-15.9797490331987,-13.6187777866059,
117.724086355187)) ;
#162441=CARTESIAN_POINT('Ctrl Pts',(-15.9564523748508,-13.6051885128316,
117.653128494185)) ;
#162442=CARTESIAN_POINT('Ctrl Pts',(-16.0302562137773,-13.6051885851199,
117.628897438813)) ;
#162443=CARTESIAN_POINT('Ctrl Pts',(-16.1040600527037,-13.6051886574082,
117.604666383441)) ;
#162444=CARTESIAN_POINT('Ctrl Pts',(-16.1273567110516,-13.6187779311824,
117.675624244442)) ;
#162445=CARTESIAN_POINT('Ctrl Pts',(-16.1506533693995,-13.6323672049567,
117.746582105443)) ;
#162446=CARTESIAN_POINT('Ctrl Pts',(-16.0768495304731,-13.6323671326684,
117.770813160816)) ;
#162447=CARTESIAN_POINT('Ctrl Pts',(-16.0030456915466,-13.6323670603802,
117.795044216188)) ;
#162448=CARTESIAN_POINT('Ctrl Pts',(-15.9797490331987,-13.6187777866059,
117.724086355187)) ;
#162449=CARTESIAN_POINT('Ctrl Pts',(-15.9616058932464,-13.8959727795492,
117.633255070877)) ;
#162450=CARTESIAN_POINT('Ctrl Pts',(-15.9402766412006,-13.863009115872,
117.568289611858)) ;
#162451=CARTESIAN_POINT('Ctrl Pts',(-16.0140804755236,-13.8630091736306,
117.544058542464)) ;
#162452=CARTESIAN_POINT('Ctrl Pts',(-16.0878843098467,-13.8630092313891,
117.519827473071)) ;
#162453=CARTESIAN_POINT('Ctrl Pts',(-16.1092135618925,-13.8959728950663,
117.58479293209)) ;
#162454=CARTESIAN_POINT('Ctrl Pts',(-16.1305428139384,-13.9289365587434,
117.64975839111)) ;
#162455=CARTESIAN_POINT('Ctrl Pts',(-16.0567389796153,-13.9289365009848,
117.673989460503)) ;
#162456=CARTESIAN_POINT('Ctrl Pts',(-15.9829351452922,-13.9289364432263,
117.698220529897)) ;
#162457=CARTESIAN_POINT('Ctrl Pts',(-15.9616058932464,-13.8959727795492,
117.633255070877)) ;
#162458=CARTESIAN_POINT('Ctrl Pts',(-15.92165968614,-14.1380897314584,117.476125293794)) ;
#162459=CARTESIAN_POINT('Ctrl Pts',(-15.9038209335532,-14.0881713161907,
117.421791332774)) ;
#162460=CARTESIAN_POINT('Ctrl Pts',(-15.9776247651568,-14.0881713577831,
117.397560255097)) ;
#162461=CARTESIAN_POINT('Ctrl Pts',(-16.0514285967603,-14.0881713993755,
117.37332917742)) ;
#162462=CARTESIAN_POINT('Ctrl Pts',(-16.0692673493471,-14.1380898146432,
117.427663138441)) ;
#162463=CARTESIAN_POINT('Ctrl Pts',(-16.0871061019338,-14.1880082299108,
117.481997099461)) ;
#162464=CARTESIAN_POINT('Ctrl Pts',(-16.0133022703303,-14.1880081883184,
117.506228177138)) ;
#162465=CARTESIAN_POINT('Ctrl Pts',(-15.9394984387268,-14.188008146726,
117.530459254814)) ;
#162466=CARTESIAN_POINT('Ctrl Pts',(-15.92165968614,-14.1380897314584,117.476125293794)) ;
#162467=CARTESIAN_POINT('Ctrl Pts',(-15.8633008249773,-14.3289912800735,
117.262814844311)) ;
#162468=CARTESIAN_POINT('Ctrl Pts',(-15.8502454740091,-14.2656678675504,
117.223050352636)) ;
#162469=CARTESIAN_POINT('Ctrl Pts',(-15.9240493051082,-14.2656678924027,
117.198819273423)) ;
#162470=CARTESIAN_POINT('Ctrl Pts',(-15.9978531362073,-14.2656679172549,
117.17458819421)) ;
#162471=CARTESIAN_POINT('Ctrl Pts',(-16.0109084871756,-14.3289913297781,
117.214352685885)) ;
#162472=CARTESIAN_POINT('Ctrl Pts',(-16.0239638381439,-14.3923147423012,
117.25411717756)) ;
#162473=CARTESIAN_POINT('Ctrl Pts',(-15.9501600070448,-14.3923147174489,
117.278348256773)) ;
#162474=CARTESIAN_POINT('Ctrl Pts',(-15.8763561759456,-14.3923146925966,
117.302579335987)) ;
#162475=CARTESIAN_POINT('Ctrl Pts',(-15.8633008249773,-14.3289912800735,
117.262814844311)) ;
#162476=CARTESIAN_POINT('Ctrl Pts',(-15.7921118917969,-14.4536834307714,
117.01067142375)) ;
#162477=CARTESIAN_POINT('Ctrl Pts',(-15.7847381201067,-14.3815580790825,
116.988212105697)) ;
#162478=CARTESIAN_POINT('Ctrl Pts',(-15.8585419517498,-14.381558090492,
116.963981028141)) ;
#162479=CARTESIAN_POINT('Ctrl Pts',(-15.9323457833928,-14.3815581019016,
116.939749950584)) ;
#162480=CARTESIAN_POINT('Ctrl Pts',(-15.9397195550829,-14.4536834535906,
116.962209268637)) ;
#162481=CARTESIAN_POINT('Ctrl Pts',(-15.947093326773,-14.5258088052795,
116.984668586689)) ;
#162482=CARTESIAN_POINT('Ctrl Pts',(-15.87328949513,-14.52580879387,117.008899664246)) ;
#162483=CARTESIAN_POINT('Ctrl Pts',(-15.799485663487,-14.5258087824604,
117.033130741802)) ;
#162484=CARTESIAN_POINT('Ctrl Pts',(-15.7921118917969,-14.4536834307714,
117.01067142375)) ;
#162485=CARTESIAN_POINT('Ctrl Pts',(-15.7132086075603,-14.5050447602448,
116.734875307883)) ;
#162486=CARTESIAN_POINT('Ctrl Pts',(-15.7120668798563,-14.4292238155188,
116.731397790109)) ;
#162487=CARTESIAN_POINT('Ctrl Pts',(-15.7858707136532,-14.4292238160263,
116.707166719113)) ;
#162488=CARTESIAN_POINT('Ctrl Pts',(-15.8596745474501,-14.4292238165338,
116.682935648117)) ;
#162489=CARTESIAN_POINT('Ctrl Pts',(-15.8608162751541,-14.5050447612597,
116.686413165891)) ;
#162490=CARTESIAN_POINT('Ctrl Pts',(-15.8619580028581,-14.5808657059856,
116.689890683665)) ;
#162491=CARTESIAN_POINT('Ctrl Pts',(-15.7881541690612,-14.5808657054781,
116.714121754661)) ;
#162492=CARTESIAN_POINT('Ctrl Pts',(-15.7143503352643,-14.5808657049707,
116.738352825657)) ;
#162493=CARTESIAN_POINT('Ctrl Pts',(-15.7132086075603,-14.5050447602448,
116.734875307883)) ;
#162494=CARTESIAN_POINT('Ctrl Pts',(-15.6332196110999,-14.4782940097224,
116.455753006044)) ;
#162495=CARTESIAN_POINT('Ctrl Pts',(-15.6383957039192,-14.4042259752822,
116.471518550047)) ;
#162496=CARTESIAN_POINT('Ctrl Pts',(-15.7121995405475,-14.4042259695799,
116.447287487674)) ;
#162497=CARTESIAN_POINT('Ctrl Pts',(-15.7860033771757,-14.4042259638776,
116.423056425302)) ;
#162498=CARTESIAN_POINT('Ctrl Pts',(-15.7808272843565,-14.4782939983178,
116.4072908813)) ;
#162499=CARTESIAN_POINT('Ctrl Pts',(-15.7756511915372,-14.552362032758,
116.391525337298)) ;
#162500=CARTESIAN_POINT('Ctrl Pts',(-15.7018473549089,-14.5523620384603,
116.41575639967)) ;
#162501=CARTESIAN_POINT('Ctrl Pts',(-15.6280435182807,-14.5523620441626,
116.439987462042)) ;
#162502=CARTESIAN_POINT('Ctrl Pts',(-15.6332196110999,-14.4782940097224,
116.455753006044)) ;
#162503=CARTESIAN_POINT('Ctrl Pts',(-15.5587696998728,-14.3758709565101,
116.193557985972)) ;
#162504=CARTESIAN_POINT('Ctrl Pts',(-15.5698852741414,-14.3088425929799,
116.227414231996)) ;
#162505=CARTESIAN_POINT('Ctrl Pts',(-15.6436891134963,-14.3088425851836,
116.203183177928)) ;
#162506=CARTESIAN_POINT('Ctrl Pts',(-15.7174929528511,-14.3088425773873,
116.17895212386)) ;
#162507=CARTESIAN_POINT('Ctrl Pts',(-15.7063773785825,-14.3758709409175,
116.145095877837)) ;
#162508=CARTESIAN_POINT('Ctrl Pts',(-15.6952618043138,-14.4428993044478,
116.111239631813)) ;
#162509=CARTESIAN_POINT('Ctrl Pts',(-15.621457964959,-14.442899312244,116.13547068588)) ;
#162510=CARTESIAN_POINT('Ctrl Pts',(-15.5476541256042,-14.4428993200403,
116.159701739948)) ;
#162511=CARTESIAN_POINT('Ctrl Pts',(-15.5587696998728,-14.3758709565101,
116.193557985972)) ;
#162512=CARTESIAN_POINT('Ctrl Pts',(-15.4956323923376,-14.2038414128419,
115.965654894124)) ;
#162513=CARTESIAN_POINT('Ctrl Pts',(-15.5119101272549,-14.1487238719563,
116.015234248429)) ;
#162514=CARTESIAN_POINT('Ctrl Pts',(-15.5857139690308,-14.1487238662438,
115.991003201736)) ;
#162515=CARTESIAN_POINT('Ctrl Pts',(-15.6595178108066,-14.1487238605313,
115.966772155042)) ;
#162516=CARTESIAN_POINT('Ctrl Pts',(-15.6432400758893,-14.2038414014169,
115.917192800737)) ;
#162517=CARTESIAN_POINT('Ctrl Pts',(-15.6269623409719,-14.2589589423024,
115.867613446432)) ;
#162518=CARTESIAN_POINT('Ctrl Pts',(-15.553158499196,-14.2589589480149,
115.891844493126)) ;
#162519=CARTESIAN_POINT('Ctrl Pts',(-15.4793546574202,-14.2589589537274,
115.91607553982)) ;
#162520=CARTESIAN_POINT('Ctrl Pts',(-15.4956323923376,-14.2038414128419,
115.965654894124)) ;
#162521=CARTESIAN_POINT('Ctrl Pts',(-15.4497236558171,-13.9777022974474,
115.790578372436)) ;
#162522=CARTESIAN_POINT('Ctrl Pts',(-15.469960680649,-13.9382924680263,
115.85221708491)) ;
#162523=CARTESIAN_POINT('Ctrl Pts',(-15.5437645236048,-13.9382924647888,
115.827986041811)) ;
#162524=CARTESIAN_POINT('Ctrl Pts',(-15.6175683665605,-13.9382924615514,
115.803754998711)) ;
#162525=CARTESIAN_POINT('Ctrl Pts',(-15.5973313417286,-13.9777022909725,
115.742116286236)) ;
#162526=CARTESIAN_POINT('Ctrl Pts',(-15.5770943168967,-14.0171121203935,
115.680477573762)) ;
#162527=CARTESIAN_POINT('Ctrl Pts',(-15.503290473941,-14.017112123631,115.704708616861)) ;
#162528=CARTESIAN_POINT('Ctrl Pts',(-15.4294866309852,-14.0171121268685,
115.728939659961)) ;
#162529=CARTESIAN_POINT('Ctrl Pts',(-15.4497236558171,-13.9777022974474,
115.790578372436)) ;
#162530=CARTESIAN_POINT('Ctrl Pts',(-15.4242298945828,-13.7081471730545,
115.677198196239)) ;
#162531=CARTESIAN_POINT('Ctrl Pts',(-15.4470171331945,-13.6875008672276,
115.746604448313)) ;
#162532=CARTESIAN_POINT('Ctrl Pts',(-15.5208209768319,-13.6875008686463,
115.722373407289)) ;
#162533=CARTESIAN_POINT('Ctrl Pts',(-15.5946248204693,-13.687500870065,
115.698142366266)) ;
#162534=CARTESIAN_POINT('Ctrl Pts',(-15.5718375818576,-13.7081471758919,
115.628736114192)) ;
#162535=CARTESIAN_POINT('Ctrl Pts',(-15.5490503432458,-13.7287934817188,
115.559329862118)) ;
#162536=CARTESIAN_POINT('Ctrl Pts',(-15.4752464996084,-13.7287934803001,
115.583560903142)) ;
#162537=CARTESIAN_POINT('Ctrl Pts',(-15.401442655971,-13.7287934788814,
115.607791944166)) ;
#162538=CARTESIAN_POINT('Ctrl Pts',(-15.4242298945828,-13.7081471730545,
115.677198196239)) ;
#162539=CARTESIAN_POINT('Ctrl Pts',(-15.4224756486748,-13.4207218926891,
115.636530543552)) ;
#162540=CARTESIAN_POINT('Ctrl Pts',(-15.4461502225077,-13.4201152017274,
115.70863947551)) ;
#162541=CARTESIAN_POINT('Ctrl Pts',(-15.5199540659324,-13.4201152047761,
115.684408433839)) ;
#162542=CARTESIAN_POINT('Ctrl Pts',(-15.593757909357,-13.4201152078248,
115.660177392167)) ;
#162543=CARTESIAN_POINT('Ctrl Pts',(-15.5700833355241,-13.4207218987865,
115.588068460209)) ;
#162544=CARTESIAN_POINT('Ctrl Pts',(-15.5464087616913,-13.4213285897482,
115.515959528251)) ;
#162545=CARTESIAN_POINT('Ctrl Pts',(-15.4726049182666,-13.4213285866995,
115.540190569923)) ;
#162546=CARTESIAN_POINT('Ctrl Pts',(-15.398801074842,-13.4213285836508,
115.564421611594)) ;
#162547=CARTESIAN_POINT('Ctrl Pts',(-15.4224756486748,-13.4207218926891,
115.636530543552)) ;
#162548=CARTESIAN_POINT('Ctrl Pts',(-15.4448455283626,-13.1323473586493,
115.669233043994)) ;
#162549=CARTESIAN_POINT('Ctrl Pts',(-15.4677263606914,-13.1518767361785,
115.738924367398)) ;
#162550=CARTESIAN_POINT('Ctrl Pts',(-15.541530203822,-13.1518767392038,
115.714693324831)) ;
#162551=CARTESIAN_POINT('Ctrl Pts',(-15.6153340469527,-13.1518767422291,
115.690462282264)) ;
#162552=CARTESIAN_POINT('Ctrl Pts',(-15.592453214624,-13.1323473646999,
115.62077095886)) ;
#162553=CARTESIAN_POINT('Ctrl Pts',(-15.5695723822952,-13.1128179871707,
115.551079635456)) ;
#162554=CARTESIAN_POINT('Ctrl Pts',(-15.4957685391646,-13.1128179841454,
115.575310678023)) ;
#162555=CARTESIAN_POINT('Ctrl Pts',(-15.4219646960339,-13.1128179811201,
115.59954172059)) ;
#162556=CARTESIAN_POINT('Ctrl Pts',(-15.4448455283626,-13.1323473586493,
115.669233043994)) ;
#162557=CARTESIAN_POINT('Ctrl Pts',(-15.4907259221535,-12.8640039527127,
115.773502605509)) ;
#162558=CARTESIAN_POINT('Ctrl Pts',(-15.5111708603039,-12.9022999989721,
115.835774588317)) ;
#162559=CARTESIAN_POINT('Ctrl Pts',(-15.5849747034648,-12.9022999996752,
115.811543545842)) ;
#162560=CARTESIAN_POINT('Ctrl Pts',(-15.6587785466256,-12.9023000003783,
115.787312503367)) ;
#162561=CARTESIAN_POINT('Ctrl Pts',(-15.6383336084751,-12.8640039541189,
115.725040520558)) ;
#162562=CARTESIAN_POINT('Ctrl Pts',(-15.6178886703247,-12.8257079078595,
115.66276853775)) ;
#162563=CARTESIAN_POINT('Ctrl Pts',(-15.5440848271639,-12.8257079071564,
115.686999580226)) ;
#162564=CARTESIAN_POINT('Ctrl Pts',(-15.4702809840031,-12.8257079064533,
115.711230622701)) ;
#162565=CARTESIAN_POINT('Ctrl Pts',(-15.4907259221535,-12.8640039527127,
115.773502605509)) ;
#162566=CARTESIAN_POINT('Ctrl Pts',(-15.5576964345495,-12.6351955964259,
115.941952413121)) ;
#162567=CARTESIAN_POINT('Ctrl Pts',(-15.5742303280639,-12.6895248162975,
115.992311985098)) ;
#162568=CARTESIAN_POINT('Ctrl Pts',(-15.6480341721483,-12.6895248136964,
115.968080945436)) ;
#162569=CARTESIAN_POINT('Ctrl Pts',(-15.7218380162327,-12.6895248110954,
115.943849905773)) ;
#162570=CARTESIAN_POINT('Ctrl Pts',(-15.7053041227182,-12.6351955912238,
115.893490333797)) ;
#162571=CARTESIAN_POINT('Ctrl Pts',(-15.6887702292038,-12.5808663713523,
115.84313076182)) ;
#162572=CARTESIAN_POINT('Ctrl Pts',(-15.6149663851194,-12.5808663739533,
115.867361801483)) ;
#162573=CARTESIAN_POINT('Ctrl Pts',(-15.541162541035,-12.5808663765543,
115.891592841145)) ;
#162574=CARTESIAN_POINT('Ctrl Pts',(-15.5576964345495,-12.6351955964259,
115.941952413121)) ;
#162575=CARTESIAN_POINT('Ctrl Pts',(-15.6410494594336,-12.4633049543151,
116.160508256525)) ;
#162576=CARTESIAN_POINT('Ctrl Pts',(-15.6525183306037,-12.5297151872054,
116.195440587766)) ;
#162577=CARTESIAN_POINT('Ctrl Pts',(-15.7263221760862,-12.5297151829142,
116.171209552362)) ;
#162578=CARTESIAN_POINT('Ctrl Pts',(-15.8001260215687,-12.529715178623,
116.146978516958)) ;
#162579=CARTESIAN_POINT('Ctrl Pts',(-15.7886571503986,-12.4633049457328,
116.112046185718)) ;
#162580=CARTESIAN_POINT('Ctrl Pts',(-15.7771882792285,-12.3968947128425,
116.077113854477)) ;
#162581=CARTESIAN_POINT('Ctrl Pts',(-15.703384433746,-12.3968947171337,
116.101344889881)) ;
#162582=CARTESIAN_POINT('Ctrl Pts',(-15.6295805882636,-12.3968947214249,
116.125575925284)) ;
#162583=CARTESIAN_POINT('Ctrl Pts',(-15.6410494594336,-12.4633049543151,
116.160508256525)) ;
#162584=CARTESIAN_POINT('Ctrl Pts',(-15.73692924491,-12.3586842738095,116.416876897232)) ;
#162585=CARTESIAN_POINT('Ctrl Pts',(-15.7424581639716,-12.4324967253125,
116.433717092915)) ;
#162586=CARTESIAN_POINT('Ctrl Pts',(-15.8162620121878,-12.432496720994,
116.409486065837)) ;
#162587=CARTESIAN_POINT('Ctrl Pts',(-15.890065860404,-12.4324967166755,
116.38525503876)) ;
#162588=CARTESIAN_POINT('Ctrl Pts',(-15.8845369413424,-12.3586842651726,
116.368414843077)) ;
#162589=CARTESIAN_POINT('Ctrl Pts',(-15.8790080222809,-12.2848718136696,
116.351574647394)) ;
#162590=CARTESIAN_POINT('Ctrl Pts',(-15.8052041740647,-12.284871817988,
116.375805674472)) ;
#162591=CARTESIAN_POINT('Ctrl Pts',(-15.7314003258485,-12.2848718223065,
116.400036701549)) ;
#162592=CARTESIAN_POINT('Ctrl Pts',(-15.73692924491,-12.3586842738095,116.416876897232)) ;
#162593=CARTESIAN_POINT('Ctrl Pts',(-15.837547597677,-12.3308701665295,
116.687989713795)) ;
#162594=CARTESIAN_POINT('Ctrl Pts',(-15.8367907309467,-12.4067313032611,
116.685684420293)) ;
#162595=CARTESIAN_POINT('Ctrl Pts',(-15.9105945814395,-12.4067313035056,
116.66145340015)) ;
#162596=CARTESIAN_POINT('Ctrl Pts',(-15.9843984319324,-12.4067313037501,
116.637222380007)) ;
#162597=CARTESIAN_POINT('Ctrl Pts',(-15.9851552986627,-12.3308701670186,
116.639527673509)) ;
#162598=CARTESIAN_POINT('Ctrl Pts',(-15.985912165393,-12.2550090302871,
116.641832967011)) ;
#162599=CARTESIAN_POINT('Ctrl Pts',(-15.9121083149001,-12.2550090300425,
116.666063987154)) ;
#162600=CARTESIAN_POINT('Ctrl Pts',(-15.8383044644072,-12.255009029798,
116.690295007297)) ;
#162601=CARTESIAN_POINT('Ctrl Pts',(-15.837547597677,-12.3308701665295,
116.687989713795)) ;
#162602=CARTESIAN_POINT('Ctrl Pts',(-15.9375214249544,-12.3804185210795,
116.95704231323)) ;
#162603=CARTESIAN_POINT('Ctrl Pts',(-15.930516766912,-12.4529298980233,
116.935707255623)) ;
#162604=CARTESIAN_POINT('Ctrl Pts',(-16.0043206195212,-12.452929906521,
116.911476241926)) ;
#162605=CARTESIAN_POINT('Ctrl Pts',(-16.0781244721304,-12.4529299150187,
116.887245228229)) ;
#162606=CARTESIAN_POINT('Ctrl Pts',(-16.0851291301728,-12.380418538075,
116.908580285836)) ;
#162607=CARTESIAN_POINT('Ctrl Pts',(-16.0921337882152,-12.3079071611312,
116.929915343443)) ;
#162608=CARTESIAN_POINT('Ctrl Pts',(-16.018329935606,-12.3079071526335,
116.95414635714)) ;
#162609=CARTESIAN_POINT('Ctrl Pts',(-15.9445260829967,-12.3079071441357,
116.978377370836)) ;
#162610=CARTESIAN_POINT('Ctrl Pts',(-15.9375214249544,-12.3804185210795,
116.95704231323)) ;
#162611=CARTESIAN_POINT('Ctrl Pts',(-16.0302559090412,-12.5045865657479,
117.204009987315)) ;
#162612=CARTESIAN_POINT('Ctrl Pts',(-16.0175006624101,-12.5685333529208,
117.165159564891)) ;
#162613=CARTESIAN_POINT('Ctrl Pts',(-16.0913045162659,-12.5685333737573,
117.14092855499)) ;
#162614=CARTESIAN_POINT('Ctrl Pts',(-16.1651083701216,-12.5685333945939,
117.11669754509)) ;
#162615=CARTESIAN_POINT('Ctrl Pts',(-16.1778636167527,-12.504586607421,
117.155547967515)) ;
#162616=CARTESIAN_POINT('Ctrl Pts',(-16.1906188633838,-12.4406398202481,
117.194398389939)) ;
#162617=CARTESIAN_POINT('Ctrl Pts',(-16.1168150095281,-12.4406397994116,
117.218629399839)) ;
#162618=CARTESIAN_POINT('Ctrl Pts',(-16.0430111556723,-12.440639778575,
117.242860409739)) ;
#162619=CARTESIAN_POINT('Ctrl Pts',(-16.0302559090412,-12.5045865657479,
117.204009987315)) ;
#162620=CARTESIAN_POINT('Ctrl Pts',(-16.1096439036277,-12.6936012415773,
117.410410771102)) ;
#162621=CARTESIAN_POINT('Ctrl Pts',(-16.0920599995317,-12.7444433865652,
117.356853037297)) ;
#162622=CARTESIAN_POINT('Ctrl Pts',(-16.165863853018,-12.7444434214993,
117.332622026272)) ;
#162623=CARTESIAN_POINT('Ctrl Pts',(-16.2396677065044,-12.7444434564334,
117.308391015246)) ;
#162624=CARTESIAN_POINT('Ctrl Pts',(-16.2572516106004,-12.6936013114455,
117.361948749051)) ;
#162625=CARTESIAN_POINT('Ctrl Pts',(-16.2748355146964,-12.6427591664577,
117.415506482856)) ;
#162626=CARTESIAN_POINT('Ctrl Pts',(-16.20103166121,-12.6427591315236,117.439737493882)) ;
#162627=CARTESIAN_POINT('Ctrl Pts',(-16.1272278077237,-12.6427590965895,
117.463968504907)) ;
#162628=CARTESIAN_POINT('Ctrl Pts',(-16.1096439036277,-12.6936012415773,
117.410410771102)) ;
#162629=CARTESIAN_POINT('Ctrl Pts',(-16.1712738995267,-12.9362801376937,
117.56247016244)) ;
#162630=CARTESIAN_POINT('Ctrl Pts',(-16.1500992985322,-12.9702525737982,
117.497975745442)) ;
#162631=CARTESIAN_POINT('Ctrl Pts',(-16.2239031501781,-12.9702526255318,
117.473744728811)) ;
#162632=CARTESIAN_POINT('Ctrl Pts',(-16.297707001824,-12.9702526772653,
117.44951371218)) ;
#162633=CARTESIAN_POINT('Ctrl Pts',(-16.3188816028185,-12.9362802411607,
117.514008129178)) ;
#162634=CARTESIAN_POINT('Ctrl Pts',(-16.340056203813,-12.9023078050562,
117.578502546175)) ;
#162635=CARTESIAN_POINT('Ctrl Pts',(-16.2662523521671,-12.9023077533226,
117.602733562806)) ;
#162636=CARTESIAN_POINT('Ctrl Pts',(-16.1924485005212,-12.9023077015891,
117.626964579437)) ;
#162637=CARTESIAN_POINT('Ctrl Pts',(-16.1712738995267,-12.9362801376937,
117.56247016244)) ;
#162638=CARTESIAN_POINT('Ctrl Pts',(-16.2106239956556,-13.2112926431605,
117.646987028832)) ;
#162639=CARTESIAN_POINT('Ctrl Pts',(-16.1874027324492,-13.2261131719055,
117.576258809104)) ;
#162640=CARTESIAN_POINT('Ctrl Pts',(-16.2612065799304,-13.2261132359039,
117.552027779788)) ;
#162641=CARTESIAN_POINT('Ctrl Pts',(-16.3350104274116,-13.2261132999022,
117.527796750472)) ;
#162642=CARTESIAN_POINT('Ctrl Pts',(-16.358231690618,-13.2112927711572,
117.5985249702)) ;
#162643=CARTESIAN_POINT('Ctrl Pts',(-16.3814529538244,-13.1964722424121,
117.669253189928)) ;
#162644=CARTESIAN_POINT('Ctrl Pts',(-16.3076491063432,-13.1964721784138,
117.693484219244)) ;
#162645=CARTESIAN_POINT('Ctrl Pts',(-16.233845258862,-13.1964721144154,
117.71771524856)) ;
#162646=CARTESIAN_POINT('Ctrl Pts',(-16.2106239956556,-13.2112926431605,
117.646987028832)) ;
#162647=CARTESIAN_POINT('Ctrl Pts',(-16.2263302334408,-13.5026318637497,
117.659280382526)) ;
#162648=CARTESIAN_POINT('Ctrl Pts',(-16.2027142030157,-13.4971333433814,
117.587349765715)) ;
#162649=CARTESIAN_POINT('Ctrl Pts',(-16.2765180448406,-13.4971334172492,
117.563118719171)) ;
#162650=CARTESIAN_POINT('Ctrl Pts',(-16.3503218866654,-13.4971334911169,
117.538887672627)) ;
#162651=CARTESIAN_POINT('Ctrl Pts',(-16.3739379170905,-13.5026320114853,
117.610818289438)) ;
#162652=CARTESIAN_POINT('Ctrl Pts',(-16.3975539475155,-13.5081305318536,
117.682748906249)) ;
#162653=CARTESIAN_POINT('Ctrl Pts',(-16.3237501056907,-13.5081304579859,
117.706979952793)) ;
#162654=CARTESIAN_POINT('Ctrl Pts',(-16.2499462638658,-13.5081303841181,
117.731210999337)) ;
#162655=CARTESIAN_POINT('Ctrl Pts',(-16.2263302334408,-13.5026318637497,
117.659280382526)) ;
#162656=CARTESIAN_POINT('Ctrl Pts',(-16.2177424879971,-13.7865927515763,
117.59774844092)) ;
#162657=CARTESIAN_POINT('Ctrl Pts',(-16.1954238427971,-13.7612608950297,
117.529769450301)) ;
#162658=CARTESIAN_POINT('Ctrl Pts',(-16.2692276778268,-13.7612609711619,
117.50553838306)) ;
#162659=CARTESIAN_POINT('Ctrl Pts',(-16.3430315128565,-13.7612610472941,
117.481307315818)) ;
#162660=CARTESIAN_POINT('Ctrl Pts',(-16.3653501580564,-13.7865929038406,
117.549286306437)) ;
#162661=CARTESIAN_POINT('Ctrl Pts',(-16.3876688032563,-13.8119247603871,
117.617265297056)) ;
#162662=CARTESIAN_POINT('Ctrl Pts',(-16.3138649682267,-13.811924684255,
117.641496364297)) ;
#162663=CARTESIAN_POINT('Ctrl Pts',(-16.240061133197,-13.8119246081228,
117.665727431539)) ;
#162664=CARTESIAN_POINT('Ctrl Pts',(-16.2177424879971,-13.7865927515763,
117.59774844092)) ;
#162665=CARTESIAN_POINT('Ctrl Pts',(-16.1863917194238,-14.0445932154009,
117.466837858413)) ;
#162666=CARTESIAN_POINT('Ctrl Pts',(-16.1669624264012,-14.0012118501805,
117.407659368456)) ;
#162667=CARTESIAN_POINT('Ctrl Pts',(-16.2407662542766,-14.001211921774,
117.383428279424)) ;
#162668=CARTESIAN_POINT('Ctrl Pts',(-16.3145700821519,-14.0012119933675,
117.359197190392)) ;
#162669=CARTESIAN_POINT('Ctrl Pts',(-16.3339993751745,-14.0445933585879,
117.418375680349)) ;
#162670=CARTESIAN_POINT('Ctrl Pts',(-16.3534286681971,-14.0879747238084,
117.477554170305)) ;
#162671=CARTESIAN_POINT('Ctrl Pts',(-16.2796248403217,-14.0879746522149,
117.501785259337)) ;
#162672=CARTESIAN_POINT('Ctrl Pts',(-16.2058210124464,-14.0879745806213,
117.526016348369)) ;
#162673=CARTESIAN_POINT('Ctrl Pts',(-16.1863917194238,-14.0445932154009,
117.466837858413)) ;
#162674=CARTESIAN_POINT('Ctrl Pts',(-16.1351369456625,-14.2581092551482,
117.275260073732)) ;
#162675=CARTESIAN_POINT('Ctrl Pts',(-16.1199915913662,-14.199757820622,
117.229129770043)) ;
#162676=CARTESIAN_POINT('Ctrl Pts',(-16.1937954124028,-14.199757880284,
117.204898660181)) ;
#162677=CARTESIAN_POINT('Ctrl Pts',(-16.2675992334394,-14.199757939946,
117.180667550319)) ;
#162678=CARTESIAN_POINT('Ctrl Pts',(-16.2827445877356,-14.2581093744722,
117.226797854008)) ;
#162679=CARTESIAN_POINT('Ctrl Pts',(-16.2978899420319,-14.3164608089984,
117.272928157698)) ;
#162680=CARTESIAN_POINT('Ctrl Pts',(-16.2240861209953,-14.3164607493364,
117.29715926756)) ;
#162681=CARTESIAN_POINT('Ctrl Pts',(-16.1502822999588,-14.3164606896743,
117.321390377422)) ;
#162682=CARTESIAN_POINT('Ctrl Pts',(-16.1351369456625,-14.2581092551482,
117.275260073732)) ;
#162683=CARTESIAN_POINT('Ctrl Pts',(-16.0682061521682,-14.4117380229187,
117.035830487134)) ;
#162684=CARTESIAN_POINT('Ctrl Pts',(-16.0584474319418,-14.3425754066096,
117.0061070018)) ;
#162685=CARTESIAN_POINT('Ctrl Pts',(-16.1322512472086,-14.3425754472621,
116.981875874365)) ;
#162686=CARTESIAN_POINT('Ctrl Pts',(-16.2060550624755,-14.3425754879145,
116.957644746929)) ;
#162687=CARTESIAN_POINT('Ctrl Pts',(-16.2158137827019,-14.4117381042236,
116.987368232263)) ;
#162688=CARTESIAN_POINT('Ctrl Pts',(-16.2255725029284,-14.4809007205327,
117.017091717597)) ;
#162689=CARTESIAN_POINT('Ctrl Pts',(-16.1517686876615,-14.4809006798802,
117.041322845032)) ;
#162690=CARTESIAN_POINT('Ctrl Pts',(-16.0779648723947,-14.4809006392278,
117.065553972468)) ;
#162691=CARTESIAN_POINT('Ctrl Pts',(-16.0682061521682,-14.4117380229187,
117.035830487134)) ;
#162692=CARTESIAN_POINT('Ctrl Pts',(-15.9915317982417,-14.4936441507055,
116.76682264577)) ;
#162693=CARTESIAN_POINT('Ctrl Pts',(-15.9878458146668,-14.4186618661927,
116.755595736523)) ;
#162694=CARTESIAN_POINT('Ctrl Pts',(-16.0616496263278,-14.4186618819305,
116.731364598104)) ;
#162695=CARTESIAN_POINT('Ctrl Pts',(-16.1354534379888,-14.4186618976683,
116.707133459686)) ;
#162696=CARTESIAN_POINT('Ctrl Pts',(-16.1391394215636,-14.4936441821811,
116.718360368933)) ;
#162697=CARTESIAN_POINT('Ctrl Pts',(-16.1428254051384,-14.5686264666939,
116.729587278181)) ;
#162698=CARTESIAN_POINT('Ctrl Pts',(-16.0690215934775,-14.5686264509561,
116.753818416599)) ;
#162699=CARTESIAN_POINT('Ctrl Pts',(-15.9952177818165,-14.5686264352184,
116.778049555018)) ;
#162700=CARTESIAN_POINT('Ctrl Pts',(-15.9915317982417,-14.4936441507055,
116.76682264577)) ;
#162701=CARTESIAN_POINT('Ctrl Pts',(-15.9111646098176,-14.4983888239063,
116.486541384417)) ;
#162702=CARTESIAN_POINT('Ctrl Pts',(-15.9138185855326,-14.422965043811,
116.494624968275)) ;
#162703=CARTESIAN_POINT('Ctrl Pts',(-15.9876223961134,-14.4229650315207,
116.470393826567)) ;
#162704=CARTESIAN_POINT('Ctrl Pts',(-16.0614262066943,-14.4229650192305,
116.446162684859)) ;
#162705=CARTESIAN_POINT('Ctrl Pts',(-16.0587722309793,-14.4983887993257,
116.438079101)) ;
#162706=CARTESIAN_POINT('Ctrl Pts',(-16.0561182552643,-14.573812579421,
116.429995517142)) ;
#162707=CARTESIAN_POINT('Ctrl Pts',(-15.9823144446834,-14.5738125917113,
116.45422665885)) ;
#162708=CARTESIAN_POINT('Ctrl Pts',(-15.9085106341026,-14.5738126040015,
116.478457800559)) ;
#162709=CARTESIAN_POINT('Ctrl Pts',(-15.9111646098176,-14.4983888239063,
116.486541384417)) ;
#162710=CARTESIAN_POINT('Ctrl Pts',(-15.8339367194652,-14.426207251784,
116.215966892118)) ;
#162711=CARTESIAN_POINT('Ctrl Pts',(-15.8427178234298,-14.3557121733631,
116.242712720049)) ;
#162712=CARTESIAN_POINT('Ctrl Pts',(-15.9165216357164,-14.355712132954,
116.218481583536)) ;
#162713=CARTESIAN_POINT('Ctrl Pts',(-15.9903254480029,-14.3557120925449,
116.194250447023)) ;
#162714=CARTESIAN_POINT('Ctrl Pts',(-15.9815443440383,-14.4262071709657,
116.167504619092)) ;
#162715=CARTESIAN_POINT('Ctrl Pts',(-15.9727632400736,-14.4967022493866,
116.140758791161)) ;
#162716=CARTESIAN_POINT('Ctrl Pts',(-15.8989594277871,-14.4967022897957,
116.164989927674)) ;
#162717=CARTESIAN_POINT('Ctrl Pts',(-15.8251556155005,-14.4967023302048,
116.189221064187)) ;
#162718=CARTESIAN_POINT('Ctrl Pts',(-15.8339367194652,-14.426207251784,
116.215966892118)) ;
#162719=CARTESIAN_POINT('Ctrl Pts',(-15.7654080575456,-14.2809809264381,
115.971651595224)) ;
#162720=CARTESIAN_POINT('Ctrl Pts',(-15.7797229341676,-14.2205203869784,
116.015252401813)) ;
#162721=CARTESIAN_POINT('Ctrl Pts',(-15.8535267507502,-14.2205203209335,
115.991021278385)) ;
#162722=CARTESIAN_POINT('Ctrl Pts',(-15.9273305673328,-14.2205202548886,
115.966790154957)) ;
#162723=CARTESIAN_POINT('Ctrl Pts',(-15.9130156907108,-14.2809807943484,
115.923189348368)) ;
#162724=CARTESIAN_POINT('Ctrl Pts',(-15.8987008140888,-14.3414413338082,
115.879588541778)) ;
#162725=CARTESIAN_POINT('Ctrl Pts',(-15.8248969975061,-14.3414413998531,
115.903819665206)) ;
#162726=CARTESIAN_POINT('Ctrl Pts',(-15.7510931809235,-14.3414414658979,
115.928050788634)) ;
#162727=CARTESIAN_POINT('Ctrl Pts',(-15.7654080575456,-14.2809809264381,
115.971651595224)) ;
#162728=CARTESIAN_POINT('Ctrl Pts',(-15.7121638592197,-14.0755731076895,
115.774205354296)) ;
#162729=CARTESIAN_POINT('Ctrl Pts',(-15.7309470596531,-14.0293643773253,
115.831415954248)) ;
#162730=CARTESIAN_POINT('Ctrl Pts',(-15.8047508827093,-14.0293642911148,
115.807184850537)) ;
#162731=CARTESIAN_POINT('Ctrl Pts',(-15.8785547057655,-14.0293642049043,
115.782953746827)) ;
#162732=CARTESIAN_POINT('Ctrl Pts',(-15.8597715053321,-14.0755729352685,
115.725743146875)) ;
#162733=CARTESIAN_POINT('Ctrl Pts',(-15.8409883048986,-14.1217816656326,
115.668532546923)) ;
#162734=CARTESIAN_POINT('Ctrl Pts',(-15.7671844818424,-14.1217817518431,
115.692763650634)) ;
#162735=CARTESIAN_POINT('Ctrl Pts',(-15.6933806587863,-14.1217818380536,
115.716994754344)) ;
#162736=CARTESIAN_POINT('Ctrl Pts',(-15.7121638592197,-14.0755731076895,
115.774205354296)) ;
#162737=CARTESIAN_POINT('Ctrl Pts',(-15.6778558958867,-13.8214647968314,
115.634145099666)) ;
#162738=CARTESIAN_POINT('Ctrl Pts',(-15.699798207312,-13.7929280082953,
115.700977841948)) ;
#162739=CARTESIAN_POINT('Ctrl Pts',(-15.7736020384604,-13.7929279092314,
115.676746762885)) ;
#162740=CARTESIAN_POINT('Ctrl Pts',(-15.8474058696088,-13.7929278101675,
115.652515683822)) ;
#162741=CARTESIAN_POINT('Ctrl Pts',(-15.8254635581835,-13.8214645987035,
115.58568294154)) ;
#162742=CARTESIAN_POINT('Ctrl Pts',(-15.8035212467582,-13.8500013872396,
115.518850199258)) ;
#162743=CARTESIAN_POINT('Ctrl Pts',(-15.7297174156098,-13.8500014863035,
115.543081278321)) ;
#162744=CARTESIAN_POINT('Ctrl Pts',(-15.6559135844614,-13.8500015853674,
115.567312357384)) ;
#162745=CARTESIAN_POINT('Ctrl Pts',(-15.6778558958867,-13.8214647968314,
115.634145099666)) ;
#162746=CARTESIAN_POINT('Ctrl Pts',(-15.6663008904224,-13.5390721929965,
115.563497706539)) ;
#162747=CARTESIAN_POINT('Ctrl Pts',(-15.6898162477156,-13.5302086359891,
115.635121692674)) ;
#162748=CARTESIAN_POINT('Ctrl Pts',(-15.7636200876184,-13.5302085326853,
115.610890640275)) ;
#162749=CARTESIAN_POINT('Ctrl Pts',(-15.8374239275211,-13.5302084293816,
115.586659587877)) ;
#162750=CARTESIAN_POINT('Ctrl Pts',(-15.8139085702279,-13.539071986389,
115.515035601742)) ;
#162751=CARTESIAN_POINT('Ctrl Pts',(-15.7903932129347,-13.5479355433964,
115.443411615607)) ;
#162752=CARTESIAN_POINT('Ctrl Pts',(-15.7165893730319,-13.5479356467002,
115.467642668006)) ;
#162753=CARTESIAN_POINT('Ctrl Pts',(-15.6427855331292,-13.5479357500039,
115.491873720405)) ;
#162754=CARTESIAN_POINT('Ctrl Pts',(-15.6663008904224,-13.5390721929965,
115.563497706539)) ;
#162755=CARTESIAN_POINT('Ctrl Pts',(-15.6788710235298,-13.2479213210197,
115.566312381468)) ;
#162756=CARTESIAN_POINT('Ctrl Pts',(-15.7022779391019,-13.2593718199025,
115.637606071544)) ;
#162757=CARTESIAN_POINT('Ctrl Pts',(-15.7760817875237,-13.2593717210079,
115.613375045094)) ;
#162758=CARTESIAN_POINT('Ctrl Pts',(-15.8498856359456,-13.2593716221134,
115.589144018643)) ;
#162759=CARTESIAN_POINT('Ctrl Pts',(-15.8264787203735,-13.2479211232306,
115.517850328566)) ;
#162760=CARTESIAN_POINT('Ctrl Pts',(-15.8030718048014,-13.2364706243478,
115.446556638489)) ;
#162761=CARTESIAN_POINT('Ctrl Pts',(-15.7292679563796,-13.2364707232423,
115.47078766494)) ;
#162762=CARTESIAN_POINT('Ctrl Pts',(-15.6554641079578,-13.2364708221369,
115.495018691391)) ;
#162763=CARTESIAN_POINT('Ctrl Pts',(-15.6788710235298,-13.2479213210197,
115.566312381468)) ;
#162764=CARTESIAN_POINT('Ctrl Pts',(-15.7154570310451,-12.9689956696526,
115.642283838143)) ;
#162765=CARTESIAN_POINT('Ctrl Pts',(-15.7370785345889,-12.9999372691398,
115.708139451166)) ;
#162766=CARTESIAN_POINT('Ctrl Pts',(-15.8108823904318,-12.9999371823959,
115.683908447318)) ;
#162767=CARTESIAN_POINT('Ctrl Pts',(-15.8846862462746,-12.9999370956519,
115.65967744347)) ;
#162768=CARTESIAN_POINT('Ctrl Pts',(-15.8630647427309,-12.9689954961647,
115.593821830448)) ;
#162769=CARTESIAN_POINT('Ctrl Pts',(-15.8414432391871,-12.9380538966775,
115.527966217425)) ;
#162770=CARTESIAN_POINT('Ctrl Pts',(-15.7676393833442,-12.9380539834215,
115.552197221273)) ;
#162771=CARTESIAN_POINT('Ctrl Pts',(-15.6938355275013,-12.9380540701654,
115.57642822512)) ;
#162772=CARTESIAN_POINT('Ctrl Pts',(-15.7154570310451,-12.9689956696526,
115.642283838143)) ;
#162773=CARTESIAN_POINT('Ctrl Pts',(-15.7742309880506,-12.7220961737177,
115.785813685881)) ;
#162774=CARTESIAN_POINT('Ctrl Pts',(-15.7925158427138,-12.7703223930981,
115.841506404667)) ;
#162775=CARTESIAN_POINT('Ctrl Pts',(-15.8663197041459,-12.7703223245763,
115.817275417843)) ;
#162776=CARTESIAN_POINT('Ctrl Pts',(-15.9401235655779,-12.7703222560545,
115.793044431019)) ;
#162777=CARTESIAN_POINT('Ctrl Pts',(-15.9218387109147,-12.7220960366741,
115.737351712233)) ;
#162778=CARTESIAN_POINT('Ctrl Pts',(-15.9035538562515,-12.6738698172937,
115.681658993447)) ;
#162779=CARTESIAN_POINT('Ctrl Pts',(-15.8297499948195,-12.6738698858155,
115.705889980271)) ;
#162780=CARTESIAN_POINT('Ctrl Pts',(-15.7559461333875,-12.6738699543374,
115.730120967095)) ;
#162781=CARTESIAN_POINT('Ctrl Pts',(-15.7742309880506,-12.7220961737177,
115.785813685881)) ;
#162782=CARTESIAN_POINT('Ctrl Pts',(-15.8515784407682,-12.5254520180373,
115.985975276655)) ;
#162783=CARTESIAN_POINT('Ctrl Pts',(-15.8652235858158,-12.5874803484278,
116.027536188445)) ;
#162784=CARTESIAN_POINT('Ctrl Pts',(-15.9390274506629,-12.5874803012304,
116.003305212022)) ;
#162785=CARTESIAN_POINT('Ctrl Pts',(-16.0128313155099,-12.5874802540331,
115.9790742356)) ;
#162786=CARTESIAN_POINT('Ctrl Pts',(-15.9991861704623,-12.5254519236426,
115.93751332381)) ;
#162787=CARTESIAN_POINT('Ctrl Pts',(-15.9855410254147,-12.463423593252,
115.89595241202)) ;
#162788=CARTESIAN_POINT('Ctrl Pts',(-15.9117371605676,-12.4634236404494,
115.920183388442)) ;
#162789=CARTESIAN_POINT('Ctrl Pts',(-15.8379332957206,-12.4634236876467,
115.944414364864)) ;
#162790=CARTESIAN_POINT('Ctrl Pts',(-15.8515784407682,-12.5254520180373,
115.985975276655)) ;
#162791=CARTESIAN_POINT('Ctrl Pts',(-15.94270937751,-12.3924871288094,116.22814157512)) ;
#162792=CARTESIAN_POINT('Ctrl Pts',(-15.9507450204375,-12.4638924990082,
116.252616848413)) ;
#162793=CARTESIAN_POINT('Ctrl Pts',(-16.0245488864703,-12.4638924741093,
116.228385875602)) ;
#162794=CARTESIAN_POINT('Ctrl Pts',(-16.0983527525031,-12.4638924492103,
116.204154902791)) ;
#162795=CARTESIAN_POINT('Ctrl Pts',(-16.0903171095756,-12.3924870790115,
116.179679629498)) ;
#162796=CARTESIAN_POINT('Ctrl Pts',(-16.0822814666481,-12.3210817088127,
116.155204356205)) ;
#162797=CARTESIAN_POINT('Ctrl Pts',(-16.0084776006153,-12.3210817337116,
116.179435329016)) ;
#162798=CARTESIAN_POINT('Ctrl Pts',(-15.9346737345826,-12.3210817586106,
116.203666301827)) ;
#162799=CARTESIAN_POINT('Ctrl Pts',(-15.94270937751,-12.3924871288094,116.22814157512)) ;
#162800=CARTESIAN_POINT('Ctrl Pts',(-16.0425166341127,-12.3327720085306,
116.496536154784)) ;
#162801=CARTESIAN_POINT('Ctrl Pts',(-16.0443326725553,-12.4084551705648,
116.502067516169)) ;
#162802=CARTESIAN_POINT('Ctrl Pts',(-16.1181365370123,-12.4084551665108,
116.477836538559)) ;
#162803=CARTESIAN_POINT('Ctrl Pts',(-16.1919404014694,-12.4084551624567,
116.453605560949)) ;
#162804=CARTESIAN_POINT('Ctrl Pts',(-16.1901243630268,-12.3327720004226,
116.448074199563)) ;
#162805=CARTESIAN_POINT('Ctrl Pts',(-16.1883083245843,-12.2570888383885,
116.442542838178)) ;
#162806=CARTESIAN_POINT('Ctrl Pts',(-16.1145044601272,-12.2570888424425,
116.466773815788)) ;
#162807=CARTESIAN_POINT('Ctrl Pts',(-16.0407005956702,-12.2570888464965,
116.491004793398)) ;
#162808=CARTESIAN_POINT('Ctrl Pts',(-16.0425166341127,-12.3327720085306,
116.496536154784)) ;
#162809=CARTESIAN_POINT('Ctrl Pts',(-16.1432965454572,-12.3509988977752,
116.768165464397)) ;
#162810=CARTESIAN_POINT('Ctrl Pts',(-16.1388098877865,-12.4255237330698,
116.754499830221)) ;
#162811=CARTESIAN_POINT('Ctrl Pts',(-16.2126137496675,-12.4255237455323,
116.730268844765)) ;
#162812=CARTESIAN_POINT('Ctrl Pts',(-16.2864176115484,-12.4255237579948,
116.706037859308)) ;
#162813=CARTESIAN_POINT('Ctrl Pts',(-16.2909042692191,-12.3509989227002,
116.719703493484)) ;
#162814=CARTESIAN_POINT('Ctrl Pts',(-16.2953909268898,-12.2764740874057,
116.733369127659)) ;
#162815=CARTESIAN_POINT('Ctrl Pts',(-16.2215870650088,-12.2764740749432,
116.757600113116)) ;
#162816=CARTESIAN_POINT('Ctrl Pts',(-16.1477832031279,-12.2764740624807,
116.781831098573)) ;
#162817=CARTESIAN_POINT('Ctrl Pts',(-16.1432965454572,-12.3509988977752,
116.768165464397)) ;
#162818=CARTESIAN_POINT('Ctrl Pts',(-16.2397734663179,-12.4453838611795,
117.026540426964)) ;
#162819=CARTESIAN_POINT('Ctrl Pts',(-16.2292780482387,-12.5134317382336,
116.994573077925)) ;
#162820=CARTESIAN_POINT('Ctrl Pts',(-16.3030819059699,-12.5134317622461,
116.970342079829)) ;
#162821=CARTESIAN_POINT('Ctrl Pts',(-16.3768857637012,-12.5134317862586,
116.946111081733)) ;
#162822=CARTESIAN_POINT('Ctrl Pts',(-16.3873811817803,-12.4453839092044,
116.978078430772)) ;
#162823=CARTESIAN_POINT('Ctrl Pts',(-16.3978765998595,-12.3773360321503,
117.01004577981)) ;
#162824=CARTESIAN_POINT('Ctrl Pts',(-16.3240727421283,-12.3773360081379,
117.034276777906)) ;
#162825=CARTESIAN_POINT('Ctrl Pts',(-16.2502688843971,-12.3773359841254,
117.058507776003)) ;
#162826=CARTESIAN_POINT('Ctrl Pts',(-16.2397734663179,-12.4453838611795,
117.026540426964)) ;
#162827=CARTESIAN_POINT('Ctrl Pts',(-16.3254447848863,-12.6100760699984,
117.251940625839)) ;
#162828=CARTESIAN_POINT('Ctrl Pts',(-16.3096871062923,-12.6667282433853,
117.203945280152)) ;
#162829=CARTESIAN_POINT('Ctrl Pts',(-16.3834909593544,-12.6667282722992,
117.179714267834)) ;
#162830=CARTESIAN_POINT('Ctrl Pts',(-16.4572948124166,-12.6667283012131,
117.155483255517)) ;
#162831=CARTESIAN_POINT('Ctrl Pts',(-16.4730524910106,-12.6100761278262,
117.203478601204)) ;
#162832=CARTESIAN_POINT('Ctrl Pts',(-16.4888101696046,-12.5534239544393,
117.251473946891)) ;
#162833=CARTESIAN_POINT('Ctrl Pts',(-16.4150063165425,-12.5534239255254,
117.275704959209)) ;
#162834=CARTESIAN_POINT('Ctrl Pts',(-16.3412024634803,-12.5534238966115,
117.299935971526)) ;
#162835=CARTESIAN_POINT('Ctrl Pts',(-16.3254447848863,-12.6100760699984,
117.251940625839)) ;
#162836=CARTESIAN_POINT('Ctrl Pts',(-16.3945559404646,-12.8316470477012,
117.427060764436)) ;
#162837=CARTESIAN_POINT('Ctrl Pts',(-16.3746810642588,-12.8729143960197,
117.366525098979)) ;
#162838=CARTESIAN_POINT('Ctrl Pts',(-16.4484849132355,-12.8729144255077,
117.342294074218)) ;
#162839=CARTESIAN_POINT('Ctrl Pts',(-16.5222887622122,-12.8729144549957,
117.318063049457)) ;
#162840=CARTESIAN_POINT('Ctrl Pts',(-16.542163638418,-12.8316471066773,
117.378598714914)) ;
#162841=CARTESIAN_POINT('Ctrl Pts',(-16.5620385146238,-12.7903797583588,
117.439134380371)) ;
#162842=CARTESIAN_POINT('Ctrl Pts',(-16.4882346656471,-12.7903797288708,
117.463365405132)) ;
#162843=CARTESIAN_POINT('Ctrl Pts',(-16.4144308166704,-12.7903796993828,
117.487596429893)) ;
#162844=CARTESIAN_POINT('Ctrl Pts',(-16.3945559404646,-12.8316470477012,
117.427060764436)) ;
#162845=CARTESIAN_POINT('Ctrl Pts',(-16.4435312853677,-13.0973555362981,
117.540560244616)) ;
#162846=CARTESIAN_POINT('Ctrl Pts',(-16.4209446285881,-13.1201328482756,
117.471764932878)) ;
#162847=CARTESIAN_POINT('Ctrl Pts',(-16.4947484740099,-13.1201328716907,
117.44753389729)) ;
#162848=CARTESIAN_POINT('Ctrl Pts',(-16.5685523194317,-13.1201328951058,
117.423302861701)) ;
#162849=CARTESIAN_POINT('Ctrl Pts',(-16.5911389762113,-13.0973555831283,
117.492098173439)) ;
#162850=CARTESIAN_POINT('Ctrl Pts',(-16.6137256329909,-13.0745782711508,
117.560893485177)) ;
#162851=CARTESIAN_POINT('Ctrl Pts',(-16.5399217875691,-13.0745782477357,
117.585124520766)) ;
#162852=CARTESIAN_POINT('Ctrl Pts',(-16.4661179421473,-13.0745782243206,
117.609355556355)) ;
#162853=CARTESIAN_POINT('Ctrl Pts',(-16.4435312853677,-13.0973555362981,
117.540560244616)) ;
#162854=CARTESIAN_POINT('Ctrl Pts',(-16.4688621130792,-13.3829827267331,
117.582449970111)) ;
#162855=CARTESIAN_POINT('Ctrl Pts',(-16.4452025092137,-13.3858507921175,
117.510386634553)) ;
#162856=CARTESIAN_POINT('Ctrl Pts',(-16.5190063526211,-13.3858508103817,
117.486155592829)) ;
#162857=CARTESIAN_POINT('Ctrl Pts',(-16.5928101960284,-13.3858508286459,
117.461924551104)) ;
#162858=CARTESIAN_POINT('Ctrl Pts',(-16.6164697998939,-13.3829827632615,
117.533987886662)) ;
#162859=CARTESIAN_POINT('Ctrl Pts',(-16.6401294037594,-13.380114697877,
117.60605122222)) ;
#162860=CARTESIAN_POINT('Ctrl Pts',(-16.566325560352,-13.3801146796128,
117.630282263945)) ;
#162861=CARTESIAN_POINT('Ctrl Pts',(-16.4925217169447,-13.3801146613487,
117.654513305669)) ;
#162862=CARTESIAN_POINT('Ctrl Pts',(-16.4688621130792,-13.3829827267331,
117.582449970111)) ;
#162863=CARTESIAN_POINT('Ctrl Pts',(-16.470124542703,-13.6735145155205,
117.550719313167)) ;
#162864=CARTESIAN_POINT('Ctrl Pts',(-16.4470771654852,-13.6561003398034,
117.480520721043)) ;
#162865=CARTESIAN_POINT('Ctrl Pts',(-16.5208810079376,-13.6561003497692,
117.45628967641)) ;
#162866=CARTESIAN_POINT('Ctrl Pts',(-16.5946848503899,-13.656100359735,
117.432058631777)) ;
#162867=CARTESIAN_POINT('Ctrl Pts',(-16.6177322276078,-13.673514535452,
117.502257223901)) ;
#162868=CARTESIAN_POINT('Ctrl Pts',(-16.6407796048256,-13.690928711169,
117.572455816025)) ;
#162869=CARTESIAN_POINT('Ctrl Pts',(-16.5669757623732,-13.6909287012033,
117.596686860658)) ;
#162870=CARTESIAN_POINT('Ctrl Pts',(-16.4931719199208,-13.6909286912375,
117.620917905291)) ;
#162871=CARTESIAN_POINT('Ctrl Pts',(-16.470124542703,-13.6735145155205,
117.550719313167)) ;
#162872=CARTESIAN_POINT('Ctrl Pts',(-16.4477134830108,-13.9443960540442,
117.447059781621)) ;
#162873=CARTESIAN_POINT('Ctrl Pts',(-16.4269288979224,-13.9080411308625,
117.383753289118)) ;
#162874=CARTESIAN_POINT('Ctrl Pts',(-16.5007327404672,-13.9080411350017,
117.359522244767)) ;
#162875=CARTESIAN_POINT('Ctrl Pts',(-16.574536583012,-13.9080411391408,
117.335291200415)) ;
#162876=CARTESIAN_POINT('Ctrl Pts',(-16.5953211681005,-13.9443960623225,
117.398597692918)) ;
#162877=CARTESIAN_POINT('Ctrl Pts',(-16.616105753189,-13.9807509855041,
117.461904185421)) ;
#162878=CARTESIAN_POINT('Ctrl Pts',(-16.5423019106441,-13.980750981365,
117.486135229772)) ;
#162879=CARTESIAN_POINT('Ctrl Pts',(-16.4684980680993,-13.9807509772258,
117.510366274124)) ;
#162880=CARTESIAN_POINT('Ctrl Pts',(-16.4477134830108,-13.9443960540442,
117.447059781621)) ;
#162881=CARTESIAN_POINT('Ctrl Pts',(-16.4040416496053,-14.1780473237906,
117.278577420489)) ;
#162882=CARTESIAN_POINT('Ctrl Pts',(-16.3870093108388,-14.125322660068,
117.226699664773)) ;
#162883=CARTESIAN_POINT('Ctrl Pts',(-16.460813154071,-14.12532266015,117.202468622515)) ;
#162884=CARTESIAN_POINT('Ctrl Pts',(-16.5346169973033,-14.1253226602321,
117.178237580257)) ;
#162885=CARTESIAN_POINT('Ctrl Pts',(-16.5516493360698,-14.1780473239547,
117.230115335974)) ;
#162886=CARTESIAN_POINT('Ctrl Pts',(-16.5686816748364,-14.2307719876773,
117.28199309169)) ;
#162887=CARTESIAN_POINT('Ctrl Pts',(-16.4948778316041,-14.2307719875953,
117.306224133948)) ;
#162888=CARTESIAN_POINT('Ctrl Pts',(-16.4210739883719,-14.2307719875132,
117.330455176205)) ;
#162889=CARTESIAN_POINT('Ctrl Pts',(-16.4040416496053,-14.1780473237906,
117.278577420489)) ;
#162890=CARTESIAN_POINT('Ctrl Pts',(-16.3431014881368,-14.3571729772058,
117.057559267268)) ;
#162891=CARTESIAN_POINT('Ctrl Pts',(-16.3310317024854,-14.2918617658065,
117.020796647579)) ;
#162892=CARTESIAN_POINT('Ctrl Pts',(-16.4048355465375,-14.2918617643923,
116.996565607819)) ;
#162893=CARTESIAN_POINT('Ctrl Pts',(-16.4786393905896,-14.291861762978,
116.972334568058)) ;
#162894=CARTESIAN_POINT('Ctrl Pts',(-16.4907091762409,-14.3571729743773,
117.009097187747)) ;
#162895=CARTESIAN_POINT('Ctrl Pts',(-16.5027789618923,-14.4224841857766,
117.045859807437)) ;
#162896=CARTESIAN_POINT('Ctrl Pts',(-16.4289751178402,-14.4224841871909,
117.070090847197)) ;
#162897=CARTESIAN_POINT('Ctrl Pts',(-16.3551712737882,-14.4224841886051,
117.094321886958)) ;
#162898=CARTESIAN_POINT('Ctrl Pts',(-16.3431014881368,-14.3571729772058,
117.057559267268)) ;
#162899=CARTESIAN_POINT('Ctrl Pts',(-16.2692843220695,-14.4697035049953,
116.797034589842)) ;
#162900=CARTESIAN_POINT('Ctrl Pts',(-16.2630899618578,-14.3964364704153,
116.778167568028)) ;
#162901=CARTESIAN_POINT('Ctrl Pts',(-16.3368938062969,-14.3964364695808,
116.753936529446)) ;
#162902=CARTESIAN_POINT('Ctrl Pts',(-16.410697650736,-14.3964364687462,
116.729705490864)) ;
#162903=CARTESIAN_POINT('Ctrl Pts',(-16.4168920109476,-14.4697035033262,
116.748572512678)) ;
#162904=CARTESIAN_POINT('Ctrl Pts',(-16.4230863711593,-14.5429705379062,
116.767439534492)) ;
#162905=CARTESIAN_POINT('Ctrl Pts',(-16.3492825267203,-14.5429705387408,
116.791670573074)) ;
#162906=CARTESIAN_POINT('Ctrl Pts',(-16.2754786822812,-14.5429705395753,
116.815901611656)) ;
#162907=CARTESIAN_POINT('Ctrl Pts',(-16.2692843220695,-14.4697035049953,
116.797034589842)) ;
#162908=CARTESIAN_POINT('Ctrl Pts',(-16.189974204939,-14.5058316151569,
116.520142021784)) ;
#162909=CARTESIAN_POINT('Ctrl Pts',(-16.1900398398108,-14.4299343068103,
116.520341934979)) ;
#162910=CARTESIAN_POINT('Ctrl Pts',(-16.2638436837928,-14.4299343070279,
116.496110895004)) ;
#162911=CARTESIAN_POINT('Ctrl Pts',(-16.3376475277747,-14.4299343072455,
116.47187985503)) ;
#162912=CARTESIAN_POINT('Ctrl Pts',(-16.3375818929029,-14.5058316155922,
116.471679941836)) ;
#162913=CARTESIAN_POINT('Ctrl Pts',(-16.3375162580311,-14.5817289239388,
116.471480028642)) ;
#162914=CARTESIAN_POINT('Ctrl Pts',(-16.2637124140491,-14.5817289237212,
116.495711068616)) ;
#162915=CARTESIAN_POINT('Ctrl Pts',(-16.1899085700672,-14.5817289235035,
116.51994210859)) ;
#162916=CARTESIAN_POINT('Ctrl Pts',(-16.189974204939,-14.5058316151569,
116.520142021784)) ;
#162917=CARTESIAN_POINT('Ctrl Pts',(-16.1107202304642,-14.4647781183691,
116.243348321315)) ;
#162918=CARTESIAN_POINT('Ctrl Pts',(-16.1170525275077,-14.3916362177671,
116.262635476418)) ;
#162919=CARTESIAN_POINT('Ctrl Pts',(-16.1908563705672,-14.3916362178144,
116.238404433634)) ;
#162920=CARTESIAN_POINT('Ctrl Pts',(-16.2646602136268,-14.3916362178617,
116.21417339085)) ;
#162921=CARTESIAN_POINT('Ctrl Pts',(-16.2583279165833,-14.4647781184637,
116.194886235748)) ;
#162922=CARTESIAN_POINT('Ctrl Pts',(-16.2519956195399,-14.5379200190658,
116.175599080645)) ;
#162923=CARTESIAN_POINT('Ctrl Pts',(-16.1781917764803,-14.5379200190184,
116.199830123429)) ;
#162924=CARTESIAN_POINT('Ctrl Pts',(-16.1043879334208,-14.5379200189711,
116.224061166212)) ;
#162925=CARTESIAN_POINT('Ctrl Pts',(-16.1107202304642,-14.4647781183691,
116.243348321315)) ;
#162926=CARTESIAN_POINT('Ctrl Pts',(-16.03788617739,-14.3484987257117,115.986015587949)) ;
#162927=CARTESIAN_POINT('Ctrl Pts',(-16.0500479103369,-14.2833691759875,
116.023058264334)) ;
#162928=CARTESIAN_POINT('Ctrl Pts',(-16.1238517520509,-14.2833691732841,
115.998827217452)) ;
#162929=CARTESIAN_POINT('Ctrl Pts',(-16.1976555937649,-14.2833691705807,
115.97459617057)) ;
#162930=CARTESIAN_POINT('Ctrl Pts',(-16.1854938608181,-14.3484987203049,
115.937553494185)) ;
#162931=CARTESIAN_POINT('Ctrl Pts',(-16.1733321278713,-14.4136282700291,
115.9005108178)) ;
#162932=CARTESIAN_POINT('Ctrl Pts',(-16.0995282861572,-14.4136282727325,
115.924741864682)) ;
#162933=CARTESIAN_POINT('Ctrl Pts',(-16.0257244444432,-14.4136282754358,
115.948972911564)) ;
#162934=CARTESIAN_POINT('Ctrl Pts',(-16.03788617739,-14.3484987257117,115.986015587949)) ;
#162935=CARTESIAN_POINT('Ctrl Pts',(-15.9776687836141,-14.1655053892491,
115.767116814539)) ;
#162936=CARTESIAN_POINT('Ctrl Pts',(-15.994787213724,-14.1130583565086,
115.819256790845)) ;
#162937=CARTESIAN_POINT('Ctrl Pts',(-16.0685910543299,-14.1130583479537,
115.795025740588)) ;
#162938=CARTESIAN_POINT('Ctrl Pts',(-16.1423948949358,-14.1130583393988,
115.77079469033)) ;
#162939=CARTESIAN_POINT('Ctrl Pts',(-16.1252764648259,-14.1655053721393,
115.718654714025)) ;
#162940=CARTESIAN_POINT('Ctrl Pts',(-16.1081580347159,-14.2179524048798,
115.666514737719)) ;
#162941=CARTESIAN_POINT('Ctrl Pts',(-16.0343541941101,-14.2179524134347,
115.690745787976)) ;
#162942=CARTESIAN_POINT('Ctrl Pts',(-15.9605503535042,-14.2179524219896,
115.714976838234)) ;
#162943=CARTESIAN_POINT('Ctrl Pts',(-15.9776687836141,-14.1655053892491,
115.767116814539)) ;
#162944=CARTESIAN_POINT('Ctrl Pts',(-15.9351536436701,-13.9286208259661,
115.602105173613)) ;
#162945=CARTESIAN_POINT('Ctrl Pts',(-15.9560004743455,-13.8926376196403,
115.665601256615)) ;
#162946=CARTESIAN_POINT('Ctrl Pts',(-16.0298043146523,-13.8926376022121,
115.641370205447)) ;
#162947=CARTESIAN_POINT('Ctrl Pts',(-16.1036081549591,-13.8926375847838,
115.617139154278)) ;
#162948=CARTESIAN_POINT('Ctrl Pts',(-16.0827613242837,-13.9286207911095,
115.553643071277)) ;
#162949=CARTESIAN_POINT('Ctrl Pts',(-16.0619144936083,-13.9646039974353,
115.490146988275)) ;
#162950=CARTESIAN_POINT('Ctrl Pts',(-15.9881106533015,-13.9646040148635,
115.514378039444)) ;
#162951=CARTESIAN_POINT('Ctrl Pts',(-15.9143068129948,-13.9646040322918,
115.538609090612)) ;
#162952=CARTESIAN_POINT('Ctrl Pts',(-15.9351536436701,-13.9286208259661,
115.602105173613)) ;
#162953=CARTESIAN_POINT('Ctrl Pts',(-15.9141622270948,-13.6565946963034,
115.502836000379)) ;
#162954=CARTESIAN_POINT('Ctrl Pts',(-15.9372359188981,-13.6395527561257,
115.573114743203)) ;
#162955=CARTESIAN_POINT('Ctrl Pts',(-16.0110397602486,-13.6395527301396,
115.548883695214)) ;
#162956=CARTESIAN_POINT('Ctrl Pts',(-16.0848436015992,-13.6395527041535,
115.524652647225)) ;
#162957=CARTESIAN_POINT('Ctrl Pts',(-16.0617699097959,-13.6565946443312,
115.454373904401)) ;
#162958=CARTESIAN_POINT('Ctrl Pts',(-16.0386962179926,-13.6736365845089,
115.384095161576)) ;
#162959=CARTESIAN_POINT('Ctrl Pts',(-15.9648923766421,-13.673636610495,
115.408326209565)) ;
#162960=CARTESIAN_POINT('Ctrl Pts',(-15.8910885352915,-13.6736366364811,
115.432557257555)) ;
#162961=CARTESIAN_POINT('Ctrl Pts',(-15.9141622270948,-13.6565946963034,
115.502836000379)) ;
#162962=CARTESIAN_POINT('Ctrl Pts',(-15.9168400704658,-13.3650274692435,
115.475347116262)) ;
#162963=CARTESIAN_POINT('Ctrl Pts',(-15.9404979400582,-13.3683183370286,
115.547405170571)) ;
#162964=CARTESIAN_POINT('Ctrl Pts',(-16.0143017837554,-13.368318300107,
115.52317412973)) ;
#162965=CARTESIAN_POINT('Ctrl Pts',(-16.0881056274526,-13.3683182631854,
115.498943088888)) ;
#162966=CARTESIAN_POINT('Ctrl Pts',(-16.0644477578601,-13.3650273954003,
115.426885034579)) ;
#162967=CARTESIAN_POINT('Ctrl Pts',(-16.0407898882677,-13.3617365276153,
115.35482698027)) ;
#162968=CARTESIAN_POINT('Ctrl Pts',(-15.9669860445706,-13.3617365645369,
115.379058021112)) ;
#162969=CARTESIAN_POINT('Ctrl Pts',(-15.8931822008734,-13.3617366014585,
115.403289061953)) ;
#162970=CARTESIAN_POINT('Ctrl Pts',(-15.9168400704658,-13.3650274692435,
115.475347116262)) ;
#162971=CARTESIAN_POINT('Ctrl Pts',(-15.943917468856,-13.0788343995772,
115.522370330454)) ;
#162972=CARTESIAN_POINT('Ctrl Pts',(-15.9664525229632,-13.1021119946019,
115.591008470126)) ;
#162973=CARTESIAN_POINT('Ctrl Pts',(-16.0402563706024,-13.1021119511676,
115.566777441291)) ;
#162974=CARTESIAN_POINT('Ctrl Pts',(-16.1140602182415,-13.1021119077334,
115.542546412456)) ;
#162975=CARTESIAN_POINT('Ctrl Pts',(-16.0915251641342,-13.0788343127088,
115.473908272784)) ;
#162976=CARTESIAN_POINT('Ctrl Pts',(-16.068990110027,-13.0555567176841,
115.405270133111)) ;
#162977=CARTESIAN_POINT('Ctrl Pts',(-15.9951862623878,-13.0555567611183,
115.429501161946)) ;
#162978=CARTESIAN_POINT('Ctrl Pts',(-15.9213824147487,-13.0555568045526,
115.453732190781)) ;
#162979=CARTESIAN_POINT('Ctrl Pts',(-15.943917468856,-13.0788343995772,
115.522370330454)) ;
#162980=CARTESIAN_POINT('Ctrl Pts',(-15.9938421820601,-12.8175211583994,
115.639074782229)) ;
#162981=CARTESIAN_POINT('Ctrl Pts',(-16.0136556516188,-12.8590768776832,
115.699423414641)) ;
#162982=CARTESIAN_POINT('Ctrl Pts',(-16.0874595039968,-12.8590768329722,
115.67519240024)) ;
#162983=CARTESIAN_POINT('Ctrl Pts',(-16.1612633563749,-12.8590767882613,
115.650961385839)) ;
#162984=CARTESIAN_POINT('Ctrl Pts',(-16.1414498868162,-12.8175210689774,
115.590612753427)) ;
#162985=CARTESIAN_POINT('Ctrl Pts',(-16.1216364172575,-12.7759653496935,
115.530264121016)) ;
#162986=CARTESIAN_POINT('Ctrl Pts',(-16.0478325648795,-12.7759653944045,
115.554495135417)) ;
#162987=CARTESIAN_POINT('Ctrl Pts',(-15.9740287125014,-12.7759654391155,
115.578726149818)) ;
#162988=CARTESIAN_POINT('Ctrl Pts',(-15.9938421820601,-12.8175211583994,
115.639074782229)) ;
#162989=CARTESIAN_POINT('Ctrl Pts',(-16.0641439891467,-12.5984995679009,
115.817749196681)) ;
#162990=CARTESIAN_POINT('Ctrl Pts',(-16.0798113378379,-12.6554070787726,
115.865469414067)) ;
#162991=CARTESIAN_POINT('Ctrl Pts',(-16.1536151955778,-12.6554070377801,
115.841238415998)) ;
#162992=CARTESIAN_POINT('Ctrl Pts',(-16.2274190533178,-12.6554069967877,
115.817007417928)) ;
#162993=CARTESIAN_POINT('Ctrl Pts',(-16.2117517046266,-12.5984994859161,
115.769287200542)) ;
#162994=CARTESIAN_POINT('Ctrl Pts',(-16.1960843559353,-12.5415919750444,
115.721566983155)) ;
#162995=CARTESIAN_POINT('Ctrl Pts',(-16.1222804981954,-12.5415920160368,
115.745797981225)) ;
#162996=CARTESIAN_POINT('Ctrl Pts',(-16.0484766404554,-12.5415920570292,
115.770028979294)) ;
#162997=CARTESIAN_POINT('Ctrl Pts',(-16.0641439891467,-12.5984995679009,
115.817749196681)) ;
#162998=CARTESIAN_POINT('Ctrl Pts',(-16.1502868270294,-12.4381081950322,
116.044719588303)) ;
#162999=CARTESIAN_POINT('Ctrl Pts',(-16.1606951475451,-12.5062960463662,
116.076421654558)) ;
#163000=CARTESIAN_POINT('Ctrl Pts',(-16.2344990103366,-12.5062960154841,
116.052190671875)) ;
#163001=CARTESIAN_POINT('Ctrl Pts',(-16.3083028731281,-12.506295984602,
116.027959689191)) ;
#163002=CARTESIAN_POINT('Ctrl Pts',(-16.2978945526124,-12.4381081332681,
115.996257622937)) ;
#163003=CARTESIAN_POINT('Ctrl Pts',(-16.2874862320967,-12.3699202819341,
115.964555556682)) ;
#163004=CARTESIAN_POINT('Ctrl Pts',(-16.2136823693052,-12.3699203128162,
115.988786539365)) ;
#163005=CARTESIAN_POINT('Ctrl Pts',(-16.1398785065137,-12.3699203436983,
116.013017522048)) ;
#163006=CARTESIAN_POINT('Ctrl Pts',(-16.1502868270294,-12.4381081950322,
116.044719588303)) ;
#163007=CARTESIAN_POINT('Ctrl Pts',(-16.2478432903342,-12.3474840033873,
116.306149605933)) ;
#163008=CARTESIAN_POINT('Ctrl Pts',(-16.2521946188714,-12.4220984887537,
116.319403052103)) ;
#163009=CARTESIAN_POINT('Ctrl Pts',(-16.3259984865435,-12.4220984739895,
116.295172084286)) ;
#163010=CARTESIAN_POINT('Ctrl Pts',(-16.3998023542157,-12.4220984592253,
116.270941116468)) ;
#163011=CARTESIAN_POINT('Ctrl Pts',(-16.3954510256785,-12.3474839738589,
116.257687670298)) ;
#163012=CARTESIAN_POINT('Ctrl Pts',(-16.3910996971414,-12.2728694884925,
116.244434224128)) ;
#163013=CARTESIAN_POINT('Ctrl Pts',(-16.3172958294692,-12.2728695032567,
116.268665191945)) ;
#163014=CARTESIAN_POINT('Ctrl Pts',(-16.243491961797,-12.2728695180209,
116.292896159763)) ;
#163015=CARTESIAN_POINT('Ctrl Pts',(-16.2478432903342,-12.3474840033873,
116.306149605933)) ;
#163016=CARTESIAN_POINT('Ctrl Pts',(-16.3485101468529,-12.3342746176406,
116.577507728098)) ;
#163017=CARTESIAN_POINT('Ctrl Pts',(-16.3465689953954,-12.4099190416296,
116.571595295596)) ;
#163018=CARTESIAN_POINT('Ctrl Pts',(-16.4203728650902,-12.4099190485564,
116.547364333939)) ;
#163019=CARTESIAN_POINT('Ctrl Pts',(-16.4941767347851,-12.4099190554831,
116.523133372282)) ;
#163020=CARTESIAN_POINT('Ctrl Pts',(-16.4961178862426,-12.3342746314941,
116.529045804785)) ;
#163021=CARTESIAN_POINT('Ctrl Pts',(-16.4980590377001,-12.2586302075051,
116.534958237287)) ;
#163022=CARTESIAN_POINT('Ctrl Pts',(-16.4242551680053,-12.2586302005783,
116.559189198944)) ;
#163023=CARTESIAN_POINT('Ctrl Pts',(-16.3504512983104,-12.2586301936515,
116.5834201606)) ;
#163024=CARTESIAN_POINT('Ctrl Pts',(-16.3485101468529,-12.3342746176406,
116.577507728098)) ;
#163025=CARTESIAN_POINT('Ctrl Pts',(-16.4477907403322,-12.3983523506611,
116.844372055818)) ;
#163026=CARTESIAN_POINT('Ctrl Pts',(-16.4396504910612,-12.4696333213927,
116.819578171729)) ;
#163027=CARTESIAN_POINT('Ctrl Pts',(-16.513454361231,-12.4696333527669,
116.795347211519)) ;
#163028=CARTESIAN_POINT('Ctrl Pts',(-16.5872582314008,-12.4696333841411,
116.771116251309)) ;
#163029=CARTESIAN_POINT('Ctrl Pts',(-16.5953984806718,-12.3983524134095,
116.795910135398)) ;
#163030=CARTESIAN_POINT('Ctrl Pts',(-16.6035387299428,-12.3270714426779,
116.820704019487)) ;
#163031=CARTESIAN_POINT('Ctrl Pts',(-16.529734859773,-12.3270714113037,
116.844934979697)) ;
#163032=CARTESIAN_POINT('Ctrl Pts',(-16.4559309896032,-12.3270713799295,
116.869165939907)) ;
#163033=CARTESIAN_POINT('Ctrl Pts',(-16.4477907403322,-12.3983523506611,
116.844372055818)) ;
#163034=CARTESIAN_POINT('Ctrl Pts',(-16.5383794781962,-12.5353914606374,
117.084853142342)) ;
#163035=CARTESIAN_POINT('Ctrl Pts',(-16.5246360542602,-12.5972087494759,
117.042992892395)) ;
#163036=CARTESIAN_POINT('Ctrl Pts',(-16.5984399222197,-12.5972088056809,
117.018761925452)) ;
#163037=CARTESIAN_POINT('Ctrl Pts',(-16.6722437901792,-12.5972088618859,
116.99453095851)) ;
#163038=CARTESIAN_POINT('Ctrl Pts',(-16.6859872141153,-12.5353915730474,
117.036391208458)) ;
#163039=CARTESIAN_POINT('Ctrl Pts',(-16.6997306380514,-12.4735742842089,
117.078251458405)) ;
#163040=CARTESIAN_POINT('Ctrl Pts',(-16.6259267700919,-12.4735742280039,
117.102482425347)) ;
#163041=CARTESIAN_POINT('Ctrl Pts',(-16.5521229021323,-12.4735741717989,
117.12671339229)) ;
#163042=CARTESIAN_POINT('Ctrl Pts',(-16.5383794781962,-12.5353914606374,
117.084853142342)) ;
#163043=CARTESIAN_POINT('Ctrl Pts',(-16.6151024200091,-12.7368848040207,
117.282902758644)) ;
#163044=CARTESIAN_POINT('Ctrl Pts',(-16.5967196831152,-12.7847255574639,
117.226911910079)) ;
#163045=CARTESIAN_POINT('Ctrl Pts',(-16.6705235464973,-12.7847256367286,
117.202680929194)) ;
#163046=CARTESIAN_POINT('Ctrl Pts',(-16.7443274098794,-12.7847257159933,
117.17844994831)) ;
#163047=CARTESIAN_POINT('Ctrl Pts',(-16.7627101467733,-12.7368849625501,
117.234440796876)) ;
#163048=CARTESIAN_POINT('Ctrl Pts',(-16.7810928836672,-12.6890442091069,
117.290431645442)) ;
#163049=CARTESIAN_POINT('Ctrl Pts',(-16.7072890202851,-12.6890441298422,
117.314662626326)) ;
#163050=CARTESIAN_POINT('Ctrl Pts',(-16.633485156903,-12.6890440505775,
117.33889360721)) ;
#163051=CARTESIAN_POINT('Ctrl Pts',(-16.6151024200091,-12.7368848040207,
117.282902758644)) ;
#163052=CARTESIAN_POINT('Ctrl Pts',(-16.6722339594684,-12.9849643669818,
117.421634700217)) ;
#163053=CARTESIAN_POINT('Ctrl Pts',(-16.6505656858349,-13.0155548424745,
117.355636636913)) ;
#163054=CARTESIAN_POINT('Ctrl Pts',(-16.7243695422743,-13.0155549383142,
117.331405634882)) ;
#163055=CARTESIAN_POINT('Ctrl Pts',(-16.7981733987138,-13.0155550341539,
117.307174632852)) ;
#163056=CARTESIAN_POINT('Ctrl Pts',(-16.8198416723473,-12.9849645586612,
117.373172696156)) ;
#163057=CARTESIAN_POINT('Ctrl Pts',(-16.8415099459808,-12.9543740831685,
117.43917075946)) ;
#163058=CARTESIAN_POINT('Ctrl Pts',(-16.7677060895413,-12.9543739873288,
117.46340176149)) ;
#163059=CARTESIAN_POINT('Ctrl Pts',(-16.6939022331019,-12.9543738914891,
117.487632763521)) ;
#163060=CARTESIAN_POINT('Ctrl Pts',(-16.6722339594684,-12.9849643669818,
117.421634700217)) ;
#163061=CARTESIAN_POINT('Ctrl Pts',(-16.7074953741335,-13.2657001242146,
117.493501410732)) ;
#163062=CARTESIAN_POINT('Ctrl Pts',(-16.6840686069065,-13.2767359206685,
117.422147259724)) ;
#163063=CARTESIAN_POINT('Ctrl Pts',(-16.7578724550329,-13.2767360267194,
117.397916232373)) ;
#163064=CARTESIAN_POINT('Ctrl Pts',(-16.8316763031593,-13.2767361327703,
117.373685205023)) ;
#163065=CARTESIAN_POINT('Ctrl Pts',(-16.8551030703862,-13.2657003363164,
117.445039356031)) ;
#163066=CARTESIAN_POINT('Ctrl Pts',(-16.8785298376132,-13.2546645398624,
117.516393507038)) ;
#163067=CARTESIAN_POINT('Ctrl Pts',(-16.8047259894868,-13.2546644338116,
117.540624534389)) ;
#163068=CARTESIAN_POINT('Ctrl Pts',(-16.7309221413604,-13.2546643277607,
117.56485556174)) ;
#163069=CARTESIAN_POINT('Ctrl Pts',(-16.7074953741335,-13.2657001242146,
117.493501410732)) ;
#163070=CARTESIAN_POINT('Ctrl Pts',(-16.7185435095042,-13.5562446654925,
117.491765214544)) ;
#163071=CARTESIAN_POINT('Ctrl Pts',(-16.6950431078555,-13.5470119024509,
117.420186784989)) ;
#163072=CARTESIAN_POINT('Ctrl Pts',(-16.7688469469812,-13.5470120097675,
117.395955730224)) ;
#163073=CARTESIAN_POINT('Ctrl Pts',(-16.842650786107,-13.5470121170841,
117.371724675459)) ;
#163074=CARTESIAN_POINT('Ctrl Pts',(-16.8661511877557,-13.5562448801257,
117.443303105014)) ;
#163075=CARTESIAN_POINT('Ctrl Pts',(-16.8896515894044,-13.5654776431673,
117.514881534569)) ;
#163076=CARTESIAN_POINT('Ctrl Pts',(-16.8158477502786,-13.5654775358507,
117.539112589334)) ;
#163077=CARTESIAN_POINT('Ctrl Pts',(-16.7420439111529,-13.5654774285341,
117.5633436441)) ;
#163078=CARTESIAN_POINT('Ctrl Pts',(-16.7185435095042,-13.5562446654925,
117.491765214544)) ;
#163079=CARTESIAN_POINT('Ctrl Pts',(-16.7056071827156,-13.837740260252,
117.416879374421)) ;
#163080=CARTESIAN_POINT('Ctrl Pts',(-16.6837093500279,-13.8088409661864,
117.350182111352)) ;
#163081=CARTESIAN_POINT('Ctrl Pts',(-16.7575131803557,-13.8088410662031,
117.32595102979)) ;
#163082=CARTESIAN_POINT('Ctrl Pts',(-16.8313170106835,-13.8088411662199,
117.301719948228)) ;
#163083=CARTESIAN_POINT('Ctrl Pts',(-16.8532148433712,-13.8377404602855,
117.368417211296)) ;
#163084=CARTESIAN_POINT('Ctrl Pts',(-16.8751126760589,-13.8666397543512,
117.435114474365)) ;
#163085=CARTESIAN_POINT('Ctrl Pts',(-16.8013088457311,-13.8666396543344,
117.459345555927)) ;
#163086=CARTESIAN_POINT('Ctrl Pts',(-16.7275050154033,-13.8666395543177,
117.483576637489)) ;
#163087=CARTESIAN_POINT('Ctrl Pts',(-16.7056071827156,-13.837740260252,
117.416879374421)) ;
#163088=CARTESIAN_POINT('Ctrl Pts',(-16.6698983566585,-14.0900089023239,
117.272469305418)) ;
#163089=CARTESIAN_POINT('Ctrl Pts',(-16.6511984458618,-14.0434540249531,
117.215512396418)) ;
#163090=CARTESIAN_POINT('Ctrl Pts',(-16.7250022686231,-14.0434541089459,
117.191281291809)) ;
#163091=CARTESIAN_POINT('Ctrl Pts',(-16.7988060913844,-14.0434541929387,
117.167050187201)) ;
#163092=CARTESIAN_POINT('Ctrl Pts',(-16.8175060021811,-14.0900090703095,
117.224007096201)) ;
#163093=CARTESIAN_POINT('Ctrl Pts',(-16.8362059129778,-14.1365639476803,
117.280964005202)) ;
#163094=CARTESIAN_POINT('Ctrl Pts',(-16.7624020902165,-14.1365638636875,
117.30519510981)) ;
#163095=CARTESIAN_POINT('Ctrl Pts',(-16.6885982674552,-14.1365637796947,
117.329426214419)) ;
#163096=CARTESIAN_POINT('Ctrl Pts',(-16.6698983566585,-14.0900089023239,
117.272469305418)) ;
#163097=CARTESIAN_POINT('Ctrl Pts',(-16.615678314691,-14.2916996646196,
117.072102717414)) ;
#163098=CARTESIAN_POINT('Ctrl Pts',(-16.6014650259406,-14.2309943169081,
117.028811335221)) ;
#163099=CARTESIAN_POINT('Ctrl Pts',(-16.6752688429158,-14.230994379438,
117.004580212989)) ;
#163100=CARTESIAN_POINT('Ctrl Pts',(-16.749072659891,-14.2309944419679,
116.980349090757)) ;
#163101=CARTESIAN_POINT('Ctrl Pts',(-16.7632859486414,-14.2916997896794,
117.023640472949)) ;
#163102=CARTESIAN_POINT('Ctrl Pts',(-16.7774992373917,-14.3524051373909,
117.066931855141)) ;
#163103=CARTESIAN_POINT('Ctrl Pts',(-16.7036954204165,-14.352405074861,
117.091162977374)) ;
#163104=CARTESIAN_POINT('Ctrl Pts',(-16.6298916034414,-14.352405012331,
117.115394099606)) ;
#163105=CARTESIAN_POINT('Ctrl Pts',(-16.615678314691,-14.2916996646196,
117.072102717414)) ;
#163106=CARTESIAN_POINT('Ctrl Pts',(-16.5462715072985,-14.4330905333239,
116.82503637481)) ;
#163107=CARTESIAN_POINT('Ctrl Pts',(-16.5376205247406,-14.362422601594,
116.798686879729)) ;
#163108=CARTESIAN_POINT('Ctrl Pts',(-16.6114243386022,-14.3624226376889,
116.774455748013)) ;
#163109=CARTESIAN_POINT('Ctrl Pts',(-16.6852281524637,-14.3624226737838,
116.750224616297)) ;
#163110=CARTESIAN_POINT('Ctrl Pts',(-16.6938791350216,-14.4330906055137,
116.776574111379)) ;
#163111=CARTESIAN_POINT('Ctrl Pts',(-16.7025301175795,-14.5037585372437,
116.80292360646)) ;
#163112=CARTESIAN_POINT('Ctrl Pts',(-16.628726303718,-14.5037585011487,
116.827154738176)) ;
#163113=CARTESIAN_POINT('Ctrl Pts',(-16.5549224898564,-14.5037584650538,
116.851385869892)) ;
#163114=CARTESIAN_POINT('Ctrl Pts',(-16.5462715072985,-14.4330905333239,
116.82503637481)) ;
#163115=CARTESIAN_POINT('Ctrl Pts',(-16.4684461424741,-14.5004556458798,
116.552546390901)) ;
#163116=CARTESIAN_POINT('Ctrl Pts',(-16.4659492440457,-14.424978464963,
116.544941243033)) ;
#163117=CARTESIAN_POINT('Ctrl Pts',(-16.5397530573826,-14.4249784742085,
116.520710109719)) ;
#163118=CARTESIAN_POINT('Ctrl Pts',(-16.6135568707195,-14.4249784834539,
116.496478976405)) ;
#163119=CARTESIAN_POINT('Ctrl Pts',(-16.6160537691479,-14.5004556643706,
116.504084124273)) ;
#163120=CARTESIAN_POINT('Ctrl Pts',(-16.6185506675763,-14.5759328452874,
116.51168927214)) ;
#163121=CARTESIAN_POINT('Ctrl Pts',(-16.5447468542394,-14.5759328360419,
116.535920405454)) ;
#163122=CARTESIAN_POINT('Ctrl Pts',(-16.4709430409025,-14.5759328267965,
116.560151538768)) ;
#163123=CARTESIAN_POINT('Ctrl Pts',(-16.4684461424741,-14.5004556458798,
116.552546390901)) ;
#163124=CARTESIAN_POINT('Ctrl Pts',(-16.3884429132822,-14.4906784452632,
116.273515768952)) ;
#163125=CARTESIAN_POINT('Ctrl Pts',(-16.3922594977658,-14.4157707960699,
116.285140471267)) ;
#163126=CARTESIAN_POINT('Ctrl Pts',(-16.4660633128443,-14.4157707802425,
116.260909343258)) ;
#163127=CARTESIAN_POINT('Ctrl Pts',(-16.5398671279229,-14.4157707644151,
116.236678215249)) ;
#163128=CARTESIAN_POINT('Ctrl Pts',(-16.5360505434393,-14.4906784136084,
116.225053512934)) ;
#163129=CARTESIAN_POINT('Ctrl Pts',(-16.5322339589558,-14.5655860628017,
116.213428810619)) ;
#163130=CARTESIAN_POINT('Ctrl Pts',(-16.4584301438772,-14.5655860786291,
116.237659938628)) ;
#163131=CARTESIAN_POINT('Ctrl Pts',(-16.3846263287987,-14.5655860944565,
116.261891066637)) ;
#163132=CARTESIAN_POINT('Ctrl Pts',(-16.3884429132822,-14.4906784452632,
116.273515768952)) ;
#163133=CARTESIAN_POINT('Ctrl Pts',(-16.3122978006783,-14.4044504861589,
116.006169416252)) ;
#163134=CARTESIAN_POINT('Ctrl Pts',(-16.3221693671015,-14.3354504116019,
116.036236616476)) ;
#163135=CARTESIAN_POINT('Ctrl Pts',(-16.3959731861657,-14.3354503745246,
116.012005500606)) ;
#163136=CARTESIAN_POINT('Ctrl Pts',(-16.4697770052299,-14.3354503374474,
115.987774384737)) ;
#163137=CARTESIAN_POINT('Ctrl Pts',(-16.4599054388067,-14.4044504120043,
115.957707184513)) ;
#163138=CARTESIAN_POINT('Ctrl Pts',(-16.4500338723836,-14.4734504865613,
115.92763998429)) ;
#163139=CARTESIAN_POINT('Ctrl Pts',(-16.3762300533194,-14.4734505236385,
115.95187110016)) ;
#163140=CARTESIAN_POINT('Ctrl Pts',(-16.3024262342552,-14.4734505607158,
115.976102216029)) ;
#163141=CARTESIAN_POINT('Ctrl Pts',(-16.3122978006783,-14.4044504861589,
116.006169416252)) ;
#163142=CARTESIAN_POINT('Ctrl Pts',(-16.2460229579914,-14.2464177648016,
115.768663223049)) ;
#163143=CARTESIAN_POINT('Ctrl Pts',(-16.2612742676278,-14.1883465874269,
115.815116252918)) ;
#163144=CARTESIAN_POINT('Ctrl Pts',(-16.3350780926779,-14.1883465362759,
115.790885155281)) ;
#163145=CARTESIAN_POINT('Ctrl Pts',(-16.4088819177281,-14.1883464851249,
115.766654057644)) ;
#163146=CARTESIAN_POINT('Ctrl Pts',(-16.3936306080916,-14.2464176624996,
115.720201027774)) ;
#163147=CARTESIAN_POINT('Ctrl Pts',(-16.3783792984552,-14.3044888398743,
115.673747997904)) ;
#163148=CARTESIAN_POINT('Ctrl Pts',(-16.304575473405,-14.3044888910253,
115.697979095542)) ;
#163149=CARTESIAN_POINT('Ctrl Pts',(-16.2307716483549,-14.3044889421763,
115.722210193179)) ;
#163150=CARTESIAN_POINT('Ctrl Pts',(-16.2460229579914,-14.2464177648016,
115.768663223049)) ;
#163151=CARTESIAN_POINT('Ctrl Pts',(-16.1959322208732,-14.0296079395376,
115.58064014647)) ;
#163152=CARTESIAN_POINT('Ctrl Pts',(-16.2154375855199,-13.9865865421538,
115.640050341363)) ;
#163153=CARTESIAN_POINT('Ctrl Pts',(-16.2892414167736,-13.9865864836806,
115.615819262621)) ;
#163154=CARTESIAN_POINT('Ctrl Pts',(-16.3630452480274,-13.9865864252074,
115.591588183879)) ;
#163155=CARTESIAN_POINT('Ctrl Pts',(-16.3435398833807,-14.0296078225912,
115.532177988986)) ;
#163156=CARTESIAN_POINT('Ctrl Pts',(-16.324034518734,-14.072629219975,115.472767794093)) ;
#163157=CARTESIAN_POINT('Ctrl Pts',(-16.2502306874803,-14.0726292784482,
115.496998872835)) ;
#163158=CARTESIAN_POINT('Ctrl Pts',(-16.1764268562265,-14.0726293369214,
115.521229951577)) ;
#163159=CARTESIAN_POINT('Ctrl Pts',(-16.1959322208732,-14.0296079395376,
115.58064014647)) ;
#163160=CARTESIAN_POINT('Ctrl Pts',(-16.1659524449804,-13.7700542634679,
115.453985376571)) ;
#163161=CARTESIAN_POINT('Ctrl Pts',(-16.1883117544927,-13.7450900092007,
115.522088226907)) ;
#163162=CARTESIAN_POINT('Ctrl Pts',(-16.2621155917233,-13.7450899491233,
115.497857166369)) ;
#163163=CARTESIAN_POINT('Ctrl Pts',(-16.3359194289538,-13.7450898890458,
115.473626105831)) ;
#163164=CARTESIAN_POINT('Ctrl Pts',(-16.3135601194414,-13.7700541433129,
115.405523255495)) ;
#163165=CARTESIAN_POINT('Ctrl Pts',(-16.2912008099291,-13.79501839758,115.337420405159)) ;
#163166=CARTESIAN_POINT('Ctrl Pts',(-16.2173969726985,-13.7950184576575,
115.361651465697)) ;
#163167=CARTESIAN_POINT('Ctrl Pts',(-16.143593135468,-13.795018517735,115.385882526235)) ;
#163168=CARTESIAN_POINT('Ctrl Pts',(-16.1659524449804,-13.7700542634679,
115.453985376571)) ;
#163169=CARTESIAN_POINT('Ctrl Pts',(-16.1588094450499,-13.4844393542531,
115.396766680954)) ;
#163170=CARTESIAN_POINT('Ctrl Pts',(-16.1824352013854,-13.4793790766449,
115.468726923808)) ;
#163171=CARTESIAN_POINT('Ctrl Pts',(-16.2562390440075,-13.4793790219259,
115.444495879692)) ;
#163172=CARTESIAN_POINT('Ctrl Pts',(-16.3300428866296,-13.479378967207,
115.420264835576)) ;
#163173=CARTESIAN_POINT('Ctrl Pts',(-16.3064171302942,-13.4844392448151,
115.348304592722)) ;
#163174=CARTESIAN_POINT('Ctrl Pts',(-16.2827913739587,-13.4894995224233,
115.276344349867)) ;
#163175=CARTESIAN_POINT('Ctrl Pts',(-16.2089875313366,-13.4894995771423,
115.300575393983)) ;
#163176=CARTESIAN_POINT('Ctrl Pts',(-16.1351836887144,-13.4894996318613,
115.324806438099)) ;
#163177=CARTESIAN_POINT('Ctrl Pts',(-16.1588094450499,-13.4844393542531,
115.396766680954)) ;
#163178=CARTESIAN_POINT('Ctrl Pts',(-16.1759899887603,-13.1938467066394,
115.413606223146)) ;
#163179=CARTESIAN_POINT('Ctrl Pts',(-16.1991864289273,-13.2090684129076,
115.484258838048)) ;
#163180=CARTESIAN_POINT('Ctrl Pts',(-16.27299027552,-13.2090683682137,115.460027806026)) ;
#163181=CARTESIAN_POINT('Ctrl Pts',(-16.3467941221126,-13.2090683235198,
115.435796774003)) ;
#163182=CARTESIAN_POINT('Ctrl Pts',(-16.3235976819456,-13.1938466172516,
115.365144159101)) ;
#163183=CARTESIAN_POINT('Ctrl Pts',(-16.3004012417786,-13.1786249109835,
115.294491544198)) ;
#163184=CARTESIAN_POINT('Ctrl Pts',(-16.226597395186,-13.1786249556774,
115.318722576221)) ;
#163185=CARTESIAN_POINT('Ctrl Pts',(-16.1527935485933,-13.1786250003713,
115.342953608243)) ;
#163186=CARTESIAN_POINT('Ctrl Pts',(-16.1759899887603,-13.1938467066394,
115.413606223146)) ;
#163187=CARTESIAN_POINT('Ctrl Pts',(-16.2169131908586,-12.9193998282655,
115.502784611301)) ;
#163188=CARTESIAN_POINT('Ctrl Pts',(-16.2380214175388,-12.9538071121124,
115.567076864686)) ;
#163189=CARTESIAN_POINT('Ctrl Pts',(-16.3118252664966,-12.9538070795867,
115.542845839867)) ;
#163190=CARTESIAN_POINT('Ctrl Pts',(-16.3856291154545,-12.9538070470611,
115.518614815049)) ;
#163191=CARTESIAN_POINT('Ctrl Pts',(-16.3645208887744,-12.9193997632142,
115.454322561664)) ;
#163192=CARTESIAN_POINT('Ctrl Pts',(-16.3434126620942,-12.8849924793673,
115.39003030828)) ;
#163193=CARTESIAN_POINT('Ctrl Pts',(-16.2696088131364,-12.884992511893,
115.414261333098)) ;
#163194=CARTESIAN_POINT('Ctrl Pts',(-16.1958049641785,-12.8849925444186,
115.438492357917)) ;
#163195=CARTESIAN_POINT('Ctrl Pts',(-16.2169131908586,-12.9193998282655,
115.502784611301)) ;
#163196=CARTESIAN_POINT('Ctrl Pts',(-16.2798288449759,-12.679977460876,
115.658797492625)) ;
#163197=CARTESIAN_POINT('Ctrl Pts',(-16.2973132491563,-12.7311545599109,
115.712052167187)) ;
#163198=CARTESIAN_POINT('Ctrl Pts',(-16.371117098481,-12.7311545403401,
115.687821143486)) ;
#163199=CARTESIAN_POINT('Ctrl Pts',(-16.4449209478057,-12.7311545207693,
115.663590119785)) ;
#163200=CARTESIAN_POINT('Ctrl Pts',(-16.4274365436253,-12.6799774217345,
115.610335445223)) ;
#163201=CARTESIAN_POINT('Ctrl Pts',(-16.4099521394449,-12.6288003226997,
115.557080770662)) ;
#163202=CARTESIAN_POINT('Ctrl Pts',(-16.3361482901202,-12.6288003422704,
115.581311794363)) ;
#163203=CARTESIAN_POINT('Ctrl Pts',(-16.2623444407955,-12.6288003618412,
115.605542818064)) ;
#163204=CARTESIAN_POINT('Ctrl Pts',(-16.2798288449759,-12.679977460876,
115.658797492625)) ;
#163205=CARTESIAN_POINT('Ctrl Pts',(-16.3596321413727,-12.4956043021029,
115.866685267832)) ;
#163206=CARTESIAN_POINT('Ctrl Pts',(-16.3722987255031,-12.5597317655866,
115.905265639768)) ;
#163207=CARTESIAN_POINT('Ctrl Pts',(-16.4461025747697,-12.5597317545878,
115.88103461589)) ;
#163208=CARTESIAN_POINT('Ctrl Pts',(-16.5199064240364,-12.5597317435889,
115.856803592012)) ;
#163209=CARTESIAN_POINT('Ctrl Pts',(-16.507239839906,-12.4956042801052,
115.818223220076)) ;
#163210=CARTESIAN_POINT('Ctrl Pts',(-16.4945732557756,-12.4314768166214,
115.77964284814)) ;
#163211=CARTESIAN_POINT('Ctrl Pts',(-16.420769406509,-12.4314768276203,
115.803873872018)) ;
#163212=CARTESIAN_POINT('Ctrl Pts',(-16.3469655572423,-12.4314768386191,
115.828104895896)) ;
#163213=CARTESIAN_POINT('Ctrl Pts',(-16.3596321413727,-12.4956043021029,
115.866685267832)) ;
#163214=CARTESIAN_POINT('Ctrl Pts',(-16.4533735886139,-12.3751190535725,
116.11656191809)) ;
#163215=CARTESIAN_POINT('Ctrl Pts',(-16.4602515014048,-12.4477568900421,
116.137510930954)) ;
#163216=CARTESIAN_POINT('Ctrl Pts',(-16.5340553487443,-12.4477568870231,
116.113279901206)) ;
#163217=CARTESIAN_POINT('Ctrl Pts',(-16.6078591960839,-12.4477568840041,
116.089048871459)) ;
#163218=CARTESIAN_POINT('Ctrl Pts',(-16.6009812832931,-12.3751190475345,
116.068099858596)) ;
#163219=CARTESIAN_POINT('Ctrl Pts',(-16.5941033705022,-12.3024812110649,
116.047150845732)) ;
#163220=CARTESIAN_POINT('Ctrl Pts',(-16.5202995231627,-12.3024812140839,
116.07138187548)) ;
#163221=CARTESIAN_POINT('Ctrl Pts',(-16.4464956758231,-12.3024812171029,
116.095612905227)) ;
#163222=CARTESIAN_POINT('Ctrl Pts',(-16.4533735886139,-12.3751190535725,
116.11656191809)) ;
#163223=CARTESIAN_POINT('Ctrl Pts',(-16.5533514223054,-12.3303020351126,
116.385717677923)) ;
#163224=CARTESIAN_POINT('Ctrl Pts',(-16.5539904411733,-12.4061784488461,
116.387664026431)) ;
#163225=CARTESIAN_POINT('Ctrl Pts',(-16.627794286868,-12.4061784491626,
116.363432991674)) ;
#163226=CARTESIAN_POINT('Ctrl Pts',(-16.7015981325627,-12.4061784494791,
116.339201956916)) ;
#163227=CARTESIAN_POINT('Ctrl Pts',(-16.7009591136948,-12.3303020357456,
116.337255608408)) ;
#163228=CARTESIAN_POINT('Ctrl Pts',(-16.7003200948268,-12.2544256220122,
116.335309259899)) ;
#163229=CARTESIAN_POINT('Ctrl Pts',(-16.6265162491321,-12.2544256216956,
116.359540294657)) ;
#163230=CARTESIAN_POINT('Ctrl Pts',(-16.5527124034374,-12.2544256213791,
116.383771329414)) ;
#163231=CARTESIAN_POINT('Ctrl Pts',(-16.5533514223054,-12.3303020351126,
116.385717677923)) ;
#163232=CARTESIAN_POINT('Ctrl Pts',(-16.6543061351395,-12.3631774170788,
116.657672551658)) ;
#163233=CARTESIAN_POINT('Ctrl Pts',(-16.6486321491688,-12.4368724586972,
116.64039050592)) ;
#163234=CARTESIAN_POINT('Ctrl Pts',(-16.7224359930919,-12.4368724595397,
116.616159465767)) ;
#163235=CARTESIAN_POINT('Ctrl Pts',(-16.796239837015,-12.4368724603823,
116.591928425613)) ;
#163236=CARTESIAN_POINT('Ctrl Pts',(-16.8019138229856,-12.363177418764,
116.609210471351)) ;
#163237=CARTESIAN_POINT('Ctrl Pts',(-16.8075878089563,-12.2894823771457,
116.626492517088)) ;
#163238=CARTESIAN_POINT('Ctrl Pts',(-16.7337839650332,-12.2894823763031,
116.650723557242)) ;
#163239=CARTESIAN_POINT('Ctrl Pts',(-16.6599801211101,-12.2894823754605,
116.674954597395)) ;
#163240=CARTESIAN_POINT('Ctrl Pts',(-16.6543061351395,-12.3631774170788,
116.657672551658)) ;
#163241=CARTESIAN_POINT('Ctrl Pts',(-16.7488808914051,-12.4713342743348,
116.91035898593)) ;
#163242=CARTESIAN_POINT('Ctrl Pts',(-16.7373265919045,-12.5375870378766,
116.875166453904)) ;
#163243=CARTESIAN_POINT('Ctrl Pts',(-16.8111304348947,-12.5375870373685,
116.850935410909)) ;
#163244=CARTESIAN_POINT('Ctrl Pts',(-16.884934277885,-12.5375870368604,
116.826704367914)) ;
#163245=CARTESIAN_POINT('Ctrl Pts',(-16.8964885773856,-12.4713342733185,
116.861896899941)) ;
#163246=CARTESIAN_POINT('Ctrl Pts',(-16.9080428768862,-12.4050815097766,
116.897089431967)) ;
#163247=CARTESIAN_POINT('Ctrl Pts',(-16.8342390338959,-12.4050815102848,
116.921320474962)) ;
#163248=CARTESIAN_POINT('Ctrl Pts',(-16.7604351909057,-12.4050815107929,
116.945551517957)) ;
#163249=CARTESIAN_POINT('Ctrl Pts',(-16.7488808914051,-12.4713342743348,
116.91035898593)) ;
#163250=CARTESIAN_POINT('Ctrl Pts',(-16.8318207118205,-12.6476404276989,
117.12747273466)) ;
#163251=CARTESIAN_POINT('Ctrl Pts',(-16.8151924034807,-12.7016806543081,
117.07682559036)) ;
#163252=CARTESIAN_POINT('Ctrl Pts',(-16.8889962461316,-12.7016806520052,
117.052594546332)) ;
#163253=CARTESIAN_POINT('Ctrl Pts',(-16.9628000887825,-12.7016806497023,
117.028363502303)) ;
#163254=CARTESIAN_POINT('Ctrl Pts',(-16.9794283971223,-12.6476404230932,
117.079010646603)) ;
#163255=CARTESIAN_POINT('Ctrl Pts',(-16.9960567054621,-12.5936001964841,
117.129657790903)) ;
#163256=CARTESIAN_POINT('Ctrl Pts',(-16.9222528628112,-12.5936001987869,
117.153888834932)) ;
#163257=CARTESIAN_POINT('Ctrl Pts',(-16.8484490201604,-12.5936002010898,
117.17811987896)) ;
#163258=CARTESIAN_POINT('Ctrl Pts',(-16.8318207118205,-12.6476404276989,
117.12747273466)) ;
#163259=CARTESIAN_POINT('Ctrl Pts',(-16.8975001296176,-12.8790215196565,
117.292056197982)) ;
#163260=CARTESIAN_POINT('Ctrl Pts',(-16.8769948136313,-12.9169844114343,
117.229600313953)) ;
#163261=CARTESIAN_POINT('Ctrl Pts',(-16.9507986566424,-12.916984408831,
117.205369271022)) ;
#163262=CARTESIAN_POINT('Ctrl Pts',(-17.0246024996535,-12.9169844062277,
117.18113822809)) ;
#163263=CARTESIAN_POINT('Ctrl Pts',(-17.0451078156398,-12.87902151445,117.24359411212)) ;
#163264=CARTESIAN_POINT('Ctrl Pts',(-17.0656131316261,-12.8410586226723,
117.306049996149)) ;
#163265=CARTESIAN_POINT('Ctrl Pts',(-16.991809288615,-12.8410586252756,
117.330281039081)) ;
#163266=CARTESIAN_POINT('Ctrl Pts',(-16.9180054456039,-12.8410586278788,
117.354512082012)) ;
#163267=CARTESIAN_POINT('Ctrl Pts',(-16.8975001296176,-12.8790215196565,
117.292056197982)) ;
#163268=CARTESIAN_POINT('Ctrl Pts',(-16.942134561038,-13.1499133657009,
117.392426703096)) ;
#163269=CARTESIAN_POINT('Ctrl Pts',(-16.9192185652055,-13.1690162421117,
117.322628277277)) ;
#163270=CARTESIAN_POINT('Ctrl Pts',(-16.9930224087252,-13.1690162422106,
117.298397235895)) ;
#163271=CARTESIAN_POINT('Ctrl Pts',(-17.0668262522449,-13.1690162423095,
117.274166194512)) ;
#163272=CARTESIAN_POINT('Ctrl Pts',(-17.0897422480774,-13.1499133658987,
117.343964620332)) ;
#163273=CARTESIAN_POINT('Ctrl Pts',(-17.1126582439099,-13.1308104894879,
117.413763046152)) ;
#163274=CARTESIAN_POINT('Ctrl Pts',(-17.0388544003902,-13.130810489389,
117.437994087534)) ;
#163275=CARTESIAN_POINT('Ctrl Pts',(-16.9650505568705,-13.1308104892901,
117.462225128916)) ;
#163276=CARTESIAN_POINT('Ctrl Pts',(-16.942134561038,-13.1499133657009,
117.392426703096)) ;
#163277=CARTESIAN_POINT('Ctrl Pts',(-16.9630233535542,-13.4386144880716,
117.420658950536)) ;
#163278=CARTESIAN_POINT('Ctrl Pts',(-16.9393477399357,-13.437586579743,
117.348546851583)) ;
#163279=CARTESIAN_POINT('Ctrl Pts',(-17.0131515834676,-13.4375865840391,
117.324315810238)) ;
#163280=CARTESIAN_POINT('Ctrl Pts',(-17.0869554269994,-13.4375865883353,
117.300084768893)) ;
#163281=CARTESIAN_POINT('Ctrl Pts',(-17.1106310406178,-13.438614496664,
117.372196867845)) ;
#163282=CARTESIAN_POINT('Ctrl Pts',(-17.1343066542363,-13.4396424049927,
117.444308966798)) ;
#163283=CARTESIAN_POINT('Ctrl Pts',(-17.0605028107044,-13.4396424006965,
117.468540008143)) ;
#163284=CARTESIAN_POINT('Ctrl Pts',(-16.9866989671726,-13.4396423964003,
117.492771049488)) ;
#163285=CARTESIAN_POINT('Ctrl Pts',(-16.9630233535542,-13.4386144880716,
117.420658950536)) ;
#163286=CARTESIAN_POINT('Ctrl Pts',(-16.9596443378371,-13.7268235527867,
117.37484372471)) ;
#163287=CARTESIAN_POINT('Ctrl Pts',(-16.9369052317055,-13.7056699529127,
117.305584076576)) ;
#163288=CARTESIAN_POINT('Ctrl Pts',(-17.0107090743469,-13.7056699630902,
117.281353032519)) ;
#163289=CARTESIAN_POINT('Ctrl Pts',(-17.0845129169883,-13.7056699732676,
117.257121988462)) ;
#163290=CARTESIAN_POINT('Ctrl Pts',(-17.10725202312,-13.7268235731417,117.326381636595)) ;
#163291=CARTESIAN_POINT('Ctrl Pts',(-17.1299911292516,-13.7479771730157,
117.395641284728)) ;
#163292=CARTESIAN_POINT('Ctrl Pts',(-17.0561872866102,-13.7479771628382,
117.419872328786)) ;
#163293=CARTESIAN_POINT('Ctrl Pts',(-16.9823834439688,-13.7479771526607,
117.444103372843)) ;
#163294=CARTESIAN_POINT('Ctrl Pts',(-16.9596443378371,-13.7268235527867,
117.37484372471)) ;
#163295=CARTESIAN_POINT('Ctrl Pts',(-16.9330916364897,-13.9914324144424,
117.258649259076)) ;
#163296=CARTESIAN_POINT('Ctrl Pts',(-16.912904485559,-13.9517725540924,
117.197162454839)) ;
#163297=CARTESIAN_POINT('Ctrl Pts',(-16.9867083264563,-13.9517725681727,
117.17293140547)) ;
#163298=CARTESIAN_POINT('Ctrl Pts',(-17.0605121673537,-13.9517725822531,
117.148700356101)) ;
#163299=CARTESIAN_POINT('Ctrl Pts',(-17.0806993182844,-13.9914324426031,
117.210187160338)) ;
#163300=CARTESIAN_POINT('Ctrl Pts',(-17.1008864692151,-14.0310923029532,
117.271673964574)) ;
#163301=CARTESIAN_POINT('Ctrl Pts',(-17.0270826283177,-14.0310922888728,
117.295905013944)) ;
#163302=CARTESIAN_POINT('Ctrl Pts',(-16.9532787874204,-14.0310922747924,
117.320136063313)) ;
#163303=CARTESIAN_POINT('Ctrl Pts',(-16.9330916364897,-13.9914324144424,
117.258649259076)) ;
#163304=CARTESIAN_POINT('Ctrl Pts',(-16.8858015410838,-14.2164140691066,
117.079108171634)) ;
#163305=CARTESIAN_POINT('Ctrl Pts',(-16.8696216727807,-14.1609879110475,
117.029826903861)) ;
#163306=CARTESIAN_POINT('Ctrl Pts',(-16.9434255108324,-14.1609879280051,
117.005595845824)) ;
#163307=CARTESIAN_POINT('Ctrl Pts',(-17.0172293488841,-14.1609879449628,
116.981364787787)) ;
#163308=CARTESIAN_POINT('Ctrl Pts',(-17.0334092171872,-14.2164141030218,
117.03064605556)) ;
#163309=CARTESIAN_POINT('Ctrl Pts',(-17.0495890854903,-14.2718402610809,
117.079927323333)) ;
#163310=CARTESIAN_POINT('Ctrl Pts',(-16.9757852474386,-14.2718402441232,
117.10415838137)) ;
#163311=CARTESIAN_POINT('Ctrl Pts',(-16.9019814093869,-14.2718402271656,
117.128389439407)) ;
#163312=CARTESIAN_POINT('Ctrl Pts',(-16.8858015410838,-14.2164140691066,
117.079108171634)) ;
#163313=CARTESIAN_POINT('Ctrl Pts',(-16.8218713013157,-14.384032579335,
116.848865519025)) ;
#163314=CARTESIAN_POINT('Ctrl Pts',(-16.8108667298453,-14.3168227397863,
116.815347370544)) ;
#163315=CARTESIAN_POINT('Ctrl Pts',(-16.8846705642333,-14.3168227556033,
116.791116301349)) ;
#163316=CARTESIAN_POINT('Ctrl Pts',(-16.9584743986213,-14.3168227714204,
116.766885232153)) ;
#163317=CARTESIAN_POINT('Ctrl Pts',(-16.9694789700917,-14.3840326109691,
116.800403380634)) ;
#163318=CARTESIAN_POINT('Ctrl Pts',(-16.9804835415621,-14.4512424505178,
116.833921529114)) ;
#163319=CARTESIAN_POINT('Ctrl Pts',(-16.906679707174,-14.4512424347008,
116.85815259831)) ;
#163320=CARTESIAN_POINT('Ctrl Pts',(-16.832875872786,-14.4512424188837,
116.882383667506)) ;
#163321=CARTESIAN_POINT('Ctrl Pts',(-16.8218713013157,-14.384032579335,
116.848865519025)) ;
#163322=CARTESIAN_POINT('Ctrl Pts',(-16.7469781937031,-14.4820529544929,
116.585338242812)) ;
#163323=CARTESIAN_POINT('Ctrl Pts',(-16.7419196115825,-14.40790231883,116.569930618666)) ;
#163324=CARTESIAN_POINT('Ctrl Pts',(-16.8157234425129,-14.4079023280758,
116.545699538938)) ;
#163325=CARTESIAN_POINT('Ctrl Pts',(-16.8895272734432,-14.4079023373216,
116.521468459211)) ;
#163326=CARTESIAN_POINT('Ctrl Pts',(-16.8945858555639,-14.4820529729845,
116.536876083358)) ;
#163327=CARTESIAN_POINT('Ctrl Pts',(-16.8996444376845,-14.5562036086474,
116.552283707504)) ;
#163328=CARTESIAN_POINT('Ctrl Pts',(-16.8258406067541,-14.5562035994016,
116.576514787232)) ;
#163329=CARTESIAN_POINT('Ctrl Pts',(-16.7520367758238,-14.5562035901558,
116.600745866959)) ;
#163330=CARTESIAN_POINT('Ctrl Pts',(-16.7469781937031,-14.4820529544929,
116.585338242812)) ;
#163331=CARTESIAN_POINT('Ctrl Pts',(-16.6668754248099,-14.5042250600488,
116.305877110692)) ;
#163332=CARTESIAN_POINT('Ctrl Pts',(-16.668136431742,-14.4284191898376,
116.309717935311)) ;
#163333=CARTESIAN_POINT('Ctrl Pts',(-16.7419402595713,-14.4284191877868,
116.285486846138)) ;
#163334=CARTESIAN_POINT('Ctrl Pts',(-16.8157440874006,-14.428419185736,
116.261255756966)) ;
#163335=CARTESIAN_POINT('Ctrl Pts',(-16.8144830804684,-14.5042250559472,
116.257414932347)) ;
#163336=CARTESIAN_POINT('Ctrl Pts',(-16.8132220735362,-14.5800309261584,
116.253574107729)) ;
#163337=CARTESIAN_POINT('Ctrl Pts',(-16.739418245707,-14.5800309282092,
116.277805196901)) ;
#163338=CARTESIAN_POINT('Ctrl Pts',(-16.6656144178777,-14.58003093026,116.302036286074)) ;
#163339=CARTESIAN_POINT('Ctrl Pts',(-16.6668754248099,-14.5042250600488,
116.305877110692)) ;
#163340=CARTESIAN_POINT('Ctrl Pts',(-16.5879598850496,-14.4479097103847,
116.029910236852)) ;
#163341=CARTESIAN_POINT('Ctrl Pts',(-16.5954692147568,-14.3759257111989,
116.052782444672)) ;
#163342=CARTESIAN_POINT('Ctrl Pts',(-16.6692730404099,-14.3759256925376,
116.028551348871)) ;
#163343=CARTESIAN_POINT('Ctrl Pts',(-16.743076866063,-14.3759256738764,
116.00432025307)) ;
#163344=CARTESIAN_POINT('Ctrl Pts',(-16.7355675363558,-14.4479096730622,
115.98144804525)) ;
#163345=CARTESIAN_POINT('Ctrl Pts',(-16.7280582066486,-14.519893672248,
115.95857583743)) ;
#163346=CARTESIAN_POINT('Ctrl Pts',(-16.6542543809955,-14.5198936909092,
115.982806933231)) ;
#163347=CARTESIAN_POINT('Ctrl Pts',(-16.5804505553424,-14.5198937095705,
116.007038029031)) ;
#163348=CARTESIAN_POINT('Ctrl Pts',(-16.5879598850496,-14.4479097103847,
116.029910236852)) ;
#163349=CARTESIAN_POINT('Ctrl Pts',(-16.5174994343308,-14.3189148106109,
115.780020371028)) ;
#163350=CARTESIAN_POINT('Ctrl Pts',(-16.5306689565097,-14.2558334084202,
115.820132611976)) ;
#163351=CARTESIAN_POINT('Ctrl Pts',(-16.6044727826075,-14.2558333716659,
115.79590151753)) ;
#163352=CARTESIAN_POINT('Ctrl Pts',(-16.6782766087053,-14.2558333349115,
115.771670423084)) ;
#163353=CARTESIAN_POINT('Ctrl Pts',(-16.6651070865265,-14.3189147371022,
115.731558182136)) ;
#163354=CARTESIAN_POINT('Ctrl Pts',(-16.6519375643476,-14.3819961392929,
115.691445941188)) ;
#163355=CARTESIAN_POINT('Ctrl Pts',(-16.5781337382498,-14.3819961760472,
115.715677035634)) ;
#163356=CARTESIAN_POINT('Ctrl Pts',(-16.504329912152,-14.3819962128016,
115.73990813008)) ;
#163357=CARTESIAN_POINT('Ctrl Pts',(-16.5174994343308,-14.3189148106109,
115.780020371028)) ;
#163358=CARTESIAN_POINT('Ctrl Pts',(-16.4601033314479,-14.1239822238445,
115.569589941592)) ;
#163359=CARTESIAN_POINT('Ctrl Pts',(-16.4780361084618,-14.0744187665949,
115.624210288398)) ;
#163360=CARTESIAN_POINT('Ctrl Pts',(-16.5518399363937,-14.074418709394,
115.599979199538)) ;
#163361=CARTESIAN_POINT('Ctrl Pts',(-16.6256437643256,-14.0744186521931,
115.575748110678)) ;
#163362=CARTESIAN_POINT('Ctrl Pts',(-16.6077109873116,-14.1239821094427,
115.521127763872)) ;
#163363=CARTESIAN_POINT('Ctrl Pts',(-16.5897782102976,-14.1735455666924,
115.466507417066)) ;
#163364=CARTESIAN_POINT('Ctrl Pts',(-16.5159743823658,-14.1735456238933,
115.490738505926)) ;
#163365=CARTESIAN_POINT('Ctrl Pts',(-16.4421705544339,-14.1735456810942,
115.514969594786)) ;
#163366=CARTESIAN_POINT('Ctrl Pts',(-16.4601033314479,-14.1239822238445,
115.569589941592)) ;
#163367=CARTESIAN_POINT('Ctrl Pts',(-16.4215747130303,-13.8804446676162,
115.416952493218)) ;
#163368=CARTESIAN_POINT('Ctrl Pts',(-16.4429534477659,-13.8478127953866,
115.482068671354)) ;
#163369=CARTESIAN_POINT('Ctrl Pts',(-16.5167572801787,-13.8478127217154,
115.457837596143)) ;
#163370=CARTESIAN_POINT('Ctrl Pts',(-16.5905611125915,-13.8478126480443,
115.433606520931)) ;
#163371=CARTESIAN_POINT('Ctrl Pts',(-16.5691823778558,-13.8804445202739,
115.368490342794)) ;
#163372=CARTESIAN_POINT('Ctrl Pts',(-16.5478036431202,-13.9130763925035,
115.303374164658)) ;
#163373=CARTESIAN_POINT('Ctrl Pts',(-16.4739998107074,-13.9130764661746,
115.32760523987)) ;
#163374=CARTESIAN_POINT('Ctrl Pts',(-16.4001959782946,-13.9130765398458,
115.351836315081)) ;
#163375=CARTESIAN_POINT('Ctrl Pts',(-16.4215747130303,-13.8804446676162,
115.416952493218)) ;
#163376=CARTESIAN_POINT('Ctrl Pts',(-16.4047818629355,-13.6007259227713,
115.330092652858)) ;
#163377=CARTESIAN_POINT('Ctrl Pts',(-16.4281032255851,-13.5875751539527,
115.401125762342)) ;
#163378=CARTESIAN_POINT('Ctrl Pts',(-16.5019070640968,-13.5875750652436,
115.376894705707)) ;
#163379=CARTESIAN_POINT('Ctrl Pts',(-16.5757109026085,-13.5875749765345,
115.352663649072)) ;
#163380=CARTESIAN_POINT('Ctrl Pts',(-16.5523895399589,-13.6007257453531,
115.281630539587)) ;
#163381=CARTESIAN_POINT('Ctrl Pts',(-16.5290681773093,-13.6138765141717,
115.210597430103)) ;
#163382=CARTESIAN_POINT('Ctrl Pts',(-16.4552643387976,-13.6138766028808,
115.234828486739)) ;
#163383=CARTESIAN_POINT('Ctrl Pts',(-16.3814605002859,-13.6138766915899,
115.259059543374)) ;
#163384=CARTESIAN_POINT('Ctrl Pts',(-16.4047818629355,-13.6007259227713,
115.330092652858)) ;
#163385=CARTESIAN_POINT('Ctrl Pts',(-16.4121369550956,-13.310886389785,
115.317177989403)) ;
#163386=CARTESIAN_POINT('Ctrl Pts',(-16.4357094306014,-13.3179522424612,
115.38897594822)) ;
#163387=CARTESIAN_POINT('Ctrl Pts',(-16.5095132768189,-13.3179521481175,
115.364744915055)) ;
#163388=CARTESIAN_POINT('Ctrl Pts',(-16.5833171230364,-13.3179520537738,
115.34051388189)) ;
#163389=CARTESIAN_POINT('Ctrl Pts',(-16.5597446475305,-13.3108862010977,
115.268715923073)) ;
#163390=CARTESIAN_POINT('Ctrl Pts',(-16.5361721720247,-13.3038203484215,
115.196917964256)) ;
#163391=CARTESIAN_POINT('Ctrl Pts',(-16.4623683258072,-13.3038204427652,
115.221148997421)) ;
#163392=CARTESIAN_POINT('Ctrl Pts',(-16.3885644795897,-13.3038205371088,
115.245380030586)) ;
#163393=CARTESIAN_POINT('Ctrl Pts',(-16.4121369550956,-13.310886389785,
115.317177989403)) ;
#163394=CARTESIAN_POINT('Ctrl Pts',(-16.4435486385353,-13.0275729196668,
115.377389997303)) ;
#163395=CARTESIAN_POINT('Ctrl Pts',(-16.4656962766156,-13.0544289037497,
115.444848131314)) ;
#163396=CARTESIAN_POINT('Ctrl Pts',(-16.539500131069,-13.0544288105617,
115.420617123234)) ;
#163397=CARTESIAN_POINT('Ctrl Pts',(-16.6133039855224,-13.0544287173738,
115.396386115154)) ;
#163398=CARTESIAN_POINT('Ctrl Pts',(-16.5911563474421,-13.0275727332909,
115.328927981143)) ;
#163399=CARTESIAN_POINT('Ctrl Pts',(-16.5690087093617,-13.000716749208,
115.261469847132)) ;
#163400=CARTESIAN_POINT('Ctrl Pts',(-16.4952048549083,-13.000716842396,
115.285700855212)) ;
#163401=CARTESIAN_POINT('Ctrl Pts',(-16.4214010004549,-13.000716935584,
115.309931863291)) ;
#163402=CARTESIAN_POINT('Ctrl Pts',(-16.4435486385353,-13.0275729196668,
115.377389997303)) ;
#163403=CARTESIAN_POINT('Ctrl Pts',(-16.4978834158618,-12.7715214711428,
115.507323795441)) ;
#163404=CARTESIAN_POINT('Ctrl Pts',(-16.5170059842238,-12.8162933310401,
115.565568055265)) ;
#163405=CARTESIAN_POINT('Ctrl Pts',(-16.5908098468287,-12.8162932472945,
115.541337072013)) ;
#163406=CARTESIAN_POINT('Ctrl Pts',(-16.6646137094336,-12.8162931635489,
115.517106088762)) ;
#163407=CARTESIAN_POINT('Ctrl Pts',(-16.6454911410716,-12.7715213036516,
115.458861828938)) ;
#163408=CARTESIAN_POINT('Ctrl Pts',(-16.6263685727096,-12.7267494437543,
115.400617569114)) ;
#163409=CARTESIAN_POINT('Ctrl Pts',(-16.5525647101047,-12.7267495274999,
115.424848552366)) ;
#163410=CARTESIAN_POINT('Ctrl Pts',(-16.4787608474998,-12.7267496112455,
115.449079535617)) ;
#163411=CARTESIAN_POINT('Ctrl Pts',(-16.4978834158618,-12.7715214711428,
115.507323795441)) ;
#163412=CARTESIAN_POINT('Ctrl Pts',(-16.5717603357923,-12.5625540682405,
115.696844987537)) ;
#163413=CARTESIAN_POINT('Ctrl Pts',(-16.5864877055185,-12.6219811291845,
115.74170218153)) ;
#163414=CARTESIAN_POINT('Ctrl Pts',(-16.6602915750344,-12.6219810632867,
115.717471219328)) ;
#163415=CARTESIAN_POINT('Ctrl Pts',(-16.7340954445502,-12.6219809973889,
115.693240257126)) ;
#163416=CARTESIAN_POINT('Ctrl Pts',(-16.7193680748241,-12.5625539364449,
115.648383063133)) ;
#163417=CARTESIAN_POINT('Ctrl Pts',(-16.7046407050979,-12.5031268755009,
115.603525869141)) ;
#163418=CARTESIAN_POINT('Ctrl Pts',(-16.630836835582,-12.5031269413987,
115.627756831343)) ;
#163419=CARTESIAN_POINT('Ctrl Pts',(-16.5570329660662,-12.5031270072965,
115.651987793545)) ;
#163420=CARTESIAN_POINT('Ctrl Pts',(-16.5717603357923,-12.5625540682405,
115.696844987537)) ;
#163421=CARTESIAN_POINT('Ctrl Pts',(-16.6600063471763,-12.4155360311479,
115.930369190556)) ;
#163422=CARTESIAN_POINT('Ctrl Pts',(-16.6693238142624,-12.4853145096468,
115.958748694017)) ;
#163423=CARTESIAN_POINT('Ctrl Pts',(-16.7431276886547,-12.4853144677288,
115.934517746667)) ;
#163424=CARTESIAN_POINT('Ctrl Pts',(-16.8169315630469,-12.4853144258108,
115.910286799318)) ;
#163425=CARTESIAN_POINT('Ctrl Pts',(-16.8076140959607,-12.4155359473118,
115.881907295858)) ;
#163426=CARTESIAN_POINT('Ctrl Pts',(-16.7982966288746,-12.3457574688128,
115.853527792397)) ;
#163427=CARTESIAN_POINT('Ctrl Pts',(-16.7244927544824,-12.3457575107309,
115.877758739747)) ;
#163428=CARTESIAN_POINT('Ctrl Pts',(-16.6506888800901,-12.3457575526489,
115.901989687096)) ;
#163429=CARTESIAN_POINT('Ctrl Pts',(-16.6600063471763,-12.4155360311479,
115.930369190556)) ;
#163430=CARTESIAN_POINT('Ctrl Pts',(-16.7583961657612,-12.339199302571,
116.194502768036)) ;
#163431=CARTESIAN_POINT('Ctrl Pts',(-16.7615937653379,-12.4144106897109,
116.204242142512)) ;
#163432=CARTESIAN_POINT('Ctrl Pts',(-16.835397642295,-12.41441067568,116.180011202975)) ;
#163433=CARTESIAN_POINT('Ctrl Pts',(-16.909201519252,-12.4144106616491,
116.155780263438)) ;
#163434=CARTESIAN_POINT('Ctrl Pts',(-16.9060039196752,-12.3391992745091,
116.146040888962)) ;
#163435=CARTESIAN_POINT('Ctrl Pts',(-16.9028063200983,-12.2639878873692,
116.136301514485)) ;
#163436=CARTESIAN_POINT('Ctrl Pts',(-16.8290024431413,-12.2639879014001,
116.160532454023)) ;
#163437=CARTESIAN_POINT('Ctrl Pts',(-16.7551985661843,-12.2639879154311,
116.18476339356)) ;
#163438=CARTESIAN_POINT('Ctrl Pts',(-16.7583961657612,-12.339199302571,
116.194502768036)) ;
#163439=CARTESIAN_POINT('Ctrl Pts',(-16.8595422687567,-12.3403409953756,
116.467185667784)) ;
#163440=CARTESIAN_POINT('Ctrl Pts',(-16.8564152393437,-12.4155840268561,
116.457661242822)) ;
#163441=CARTESIAN_POINT('Ctrl Pts',(-16.9302191160928,-12.4155840418634,
116.433430302651)) ;
#163442=CARTESIAN_POINT('Ctrl Pts',(-17.0040229928419,-12.4155840568707,
116.409199362481)) ;
#163443=CARTESIAN_POINT('Ctrl Pts',(-17.0071500222549,-12.3403410253901,
116.418723787443)) ;
#163444=CARTESIAN_POINT('Ctrl Pts',(-17.0102770516679,-12.2650979939095,
116.428248212404)) ;
#163445=CARTESIAN_POINT('Ctrl Pts',(-16.9364731749188,-12.2650979789023,
116.452479152575)) ;
#163446=CARTESIAN_POINT('Ctrl Pts',(-16.8626692981697,-12.265097963895,
116.476710092745)) ;
#163447=CARTESIAN_POINT('Ctrl Pts',(-16.8595422687567,-12.3403409953756,
116.467185667784)) ;
#163448=CARTESIAN_POINT('Ctrl Pts',(-16.9578689738167,-12.4190382667156,
116.731080805892)) ;
#163449=CARTESIAN_POINT('Ctrl Pts',(-16.9486089308596,-12.488899337021,
116.702876211193)) ;
#163450=CARTESIAN_POINT('Ctrl Pts',(-17.0224128045713,-12.488899379198,
116.678645261771)) ;
#163451=CARTESIAN_POINT('Ctrl Pts',(-17.096216678283,-12.488899421375,116.654414312349)) ;
#163452=CARTESIAN_POINT('Ctrl Pts',(-17.1054767212401,-12.4190383510696,
116.682618907047)) ;
#163453=CARTESIAN_POINT('Ctrl Pts',(-17.1147367641971,-12.3491772807642,
116.710823501746)) ;
#163454=CARTESIAN_POINT('Ctrl Pts',(-17.0409328904855,-12.3491772385872,
116.735054451168)) ;
#163455=CARTESIAN_POINT('Ctrl Pts',(-16.9671290167738,-12.3491771964102,
116.75928540059)) ;
#163456=CARTESIAN_POINT('Ctrl Pts',(-16.9578689738167,-12.4190382667156,
116.731080805892)) ;
#163457=CARTESIAN_POINT('Ctrl Pts',(-17.0458999041783,-12.5685297170459,
116.963876177155)) ;
#163458=CARTESIAN_POINT('Ctrl Pts',(-17.0312110845687,-12.6280576016783,
116.919136404655)) ;
#163459=CARTESIAN_POINT('Ctrl Pts',(-17.105014953103,-12.6280576665216,
116.894905439464)) ;
#163460=CARTESIAN_POINT('Ctrl Pts',(-17.1788188216374,-12.6280577313649,
116.870674474273)) ;
#163461=CARTESIAN_POINT('Ctrl Pts',(-17.1935076412471,-12.5685298467324,
116.915414246773)) ;
#163462=CARTESIAN_POINT('Ctrl Pts',(-17.2081964608567,-12.5090019621,116.960154019273)) ;
#163463=CARTESIAN_POINT('Ctrl Pts',(-17.1343925923223,-12.5090018972567,
116.984384984464)) ;
#163464=CARTESIAN_POINT('Ctrl Pts',(-17.0605887237879,-12.5090018324134,
117.008615949655)) ;
#163465=CARTESIAN_POINT('Ctrl Pts',(-17.0458999041783,-12.5685297170459,
116.963876177155)) ;
#163466=CARTESIAN_POINT('Ctrl Pts',(-17.1191748552296,-12.7793086778933,
117.151568386626)) ;
#163467=CARTESIAN_POINT('Ctrl Pts',(-17.1000825757091,-12.8242097756673,
117.093416385657)) ;
#163468=CARTESIAN_POINT('Ctrl Pts',(-17.1738864372224,-12.8242098564781,
117.069185399081)) ;
#163469=CARTESIAN_POINT('Ctrl Pts',(-17.2476902987357,-12.8242099372889,
117.044954412505)) ;
#163470=CARTESIAN_POINT('Ctrl Pts',(-17.2667825782563,-12.7793088395149,
117.103106413474)) ;
#163471=CARTESIAN_POINT('Ctrl Pts',(-17.2858748577768,-12.7344077417409,
117.161258414442)) ;
#163472=CARTESIAN_POINT('Ctrl Pts',(-17.2120709962635,-12.7344076609301,
117.185489401019)) ;
#163473=CARTESIAN_POINT('Ctrl Pts',(-17.1382671347501,-12.7344075801193,
117.209720387595)) ;
#163474=CARTESIAN_POINT('Ctrl Pts',(-17.1191748552296,-12.7793086778933,
117.151568386626)) ;
#163475=CARTESIAN_POINT('Ctrl Pts',(-17.1727252854914,-13.0361487300971,
117.279168850677)) ;
#163476=CARTESIAN_POINT('Ctrl Pts',(-17.1506002151848,-13.0631853690337,
117.211779458213)) ;
#163477=CARTESIAN_POINT('Ctrl Pts',(-17.2244040687652,-13.0631854575266,
117.187548447474)) ;
#163478=CARTESIAN_POINT('Ctrl Pts',(-17.2982079223455,-13.0631855460195,
117.163317436735)) ;
#163479=CARTESIAN_POINT('Ctrl Pts',(-17.320332992652,-13.0361489070829,
117.230706829199)) ;
#163480=CARTESIAN_POINT('Ctrl Pts',(-17.3424580629586,-13.0091122681464,
117.298096221663)) ;
#163481=CARTESIAN_POINT('Ctrl Pts',(-17.2686542093782,-13.0091121796535,
117.322327232402)) ;
#163482=CARTESIAN_POINT('Ctrl Pts',(-17.1948503557979,-13.0091120911606,
117.346558243141)) ;
#163483=CARTESIAN_POINT('Ctrl Pts',(-17.1727252854914,-13.0361487300971,
117.279168850677)) ;
#163484=CARTESIAN_POINT('Ctrl Pts',(-17.2034288318534,-13.3199156358865,
117.337236471295)) ;
#163485=CARTESIAN_POINT('Ctrl Pts',(-17.1798603419687,-13.3271808481679,
117.265450655579)) ;
#163486=CARTESIAN_POINT('Ctrl Pts',(-17.2536641876918,-13.3271809363831,
117.241219620908)) ;
#163487=CARTESIAN_POINT('Ctrl Pts',(-17.3274680334149,-13.3271810245983,
117.216988586238)) ;
#163488=CARTESIAN_POINT('Ctrl Pts',(-17.3510365232996,-13.3199158123169,
117.288774401953)) ;
#163489=CARTESIAN_POINT('Ctrl Pts',(-17.3746050131842,-13.3126506000355,
117.360560217669)) ;
#163490=CARTESIAN_POINT('Ctrl Pts',(-17.3008011674611,-13.3126505118203,
117.38479125234)) ;
#163491=CARTESIAN_POINT('Ctrl Pts',(-17.226997321738,-13.312650423605,117.409022287011)) ;
#163492=CARTESIAN_POINT('Ctrl Pts',(-17.2034288318534,-13.3199156358865,
117.337236471295)) ;
#163493=CARTESIAN_POINT('Ctrl Pts',(-17.2099599842142,-13.61053350134,117.321699031089)) ;
#163494=CARTESIAN_POINT('Ctrl Pts',(-17.1866331051387,-13.5975190949255,
117.250649122791)) ;
#163495=CARTESIAN_POINT('Ctrl Pts',(-17.2604369438178,-13.5975191756466,
117.226418066665)) ;
#163496=CARTESIAN_POINT('Ctrl Pts',(-17.334240782497,-13.5975192563676,
117.20218701054)) ;
#163497=CARTESIAN_POINT('Ctrl Pts',(-17.3575676615725,-13.6105336627821,
117.273236918838)) ;
#163498=CARTESIAN_POINT('Ctrl Pts',(-17.3808945406481,-13.6235480691965,
117.344286827137)) ;
#163499=CARTESIAN_POINT('Ctrl Pts',(-17.3070907019689,-13.6235479884755,
117.368517883263)) ;
#163500=CARTESIAN_POINT('Ctrl Pts',(-17.2332868632897,-13.6235479077544,
117.392748939388)) ;
#163501=CARTESIAN_POINT('Ctrl Pts',(-17.2099599842142,-13.61053350134,117.321699031089)) ;
#163502=CARTESIAN_POINT('Ctrl Pts',(-17.1925797786754,-13.8877845324202,
117.233281417969)) ;
#163503=CARTESIAN_POINT('Ctrl Pts',(-17.1711652640745,-13.8553930149523,
117.168056263156)) ;
#163504=CARTESIAN_POINT('Ctrl Pts',(-17.24496909722,-13.8553930819553,117.143825190176)) ;
#163505=CARTESIAN_POINT('Ctrl Pts',(-17.3187729303654,-13.8553931489583,
117.119594117196)) ;
#163506=CARTESIAN_POINT('Ctrl Pts',(-17.3401874449663,-13.8877846664262,
117.184819272008)) ;
#163507=CARTESIAN_POINT('Ctrl Pts',(-17.3616019595672,-13.9201761838941,
117.250044426821)) ;
#163508=CARTESIAN_POINT('Ctrl Pts',(-17.2877981264218,-13.9201761168911,
117.274275499801)) ;
#163509=CARTESIAN_POINT('Ctrl Pts',(-17.2139942932763,-13.9201760498881,
117.298506572782)) ;
#163510=CARTESIAN_POINT('Ctrl Pts',(-17.1925797786754,-13.8877845324202,
117.233281417969)) ;
#163511=CARTESIAN_POINT('Ctrl Pts',(-17.1531888988296,-14.1315208949384,
117.077791857519)) ;
#163512=CARTESIAN_POINT('Ctrl Pts',(-17.135227002644,-14.0820626171462,
117.023082821159)) ;
#163513=CARTESIAN_POINT('Ctrl Pts',(-17.2090308323232,-14.0820626666498,
116.998851737621)) ;
#163514=CARTESIAN_POINT('Ctrl Pts',(-17.2828346620024,-14.0820627161535,
116.974620654083)) ;
#163515=CARTESIAN_POINT('Ctrl Pts',(-17.300796558188,-14.1315209939457,
117.029329690443)) ;
#163516=CARTESIAN_POINT('Ctrl Pts',(-17.3187584543736,-14.1809792717379,
117.084038726803)) ;
#163517=CARTESIAN_POINT('Ctrl Pts',(-17.2449546246944,-14.1809792222342,
117.108269810341)) ;
#163518=CARTESIAN_POINT('Ctrl Pts',(-17.1711507950152,-14.1809791727306,
117.132500893879)) ;
#163519=CARTESIAN_POINT('Ctrl Pts',(-17.1531888988296,-14.1315208949384,
117.077791857519)) ;
#163520=CARTESIAN_POINT('Ctrl Pts',(-17.0955345319982,-14.3236676354294,
116.866747533545)) ;
#163521=CARTESIAN_POINT('Ctrl Pts',(-17.0823042094018,-14.2607186290668,
116.826450106743)) ;
#163522=CARTESIAN_POINT('Ctrl Pts',(-17.1561080375986,-14.260718660624,
116.80221901869)) ;
#163523=CARTESIAN_POINT('Ctrl Pts',(-17.2299118657954,-14.2607186921811,
116.777987930637)) ;
#163524=CARTESIAN_POINT('Ctrl Pts',(-17.2431421883918,-14.3236676985437,
116.818285357438)) ;
#163525=CARTESIAN_POINT('Ctrl Pts',(-17.2563725109882,-14.3866167049062,
116.85858278424)) ;
#163526=CARTESIAN_POINT('Ctrl Pts',(-17.1825686827914,-14.3866166733491,
116.882813872293)) ;
#163527=CARTESIAN_POINT('Ctrl Pts',(-17.1087648545946,-14.3866166417919,
116.907044960346)) ;
#163528=CARTESIAN_POINT('Ctrl Pts',(-17.0955345319982,-14.3236676354294,
116.866747533545)) ;
#163529=CARTESIAN_POINT('Ctrl Pts',(-17.0243702739968,-14.451213086268,
116.614520189238)) ;
#163530=CARTESIAN_POINT('Ctrl Pts',(-17.016822677996,-14.3792631912131,
116.591531430573)) ;
#163531=CARTESIAN_POINT('Ctrl Pts',(-17.0906265067015,-14.3792632058746,
116.567300344069)) ;
#163532=CARTESIAN_POINT('Ctrl Pts',(-17.164430335407,-14.3792632205361,
116.543069257566)) ;
#163533=CARTESIAN_POINT('Ctrl Pts',(-17.1719779314079,-14.451213115591,
116.56605801623)) ;
#163534=CARTESIAN_POINT('Ctrl Pts',(-17.1795255274087,-14.5231630106458,
116.589046774895)) ;
#163535=CARTESIAN_POINT('Ctrl Pts',(-17.1057216987032,-14.5231629959843,
116.613277861399)) ;
#163536=CARTESIAN_POINT('Ctrl Pts',(-17.0319178699977,-14.5231629813228,
116.637508947902)) ;
#163537=CARTESIAN_POINT('Ctrl Pts',(-17.0243702739968,-14.451213086268,
116.614520189238)) ;
#163538=CARTESIAN_POINT('Ctrl Pts',(-16.9454296666756,-14.5046478984509,
116.338545787343)) ;
#163539=CARTESIAN_POINT('Ctrl Pts',(-16.9441177229474,-14.4288576762163,
116.3345498192)) ;
#163540=CARTESIAN_POINT('Ctrl Pts',(-17.0179215539013,-14.4288576774106,
116.310318739545)) ;
#163541=CARTESIAN_POINT('Ctrl Pts',(-17.0917253848553,-14.4288576786049,
116.286087659889)) ;
#163542=CARTESIAN_POINT('Ctrl Pts',(-17.0930373285836,-14.5046479008395,
116.290083628032)) ;
#163543=CARTESIAN_POINT('Ctrl Pts',(-17.0943492723118,-14.5804381230741,
116.294079596175)) ;
#163544=CARTESIAN_POINT('Ctrl Pts',(-17.0205454413578,-14.5804381218798,
116.318310675831)) ;
#163545=CARTESIAN_POINT('Ctrl Pts',(-16.9467416104039,-14.5804381206855,
116.342541755486)) ;
#163546=CARTESIAN_POINT('Ctrl Pts',(-16.9454296666756,-14.5046478984509,
116.338545787343)) ;
#163547=CARTESIAN_POINT('Ctrl Pts',(-16.8656122340257,-14.4801334339684,
116.060046712965)) ;
#163548=CARTESIAN_POINT('Ctrl Pts',(-16.8706036868272,-14.4059401882447,
116.075249873451)) ;
#163549=CARTESIAN_POINT('Ctrl Pts',(-16.9444075204913,-14.405940180657,
116.051018802051)) ;
#163550=CARTESIAN_POINT('Ctrl Pts',(-17.0182113541555,-14.4059401730692,
116.02678773065)) ;
#163551=CARTESIAN_POINT('Ctrl Pts',(-17.013219901354,-14.4801334187929,
116.011584570164)) ;
#163552=CARTESIAN_POINT('Ctrl Pts',(-17.0082284485525,-14.5543266645165,
115.996381409677)) ;
#163553=CARTESIAN_POINT('Ctrl Pts',(-16.9344246148884,-14.5543266721042,
116.020612481078)) ;
#163554=CARTESIAN_POINT('Ctrl Pts',(-16.8606207812242,-14.554326679692,
116.044843552478)) ;
#163555=CARTESIAN_POINT('Ctrl Pts',(-16.8656122340257,-14.4801334339684,
116.060046712965)) ;
#163556=CARTESIAN_POINT('Ctrl Pts',(-16.790980956793,-14.3800974324411,
115.797335713982)) ;
#163557=CARTESIAN_POINT('Ctrl Pts',(-16.801923417816,-14.3127767665056,
115.830664685171)) ;
#163558=CARTESIAN_POINT('Ctrl Pts',(-16.8757272545943,-14.3127767543614,
115.806433623256)) ;
#163559=CARTESIAN_POINT('Ctrl Pts',(-16.9495310913725,-14.3127767422172,
115.78220256134)) ;
#163560=CARTESIAN_POINT('Ctrl Pts',(-16.9385886303495,-14.3800974081526,
115.748873590151)) ;
#163561=CARTESIAN_POINT('Ctrl Pts',(-16.9276461693265,-14.4474180740881,
115.715544618961)) ;
#163562=CARTESIAN_POINT('Ctrl Pts',(-16.8538423325482,-14.4474180862324,
115.739775680876)) ;
#163563=CARTESIAN_POINT('Ctrl Pts',(-16.78003849577,-14.4474180983766,115.764006742792)) ;
#163564=CARTESIAN_POINT('Ctrl Pts',(-16.790980956793,-14.3800974324411,
115.797335713982)) ;
#163565=CARTESIAN_POINT('Ctrl Pts',(-16.7272992435064,-14.2097836883392,
115.567723704897)) ;
#163566=CARTESIAN_POINT('Ctrl Pts',(-16.7434426567899,-14.1542529210645,
115.616893937324)) ;
#163567=CARTESIAN_POINT('Ctrl Pts',(-16.8172464968672,-14.1542529100711,
115.592662885457)) ;
#163568=CARTESIAN_POINT('Ctrl Pts',(-16.8910503369444,-14.1542528990776,
115.568431833589)) ;
#163569=CARTESIAN_POINT('Ctrl Pts',(-16.8749069236608,-14.2097836663522,
115.519261601162)) ;
#163570=CARTESIAN_POINT('Ctrl Pts',(-16.8587635103773,-14.2653144336269,
115.470091368735)) ;
#163571=CARTESIAN_POINT('Ctrl Pts',(-16.7849596703,-14.2653144446203,115.494322420602)) ;
#163572=CARTESIAN_POINT('Ctrl Pts',(-16.7111558302228,-14.2653144556138,
115.518553472469)) ;
#163573=CARTESIAN_POINT('Ctrl Pts',(-16.7272992435064,-14.2097836883392,
115.567723704897)) ;
#163574=CARTESIAN_POINT('Ctrl Pts',(-16.6808108315259,-13.9844447661634,
115.3908060488)) ;
#163575=CARTESIAN_POINT('Ctrl Pts',(-16.7009554993096,-13.944564790948,
115.452163456727)) ;
#163576=CARTESIAN_POINT('Ctrl Pts',(-16.7747593412743,-13.9445647824093,
115.427932410608)) ;
#163577=CARTESIAN_POINT('Ctrl Pts',(-16.848563183239,-13.9445647738706,
115.40370136449)) ;
#163578=CARTESIAN_POINT('Ctrl Pts',(-16.8284185154553,-13.984444749086,
115.342343956563)) ;
#163579=CARTESIAN_POINT('Ctrl Pts',(-16.8082738476717,-14.0243247243014,
115.280986548637)) ;
#163580=CARTESIAN_POINT('Ctrl Pts',(-16.734470005707,-14.0243247328401,
115.305217594755)) ;
#163581=CARTESIAN_POINT('Ctrl Pts',(-16.6606661637423,-14.0243247413788,
115.329448640873)) ;
#163582=CARTESIAN_POINT('Ctrl Pts',(-16.6808108315259,-13.9844447661634,
115.3908060488)) ;
#163583=CARTESIAN_POINT('Ctrl Pts',(-16.6547738612727,-13.7175338810347,
115.275995973862)) ;
#163584=CARTESIAN_POINT('Ctrl Pts',(-16.6775017259514,-13.6962312533339,
115.345221382617)) ;
#163585=CARTESIAN_POINT('Ctrl Pts',(-16.7513055691903,-13.6962312496336,
115.32099034038)) ;
#163586=CARTESIAN_POINT('Ctrl Pts',(-16.8251094124292,-13.6962312459334,
115.296759298142)) ;
#163587=CARTESIAN_POINT('Ctrl Pts',(-16.8023815477505,-13.7175338736341,
115.227533889387)) ;
#163588=CARTESIAN_POINT('Ctrl Pts',(-16.7796536830717,-13.7388365013348,
115.158308480631)) ;
#163589=CARTESIAN_POINT('Ctrl Pts',(-16.7058498398329,-13.7388365050351,
115.182539522869)) ;
#163590=CARTESIAN_POINT('Ctrl Pts',(-16.632045996594,-13.7388365087354,
115.206770565106)) ;
#163591=CARTESIAN_POINT('Ctrl Pts',(-16.6547738612727,-13.7175338810347,
115.275995973862)) ;
#163592=CARTESIAN_POINT('Ctrl Pts',(-16.6522344647069,-13.4290941380284,
115.232763303442)) ;
#163593=CARTESIAN_POINT('Ctrl Pts',(-16.6759083668004,-13.42790072271,115.304870189438)) ;
#163594=CARTESIAN_POINT('Ctrl Pts',(-16.7497122103021,-13.4279007232461,
115.280639148001)) ;
#163595=CARTESIAN_POINT('Ctrl Pts',(-16.8235160538039,-13.4279007237822,
115.256408106565)) ;
#163596=CARTESIAN_POINT('Ctrl Pts',(-16.7998421517105,-13.4290941391006,
115.184301220568)) ;
#163597=CARTESIAN_POINT('Ctrl Pts',(-16.7761682496171,-13.430287554419,
115.112194334572)) ;
#163598=CARTESIAN_POINT('Ctrl Pts',(-16.7023644061153,-13.4302875538829,
115.136425376008)) ;
#163599=CARTESIAN_POINT('Ctrl Pts',(-16.6285605626135,-13.4302875533468,
115.160656417445)) ;
#163600=CARTESIAN_POINT('Ctrl Pts',(-16.6522344647069,-13.4290941380284,
115.232763303442)) ;
#163601=CARTESIAN_POINT('Ctrl Pts',(-16.6738872742428,-13.1407025280343,
115.263323344163)) ;
#163602=CARTESIAN_POINT('Ctrl Pts',(-16.6968168802155,-13.1596450179659,
115.333163224222)) ;
#163603=CARTESIAN_POINT('Ctrl Pts',(-16.7706207234299,-13.1596450208018,
115.30893218191)) ;
#163604=CARTESIAN_POINT('Ctrl Pts',(-16.8444245666443,-13.1596450236377,
115.284701139598)) ;
#163605=CARTESIAN_POINT('Ctrl Pts',(-16.8214949606715,-13.1407025337061,
115.214861259539)) ;
#163606=CARTESIAN_POINT('Ctrl Pts',(-16.7985653546987,-13.1217600437745,
115.14502137948)) ;
#163607=CARTESIAN_POINT('Ctrl Pts',(-16.7247615114844,-13.1217600409386,
115.169252421792)) ;
#163608=CARTESIAN_POINT('Ctrl Pts',(-16.65095766827,-13.1217600381026,115.193483464104)) ;
#163609=CARTESIAN_POINT('Ctrl Pts',(-16.6738872742428,-13.1407025280343,
115.263323344163)) ;
#163610=CARTESIAN_POINT('Ctrl Pts',(-16.7192914965339,-12.8707969653127,
115.366034947544)) ;
#163611=CARTESIAN_POINT('Ctrl Pts',(-16.7398209850698,-12.9086154474282,
115.428564457142)) ;
#163612=CARTESIAN_POINT('Ctrl Pts',(-16.8136248279612,-12.9086154501767,
115.404333413846)) ;
#163613=CARTESIAN_POINT('Ctrl Pts',(-16.8874286708526,-12.9086154529253,
115.38010237055)) ;
#163614=CARTESIAN_POINT('Ctrl Pts',(-16.8668991823167,-12.8707969708098,
115.317572860953)) ;
#163615=CARTESIAN_POINT('Ctrl Pts',(-16.8463696937809,-12.8329784886943,
115.255043351355)) ;
#163616=CARTESIAN_POINT('Ctrl Pts',(-16.7725658508895,-12.8329784859458,
115.279274394651)) ;
#163617=CARTESIAN_POINT('Ctrl Pts',(-16.698762007998,-12.8329784831972,
115.303505437946)) ;
#163618=CARTESIAN_POINT('Ctrl Pts',(-16.7192914965339,-12.8707969653127,
115.366034947544)) ;
#163619=CARTESIAN_POINT('Ctrl Pts',(-16.7852951087572,-12.6417711077458,
115.53174600974)) ;
#163620=CARTESIAN_POINT('Ctrl Pts',(-16.8019769392628,-12.6956372286185,
115.582556173826)) ;
#163621=CARTESIAN_POINT('Ctrl Pts',(-16.8757807822629,-12.6956372295276,
115.558325130861)) ;
#163622=CARTESIAN_POINT('Ctrl Pts',(-16.9495846252629,-12.6956372304368,
115.534094087896)) ;
#163623=CARTESIAN_POINT('Ctrl Pts',(-16.9329027947574,-12.6417711095641,
115.48328392381)) ;
#163624=CARTESIAN_POINT('Ctrl Pts',(-16.9162209642519,-12.5879049886915,
115.432473759724)) ;
#163625=CARTESIAN_POINT('Ctrl Pts',(-16.8424171212518,-12.5879049877823,
115.456704802689)) ;
#163626=CARTESIAN_POINT('Ctrl Pts',(-16.7686132782517,-12.5879049868731,
115.480935845654)) ;
#163627=CARTESIAN_POINT('Ctrl Pts',(-16.7852951087572,-12.6417711077458,
115.53174600974)) ;
#163628=CARTESIAN_POINT('Ctrl Pts',(-16.8687385029215,-12.4670674817275,
115.750354845925)) ;
#163629=CARTESIAN_POINT('Ctrl Pts',(-16.8803538371374,-12.5332118470618,
115.785733279865)) ;
#163630=CARTESIAN_POINT('Ctrl Pts',(-16.9541576811356,-12.5332118456008,
115.761502239941)) ;
#163631=CARTESIAN_POINT('Ctrl Pts',(-17.0279615251339,-12.5332118441398,
115.737271200016)) ;
#163632=CARTESIAN_POINT('Ctrl Pts',(-17.016346190918,-12.4670674788054,
115.701892766076)) ;
#163633=CARTESIAN_POINT('Ctrl Pts',(-17.0047308567021,-12.4009231134711,
115.666514332135)) ;
#163634=CARTESIAN_POINT('Ctrl Pts',(-16.9309270127038,-12.4009231149321,
115.69074537206)) ;
#163635=CARTESIAN_POINT('Ctrl Pts',(-16.8571231687056,-12.4009231163931,
115.714976411984)) ;
#163636=CARTESIAN_POINT('Ctrl Pts',(-16.8687385029215,-12.4670674817275,
115.750354845925)) ;
#163637=CARTESIAN_POINT('Ctrl Pts',(-16.9635606886986,-12.3610581795072,
116.003803286491)) ;
#163638=CARTESIAN_POINT('Ctrl Pts',(-16.9693038547935,-12.434700867629,
116.021296043894)) ;
#163639=CARTESIAN_POINT('Ctrl Pts',(-17.0431077002693,-12.4347008654183,
115.997065008469)) ;
#163640=CARTESIAN_POINT('Ctrl Pts',(-17.116911545745,-12.4347008632077,
115.972833973045)) ;
#163641=CARTESIAN_POINT('Ctrl Pts',(-17.11116837965,-12.3610581750859,115.955341215642)) ;
#163642=CARTESIAN_POINT('Ctrl Pts',(-17.1054252135551,-12.2874154869641,
115.937848458239)) ;
#163643=CARTESIAN_POINT('Ctrl Pts',(-17.0316213680793,-12.2874154891748,
115.962079493663)) ;
#163644=CARTESIAN_POINT('Ctrl Pts',(-16.9578175226036,-12.2874154913854,
115.986310529088)) ;
#163645=CARTESIAN_POINT('Ctrl Pts',(-16.9635606886986,-12.3610581795072,
116.003803286491)) ;
#163646=CARTESIAN_POINT('Ctrl Pts',(-17.0649420670116,-12.3304705905987,
116.27693713892)) ;
#163647=CARTESIAN_POINT('Ctrl Pts',(-17.0643525739706,-12.4063567534876,
116.275141638518)) ;
#163648=CARTESIAN_POINT('Ctrl Pts',(-17.138156421995,-12.4063567532817,
116.250910610856)) ;
#163649=CARTESIAN_POINT('Ctrl Pts',(-17.2119602700193,-12.4063567530759,
116.226679583194)) ;
#163650=CARTESIAN_POINT('Ctrl Pts',(-17.2125497630602,-12.330470590187,
116.228475083596)) ;
#163651=CARTESIAN_POINT('Ctrl Pts',(-17.2131392561011,-12.2545844272981,
116.230270583998)) ;
#163652=CARTESIAN_POINT('Ctrl Pts',(-17.1393354080768,-12.254584427504,
116.25450161166)) ;
#163653=CARTESIAN_POINT('Ctrl Pts',(-17.0655315600525,-12.2545844277098,
116.278732639322)) ;
#163654=CARTESIAN_POINT('Ctrl Pts',(-17.0649420670116,-12.3304705905987,
116.27693713892)) ;
#163655=CARTESIAN_POINT('Ctrl Pts',(-17.1648109896159,-12.3780041179342,
116.545751053977)) ;
#163656=CARTESIAN_POINT('Ctrl Pts',(-17.1579795166612,-12.4506811357788,
116.524943490027)) ;
#163657=CARTESIAN_POINT('Ctrl Pts',(-17.2317833665539,-12.4506811414498,
116.500712468056)) ;
#163658=CARTESIAN_POINT('Ctrl Pts',(-17.3055872164466,-12.4506811471207,
116.476481446085)) ;
#163659=CARTESIAN_POINT('Ctrl Pts',(-17.3124186894012,-12.3780041292761,
116.497289010035)) ;
#163660=CARTESIAN_POINT('Ctrl Pts',(-17.3192501623558,-12.3053271114316,
116.518096573985)) ;
#163661=CARTESIAN_POINT('Ctrl Pts',(-17.2454463124632,-12.3053271057606,
116.542327595956)) ;
#163662=CARTESIAN_POINT('Ctrl Pts',(-17.1716424625705,-12.3053271000897,
116.566558617927)) ;
#163663=CARTESIAN_POINT('Ctrl Pts',(-17.1648109896159,-12.3780041179342,
116.545751053977)) ;
#163664=CARTESIAN_POINT('Ctrl Pts',(-17.2579372276331,-12.5002675543906,
116.79387021803)) ;
#163665=CARTESIAN_POINT('Ctrl Pts',(-17.2453288035709,-12.5645133223993,
116.755466993281)) ;
#163666=CARTESIAN_POINT('Ctrl Pts',(-17.3191326550243,-12.5645133380227,
116.731235976064)) ;
#163667=CARTESIAN_POINT('Ctrl Pts',(-17.3929365064777,-12.5645133536461,
116.707004958847)) ;
#163668=CARTESIAN_POINT('Ctrl Pts',(-17.40554493054,-12.5002675856374,116.745408183595)) ;
#163669=CARTESIAN_POINT('Ctrl Pts',(-17.4181533546022,-12.4360218176287,
116.783811408344)) ;
#163670=CARTESIAN_POINT('Ctrl Pts',(-17.3443495031488,-12.4360218020053,
116.808042425561)) ;
#163671=CARTESIAN_POINT('Ctrl Pts',(-17.2705456516954,-12.4360217863819,
116.832273442779)) ;
#163672=CARTESIAN_POINT('Ctrl Pts',(-17.2579372276331,-12.5002675543906,
116.79387021803)) ;
#163673=CARTESIAN_POINT('Ctrl Pts',(-17.3375779201861,-12.6872113223539,
117.001122929289)) ;
#163674=CARTESIAN_POINT('Ctrl Pts',(-17.3201216848697,-12.7384971666027,
116.947954053789)) ;
#163675=CARTESIAN_POINT('Ctrl Pts',(-17.3939255362724,-12.7384971937162,
116.923723036417)) ;
#163676=CARTESIAN_POINT('Ctrl Pts',(-17.4677293876751,-12.7384972208297,
116.899492019045)) ;
#163677=CARTESIAN_POINT('Ctrl Pts',(-17.4851856229915,-12.6872113765809,
116.952660894545)) ;
#163678=CARTESIAN_POINT('Ctrl Pts',(-17.5026418583079,-12.635925532332,
117.005829770045)) ;
#163679=CARTESIAN_POINT('Ctrl Pts',(-17.4288380069052,-12.6359255052185,
117.030060787417)) ;
#163680=CARTESIAN_POINT('Ctrl Pts',(-17.3550341555026,-12.635925478105,
117.054291804789)) ;
#163681=CARTESIAN_POINT('Ctrl Pts',(-17.3375779201861,-12.6872113223539,
117.001122929289)) ;
#163682=CARTESIAN_POINT('Ctrl Pts',(-17.3998316457169,-12.928470822573,
117.155087519117)) ;
#163683=CARTESIAN_POINT('Ctrl Pts',(-17.3787411946458,-12.9629864518457,
117.09084940901)) ;
#163684=CARTESIAN_POINT('Ctrl Pts',(-17.4525450450027,-12.9629864941427,
117.066618388453)) ;
#163685=CARTESIAN_POINT('Ctrl Pts',(-17.5263488953595,-12.9629865364398,
117.042387367896)) ;
#163686=CARTESIAN_POINT('Ctrl Pts',(-17.5474393464306,-12.9284709071671,
117.106625478002)) ;
#163687=CARTESIAN_POINT('Ctrl Pts',(-17.5685297975017,-12.8939552778944,
117.170863588109)) ;
#163688=CARTESIAN_POINT('Ctrl Pts',(-17.4947259471448,-12.8939552355973,
117.195094608666)) ;
#163689=CARTESIAN_POINT('Ctrl Pts',(-17.420922096788,-12.8939551933003,
117.219325629224)) ;
#163690=CARTESIAN_POINT('Ctrl Pts',(-17.3998316457169,-12.928470822573,
117.155087519117)) ;
#163691=CARTESIAN_POINT('Ctrl Pts',(-17.4399174994754,-13.2034657060163,
117.241757837914)) ;
#163692=CARTESIAN_POINT('Ctrl Pts',(-17.416730872886,-13.2188313176784,
117.171135115555)) ;
#163693=CARTESIAN_POINT('Ctrl Pts',(-17.4905347199573,-13.2188313725587,
117.146904084991)) ;
#163694=CARTESIAN_POINT('Ctrl Pts',(-17.5643385670287,-13.218831427439,
117.122673054427)) ;
#163695=CARTESIAN_POINT('Ctrl Pts',(-17.5875251936181,-13.2034658157769,
117.193295776785)) ;
#163696=CARTESIAN_POINT('Ctrl Pts',(-17.6107118202076,-13.1881002041148,
117.263918499144)) ;
#163697=CARTESIAN_POINT('Ctrl Pts',(-17.5369079731363,-13.1881001492345,
117.288149529709)) ;
#163698=CARTESIAN_POINT('Ctrl Pts',(-17.4631041260649,-13.1881000943542,
117.312380560273)) ;
#163699=CARTESIAN_POINT('Ctrl Pts',(-17.4399174994754,-13.2034657060163,
117.241757837914)) ;
#163700=CARTESIAN_POINT('Ctrl Pts',(-17.4562690855038,-13.4939400108665,
117.256107218264)) ;
#163701=CARTESIAN_POINT('Ctrl Pts',(-17.4326409399332,-13.4890474543543,
117.184139700489)) ;
#163702=CARTESIAN_POINT('Ctrl Pts',(-17.5064447821528,-13.4890475187126,
117.159908655147)) ;
#163703=CARTESIAN_POINT('Ctrl Pts',(-17.5802486243724,-13.4890475830709,
117.135677609805)) ;
#163704=CARTESIAN_POINT('Ctrl Pts',(-17.603876769943,-13.4939401395831,
117.20764512758)) ;
#163705=CARTESIAN_POINT('Ctrl Pts',(-17.6275049155135,-13.4988326960953,
117.279612645354)) ;
#163706=CARTESIAN_POINT('Ctrl Pts',(-17.553701073294,-13.498832631737,117.303843690697)) ;
#163707=CARTESIAN_POINT('Ctrl Pts',(-17.4798972310744,-13.4988325673787,
117.328074736039)) ;
#163708=CARTESIAN_POINT('Ctrl Pts',(-17.4562690855038,-13.4939400108665,
117.256107218264)) ;
#163709=CARTESIAN_POINT('Ctrl Pts',(-17.4483972852435,-13.7785749983251,
117.196730556268)) ;
#163710=CARTESIAN_POINT('Ctrl Pts',(-17.4260170952016,-13.7538028114636,
117.128564109822)) ;
#163711=CARTESIAN_POINT('Ctrl Pts',(-17.4998209313486,-13.7538028795782,
117.104333045984)) ;
#163712=CARTESIAN_POINT('Ctrl Pts',(-17.5736247674956,-13.7538029476928,
117.080101982146)) ;
#163713=CARTESIAN_POINT('Ctrl Pts',(-17.5960049575374,-13.7785751345543,
117.148268428592)) ;
#163714=CARTESIAN_POINT('Ctrl Pts',(-17.6183851475792,-13.8033473214157,
117.216434875038)) ;
#163715=CARTESIAN_POINT('Ctrl Pts',(-17.5445813114322,-13.8033472533012,
117.240665938876)) ;
#163716=CARTESIAN_POINT('Ctrl Pts',(-17.4707774752853,-13.8033471851866,
117.264897002714)) ;
#163717=CARTESIAN_POINT('Ctrl Pts',(-17.4483972852435,-13.7785749983251,
117.196730556268)) ;
#163718=CARTESIAN_POINT('Ctrl Pts',(-17.4176717828043,-14.0376123935157,
117.067726587636)) ;
#163719=CARTESIAN_POINT('Ctrl Pts',(-17.398137247503,-13.9947190826741,
117.008227546524)) ;
#163720=CARTESIAN_POINT('Ctrl Pts',(-17.4719410769957,-13.9947191481114,
116.983996462419)) ;
#163721=CARTESIAN_POINT('Ctrl Pts',(-17.5457449064884,-13.9947192135486,
116.959765378313)) ;
#163722=CARTESIAN_POINT('Ctrl Pts',(-17.5652794417897,-14.0376125243903,
117.019264419424)) ;
#163723=CARTESIAN_POINT('Ctrl Pts',(-17.584813977091,-14.0805058352319,
117.078763460535)) ;
#163724=CARTESIAN_POINT('Ctrl Pts',(-17.5110101475983,-14.0805057697947,
117.102994544641)) ;
#163725=CARTESIAN_POINT('Ctrl Pts',(-17.4372063181056,-14.0805057043574,
117.127225628747)) ;
#163726=CARTESIAN_POINT('Ctrl Pts',(-17.4176717828043,-14.0376123935157,
117.067726587636)) ;
#163727=CARTESIAN_POINT('Ctrl Pts',(-17.3669381628985,-14.2526152270872,
116.877737714805)) ;
#163728=CARTESIAN_POINT('Ctrl Pts',(-17.3516510972301,-14.1946488297789,
116.831175781003)) ;
#163729=CARTESIAN_POINT('Ctrl Pts',(-17.4254549201375,-14.1946488854693,
116.80694467684)) ;
#163730=CARTESIAN_POINT('Ctrl Pts',(-17.499258743045,-14.1946489411597,
116.782713572676)) ;
#163731=CARTESIAN_POINT('Ctrl Pts',(-17.5145458087134,-14.252615338468,
116.829275506478)) ;
#163732=CARTESIAN_POINT('Ctrl Pts',(-17.5298328743817,-14.3105817357762,
116.87583744028)) ;
#163733=CARTESIAN_POINT('Ctrl Pts',(-17.4560290514743,-14.3105816800858,
116.900068544444)) ;
#163734=CARTESIAN_POINT('Ctrl Pts',(-17.3822252285668,-14.3105816243954,
116.924299648607)) ;
#163735=CARTESIAN_POINT('Ctrl Pts',(-17.3669381628985,-14.2526152270872,
116.877737714805)) ;
#163736=CARTESIAN_POINT('Ctrl Pts',(-17.300521743148,-14.4080507138092,
116.639938676009)) ;
#163737=CARTESIAN_POINT('Ctrl Pts',(-17.2905840086684,-14.3391479238767,
116.609669942021)) ;
#163738=CARTESIAN_POINT('Ctrl Pts',(-17.3643878258509,-14.3391479627699,
116.585438820421)) ;
#163739=CARTESIAN_POINT('Ctrl Pts',(-17.4381916430334,-14.3391480016631,
116.56120769882)) ;
#163740=CARTESIAN_POINT('Ctrl Pts',(-17.448129377513,-14.4080507915956,
116.591476432807)) ;
#163741=CARTESIAN_POINT('Ctrl Pts',(-17.4580671119925,-14.4769535815281,
116.621745166794)) ;
#163742=CARTESIAN_POINT('Ctrl Pts',(-17.38426329481,-14.4769535426349,116.645976288395)) ;
#163743=CARTESIAN_POINT('Ctrl Pts',(-17.3104594776275,-14.4769535037417,
116.670207409996)) ;
#163744=CARTESIAN_POINT('Ctrl Pts',(-17.300521743148,-14.4080507138092,
116.639938676009)) ;
#163745=CARTESIAN_POINT('Ctrl Pts',(-17.2239015581171,-14.4922598223547,
116.371021974036)) ;
#163746=CARTESIAN_POINT('Ctrl Pts',(-17.2200340718307,-14.4173770699575,
116.359242236723)) ;
#163747=CARTESIAN_POINT('Ctrl Pts',(-17.2938378850058,-14.4173770858156,
116.335011102916)) ;
#163748=CARTESIAN_POINT('Ctrl Pts',(-17.367641698181,-14.4173771016737,
116.31077996911)) ;
#163749=CARTESIAN_POINT('Ctrl Pts',(-17.3715091844673,-14.4922598540709,
116.322559706423)) ;
#163750=CARTESIAN_POINT('Ctrl Pts',(-17.3753766707537,-14.5671426064681,
116.334339443736)) ;
#163751=CARTESIAN_POINT('Ctrl Pts',(-17.3015728575786,-14.56714259061,116.358570577543)) ;
#163752=CARTESIAN_POINT('Ctrl Pts',(-17.2277690444035,-14.5671425747519,
116.38280171135)) ;
#163753=CARTESIAN_POINT('Ctrl Pts',(-17.2239015581171,-14.4922598223547,
116.371021974036)) ;
#163754=CARTESIAN_POINT('Ctrl Pts',(-17.1439517410193,-14.4995566650645,
116.092195902509)) ;
#163755=CARTESIAN_POINT('Ctrl Pts',(-17.1463910960368,-14.4240553765711,
116.099625786271)) ;
#163756=CARTESIAN_POINT('Ctrl Pts',(-17.2201949078783,-14.4240553658153,
116.075394648402)) ;
#163757=CARTESIAN_POINT('Ctrl Pts',(-17.2939987197198,-14.4240553550595,
116.051163510533)) ;
#163758=CARTESIAN_POINT('Ctrl Pts',(-17.2915593647023,-14.4995566435528,
116.043733626772)) ;
#163759=CARTESIAN_POINT('Ctrl Pts',(-17.2891200096848,-14.5750579320462,
116.03630374301)) ;
#163760=CARTESIAN_POINT('Ctrl Pts',(-17.2153161978433,-14.575057942802,
116.060534880879)) ;
#163761=CARTESIAN_POINT('Ctrl Pts',(-17.1415123860018,-14.5750579535578,
116.084766018747)) ;
#163762=CARTESIAN_POINT('Ctrl Pts',(-17.1439517410193,-14.4995566650645,
116.092195902509)) ;
#163763=CARTESIAN_POINT('Ctrl Pts',(-17.0659766810491,-14.4291954268347,
115.819082015723)) ;
#163764=CARTESIAN_POINT('Ctrl Pts',(-17.0746003967584,-14.3584951723125,
115.845348464383)) ;
#163765=CARTESIAN_POINT('Ctrl Pts',(-17.1484042095327,-14.3584951335383,
115.821117329355)) ;
#163766=CARTESIAN_POINT('Ctrl Pts',(-17.2222080223069,-14.358495094764,
115.796886194328)) ;
#163767=CARTESIAN_POINT('Ctrl Pts',(-17.2135843065975,-14.4291953492863,
115.770619745668)) ;
#163768=CARTESIAN_POINT('Ctrl Pts',(-17.2049605908881,-14.4998956038086,
115.744353297008)) ;
#163769=CARTESIAN_POINT('Ctrl Pts',(-17.1311567781139,-14.4998956425828,
115.768584432035)) ;
#163770=CARTESIAN_POINT('Ctrl Pts',(-17.0573529653397,-14.499895681357,
115.792815567063)) ;
#163771=CARTESIAN_POINT('Ctrl Pts',(-17.0659766810491,-14.4291954268347,
115.819082015723)) ;
#163772=CARTESIAN_POINT('Ctrl Pts',(-16.9973489861747,-14.2862746553945,
115.574590132372)) ;
#163773=CARTESIAN_POINT('Ctrl Pts',(-17.0115105195248,-14.2254484542933,
115.617723880079)) ;
#163774=CARTESIAN_POINT('Ctrl Pts',(-17.0853143361643,-14.2254483895805,
115.593492756825)) ;
#163775=CARTESIAN_POINT('Ctrl Pts',(-17.1591181528039,-14.2254483248678,
115.56926163357)) ;
#163776=CARTESIAN_POINT('Ctrl Pts',(-17.1449566194538,-14.286274525969,
115.526127885863)) ;
#163777=CARTESIAN_POINT('Ctrl Pts',(-17.1307950861037,-14.3471007270702,
115.482994138157)) ;
#163778=CARTESIAN_POINT('Ctrl Pts',(-17.0569912694642,-14.347100791783,
115.507225261411)) ;
#163779=CARTESIAN_POINT('Ctrl Pts',(-16.9831874528246,-14.3471008564957,
115.531456384666)) ;
#163780=CARTESIAN_POINT('Ctrl Pts',(-16.9973489861747,-14.2862746553945,
115.574590132372)) ;
#163781=CARTESIAN_POINT('Ctrl Pts',(-16.943507599311,-14.0821782924177,
115.375260361907)) ;
#163782=CARTESIAN_POINT('Ctrl Pts',(-16.9621801863693,-14.0355118999346,
115.432134051369)) ;
#163783=CARTESIAN_POINT('Ctrl Pts',(-17.0359840091523,-14.0355118141507,
115.407902946826)) ;
#163784=CARTESIAN_POINT('Ctrl Pts',(-17.1097878319353,-14.0355117283667,
115.383671842284)) ;
#163785=CARTESIAN_POINT('Ctrl Pts',(-17.091115244877,-14.0821781208498,
115.326798152822)) ;
#163786=CARTESIAN_POINT('Ctrl Pts',(-17.0724426578187,-14.1288445133328,
115.26992446336)) ;
#163787=CARTESIAN_POINT('Ctrl Pts',(-16.9986388350357,-14.1288445991168,
115.294155567902)) ;
#163788=CARTESIAN_POINT('Ctrl Pts',(-16.9248350122527,-14.1288446849008,
115.318386672445)) ;
#163789=CARTESIAN_POINT('Ctrl Pts',(-16.943507599311,-14.0821782924177,
115.375260361907)) ;
#163790=CARTESIAN_POINT('Ctrl Pts',(-16.9086511894243,-13.8298750263426,
115.233624849604)) ;
#163791=CARTESIAN_POINT('Ctrl Pts',(-16.9305188675121,-13.8007543288235,
115.300230270815)) ;
#163792=CARTESIAN_POINT('Ctrl Pts',(-17.0043226981659,-13.8007542285384,
115.275999190246)) ;
#163793=CARTESIAN_POINT('Ctrl Pts',(-17.0781265288196,-13.8007541282534,
115.251768109676)) ;
#163794=CARTESIAN_POINT('Ctrl Pts',(-17.0562588507318,-13.8298748257726,
115.185162688465)) ;
#163795=CARTESIAN_POINT('Ctrl Pts',(-17.0343911726441,-13.8589955232917,
115.118557267253)) ;
#163796=CARTESIAN_POINT('Ctrl Pts',(-16.9605873419903,-13.8589956235767,
115.142788347823)) ;
#163797=CARTESIAN_POINT('Ctrl Pts',(-16.8867835113365,-13.8589957238618,
115.167019428392)) ;
#163798=CARTESIAN_POINT('Ctrl Pts',(-16.9086511894243,-13.8298750263426,
115.233624849604)) ;
#163799=CARTESIAN_POINT('Ctrl Pts',(-16.8963479197035,-13.5470860719876,
115.160572447035)) ;
#163800=CARTESIAN_POINT('Ctrl Pts',(-16.9198433509072,-13.5376651784076,
115.232135741571)) ;
#163801=CARTESIAN_POINT('Ctrl Pts',(-16.993647190433,-13.5376650723535,
115.207904688025)) ;
#163802=CARTESIAN_POINT('Ctrl Pts',(-17.0674510299589,-13.5376649662995,
115.183673634478)) ;
#163803=CARTESIAN_POINT('Ctrl Pts',(-17.0439555987552,-13.5470858598794,
115.112110339942)) ;
#163804=CARTESIAN_POINT('Ctrl Pts',(-17.0204601675516,-13.5565067534594,
115.040547045406)) ;
#163805=CARTESIAN_POINT('Ctrl Pts',(-16.9466563280257,-13.5565068595135,
115.064778098952)) ;
#163806=CARTESIAN_POINT('Ctrl Pts',(-16.8728524884998,-13.5565069655676,
115.089009152499)) ;
#163807=CARTESIAN_POINT('Ctrl Pts',(-16.8963479197035,-13.5470860719876,
115.160572447035)) ;
#163808=CARTESIAN_POINT('Ctrl Pts',(-16.90824578111,-13.2560613841224,115.161364252542)) ;
#163809=CARTESIAN_POINT('Ctrl Pts',(-16.9316790297655,-13.2669448864172,
115.232738149021)) ;
#163810=CARTESIAN_POINT('Ctrl Pts',(-17.0054828781172,-13.266944783336,
115.208507122357)) ;
#163811=CARTESIAN_POINT('Ctrl Pts',(-17.0792867264688,-13.2669446802549,
115.184276095692)) ;
#163812=CARTESIAN_POINT('Ctrl Pts',(-17.0558534778133,-13.2560611779601,
115.112902199213)) ;
#163813=CARTESIAN_POINT('Ctrl Pts',(-17.0324202291578,-13.2451776756653,
115.041528302733)) ;
#163814=CARTESIAN_POINT('Ctrl Pts',(-16.9586163808062,-13.2451777787465,
115.065759329398)) ;
#163815=CARTESIAN_POINT('Ctrl Pts',(-16.8848125324545,-13.2451778818276,
115.089990356062)) ;
#163816=CARTESIAN_POINT('Ctrl Pts',(-16.90824578111,-13.2560613841224,115.161364252542)) ;
#163817=CARTESIAN_POINT('Ctrl Pts',(-16.9442254493305,-12.9762949722028,
115.235455446136)) ;
#163818=CARTESIAN_POINT('Ctrl Pts',(-16.9659162848826,-13.0067272528639,
115.301522233367)) ;
#163819=CARTESIAN_POINT('Ctrl Pts',(-17.0397201411344,-13.0067271611354,
115.277291230766)) ;
#163820=CARTESIAN_POINT('Ctrl Pts',(-17.1135239973862,-13.0067270694068,
115.253060228164)) ;
#163821=CARTESIAN_POINT('Ctrl Pts',(-17.0918331618342,-12.9762947887458,
115.186993440932)) ;
#163822=CARTESIAN_POINT('Ctrl Pts',(-17.0701423262821,-12.9458625080848,
115.120926653701)) ;
#163823=CARTESIAN_POINT('Ctrl Pts',(-16.9963384700303,-12.9458625998133,
115.145157656303)) ;
#163824=CARTESIAN_POINT('Ctrl Pts',(-16.9225346137784,-12.9458626915418,
115.169388658905)) ;
#163825=CARTESIAN_POINT('Ctrl Pts',(-16.9442254493305,-12.9762949722028,
115.235455446136)) ;
#163826=CARTESIAN_POINT('Ctrl Pts',(-17.0022072372073,-12.729021213087,
115.376690040029)) ;
#163827=CARTESIAN_POINT('Ctrl Pts',(-17.0206142060272,-12.7767631435002,
115.432754698965)) ;
#163828=CARTESIAN_POINT('Ctrl Pts',(-17.0944180685995,-12.7767630691524,
115.408523715614)) ;
#163829=CARTESIAN_POINT('Ctrl Pts',(-17.1682219311719,-12.7767629948046,
115.384292732264)) ;
#163830=CARTESIAN_POINT('Ctrl Pts',(-17.1498149623519,-12.7290210643915,
115.328228073327)) ;
#163831=CARTESIAN_POINT('Ctrl Pts',(-17.131407993532,-12.6812791339783,
115.272163414391)) ;
#163832=CARTESIAN_POINT('Ctrl Pts',(-17.0576041309596,-12.6812792083261,
115.296394397742)) ;
#163833=CARTESIAN_POINT('Ctrl Pts',(-16.9838002683873,-12.6812792826738,
115.320625381093)) ;
#163834=CARTESIAN_POINT('Ctrl Pts',(-17.0022072372073,-12.729021213087,
115.376690040029)) ;
#163835=CARTESIAN_POINT('Ctrl Pts',(-17.0792272362676,-12.5300504685621,
115.575764889513)) ;
#163836=CARTESIAN_POINT('Ctrl Pts',(-17.0930194529222,-12.5917559666324,
115.617773757829)) ;
#163837=CARTESIAN_POINT('Ctrl Pts',(-17.1668233195247,-12.5917559147477,
115.593542786754)) ;
#163838=CARTESIAN_POINT('Ctrl Pts',(-17.2406271861272,-12.5917558628629,
115.569311815679)) ;
#163839=CARTESIAN_POINT('Ctrl Pts',(-17.2268349694727,-12.5300503647925,
115.527302947363)) ;
#163840=CARTESIAN_POINT('Ctrl Pts',(-17.2130427528181,-12.4683448667222,
115.485294079046)) ;
#163841=CARTESIAN_POINT('Ctrl Pts',(-17.1392388862155,-12.468344918607,
115.509525050122)) ;
#163842=CARTESIAN_POINT('Ctrl Pts',(-17.065435019613,-12.4683449704918,
115.533756021197)) ;
#163843=CARTESIAN_POINT('Ctrl Pts',(-17.0792272362676,-12.5300504685621,
115.575764889513)) ;
#163844=CARTESIAN_POINT('Ctrl Pts',(-17.1704529515286,-12.3949013412461,
115.818078836631)) ;
#163845=CARTESIAN_POINT('Ctrl Pts',(-17.1786322750179,-12.4661360013531,
115.842991737866)) ;
#163846=CARTESIAN_POINT('Ctrl Pts',(-17.2524361430164,-12.4661359735393,
115.818760771042)) ;
#163847=CARTESIAN_POINT('Ctrl Pts',(-17.3262400110149,-12.4661359457255,
115.794529804219)) ;
#163848=CARTESIAN_POINT('Ctrl Pts',(-17.3180606875257,-12.3949012856185,
115.769616902984)) ;
#163849=CARTESIAN_POINT('Ctrl Pts',(-17.3098813640364,-12.3236666255115,
115.744704001749)) ;
#163850=CARTESIAN_POINT('Ctrl Pts',(-17.2360774960379,-12.3236666533253,
115.768934968573)) ;
#163851=CARTESIAN_POINT('Ctrl Pts',(-17.1622736280394,-12.3236666811392,
115.793165935396)) ;
#163852=CARTESIAN_POINT('Ctrl Pts',(-17.1704529515286,-12.3949013412461,
115.818078836631)) ;
#163853=CARTESIAN_POINT('Ctrl Pts',(-17.2696316491355,-12.3334783627152,
116.084736767084)) ;
#163854=CARTESIAN_POINT('Ctrl Pts',(-17.2716317461079,-12.4091090544744,
116.090828741229)) ;
#163855=CARTESIAN_POINT('Ctrl Pts',(-17.3454356133753,-12.4091090490569,
116.066597772179)) ;
#163856=CARTESIAN_POINT('Ctrl Pts',(-17.4192394806428,-12.4091090436395,
116.042366803129)) ;
#163857=CARTESIAN_POINT('Ctrl Pts',(-17.4172393836704,-12.3334783518803,
116.036274828984)) ;
#163858=CARTESIAN_POINT('Ctrl Pts',(-17.415239286698,-12.2578476601211,
116.030182854838)) ;
#163859=CARTESIAN_POINT('Ctrl Pts',(-17.3414354194305,-12.2578476655386,
116.054413823888)) ;
#163860=CARTESIAN_POINT('Ctrl Pts',(-17.2676315521631,-12.257847670956,
116.078644792938)) ;
#163861=CARTESIAN_POINT('Ctrl Pts',(-17.2696316491355,-12.3334783627152,
116.084736767084)) ;
#163862=CARTESIAN_POINT('Ctrl Pts',(-17.3706199437548,-12.3494129205617,
116.356939612366)) ;
#163863=CARTESIAN_POINT('Ctrl Pts',(-17.3663044203247,-12.4240452801496,
116.343795225649)) ;
#163864=CARTESIAN_POINT('Ctrl Pts',(-17.4401082850067,-12.4240452938977,
116.319564248724)) ;
#163865=CARTESIAN_POINT('Ctrl Pts',(-17.5139121496887,-12.4240453076458,
116.295333271799)) ;
#163866=CARTESIAN_POINT('Ctrl Pts',(-17.5182276731188,-12.3494129480579,
116.308477658515)) ;
#163867=CARTESIAN_POINT('Ctrl Pts',(-17.5225431965489,-12.27478058847,116.321622045232)) ;
#163868=CARTESIAN_POINT('Ctrl Pts',(-17.4487393318669,-12.2747805747219,
116.345853022157)) ;
#163869=CARTESIAN_POINT('Ctrl Pts',(-17.3749354671849,-12.2747805609737,
116.370083999082)) ;
#163870=CARTESIAN_POINT('Ctrl Pts',(-17.3706199437548,-12.3494129205617,
116.356939612366)) ;
#163871=CARTESIAN_POINT('Ctrl Pts',(-17.4673694639669,-12.4418688951199,
116.61612522571)) ;
#163872=CARTESIAN_POINT('Ctrl Pts',(-17.4570268792605,-12.5101591784945,
116.584623382643)) ;
#163873=CARTESIAN_POINT('Ctrl Pts',(-17.5308307396141,-12.5101592062549,
116.560392392534)) ;
#163874=CARTESIAN_POINT('Ctrl Pts',(-17.6046345999678,-12.5101592340153,
116.536161402426)) ;
#163875=CARTESIAN_POINT('Ctrl Pts',(-17.6149771846741,-12.4418689506407,
116.567663245492)) ;
#163876=CARTESIAN_POINT('Ctrl Pts',(-17.6253197693805,-12.373578667266,
116.599165088559)) ;
#163877=CARTESIAN_POINT('Ctrl Pts',(-17.5515159090268,-12.3735786395056,
116.623396078668)) ;
#163878=CARTESIAN_POINT('Ctrl Pts',(-17.4777120486732,-12.3735786117452,
116.647627068776)) ;
#163879=CARTESIAN_POINT('Ctrl Pts',(-17.4673694639669,-12.4418688951199,
116.61612522571)) ;
#163880=CARTESIAN_POINT('Ctrl Pts',(-17.5535183531139,-12.6051421932678,
116.842927305494)) ;
#163881=CARTESIAN_POINT('Ctrl Pts',(-17.5378815244524,-12.6621364558016,
116.795300049372)) ;
#163882=CARTESIAN_POINT('Ctrl Pts',(-17.6116853796284,-12.6621364903346,
116.771069043494)) ;
#163883=CARTESIAN_POINT('Ctrl Pts',(-17.6854892348045,-12.6621365248676,
116.746838037615)) ;
#163884=CARTESIAN_POINT('Ctrl Pts',(-17.701126063466,-12.6051422623338,
116.794465293737)) ;
#163885=CARTESIAN_POINT('Ctrl Pts',(-17.7167628921274,-12.5481479998,116.842092549858)) ;
#163886=CARTESIAN_POINT('Ctrl Pts',(-17.6429590369514,-12.548147965267,
116.866323555737)) ;
#163887=CARTESIAN_POINT('Ctrl Pts',(-17.5691551817754,-12.548147930734,
116.890554561616)) ;
#163888=CARTESIAN_POINT('Ctrl Pts',(-17.5535183531139,-12.6051421932678,
116.842927305494)) ;
#163889=CARTESIAN_POINT('Ctrl Pts',(-17.6228267175663,-12.824581983231,
117.018781891196)) ;
#163890=CARTESIAN_POINT('Ctrl Pts',(-17.6030564632207,-12.866340572483,
116.958564887239)) ;
#163891=CARTESIAN_POINT('Ctrl Pts',(-17.6768603140324,-12.8663406101773,
116.934333868067)) ;
#163892=CARTESIAN_POINT('Ctrl Pts',(-17.7506641648441,-12.8663406478716,
116.910102848895)) ;
#163893=CARTESIAN_POINT('Ctrl Pts',(-17.7704344191897,-12.8245820586196,
116.970319852852)) ;
#163894=CARTESIAN_POINT('Ctrl Pts',(-17.7902046735353,-12.7828234693676,
117.030536856809)) ;
#163895=CARTESIAN_POINT('Ctrl Pts',(-17.7164008227236,-12.7828234316733,
117.054767875981)) ;
#163896=CARTESIAN_POINT('Ctrl Pts',(-17.6425969719119,-12.782823393979,
117.078998895153)) ;
#163897=CARTESIAN_POINT('Ctrl Pts',(-17.6228267175663,-12.824581983231,
117.018781891196)) ;
#163898=CARTESIAN_POINT('Ctrl Pts',(-17.6723197045104,-13.0878606072953,
117.134031445032)) ;
#163899=CARTESIAN_POINT('Ctrl Pts',(-17.6497982889685,-13.1112998695193,
117.065434847795)) ;
#163900=CARTESIAN_POINT('Ctrl Pts',(-17.7236021355016,-13.1112999036755,
117.041203815592)) ;
#163901=CARTESIAN_POINT('Ctrl Pts',(-17.7974059820347,-13.1112999378317,
117.016972783388)) ;
#163902=CARTESIAN_POINT('Ctrl Pts',(-17.8199273975766,-13.0878606756077,
117.085569380624)) ;
#163903=CARTESIAN_POINT('Ctrl Pts',(-17.8424488131185,-13.0644214133836,
117.15416597786)) ;
#163904=CARTESIAN_POINT('Ctrl Pts',(-17.7686449665854,-13.0644213792274,
117.178397010064)) ;
#163905=CARTESIAN_POINT('Ctrl Pts',(-17.6948411200522,-13.0644213450712,
117.202628042268)) ;
#163906=CARTESIAN_POINT('Ctrl Pts',(-17.6723197045104,-13.0878606072953,
117.134031445032)) ;
#163907=CARTESIAN_POINT('Ctrl Pts',(-17.6985731634041,-13.3747557627756,
117.178522404017)) ;
#163908=CARTESIAN_POINT('Ctrl Pts',(-17.6749185440874,-13.378198596209,
117.10647425076)) ;
#163909=CARTESIAN_POINT('Ctrl Pts',(-17.7487223875847,-13.3781986232595,
117.082243209309)) ;
#163910=CARTESIAN_POINT('Ctrl Pts',(-17.822526231082,-13.37819865031,117.058012167859)) ;
#163911=CARTESIAN_POINT('Ctrl Pts',(-17.8461808503987,-13.3747558168767,
117.130060321116)) ;
#163912=CARTESIAN_POINT('Ctrl Pts',(-17.8698354697153,-13.3713129834433,
117.202108474372)) ;
#163913=CARTESIAN_POINT('Ctrl Pts',(-17.796031626218,-13.3713129563928,
117.226339515823)) ;
#163914=CARTESIAN_POINT('Ctrl Pts',(-17.7222277827207,-13.3713129293423,
117.250570557273)) ;
#163915=CARTESIAN_POINT('Ctrl Pts',(-17.6985731634041,-13.3747557627756,
117.178522404017)) ;
#163916=CARTESIAN_POINT('Ctrl Pts',(-17.7004702306017,-13.6654070056361,
117.148736694593)) ;
#163917=CARTESIAN_POINT('Ctrl Pts',(-17.6773832073947,-13.648560400251,
117.078417347336)) ;
#163918=CARTESIAN_POINT('Ctrl Pts',(-17.751187049296,-13.6485604179734,
117.054186301025)) ;
#163919=CARTESIAN_POINT('Ctrl Pts',(-17.8249908911973,-13.6485604356957,
117.029955254713)) ;
#163920=CARTESIAN_POINT('Ctrl Pts',(-17.8480779144043,-13.6654070410809,
117.10027460197)) ;
#163921=CARTESIAN_POINT('Ctrl Pts',(-17.8711649376114,-13.682253646466,
117.170593949227)) ;
#163922=CARTESIAN_POINT('Ctrl Pts',(-17.7973610957101,-13.6822536287436,
117.194824995538)) ;
#163923=CARTESIAN_POINT('Ctrl Pts',(-17.7235572538088,-13.6822536110213,
117.21905604185)) ;
#163924=CARTESIAN_POINT('Ctrl Pts',(-17.7004702306017,-13.6654070056361,
117.148736694593)) ;
#163925=CARTESIAN_POINT('Ctrl Pts',(-17.6787592525954,-13.9370542943595,
117.047221465574)) ;
#163926=CARTESIAN_POINT('Ctrl Pts',(-17.6578856782785,-13.901214603103,
116.983643926372)) ;
#163927=CARTESIAN_POINT('Ctrl Pts',(-17.7316895197608,-13.9012146131836,
116.959412878784)) ;
#163928=CARTESIAN_POINT('Ctrl Pts',(-17.8054933612432,-13.9012146232642,
116.935181831197)) ;
#163929=CARTESIAN_POINT('Ctrl Pts',(-17.8263669355601,-13.9370543145207,
116.998759370399)) ;
#163930=CARTESIAN_POINT('Ctrl Pts',(-17.847240509877,-13.9728940057772,
117.062336909601)) ;
#163931=CARTESIAN_POINT('Ctrl Pts',(-17.7734366683946,-13.9728939956966,
117.086567957188)) ;
#163932=CARTESIAN_POINT('Ctrl Pts',(-17.6996328269123,-13.972893985616,
117.110799004776)) ;
#163933=CARTESIAN_POINT('Ctrl Pts',(-17.6787592525954,-13.9370542943595,
117.047221465574)) ;
#163934=CARTESIAN_POINT('Ctrl Pts',(-17.6354116057115,-14.1729033532404,
116.879576215049)) ;
#163935=CARTESIAN_POINT('Ctrl Pts',(-17.6182703678625,-14.1205407691761,
116.827366770384)) ;
#163936=CARTESIAN_POINT('Ctrl Pts',(-17.6920742101075,-14.1205407723559,
116.803135725119)) ;
#163937=CARTESIAN_POINT('Ctrl Pts',(-17.7658780523526,-14.1205407755357,
116.778904679855)) ;
#163938=CARTESIAN_POINT('Ctrl Pts',(-17.7830192902016,-14.1729033596,116.83111412452)) ;
#163939=CARTESIAN_POINT('Ctrl Pts',(-17.8001605280506,-14.2252659436643,
116.883323569186)) ;
#163940=CARTESIAN_POINT('Ctrl Pts',(-17.7263566858056,-14.2252659404845,
116.90755461445)) ;
#163941=CARTESIAN_POINT('Ctrl Pts',(-17.6525528435606,-14.2252659373047,
116.931785659715)) ;
#163942=CARTESIAN_POINT('Ctrl Pts',(-17.6354116057115,-14.1729033532404,
116.879576215049)) ;
#163943=CARTESIAN_POINT('Ctrl Pts',(-17.5750711191891,-14.3528610645483,
116.660517699246)) ;
#163944=CARTESIAN_POINT('Ctrl Pts',(-17.5628475105947,-14.2878546501218,
116.623286559762)) ;
#163945=CARTESIAN_POINT('Ctrl Pts',(-17.6366513536394,-14.2878546504462,
116.599055516933)) ;
#163946=CARTESIAN_POINT('Ctrl Pts',(-17.7104551966841,-14.2878546507707,
116.574824474105)) ;
#163947=CARTESIAN_POINT('Ctrl Pts',(-17.7226788052785,-14.3528610651972,
116.612055613588)) ;
#163948=CARTESIAN_POINT('Ctrl Pts',(-17.7349024138729,-14.4178674796237,
116.649286753072)) ;
#163949=CARTESIAN_POINT('Ctrl Pts',(-17.6610985708282,-14.4178674792993,
116.673517795901)) ;
#163950=CARTESIAN_POINT('Ctrl Pts',(-17.5872947277835,-14.4178674789748,
116.69774883873)) ;
#163951=CARTESIAN_POINT('Ctrl Pts',(-17.5750711191891,-14.3528610645483,
116.660517699246)) ;
#163952=CARTESIAN_POINT('Ctrl Pts',(-17.5017177853474,-14.4673900074207,
116.401484107417)) ;
#163953=CARTESIAN_POINT('Ctrl Pts',(-17.4953350224789,-14.3942885636895,
116.382043241526)) ;
#163954=CARTESIAN_POINT('Ctrl Pts',(-17.5691388666226,-14.39428856281,116.357812202044)) ;
#163955=CARTESIAN_POINT('Ctrl Pts',(-17.6429427107664,-14.3942885619306,
116.333581162563)) ;
#163956=CARTESIAN_POINT('Ctrl Pts',(-17.6493254736349,-14.4673900056618,
116.353022028454)) ;
#163957=CARTESIAN_POINT('Ctrl Pts',(-17.6557082365034,-14.5404914493931,
116.372462894345)) ;
#163958=CARTESIAN_POINT('Ctrl Pts',(-17.5819043923597,-14.5404914502725,
116.396693933826)) ;
#163959=CARTESIAN_POINT('Ctrl Pts',(-17.508100548216,-14.540491451152,116.420924973308)) ;
#163960=CARTESIAN_POINT('Ctrl Pts',(-17.5017177853474,-14.4673900074207,
116.401484107417)) ;
#163961=CARTESIAN_POINT('Ctrl Pts',(-17.4223560273365,-14.5059091307987,
116.124370136875)) ;
#163962=CARTESIAN_POINT('Ctrl Pts',(-17.4222379725532,-14.4300095722764,
116.124010560988)) ;
#163963=CARTESIAN_POINT('Ctrl Pts',(-17.4960418170078,-14.4300095722936,
116.099779522454)) ;
#163964=CARTESIAN_POINT('Ctrl Pts',(-17.5698456614624,-14.4300095723109,
116.075548483919)) ;
#163965=CARTESIAN_POINT('Ctrl Pts',(-17.5699637162457,-14.5059091308332,
116.075908059805)) ;
#163966=CARTESIAN_POINT('Ctrl Pts',(-17.5700817710291,-14.5818086893555,
116.076267635692)) ;
#163967=CARTESIAN_POINT('Ctrl Pts',(-17.4962779265745,-14.5818086893382,
116.100498674226)) ;
#163968=CARTESIAN_POINT('Ctrl Pts',(-17.4224740821199,-14.581808689321,
116.124729712761)) ;
#163969=CARTESIAN_POINT('Ctrl Pts',(-17.4223560273365,-14.5059091307987,
116.124370136875)) ;
#163970=CARTESIAN_POINT('Ctrl Pts',(-17.3429501969861,-14.467003448986,
115.847090385579)) ;
#163971=CARTESIAN_POINT('Ctrl Pts',(-17.3491098301786,-14.3937086480908,
115.865851634383)) ;
#163972=CARTESIAN_POINT('Ctrl Pts',(-17.4229136742994,-14.3937086489183,
115.841620594832)) ;
#163973=CARTESIAN_POINT('Ctrl Pts',(-17.4967175184202,-14.3937086497458,
115.81738955528)) ;
#163974=CARTESIAN_POINT('Ctrl Pts',(-17.4905578852277,-14.4670034506409,
115.798628306476)) ;
#163975=CARTESIAN_POINT('Ctrl Pts',(-17.4843982520352,-14.5402982515361,
115.779867057672)) ;
#163976=CARTESIAN_POINT('Ctrl Pts',(-17.4105944079144,-14.5402982507086,
115.804098097223)) ;
#163977=CARTESIAN_POINT('Ctrl Pts',(-17.3367905637937,-14.5402982498811,
115.828329136774)) ;
#163978=CARTESIAN_POINT('Ctrl Pts',(-17.3429501969861,-14.467003448986,
115.847090385579)) ;
#163979=CARTESIAN_POINT('Ctrl Pts',(-17.2698268935793,-14.3526296857438,
115.58886231961)) ;
#163980=CARTESIAN_POINT('Ctrl Pts',(-17.281836401589,-14.2872135873285,
115.625441343297)) ;
#163981=CARTESIAN_POINT('Ctrl Pts',(-17.3556402447308,-14.2872135872054,
115.601210300764)) ;
#163982=CARTESIAN_POINT('Ctrl Pts',(-17.4294440878725,-14.2872135870823,
115.57697925823)) ;
#163983=CARTESIAN_POINT('Ctrl Pts',(-17.4174345798628,-14.3526296854977,
115.540400234544)) ;
#163984=CARTESIAN_POINT('Ctrl Pts',(-17.4054250718531,-14.418045783913,
115.503821210857)) ;
#163985=CARTESIAN_POINT('Ctrl Pts',(-17.3316212287113,-14.4180457840361,
115.528052253391)) ;
#163986=CARTESIAN_POINT('Ctrl Pts',(-17.2578173855695,-14.4180457841592,
115.552283295924)) ;
#163987=CARTESIAN_POINT('Ctrl Pts',(-17.2698268935793,-14.3526296857438,
115.58886231961)) ;
#163988=CARTESIAN_POINT('Ctrl Pts',(-17.209359096455,-14.1719531187117,
115.369308707155)) ;
#163989=CARTESIAN_POINT('Ctrl Pts',(-17.2263404094475,-14.1190573784708,
115.421031046702)) ;
#163990=CARTESIAN_POINT('Ctrl Pts',(-17.3001442516719,-14.1190573751839,
115.396800001374)) ;
#163991=CARTESIAN_POINT('Ctrl Pts',(-17.3739480938962,-14.119057371897,
115.372568956047)) ;
#163992=CARTESIAN_POINT('Ctrl Pts',(-17.3569667809037,-14.1719531121379,
115.3208466165)) ;
#163993=CARTESIAN_POINT('Ctrl Pts',(-17.3399854679112,-14.2248488523788,
115.269124276952)) ;
#163994=CARTESIAN_POINT('Ctrl Pts',(-17.2661816256868,-14.2248488556657,
115.29335532228)) ;
#163995=CARTESIAN_POINT('Ctrl Pts',(-17.1923777834625,-14.2248488589527,
115.317586367608)) ;
#163996=CARTESIAN_POINT('Ctrl Pts',(-17.209359096455,-14.1719531187117,
115.369308707155)) ;
#163997=CARTESIAN_POINT('Ctrl Pts',(-17.1661919090706,-13.936583984801,
115.202313468294)) ;
#163998=CARTESIAN_POINT('Ctrl Pts',(-17.1869470728886,-13.9000456634002,
115.265530348668)) ;
#163999=CARTESIAN_POINT('Ctrl Pts',(-17.2607509144556,-13.9000456537943,
115.241299301338)) ;
#164000=CARTESIAN_POINT('Ctrl Pts',(-17.3345547560226,-13.9000456441885,
115.217068254008)) ;
#164001=CARTESIAN_POINT('Ctrl Pts',(-17.3137995922046,-13.9365839655893,
115.153851373634)) ;
#164002=CARTESIAN_POINT('Ctrl Pts',(-17.2930444283865,-13.9731222869902,
115.09063449326)) ;
#164003=CARTESIAN_POINT('Ctrl Pts',(-17.2192405868196,-13.973122296596,
115.11486554059)) ;
#164004=CARTESIAN_POINT('Ctrl Pts',(-17.1454367452526,-13.9731223062019,
115.13909658792)) ;
#164005=CARTESIAN_POINT('Ctrl Pts',(-17.1661919090706,-13.936583984801,
115.202313468294)) ;
#164006=CARTESIAN_POINT('Ctrl Pts',(-17.1445055243567,-13.6642946874373,
115.100795313256)) ;
#164007=CARTESIAN_POINT('Ctrl Pts',(-17.1675389258918,-13.6467154172206,
115.170951338261)) ;
#164008=CARTESIAN_POINT('Ctrl Pts',(-17.2413427678139,-13.646715399489,
115.146720292013)) ;
#164009=CARTESIAN_POINT('Ctrl Pts',(-17.315146609736,-13.6467153817574,
115.122489245764)) ;
#164010=CARTESIAN_POINT('Ctrl Pts',(-17.2921132082009,-13.664294651974,
115.052333220759)) ;
#164011=CARTESIAN_POINT('Ctrl Pts',(-17.2690798066658,-13.6818739221906,
114.982177195754)) ;
#164012=CARTESIAN_POINT('Ctrl Pts',(-17.1952759647437,-13.6818739399222,
115.006408242002)) ;
#164013=CARTESIAN_POINT('Ctrl Pts',(-17.1214721228216,-13.6818739576539,
115.030639288251)) ;
#164014=CARTESIAN_POINT('Ctrl Pts',(-17.1445055243567,-13.6642946874373,
115.100795313256)) ;
#164015=CARTESIAN_POINT('Ctrl Pts',(-17.1464540999734,-13.3747428455626,
115.07130654278)) ;
#164016=CARTESIAN_POINT('Ctrl Pts',(-17.1701178080888,-13.377355159395,
115.143382380073)) ;
#164017=CARTESIAN_POINT('Ctrl Pts',(-17.2439216515979,-13.3773551335995,
115.119151338658)) ;
#164018=CARTESIAN_POINT('Ctrl Pts',(-17.3177254951069,-13.3773551078041,
115.094920297244)) ;
#164019=CARTESIAN_POINT('Ctrl Pts',(-17.2940617869915,-13.3747427939718,
115.022844459951)) ;
#164020=CARTESIAN_POINT('Ctrl Pts',(-17.270398078876,-13.3721304801394,
114.950768622658)) ;
#164021=CARTESIAN_POINT('Ctrl Pts',(-17.196594235367,-13.3721305059348,
114.974999664072)) ;
#164022=CARTESIAN_POINT('Ctrl Pts',(-17.1227903918579,-13.3721305317302,
114.999230705487)) ;
#164023=CARTESIAN_POINT('Ctrl Pts',(-17.1464540999734,-13.3747428455626,
115.07130654278)) ;
#164024=CARTESIAN_POINT('Ctrl Pts',(-17.1727178775642,-13.0876482903165,
115.115799669676)) ;
#164025=CARTESIAN_POINT('Ctrl Pts',(-17.1953167302795,-13.1103096275797,
115.184632129402)) ;
#164026=CARTESIAN_POINT('Ctrl Pts',(-17.26912057672,-13.1103095944857,115.160401096916)) ;
#164027=CARTESIAN_POINT('Ctrl Pts',(-17.3429244231604,-13.1103095613917,
115.136170064429)) ;
#164028=CARTESIAN_POINT('Ctrl Pts',(-17.320325570445,-13.0876482241285,
115.067337604704)) ;
#164029=CARTESIAN_POINT('Ctrl Pts',(-17.2977267177297,-13.0649868868653,
114.998505144978)) ;
#164030=CARTESIAN_POINT('Ctrl Pts',(-17.2239228712894,-13.0649869199593,
115.022736177464)) ;
#164031=CARTESIAN_POINT('Ctrl Pts',(-17.150119024849,-13.0649869530533,
115.04696720995)) ;
#164032=CARTESIAN_POINT('Ctrl Pts',(-17.1727178775642,-13.0876482903165,
115.115799669676)) ;
#164033=CARTESIAN_POINT('Ctrl Pts',(-17.2222028953257,-12.8243385253649,
115.231028671208)) ;
#164034=CARTESIAN_POINT('Ctrl Pts',(-17.242113859428,-12.8654169528501,
115.291674256081)) ;
#164035=CARTESIAN_POINT('Ctrl Pts',(-17.3159177100322,-12.8654169160371,
115.267443236277)) ;
#164036=CARTESIAN_POINT('Ctrl Pts',(-17.3897215606363,-12.8654168792241,
115.243212216473)) ;
#164037=CARTESIAN_POINT('Ctrl Pts',(-17.369810596534,-12.824338451739,115.1825666316)) ;
#164038=CARTESIAN_POINT('Ctrl Pts',(-17.3498996324317,-12.7832600242539,
115.121921046727)) ;
#164039=CARTESIAN_POINT('Ctrl Pts',(-17.2760957818276,-12.7832600610668,
115.146152066531)) ;
#164040=CARTESIAN_POINT('Ctrl Pts',(-17.2022919312234,-12.7832600978798,
115.170383086335)) ;
#164041=CARTESIAN_POINT('Ctrl Pts',(-17.2222028953257,-12.8243385253649,
115.231028671208)) ;
#164042=CARTESIAN_POINT('Ctrl Pts',(-17.2919810291401,-12.6038922563675,
115.408113946603)) ;
#164043=CARTESIAN_POINT('Ctrl Pts',(-17.3077823918333,-12.6604213844926,
115.456242348831)) ;
#164044=CARTESIAN_POINT('Ctrl Pts',(-17.3815862472237,-12.6604213494665,
115.432011343605)) ;
#164045=CARTESIAN_POINT('Ctrl Pts',(-17.4553901026141,-12.6604213144404,
115.407780338379)) ;
#164046=CARTESIAN_POINT('Ctrl Pts',(-17.4395887399208,-12.6038921863153,
115.359651936151)) ;
#164047=CARTESIAN_POINT('Ctrl Pts',(-17.4237873772276,-12.5473630581902,
115.311523533924)) ;
#164048=CARTESIAN_POINT('Ctrl Pts',(-17.3499835218372,-12.5473630932163,
115.33575453915)) ;
#164049=CARTESIAN_POINT('Ctrl Pts',(-17.2761796664468,-12.5473631282424,
115.359985544376)) ;
#164050=CARTESIAN_POINT('Ctrl Pts',(-17.2919810291401,-12.6038922563675,
115.408113946603)) ;
#164051=CARTESIAN_POINT('Ctrl Pts',(-17.3779184788419,-12.4415502102937,
115.634396370926)) ;
#164052=CARTESIAN_POINT('Ctrl Pts',(-17.3884766007028,-12.5094955214015,
115.666554707739)) ;
#164053=CARTESIAN_POINT('Ctrl Pts',(-17.4622804609849,-12.5094954939584,
115.642323717413)) ;
#164054=CARTESIAN_POINT('Ctrl Pts',(-17.5360843212669,-12.5094954665153,
115.618092727086)) ;
#164055=CARTESIAN_POINT('Ctrl Pts',(-17.5255261994061,-12.4415501554076,
115.585934390273)) ;
#164056=CARTESIAN_POINT('Ctrl Pts',(-17.5149680775452,-12.3736048442999,
115.553776053459)) ;
#164057=CARTESIAN_POINT('Ctrl Pts',(-17.4411642172631,-12.3736048717429,
115.578007043786)) ;
#164058=CARTESIAN_POINT('Ctrl Pts',(-17.3673603569811,-12.373604899186,
115.602238034113)) ;
#164059=CARTESIAN_POINT('Ctrl Pts',(-17.3779184788419,-12.4415502102937,
115.634396370926)) ;
#164060=CARTESIAN_POINT('Ctrl Pts',(-17.4746658472938,-12.3493107874977,
115.89357675197)) ;
#164061=CARTESIAN_POINT('Ctrl Pts',(-17.4792190454332,-12.4237944597024,
115.907445060184)) ;
#164062=CARTESIAN_POINT('Ctrl Pts',(-17.5530229099982,-12.4237944461757,
115.883214082902)) ;
#164063=CARTESIAN_POINT('Ctrl Pts',(-17.6268267745631,-12.4237944326489,
115.85898310562)) ;
#164064=CARTESIAN_POINT('Ctrl Pts',(-17.6222735764238,-12.3493107604442,
115.845114797407)) ;
#164065=CARTESIAN_POINT('Ctrl Pts',(-17.6177203782844,-12.2748270882395,
115.831246489193)) ;
#164066=CARTESIAN_POINT('Ctrl Pts',(-17.5439165137194,-12.2748271017662,
115.855477466475)) ;
#164067=CARTESIAN_POINT('Ctrl Pts',(-17.4701126491544,-12.274827115293,
115.879708443756)) ;
#164068=CARTESIAN_POINT('Ctrl Pts',(-17.4746658472938,-12.3493107874977,
115.89357675197)) ;
#164069=CARTESIAN_POINT('Ctrl Pts',(-17.5755185168944,-12.3333698024851,
116.165420915511)) ;
#164070=CARTESIAN_POINT('Ctrl Pts',(-17.5737682061993,-12.409073916813,
116.160089753013)) ;
#164071=CARTESIAN_POINT('Ctrl Pts',(-17.6475720732458,-12.409073922124,
116.135858783289)) ;
#164072=CARTESIAN_POINT('Ctrl Pts',(-17.7213759402922,-12.4090739274351,
116.111627813566)) ;
#164073=CARTESIAN_POINT('Ctrl Pts',(-17.7231262509873,-12.3333698131071,
116.116958976064)) ;
#164074=CARTESIAN_POINT('Ctrl Pts',(-17.7248765616823,-12.2576656987791,
116.122290138562)) ;
#164075=CARTESIAN_POINT('Ctrl Pts',(-17.6510726946359,-12.2576656934681,
116.146521108286)) ;
#164076=CARTESIAN_POINT('Ctrl Pts',(-17.5772688275895,-12.2576656881571,
116.170752078009)) ;
#164077=CARTESIAN_POINT('Ctrl Pts',(-17.5755185168944,-12.3333698024851,
116.165420915511)) ;
#164078=CARTESIAN_POINT('Ctrl Pts',(-17.6754893328123,-12.3958418590805,
116.434192181454)) ;
#164079=CARTESIAN_POINT('Ctrl Pts',(-17.6674960258275,-12.4672950791635,
116.40984585974)) ;
#164080=CARTESIAN_POINT('Ctrl Pts',(-17.7412998942639,-12.467295107772,
116.38561489425)) ;
#164081=CARTESIAN_POINT('Ctrl Pts',(-17.8151037627004,-12.4672951363806,
116.361383928761)) ;
#164082=CARTESIAN_POINT('Ctrl Pts',(-17.8230970696853,-12.3958419162977,
116.385730250475)) ;
#164083=CARTESIAN_POINT('Ctrl Pts',(-17.8310903766701,-12.3243886962147,
116.410076572189)) ;
#164084=CARTESIAN_POINT('Ctrl Pts',(-17.7572865082336,-12.3243886676062,
116.434307537679)) ;
#164085=CARTESIAN_POINT('Ctrl Pts',(-17.6834826397972,-12.3243886389976,
116.458538503168)) ;
#164086=CARTESIAN_POINT('Ctrl Pts',(-17.6754893328123,-12.3958418590805,
116.434192181454)) ;
#164087=CARTESIAN_POINT('Ctrl Pts',(-17.7659177540856,-12.5305465195612,
116.674353272671)) ;
#164088=CARTESIAN_POINT('Ctrl Pts',(-17.7523292107677,-12.5926984144573,
116.632964763969)) ;
#164089=CARTESIAN_POINT('Ctrl Pts',(-17.8261330771754,-12.592698466259,
116.6087337923)) ;
#164090=CARTESIAN_POINT('Ctrl Pts',(-17.8999369435831,-12.5926985180608,
116.584502820631)) ;
#164091=CARTESIAN_POINT('Ctrl Pts',(-17.913525486901,-12.5305466231647,
116.625891329333)) ;
#164092=CARTESIAN_POINT('Ctrl Pts',(-17.9271140302189,-12.4683947282686,
116.667279838035)) ;
#164093=CARTESIAN_POINT('Ctrl Pts',(-17.8533101638112,-12.4683946764668,
116.691510809704)) ;
#164094=CARTESIAN_POINT('Ctrl Pts',(-17.7795062974035,-12.4683946246651,
116.715741781372)) ;
#164095=CARTESIAN_POINT('Ctrl Pts',(-17.7659177540856,-12.5305465195612,
116.674353272671)) ;
#164096=CARTESIAN_POINT('Ctrl Pts',(-17.8428696280429,-12.7291635452138,
116.873260297753)) ;
#164097=CARTESIAN_POINT('Ctrl Pts',(-17.8246228394944,-12.7775393659294,
116.817683525794)) ;
#164098=CARTESIAN_POINT('Ctrl Pts',(-17.8984267019353,-12.7775394398199,
116.793452542043)) ;
#164099=CARTESIAN_POINT('Ctrl Pts',(-17.9722305643762,-12.7775395137104,
116.769221558292)) ;
#164100=CARTESIAN_POINT('Ctrl Pts',(-17.9904773529247,-12.7291636929948,
116.824798330251)) ;
#164101=CARTESIAN_POINT('Ctrl Pts',(-18.0087241414732,-12.6807878722793,
116.880375102209)) ;
#164102=CARTESIAN_POINT('Ctrl Pts',(-17.9349202790323,-12.6807877983888,
116.90460608596)) ;
#164103=CARTESIAN_POINT('Ctrl Pts',(-17.8611164165914,-12.6807877244983,
116.928837069711)) ;
#164104=CARTESIAN_POINT('Ctrl Pts',(-17.8428696280429,-12.7291635452138,
116.873260297753)) ;
#164105=CARTESIAN_POINT('Ctrl Pts',(-17.900952909542,-12.9771312925897,
117.014719731031)) ;
#164106=CARTESIAN_POINT('Ctrl Pts',(-17.8793578779453,-13.0082656414961,
116.948944751075)) ;
#164107=CARTESIAN_POINT('Ctrl Pts',(-17.9531617341492,-13.0082657332076,
116.924713748327)) ;
#164108=CARTESIAN_POINT('Ctrl Pts',(-18.0269655903531,-13.008265824919,
116.900482745579)) ;
#164109=CARTESIAN_POINT('Ctrl Pts',(-18.0485606219498,-12.9771314760126,
116.966257725535)) ;
#164110=CARTESIAN_POINT('Ctrl Pts',(-18.0701556535464,-12.9459971271062,
117.032032705491)) ;
#164111=CARTESIAN_POINT('Ctrl Pts',(-17.9963517973425,-12.9459970353947,
117.056263708239)) ;
#164112=CARTESIAN_POINT('Ctrl Pts',(-17.9225479411386,-12.9459969436833,
117.080494710987)) ;
#164113=CARTESIAN_POINT('Ctrl Pts',(-17.900952909542,-12.9771312925897,
117.014719731031)) ;
#164114=CARTESIAN_POINT('Ctrl Pts',(-17.9368966294271,-13.2574946761857,
117.088639322891)) ;
#164115=CARTESIAN_POINT('Ctrl Pts',(-17.9134961833614,-13.269101018714,
117.017365341841)) ;
#164116=CARTESIAN_POINT('Ctrl Pts',(-17.9873000316532,-13.2691011219862,
116.993134314994)) ;
#164117=CARTESIAN_POINT('Ctrl Pts',(-18.061103879945,-13.2691012252584,
116.968903288147)) ;
#164118=CARTESIAN_POINT('Ctrl Pts',(-18.0845043260107,-13.2574948827302,
117.040177269197)) ;
#164119=CARTESIAN_POINT('Ctrl Pts',(-18.1079047720765,-13.2458885402019,
117.111451250246)) ;
#164120=CARTESIAN_POINT('Ctrl Pts',(-18.0341009237846,-13.2458884369297,
117.135682277093)) ;
#164121=CARTESIAN_POINT('Ctrl Pts',(-17.9602970754928,-13.2458883336575,
117.15991330394)) ;
#164122=CARTESIAN_POINT('Ctrl Pts',(-17.9368966294271,-13.2574946761857,
117.088639322891)) ;
#164123=CARTESIAN_POINT('Ctrl Pts',(-17.9486369502931,-13.5486172877669,
117.088938884935)) ;
#164124=CARTESIAN_POINT('Ctrl Pts',(-17.9251161316749,-13.5399156323179,
117.017298268559)) ;
#164125=CARTESIAN_POINT('Ctrl Pts',(-17.9989199711168,-13.5399157383977,
116.993067214757)) ;
#164126=CARTESIAN_POINT('Ctrl Pts',(-18.0727238105588,-13.5399158444775,
116.968836160955)) ;
#164127=CARTESIAN_POINT('Ctrl Pts',(-18.096244629177,-13.5486174999264,
117.040476777331)) ;
#164128=CARTESIAN_POINT('Ctrl Pts',(-18.1197654477952,-13.5573191553753,
117.112117393707)) ;
#164129=CARTESIAN_POINT('Ctrl Pts',(-18.0459616083532,-13.5573190492956,
117.136348447509)) ;
#164130=CARTESIAN_POINT('Ctrl Pts',(-17.9721577689113,-13.5573189432158,
117.160579501311)) ;
#164131=CARTESIAN_POINT('Ctrl Pts',(-17.9486369502931,-13.5486172877669,
117.088938884935)) ;
#164132=CARTESIAN_POINT('Ctrl Pts',(-17.9363162489277,-13.8299622964239,
117.016005420011)) ;
#164133=CARTESIAN_POINT('Ctrl Pts',(-17.9143535893981,-13.8016053515907,
116.949110704836)) ;
#164134=CARTESIAN_POINT('Ctrl Pts',(-17.9881574200438,-13.8016054516698,
116.924879624242)) ;
#164135=CARTESIAN_POINT('Ctrl Pts',(-18.0619612506894,-13.8016055517489,
116.900648543647)) ;
#164136=CARTESIAN_POINT('Ctrl Pts',(-18.0839239102189,-13.8299624965821,
116.967543258822)) ;
#164137=CARTESIAN_POINT('Ctrl Pts',(-18.1058865697484,-13.8583194414153,
117.034437973997)) ;
#164138=CARTESIAN_POINT('Ctrl Pts',(-18.0320827391028,-13.8583193413362,
117.058669054592)) ;
#164139=CARTESIAN_POINT('Ctrl Pts',(-17.9582789084571,-13.8583192412571,
117.082900135186)) ;
#164140=CARTESIAN_POINT('Ctrl Pts',(-17.9363162489277,-13.8299622964239,
117.016005420011)) ;
#164141=CARTESIAN_POINT('Ctrl Pts',(-17.9015308192628,-14.082140489746,
116.874612226591)) ;
#164142=CARTESIAN_POINT('Ctrl Pts',(-17.8826976264503,-14.0361354675862,
116.817249362104)) ;
#164143=CARTESIAN_POINT('Ctrl Pts',(-17.9565014492006,-14.0361355534221,
116.793018257462)) ;
#164144=CARTESIAN_POINT('Ctrl Pts',(-18.0303052719508,-14.0361356392581,
116.768787152819)) ;
#164145=CARTESIAN_POINT('Ctrl Pts',(-18.0491384647633,-14.0821406614179,
116.826150017306)) ;
#164146=CARTESIAN_POINT('Ctrl Pts',(-18.0679716575757,-14.1281456835778,
116.883512881793)) ;
#164147=CARTESIAN_POINT('Ctrl Pts',(-17.9941678348255,-14.1281455977418,
116.907743986436)) ;
#164148=CARTESIAN_POINT('Ctrl Pts',(-17.9203640120752,-14.1281455119059,
116.931975091078)) ;
#164149=CARTESIAN_POINT('Ctrl Pts',(-17.9015308192628,-14.082140489746,
116.874612226591)) ;
#164150=CARTESIAN_POINT('Ctrl Pts',(-17.8474297188587,-14.2871395255682,
116.67433526165)) ;
#164151=CARTESIAN_POINT('Ctrl Pts',(-17.8330800933996,-14.2267539066878,
116.630628619884)) ;
#164152=CARTESIAN_POINT('Ctrl Pts',(-17.906883909967,-14.2267539712464,
116.606397496409)) ;
#164153=CARTESIAN_POINT('Ctrl Pts',(-17.9806877265344,-14.2267540358049,
116.582166372935)) ;
#164154=CARTESIAN_POINT('Ctrl Pts',(-17.9950373519935,-14.2871396546853,
116.625873014701)) ;
#164155=CARTESIAN_POINT('Ctrl Pts',(-18.0093869774526,-14.3475252735657,
116.669579656467)) ;
#164156=CARTESIAN_POINT('Ctrl Pts',(-17.9355831608852,-14.3475252090071,
116.693810779941)) ;
#164157=CARTESIAN_POINT('Ctrl Pts',(-17.8617793443178,-14.3475251444486,
116.718041903416)) ;
#164158=CARTESIAN_POINT('Ctrl Pts',(-17.8474297188587,-14.2871395255682,
116.67433526165)) ;
#164159=CARTESIAN_POINT('Ctrl Pts',(-17.7784858967829,-14.4298488440199,
116.428771121435)) ;
#164160=CARTESIAN_POINT('Ctrl Pts',(-17.7696642881067,-14.3594095209829,
116.401901926801)) ;
#164161=CARTESIAN_POINT('Ctrl Pts',(-17.8434681009777,-14.3594095593736,
116.377670792068)) ;
#164162=CARTESIAN_POINT('Ctrl Pts',(-17.9172719138486,-14.3594095977643,
116.353439657335)) ;
#164163=CARTESIAN_POINT('Ctrl Pts',(-17.9260935225248,-14.4298489208013,
116.380308851969)) ;
#164164=CARTESIAN_POINT('Ctrl Pts',(-17.934915131201,-14.5002882438384,
116.407178046602)) ;
#164165=CARTESIAN_POINT('Ctrl Pts',(-17.86111131833,-14.5002882054477,116.431409181336)) ;
#164166=CARTESIAN_POINT('Ctrl Pts',(-17.7873075054591,-14.500288167057,
116.455640316069)) ;
#164167=CARTESIAN_POINT('Ctrl Pts',(-17.7784858967829,-14.4298488440199,
116.428771121435)) ;
#164168=CARTESIAN_POINT('Ctrl Pts',(-17.7011619828439,-14.4994383097765,
116.157945215762)) ;
#164169=CARTESIAN_POINT('Ctrl Pts',(-17.6984564474787,-14.4240356160354,
116.149704593557)) ;
#164170=CARTESIAN_POINT('Ctrl Pts',(-17.7722602590906,-14.4240356268717,
116.125473454989)) ;
#164171=CARTESIAN_POINT('Ctrl Pts',(-17.8460640707025,-14.424035637708,
116.101242316421)) ;
#164172=CARTESIAN_POINT('Ctrl Pts',(-17.8487696060677,-14.4994383314491,
116.109482938626)) ;
#164173=CARTESIAN_POINT('Ctrl Pts',(-17.8514751414329,-14.5748410251902,
116.11772356083)) ;
#164174=CARTESIAN_POINT('Ctrl Pts',(-17.777671329821,-14.5748410143539,
116.141954699398)) ;
#164175=CARTESIAN_POINT('Ctrl Pts',(-17.7038675182091,-14.5748410035177,
116.166185837966)) ;
#164176=CARTESIAN_POINT('Ctrl Pts',(-17.7011619828439,-14.4994383097765,
116.157945215762)) ;
#164177=CARTESIAN_POINT('Ctrl Pts',(-17.6208255769599,-14.4922423916848,
115.877768836137)) ;
#164178=CARTESIAN_POINT('Ctrl Pts',(-17.6244590729136,-14.4172290917828,
115.888835880451)) ;
#164179=CARTESIAN_POINT('Ctrl Pts',(-17.6982628860497,-14.4172290756449,
115.864604746526)) ;
#164180=CARTESIAN_POINT('Ctrl Pts',(-17.7720666991857,-14.417229059507,
115.8403736126)) ;
#164181=CARTESIAN_POINT('Ctrl Pts',(-17.768433203232,-14.492242359409,115.829306568286)) ;
#164182=CARTESIAN_POINT('Ctrl Pts',(-17.7647997072783,-14.567255659311,
115.818239523972)) ;
#164183=CARTESIAN_POINT('Ctrl Pts',(-17.6909958941422,-14.5672556754489,
115.842470657898)) ;
#164184=CARTESIAN_POINT('Ctrl Pts',(-17.6171920810061,-14.5672556915868,
115.866701791824)) ;
#164185=CARTESIAN_POINT('Ctrl Pts',(-17.6208255769599,-14.4922423916848,
115.877768836137)) ;
#164186=CARTESIAN_POINT('Ctrl Pts',(-17.5442238721124,-14.4074859363464,
115.60889672167)) ;
#164187=CARTESIAN_POINT('Ctrl Pts',(-17.5539467158505,-14.3382771247353,
115.638510936711)) ;
#164188=CARTESIAN_POINT('Ctrl Pts',(-17.6277505330549,-14.3382770857767,
115.614279815176)) ;
#164189=CARTESIAN_POINT('Ctrl Pts',(-17.7015543502592,-14.3382770468181,
115.590048693642)) ;
#164190=CARTESIAN_POINT('Ctrl Pts',(-17.6918315065211,-14.4074858584293,
115.560434478601)) ;
#164191=CARTESIAN_POINT('Ctrl Pts',(-17.6821086627829,-14.4766946700404,
115.53082026356)) ;
#164192=CARTESIAN_POINT('Ctrl Pts',(-17.6083048455786,-14.476694708999,
115.555051385095)) ;
#164193=CARTESIAN_POINT('Ctrl Pts',(-17.5345010283743,-14.4766947479576,
115.579282506629)) ;
#164194=CARTESIAN_POINT('Ctrl Pts',(-17.5442238721124,-14.4074859363464,
115.60889672167)) ;
#164195=CARTESIAN_POINT('Ctrl Pts',(-17.4781148630412,-14.2527213410347,
115.372193987303)) ;
#164196=CARTESIAN_POINT('Ctrl Pts',(-17.4931993104765,-14.1942140636659,
115.418138782012)) ;
#164197=CARTESIAN_POINT('Ctrl Pts',(-17.5670031331039,-14.1942140071928,
115.393907676996)) ;
#164198=CARTESIAN_POINT('Ctrl Pts',(-17.6408069557314,-14.1942139507198,
115.369676571979)) ;
#164199=CARTESIAN_POINT('Ctrl Pts',(-17.6257225082961,-14.2527212280886,
115.32373177727)) ;
#164200=CARTESIAN_POINT('Ctrl Pts',(-17.6106380608608,-14.3112285054574,
115.27778698256)) ;
#164201=CARTESIAN_POINT('Ctrl Pts',(-17.5368342382334,-14.3112285619304,
115.302018087577)) ;
#164202=CARTESIAN_POINT('Ctrl Pts',(-17.4630304156059,-14.3112286184035,
115.326249192593)) ;
#164203=CARTESIAN_POINT('Ctrl Pts',(-17.4781148630412,-14.2527213410347,
115.372193987303)) ;
#164204=CARTESIAN_POINT('Ctrl Pts',(-17.4272659714627,-14.0372448891262,
115.181771156024)) ;
#164205=CARTESIAN_POINT('Ctrl Pts',(-17.4466589469468,-13.9936933807782,
115.240839031848)) ;
#164206=CARTESIAN_POINT('Ctrl Pts',(-17.5204627763427,-13.993693314701,
115.216607947447)) ;
#164207=CARTESIAN_POINT('Ctrl Pts',(-17.5942666057386,-13.9936932486239,
115.192376863046)) ;
#164208=CARTESIAN_POINT('Ctrl Pts',(-17.5748736302544,-14.0372447569719,
115.133308987222)) ;
#164209=CARTESIAN_POINT('Ctrl Pts',(-17.5554806547702,-14.08079626532,115.074241111398)) ;
#164210=CARTESIAN_POINT('Ctrl Pts',(-17.4816768253743,-14.0807963313971,
115.098472195799)) ;
#164211=CARTESIAN_POINT('Ctrl Pts',(-17.4078729959785,-14.0807963974743,
115.1227032802)) ;
#164212=CARTESIAN_POINT('Ctrl Pts',(-17.4272659714627,-14.0372448891262,
115.181771156024)) ;
#164213=CARTESIAN_POINT('Ctrl Pts',(-17.3965606435217,-13.7782273369584,
115.052841406963)) ;
#164214=CARTESIAN_POINT('Ctrl Pts',(-17.4188593760479,-13.7526945200312,
115.120759749758)) ;
#164215=CARTESIAN_POINT('Ctrl Pts',(-17.4926632121621,-13.75269445107,115.09652868582)) ;
#164216=CARTESIAN_POINT('Ctrl Pts',(-17.5664670482762,-13.7526943821088,
115.072297621882)) ;
#164217=CARTESIAN_POINT('Ctrl Pts',(-17.5441683157501,-13.778227199036,
115.004379279087)) ;
#164218=CARTESIAN_POINT('Ctrl Pts',(-17.5218695832239,-13.8037600159632,
114.936460936292)) ;
#164219=CARTESIAN_POINT('Ctrl Pts',(-17.4480657471097,-13.8037600849244,
114.96069200023)) ;
#164220=CARTESIAN_POINT('Ctrl Pts',(-17.3742619109955,-13.8037601538856,
114.984923064168)) ;
#164221=CARTESIAN_POINT('Ctrl Pts',(-17.3965606435217,-13.7782273369584,
115.052841406963)) ;
#164222=CARTESIAN_POINT('Ctrl Pts',(-17.3887643996198,-13.4921296981973,
114.993517684583)) ;
#164223=CARTESIAN_POINT('Ctrl Pts',(-17.4123775387182,-13.4865334475081,
115.065439497541)) ;
#164224=CARTESIAN_POINT('Ctrl Pts',(-17.4861813810062,-13.4865333838988,
115.041208452408)) ;
#164225=CARTESIAN_POINT('Ctrl Pts',(-17.5599852232941,-13.4865333202894,
115.016977407274)) ;
#164226=CARTESIAN_POINT('Ctrl Pts',(-17.5363720841956,-13.4921295709785,
114.945055594315)) ;
#164227=CARTESIAN_POINT('Ctrl Pts',(-17.5127589450972,-13.4977258216677,
114.873133781356)) ;
#164228=CARTESIAN_POINT('Ctrl Pts',(-17.4389551028092,-13.497725885277,
114.89736482649)) ;
#164229=CARTESIAN_POINT('Ctrl Pts',(-17.3651512605213,-13.4977259488864,
114.921595871624)) ;
#164230=CARTESIAN_POINT('Ctrl Pts',(-17.3887643996198,-13.4921296981973,
114.993517684583)) ;
#164231=CARTESIAN_POINT('Ctrl Pts',(-17.4051724491236,-13.2025980491625,
115.008157982313)) ;
#164232=CARTESIAN_POINT('Ctrl Pts',(-17.4284068472422,-13.2172086619386,
115.078926211216)) ;
#164233=CARTESIAN_POINT('Ctrl Pts',(-17.5022106943674,-13.2172086067816,
115.054695180816)) ;
#164234=CARTESIAN_POINT('Ctrl Pts',(-17.5760145414926,-13.2172085516246,
115.030464150416)) ;
#164235=CARTESIAN_POINT('Ctrl Pts',(-17.552780143374,-13.2025979388484,
114.959695921512)) ;
#164236=CARTESIAN_POINT('Ctrl Pts',(-17.5295457452554,-13.1879873260723,
114.888927692608)) ;
#164237=CARTESIAN_POINT('Ctrl Pts',(-17.4557418981302,-13.1879873812294,
114.913158723009)) ;
#164238=CARTESIAN_POINT('Ctrl Pts',(-17.3819380510049,-13.1879874363864,
114.937389753409)) ;
#164239=CARTESIAN_POINT('Ctrl Pts',(-17.4051724491236,-13.2025980491625,
115.008157982313)) ;
#164240=CARTESIAN_POINT('Ctrl Pts',(-17.4455328120095,-12.9267373644591,
115.095528220572)) ;
#164241=CARTESIAN_POINT('Ctrl Pts',(-17.4667203967007,-12.960631185249,
115.160062185842)) ;
#164242=CARTESIAN_POINT('Ctrl Pts',(-17.5405242469435,-12.9606311438607,
115.135831164937)) ;
#164243=CARTESIAN_POINT('Ctrl Pts',(-17.6143280971863,-12.9606311024724,
115.111600144033)) ;
#164244=CARTESIAN_POINT('Ctrl Pts',(-17.5931405124951,-12.9267372816824,
115.047066178763)) ;
#164245=CARTESIAN_POINT('Ctrl Pts',(-17.5719529278039,-12.8928434608925,
114.982532213493)) ;
#164246=CARTESIAN_POINT('Ctrl Pts',(-17.4981490775612,-12.8928435022808,
115.006763234398)) ;
#164247=CARTESIAN_POINT('Ctrl Pts',(-17.4243452273184,-12.8928435436691,
115.030994255302)) ;
#164248=CARTESIAN_POINT('Ctrl Pts',(-17.4455328120095,-12.9267373644591,
115.095528220572)) ;
#164249=CARTESIAN_POINT('Ctrl Pts',(-17.5074914960105,-12.6871394629104,
115.248815418354)) ;
#164250=CARTESIAN_POINT('Ctrl Pts',(-17.5251182336107,-12.7378139602179,
115.302503617764)) ;
#164251=CARTESIAN_POINT('Ctrl Pts',(-17.5989220852435,-12.7378139322017,
115.278272601093)) ;
#164252=CARTESIAN_POINT('Ctrl Pts',(-17.6727259368762,-12.7378139041855,
115.254041584421)) ;
#164253=CARTESIAN_POINT('Ctrl Pts',(-17.655099199276,-12.687139406878,115.200353385011)) ;
#164254=CARTESIAN_POINT('Ctrl Pts',(-17.6374724616758,-12.6364649095704,
115.146665185601)) ;
#164255=CARTESIAN_POINT('Ctrl Pts',(-17.5636686100431,-12.6364649375867,
115.170896202273)) ;
#164256=CARTESIAN_POINT('Ctrl Pts',(-17.4898647584103,-12.6364649656029,
115.195127218944)) ;
#164257=CARTESIAN_POINT('Ctrl Pts',(-17.5074914960105,-12.6871394629104,
115.248815418354)) ;
#164258=CARTESIAN_POINT('Ctrl Pts',(-17.5873854112055,-12.4995507390681,
115.456720343984)) ;
#164259=CARTESIAN_POINT('Ctrl Pts',(-17.6001938103164,-12.5633999915825,
115.495732661631)) ;
#164260=CARTESIAN_POINT('Ctrl Pts',(-17.6739976618083,-12.5633999761432,
115.471501644531)) ;
#164261=CARTESIAN_POINT('Ctrl Pts',(-17.7478015133002,-12.5633999607039,
115.447270627431)) ;
#164262=CARTESIAN_POINT('Ctrl Pts',(-17.7349931141894,-12.4995507081895,
115.408258309784)) ;
#164263=CARTESIAN_POINT('Ctrl Pts',(-17.7221847150785,-12.4357014556752,
115.369245992137)) ;
#164264=CARTESIAN_POINT('Ctrl Pts',(-17.6483808635866,-12.4357014711144,
115.393477009237)) ;
#164265=CARTESIAN_POINT('Ctrl Pts',(-17.5745770120946,-12.4357014865537,
115.417708026337)) ;
#164266=CARTESIAN_POINT('Ctrl Pts',(-17.5873854112055,-12.4995507390681,
115.456720343984)) ;
#164267=CARTESIAN_POINT('Ctrl Pts',(-17.6808646336861,-12.3773999719713,
115.705811950101)) ;
#164268=CARTESIAN_POINT('Ctrl Pts',(-17.6879027033359,-12.4498755259628,
115.727248775064)) ;
#164269=CARTESIAN_POINT('Ctrl Pts',(-17.7617065529551,-12.4498755206207,
115.70301775226)) ;
#164270=CARTESIAN_POINT('Ctrl Pts',(-17.8355104025744,-12.4498755152786,
115.678786729456)) ;
#164271=CARTESIAN_POINT('Ctrl Pts',(-17.8284723329247,-12.377399961287,
115.657349904494)) ;
#164272=CARTESIAN_POINT('Ctrl Pts',(-17.8214342632749,-12.3049244072955,
115.635913079531)) ;
#164273=CARTESIAN_POINT('Ctrl Pts',(-17.7476304136556,-12.3049244126376,
115.660144102334)) ;
#164274=CARTESIAN_POINT('Ctrl Pts',(-17.6738265640363,-12.3049244179797,
115.684375125138)) ;
#164275=CARTESIAN_POINT('Ctrl Pts',(-17.6808646336861,-12.3773999719713,
115.705811950101)) ;
#164276=CARTESIAN_POINT('Ctrl Pts',(-17.780520996489,-12.3305982965088,
115.974059722386)) ;
#164277=CARTESIAN_POINT('Ctrl Pts',(-17.7813415036169,-12.4064507655152,
115.976558854994)) ;
#164278=CARTESIAN_POINT('Ctrl Pts',(-17.8551453516194,-12.4064507656023,
115.952327827266)) ;
#164279=CARTESIAN_POINT('Ctrl Pts',(-17.9289491996219,-12.4064507656893,
115.928096799537)) ;
#164280=CARTESIAN_POINT('Ctrl Pts',(-17.928128692494,-12.3305982966829,
115.92559766693)) ;
#164281=CARTESIAN_POINT('Ctrl Pts',(-17.9273081853662,-12.2547458276765,
115.923098534322)) ;
#164282=CARTESIAN_POINT('Ctrl Pts',(-17.8535043373637,-12.2547458275895,
115.94732956205)) ;
#164283=CARTESIAN_POINT('Ctrl Pts',(-17.7797004893612,-12.2547458275024,
115.971560589778)) ;
#164284=CARTESIAN_POINT('Ctrl Pts',(-17.780520996489,-12.3305982965088,
115.974059722386)) ;
#164285=CARTESIAN_POINT('Ctrl Pts',(-17.8813348577661,-12.3609522062499,
116.245667417945)) ;
#164286=CARTESIAN_POINT('Ctrl Pts',(-17.8758509588025,-12.4347996190351,
116.228964346684)) ;
#164287=CARTESIAN_POINT('Ctrl Pts',(-17.9496548046379,-12.4347996215548,
116.204733312355)) ;
#164288=CARTESIAN_POINT('Ctrl Pts',(-18.0234586504734,-12.4347996240744,
116.180502278026)) ;
#164289=CARTESIAN_POINT('Ctrl Pts',(-18.028942549437,-12.3609522112891,
116.197205349288)) ;
#164290=CARTESIAN_POINT('Ctrl Pts',(-18.0344264484005,-12.2871047985038,
116.21390842055)) ;
#164291=CARTESIAN_POINT('Ctrl Pts',(-17.9606226025651,-12.2871047959842,
116.238139454878)) ;
#164292=CARTESIAN_POINT('Ctrl Pts',(-17.8868187567297,-12.2871047934646,
116.262370489207)) ;
#164293=CARTESIAN_POINT('Ctrl Pts',(-17.8813348577661,-12.3609522062499,
116.245667417945)) ;
#164294=CARTESIAN_POINT('Ctrl Pts',(-17.9766684026926,-12.4676416333475,
116.500474417848)) ;
#164295=CARTESIAN_POINT('Ctrl Pts',(-17.9652553121859,-12.5341505224267,
116.465711985703)) ;
#164296=CARTESIAN_POINT('Ctrl Pts',(-18.0390591561462,-12.5341505238971,
116.441480945663)) ;
#164297=CARTESIAN_POINT('Ctrl Pts',(-18.1128630001066,-12.5341505253675,
116.417249905623)) ;
#164298=CARTESIAN_POINT('Ctrl Pts',(-18.1242760906133,-12.4676416362883,
116.452012337768)) ;
#164299=CARTESIAN_POINT('Ctrl Pts',(-18.1356891811201,-12.4011327472091,
116.486774769912)) ;
#164300=CARTESIAN_POINT('Ctrl Pts',(-18.0618853371597,-12.4011327457387,
116.511005809952)) ;
#164301=CARTESIAN_POINT('Ctrl Pts',(-17.9880814931994,-12.4011327442682,
116.535236849992)) ;
#164302=CARTESIAN_POINT('Ctrl Pts',(-17.9766684026926,-12.4676416333475,
116.500474417848)) ;
#164303=CARTESIAN_POINT('Ctrl Pts',(-18.0597927746856,-12.6420295507419,
116.718229948439)) ;
#164304=CARTESIAN_POINT('Ctrl Pts',(-18.0432914214384,-12.6964607838734,
116.667969488908)) ;
#164305=CARTESIAN_POINT('Ctrl Pts',(-18.1170952645228,-12.6964607831673,
116.6437384462)) ;
#164306=CARTESIAN_POINT('Ctrl Pts',(-18.1908991076072,-12.6964607824612,
116.619507403492)) ;
#164307=CARTESIAN_POINT('Ctrl Pts',(-18.2074004608543,-12.6420295493297,
116.669767863023)) ;
#164308=CARTESIAN_POINT('Ctrl Pts',(-18.2239018141015,-12.5875983161982,
116.720028322554)) ;
#164309=CARTESIAN_POINT('Ctrl Pts',(-18.1500979710171,-12.5875983169043,
116.744259365262)) ;
#164310=CARTESIAN_POINT('Ctrl Pts',(-18.0762941279327,-12.5875983176104,
116.76849040797)) ;
#164311=CARTESIAN_POINT('Ctrl Pts',(-18.0597927746856,-12.6420295507419,
116.718229948439)) ;
#164312=CARTESIAN_POINT('Ctrl Pts',(-18.1258671840581,-12.8715204701867,
116.884091854367)) ;
#164313=CARTESIAN_POINT('Ctrl Pts',(-18.1054598564483,-12.9100077875802,
116.821934427118)) ;
#164314=CARTESIAN_POINT('Ctrl Pts',(-18.1792636993406,-12.9100077849432,
116.797703383825)) ;
#164315=CARTESIAN_POINT('Ctrl Pts',(-18.253067542233,-12.9100077823063,
116.773472340532)) ;
#164316=CARTESIAN_POINT('Ctrl Pts',(-18.2734748698428,-12.8715204649127,
116.835629767782)) ;
#164317=CARTESIAN_POINT('Ctrl Pts',(-18.2938821974526,-12.8330331475192,
116.897787195031)) ;
#164318=CARTESIAN_POINT('Ctrl Pts',(-18.2200783545602,-12.8330331501562,
116.922018238324)) ;
#164319=CARTESIAN_POINT('Ctrl Pts',(-18.1462745116679,-12.8330331527932,
116.946249281617)) ;
#164320=CARTESIAN_POINT('Ctrl Pts',(-18.1258671840581,-12.8715204701867,
116.884091854367)) ;
#164321=CARTESIAN_POINT('Ctrl Pts',(-18.1711371153448,-13.1406452081899,
116.986504143615)) ;
#164322=CARTESIAN_POINT('Ctrl Pts',(-18.1482724742896,-13.1603966221908,
116.916862136095)) ;
#164323=CARTESIAN_POINT('Ctrl Pts',(-18.2220763174873,-13.1603966190533,
116.892631093732)) ;
#164324=CARTESIAN_POINT('Ctrl Pts',(-18.295880160685,-13.1603966159158,
116.868400051369)) ;
#164325=CARTESIAN_POINT('Ctrl Pts',(-18.3187448017401,-13.1406452019148,
116.938042058889)) ;
#164326=CARTESIAN_POINT('Ctrl Pts',(-18.3416094427953,-13.1208937879139,
117.007684066409)) ;
#164327=CARTESIAN_POINT('Ctrl Pts',(-18.2678055995976,-13.1208937910514,
117.031915108772)) ;
#164328=CARTESIAN_POINT('Ctrl Pts',(-18.1940017564,-13.1208937941889,117.056146151135)) ;
#164329=CARTESIAN_POINT('Ctrl Pts',(-18.1711371153448,-13.1406452081899,
116.986504143615)) ;
#164330=CARTESIAN_POINT('Ctrl Pts',(-18.1928638298168,-13.4310927688211,
117.017038288082)) ;
#164331=CARTESIAN_POINT('Ctrl Pts',(-18.1691858546894,-13.4305915609801,
116.944918996267)) ;
#164332=CARTESIAN_POINT('Ctrl Pts',(-18.2429896982003,-13.4305915607747,
116.920687954858)) ;
#164333=CARTESIAN_POINT('Ctrl Pts',(-18.3167935417111,-13.4305915605693,
116.896456913449)) ;
#164334=CARTESIAN_POINT('Ctrl Pts',(-18.3404715168385,-13.4310927684104,
116.968576205264)) ;
#164335=CARTESIAN_POINT('Ctrl Pts',(-18.3641494919659,-13.4315939762514,
117.040695497079)) ;
#164336=CARTESIAN_POINT('Ctrl Pts',(-18.290345648455,-13.4315939764568,
117.064926538488)) ;
#164337=CARTESIAN_POINT('Ctrl Pts',(-18.2165418049442,-13.4315939766622,
117.089157579897)) ;
#164338=CARTESIAN_POINT('Ctrl Pts',(-18.1928638298168,-13.4310927688211,
117.017038288082)) ;
#164339=CARTESIAN_POINT('Ctrl Pts',(-18.1901471905866,-13.7181744540682,
116.973422879624)) ;
#164340=CARTESIAN_POINT('Ctrl Pts',(-18.1673557325083,-13.6976269857138,
116.904003775774)) ;
#164341=CARTESIAN_POINT('Ctrl Pts',(-18.2411595757253,-13.6976269892172,
116.87977273347)) ;
#164342=CARTESIAN_POINT('Ctrl Pts',(-18.3149634189423,-13.6976269927207,
116.855541691165)) ;
#164343=CARTESIAN_POINT('Ctrl Pts',(-18.3377548770205,-13.718174461075,
116.924960795015)) ;
#164344=CARTESIAN_POINT('Ctrl Pts',(-18.3605463350987,-13.7387219294293,
116.994379898865)) ;
#164345=CARTESIAN_POINT('Ctrl Pts',(-18.2867424918817,-13.7387219259259,
117.018610941169)) ;
#164346=CARTESIAN_POINT('Ctrl Pts',(-18.2129386486648,-13.7387219224225,
117.042841983473)) ;
#164347=CARTESIAN_POINT('Ctrl Pts',(-18.1901471905866,-13.7181744540682,
116.973422879624)) ;
#164348=CARTESIAN_POINT('Ctrl Pts',(-18.1642251375399,-13.9844854804917,
116.85905117826)) ;
#164349=CARTESIAN_POINT('Ctrl Pts',(-18.1439433958895,-13.9453130684822,
116.797276265807)) ;
#164350=CARTESIAN_POINT('Ctrl Pts',(-18.2177472380384,-13.9453130761656,
116.77304522025)) ;
#164351=CARTESIAN_POINT('Ctrl Pts',(-18.2915510801873,-13.945313083849,
116.748814174693)) ;
#164352=CARTESIAN_POINT('Ctrl Pts',(-18.3118328218377,-13.9844854958585,
116.810589087145)) ;
#164353=CARTESIAN_POINT('Ctrl Pts',(-18.3321145634881,-14.023657907868,
116.872363999598)) ;
#164354=CARTESIAN_POINT('Ctrl Pts',(-18.2583107213392,-14.0236579001846,
116.896595045155)) ;
#164355=CARTESIAN_POINT('Ctrl Pts',(-18.1845068791902,-14.0236578925012,
116.920826090713)) ;
#164356=CARTESIAN_POINT('Ctrl Pts',(-18.1642251375399,-13.9844854804917,
116.85905117826)) ;
#164357=CARTESIAN_POINT('Ctrl Pts',(-18.1174211789805,-14.2108138750807,
116.680986260838)) ;
#164358=CARTESIAN_POINT('Ctrl Pts',(-18.1011127388961,-14.1557813405772,
116.631313384001)) ;
#164359=CARTESIAN_POINT('Ctrl Pts',(-18.174916578883,-14.1557813517834,
116.607082331859)) ;
#164360=CARTESIAN_POINT('Ctrl Pts',(-18.24872041887,-14.1557813629896,116.582851279717)) ;
#164361=CARTESIAN_POINT('Ctrl Pts',(-18.2650288589544,-14.2108138974931,
116.632524156554)) ;
#164362=CARTESIAN_POINT('Ctrl Pts',(-18.2813372990388,-14.2658464319965,
116.682197033391)) ;
#164363=CARTESIAN_POINT('Ctrl Pts',(-18.2075334590519,-14.2658464207903,
116.706428085533)) ;
#164364=CARTESIAN_POINT('Ctrl Pts',(-18.133729619065,-14.2658464095841,
116.730659137676)) ;
#164365=CARTESIAN_POINT('Ctrl Pts',(-18.1174211789805,-14.2108138750807,
116.680986260838)) ;
#164366=CARTESIAN_POINT('Ctrl Pts',(-18.0540206588753,-14.3800184665147,
116.452418834705)) ;
#164367=CARTESIAN_POINT('Ctrl Pts',(-18.0428491294689,-14.313091902712,
116.418392159101)) ;
#164368=CARTESIAN_POINT('Ctrl Pts',(-18.1166529665764,-14.3130919141767,
116.394161098189)) ;
#164369=CARTESIAN_POINT('Ctrl Pts',(-18.190456803684,-14.3130919256413,
116.369930037277)) ;
#164370=CARTESIAN_POINT('Ctrl Pts',(-18.2016283330905,-14.3800184894439,
116.40395671288)) ;
#164371=CARTESIAN_POINT('Ctrl Pts',(-18.2127998624969,-14.4469450532465,
116.437983388484)) ;
#164372=CARTESIAN_POINT('Ctrl Pts',(-18.1389960253894,-14.4469450417819,
116.462214449397)) ;
#164373=CARTESIAN_POINT('Ctrl Pts',(-18.0651921882818,-14.4469450303173,
116.486445510309)) ;
#164374=CARTESIAN_POINT('Ctrl Pts',(-18.0540206588753,-14.3800184665147,
116.452418834705)) ;
#164375=CARTESIAN_POINT('Ctrl Pts',(-17.9792474553968,-14.4803359496639,
116.189200422911)) ;
#164376=CARTESIAN_POINT('Ctrl Pts',(-17.9740145271626,-14.4063082157353,
116.173261768448)) ;
#164377=CARTESIAN_POINT('Ctrl Pts',(-18.0478183610358,-14.4063082232175,
116.149030697684)) ;
#164378=CARTESIAN_POINT('Ctrl Pts',(-18.1216221949091,-14.4063082306997,
116.124799626921)) ;
#164379=CARTESIAN_POINT('Ctrl Pts',(-18.1268551231433,-14.4803359646283,
116.140738281384)) ;
#164380=CARTESIAN_POINT('Ctrl Pts',(-18.1320880513776,-14.554363698557,
116.156676935847)) ;
#164381=CARTESIAN_POINT('Ctrl Pts',(-18.0582842175043,-14.5543636910748,
116.180908006611)) ;
#164382=CARTESIAN_POINT('Ctrl Pts',(-17.9844803836311,-14.5543636835926,
116.205139077375)) ;
#164383=CARTESIAN_POINT('Ctrl Pts',(-17.9792474553968,-14.4803359496639,
116.189200422911)) ;
#164384=CARTESIAN_POINT('Ctrl Pts',(-17.8993604815513,-14.5045829128103,
115.910464657861)) ;
#164385=CARTESIAN_POINT('Ctrl Pts',(-17.9004305121953,-14.4287553960091,
115.913723799318)) ;
#164386=CARTESIAN_POINT('Ctrl Pts',(-17.9742343432803,-14.4287553947463,
115.889492720062)) ;
#164387=CARTESIAN_POINT('Ctrl Pts',(-18.0480381743654,-14.4287553934836,
115.865261640806)) ;
#164388=CARTESIAN_POINT('Ctrl Pts',(-18.0469681437214,-14.5045829102848,
115.862002499349)) ;
#164389=CARTESIAN_POINT('Ctrl Pts',(-18.0458981130775,-14.580410427086,
115.858743357893)) ;
#164390=CARTESIAN_POINT('Ctrl Pts',(-17.9720942819924,-14.5804104283487,
115.882974437149)) ;
#164391=CARTESIAN_POINT('Ctrl Pts',(-17.8982904509073,-14.5804104296115,
115.907205516405)) ;
#164392=CARTESIAN_POINT('Ctrl Pts',(-17.8993604815513,-14.5045829128103,
115.910464657861)) ;
#164393=CARTESIAN_POINT('Ctrl Pts',(-17.8204973524233,-14.4510580252238,
115.634757477043)) ;
#164394=CARTESIAN_POINT('Ctrl Pts',(-17.8278097544475,-14.3788579006376,
115.657029874697)) ;
#164395=CARTESIAN_POINT('Ctrl Pts',(-17.9016135833738,-14.3788578861591,
115.632798788866)) ;
#164396=CARTESIAN_POINT('Ctrl Pts',(-17.9754174123,-14.3788578716805,115.608567703034)) ;
#164397=CARTESIAN_POINT('Ctrl Pts',(-17.9681050102758,-14.4510579962666,
115.58629530538)) ;
#164398=CARTESIAN_POINT('Ctrl Pts',(-17.9607926082516,-14.5232581208527,
115.564022907727)) ;
#164399=CARTESIAN_POINT('Ctrl Pts',(-17.8869887793254,-14.5232581353313,
115.588253993558)) ;
#164400=CARTESIAN_POINT('Ctrl Pts',(-17.8131849503991,-14.5232581498099,
115.612485079389)) ;
#164401=CARTESIAN_POINT('Ctrl Pts',(-17.8204973524233,-14.4510580252238,
115.634757477043)) ;
#164402=CARTESIAN_POINT('Ctrl Pts',(-17.7492736539393,-14.3231627979094,
115.382303854319)) ;
#164403=CARTESIAN_POINT('Ctrl Pts',(-17.7623043373633,-14.2597876685306,
115.421993214653)) ;
#164404=CARTESIAN_POINT('Ctrl Pts',(-17.8361081656518,-14.2597876370506,
115.397762126879)) ;
#164405=CARTESIAN_POINT('Ctrl Pts',(-17.9099119939404,-14.2597876055706,
115.373531039106)) ;
#164406=CARTESIAN_POINT('Ctrl Pts',(-17.8968813105165,-14.3231627349493,
115.333841678772)) ;
#164407=CARTESIAN_POINT('Ctrl Pts',(-17.8838506270926,-14.386537864328,
115.294152318439)) ;
#164408=CARTESIAN_POINT('Ctrl Pts',(-17.810046798804,-14.3865378958081,
115.318383406212)) ;
#164409=CARTESIAN_POINT('Ctrl Pts',(-17.7362429705154,-14.3865379272881,
115.342614493986)) ;
#164410=CARTESIAN_POINT('Ctrl Pts',(-17.7492736539393,-14.3231627979094,
115.382303854319)) ;
#164411=CARTESIAN_POINT('Ctrl Pts',(-17.6917549715632,-14.1311846385056,
115.17173247464)) ;
#164412=CARTESIAN_POINT('Ctrl Pts',(-17.7095523530007,-14.0811216324566,
115.225940428166)) ;
#164413=CARTESIAN_POINT('Ctrl Pts',(-17.783356182875,-14.0811215835067,
115.201709345222)) ;
#164414=CARTESIAN_POINT('Ctrl Pts',(-17.8571600127492,-14.0811215345568,
115.177478262278)) ;
#164415=CARTESIAN_POINT('Ctrl Pts',(-17.8393626313117,-14.1311845406059,
115.123270308753)) ;
#164416=CARTESIAN_POINT('Ctrl Pts',(-17.8215652498742,-14.181247546655,
115.069062355227)) ;
#164417=CARTESIAN_POINT('Ctrl Pts',(-17.7477614199999,-14.1812475956048,
115.093293438171)) ;
#164418=CARTESIAN_POINT('Ctrl Pts',(-17.6739575901257,-14.1812476445547,
115.117524521115)) ;
#164419=CARTESIAN_POINT('Ctrl Pts',(-17.6917549715632,-14.1311846385056,
115.17173247464)) ;
#164420=CARTESIAN_POINT('Ctrl Pts',(-17.6523872903775,-13.8873682377616,
115.016307959891)) ;
#164421=CARTESIAN_POINT('Ctrl Pts',(-17.6736939375746,-13.8542552865156,
115.081204570868)) ;
#164422=CARTESIAN_POINT('Ctrl Pts',(-17.7474977708464,-13.8542552201397,
115.056973498272)) ;
#164423=CARTESIAN_POINT('Ctrl Pts',(-17.8213016041181,-13.8542551537638,
115.032742425676)) ;
#164424=CARTESIAN_POINT('Ctrl Pts',(-17.799994956921,-13.8873681050098,
114.9678458147)) ;
#164425=CARTESIAN_POINT('Ctrl Pts',(-17.7786883097238,-13.9204810562558,
114.902949203724)) ;
#164426=CARTESIAN_POINT('Ctrl Pts',(-17.7048844764521,-13.9204811226317,
114.92718027632)) ;
#164427=CARTESIAN_POINT('Ctrl Pts',(-17.6310806431803,-13.9204811890076,
114.951411348915)) ;
#164428=CARTESIAN_POINT('Ctrl Pts',(-17.6523872903775,-13.8873682377616,
115.016307959891)) ;
#164429=CARTESIAN_POINT('Ctrl Pts',(-17.6350445358594,-13.6103444957185,
114.928037639431)) ;
#164430=CARTESIAN_POINT('Ctrl Pts',(-17.65832634955,-13.5965245493847,114.998950288995)) ;
#164431=CARTESIAN_POINT('Ctrl Pts',(-17.7321301883026,-13.5965244695658,
114.974719233093)) ;
#164432=CARTESIAN_POINT('Ctrl Pts',(-17.8059340270552,-13.5965243897469,
114.950488177192)) ;
#164433=CARTESIAN_POINT('Ctrl Pts',(-17.7826522133646,-13.6103443360808,
114.879575527628)) ;
#164434=CARTESIAN_POINT('Ctrl Pts',(-17.7593703996741,-13.6241642824146,
114.808662878064)) ;
#164435=CARTESIAN_POINT('Ctrl Pts',(-17.6855665609215,-13.6241643622335,
114.832893933966)) ;
#164436=CARTESIAN_POINT('Ctrl Pts',(-17.6117627221689,-13.6241644420523,
114.857124989867)) ;
#164437=CARTESIAN_POINT('Ctrl Pts',(-17.6350445358594,-13.6103444957185,
114.928037639431)) ;
#164438=CARTESIAN_POINT('Ctrl Pts',(-17.6416077422069,-13.3193309051749,
114.912549638039)) ;
#164439=CARTESIAN_POINT('Ctrl Pts',(-17.66519928261,-13.3258084661624,114.984405665328)) ;
#164440=CARTESIAN_POINT('Ctrl Pts',(-17.7390031283457,-13.3258083784264,
114.960174630696)) ;
#164441=CARTESIAN_POINT('Ctrl Pts',(-17.8128069740815,-13.3258082906904,
114.935943596063)) ;
#164442=CARTESIAN_POINT('Ctrl Pts',(-17.7892154336784,-13.3193307297029,
114.864087568775)) ;
#164443=CARTESIAN_POINT('Ctrl Pts',(-17.7656238932752,-13.3128531687154,
114.792231541486)) ;
#164444=CARTESIAN_POINT('Ctrl Pts',(-17.6918200475395,-13.3128532564514,
114.816462576118)) ;
#164445=CARTESIAN_POINT('Ctrl Pts',(-17.6180162018037,-13.3128533441874,
114.84069361075)) ;
#164446=CARTESIAN_POINT('Ctrl Pts',(-17.6416077422069,-13.3193309051749,
114.912549638039)) ;
#164447=CARTESIAN_POINT('Ctrl Pts',(-17.6723780315053,-13.0356124679736,
114.970821374696)) ;
#164448=CARTESIAN_POINT('Ctrl Pts',(-17.6945891508528,-13.0619076839879,
115.038472862292)) ;
#164449=CARTESIAN_POINT('Ctrl Pts',(-17.7683930044287,-13.061907595961,
115.01424185154)) ;
#164450=CARTESIAN_POINT('Ctrl Pts',(-17.8421968580047,-13.061907507934,
114.990010840787)) ;
#164451=CARTESIAN_POINT('Ctrl Pts',(-17.8199857386572,-13.0356122919197,
114.922359353192)) ;
#164452=CARTESIAN_POINT('Ctrl Pts',(-17.7977746193098,-13.0093170759053,
114.854707865596)) ;
#164453=CARTESIAN_POINT('Ctrl Pts',(-17.7239707657338,-13.0093171639322,
114.878938876348)) ;
#164454=CARTESIAN_POINT('Ctrl Pts',(-17.6501669121579,-13.0093172519592,
114.903169887101)) ;
#164455=CARTESIAN_POINT('Ctrl Pts',(-17.6723780315053,-13.0356124679736,
114.970821374696)) ;
#164456=CARTESIAN_POINT('Ctrl Pts',(-17.7258605936467,-12.7792808148317,
115.098276186666)) ;
#164457=CARTESIAN_POINT('Ctrl Pts',(-17.7451035698503,-12.8235105133311,
115.156887189249)) ;
#164458=CARTESIAN_POINT('Ctrl Pts',(-17.8189074312596,-12.8235104331366,
115.132656202356)) ;
#164459=CARTESIAN_POINT('Ctrl Pts',(-17.892711292669,-12.8235103529421,
115.108425215463)) ;
#164460=CARTESIAN_POINT('Ctrl Pts',(-17.8734683164654,-12.7792806544427,
115.04981421288)) ;
#164461=CARTESIAN_POINT('Ctrl Pts',(-17.8542253402618,-12.7350509559433,
114.991203210297)) ;
#164462=CARTESIAN_POINT('Ctrl Pts',(-17.7804214788524,-12.7350510361378,
115.01543419719)) ;
#164463=CARTESIAN_POINT('Ctrl Pts',(-17.706617617443,-12.7350511163323,
115.039665184083)) ;
#164464=CARTESIAN_POINT('Ctrl Pts',(-17.7258605936467,-12.7792808148317,
115.098276186666)) ;
#164465=CARTESIAN_POINT('Ctrl Pts',(-17.7991432643167,-12.568318140118,
115.285978414549)) ;
#164466=CARTESIAN_POINT('Ctrl Pts',(-17.8140327994455,-12.6273412297626,
115.331329538125)) ;
#164467=CARTESIAN_POINT('Ctrl Pts',(-17.8878366678983,-12.6273411651946,
115.307098572685)) ;
#164468=CARTESIAN_POINT('Ctrl Pts',(-17.9616405363511,-12.6273411006266,
115.282867607246)) ;
#164469=CARTESIAN_POINT('Ctrl Pts',(-17.9467510012223,-12.568318010982,
115.23751648367)) ;
#164470=CARTESIAN_POINT('Ctrl Pts',(-17.9318614660935,-12.5092949213373,
115.192165360094)) ;
#164471=CARTESIAN_POINT('Ctrl Pts',(-17.8580575976407,-12.5092949859053,
115.216396325534)) ;
#164472=CARTESIAN_POINT('Ctrl Pts',(-17.7842537291879,-12.5092950504733,
115.240627290974)) ;
#164473=CARTESIAN_POINT('Ctrl Pts',(-17.7991432643167,-12.568318140118,
115.285978414549)) ;
#164474=CARTESIAN_POINT('Ctrl Pts',(-17.8875976416786,-12.4185302079718,
115.519914986139)) ;
#164475=CARTESIAN_POINT('Ctrl Pts',(-17.897067677724,-12.4880976547663,
115.548759189997)) ;
#164476=CARTESIAN_POINT('Ctrl Pts',(-17.9708715514779,-12.4880976127796,
115.524528240703)) ;
#164477=CARTESIAN_POINT('Ctrl Pts',(-18.0446754252318,-12.4880975707929,
115.50029729141)) ;
#164478=CARTESIAN_POINT('Ctrl Pts',(-18.0352053891865,-12.4185301239984,
115.471453087553)) ;
#164479=CARTESIAN_POINT('Ctrl Pts',(-18.0257353531411,-12.3489626772039,
115.442608883696)) ;
#164480=CARTESIAN_POINT('Ctrl Pts',(-17.9519314793872,-12.3489627191906,
115.466839832989)) ;
#164481=CARTESIAN_POINT('Ctrl Pts',(-17.8781276056333,-12.3489627611773,
115.491070782282)) ;
#164482=CARTESIAN_POINT('Ctrl Pts',(-17.8875976416786,-12.4185302079718,
115.519914986139)) ;
#164483=CARTESIAN_POINT('Ctrl Pts',(-17.9853421141221,-12.3404555156159,
115.782254580192)) ;
#164484=CARTESIAN_POINT('Ctrl Pts',(-17.9887338460983,-12.415576081878,
115.792585250618)) ;
#164485=CARTESIAN_POINT('Ctrl Pts',(-18.0625377227563,-12.415576066971,
115.76835431017)) ;
#164486=CARTESIAN_POINT('Ctrl Pts',(-18.1363415994144,-12.415576052064,
115.744123369722)) ;
#164487=CARTESIAN_POINT('Ctrl Pts',(-18.1329498674381,-12.3404554858018,
115.733792699297)) ;
#164488=CARTESIAN_POINT('Ctrl Pts',(-18.1295581354619,-12.2653349195397,
115.723462028871)) ;
#164489=CARTESIAN_POINT('Ctrl Pts',(-18.0557542588039,-12.2653349344467,
115.747692969319)) ;
#164490=CARTESIAN_POINT('Ctrl Pts',(-17.9819503821459,-12.2653349493537,
115.771923909767)) ;
#164491=CARTESIAN_POINT('Ctrl Pts',(-17.9853421141221,-12.3404555156159,
115.782254580192)) ;
#164492=CARTESIAN_POINT('Ctrl Pts',(-18.0868118255984,-12.3391866191646,
116.05580631284)) ;
#164493=CARTESIAN_POINT('Ctrl Pts',(-18.0838591070142,-12.414506911119,
116.046812810549)) ;
#164494=CARTESIAN_POINT('Ctrl Pts',(-18.1576629839821,-12.4145069252737,
116.022581871045)) ;
#164495=CARTESIAN_POINT('Ctrl Pts',(-18.2314668609501,-12.4145069394284,
115.998350931541)) ;
#164496=CARTESIAN_POINT('Ctrl Pts',(-18.2344195795343,-12.339186647474,
116.007344433833)) ;
#164497=CARTESIAN_POINT('Ctrl Pts',(-18.2373722981186,-12.2638663555197,
116.016337936124)) ;
#164498=CARTESIAN_POINT('Ctrl Pts',(-18.1635684211506,-12.263866341365,
116.040568875628)) ;
#164499=CARTESIAN_POINT('Ctrl Pts',(-18.0897645441826,-12.2638663272102,
116.064799815132)) ;
#164500=CARTESIAN_POINT('Ctrl Pts',(-18.0868118255984,-12.3391866191646,
116.05580631284)) ;
#164501=CARTESIAN_POINT('Ctrl Pts',(-18.1852509236495,-12.4158174303531,
116.320068764456)) ;
#164502=CARTESIAN_POINT('Ctrl Pts',(-18.1761571098729,-12.4858997019266,
116.292370477058)) ;
#164503=CARTESIAN_POINT('Ctrl Pts',(-18.2499609842654,-12.4858997440293,
116.26813952971)) ;
#164504=CARTESIAN_POINT('Ctrl Pts',(-18.3237648586579,-12.4858997861321,
116.243908582362)) ;
#164505=CARTESIAN_POINT('Ctrl Pts',(-18.3328586724345,-12.4158175145586,
116.271606869759)) ;
#164506=CARTESIAN_POINT('Ctrl Pts',(-18.3419524862111,-12.3457352429851,
116.299305157156)) ;
#164507=CARTESIAN_POINT('Ctrl Pts',(-18.2681486118186,-12.3457352008824,
116.323536104504)) ;
#164508=CARTESIAN_POINT('Ctrl Pts',(-18.1943447374261,-12.3457351587796,
116.347767051853)) ;
#164509=CARTESIAN_POINT('Ctrl Pts',(-18.1852509236495,-12.4158174303531,
116.320068764456)) ;
#164510=CARTESIAN_POINT('Ctrl Pts',(-18.2736690699775,-12.5633739390689,
116.554033969862)) ;
#164511=CARTESIAN_POINT('Ctrl Pts',(-18.2591199740358,-12.6232581610032,
116.50971977317)) ;
#164512=CARTESIAN_POINT('Ctrl Pts',(-18.3329238434958,-12.623258227084,
116.485488810798)) ;
#164513=CARTESIAN_POINT('Ctrl Pts',(-18.4067277129559,-12.6232582931649,
116.461257848426)) ;
#164514=CARTESIAN_POINT('Ctrl Pts',(-18.4212768088976,-12.5633740712307,
116.505572045118)) ;
#164515=CARTESIAN_POINT('Ctrl Pts',(-18.4358259048393,-12.5034898492964,
116.549886241811)) ;
#164516=CARTESIAN_POINT('Ctrl Pts',(-18.3620220353792,-12.5034897832155,
116.574117204182)) ;
#164517=CARTESIAN_POINT('Ctrl Pts',(-18.2882181659192,-12.5034897171346,
116.598348166554)) ;
#164518=CARTESIAN_POINT('Ctrl Pts',(-18.2736690699775,-12.5633739390689,
116.554033969862)) ;
#164519=CARTESIAN_POINT('Ctrl Pts',(-18.34761454464,-12.7732714821549,116.743674390911)) ;
#164520=CARTESIAN_POINT('Ctrl Pts',(-18.3286173868234,-12.8185910964645,
116.685812115381)) ;
#164521=CARTESIAN_POINT('Ctrl Pts',(-18.4024212492602,-12.8185911800319,
116.661581131617)) ;
#164522=CARTESIAN_POINT('Ctrl Pts',(-18.4762251116969,-12.8185912635994,
116.637350147854)) ;
#164523=CARTESIAN_POINT('Ctrl Pts',(-18.4952222695136,-12.7732716492898,
116.695212423384)) ;
#164524=CARTESIAN_POINT('Ctrl Pts',(-18.5142194273302,-12.7279520349803,
116.753074698914)) ;
#164525=CARTESIAN_POINT('Ctrl Pts',(-18.4404155648934,-12.7279519514128,
116.777305682677)) ;
#164526=CARTESIAN_POINT('Ctrl Pts',(-18.3666117024567,-12.7279518678453,
116.801536666441)) ;
#164527=CARTESIAN_POINT('Ctrl Pts',(-18.34761454464,-12.7732714821549,116.743674390911)) ;
#164528=CARTESIAN_POINT('Ctrl Pts',(-18.4016381348897,-13.0290278048664,
116.87274105532)) ;
#164529=CARTESIAN_POINT('Ctrl Pts',(-18.3795748783009,-13.0565590545988,
116.805539937565)) ;
#164530=CARTESIAN_POINT('Ctrl Pts',(-18.4533787326858,-13.0565591475459,
116.781308929277)) ;
#164531=CARTESIAN_POINT('Ctrl Pts',(-18.5271825870708,-13.056559240493,
116.757077920989)) ;
#164532=CARTESIAN_POINT('Ctrl Pts',(-18.5492458436597,-13.0290279907607,
116.824279038744)) ;
#164533=CARTESIAN_POINT('Ctrl Pts',(-18.5713091002485,-13.0014967410283,
116.891480156499)) ;
#164534=CARTESIAN_POINT('Ctrl Pts',(-18.4975052458635,-13.0014966480811,
116.915711164788)) ;
#164535=CARTESIAN_POINT('Ctrl Pts',(-18.4237013914785,-13.001496555134,
116.939942173076)) ;
#164536=CARTESIAN_POINT('Ctrl Pts',(-18.4016381348897,-13.0290278048664,
116.87274105532)) ;
#164537=CARTESIAN_POINT('Ctrl Pts',(-18.4328995250642,-13.311039520292,
116.932661649428)) ;
#164538=CARTESIAN_POINT('Ctrl Pts',(-18.4093510570389,-13.3189223773524,
116.860936817201)) ;
#164539=CARTESIAN_POINT('Ctrl Pts',(-18.4831549032372,-13.3189224724508,
116.836705783977)) ;
#164540=CARTESIAN_POINT('Ctrl Pts',(-18.5569587494355,-13.3189225675491,
116.812474750754)) ;
#164541=CARTESIAN_POINT('Ctrl Pts',(-18.5805072174607,-13.3110397104886,
116.884199582981)) ;
#164542=CARTESIAN_POINT('Ctrl Pts',(-18.6040556854859,-13.3031568534281,
116.955924415209)) ;
#164543=CARTESIAN_POINT('Ctrl Pts',(-18.5302518392876,-13.3031567583298,
116.980155448432)) ;
#164544=CARTESIAN_POINT('Ctrl Pts',(-18.4564479930894,-13.3031566632315,
117.004386481656)) ;
#164545=CARTESIAN_POINT('Ctrl Pts',(-18.4328995250642,-13.311039520292,
116.932661649428)) ;
#164546=CARTESIAN_POINT('Ctrl Pts',(-18.4402061721739,-13.6025944687999,
116.919383947434)) ;
#164547=CARTESIAN_POINT('Ctrl Pts',(-18.4168473145123,-13.5901335291486,
116.848236637664)) ;
#164548=CARTESIAN_POINT('Ctrl Pts',(-18.4906511529816,-13.5901336172138,
116.824005580899)) ;
#164549=CARTESIAN_POINT('Ctrl Pts',(-18.5644549914509,-13.5901337052789,
116.799774524135)) ;
#164550=CARTESIAN_POINT('Ctrl Pts',(-18.5878138491125,-13.6025946449302,
116.870921833905)) ;
#164551=CARTESIAN_POINT('Ctrl Pts',(-18.611172706774,-13.6150555845815,
116.942069143675)) ;
#164552=CARTESIAN_POINT('Ctrl Pts',(-18.5373688683047,-13.6150554965163,
116.96630020044)) ;
#164553=CARTESIAN_POINT('Ctrl Pts',(-18.4635650298354,-13.6150554084512,
116.990531257205)) ;
#164554=CARTESIAN_POINT('Ctrl Pts',(-18.4402061721739,-13.6025944687999,
116.919383947434)) ;
#164555=CARTESIAN_POINT('Ctrl Pts',(-18.4233520704334,-13.8812809383862,
116.83246376881)) ;
#164556=CARTESIAN_POINT('Ctrl Pts',(-18.4018709139164,-13.8493436684039,
116.767035633613)) ;
#164557=CARTESIAN_POINT('Ctrl Pts',(-18.475674746248,-13.8493437421996,
116.742804558154)) ;
#164558=CARTESIAN_POINT('Ctrl Pts',(-18.5494785785796,-13.8493438159953,
116.718573482695)) ;
#164559=CARTESIAN_POINT('Ctrl Pts',(-18.5709597350966,-13.8812810859776,
116.784001617891)) ;
#164560=CARTESIAN_POINT('Ctrl Pts',(-18.5924408916136,-13.91321835596,116.849429753088)) ;
#164561=CARTESIAN_POINT('Ctrl Pts',(-18.518637059282,-13.9132182821642,
116.873660828547)) ;
#164562=CARTESIAN_POINT('Ctrl Pts',(-18.4448332269504,-13.9132182083685,
116.897891904006)) ;
#164563=CARTESIAN_POINT('Ctrl Pts',(-18.4233520704334,-13.8812809383862,
116.83246376881)) ;
#164564=CARTESIAN_POINT('Ctrl Pts',(-18.3845330845332,-14.1255805603194,
116.67878294439)) ;
#164565=CARTESIAN_POINT('Ctrl Pts',(-18.3664632252227,-14.0765381533461,
116.623745069933)) ;
#164566=CARTESIAN_POINT('Ctrl Pts',(-18.4402670533431,-14.0765382096367,
116.599513981648)) ;
#164567=CARTESIAN_POINT('Ctrl Pts',(-18.5140708814636,-14.0765382659272,
116.575282893362)) ;
#164568=CARTESIAN_POINT('Ctrl Pts',(-18.5321407407742,-14.1255806729005,
116.630320767818)) ;
#164569=CARTESIAN_POINT('Ctrl Pts',(-18.5502106000847,-14.1746230798738,
116.685358642275)) ;
#164570=CARTESIAN_POINT('Ctrl Pts',(-18.4764067719642,-14.1746230235832,
116.70958973056)) ;
#164571=CARTESIAN_POINT('Ctrl Pts',(-18.4026029438438,-14.1746229672927,
116.733820818846)) ;
#164572=CARTESIAN_POINT('Ctrl Pts',(-18.3845330845332,-14.1255805603194,
116.67878294439)) ;
#164573=CARTESIAN_POINT('Ctrl Pts',(-18.327532397449,-14.3187775567506,
116.469844757912)) ;
#164574=CARTESIAN_POINT('Ctrl Pts',(-18.3141460031641,-14.2561721996919,
116.429071962122)) ;
#164575=CARTESIAN_POINT('Ctrl Pts',(-18.3879498288931,-14.2561722372695,
116.404840866552)) ;
#164576=CARTESIAN_POINT('Ctrl Pts',(-18.461753654622,-14.256172274847,116.380609770982)) ;
#164577=CARTESIAN_POINT('Ctrl Pts',(-18.4751400489069,-14.3187776319056,
116.421382566773)) ;
#164578=CARTESIAN_POINT('Ctrl Pts',(-18.4885264431918,-14.3813829889642,
116.462155362563)) ;
#164579=CARTESIAN_POINT('Ctrl Pts',(-18.4147226174628,-14.3813829513867,
116.486386458133)) ;
#164580=CARTESIAN_POINT('Ctrl Pts',(-18.3409187917339,-14.3813829138092,
116.510617553703)) ;
#164581=CARTESIAN_POINT('Ctrl Pts',(-18.327532397449,-14.3187775567506,
116.469844757912)) ;
#164582=CARTESIAN_POINT('Ctrl Pts',(-18.2567230506167,-14.4483980300764,
116.218709261403)) ;
#164583=CARTESIAN_POINT('Ctrl Pts',(-18.2489940958028,-14.3766476693991,
116.195168113257)) ;
#164584=CARTESIAN_POINT('Ctrl Pts',(-18.3227979214796,-14.3766476878194,
116.170937017528)) ;
#164585=CARTESIAN_POINT('Ctrl Pts',(-18.3966017471563,-14.3766477062396,
116.146705921799)) ;
#164586=CARTESIAN_POINT('Ctrl Pts',(-18.4043307019702,-14.4483980669169,
116.170247069945)) ;
#164587=CARTESIAN_POINT('Ctrl Pts',(-18.4120596567841,-14.5201484275943,
116.193788218092)) ;
#164588=CARTESIAN_POINT('Ctrl Pts',(-18.3382558311073,-14.520148409174,
116.218019313821)) ;
#164589=CARTESIAN_POINT('Ctrl Pts',(-18.2644520054306,-14.5201483907537,
116.24225040955)) ;
#164590=CARTESIAN_POINT('Ctrl Pts',(-18.2567230506167,-14.4483980300764,
116.218709261403)) ;
#164591=CARTESIAN_POINT('Ctrl Pts',(-18.1778970771393,-14.5042941688686,
115.943075214892)) ;
#164592=CARTESIAN_POINT('Ctrl Pts',(-18.1763955676776,-14.4285319857966,
115.938501860312)) ;
#164593=CARTESIAN_POINT('Ctrl Pts',(-18.2501993953997,-14.4285319877587,
115.914270770813)) ;
#164594=CARTESIAN_POINT('Ctrl Pts',(-18.3240032231218,-14.4285319897207,
115.890039681315)) ;
#164595=CARTESIAN_POINT('Ctrl Pts',(-18.3255047325835,-14.5042941727927,
115.894613035894)) ;
#164596=CARTESIAN_POINT('Ctrl Pts',(-18.3270062420453,-14.5800563558646,
115.899186390474)) ;
#164597=CARTESIAN_POINT('Ctrl Pts',(-18.2532024143231,-14.5800563539026,
115.923417479973)) ;
#164598=CARTESIAN_POINT('Ctrl Pts',(-18.179398586601,-14.5800563519406,
115.947648569472)) ;
#164599=CARTESIAN_POINT('Ctrl Pts',(-18.1778970771393,-14.5042941688686,
115.943075214892)) ;
#164600=CARTESIAN_POINT('Ctrl Pts',(-18.0975716050986,-14.4816544194473,
115.662825279825)) ;
#164601=CARTESIAN_POINT('Ctrl Pts',(-18.1024128481373,-14.4073576522614,
115.677570925769)) ;
#164602=CARTESIAN_POINT('Ctrl Pts',(-18.1762166792796,-14.4073576431116,
115.653339846688)) ;
#164603=CARTESIAN_POINT('Ctrl Pts',(-18.2500205104219,-14.4073576339619,
115.629108767606)) ;
#164604=CARTESIAN_POINT('Ctrl Pts',(-18.2451792673833,-14.4816544011478,
115.614363121662)) ;
#164605=CARTESIAN_POINT('Ctrl Pts',(-18.2403380243447,-14.5559511683337,
115.599617475718)) ;
#164606=CARTESIAN_POINT('Ctrl Pts',(-18.1665341932024,-14.5559511774834,
115.6238485548)) ;
#164607=CARTESIAN_POINT('Ctrl Pts',(-18.09273036206,-14.5559511866331,115.648079633881)) ;
#164608=CARTESIAN_POINT('Ctrl Pts',(-18.0975716050986,-14.4816544194473,
115.662825279825)) ;
#164609=CARTESIAN_POINT('Ctrl Pts',(-18.0231445471785,-14.3839486349316,
115.400927760202)) ;
#164610=CARTESIAN_POINT('Ctrl Pts',(-18.0339182338649,-14.3163620052717,
115.433742672184)) ;
#164611=CARTESIAN_POINT('Ctrl Pts',(-18.1077220678756,-14.3163619889056,
115.409511601839)) ;
#164612=CARTESIAN_POINT('Ctrl Pts',(-18.1815259018863,-14.3163619725394,
115.385280531494)) ;
#164613=CARTESIAN_POINT('Ctrl Pts',(-18.1707522151998,-14.3839486021993,
115.352465619512)) ;
#164614=CARTESIAN_POINT('Ctrl Pts',(-18.1599785285133,-14.4515352318592,
115.31965070753)) ;
#164615=CARTESIAN_POINT('Ctrl Pts',(-18.0861746945026,-14.4515352482253,
115.343881777875)) ;
#164616=CARTESIAN_POINT('Ctrl Pts',(-18.012370860492,-14.4515352645915,
115.36811284822)) ;
#164617=CARTESIAN_POINT('Ctrl Pts',(-18.0231445471785,-14.3839486349316,
115.400927760202)) ;
#164618=CARTESIAN_POINT('Ctrl Pts',(-17.9590787883367,-14.2160711628555,
115.170200653751)) ;
#164619=CARTESIAN_POINT('Ctrl Pts',(-17.9750787167157,-14.1601035188724,
115.218933854492)) ;
#164620=CARTESIAN_POINT('Ctrl Pts',(-18.0488825546563,-14.1601035014112,
115.194702796117)) ;
#164621=CARTESIAN_POINT('Ctrl Pts',(-18.1226863925968,-14.1601034839499,
115.170471737741)) ;
#164622=CARTESIAN_POINT('Ctrl Pts',(-18.1066864642176,-14.216071127933,
115.121738537)) ;
#164623=CARTESIAN_POINT('Ctrl Pts',(-18.0906865358385,-14.272038771916,
115.073005336258)) ;
#164624=CARTESIAN_POINT('Ctrl Pts',(-18.016882697898,-14.2720387893772,
115.097236394634)) ;
#164625=CARTESIAN_POINT('Ctrl Pts',(-17.9430788599575,-14.2720388068385,
115.121467453009)) ;
#164626=CARTESIAN_POINT('Ctrl Pts',(-17.9590787883367,-14.2160711628555,
115.170200653751)) ;
#164627=CARTESIAN_POINT('Ctrl Pts',(-17.9118274735837,-13.9907700541576,
114.990758589762)) ;
#164628=CARTESIAN_POINT('Ctrl Pts',(-17.9318860793349,-13.9504492968838,
115.051853866757)) ;
#164629=CARTESIAN_POINT('Ctrl Pts',(-18.0056899201662,-13.950449282471,
115.027622817187)) ;
#164630=CARTESIAN_POINT('Ctrl Pts',(-18.0794937609976,-13.9504492680581,
115.003391767616)) ;
#164631=CARTESIAN_POINT('Ctrl Pts',(-18.0594351552463,-13.9907700253318,
114.942296490621)) ;
#164632=CARTESIAN_POINT('Ctrl Pts',(-18.0393765494951,-14.0310907826056,
114.881201213626)) ;
#164633=CARTESIAN_POINT('Ctrl Pts',(-17.9655727086638,-14.0310907970185,
114.905432263197)) ;
#164634=CARTESIAN_POINT('Ctrl Pts',(-17.8917688678324,-14.0310908114314,
114.929663312767)) ;
#164635=CARTESIAN_POINT('Ctrl Pts',(-17.9118274735837,-13.9907700541576,
114.990758589762)) ;
#164636=CARTESIAN_POINT('Ctrl Pts',(-17.8853349244506,-13.7263636069236,
114.874779149551)) ;
#164637=CARTESIAN_POINT('Ctrl Pts',(-17.9080037216021,-13.7044442251976,
114.943824648292)) ;
#164638=CARTESIAN_POINT('Ctrl Pts',(-17.9818075642068,-13.7044442144499,
114.919593604122)) ;
#164639=CARTESIAN_POINT('Ctrl Pts',(-18.0556114068114,-13.7044442037021,
114.895362559953)) ;
#164640=CARTESIAN_POINT('Ctrl Pts',(-18.0329426096599,-13.7263635854281,
114.826317061213)) ;
#164641=CARTESIAN_POINT('Ctrl Pts',(-18.0102738125084,-13.7482829671541,
114.757271562473)) ;
#164642=CARTESIAN_POINT('Ctrl Pts',(-17.9364699699037,-13.7482829779018,
114.781502606642)) ;
#164643=CARTESIAN_POINT('Ctrl Pts',(-17.862666127299,-13.7482829886496,
114.805733650811)) ;
#164644=CARTESIAN_POINT('Ctrl Pts',(-17.8853349244506,-13.7263636069236,
114.874779149551)) ;
#164645=CARTESIAN_POINT('Ctrl Pts',(-17.8819867361428,-13.4372481920934,
114.82895312637)) ;
#164646=CARTESIAN_POINT('Ctrl Pts',(-17.9056609354751,-13.4354837655308,
114.901060917796)) ;
#164647=CARTESIAN_POINT('Ctrl Pts',(-17.9794647790321,-13.4354837614887,
114.876829876527)) ;
#164648=CARTESIAN_POINT('Ctrl Pts',(-18.053268622589,-13.4354837574465,
114.852598835258)) ;
#164649=CARTESIAN_POINT('Ctrl Pts',(-18.0295944232567,-13.4372481840091,
114.780491043832)) ;
#164650=CARTESIAN_POINT('Ctrl Pts',(-18.0059202239244,-13.4390126105717,
114.708383252406)) ;
#164651=CARTESIAN_POINT('Ctrl Pts',(-17.9321163803675,-13.4390126146139,
114.732614293675)) ;
#164652=CARTESIAN_POINT('Ctrl Pts',(-17.8583125368106,-13.4390126186561,
114.756845334944)) ;
#164653=CARTESIAN_POINT('Ctrl Pts',(-17.8819867361428,-13.4372481920934,
114.82895312637)) ;
#164654=CARTESIAN_POINT('Ctrl Pts',(-17.9031430677446,-13.1479585724495,
114.857914437922)) ;
#164655=CARTESIAN_POINT('Ctrl Pts',(-17.926109656016,-13.1663919966203,
114.927866960149)) ;
#164656=CARTESIAN_POINT('Ctrl Pts',(-17.9999134994939,-13.1663919968395,
114.903635918639)) ;
#164657=CARTESIAN_POINT('Ctrl Pts',(-18.0737173429717,-13.1663919970587,
114.879404877129)) ;
#164658=CARTESIAN_POINT('Ctrl Pts',(-18.0507507547003,-13.1479585728878,
114.809452354903)) ;
#164659=CARTESIAN_POINT('Ctrl Pts',(-18.0277841664289,-13.1295251487169,
114.739499832676)) ;
#164660=CARTESIAN_POINT('Ctrl Pts',(-17.953980322951,-13.1295251484978,
114.763730874186)) ;
#164661=CARTESIAN_POINT('Ctrl Pts',(-17.8801764794732,-13.1295251482786,
114.787961915695)) ;
#164662=CARTESIAN_POINT('Ctrl Pts',(-17.9031430677446,-13.1479585724495,
114.857914437922)) ;
#164663=CARTESIAN_POINT('Ctrl Pts',(-17.9474975165383,-12.8791408632362,
114.957698840491)) ;
#164664=CARTESIAN_POINT('Ctrl Pts',(-17.9681319086065,-12.9163723052174,
115.020547869334)) ;
#164665=CARTESIAN_POINT('Ctrl Pts',(-18.0419357516641,-12.9163723075118,
114.996316826545)) ;
#164666=CARTESIAN_POINT('Ctrl Pts',(-18.1157395947218,-12.9163723098062,
114.972085783755)) ;
#164667=CARTESIAN_POINT('Ctrl Pts',(-18.0951052026536,-12.8791408678251,
114.909236754912)) ;
#164668=CARTESIAN_POINT('Ctrl Pts',(-18.0744708105855,-12.8419094258439,
114.846387726068)) ;
#164669=CARTESIAN_POINT('Ctrl Pts',(-18.0006669675278,-12.8419094235494,
114.870618768858)) ;
#164670=CARTESIAN_POINT('Ctrl Pts',(-17.9268631244702,-12.841909421255,
114.894849811647)) ;
#164671=CARTESIAN_POINT('Ctrl Pts',(-17.9474975165383,-12.8791408632362,
114.957698840491)) ;
#164672=CARTESIAN_POINT('Ctrl Pts',(-18.0134578929904,-12.6468837882592,
115.122990730371)) ;
#164673=CARTESIAN_POINT('Ctrl Pts',(-18.0302539814303,-12.7003895422397,
115.174148905655)) ;
#164674=CARTESIAN_POINT('Ctrl Pts',(-18.1040578240845,-12.7003895445952,
115.149917861637)) ;
#164675=CARTESIAN_POINT('Ctrl Pts',(-18.1778616667387,-12.7003895469507,
115.125686817618)) ;
#164676=CARTESIAN_POINT('Ctrl Pts',(-18.1610655782988,-12.6468837929702,
115.074528642334)) ;
#164677=CARTESIAN_POINT('Ctrl Pts',(-18.1442694898589,-12.5933780389898,
115.02337046705)) ;
#164678=CARTESIAN_POINT('Ctrl Pts',(-18.0704656472047,-12.5933780366342,
115.047601511069)) ;
#164679=CARTESIAN_POINT('Ctrl Pts',(-17.9966618045505,-12.5933780342787,
115.071832555087)) ;
#164680=CARTESIAN_POINT('Ctrl Pts',(-18.0134578929904,-12.6468837882592,
115.122990730371)) ;
#164681=CARTESIAN_POINT('Ctrl Pts',(-18.0960334426616,-12.471578495706,
115.33917013554)) ;
#164682=CARTESIAN_POINT('Ctrl Pts',(-18.1078193608246,-12.5374039130151,
115.375068140577)) ;
#164683=CARTESIAN_POINT('Ctrl Pts',(-18.1816232036953,-12.5374039137778,
115.350837097218)) ;
#164684=CARTESIAN_POINT('Ctrl Pts',(-18.255427046566,-12.5374039145406,
115.326606053859)) ;
#164685=CARTESIAN_POINT('Ctrl Pts',(-18.243641128403,-12.4715784972316,
115.290708048822)) ;
#164686=CARTESIAN_POINT('Ctrl Pts',(-18.23185521024,-12.4057530799226,115.254810043784)) ;
#164687=CARTESIAN_POINT('Ctrl Pts',(-18.1580513673693,-12.4057530791598,
115.279041087143)) ;
#164688=CARTESIAN_POINT('Ctrl Pts',(-18.0842475244987,-12.405753078397,
115.303272130502)) ;
#164689=CARTESIAN_POINT('Ctrl Pts',(-18.0960334426616,-12.471578495706,
115.33917013554)) ;
#164690=CARTESIAN_POINT('Ctrl Pts',(-18.1907887497896,-12.3629963199509,
115.592326495504)) ;
#164691=CARTESIAN_POINT('Ctrl Pts',(-18.1967092010793,-12.4365002767228,
115.610359234894)) ;
#164692=CARTESIAN_POINT('Ctrl Pts',(-18.270513044814,-12.4365002760064,
115.586128194167)) ;
#164693=CARTESIAN_POINT('Ctrl Pts',(-18.3443168885486,-12.4365002752899,
115.561897153439)) ;
#164694=CARTESIAN_POINT('Ctrl Pts',(-18.3383964372588,-12.362996318518,
115.543864414049)) ;
#164695=CARTESIAN_POINT('Ctrl Pts',(-18.332475985969,-12.289492361746,115.525831674658)) ;
#164696=CARTESIAN_POINT('Ctrl Pts',(-18.2586721422344,-12.2894923624625,
115.550062715386)) ;
#164697=CARTESIAN_POINT('Ctrl Pts',(-18.1848682984998,-12.289492363179,
115.574293756114)) ;
#164698=CARTESIAN_POINT('Ctrl Pts',(-18.1907887497896,-12.3629963199509,
115.592326495504)) ;
#164699=CARTESIAN_POINT('Ctrl Pts',(-18.2921752354518,-12.3302292617424,
115.86545414009)) ;
#164700=CARTESIAN_POINT('Ctrl Pts',(-18.291763234642,-12.4061292172083,
115.864199252246)) ;
#164701=CARTESIAN_POINT('Ctrl Pts',(-18.3655670804045,-12.4061292167983,
115.839968217695)) ;
#164702=CARTESIAN_POINT('Ctrl Pts',(-18.439370926167,-12.4061292163883,
115.815737183144)) ;
#164703=CARTESIAN_POINT('Ctrl Pts',(-18.4397829269768,-12.3302292609224,
115.816992070988)) ;
#164704=CARTESIAN_POINT('Ctrl Pts',(-18.4401949277865,-12.2543293054565,
115.818246958833)) ;
#164705=CARTESIAN_POINT('Ctrl Pts',(-18.366391082024,-12.2543293058665,
115.842477993384)) ;
#164706=CARTESIAN_POINT('Ctrl Pts',(-18.2925872362615,-12.2543293062765,
115.866709027935)) ;
#164707=CARTESIAN_POINT('Ctrl Pts',(-18.2921752354518,-12.3302292617424,
115.86545414009)) ;
#164708=CARTESIAN_POINT('Ctrl Pts',(-18.3922296544393,-12.3757631813199,
116.134800023647)) ;
#164709=CARTESIAN_POINT('Ctrl Pts',(-18.3855635309461,-12.4485939704729,
116.114496087324)) ;
#164710=CARTESIAN_POINT('Ctrl Pts',(-18.4593673784764,-12.448593973849,
116.090265058158)) ;
#164711=CARTESIAN_POINT('Ctrl Pts',(-18.5331712260067,-12.448593977225,
116.066034028991)) ;
#164712=CARTESIAN_POINT('Ctrl Pts',(-18.5398373495,-12.3757631880721,116.086337965314)) ;
#164713=CARTESIAN_POINT('Ctrl Pts',(-18.5465034729932,-12.3029323989191,
116.106641901636)) ;
#164714=CARTESIAN_POINT('Ctrl Pts',(-18.4726996254629,-12.302932395543,
116.130872930802)) ;
#164715=CARTESIAN_POINT('Ctrl Pts',(-18.3988957779326,-12.302932392167,
116.155103959969)) ;
#164716=CARTESIAN_POINT('Ctrl Pts',(-18.3922296544393,-12.3757631813199,
116.134800023647)) ;
#164717=CARTESIAN_POINT('Ctrl Pts',(-18.4853365945326,-12.4955339259777,
116.382983514906)) ;
#164718=CARTESIAN_POINT('Ctrl Pts',(-18.4728925169486,-12.560107521336,
116.345080862824)) ;
#164719=CARTESIAN_POINT('Ctrl Pts',(-18.5466963658544,-12.5601075316302,
116.320849837847)) ;
#164720=CARTESIAN_POINT('Ctrl Pts',(-18.6205002147602,-12.5601075419243,
116.29661881287)) ;
#164721=CARTESIAN_POINT('Ctrl Pts',(-18.6329442923442,-12.495533946566,
116.334521464952)) ;
#164722=CARTESIAN_POINT('Ctrl Pts',(-18.6453883699281,-12.4309603512076,
116.372424117033)) ;
#164723=CARTESIAN_POINT('Ctrl Pts',(-18.5715845210223,-12.4309603409135,
116.39665514201)) ;
#164724=CARTESIAN_POINT('Ctrl Pts',(-18.4977806721165,-12.4309603306194,
116.420886166987)) ;
#164725=CARTESIAN_POINT('Ctrl Pts',(-18.4853365945326,-12.4955339259777,
116.382983514906)) ;
#164726=CARTESIAN_POINT('Ctrl Pts',(-18.5656035304385,-12.6811191445398,
116.592065198689)) ;
#164727=CARTESIAN_POINT('Ctrl Pts',(-18.5482696175564,-12.7328282545194,
116.539268897404)) ;
#164728=CARTESIAN_POINT('Ctrl Pts',(-18.622073466999,-12.7328282744618,
116.515037874062)) ;
#164729=CARTESIAN_POINT('Ctrl Pts',(-18.6958773164415,-12.7328282944042,
116.49080685072)) ;
#164730=CARTESIAN_POINT('Ctrl Pts',(-18.7132112293236,-12.6811191844247,
116.543603152005)) ;
#164731=CARTESIAN_POINT('Ctrl Pts',(-18.7305451422058,-12.6294100744451,
116.596399453291)) ;
#164732=CARTESIAN_POINT('Ctrl Pts',(-18.6567412927632,-12.6294100545027,
116.620630476633)) ;
#164733=CARTESIAN_POINT('Ctrl Pts',(-18.5829374433206,-12.6294100345603,
116.644861499975)) ;
#164734=CARTESIAN_POINT('Ctrl Pts',(-18.5656035304385,-12.6811191445398,
116.592065198689)) ;
#164735=CARTESIAN_POINT('Ctrl Pts',(-18.628225520823,-12.9201897809832,
116.747282894815)) ;
#164736=CARTESIAN_POINT('Ctrl Pts',(-18.6072291656349,-12.9552816729516,
116.683331385371)) ;
#164737=CARTESIAN_POINT('Ctrl Pts',(-18.6810330145034,-12.9552817052441,
116.659100360281)) ;
#164738=CARTESIAN_POINT('Ctrl Pts',(-18.7548368633718,-12.9552817375366,
116.63486933519)) ;
#164739=CARTESIAN_POINT('Ctrl Pts',(-18.77583321856,-12.9201898455682,116.698820844634)) ;
#164740=CARTESIAN_POINT('Ctrl Pts',(-18.7968295737481,-12.8850979535998,
116.762772354078)) ;
#164741=CARTESIAN_POINT('Ctrl Pts',(-18.7230257248796,-12.8850979213072,
116.787003379169)) ;
#164742=CARTESIAN_POINT('Ctrl Pts',(-18.6492218760112,-12.8850978890147,
116.811234404259)) ;
#164743=CARTESIAN_POINT('Ctrl Pts',(-18.628225520823,-12.9201897809832,
116.747282894815)) ;
#164744=CARTESIAN_POINT('Ctrl Pts',(-18.6690904271768,-13.1945616988577,
116.836294766696)) ;
#164745=CARTESIAN_POINT('Ctrl Pts',(-18.645944233313,-13.2105476900329,
116.765795195688)) ;
#164746=CARTESIAN_POINT('Ctrl Pts',(-18.7197480798482,-13.2105477342474,
116.741564163491)) ;
#164747=CARTESIAN_POINT('Ctrl Pts',(-18.7935519263835,-13.2105477784618,
116.717333131293)) ;
#164748=CARTESIAN_POINT('Ctrl Pts',(-18.8166981202473,-13.1945617872866,
116.787832702302)) ;
#164749=CARTESIAN_POINT('Ctrl Pts',(-18.8398443141111,-13.1785757961114,
116.85833227331)) ;
#164750=CARTESIAN_POINT('Ctrl Pts',(-18.7660404675759,-13.178575751897,
116.882563305508)) ;
#164751=CARTESIAN_POINT('Ctrl Pts',(-18.6922366210406,-13.1785757076825,
116.906794337705)) ;
#164752=CARTESIAN_POINT('Ctrl Pts',(-18.6690904271768,-13.1945616988577,
116.836294766696)) ;
#164753=CARTESIAN_POINT('Ctrl Pts',(-18.6862129676211,-13.4849425718836,
116.8529861804)) ;
#164754=CARTESIAN_POINT('Ctrl Pts',(-18.6625716253769,-13.4806775745737,
116.780978467484)) ;
#164755=CARTESIAN_POINT('Ctrl Pts',(-18.7363754679992,-13.4806776285265,
116.756747423369)) ;
#164756=CARTESIAN_POINT('Ctrl Pts',(-18.8101793106214,-13.4806776824793,
116.732516379253)) ;
#164757=CARTESIAN_POINT('Ctrl Pts',(-18.8338206528657,-13.4849426797892,
116.804524092169)) ;
#164758=CARTESIAN_POINT('Ctrl Pts',(-18.8574619951098,-13.4892076770991,
116.876531805084)) ;
#164759=CARTESIAN_POINT('Ctrl Pts',(-18.7836581524876,-13.4892076231463,
116.9007628492)) ;
#164760=CARTESIAN_POINT('Ctrl Pts',(-18.7098543098653,-13.4892075691935,
116.924993893315)) ;
#164761=CARTESIAN_POINT('Ctrl Pts',(-18.6862129676211,-13.4849425718836,
116.8529861804)) ;
#164762=CARTESIAN_POINT('Ctrl Pts',(-18.6790048652342,-13.7714537290315,
116.795457387519)) ;
#164763=CARTESIAN_POINT('Ctrl Pts',(-18.656568594331,-13.7471788354609,
116.727120127656)) ;
#164764=CARTESIAN_POINT('Ctrl Pts',(-18.730372431532,-13.7471788958938,
116.702889067029)) ;
#164765=CARTESIAN_POINT('Ctrl Pts',(-18.8041762687331,-13.7471789563267,
116.678658006401)) ;
#164766=CARTESIAN_POINT('Ctrl Pts',(-18.8266125396363,-13.7714538498972,
116.746995266264)) ;
#164767=CARTESIAN_POINT('Ctrl Pts',(-18.8490488105395,-13.7957287434678,
116.815332526127)) ;
#164768=CARTESIAN_POINT('Ctrl Pts',(-18.7752449733385,-13.7957286830349,
116.839563586755)) ;
#164769=CARTESIAN_POINT('Ctrl Pts',(-18.7014411361375,-13.7957286226021,
116.863794647382)) ;
#164770=CARTESIAN_POINT('Ctrl Pts',(-18.6790048652342,-13.7714537290315,
116.795457387519)) ;
#164771=CARTESIAN_POINT('Ctrl Pts',(-18.6487103937416,-14.0317199143361,
116.667704011276)) ;
#164772=CARTESIAN_POINT('Ctrl Pts',(-18.6290909043466,-13.9892386384962,
116.60794621356)) ;
#164773=CARTESIAN_POINT('Ctrl Pts',(-18.7028947352582,-13.9892386981122,
116.583715133776)) ;
#164774=CARTESIAN_POINT('Ctrl Pts',(-18.7766985661698,-13.9892387577282,
116.559484053992)) ;
#164775=CARTESIAN_POINT('Ctrl Pts',(-18.7963180555648,-14.0317200335681,
116.619241851708)) ;
#164776=CARTESIAN_POINT('Ctrl Pts',(-18.8159375449598,-14.074201309408,
116.678999649423)) ;
#164777=CARTESIAN_POINT('Ctrl Pts',(-18.7421337140482,-14.074201249792,
116.703230729208)) ;
#164778=CARTESIAN_POINT('Ctrl Pts',(-18.6683298831366,-14.074201190176,
116.727461808992)) ;
#164779=CARTESIAN_POINT('Ctrl Pts',(-18.6487103937416,-14.0317199143361,
116.667704011276)) ;
#164780=CARTESIAN_POINT('Ctrl Pts',(-18.5987182341278,-14.2471737495219,
116.480143302008)) ;
#164781=CARTESIAN_POINT('Ctrl Pts',(-18.5832910387344,-14.1895888186294,
116.433154555517)) ;
#164782=CARTESIAN_POINT('Ctrl Pts',(-18.6570948637155,-14.1895888696549,
116.408923457669)) ;
#164783=CARTESIAN_POINT('Ctrl Pts',(-18.7308986886966,-14.1895889206804,
116.384692359822)) ;
#164784=CARTESIAN_POINT('Ctrl Pts',(-18.74632588409,-14.2471738515729,116.431681106313)) ;
#164785=CARTESIAN_POINT('Ctrl Pts',(-18.7617530794833,-14.3047587824654,
116.478669852804)) ;
#164786=CARTESIAN_POINT('Ctrl Pts',(-18.6879492545022,-14.3047587314399,
116.502900950651)) ;
#164787=CARTESIAN_POINT('Ctrl Pts',(-18.6141454295211,-14.3047586804144,
116.527132048499)) ;
#164788=CARTESIAN_POINT('Ctrl Pts',(-18.5987182341278,-14.2471737495219,
116.480143302008)) ;
#164789=CARTESIAN_POINT('Ctrl Pts',(-18.5323754157414,-14.4050269028801,
116.242414711586)) ;
#164790=CARTESIAN_POINT('Ctrl Pts',(-18.5222953540112,-14.3363371537911,
116.211712471641)) ;
#164791=CARTESIAN_POINT('Ctrl Pts',(-18.5960991729972,-14.3363371907916,
116.187481355534)) ;
#164792=CARTESIAN_POINT('Ctrl Pts',(-18.6699029919832,-14.3363372277921,
116.163250239426)) ;
#164793=CARTESIAN_POINT('Ctrl Pts',(-18.6799830537135,-14.4050269768811,
116.193952479371)) ;
#164794=CARTESIAN_POINT('Ctrl Pts',(-18.6900631154437,-14.47371672597,116.224654719315)) ;
#164795=CARTESIAN_POINT('Ctrl Pts',(-18.6162592964577,-14.4737166889695,
116.248885835423)) ;
#164796=CARTESIAN_POINT('Ctrl Pts',(-18.5424554774717,-14.473716651969,
116.273116951531)) ;
#164797=CARTESIAN_POINT('Ctrl Pts',(-18.5323754157414,-14.4050269028801,
116.242414711586)) ;
#164798=CARTESIAN_POINT('Ctrl Pts',(-18.4563272491272,-14.4907853879862,
115.975423526265)) ;
#164799=CARTESIAN_POINT('Ctrl Pts',(-18.4522736812048,-14.4160085433366,
115.963077014191)) ;
#164800=CARTESIAN_POINT('Ctrl Pts',(-18.5260774963464,-14.4160085589544,
115.938845886374)) ;
#164801=CARTESIAN_POINT('Ctrl Pts',(-18.5998813114879,-14.4160085745722,
115.914614758556)) ;
#164802=CARTESIAN_POINT('Ctrl Pts',(-18.6039348794103,-14.4907854192218,
115.92696127063)) ;
#164803=CARTESIAN_POINT('Ctrl Pts',(-18.6079884473327,-14.5655622638714,
115.939307782704)) ;
#164804=CARTESIAN_POINT('Ctrl Pts',(-18.5341846321912,-14.5655622482536,
115.963538910521)) ;
#164805=CARTESIAN_POINT('Ctrl Pts',(-18.4603808170497,-14.5655622326357,
115.987770038338)) ;
#164806=CARTESIAN_POINT('Ctrl Pts',(-18.4563272491272,-14.4907853879862,
115.975423526265)) ;
#164807=CARTESIAN_POINT('Ctrl Pts',(-18.3762354271177,-14.5004458117326,
115.696087954161)) ;
#164808=CARTESIAN_POINT('Ctrl Pts',(-18.3784999234747,-14.4248856962509,
115.702985246563)) ;
#164809=CARTESIAN_POINT('Ctrl Pts',(-18.4523037367887,-14.4248856868723,
115.678754113179)) ;
#164810=CARTESIAN_POINT('Ctrl Pts',(-18.5261075501026,-14.4248856774938,
115.654522979795)) ;
#164811=CARTESIAN_POINT('Ctrl Pts',(-18.5238430537456,-14.5004457929755,
115.647625687394)) ;
#164812=CARTESIAN_POINT('Ctrl Pts',(-18.5215785573886,-14.5760059084573,
115.640728394992)) ;
#164813=CARTESIAN_POINT('Ctrl Pts',(-18.4477747440747,-14.5760059178358,
115.664959528376)) ;
#164814=CARTESIAN_POINT('Ctrl Pts',(-18.3739709307607,-14.5760059272144,
115.68919066176)) ;
#164815=CARTESIAN_POINT('Ctrl Pts',(-18.3762354271177,-14.5004458117326,
115.696087954161)) ;
#164816=CARTESIAN_POINT('Ctrl Pts',(-18.2982431956715,-14.4322721687238,
115.422987302609)) ;
#164817=CARTESIAN_POINT('Ctrl Pts',(-18.3066916637093,-14.3613608624439,
115.448719975064)) ;
#164818=CARTESIAN_POINT('Ctrl Pts',(-18.3804954774937,-14.3613608259143,
115.424488843113)) ;
#164819=CARTESIAN_POINT('Ctrl Pts',(-18.4542992912781,-14.3613607893847,
115.400257711162)) ;
#164820=CARTESIAN_POINT('Ctrl Pts',(-18.4458508232403,-14.4322720956646,
115.374525038708)) ;
#164821=CARTESIAN_POINT('Ctrl Pts',(-18.4374023552024,-14.5031834019444,
115.348792366253)) ;
#164822=CARTESIAN_POINT('Ctrl Pts',(-18.363598541418,-14.5031834384741,
115.373023498204)) ;
#164823=CARTESIAN_POINT('Ctrl Pts',(-18.2897947276336,-14.5031834750037,
115.397254630155)) ;
#164824=CARTESIAN_POINT('Ctrl Pts',(-18.2982431956715,-14.4322721687238,
115.422987302609)) ;
#164825=CARTESIAN_POINT('Ctrl Pts',(-18.2293158225121,-14.2916898608516,
115.177622248156)) ;
#164826=CARTESIAN_POINT('Ctrl Pts',(-18.2433218842617,-14.2304895577996,
115.220282454403)) ;
#164827=CARTESIAN_POINT('Ctrl Pts',(-18.3171257013558,-14.2304894954371,
115.196051332533)) ;
#164828=CARTESIAN_POINT('Ctrl Pts',(-18.3909295184499,-14.2304894330745,
115.171820210663)) ;
#164829=CARTESIAN_POINT('Ctrl Pts',(-18.3769234567003,-14.2916897361264,
115.129160004416)) ;
#164830=CARTESIAN_POINT('Ctrl Pts',(-18.3629173949507,-14.3528900391783,
115.086499798169)) ;
#164831=CARTESIAN_POINT('Ctrl Pts',(-18.2891135778566,-14.3528901015409,
115.110730920039)) ;
#164832=CARTESIAN_POINT('Ctrl Pts',(-18.2153097607625,-14.3528901639035,
115.134962041909)) ;
#164833=CARTESIAN_POINT('Ctrl Pts',(-18.2293158225121,-14.2916898608516,
115.177622248156)) ;
#164834=CARTESIAN_POINT('Ctrl Pts',(-18.174749864149,-14.0883182665925,
114.975935730207)) ;
#164835=CARTESIAN_POINT('Ctrl Pts',(-18.1933204074683,-14.0412264219864,
115.032498610884)) ;
#164836=CARTESIAN_POINT('Ctrl Pts',(-18.2671242302435,-14.0412263375894,
115.008267506318)) ;
#164837=CARTESIAN_POINT('Ctrl Pts',(-18.3409280530187,-14.0412262531924,
114.984036401752)) ;
#164838=CARTESIAN_POINT('Ctrl Pts',(-18.3223575096994,-14.0883180977985,
114.927473521075)) ;
#164839=CARTESIAN_POINT('Ctrl Pts',(-18.3037869663801,-14.1354099424045,
114.870910640398)) ;
#164840=CARTESIAN_POINT('Ctrl Pts',(-18.2299831436049,-14.1354100268015,
114.895141744964)) ;
#164841=CARTESIAN_POINT('Ctrl Pts',(-18.1561793208297,-14.1354101111986,
114.91937284953)) ;
#164842=CARTESIAN_POINT('Ctrl Pts',(-18.174749864149,-14.0883182665925,
114.975935730207)) ;
#164843=CARTESIAN_POINT('Ctrl Pts',(-18.1394221450982,-13.837248063462,
114.832902227183)) ;
#164844=CARTESIAN_POINT('Ctrl Pts',(-18.1612196540967,-13.8076155637165,
114.89929392467)) ;
#164845=CARTESIAN_POINT('Ctrl Pts',(-18.2350234844896,-13.8076154638135,
114.875062843306)) ;
#164846=CARTESIAN_POINT('Ctrl Pts',(-18.3088273148824,-13.8076153639105,
114.850831761941)) ;
#164847=CARTESIAN_POINT('Ctrl Pts',(-18.2870298058839,-13.837247863656,
114.784440064455)) ;
#164848=CARTESIAN_POINT('Ctrl Pts',(-18.2652322968854,-13.8668803634015,
114.718048366968)) ;
#164849=CARTESIAN_POINT('Ctrl Pts',(-18.1914284664925,-13.8668804633045,
114.742279448332)) ;
#164850=CARTESIAN_POINT('Ctrl Pts',(-18.1176246360997,-13.8668805632075,
114.766510529696)) ;
#164851=CARTESIAN_POINT('Ctrl Pts',(-18.1394221450982,-13.837248063462,
114.832902227183)) ;
#164852=CARTESIAN_POINT('Ctrl Pts',(-18.1264317715052,-13.5564419727403,
114.757928115676)) ;
#164853=CARTESIAN_POINT('Ctrl Pts',(-18.1499010771967,-13.5463705176912,
114.829411836148)) ;
#164854=CARTESIAN_POINT('Ctrl Pts',(-18.2237049163352,-13.5463704101859,
114.805180781422)) ;
#164855=CARTESIAN_POINT('Ctrl Pts',(-18.2975087554736,-13.5463703026806,
114.780949726695)) ;
#164856=CARTESIAN_POINT('Ctrl Pts',(-18.2740394497822,-13.5564417577297,
114.709466006223)) ;
#164857=CARTESIAN_POINT('Ctrl Pts',(-18.2505701440907,-13.5665132127787,
114.637982285751)) ;
#164858=CARTESIAN_POINT('Ctrl Pts',(-18.1767663049522,-13.5665133202841,
114.662213340477)) ;
#164859=CARTESIAN_POINT('Ctrl Pts',(-18.1029624658138,-13.5665134277894,
114.686444395204)) ;
#164860=CARTESIAN_POINT('Ctrl Pts',(-18.1264317715052,-13.5564419727403,
114.757928115676)) ;
#164861=CARTESIAN_POINT('Ctrl Pts',(-18.1376262361485,-13.2643191465395,
114.756443371031)) ;
#164862=CARTESIAN_POINT('Ctrl Pts',(-18.1610852002023,-13.2746275458087,
114.827895592519)) ;
#164863=CARTESIAN_POINT('Ctrl Pts',(-18.2348890483907,-13.2746274398407,
114.803664565357)) ;
#164864=CARTESIAN_POINT('Ctrl Pts',(-18.3086928965791,-13.2746273338727,
114.779433538195)) ;
#164865=CARTESIAN_POINT('Ctrl Pts',(-18.2852339325253,-13.2643189346036,
114.707981316708)) ;
#164866=CARTESIAN_POINT('Ctrl Pts',(-18.2617749684715,-13.2540105353345,
114.636529095221)) ;
#164867=CARTESIAN_POINT('Ctrl Pts',(-18.1879711202831,-13.2540106413025,
114.660760122383)) ;
#164868=CARTESIAN_POINT('Ctrl Pts',(-18.1141672720947,-13.2540107472704,
114.684991149544)) ;
#164869=CARTESIAN_POINT('Ctrl Pts',(-18.1376262361485,-13.2643191465395,
114.756443371031)) ;
#164870=CARTESIAN_POINT('Ctrl Pts',(-18.1728174422769,-12.984649033957,
114.828230732684)) ;
#164871=CARTESIAN_POINT('Ctrl Pts',(-18.1945868419176,-13.0144985177463,
114.894536813537)) ;
#164872=CARTESIAN_POINT('Ctrl Pts',(-18.2683906984416,-13.0144984216522,
114.870305811764)) ;
#164873=CARTESIAN_POINT('Ctrl Pts',(-18.3421945549656,-13.0144983255582,
114.846074809991)) ;
#164874=CARTESIAN_POINT('Ctrl Pts',(-18.3204251553249,-12.9846488417689,
114.779768729138)) ;
#164875=CARTESIAN_POINT('Ctrl Pts',(-18.2986557556843,-12.9547993579796,
114.713462648285)) ;
#164876=CARTESIAN_POINT('Ctrl Pts',(-18.2248518991603,-12.9547994540736,
114.737693650058)) ;
#164877=CARTESIAN_POINT('Ctrl Pts',(-18.1510480426363,-12.9547995501676,
114.761924651831)) ;
#164878=CARTESIAN_POINT('Ctrl Pts',(-18.1728174422769,-12.984649033957,
114.828230732684)) ;
#164879=CARTESIAN_POINT('Ctrl Pts',(-18.2303714670288,-12.7352694992048,
114.968035708061)) ;
#164880=CARTESIAN_POINT('Ctrl Pts',(-18.2488896504848,-12.782574545107,
115.02443910893)) ;
#164881=CARTESIAN_POINT('Ctrl Pts',(-18.3226935138459,-12.7825744663775,
115.000208127982)) ;
#164882=CARTESIAN_POINT('Ctrl Pts',(-18.396497377207,-12.782574387648,114.975977147033)) ;
#164883=CARTESIAN_POINT('Ctrl Pts',(-18.377979193751,-12.7352693417458,
114.919573746164)) ;
#164884=CARTESIAN_POINT('Ctrl Pts',(-18.3594610102951,-12.6879642958436,
114.863170345295)) ;
#164885=CARTESIAN_POINT('Ctrl Pts',(-18.285657146934,-12.6879643745731,
114.887401326243)) ;
#164886=CARTESIAN_POINT('Ctrl Pts',(-18.2118532835729,-12.6879644533026,
114.911632307191)) ;
#164887=CARTESIAN_POINT('Ctrl Pts',(-18.2303714670288,-12.7352694992048,
114.968035708061)) ;
#164888=CARTESIAN_POINT('Ctrl Pts',(-18.3068452079196,-12.5350620992742,
115.165496321728)) ;
#164889=CARTESIAN_POINT('Ctrl Pts',(-18.320785813042,-12.5964160722861,
115.207957157497)) ;
#164890=CARTESIAN_POINT('Ctrl Pts',(-18.3945896810827,-12.5964160160119,
115.183726190802)) ;
#164891=CARTESIAN_POINT('Ctrl Pts',(-18.4683935491234,-12.5964159597377,
115.159495224107)) ;
#164892=CARTESIAN_POINT('Ctrl Pts',(-18.454452944001,-12.5350619867258,
115.117034388338)) ;
#164893=CARTESIAN_POINT('Ctrl Pts',(-18.4405123388787,-12.4737080137138,
115.07457355257)) ;
#164894=CARTESIAN_POINT('Ctrl Pts',(-18.366708470838,-12.4737080699881,
115.098804519265)) ;
#164895=CARTESIAN_POINT('Ctrl Pts',(-18.2929046027973,-12.4737081262623,
115.12303548596)) ;
#164896=CARTESIAN_POINT('Ctrl Pts',(-18.3068452079196,-12.5350620992742,
115.165496321728)) ;
#164897=CARTESIAN_POINT('Ctrl Pts',(-18.3974508093172,-12.3981381252086,
115.406021891207)) ;
#164898=CARTESIAN_POINT('Ctrl Pts',(-18.4058198790453,-12.4691440372206,
115.431512729026)) ;
#164899=CARTESIAN_POINT('Ctrl Pts',(-18.4796237493277,-12.4691440057978,
115.407281769159)) ;
#164900=CARTESIAN_POINT('Ctrl Pts',(-18.5534276196102,-12.4691439743751,
115.383050809292)) ;
#164901=CARTESIAN_POINT('Ctrl Pts',(-18.5450585498822,-12.3981380623631,
115.357559971473)) ;
#164902=CARTESIAN_POINT('Ctrl Pts',(-18.5366894801541,-12.3271321503511,
115.332069133653)) ;
#164903=CARTESIAN_POINT('Ctrl Pts',(-18.4628856098716,-12.3271321817739,
115.35630009352)) ;
#164904=CARTESIAN_POINT('Ctrl Pts',(-18.3890817395891,-12.3271322131966,
115.380531053387)) ;
#164905=CARTESIAN_POINT('Ctrl Pts',(-18.3974508093172,-12.3981381252086,
115.406021891207)) ;
#164906=CARTESIAN_POINT('Ctrl Pts',(-18.4965924125013,-12.3341497286325,
115.672519382592)) ;
#164907=CARTESIAN_POINT('Ctrl Pts',(-18.498786179809,-12.4097302348877,
115.679201245499)) ;
#164908=CARTESIAN_POINT('Ctrl Pts',(-18.5725900497718,-12.4097302280834,
115.654970284658)) ;
#164909=CARTESIAN_POINT('Ctrl Pts',(-18.6463939197346,-12.409730221279,
115.630739323818)) ;
#164910=CARTESIAN_POINT('Ctrl Pts',(-18.644200152427,-12.3341497150238,
115.624057460911)) ;
#164911=CARTESIAN_POINT('Ctrl Pts',(-18.6420063851193,-12.2585692087685,
115.617375598005)) ;
#164912=CARTESIAN_POINT('Ctrl Pts',(-18.5682025151565,-12.2585692155729,
115.641606558845)) ;
#164913=CARTESIAN_POINT('Ctrl Pts',(-18.4943986451936,-12.2585692223772,
115.665837519686)) ;
#164914=CARTESIAN_POINT('Ctrl Pts',(-18.4965924125013,-12.3341497286325,
115.672519382592)) ;
#164915=CARTESIAN_POINT('Ctrl Pts',(-18.5978909913726,-12.3478638226298,
115.945574148907)) ;
#164916=CARTESIAN_POINT('Ctrl Pts',(-18.5937497675865,-12.4226010423524,
115.93296065095)) ;
#164917=CARTESIAN_POINT('Ctrl Pts',(-18.6675536349436,-12.4226010571477,
115.908729682173)) ;
#164918=CARTESIAN_POINT('Ctrl Pts',(-18.7413575023006,-12.422601071943,
115.884498713395)) ;
#164919=CARTESIAN_POINT('Ctrl Pts',(-18.7454987260867,-12.3478638522204,
115.897112211353)) ;
#164920=CARTESIAN_POINT('Ctrl Pts',(-18.7496399498727,-12.2731266324978,
115.90972570931)) ;
#164921=CARTESIAN_POINT('Ctrl Pts',(-18.6758360825156,-12.2731266177025,
115.933956678087)) ;
#164922=CARTESIAN_POINT('Ctrl Pts',(-18.6020322151586,-12.2731266029072,
115.958187646864)) ;
#164923=CARTESIAN_POINT('Ctrl Pts',(-18.5978909913726,-12.3478638226298,
115.945574148907)) ;
#164924=CARTESIAN_POINT('Ctrl Pts',(-18.6947567327243,-12.4382992209291,
116.205140753545)) ;
#164925=CARTESIAN_POINT('Ctrl Pts',(-18.6845800908453,-12.5068353759983,
116.174144345737)) ;
#164926=CARTESIAN_POINT('Ctrl Pts',(-18.7583839539381,-12.5068354072617,
116.149913363972)) ;
#164927=CARTESIAN_POINT('Ctrl Pts',(-18.832187817031,-12.5068354385251,
116.125682382207)) ;
#164928=CARTESIAN_POINT('Ctrl Pts',(-18.84236445891,-12.4382992834559,116.156678790014)) ;
#164929=CARTESIAN_POINT('Ctrl Pts',(-18.852541100789,-12.3697631283867,
116.187675197822)) ;
#164930=CARTESIAN_POINT('Ctrl Pts',(-18.7787372376961,-12.3697630971233,
116.211906179587)) ;
#164931=CARTESIAN_POINT('Ctrl Pts',(-18.7049333746032,-12.3697630658599,
116.236137161352)) ;
#164932=CARTESIAN_POINT('Ctrl Pts',(-18.6947567327243,-12.4382992209291,
116.205140753545)) ;
#164933=CARTESIAN_POINT('Ctrl Pts',(-18.7809827309636,-12.5986984925073,
116.432334829973)) ;
#164934=CARTESIAN_POINT('Ctrl Pts',(-18.7655036399242,-12.6561393028317,
116.385188017416)) ;
#164935=CARTESIAN_POINT('Ctrl Pts',(-18.8393074978484,-12.65613934453,116.360957019908)) ;
#164936=CARTESIAN_POINT('Ctrl Pts',(-18.9131113557727,-12.6561393862282,
116.3367260224)) ;
#164937=CARTESIAN_POINT('Ctrl Pts',(-18.9285904468122,-12.5986985759038,
116.383872834956)) ;
#164938=CARTESIAN_POINT('Ctrl Pts',(-18.9440695378517,-12.5412577655794,
116.431019647513)) ;
#164939=CARTESIAN_POINT('Ctrl Pts',(-18.8702656799274,-12.5412577238812,
116.455250645021)) ;
#164940=CARTESIAN_POINT('Ctrl Pts',(-18.7964618220031,-12.541257682183,
116.479481642529)) ;
#164941=CARTESIAN_POINT('Ctrl Pts',(-18.7809827309636,-12.5986984925073,
116.432334829973)) ;
#164942=CARTESIAN_POINT('Ctrl Pts',(-18.851332317076,-12.8181589219149,
116.61110894894)) ;
#164943=CARTESIAN_POINT('Ctrl Pts',(-18.831652435789,-12.8603639864266,
116.551167206913)) ;
#164944=CARTESIAN_POINT('Ctrl Pts',(-18.9054562882163,-12.8603640315663,
116.526936192662)) ;
#164945=CARTESIAN_POINT('Ctrl Pts',(-18.9792601406437,-12.8603640767059,
116.502705178411)) ;
#164946=CARTESIAN_POINT('Ctrl Pts',(-18.9989400219307,-12.8181590121942,
116.562646920439)) ;
#164947=CARTESIAN_POINT('Ctrl Pts',(-19.0186199032177,-12.7759539476825,
116.622588662466)) ;
#164948=CARTESIAN_POINT('Ctrl Pts',(-18.9448160507903,-12.7759539025429,
116.646819676717)) ;
#164949=CARTESIAN_POINT('Ctrl Pts',(-18.871012198363,-12.7759538574032,
116.671050690968)) ;
#164950=CARTESIAN_POINT('Ctrl Pts',(-18.851332317076,-12.8181589219149,
116.61110894894)) ;
#164951=CARTESIAN_POINT('Ctrl Pts',(-18.9012299138603,-13.0797516616193,
116.727706681525)) ;
#164952=CARTESIAN_POINT('Ctrl Pts',(-18.878768479364,-13.1037557901174,
116.659292777072)) ;
#164953=CARTESIAN_POINT('Ctrl Pts',(-18.9525723269898,-13.1037558337794,
116.635061748196)) ;
#164954=CARTESIAN_POINT('Ctrl Pts',(-19.0263761746156,-13.1037558774415,
116.61083071932)) ;
#164955=CARTESIAN_POINT('Ctrl Pts',(-19.0488376091119,-13.0797517489434,
116.679244623774)) ;
#164956=CARTESIAN_POINT('Ctrl Pts',(-19.0712990436082,-13.0557476204452,
116.747658528227)) ;
#164957=CARTESIAN_POINT('Ctrl Pts',(-18.9974951959824,-13.0557475767832,
116.771889557103)) ;
#164958=CARTESIAN_POINT('Ctrl Pts',(-18.9236913483566,-13.0557475331212,
116.796120585978)) ;
#164959=CARTESIAN_POINT('Ctrl Pts',(-18.9012299138603,-13.0797516616193,
116.727706681525)) ;
#164960=CARTESIAN_POINT('Ctrl Pts',(-18.9282094511315,-13.3661182947965,
116.774416487674)) ;
#164961=CARTESIAN_POINT('Ctrl Pts',(-18.9045640621688,-13.3701640997913,
116.702396448778)) ;
#164962=CARTESIAN_POINT('Ctrl Pts',(-18.9783679058639,-13.3701641367874,
116.67816540793)) ;
#164963=CARTESIAN_POINT('Ctrl Pts',(-19.0521717495589,-13.3701641737835,
116.653934367082)) ;
#164964=CARTESIAN_POINT('Ctrl Pts',(-19.0758171385217,-13.3661183687887,
116.725954405978)) ;
#164965=CARTESIAN_POINT('Ctrl Pts',(-19.0994625274844,-13.3620725637939,
116.797974444874)) ;
#164966=CARTESIAN_POINT('Ctrl Pts',(-19.0256586837894,-13.3620725267978,
116.822205485722)) ;
#164967=CARTESIAN_POINT('Ctrl Pts',(-18.9518548400943,-13.3620724898017,
116.84643652657)) ;
#164968=CARTESIAN_POINT('Ctrl Pts',(-18.9282094511315,-13.3661182947965,
116.774416487674)) ;
#164969=CARTESIAN_POINT('Ctrl Pts',(-18.9308376699889,-13.656951267572,
116.746866353868)) ;
#164970=CARTESIAN_POINT('Ctrl Pts',(-18.9077085946638,-13.6406962235438,
116.676418922825)) ;
#164971=CARTESIAN_POINT('Ctrl Pts',(-18.9815124359412,-13.6406962503813,
116.652187874613)) ;
#164972=CARTESIAN_POINT('Ctrl Pts',(-19.0553162772185,-13.6406962772189,
116.627956826401)) ;
#164973=CARTESIAN_POINT('Ctrl Pts',(-19.0784453525436,-13.6569513212471,
116.698404257444)) ;
#164974=CARTESIAN_POINT('Ctrl Pts',(-19.1015744278686,-13.6732063652754,
116.768851688486)) ;
#164975=CARTESIAN_POINT('Ctrl Pts',(-19.0277705865913,-13.6732063384378,
116.793082736698)) ;
#164976=CARTESIAN_POINT('Ctrl Pts',(-18.953966745314,-13.6732063116003,
116.81731378491)) ;
#164977=CARTESIAN_POINT('Ctrl Pts',(-18.9308376699889,-13.656951267572,
116.746866353868)) ;
#164978=CARTESIAN_POINT('Ctrl Pts',(-18.9097356138118,-13.9296721739865,
116.647159993684)) ;
#164979=CARTESIAN_POINT('Ctrl Pts',(-18.8887782207473,-13.8943500486195,
116.58332715626)) ;
#164980=CARTESIAN_POINT('Ctrl Pts',(-18.9625820610374,-13.8943500659771,
116.559096105041)) ;
#164981=CARTESIAN_POINT('Ctrl Pts',(-19.0363859013275,-13.8943500833347,
116.534865053822)) ;
#164982=CARTESIAN_POINT('Ctrl Pts',(-19.057343294392,-13.9296722087017,
116.598697891246)) ;
#164983=CARTESIAN_POINT('Ctrl Pts',(-19.0783006874565,-13.9649943340687,
116.662530728671)) ;
#164984=CARTESIAN_POINT('Ctrl Pts',(-19.0044968471664,-13.9649943167111,
116.68676177989)) ;
#164985=CARTESIAN_POINT('Ctrl Pts',(-18.9306930068763,-13.9649942993535,
116.710992831109)) ;
#164986=CARTESIAN_POINT('Ctrl Pts',(-18.9097356138118,-13.9296721739865,
116.647159993684)) ;
#164987=CARTESIAN_POINT('Ctrl Pts',(-18.867193628718,-14.1660389555352,
116.482117526194)) ;
#164988=CARTESIAN_POINT('Ctrl Pts',(-18.8499089973715,-14.1141591424512,
116.429471328224)) ;
#164989=CARTESIAN_POINT('Ctrl Pts',(-18.9237128379045,-14.114159151286,
116.405240277745)) ;
#164990=CARTESIAN_POINT('Ctrl Pts',(-18.9975166784375,-14.1141591601208,
116.381009227266)) ;
#164991=CARTESIAN_POINT('Ctrl Pts',(-19.014801309784,-14.1660389732048,
116.433655425236)) ;
#164992=CARTESIAN_POINT('Ctrl Pts',(-19.0320859411305,-14.2179187862889,
116.486301623206)) ;
#164993=CARTESIAN_POINT('Ctrl Pts',(-18.9582821005975,-14.2179187774541,
116.510532673685)) ;
#164994=CARTESIAN_POINT('Ctrl Pts',(-18.8844782600645,-14.2179187686193,
116.534763724164)) ;
#164995=CARTESIAN_POINT('Ctrl Pts',(-18.867193628718,-14.1660389555352,
116.482117526194)) ;
#164996=CARTESIAN_POINT('Ctrl Pts',(-18.8069801346924,-14.3487828478669,
116.263249434496)) ;
#164997=CARTESIAN_POINT('Ctrl Pts',(-18.7946078964765,-14.2840645582721,
116.22556559327)) ;
#164998=CARTESIAN_POINT('Ctrl Pts',(-18.8684117380704,-14.2840645612063,
116.201334546022)) ;
#164999=CARTESIAN_POINT('Ctrl Pts',(-18.9422155796643,-14.2840645641405,
116.177103498774)) ;
#165000=CARTESIAN_POINT('Ctrl Pts',(-18.9545878178802,-14.3487828537354,
116.214787340001)) ;
#165001=CARTESIAN_POINT('Ctrl Pts',(-18.9669600560961,-14.4135011433302,
116.252471181227)) ;
#165002=CARTESIAN_POINT('Ctrl Pts',(-18.8931562145022,-14.413501140396,
116.276702228475)) ;
#165003=CARTESIAN_POINT('Ctrl Pts',(-18.8193523729083,-14.4135011374618,
116.300933275723)) ;
#165004=CARTESIAN_POINT('Ctrl Pts',(-18.8069801346924,-14.3487828478669,
116.263249434496)) ;
#165005=CARTESIAN_POINT('Ctrl Pts',(-18.73423883593,-14.4648357931477,116.006250091978)) ;
#165006=CARTESIAN_POINT('Ctrl Pts',(-18.7276607481248,-14.391916747365,
115.986214297925)) ;
#165007=CARTESIAN_POINT('Ctrl Pts',(-18.8014645910197,-14.3919167474485,
115.961983254639)) ;
#165008=CARTESIAN_POINT('Ctrl Pts',(-18.8752684339146,-14.391916747532,
115.937752211354)) ;
#165009=CARTESIAN_POINT('Ctrl Pts',(-18.8818465217198,-14.4648357933146,
115.957788005407)) ;
#165010=CARTESIAN_POINT('Ctrl Pts',(-18.8884246095251,-14.5377548390973,
115.97782379946)) ;
#165011=CARTESIAN_POINT('Ctrl Pts',(-18.8146207666302,-14.5377548390138,
116.002054842746)) ;
#165012=CARTESIAN_POINT('Ctrl Pts',(-18.7408169237353,-14.5377548389303,
116.026285886031)) ;
#165013=CARTESIAN_POINT('Ctrl Pts',(-18.73423883593,-14.4648357931477,116.006250091978)) ;
#165014=CARTESIAN_POINT('Ctrl Pts',(-18.6548178924346,-14.5058959818021,
115.728874128576)) ;
#165015=CARTESIAN_POINT('Ctrl Pts',(-18.6545098781287,-14.4300007264442,
115.727935966664)) ;
#165016=CARTESIAN_POINT('Ctrl Pts',(-18.7283137220883,-14.4300007261889,
115.703704926622)) ;
#165017=CARTESIAN_POINT('Ctrl Pts',(-18.8021175660479,-14.4300007259336,
115.67947388658)) ;
#165018=CARTESIAN_POINT('Ctrl Pts',(-18.8024255803537,-14.5058959812914,
115.680412048491)) ;
#165019=CARTESIAN_POINT('Ctrl Pts',(-18.8027335946595,-14.5817912366492,
115.681350210403)) ;
#165020=CARTESIAN_POINT('Ctrl Pts',(-18.7289297506999,-14.5817912369046,
115.705581250445)) ;
#165021=CARTESIAN_POINT('Ctrl Pts',(-18.6551259067404,-14.5817912371599,
115.729812290487)) ;
#165022=CARTESIAN_POINT('Ctrl Pts',(-18.6548178924346,-14.5058959818021,
115.728874128576)) ;
#165023=CARTESIAN_POINT('Ctrl Pts',(-18.5753873202692,-14.4694242942484,
115.451559578803)) ;
#165024=CARTESIAN_POINT('Ctrl Pts',(-18.5813575551514,-14.3959630196689,
115.469743950894)) ;
#165025=CARTESIAN_POINT('Ctrl Pts',(-18.6551613996072,-14.3959630205436,
115.445512912363)) ;
#165026=CARTESIAN_POINT('Ctrl Pts',(-18.7289652440631,-14.3959630214183,
115.421281873832)) ;
#165027=CARTESIAN_POINT('Ctrl Pts',(-18.7229950091809,-14.4694242959978,
115.403097501742)) ;
#165028=CARTESIAN_POINT('Ctrl Pts',(-18.7170247742987,-14.5428855705773,
115.384913129651)) ;
#165029=CARTESIAN_POINT('Ctrl Pts',(-18.6432209298428,-14.5428855697026,
115.409144168182)) ;
#165030=CARTESIAN_POINT('Ctrl Pts',(-18.569417085387,-14.542885568828,115.433375206713)) ;
#165031=CARTESIAN_POINT('Ctrl Pts',(-18.5753873202692,-14.4694242942484,
115.451559578803)) ;
#165032=CARTESIAN_POINT('Ctrl Pts',(-18.5015763378576,-14.356381751671,
115.191027747652)) ;
#165033=CARTESIAN_POINT('Ctrl Pts',(-18.5134490185545,-14.2907051755566,
115.227190017359)) ;
#165034=CARTESIAN_POINT('Ctrl Pts',(-18.5872528625669,-14.2907051768879,
115.202958977478)) ;
#165035=CARTESIAN_POINT('Ctrl Pts',(-18.6610567065792,-14.2907051782191,
115.178727937596)) ;
#165036=CARTESIAN_POINT('Ctrl Pts',(-18.6491840258824,-14.3563817543336,
115.142565667889)) ;
#165037=CARTESIAN_POINT('Ctrl Pts',(-18.6373113451855,-14.422058330448,
115.106403398181)) ;
#165038=CARTESIAN_POINT('Ctrl Pts',(-18.5635075011732,-14.4220583291168,
115.130634438063)) ;
#165039=CARTESIAN_POINT('Ctrl Pts',(-18.4897036571608,-14.4220583277855,
115.154865477944)) ;
#165040=CARTESIAN_POINT('Ctrl Pts',(-18.5015763378576,-14.356381751671,
115.191027747652)) ;
#165041=CARTESIAN_POINT('Ctrl Pts',(-18.4409491774712,-14.1778422798436,
114.971114813848)) ;
#165042=CARTESIAN_POINT('Ctrl Pts',(-18.4578020115765,-14.1245364286659,
115.022445827339)) ;
#165043=CARTESIAN_POINT('Ctrl Pts',(-18.5316058549156,-14.1245364288381,
114.998214785407)) ;
#165044=CARTESIAN_POINT('Ctrl Pts',(-18.6054096982547,-14.1245364290103,
114.973983743475)) ;
#165045=CARTESIAN_POINT('Ctrl Pts',(-18.5885568641494,-14.177842280188,
114.922652729984)) ;
#165046=CARTESIAN_POINT('Ctrl Pts',(-18.5717040300441,-14.2311481313656,
114.871321716493)) ;
#165047=CARTESIAN_POINT('Ctrl Pts',(-18.497900186705,-14.2311481311934,
114.895552758425)) ;
#165048=CARTESIAN_POINT('Ctrl Pts',(-18.4240963433659,-14.2311481310212,
114.919783800358)) ;
#165049=CARTESIAN_POINT('Ctrl Pts',(-18.4409491774712,-14.1778422798436,
114.971114813848)) ;
#165050=CARTESIAN_POINT('Ctrl Pts',(-18.3972234500987,-13.9441247450056,
114.802451129126)) ;
#165051=CARTESIAN_POINT('Ctrl Pts',(-18.4178884384501,-13.9070603957443,
114.865393349445)) ;
#165052=CARTESIAN_POINT('Ctrl Pts',(-18.4916922810686,-13.9070603921811,
114.841162305317)) ;
#165053=CARTESIAN_POINT('Ctrl Pts',(-18.565496123687,-13.9070603886178,
114.81693126119)) ;
#165054=CARTESIAN_POINT('Ctrl Pts',(-18.5448311353355,-13.9441247378791,
114.753989040871)) ;
#165055=CARTESIAN_POINT('Ctrl Pts',(-18.524166146984,-13.9811890871404,
114.691046820552)) ;
#165056=CARTESIAN_POINT('Ctrl Pts',(-18.4503623043656,-13.9811890907036,
114.71527786468)) ;
#165057=CARTESIAN_POINT('Ctrl Pts',(-18.3765584617472,-13.9811890942669,
114.739508908807)) ;
#165058=CARTESIAN_POINT('Ctrl Pts',(-18.3972234500987,-13.9441247450056,
114.802451129126)) ;
#165059=CARTESIAN_POINT('Ctrl Pts',(-18.374886126082,-13.6724643503177,
114.698927689739)) ;
#165060=CARTESIAN_POINT('Ctrl Pts',(-18.3978753151959,-13.6543146170461,
114.768949050689)) ;
#165061=CARTESIAN_POINT('Ctrl Pts',(-18.4716791577005,-13.6543146070783,
114.744718006215)) ;
#165062=CARTESIAN_POINT('Ctrl Pts',(-18.545483000205,-13.6543145971105,
114.720486961741)) ;
#165063=CARTESIAN_POINT('Ctrl Pts',(-18.5224938110911,-13.6724643303821,
114.650465600791)) ;
#165064=CARTESIAN_POINT('Ctrl Pts',(-18.4995046219771,-13.6906140636538,
114.580444239841)) ;
#165065=CARTESIAN_POINT('Ctrl Pts',(-18.4257007794726,-13.6906140736215,
114.604675284315)) ;
#165066=CARTESIAN_POINT('Ctrl Pts',(-18.3518969369681,-13.6906140835893,
114.628906328789)) ;
#165067=CARTESIAN_POINT('Ctrl Pts',(-18.374886126082,-13.6724643503177,
114.698927689739)) ;
#165068=CARTESIAN_POINT('Ctrl Pts',(-18.3760656718454,-13.3835337156027,
114.66714876584)) ;
#165069=CARTESIAN_POINT('Ctrl Pts',(-18.3997377752189,-13.3855315872837,
114.739250173553)) ;
#165070=CARTESIAN_POINT('Ctrl Pts',(-18.4735416185495,-13.3855315707962,
114.715019131595)) ;
#165071=CARTESIAN_POINT('Ctrl Pts',(-18.54734546188,-13.3855315543086,114.690788089637)) ;
#165072=CARTESIAN_POINT('Ctrl Pts',(-18.5236733585065,-13.3835336826277,
114.618686681923)) ;
#165073=CARTESIAN_POINT('Ctrl Pts',(-18.500001255133,-13.3815358109467,
114.546585274209)) ;
#165074=CARTESIAN_POINT('Ctrl Pts',(-18.4261974118024,-13.3815358274342,
114.570816316167)) ;
#165075=CARTESIAN_POINT('Ctrl Pts',(-18.3523935684719,-13.3815358439218,
114.595047358126)) ;
#165076=CARTESIAN_POINT('Ctrl Pts',(-18.3760656718454,-13.3835337156027,
114.66714876584)) ;
#165077=CARTESIAN_POINT('Ctrl Pts',(-18.401893543203,-13.0942320536069,
114.710077646052)) ;
#165078=CARTESIAN_POINT('Ctrl Pts',(-18.4245363854837,-13.1164328568091,
114.779044090745)) ;
#165079=CARTESIAN_POINT('Ctrl Pts',(-18.4983402311482,-13.1164328311838,
114.754813055896)) ;
#165080=CARTESIAN_POINT('Ctrl Pts',(-18.5721440768125,-13.1164328055585,
114.730582021046)) ;
#165081=CARTESIAN_POINT('Ctrl Pts',(-18.5495012345318,-13.0942320023563,
114.661615576353)) ;
#165082=CARTESIAN_POINT('Ctrl Pts',(-18.526858392251,-13.0720311991542,
114.592649131659)) ;
#165083=CARTESIAN_POINT('Ctrl Pts',(-18.4530545465866,-13.0720312247795,
114.616880166509)) ;
#165084=CARTESIAN_POINT('Ctrl Pts',(-18.3792507009222,-13.0720312504048,
114.641111201359)) ;
#165085=CARTESIAN_POINT('Ctrl Pts',(-18.401893543203,-13.0942320536069,
114.710077646052)) ;
#165086=CARTESIAN_POINT('Ctrl Pts',(-18.4504581445536,-12.8318300831267,
114.822750132505)) ;
#165087=CARTESIAN_POINT('Ctrl Pts',(-18.4704721032377,-12.8723837829672,
114.883709422054)) ;
#165088=CARTESIAN_POINT('Ctrl Pts',(-18.544275952011,-12.8723837548031,
114.859478396673)) ;
#165089=CARTESIAN_POINT('Ctrl Pts',(-18.6180798007842,-12.872383726639,
114.835247371292)) ;
#165090=CARTESIAN_POINT('Ctrl Pts',(-18.5980658421001,-12.8318300267985,
114.774288081744)) ;
#165091=CARTESIAN_POINT('Ctrl Pts',(-18.578051883416,-12.791276326958,114.713328792195)) ;
#165092=CARTESIAN_POINT('Ctrl Pts',(-18.5042480346428,-12.7912763551221,
114.737559817576)) ;
#165093=CARTESIAN_POINT('Ctrl Pts',(-18.4304441858696,-12.7912763832862,
114.761790842957)) ;
#165094=CARTESIAN_POINT('Ctrl Pts',(-18.4504581445536,-12.8318300831267,
114.822750132505)) ;
#165095=CARTESIAN_POINT('Ctrl Pts',(-18.5199862768258,-12.608937228869,
114.9989168848)) ;
#165096=CARTESIAN_POINT('Ctrl Pts',(-18.5359115586374,-12.6651122393528,
115.047422724493)) ;
#165097=CARTESIAN_POINT('Ctrl Pts',(-18.6097154118356,-12.6651122100812,
115.02319171259)) ;
#165098=CARTESIAN_POINT('Ctrl Pts',(-18.6835192650338,-12.6651121808096,
114.998960700687)) ;
#165099=CARTESIAN_POINT('Ctrl Pts',(-18.6675939832222,-12.6089371703258,
114.950454860994)) ;
#165100=CARTESIAN_POINT('Ctrl Pts',(-18.6516687014106,-12.5527621598419,
114.901949021301)) ;
#165101=CARTESIAN_POINT('Ctrl Pts',(-18.5778648482124,-12.5527621891136,
114.926180033204)) ;
#165102=CARTESIAN_POINT('Ctrl Pts',(-18.5040609950142,-12.5527622183852,
114.950411045107)) ;
#165103=CARTESIAN_POINT('Ctrl Pts',(-18.5199862768258,-12.608937228869,
114.9989168848)) ;
#165104=CARTESIAN_POINT('Ctrl Pts',(-18.6052024537699,-12.4456165862493,
115.223155293183)) ;
#165105=CARTESIAN_POINT('Ctrl Pts',(-18.6159317015771,-12.5132753292444,
115.255834851816)) ;
#165106=CARTESIAN_POINT('Ctrl Pts',(-18.6897355588925,-12.5132753061601,
115.231603852453)) ;
#165107=CARTESIAN_POINT('Ctrl Pts',(-18.7635394162079,-12.5132752830759,
115.207372853091)) ;
#165108=CARTESIAN_POINT('Ctrl Pts',(-18.7528101684007,-12.4456165400809,
115.174693294458)) ;
#165109=CARTESIAN_POINT('Ctrl Pts',(-18.7420809205935,-12.3779577970859,
115.142013735824)) ;
#165110=CARTESIAN_POINT('Ctrl Pts',(-18.6682770632781,-12.3779578201701,
115.166244735187)) ;
#165111=CARTESIAN_POINT('Ctrl Pts',(-18.5944732059627,-12.3779578432543,
115.19047573455)) ;
#165112=CARTESIAN_POINT('Ctrl Pts',(-18.6052024537699,-12.4456165862493,
115.223155293183)) ;
#165113=CARTESIAN_POINT('Ctrl Pts',(-18.7017273999509,-12.3507741827119,
115.481643821493)) ;
#165114=CARTESIAN_POINT('Ctrl Pts',(-18.7064677514607,-12.4251525805178,
115.496082168485)) ;
#165115=CARTESIAN_POINT('Ctrl Pts',(-18.7802716129605,-12.425152568096,
115.471851181868)) ;
#165116=CARTESIAN_POINT('Ctrl Pts',(-18.8540754744602,-12.4251525556743,
115.44762019525)) ;
#165117=CARTESIAN_POINT('Ctrl Pts',(-18.8493351229504,-12.3507741578684,
115.433181848258)) ;
#165118=CARTESIAN_POINT('Ctrl Pts',(-18.8445947714406,-12.2763957600624,
115.418743501266)) ;
#165119=CARTESIAN_POINT('Ctrl Pts',(-18.7707909099408,-12.2763957724842,
115.442974487884)) ;
#165120=CARTESIAN_POINT('Ctrl Pts',(-18.696987048441,-12.276395784906,115.467205474501)) ;
#165121=CARTESIAN_POINT('Ctrl Pts',(-18.7017273999509,-12.3507741827119,
115.481643821493)) ;
#165122=CARTESIAN_POINT('Ctrl Pts',(-18.8032672046633,-12.3329811601702,
115.755325050277)) ;
#165123=CARTESIAN_POINT('Ctrl Pts',(-18.8016616113288,-12.4087098331506,
115.750434673372)) ;
#165124=CARTESIAN_POINT('Ctrl Pts',(-18.8754654761557,-12.4087098375423,
115.726203696888)) ;
#165125=CARTESIAN_POINT('Ctrl Pts',(-18.9492693409827,-12.408709841934,
115.701972720404)) ;
#165126=CARTESIAN_POINT('Ctrl Pts',(-18.9508749343172,-12.3329811689535,
115.70686309731)) ;
#165127=CARTESIAN_POINT('Ctrl Pts',(-18.9524805276516,-12.2572524959731,
115.711753474215)) ;
#165128=CARTESIAN_POINT('Ctrl Pts',(-18.8786766628248,-12.2572524915815,
115.735984450699)) ;
#165129=CARTESIAN_POINT('Ctrl Pts',(-18.8048727979978,-12.2572524871898,
115.760215427183)) ;
#165130=CARTESIAN_POINT('Ctrl Pts',(-18.8032672046633,-12.3329811601702,
115.755325050277)) ;
#165131=CARTESIAN_POINT('Ctrl Pts',(-18.9021329558298,-12.3924859215409,
116.021180417224)) ;
#165132=CARTESIAN_POINT('Ctrl Pts',(-18.8943523561467,-12.4641691937461,
115.997481967433)) ;
#165133=CARTESIAN_POINT('Ctrl Pts',(-18.9681562216487,-12.4641692182498,
115.973250993006)) ;
#165134=CARTESIAN_POINT('Ctrl Pts',(-19.0419600871508,-12.4641692427536,
115.949020018578)) ;
#165135=CARTESIAN_POINT('Ctrl Pts',(-19.0497406868339,-12.3924859705485,
115.97271846837)) ;
#165136=CARTESIAN_POINT('Ctrl Pts',(-19.057521286517,-12.3208026983433,
115.996416918161)) ;
#165137=CARTESIAN_POINT('Ctrl Pts',(-18.983717421015,-12.3208026738395,
116.020647892588)) ;
#165138=CARTESIAN_POINT('Ctrl Pts',(-18.9099135555129,-12.3208026493358,
116.044878867016)) ;
#165139=CARTESIAN_POINT('Ctrl Pts',(-18.9021329558298,-12.3924859215409,
116.021180417224)) ;
#165140=CARTESIAN_POINT('Ctrl Pts',(-18.9935434523282,-12.5254680767671,
116.264107206113)) ;
#165141=CARTESIAN_POINT('Ctrl Pts',(-18.9801040226674,-12.5879710242858,
116.223172873407)) ;
#165142=CARTESIAN_POINT('Ctrl Pts',(-19.0539078873367,-12.587971070974,
116.198941896443)) ;
#165143=CARTESIAN_POINT('Ctrl Pts',(-19.127711752006,-12.5879711176621,
116.174710919479)) ;
#165144=CARTESIAN_POINT('Ctrl Pts',(-19.1411511816667,-12.5254681701434,
116.215645252185)) ;
#165145=CARTESIAN_POINT('Ctrl Pts',(-19.1545906113275,-12.4629652226247,
116.256579584891)) ;
#165146=CARTESIAN_POINT('Ctrl Pts',(-19.0807867466582,-12.4629651759366,
116.280810561855)) ;
#165147=CARTESIAN_POINT('Ctrl Pts',(-19.006982881989,-12.4629651292484,
116.305041538819)) ;
#165148=CARTESIAN_POINT('Ctrl Pts',(-18.9935434523282,-12.5254680767671,
116.264107206113)) ;
#165149=CARTESIAN_POINT('Ctrl Pts',(-19.0711087442326,-12.7232333026618,
116.464791322547)) ;
#165150=CARTESIAN_POINT('Ctrl Pts',(-19.0529703146369,-12.7720201100749,
116.409544594361)) ;
#165151=CARTESIAN_POINT('Ctrl Pts',(-19.1267741760621,-12.7720201789256,
116.385313607516)) ;
#165152=CARTESIAN_POINT('Ctrl Pts',(-19.2005780374873,-12.7720202477763,
116.361082620671)) ;
#165153=CARTESIAN_POINT('Ctrl Pts',(-19.218716467083,-12.7232334403633,
116.416329348858)) ;
#165154=CARTESIAN_POINT('Ctrl Pts',(-19.2368548966787,-12.6744466329502,
116.471576077045)) ;
#165155=CARTESIAN_POINT('Ctrl Pts',(-19.1630510352535,-12.6744465640995,
116.49580706389)) ;
#165156=CARTESIAN_POINT('Ctrl Pts',(-19.0892471738283,-12.6744464952487,
116.520038050734)) ;
#165157=CARTESIAN_POINT('Ctrl Pts',(-19.0711087442326,-12.7232333026618,
116.464791322547)) ;
#165158=CARTESIAN_POINT('Ctrl Pts',(-19.1295684502511,-12.9691613747719,
116.607520966914)) ;
#165159=CARTESIAN_POINT('Ctrl Pts',(-19.1080532454145,-13.0008491150667,
116.541989126278)) ;
#165160=CARTESIAN_POINT('Ctrl Pts',(-19.1818571011284,-13.0008492011903,
116.517758122037)) ;
#165161=CARTESIAN_POINT('Ctrl Pts',(-19.2556609568422,-13.0008492873139,
116.493527117796)) ;
#165162=CARTESIAN_POINT('Ctrl Pts',(-19.2771761616788,-12.9691615470191,
116.559058958432)) ;
#165163=CARTESIAN_POINT('Ctrl Pts',(-19.2986913665153,-12.9374738067243,
116.624590799068)) ;
#165164=CARTESIAN_POINT('Ctrl Pts',(-19.2248875108014,-12.9374737206007,
116.648821803309)) ;
#165165=CARTESIAN_POINT('Ctrl Pts',(-19.1510836550876,-12.937473634477,
116.673052807549)) ;
#165166=CARTESIAN_POINT('Ctrl Pts',(-19.1295684502511,-12.9691613747719,
116.607520966914)) ;
#165167=CARTESIAN_POINT('Ctrl Pts',(-19.1662325928152,-13.2488218748192,
116.683635238154)) ;
#165168=CARTESIAN_POINT('Ctrl Pts',(-19.142861896445,-13.2610313034061,
116.612451869792)) ;
#165169=CARTESIAN_POINT('Ctrl Pts',(-19.2166657448267,-13.2610314022195,
116.588220843219)) ;
#165170=CARTESIAN_POINT('Ctrl Pts',(-19.2904695932085,-13.2610315010329,
116.563989816646)) ;
#165171=CARTESIAN_POINT('Ctrl Pts',(-19.3138402895787,-13.248822072446,
116.635173185008)) ;
#165172=CARTESIAN_POINT('Ctrl Pts',(-19.337210985949,-13.2366126438591,
116.706356553369)) ;
#165173=CARTESIAN_POINT('Ctrl Pts',(-19.2634071375672,-13.2366125450457,
116.730587579942)) ;
#165174=CARTESIAN_POINT('Ctrl Pts',(-19.1896032891855,-13.2366124462323,
116.754818606515)) ;
#165175=CARTESIAN_POINT('Ctrl Pts',(-19.1662325928152,-13.2488218748192,
116.683635238154)) ;
#165176=CARTESIAN_POINT('Ctrl Pts',(-19.1787171382524,-13.5399745855604,
116.686196204897)) ;
#165177=CARTESIAN_POINT('Ctrl Pts',(-19.1551743858641,-13.5318747593251,
116.614488781738)) ;
#165178=CARTESIAN_POINT('Ctrl Pts',(-19.2289782257133,-13.5318748625201,
116.590257729176)) ;
#165179=CARTESIAN_POINT('Ctrl Pts',(-19.3027820655625,-13.5318749657152,
116.566026676614)) ;
#165180=CARTESIAN_POINT('Ctrl Pts',(-19.3263248179508,-13.5399747919505,
116.637734099773)) ;
#165181=CARTESIAN_POINT('Ctrl Pts',(-19.349867570339,-13.5480746181859,
116.709441522932)) ;
#165182=CARTESIAN_POINT('Ctrl Pts',(-19.2760637304898,-13.5480745149908,
116.733672575494)) ;
#165183=CARTESIAN_POINT('Ctrl Pts',(-19.2022598906406,-13.5480744117958,
116.757903628056)) ;
#165184=CARTESIAN_POINT('Ctrl Pts',(-19.1787171382524,-13.5399745855604,
116.686196204897)) ;
#165185=CARTESIAN_POINT('Ctrl Pts',(-19.1670328317494,-13.8224630035439,
116.615122093039)) ;
#165186=CARTESIAN_POINT('Ctrl Pts',(-19.1450054514804,-13.7946290334854,
116.548030248902)) ;
#165187=CARTESIAN_POINT('Ctrl Pts',(-19.2188092825817,-13.7946291324029,
116.523799169696)) ;
#165188=CARTESIAN_POINT('Ctrl Pts',(-19.2926131136831,-13.7946292313203,
116.49956809049)) ;
#165189=CARTESIAN_POINT('Ctrl Pts',(-19.3146404939522,-13.8224632013788,
116.566659934627)) ;
#165190=CARTESIAN_POINT('Ctrl Pts',(-19.3366678742212,-13.8502971714373,
116.633751778763)) ;
#165191=CARTESIAN_POINT('Ctrl Pts',(-19.2628640431198,-13.8502970725198,
116.657982857969)) ;
#165192=CARTESIAN_POINT('Ctrl Pts',(-19.1890602120184,-13.8502969736024,
116.682213937175)) ;
#165193=CARTESIAN_POINT('Ctrl Pts',(-19.1670328317494,-13.8224630035439,
116.615122093039)) ;
#165194=CARTESIAN_POINT('Ctrl Pts',(-19.1329061805287,-14.0755037719121,
116.475781142016)) ;
#165195=CARTESIAN_POINT('Ctrl Pts',(-19.1139613863318,-14.0299625115252,
116.418078357712)) ;
#165196=CARTESIAN_POINT('Ctrl Pts',(-19.1877652093854,-14.0299625976229,
116.393847253993)) ;
#165197=CARTESIAN_POINT('Ctrl Pts',(-19.2615690324389,-14.0299626837205,
116.369616150274)) ;
#165198=CARTESIAN_POINT('Ctrl Pts',(-19.2805138266358,-14.0755039441074,
116.427318934579)) ;
#165199=CARTESIAN_POINT('Ctrl Pts',(-19.2994586208326,-14.1210452044942,
116.485021718884)) ;
#165200=CARTESIAN_POINT('Ctrl Pts',(-19.2256547977791,-14.1210451183966,
116.509252822602)) ;
#165201=CARTESIAN_POINT('Ctrl Pts',(-19.1518509747255,-14.121045032299,
116.533483926321)) ;
#165202=CARTESIAN_POINT('Ctrl Pts',(-19.1329061805287,-14.0755037719121,
116.475781142016)) ;
#165203=CARTESIAN_POINT('Ctrl Pts',(-19.0790275217248,-14.2826234653696,
116.276041341228)) ;
#165204=CARTESIAN_POINT('Ctrl Pts',(-19.0645534585991,-14.2225542775354,
116.231955682423)) ;
#165205=CARTESIAN_POINT('Ctrl Pts',(-19.1383572751289,-14.2225543432862,
116.207724558834)) ;
#165206=CARTESIAN_POINT('Ctrl Pts',(-19.2121610916587,-14.222554409037,
116.183493435246)) ;
#165207=CARTESIAN_POINT('Ctrl Pts',(-19.2266351547843,-14.2826235968712,
116.22757909405)) ;
#165208=CARTESIAN_POINT('Ctrl Pts',(-19.24110921791,-14.3426927847054,116.271664752854)) ;
#165209=CARTESIAN_POINT('Ctrl Pts',(-19.1673054013802,-14.3426927189546,
116.295895876443)) ;
#165210=CARTESIAN_POINT('Ctrl Pts',(-19.0935015848505,-14.3426926532038,
116.320127000032)) ;
#165211=CARTESIAN_POINT('Ctrl Pts',(-19.0790275217248,-14.2826234653696,
116.276041341228)) ;
#165212=CARTESIAN_POINT('Ctrl Pts',(-19.0110858794714,-14.4260980932151,
116.033863734951)) ;
#165213=CARTESIAN_POINT('Ctrl Pts',(-19.0020631113687,-14.3559233104312,
116.006381841212)) ;
#165214=CARTESIAN_POINT('Ctrl Pts',(-19.0758669235952,-14.3559233508218,
115.982150704516)) ;
#165215=CARTESIAN_POINT('Ctrl Pts',(-19.1496707358216,-14.3559233912124,
115.95791956782)) ;
#165216=CARTESIAN_POINT('Ctrl Pts',(-19.1586935039242,-14.4260981739963,
115.985401461558)) ;
#165217=CARTESIAN_POINT('Ctrl Pts',(-19.1677162720268,-14.4962729567803,
116.012883355297)) ;
#165218=CARTESIAN_POINT('Ctrl Pts',(-19.0939124598004,-14.4962729163896,
116.037114491993)) ;
#165219=CARTESIAN_POINT('Ctrl Pts',(-19.020108647574,-14.496272875999,116.061345628689)) ;
#165220=CARTESIAN_POINT('Ctrl Pts',(-19.0110858794714,-14.4260980932151,
116.033863734951)) ;
#165221=CARTESIAN_POINT('Ctrl Pts',(-18.9333061628567,-14.4987580687002,
115.761347729046)) ;
#165222=CARTESIAN_POINT('Ctrl Pts',(-18.9304370258749,-14.4234055963817,
115.752608802777)) ;
#165223=CARTESIAN_POINT('Ctrl Pts',(-19.0042408365051,-14.423405608344,
115.728377661219)) ;
#165224=CARTESIAN_POINT('Ctrl Pts',(-19.0780446471354,-14.4234056203062,
115.704146519661)) ;
#165225=CARTESIAN_POINT('Ctrl Pts',(-19.0809137841172,-14.4987580926247,
115.71288544593)) ;
#165226=CARTESIAN_POINT('Ctrl Pts',(-19.083782921099,-14.5741105649432,
115.721624372199)) ;
#165227=CARTESIAN_POINT('Ctrl Pts',(-19.0099791104687,-14.5741105529809,
115.745855513757)) ;
#165228=CARTESIAN_POINT('Ctrl Pts',(-18.9361752998385,-14.5741105410186,
115.770086655315)) ;
#165229=CARTESIAN_POINT('Ctrl Pts',(-18.9333061628567,-14.4987580687002,
115.761347729046)) ;
#165230=CARTESIAN_POINT('Ctrl Pts',(-18.8531245622656,-14.4933400096758,
115.481718981289)) ;
#165231=CARTESIAN_POINT('Ctrl Pts',(-18.8565818821195,-14.4182534186233,
115.492249421715)) ;
#165232=CARTESIAN_POINT('Ctrl Pts',(-18.930385693833,-14.4182534027344,
115.468018283457)) ;
#165233=CARTESIAN_POINT('Ctrl Pts',(-19.0041895055465,-14.4182533868454,
115.443787145198)) ;
#165234=CARTESIAN_POINT('Ctrl Pts',(-19.0007321856926,-14.493339977898,
115.433256704772)) ;
#165235=CARTESIAN_POINT('Ctrl Pts',(-18.9972748658387,-14.5684265689505,
115.422726264346)) ;
#165236=CARTESIAN_POINT('Ctrl Pts',(-18.9234710541252,-14.5684265848394,
115.446957402605)) ;
#165237=CARTESIAN_POINT('Ctrl Pts',(-18.8496672424117,-14.5684266007284,
115.471188540863)) ;
#165238=CARTESIAN_POINT('Ctrl Pts',(-18.8531245622656,-14.4933400096758,
115.481718981289)) ;
#165239=CARTESIAN_POINT('Ctrl Pts',(-18.7765257054284,-14.4113489345642,
115.212967154144)) ;
#165240=CARTESIAN_POINT('Ctrl Pts',(-18.7860695067199,-14.3418743538158,
115.242036034905)) ;
#165241=CARTESIAN_POINT('Ctrl Pts',(-18.8598733219957,-14.3418743129385,
115.217804907497)) ;
#165242=CARTESIAN_POINT('Ctrl Pts',(-18.9336771372715,-14.3418742720612,
115.193573780088)) ;
#165243=CARTESIAN_POINT('Ctrl Pts',(-18.9241333359799,-14.4113488528096,
115.164504899327)) ;
#165244=CARTESIAN_POINT('Ctrl Pts',(-18.9145895346884,-14.4808234335579,
115.135436018566)) ;
#165245=CARTESIAN_POINT('Ctrl Pts',(-18.8407857194126,-14.4808234744352,
115.159667145975)) ;
#165246=CARTESIAN_POINT('Ctrl Pts',(-18.7669819041369,-14.4808235153125,
115.183898273383)) ;
#165247=CARTESIAN_POINT('Ctrl Pts',(-18.7765257054284,-14.4113489345642,
115.212967154144)) ;
#165248=CARTESIAN_POINT('Ctrl Pts',(-18.709586077983,-14.2570982982162,
114.973460633558)) ;
#165249=CARTESIAN_POINT('Ctrl Pts',(-18.7245548673285,-14.1982882942638,
115.019053152496)) ;
#165250=CARTESIAN_POINT('Ctrl Pts',(-18.798358688464,-14.1982882346942,
114.994822042935)) ;
#165251=CARTESIAN_POINT('Ctrl Pts',(-18.8721625095994,-14.1982881751247,
114.970590933375)) ;
#165252=CARTESIAN_POINT('Ctrl Pts',(-18.8571937202539,-14.2570981790771,
114.924998414437)) ;
#165253=CARTESIAN_POINT('Ctrl Pts',(-18.8422249309084,-14.3159081830295,
114.879405895499)) ;
#165254=CARTESIAN_POINT('Ctrl Pts',(-18.768421109773,-14.3159082425991,
114.903637005059)) ;
#165255=CARTESIAN_POINT('Ctrl Pts',(-18.6946172886376,-14.3159083021687,
114.92786811462)) ;
#165256=CARTESIAN_POINT('Ctrl Pts',(-18.709586077983,-14.2570982982162,
114.973460633558)) ;
#165257=CARTESIAN_POINT('Ctrl Pts',(-18.6586281342935,-14.044633200838,
114.782977159409)) ;
#165258=CARTESIAN_POINT('Ctrl Pts',(-18.6779070569103,-14.000569128791,
114.841697648763)) ;
#165259=CARTESIAN_POINT('Ctrl Pts',(-18.7517108846106,-14.0005690563028,
114.817466559198)) ;
#165260=CARTESIAN_POINT('Ctrl Pts',(-18.8255147123109,-14.0005689838146,
114.793235469633)) ;
#165261=CARTESIAN_POINT('Ctrl Pts',(-18.8062357896941,-14.0446330558616,
114.734514980278)) ;
#165262=CARTESIAN_POINT('Ctrl Pts',(-18.7869568670774,-14.0886971279086,
114.675794490924)) ;
#165263=CARTESIAN_POINT('Ctrl Pts',(-18.713153039377,-14.0886972003968,
114.700025580489)) ;
#165264=CARTESIAN_POINT('Ctrl Pts',(-18.6393492116767,-14.088697272885,
114.724256670054)) ;
#165265=CARTESIAN_POINT('Ctrl Pts',(-18.6586281342935,-14.044633200838,
114.782977159409)) ;
#165266=CARTESIAN_POINT('Ctrl Pts',(-18.6271547830504,-13.785410087343,
114.651525939314)) ;
#165267=CARTESIAN_POINT('Ctrl Pts',(-18.6493967146293,-13.7593778661625,
114.719271275738)) ;
#165268=CARTESIAN_POINT('Ctrl Pts',(-18.7232005497368,-13.7593777900464,
114.695040208734)) ;
#165269=CARTESIAN_POINT('Ctrl Pts',(-18.7970043848443,-13.7593777139303,
114.67080914173)) ;
#165270=CARTESIAN_POINT('Ctrl Pts',(-18.7747624532654,-13.7854099351107,
114.603063805305)) ;
#165271=CARTESIAN_POINT('Ctrl Pts',(-18.7525205216865,-13.8114421562912,
114.535318468881)) ;
#165272=CARTESIAN_POINT('Ctrl Pts',(-18.678716686579,-13.8114422324073,
114.559549535885)) ;
#165273=CARTESIAN_POINT('Ctrl Pts',(-18.6049128514715,-13.8114423085234,
114.583780602889)) ;
#165274=CARTESIAN_POINT('Ctrl Pts',(-18.6271547830504,-13.785410087343,
114.651525939314)) ;
#165275=CARTESIAN_POINT('Ctrl Pts',(-18.6186793550776,-13.5013707464361,
114.590343252288)) ;
#165276=CARTESIAN_POINT('Ctrl Pts',(-18.6422784319961,-13.4951307017579,
114.662222234314)) ;
#165277=CARTESIAN_POINT('Ctrl Pts',(-18.7160822738892,-13.4951306279953,
114.637991187977)) ;
#165278=CARTESIAN_POINT('Ctrl Pts',(-18.7898861157823,-13.4951305542326,
114.613760141641)) ;
#165279=CARTESIAN_POINT('Ctrl Pts',(-18.7662870388639,-13.5013705989108,
114.541881159615)) ;
#165280=CARTESIAN_POINT('Ctrl Pts',(-18.7426879619454,-13.507610643589,
114.470002177589)) ;
#165281=CARTESIAN_POINT('Ctrl Pts',(-18.6688841200523,-13.5076107173517,
114.494233223926)) ;
#165282=CARTESIAN_POINT('Ctrl Pts',(-18.5950802781592,-13.5076107911143,
114.518464270262)) ;
#165283=CARTESIAN_POINT('Ctrl Pts',(-18.6186793550776,-13.5013707464361,
114.590343252288)) ;
#165284=CARTESIAN_POINT('Ctrl Pts',(-18.6346005883907,-13.209135818783,
114.60317395719)) ;
#165285=CARTESIAN_POINT('Ctrl Pts',(-18.657861930824,-13.2232901390273,
114.674024254277)) ;
#165286=CARTESIAN_POINT('Ctrl Pts',(-18.7316657782842,-13.2232900762476,
114.649793224897)) ;
#165287=CARTESIAN_POINT('Ctrl Pts',(-18.8054696257443,-13.2232900134679,
114.625562195517)) ;
#165288=CARTESIAN_POINT('Ctrl Pts',(-18.7822082833109,-13.2091356932237,
114.55471189843)) ;
#165289=CARTESIAN_POINT('Ctrl Pts',(-18.7589469408775,-13.1949813729794,
114.483861601343)) ;
#165290=CARTESIAN_POINT('Ctrl Pts',(-18.6851430934174,-13.1949814357591,
114.508092630724)) ;
#165291=CARTESIAN_POINT('Ctrl Pts',(-18.6113392459573,-13.1949814985388,
114.532323660104)) ;
#165292=CARTESIAN_POINT('Ctrl Pts',(-18.6346005883907,-13.209135818783,
114.60317395719)) ;
#165293=CARTESIAN_POINT('Ctrl Pts',(-18.6739150075071,-12.935507537228,
114.68774371454)) ;
#165294=CARTESIAN_POINT('Ctrl Pts',(-18.6951942663002,-12.9687880563088,
114.752556904557)) ;
#165295=CARTESIAN_POINT('Ctrl Pts',(-18.7689981179826,-12.9687880043352,
114.728325888037)) ;
#165296=CARTESIAN_POINT('Ctrl Pts',(-18.842801969665,-12.9687879523617,
114.704094871517)) ;
#165297=CARTESIAN_POINT('Ctrl Pts',(-18.8215227108719,-12.9355074332809,
114.639281681501)) ;
#165298=CARTESIAN_POINT('Ctrl Pts',(-18.8002434520789,-12.9022269142001,
114.574468491484)) ;
#165299=CARTESIAN_POINT('Ctrl Pts',(-18.7264396003964,-12.9022269661736,
114.598699508004)) ;
#165300=CARTESIAN_POINT('Ctrl Pts',(-18.652635748714,-12.9022270181472,
114.622930524524)) ;
#165301=CARTESIAN_POINT('Ctrl Pts',(-18.6739150075071,-12.935507537228,
114.68774371454)) ;
#165302=CARTESIAN_POINT('Ctrl Pts',(-18.7355531362002,-12.6930981261278,
114.839845302761)) ;
#165303=CARTESIAN_POINT('Ctrl Pts',(-18.7532986257394,-12.7433547054021,
114.893895201602)) ;
#165304=CARTESIAN_POINT('Ctrl Pts',(-18.8271024793354,-12.7433546700873,
114.869664190911)) ;
#165305=CARTESIAN_POINT('Ctrl Pts',(-18.9009063329314,-12.7433546347726,
114.845433180219)) ;
#165306=CARTESIAN_POINT('Ctrl Pts',(-18.8831608433922,-12.6930980554983,
114.791383281379)) ;
#165307=CARTESIAN_POINT('Ctrl Pts',(-18.865415353853,-12.642841476224,114.737333382538)) ;
#165308=CARTESIAN_POINT('Ctrl Pts',(-18.791611500257,-12.6428415115388,
114.761564393229)) ;
#165309=CARTESIAN_POINT('Ctrl Pts',(-18.7178076466611,-12.6428415468535,
114.78579540392)) ;
#165310=CARTESIAN_POINT('Ctrl Pts',(-18.7355531362002,-12.6930981261278,
114.839845302761)) ;
#165311=CARTESIAN_POINT('Ctrl Pts',(-18.8147640138156,-12.5044954568888,
115.045790079313)) ;
#165312=CARTESIAN_POINT('Ctrl Pts',(-18.8277365331886,-12.5679966014652,
115.085302281002)) ;
#165313=CARTESIAN_POINT('Ctrl Pts',(-18.901540387397,-12.5679965800268,
115.061071272176)) ;
#165314=CARTESIAN_POINT('Ctrl Pts',(-18.9753442416054,-12.5679965585884,
115.03684026335)) ;
#165315=CARTESIAN_POINT('Ctrl Pts',(-18.9623717222324,-12.504495414012,
114.997328061661)) ;
#165316=CARTESIAN_POINT('Ctrl Pts',(-18.9493992028594,-12.4409942694355,
114.957815859971)) ;
#165317=CARTESIAN_POINT('Ctrl Pts',(-18.875595348651,-12.440994290874,114.982046868797)) ;
#165318=CARTESIAN_POINT('Ctrl Pts',(-18.8017914944426,-12.4409943123124,
115.006277877623)) ;
#165319=CARTESIAN_POINT('Ctrl Pts',(-18.8147640138156,-12.5044954568888,
115.045790079313)) ;
#165320=CARTESIAN_POINT('Ctrl Pts',(-18.9079928918168,-12.3799491141259,
115.294083315744)) ;
#165321=CARTESIAN_POINT('Ctrl Pts',(-18.9152137115967,-12.4522433406483,
115.316076768303)) ;
#165322=CARTESIAN_POINT('Ctrl Pts',(-18.9890175640882,-12.4522433323691,
115.291845754247)) ;
#165323=CARTESIAN_POINT('Ctrl Pts',(-19.0628214165796,-12.4522433240898,
115.267614740191)) ;
#165324=CARTESIAN_POINT('Ctrl Pts',(-19.0556005967997,-12.3799490975675,
115.245621287633)) ;
#165325=CARTESIAN_POINT('Ctrl Pts',(-19.0483797770198,-12.3076548710451,
115.223627835074)) ;
#165326=CARTESIAN_POINT('Ctrl Pts',(-18.9745759245284,-12.3076548793244,
115.247858849129)) ;
#165327=CARTESIAN_POINT('Ctrl Pts',(-18.9007720720369,-12.3076548876036,
115.272089863185)) ;
#165328=CARTESIAN_POINT('Ctrl Pts',(-18.9079928918168,-12.3799491141259,
115.294083315744)) ;
#165329=CARTESIAN_POINT('Ctrl Pts',(-19.0076357668637,-12.3308555788642,
115.562256980437)) ;
#165330=CARTESIAN_POINT('Ctrl Pts',(-19.0086410153361,-12.4066867963508,
115.56531880554)) ;
#165331=CARTESIAN_POINT('Ctrl Pts',(-19.0824448660441,-12.4066867960904,
115.541087786052)) ;
#165332=CARTESIAN_POINT('Ctrl Pts',(-19.1562487167521,-12.4066867958299,
115.516856766564)) ;
#165333=CARTESIAN_POINT('Ctrl Pts',(-19.1552434682797,-12.3308555783432,
115.513794941461)) ;
#165334=CARTESIAN_POINT('Ctrl Pts',(-19.1542382198073,-12.2550243608565,
115.510733116358)) ;
#165335=CARTESIAN_POINT('Ctrl Pts',(-19.0804343690993,-12.255024361117,
115.534964135846)) ;
#165336=CARTESIAN_POINT('Ctrl Pts',(-19.0066305183913,-12.2550243613775,
115.559195155333)) ;
#165337=CARTESIAN_POINT('Ctrl Pts',(-19.0076357668637,-12.3308555788642,
115.562256980437)) ;
#165338=CARTESIAN_POINT('Ctrl Pts',(-19.1085420809616,-12.3590358220882,
115.83413499983)) ;
#165339=CARTESIAN_POINT('Ctrl Pts',(-19.1032370638223,-12.4330140750954,
115.81797677389)) ;
#165340=CARTESIAN_POINT('Ctrl Pts',(-19.1770409119809,-12.4330140793916,
115.793745746637)) ;
#165341=CARTESIAN_POINT('Ctrl Pts',(-19.2508447601395,-12.4330140836878,
115.769514719384)) ;
#165342=CARTESIAN_POINT('Ctrl Pts',(-19.2561497772788,-12.3590358306806,
115.785672945324)) ;
#165343=CARTESIAN_POINT('Ctrl Pts',(-19.2614547944181,-12.2850575776733,
115.801831171264)) ;
#165344=CARTESIAN_POINT('Ctrl Pts',(-19.1876509462595,-12.2850575733772,
115.826062198516)) ;
#165345=CARTESIAN_POINT('Ctrl Pts',(-19.1138470981009,-12.285057569081,
115.850293225769)) ;
#165346=CARTESIAN_POINT('Ctrl Pts',(-19.1085420809616,-12.3590358220882,
115.83413499983)) ;
#165347=CARTESIAN_POINT('Ctrl Pts',(-19.2039631545433,-12.4632787296656,
116.089280063795)) ;
#165348=CARTESIAN_POINT('Ctrl Pts',(-19.1927217645793,-12.5300899100408,
116.055040603927)) ;
#165349=CARTESIAN_POINT('Ctrl Pts',(-19.2665256103156,-12.5300899147854,
116.030809569297)) ;
#165350=CARTESIAN_POINT('Ctrl Pts',(-19.3403294560519,-12.5300899195299,
116.006578534666)) ;
#165351=CARTESIAN_POINT('Ctrl Pts',(-19.3515708460159,-12.4632787391547,
116.040817994534)) ;
#165352=CARTESIAN_POINT('Ctrl Pts',(-19.3628122359799,-12.3964675587795,
116.075057454402)) ;
#165353=CARTESIAN_POINT('Ctrl Pts',(-19.2890083902436,-12.396467554035,
116.099288489033)) ;
#165354=CARTESIAN_POINT('Ctrl Pts',(-19.2152045445073,-12.3964675492904,
116.123519523663)) ;
#165355=CARTESIAN_POINT('Ctrl Pts',(-19.2039631545433,-12.4632787296656,
116.089280063795)) ;
#165356=CARTESIAN_POINT('Ctrl Pts',(-19.2877487102314,-12.6363587431469,
116.308941746476)) ;
#165357=CARTESIAN_POINT('Ctrl Pts',(-19.2713752688425,-12.6911848598895,
116.259070885909)) ;
#165358=CARTESIAN_POINT('Ctrl Pts',(-19.3451791128408,-12.6911848623011,
116.234839845984)) ;
#165359=CARTESIAN_POINT('Ctrl Pts',(-19.4189829568391,-12.6911848647128,
116.21060880606)) ;
#165360=CARTESIAN_POINT('Ctrl Pts',(-19.435356398228,-12.6363587479702,
116.260479666627)) ;
#165361=CARTESIAN_POINT('Ctrl Pts',(-19.451729839617,-12.5815326312277,
116.310350527194)) ;
#165362=CARTESIAN_POINT('Ctrl Pts',(-19.3779259956186,-12.5815326288161,
116.334581567118)) ;
#165363=CARTESIAN_POINT('Ctrl Pts',(-19.3041221516203,-12.5815326264044,
116.358812607043)) ;
#165364=CARTESIAN_POINT('Ctrl Pts',(-19.2877487102314,-12.6363587431469,
116.308941746476)) ;
#165365=CARTESIAN_POINT('Ctrl Pts',(-19.3543294992995,-12.864158222785,
116.476393219925)) ;
#165366=CARTESIAN_POINT('Ctrl Pts',(-19.3340139079031,-12.9031598637825,
116.414515206428)) ;
#165367=CARTESIAN_POINT('Ctrl Pts',(-19.4078177511336,-12.9031598633717,
116.390284164164)) ;
#165368=CARTESIAN_POINT('Ctrl Pts',(-19.481621594364,-12.9031598629608,
116.366053121901)) ;
#165369=CARTESIAN_POINT('Ctrl Pts',(-19.5019371857604,-12.8641582219634,
116.427931135398)) ;
#165370=CARTESIAN_POINT('Ctrl Pts',(-19.5222527771567,-12.8251565809659,
116.489809148895)) ;
#165371=CARTESIAN_POINT('Ctrl Pts',(-19.4484489339263,-12.8251565813767,
116.514040191159)) ;
#165372=CARTESIAN_POINT('Ctrl Pts',(-19.3746450906959,-12.8251565817875,
116.538271233422)) ;
#165373=CARTESIAN_POINT('Ctrl Pts',(-19.3543294992995,-12.864158222785,
116.476393219925)) ;
#165374=CARTESIAN_POINT('Ctrl Pts',(-19.4003945437516,-13.1343225359667,
116.580991063038)) ;
#165375=CARTESIAN_POINT('Ctrl Pts',(-19.3775707263678,-13.1545167875365,
116.511473397833)) ;
#165376=CARTESIAN_POINT('Ctrl Pts',(-19.4513745694738,-13.1545167844315,
116.487242355191)) ;
#165377=CARTESIAN_POINT('Ctrl Pts',(-19.5251784125798,-13.1545167813264,
116.463011312549)) ;
#165378=CARTESIAN_POINT('Ctrl Pts',(-19.5480022299636,-13.1343225297566,
116.532528977753)) ;
#165379=CARTESIAN_POINT('Ctrl Pts',(-19.5708260473473,-13.1141282781868,
116.602046642958)) ;
#165380=CARTESIAN_POINT('Ctrl Pts',(-19.4970222042414,-13.1141282812919,
116.6262776856)) ;
#165381=CARTESIAN_POINT('Ctrl Pts',(-19.4232183611354,-13.114128284397,
116.650508728242)) ;
#165382=CARTESIAN_POINT('Ctrl Pts',(-19.4003945437516,-13.1343225359667,
116.580991063038)) ;
#165383=CARTESIAN_POINT('Ctrl Pts',(-19.4225349879933,-13.4205967944479,
116.613269030922)) ;
#165384=CARTESIAN_POINT('Ctrl Pts',(-19.3988592410925,-13.4208311388444,
116.541156525867)) ;
#165385=CARTESIAN_POINT('Ctrl Pts',(-19.4726630845397,-13.4208311356135,
116.516925484264)) ;
#165386=CARTESIAN_POINT('Ctrl Pts',(-19.5464669279869,-13.4208311323827,
116.492694442662)) ;
#165387=CARTESIAN_POINT('Ctrl Pts',(-19.5701426748878,-13.4205967879863,
116.564806947716)) ;
#165388=CARTESIAN_POINT('Ctrl Pts',(-19.5938184217886,-13.4203624435898,
116.636919452771)) ;
#165389=CARTESIAN_POINT('Ctrl Pts',(-19.5200145783414,-13.4203624468207,
116.661150494374)) ;
#165390=CARTESIAN_POINT('Ctrl Pts',(-19.4462107348942,-13.4203624500515,
116.685381535977)) ;
#165391=CARTESIAN_POINT('Ctrl Pts',(-19.4225349879933,-13.4205967944479,
116.613269030922)) ;
#165392=CARTESIAN_POINT('Ctrl Pts',(-19.4206705194364,-13.7102521447362,
116.57197231337)) ;
#165393=CARTESIAN_POINT('Ctrl Pts',(-19.3978270561401,-13.6902603542672,
116.502394809927)) ;
#165394=CARTESIAN_POINT('Ctrl Pts',(-19.4716308997194,-13.6902603532413,
116.478163768727)) ;
#165395=CARTESIAN_POINT('Ctrl Pts',(-19.5454347432987,-13.6902603522153,
116.453932727526)) ;
#165396=CARTESIAN_POINT('Ctrl Pts',(-19.568278206595,-13.7102521426842,
116.523510230969)) ;
#165397=CARTESIAN_POINT('Ctrl Pts',(-19.5911216698912,-13.7302439331532,
116.593087734412)) ;
#165398=CARTESIAN_POINT('Ctrl Pts',(-19.5173178263119,-13.7302439341791,
116.617318775612)) ;
#165399=CARTESIAN_POINT('Ctrl Pts',(-19.4435139827326,-13.7302439352051,
116.641549816813)) ;
#165400=CARTESIAN_POINT('Ctrl Pts',(-19.4206705194364,-13.7102521447362,
116.57197231337)) ;
#165401=CARTESIAN_POINT('Ctrl Pts',(-19.3953354743405,-13.9772668612757,
116.459412299705)) ;
#165402=CARTESIAN_POINT('Ctrl Pts',(-19.3749601067379,-13.9386012749513,
116.39735221759)) ;
#165403=CARTESIAN_POINT('Ctrl Pts',(-19.4487639498612,-13.9386012773307,
116.373121175)) ;
#165404=CARTESIAN_POINT('Ctrl Pts',(-19.5225677929844,-13.9386012797101,
116.34889013241)) ;
#165405=CARTESIAN_POINT('Ctrl Pts',(-19.5429431605871,-13.9772668660344,
116.410950214526)) ;
#165406=CARTESIAN_POINT('Ctrl Pts',(-19.5633185281897,-14.0159324523587,
116.473010296642)) ;
#165407=CARTESIAN_POINT('Ctrl Pts',(-19.4895146850664,-14.0159324499793,
116.497241339231)) ;
#165408=CARTESIAN_POINT('Ctrl Pts',(-19.4157108419431,-14.0159324476,116.521472381821)) ;
#165409=CARTESIAN_POINT('Ctrl Pts',(-19.3953354743405,-13.9772668612757,
116.459412299705)) ;
#165410=CARTESIAN_POINT('Ctrl Pts',(-19.3490326024128,-14.2052355202481,
116.282832240174)) ;
#165411=CARTESIAN_POINT('Ctrl Pts',(-19.3325962215449,-14.1505953290783,
116.232769676212)) ;
#165412=CARTESIAN_POINT('Ctrl Pts',(-19.4064000631929,-14.1505953352011,
116.208538629129)) ;
#165413=CARTESIAN_POINT('Ctrl Pts',(-19.4802039048408,-14.150595341324,
116.184307582046)) ;
#165414=CARTESIAN_POINT('Ctrl Pts',(-19.4966402857087,-14.2052355324938,
116.234370146008)) ;
#165415=CARTESIAN_POINT('Ctrl Pts',(-19.5130766665765,-14.2598757236637,
116.28443270997)) ;
#165416=CARTESIAN_POINT('Ctrl Pts',(-19.4392728249286,-14.2598757175408,
116.308663757054)) ;
#165417=CARTESIAN_POINT('Ctrl Pts',(-19.3654689832807,-14.259875711418,
116.332894804137)) ;
#165418=CARTESIAN_POINT('Ctrl Pts',(-19.3490326024128,-14.2052355202481,
116.282832240174)) ;
#165419=CARTESIAN_POINT('Ctrl Pts',(-19.2861456806911,-14.3759216033723,
116.055895655754)) ;
#165420=CARTESIAN_POINT('Ctrl Pts',(-19.2748088376837,-14.3092842663228,
116.021365461424)) ;
#165421=CARTESIAN_POINT('Ctrl Pts',(-19.3486126772273,-14.309284273676,
115.997134407932)) ;
#165422=CARTESIAN_POINT('Ctrl Pts',(-19.4224165167709,-14.3092842810292,
115.972903354439)) ;
#165423=CARTESIAN_POINT('Ctrl Pts',(-19.4337533597783,-14.3759216180787,
116.007433548769)) ;
#165424=CARTESIAN_POINT('Ctrl Pts',(-19.4450902027857,-14.4425589551282,
116.041963743098)) ;
#165425=CARTESIAN_POINT('Ctrl Pts',(-19.3712863632421,-14.442558947775,
116.066194796591)) ;
#165426=CARTESIAN_POINT('Ctrl Pts',(-19.2974825236984,-14.4425589404218,
116.090425850083)) ;
#165427=CARTESIAN_POINT('Ctrl Pts',(-19.2861456806911,-14.3759216033723,
116.055895655754)) ;
#165428=CARTESIAN_POINT('Ctrl Pts',(-19.2116524882323,-14.478404639523,
115.793537621104)) ;
#165429=CARTESIAN_POINT('Ctrl Pts',(-19.2062343723869,-14.404515033937,
115.77703491487)) ;
#165430=CARTESIAN_POINT('Ctrl Pts',(-19.2800382092211,-14.4045150394246,
115.752803853124)) ;
#165431=CARTESIAN_POINT('Ctrl Pts',(-19.3538420460552,-14.4045150449122,
115.728572791379)) ;
#165432=CARTESIAN_POINT('Ctrl Pts',(-19.3592601619006,-14.4784046504982,
115.745075497613)) ;
#165433=CARTESIAN_POINT('Ctrl Pts',(-19.364678277746,-14.5522942560841,
115.761578203847)) ;
#165434=CARTESIAN_POINT('Ctrl Pts',(-19.2908744409119,-14.5522942505966,
115.785809265593)) ;
#165435=CARTESIAN_POINT('Ctrl Pts',(-19.2170706040777,-14.552294245109,
115.810040327338)) ;
#165436=CARTESIAN_POINT('Ctrl Pts',(-19.2116524882323,-14.478404639523,
115.793537621104)) ;
#165437=CARTESIAN_POINT('Ctrl Pts',(-19.1318016810032,-14.505089399069,
115.514904636501)) ;
#165438=CARTESIAN_POINT('Ctrl Pts',(-19.1326839640339,-14.4292297938268,
115.517591928826)) ;
#165439=CARTESIAN_POINT('Ctrl Pts',(-19.2064877982472,-14.4292297934085,
115.493360859098)) ;
#165440=CARTESIAN_POINT('Ctrl Pts',(-19.2802916324605,-14.4292297929902,
115.46912978937)) ;
#165441=CARTESIAN_POINT('Ctrl Pts',(-19.2794093494299,-14.5050893982325,
115.466442497045)) ;
#165442=CARTESIAN_POINT('Ctrl Pts',(-19.2785270663992,-14.5809490034747,
115.46375520472)) ;
#165443=CARTESIAN_POINT('Ctrl Pts',(-19.2047232321859,-14.580949003893,
115.487986274448)) ;
#165444=CARTESIAN_POINT('Ctrl Pts',(-19.1309193979726,-14.5809490043113,
115.512217344176)) ;
#165445=CARTESIAN_POINT('Ctrl Pts',(-19.1318016810032,-14.505089399069,
115.514904636501)) ;
#165446=CARTESIAN_POINT('Ctrl Pts',(-19.0524890416985,-14.4533114988155,
115.237672140607)) ;
#165447=CARTESIAN_POINT('Ctrl Pts',(-19.0596481858551,-14.3809567964235,
115.259477739355)) ;
#165448=CARTESIAN_POINT('Ctrl Pts',(-19.1334520173609,-14.3809567849074,
115.23524666138)) ;
#165449=CARTESIAN_POINT('Ctrl Pts',(-19.2072558488666,-14.3809567733913,
115.211015583405)) ;
#165450=CARTESIAN_POINT('Ctrl Pts',(-19.20009670471,-14.4533114757834,115.189209984658)) ;
#165451=CARTESIAN_POINT('Ctrl Pts',(-19.1929375605535,-14.5256661781754,
115.16740438591)) ;
#165452=CARTESIAN_POINT('Ctrl Pts',(-19.1191337290477,-14.5256661896915,
115.191635463884)) ;
#165453=CARTESIAN_POINT('Ctrl Pts',(-19.045329897542,-14.5256662012075,
115.215866541859)) ;
#165454=CARTESIAN_POINT('Ctrl Pts',(-19.0524890416985,-14.4533114988155,
115.237672140607)) ;
#165455=CARTESIAN_POINT('Ctrl Pts',(-18.9813656993656,-14.3281114059052,
114.985728322103)) ;
#165456=CARTESIAN_POINT('Ctrl Pts',(-18.9942316512457,-14.2643939997168,
115.024915936526)) ;
#165457=CARTESIAN_POINT('Ctrl Pts',(-19.0680354822422,-14.26439397447,115.000684857001)) ;
#165458=CARTESIAN_POINT('Ctrl Pts',(-19.1418393132387,-14.2643939492231,
114.976453777475)) ;
#165459=CARTESIAN_POINT('Ctrl Pts',(-19.1289733613586,-14.3281113554114,
114.937266163052)) ;
#165460=CARTESIAN_POINT('Ctrl Pts',(-19.1161074094785,-14.3918287615997,
114.898078548628)) ;
#165461=CARTESIAN_POINT('Ctrl Pts',(-19.042303578482,-14.3918287868466,
114.922309628154)) ;
#165462=CARTESIAN_POINT('Ctrl Pts',(-18.9684997474855,-14.3918288120935,
114.946540707679)) ;
#165463=CARTESIAN_POINT('Ctrl Pts',(-18.9813656993656,-14.3281114059052,
114.985728322103)) ;
#165464=CARTESIAN_POINT('Ctrl Pts',(-18.9231476629716,-14.1371521548342,
114.77288475777)) ;
#165465=CARTESIAN_POINT('Ctrl Pts',(-18.9408319558963,-14.0866750756418,
114.826748261758)) ;
#165466=CARTESIAN_POINT('Ctrl Pts',(-19.0146357875153,-14.0866750338847,
114.802517184128)) ;
#165467=CARTESIAN_POINT('Ctrl Pts',(-19.0884396191342,-14.0866749921275,
114.778286106498)) ;
#165468=CARTESIAN_POINT('Ctrl Pts',(-19.0707553262095,-14.1371520713199,
114.724422602511)) ;
#165469=CARTESIAN_POINT('Ctrl Pts',(-19.0530710332848,-14.1876291505123,
114.670559098523)) ;
#165470=CARTESIAN_POINT('Ctrl Pts',(-18.9792672016658,-14.1876291922694,
114.694790176153)) ;
#165471=CARTESIAN_POINT('Ctrl Pts',(-18.9054633700469,-14.1876292340265,
114.719021253783)) ;
#165472=CARTESIAN_POINT('Ctrl Pts',(-18.9231476629716,-14.1371521548342,
114.77288475777)) ;
#165473=CARTESIAN_POINT('Ctrl Pts',(-18.8833376833502,-13.8952369066383,
114.616222830795)) ;
#165474=CARTESIAN_POINT('Ctrl Pts',(-18.9045596128905,-13.8615770485299,
114.680861405271)) ;
#165475=CARTESIAN_POINT('Ctrl Pts',(-18.9783634473156,-13.861576991076,
114.656630336188)) ;
#165476=CARTESIAN_POINT('Ctrl Pts',(-19.0521672817407,-13.8615769336222,
114.632399267105)) ;
#165477=CARTESIAN_POINT('Ctrl Pts',(-19.0309453522004,-13.8952367917306,
114.567760692629)) ;
#165478=CARTESIAN_POINT('Ctrl Pts',(-19.0097234226601,-13.928896649839,
114.503122118153)) ;
#165479=CARTESIAN_POINT('Ctrl Pts',(-18.935919588235,-13.9288967072929,
114.527353187236)) ;
#165480=CARTESIAN_POINT('Ctrl Pts',(-18.8621157538098,-13.9288967647467,
114.551584256319)) ;
#165481=CARTESIAN_POINT('Ctrl Pts',(-18.8833376833502,-13.8952369066383,
114.616222830795)) ;
#165482=CARTESIAN_POINT('Ctrl Pts',(-18.8652708972368,-13.6186018565224,
114.525698941726)) ;
#165483=CARTESIAN_POINT('Ctrl Pts',(-18.8885194152068,-13.6042072181223,
114.596510177732)) ;
#165484=CARTESIAN_POINT('Ctrl Pts',(-18.9623232542295,-13.6042071468649,
114.572279122652)) ;
#165485=CARTESIAN_POINT('Ctrl Pts',(-19.0361270932522,-13.6042070756075,
114.548048067573)) ;
#165486=CARTESIAN_POINT('Ctrl Pts',(-19.0128785752822,-13.6186017140076,
114.477236831567)) ;
#165487=CARTESIAN_POINT('Ctrl Pts',(-18.9896300573122,-13.6329963524077,
114.406425595561)) ;
#165488=CARTESIAN_POINT('Ctrl Pts',(-18.9158262182895,-13.6329964236651,
114.430656650641)) ;
#165489=CARTESIAN_POINT('Ctrl Pts',(-18.8420223792668,-13.6329964949225,
114.45488770572)) ;
#165490=CARTESIAN_POINT('Ctrl Pts',(-18.8652708972368,-13.6186018565224,
114.525698941726)) ;
#165491=CARTESIAN_POINT('Ctrl Pts',(-18.8711343231666,-13.3278430882069,
114.508099714174)) ;
#165492=CARTESIAN_POINT('Ctrl Pts',(-18.8947408656178,-13.3337275360589,
114.580001435127)) ;
#165493=CARTESIAN_POINT('Ctrl Pts',(-18.9685447109095,-13.3337274561623,
114.555770399142)) ;
#165494=CARTESIAN_POINT('Ctrl Pts',(-19.0423485562011,-13.3337273762658,
114.531539363158)) ;
#165495=CARTESIAN_POINT('Ctrl Pts',(-19.01874201375,-13.3278429284139,114.459637642204)) ;
#165496=CARTESIAN_POINT('Ctrl Pts',(-18.9951354712988,-13.3219584805619,
114.387735921251)) ;
#165497=CARTESIAN_POINT('Ctrl Pts',(-18.9213316260071,-13.3219585604584,
114.411966957236)) ;
#165498=CARTESIAN_POINT('Ctrl Pts',(-18.8475277807154,-13.3219586403549,
114.436197993221)) ;
#165499=CARTESIAN_POINT('Ctrl Pts',(-18.8711343231666,-13.3278430882069,
114.508099714174)) ;
#165500=CARTESIAN_POINT('Ctrl Pts',(-18.9012499909947,-13.0431633993278,
114.564322017916)) ;
#165501=CARTESIAN_POINT('Ctrl Pts',(-18.9235229473357,-13.0689317715885,
114.632161850889)) ;
#165502=CARTESIAN_POINT('Ctrl Pts',(-18.9973267999589,-13.0689316894194,
114.607930837235)) ;
#165503=CARTESIAN_POINT('Ctrl Pts',(-19.0711306525821,-13.0689316072503,
114.583699823581)) ;
#165504=CARTESIAN_POINT('Ctrl Pts',(-19.0488576962411,-13.0431632349896,
114.515859990607)) ;
#165505=CARTESIAN_POINT('Ctrl Pts',(-19.0265847399001,-13.0173948627289,
114.448020157633)) ;
#165506=CARTESIAN_POINT('Ctrl Pts',(-18.9527808872769,-13.017394944898,
114.472251171288)) ;
#165507=CARTESIAN_POINT('Ctrl Pts',(-18.8789770346537,-13.0173950270671,
114.496482184942)) ;
#165508=CARTESIAN_POINT('Ctrl Pts',(-18.9012499909947,-13.0431633993278,
114.564322017916)) ;
#165509=CARTESIAN_POINT('Ctrl Pts',(-18.9542826657054,-12.7854826732307,
114.69034661993)) ;
#165510=CARTESIAN_POINT('Ctrl Pts',(-18.9736201800411,-12.8292789756885,
114.749245570308)) ;
#165511=CARTESIAN_POINT('Ctrl Pts',(-19.0474240403087,-12.8292788993553,
114.725014579938)) ;
#165512=CARTESIAN_POINT('Ctrl Pts',(-19.1212279005763,-12.8292788230221,
114.700783589567)) ;
#165513=CARTESIAN_POINT('Ctrl Pts',(-19.1018903862406,-12.7854825205643,
114.641884639189)) ;
#165514=CARTESIAN_POINT('Ctrl Pts',(-19.0825528719048,-12.7416862181065,
114.582985688811)) ;
#165515=CARTESIAN_POINT('Ctrl Pts',(-19.0087490116372,-12.7416862944397,
114.607216679182)) ;
#165516=CARTESIAN_POINT('Ctrl Pts',(-18.9349451513697,-12.7416863707729,
114.631447669552)) ;
#165517=CARTESIAN_POINT('Ctrl Pts',(-18.9542826657054,-12.7854826732307,
114.69034661993)) ;
#165518=CARTESIAN_POINT('Ctrl Pts',(-19.0266928617708,-12.5740916835464,
114.875572584882)) ;
#165519=CARTESIAN_POINT('Ctrl Pts',(-19.0417339574054,-12.6327102616695,
114.921385337205)) ;
#165520=CARTESIAN_POINT('Ctrl Pts',(-19.1155378244281,-12.6327101996491,
114.897154367409)) ;
#165521=CARTESIAN_POINT('Ctrl Pts',(-19.1893416914507,-12.6327101376288,
114.872923397613)) ;
#165522=CARTESIAN_POINT('Ctrl Pts',(-19.174300595816,-12.5740915595058,
114.82711064529)) ;
#165523=CARTESIAN_POINT('Ctrl Pts',(-19.1592595001814,-12.5154729813828,
114.781297892968)) ;
#165524=CARTESIAN_POINT('Ctrl Pts',(-19.0854556331588,-12.5154730434031,
114.805528862764)) ;
#165525=CARTESIAN_POINT('Ctrl Pts',(-19.0116517661362,-12.5154731054234,
114.829759832559)) ;
#165526=CARTESIAN_POINT('Ctrl Pts',(-19.0266928617708,-12.5740916835464,
114.875572584882)) ;
#165527=CARTESIAN_POINT('Ctrl Pts',(-19.1147735207953,-12.4220262848849,
115.108352144705)) ;
#165528=CARTESIAN_POINT('Ctrl Pts',(-19.1244217586792,-12.4913473054171,
115.137739122539)) ;
#165529=CARTESIAN_POINT('Ctrl Pts',(-19.1982256312606,-12.49134726396,115.113508169674)) ;
#165530=CARTESIAN_POINT('Ctrl Pts',(-19.2720295038421,-12.491347222503,
115.089277216809)) ;
#165531=CARTESIAN_POINT('Ctrl Pts',(-19.2623812659582,-12.4220262019709,
115.059890238976)) ;
#165532=CARTESIAN_POINT('Ctrl Pts',(-19.2527330280743,-12.3527051814387,
115.030503261142)) ;
#165533=CARTESIAN_POINT('Ctrl Pts',(-19.1789291554929,-12.3527052228958,
115.054734214006)) ;
#165534=CARTESIAN_POINT('Ctrl Pts',(-19.1051252829115,-12.3527052643528,
115.078965166871)) ;
#165535=CARTESIAN_POINT('Ctrl Pts',(-19.1147735207953,-12.4220262848849,
115.108352144705)) ;
#165536=CARTESIAN_POINT('Ctrl Pts',(-19.2125943662298,-12.3415697140928,
115.370830458486)) ;
#165537=CARTESIAN_POINT('Ctrl Pts',(-19.2161611902284,-12.4166096733525,
115.381694430919)) ;
#165538=CARTESIAN_POINT('Ctrl Pts',(-19.2899650661739,-12.4166096578571,
115.357463488301)) ;
#165539=CARTESIAN_POINT('Ctrl Pts',(-19.3637689421193,-12.4166096423617,
115.333232545682)) ;
#165540=CARTESIAN_POINT('Ctrl Pts',(-19.3602021181207,-12.341569683102,
115.32236857325)) ;
#165541=CARTESIAN_POINT('Ctrl Pts',(-19.356635294122,-12.2665297238424,
115.311504600817)) ;
#165542=CARTESIAN_POINT('Ctrl Pts',(-19.2828314181766,-12.2665297393378,
115.335735543435)) ;
#165543=CARTESIAN_POINT('Ctrl Pts',(-19.2090275422311,-12.2665297548332,
115.359966486053)) ;
#165544=CARTESIAN_POINT('Ctrl Pts',(-19.2125943662298,-12.3415697140928,
115.370830458486)) ;
#165545=CARTESIAN_POINT('Ctrl Pts',(-19.3139521730816,-12.3382226972324,
115.644076064424)) ;
#165546=CARTESIAN_POINT('Ctrl Pts',(-19.3111818546697,-12.4136068588393,
115.635638123609)) ;
#165547=CARTESIAN_POINT('Ctrl Pts',(-19.3849857313629,-12.413606871913,
115.611407183268)) ;
#165548=CARTESIAN_POINT('Ctrl Pts',(-19.4587896080562,-12.4136068849868,
115.587176242927)) ;
#165549=CARTESIAN_POINT('Ctrl Pts',(-19.4615599264681,-12.3382227233798,
115.595614183743)) ;
#165550=CARTESIAN_POINT('Ctrl Pts',(-19.4643302448801,-12.2628385617728,
115.604052124559)) ;
#165551=CARTESIAN_POINT('Ctrl Pts',(-19.3905263681868,-12.2628385486991,
115.6282830649)) ;
#165552=CARTESIAN_POINT('Ctrl Pts',(-19.3167224914936,-12.2628385356254,
115.65251400524)) ;
#165553=CARTESIAN_POINT('Ctrl Pts',(-19.3139521730816,-12.3382226972324,
115.644076064424)) ;
#165554=CARTESIAN_POINT('Ctrl Pts',(-19.4122471361585,-12.4121411260321,
115.90802651911)) ;
#165555=CARTESIAN_POINT('Ctrl Pts',(-19.4033434531606,-12.4824758625955,
115.880907339398)) ;
#165556=CARTESIAN_POINT('Ctrl Pts',(-19.4771473278286,-12.4824759039206,
115.856676392889)) ;
#165557=CARTESIAN_POINT('Ctrl Pts',(-19.5509512024966,-12.4824759452457,
115.832445446379)) ;
#165558=CARTESIAN_POINT('Ctrl Pts',(-19.5598548854945,-12.4121412086823,
115.859564626092)) ;
#165559=CARTESIAN_POINT('Ctrl Pts',(-19.5687585684923,-12.3418064721188,
115.886683805805)) ;
#165560=CARTESIAN_POINT('Ctrl Pts',(-19.4949546938243,-12.3418064307938,
115.910914752314)) ;
#165561=CARTESIAN_POINT('Ctrl Pts',(-19.4211508191563,-12.3418063894687,
115.935145698823)) ;
#165562=CARTESIAN_POINT('Ctrl Pts',(-19.4122471361585,-12.4121411260321,
115.90802651911)) ;
#165563=CARTESIAN_POINT('Ctrl Pts',(-19.5013836351553,-12.5582147089023,
116.144040613698)) ;
#165564=CARTESIAN_POINT('Ctrl Pts',(-19.4869777368879,-12.6184554167387,
116.100162574049)) ;
#165565=CARTESIAN_POINT('Ctrl Pts',(-19.5607816069403,-12.6184554831094,
116.075931613481)) ;
#165566=CARTESIAN_POINT('Ctrl Pts',(-19.6345854769928,-12.61845554948,116.051700652914)) ;
#165567=CARTESIAN_POINT('Ctrl Pts',(-19.6489913752602,-12.5582148416436,
116.095578692563)) ;
#165568=CARTESIAN_POINT('Ctrl Pts',(-19.6633972735277,-12.4979741338071,
116.139456732212)) ;
#165569=CARTESIAN_POINT('Ctrl Pts',(-19.5895934034752,-12.4979740674365,
116.163687692779)) ;
#165570=CARTESIAN_POINT('Ctrl Pts',(-19.5157895334227,-12.4979740010659,
116.187918653347)) ;
#165571=CARTESIAN_POINT('Ctrl Pts',(-19.5013836351553,-12.5582147089023,
116.144040613698)) ;
#165572=CARTESIAN_POINT('Ctrl Pts',(-19.5755554742575,-12.7657436426172,
116.334505232011)) ;
#165573=CARTESIAN_POINT('Ctrl Pts',(-19.5566832764055,-12.8115849189124,
116.277023564437)) ;
#165574=CARTESIAN_POINT('Ctrl Pts',(-19.6304871397366,-12.8115850045316,
116.252792583397)) ;
#165575=CARTESIAN_POINT('Ctrl Pts',(-19.7042910030678,-12.8115850901508,
116.228561602358)) ;
#165576=CARTESIAN_POINT('Ctrl Pts',(-19.7231632009198,-12.7657438138556,
116.286043269933)) ;
#165577=CARTESIAN_POINT('Ctrl Pts',(-19.7420353987717,-12.7199025375603,
116.343524937507)) ;
#165578=CARTESIAN_POINT('Ctrl Pts',(-19.6682315354406,-12.7199024519411,
116.367755918547)) ;
#165579=CARTESIAN_POINT('Ctrl Pts',(-19.5944276721094,-12.7199023663219,
116.391986899586)) ;
#165580=CARTESIAN_POINT('Ctrl Pts',(-19.5755554742575,-12.7657436426172,
116.334505232011)) ;
#165581=CARTESIAN_POINT('Ctrl Pts',(-19.6303334920016,-13.0202106019441,
116.465864508977)) ;
#165582=CARTESIAN_POINT('Ctrl Pts',(-19.6083429686133,-13.0483542398271,
116.398884924909)) ;
#165583=CARTESIAN_POINT('Ctrl Pts',(-19.682146823822,-13.0483543369911,
116.37465391913)) ;
#165584=CARTESIAN_POINT('Ctrl Pts',(-19.7559506790307,-13.0483544341551,
116.350422913351)) ;
#165585=CARTESIAN_POINT('Ctrl Pts',(-19.777941202419,-13.0202107962721,
116.417402497419)) ;
#165586=CARTESIAN_POINT('Ctrl Pts',(-19.7999317258073,-12.992067158389,
116.484382081487)) ;
#165587=CARTESIAN_POINT('Ctrl Pts',(-19.7261278705986,-12.9920670612251,
116.508613087266)) ;
#165588=CARTESIAN_POINT('Ctrl Pts',(-19.6523240153899,-12.9920669640611,
116.532844093045)) ;
#165589=CARTESIAN_POINT('Ctrl Pts',(-19.6303334920016,-13.0202106019441,
116.465864508977)) ;
#165590=CARTESIAN_POINT('Ctrl Pts',(-19.6624379392262,-13.3031020545658,
116.528178876828)) ;
#165591=CARTESIAN_POINT('Ctrl Pts',(-19.6389070181145,-13.3115371239571,
116.456507489767)) ;
#165592=CARTESIAN_POINT('Ctrl Pts',(-19.7127108647141,-13.3115372240585,
116.432276457765)) ;
#165593=CARTESIAN_POINT('Ctrl Pts',(-19.7865147113136,-13.3115373241599,
116.408045425764)) ;
#165594=CARTESIAN_POINT('Ctrl Pts',(-19.8100456324252,-13.3031022547687,
116.479716812825)) ;
#165595=CARTESIAN_POINT('Ctrl Pts',(-19.8335765535369,-13.2946671853774,
116.551388199887)) ;
#165596=CARTESIAN_POINT('Ctrl Pts',(-19.7597727069374,-13.2946670852759,
116.575619231888)) ;
#165597=CARTESIAN_POINT('Ctrl Pts',(-19.6859688603378,-13.2946669851745,
116.599850263889)) ;
#165598=CARTESIAN_POINT('Ctrl Pts',(-19.6624379392262,-13.3031020545658,
116.528178876828)) ;
#165599=CARTESIAN_POINT('Ctrl Pts',(-19.6703646074423,-13.593918747588,
116.516886330031)) ;
#165600=CARTESIAN_POINT('Ctrl Pts',(-19.6469782287227,-13.5820623140505,
116.445655195687)) ;
#165601=CARTESIAN_POINT('Ctrl Pts',(-19.7207820671414,-13.5820624088636,
116.421424138769)) ;
#165602=CARTESIAN_POINT('Ctrl Pts',(-19.7945859055601,-13.5820625036768,
116.39719308185)) ;
#165603=CARTESIAN_POINT('Ctrl Pts',(-19.8179722842797,-13.5939189372143,
116.468424216193)) ;
#165604=CARTESIAN_POINT('Ctrl Pts',(-19.8413586629993,-13.6057753707518,
116.539655350536)) ;
#165605=CARTESIAN_POINT('Ctrl Pts',(-19.7675548245806,-13.6057752759387,
116.563886407455)) ;
#165606=CARTESIAN_POINT('Ctrl Pts',(-19.6937509861619,-13.6057751811255,
116.588117464374)) ;
#165607=CARTESIAN_POINT('Ctrl Pts',(-19.6703646074423,-13.593918747588,
116.516886330031)) ;
#165608=CARTESIAN_POINT('Ctrl Pts',(-19.654361800593,-13.8723058564386,
116.432695143982)) ;
#165609=CARTESIAN_POINT('Ctrl Pts',(-19.6327910609281,-13.8409951979867,
116.366994153143)) ;
#165610=CARTESIAN_POINT('Ctrl Pts',(-19.7065948923452,-13.8409952801853,
116.342763074898)) ;
#165611=CARTESIAN_POINT('Ctrl Pts',(-19.7803987237623,-13.8409953623839,
116.318531996653)) ;
#165612=CARTESIAN_POINT('Ctrl Pts',(-19.8019694634272,-13.8723060208357,
116.384232987493)) ;
#165613=CARTESIAN_POINT('Ctrl Pts',(-19.8235402030921,-13.9036166792876,
116.449933978333)) ;
#165614=CARTESIAN_POINT('Ctrl Pts',(-19.7497363716751,-13.903616597089,
116.474165056577)) ;
#165615=CARTESIAN_POINT('Ctrl Pts',(-19.675932540258,-13.9036165148904,
116.498396134822)) ;
#165616=CARTESIAN_POINT('Ctrl Pts',(-19.654361800593,-13.8723058564386,
116.432695143982)) ;
#165617=CARTESIAN_POINT('Ctrl Pts',(-19.6160972828307,-14.118869151071,
116.28058076468)) ;
#165618=CARTESIAN_POINT('Ctrl Pts',(-19.5979014436013,-14.070296502829,
116.225159175889)) ;
#165619=CARTESIAN_POINT('Ctrl Pts',(-19.6717052700668,-14.0702965663063,
116.200928082563)) ;
#165620=CARTESIAN_POINT('Ctrl Pts',(-19.7455090965323,-14.0702966297837,
116.176696989237)) ;
#165621=CARTESIAN_POINT('Ctrl Pts',(-19.7637049357618,-14.1188692780257,
116.232118578027)) ;
#165622=CARTESIAN_POINT('Ctrl Pts',(-19.7819007749912,-14.1674419262677,
116.287540166818)) ;
#165623=CARTESIAN_POINT('Ctrl Pts',(-19.7080969485257,-14.1674418627903,
116.311771260144)) ;
#165624=CARTESIAN_POINT('Ctrl Pts',(-19.6342931220601,-14.167441799313,
116.33600235347)) ;
#165625=CARTESIAN_POINT('Ctrl Pts',(-19.6160972828307,-14.118869151071,
116.28058076468)) ;
#165626=CARTESIAN_POINT('Ctrl Pts',(-19.5594235023051,-14.3141618691383,
116.072558650633)) ;
#165627=CARTESIAN_POINT('Ctrl Pts',(-19.5458897072115,-14.2518807456653,
116.031336895932)) ;
#165628=CARTESIAN_POINT('Ctrl Pts',(-19.6196935307721,-14.2518807886643,
116.007105793758)) ;
#165629=CARTESIAN_POINT('Ctrl Pts',(-19.6934973543327,-14.2518808316633,
115.982874691584)) ;
#165630=CARTESIAN_POINT('Ctrl Pts',(-19.7070311494263,-14.3141619551363,
116.024096446284)) ;
#165631=CARTESIAN_POINT('Ctrl Pts',(-19.7205649445198,-14.3764430786093,
116.065318200985)) ;
#165632=CARTESIAN_POINT('Ctrl Pts',(-19.6467611209592,-14.3764430356103,
116.089549303159)) ;
#165633=CARTESIAN_POINT('Ctrl Pts',(-19.5729572973986,-14.3764429926113,
116.113780405334)) ;
#165634=CARTESIAN_POINT('Ctrl Pts',(-19.5594235023051,-14.3141618691383,
116.072558650633)) ;
#165635=CARTESIAN_POINT('Ctrl Pts',(-19.4889283697476,-14.4456574881185,
115.82238678645)) ;
#165636=CARTESIAN_POINT('Ctrl Pts',(-19.4810297011629,-14.3741011608773,
115.798328717722)) ;
#165637=CARTESIAN_POINT('Ctrl Pts',(-19.5548335241347,-14.3741011828996,
115.774097613754)) ;
#165638=CARTESIAN_POINT('Ctrl Pts',(-19.6286373471065,-14.3741012049218,
115.749866509787)) ;
#165639=CARTESIAN_POINT('Ctrl Pts',(-19.6365360156912,-14.4456575321631,
115.773924578514)) ;
#165640=CARTESIAN_POINT('Ctrl Pts',(-19.6444346842759,-14.5172138594043,
115.797982647242)) ;
#165641=CARTESIAN_POINT('Ctrl Pts',(-19.5706308613041,-14.5172138373821,
115.82221375121)) ;
#165642=CARTESIAN_POINT('Ctrl Pts',(-19.4968270383323,-14.5172138153598,
115.846444855178)) ;
#165643=CARTESIAN_POINT('Ctrl Pts',(-19.4889283697476,-14.4456574881185,
115.82238678645)) ;
#165644=CARTESIAN_POINT('Ctrl Pts',(-19.4104748865899,-14.5036635199146,
115.547989903385)) ;
#165645=CARTESIAN_POINT('Ctrl Pts',(-19.4087752444467,-14.4279488253923,
115.542813068833)) ;
#165646=CARTESIAN_POINT('Ctrl Pts',(-19.4825790688346,-14.4279488285843,
115.518581969179)) ;
#165647=CARTESIAN_POINT('Ctrl Pts',(-19.5563828932225,-14.4279488317762,
115.494350869525)) ;
#165648=CARTESIAN_POINT('Ctrl Pts',(-19.5580825353658,-14.5036635262985,
115.499527704076)) ;
#165649=CARTESIAN_POINT('Ctrl Pts',(-19.5597821775091,-14.5793782208208,
115.504704538628)) ;
#165650=CARTESIAN_POINT('Ctrl Pts',(-19.4859783531212,-14.5793782176288,
115.528935638283)) ;
#165651=CARTESIAN_POINT('Ctrl Pts',(-19.4121745287332,-14.5793782144369,
115.553166737937)) ;
#165652=CARTESIAN_POINT('Ctrl Pts',(-19.4104748865899,-14.5036635199146,
115.547989903385)) ;
#165653=CARTESIAN_POINT('Ctrl Pts',(-19.3301101843111,-14.4836080857303,
115.267628373719)) ;
#165654=CARTESIAN_POINT('Ctrl Pts',(-19.334755451989,-14.409178476904,115.281777110546)) ;
#165655=CARTESIAN_POINT('Ctrl Pts',(-19.4085592797642,-14.4091784657996,
115.257546021209)) ;
#165656=CARTESIAN_POINT('Ctrl Pts',(-19.4823631075395,-14.4091784546952,
115.233314931872)) ;
#165657=CARTESIAN_POINT('Ctrl Pts',(-19.4777178398616,-14.4836080635215,
115.219166195045)) ;
#165658=CARTESIAN_POINT('Ctrl Pts',(-19.4730725721837,-14.5580376723478,
115.205017458217)) ;
#165659=CARTESIAN_POINT('Ctrl Pts',(-19.3992687444084,-14.5580376834522,
115.229248547554)) ;
#165660=CARTESIAN_POINT('Ctrl Pts',(-19.3254649166332,-14.5580376945566,
115.253479636892)) ;
#165661=CARTESIAN_POINT('Ctrl Pts',(-19.3301101843111,-14.4836080857303,
115.267628373719)) ;
#165662=CARTESIAN_POINT('Ctrl Pts',(-19.2551325732941,-14.3877127605132,
115.003913883089)) ;
#165663=CARTESIAN_POINT('Ctrl Pts',(-19.2657513147536,-14.319866136678,
115.036256857093)) ;
#165664=CARTESIAN_POINT('Ctrl Pts',(-19.3395551461189,-14.3198661161146,
115.01202577869)) ;
#165665=CARTESIAN_POINT('Ctrl Pts',(-19.4133589774841,-14.3198660955512,
114.987794700287)) ;
#165666=CARTESIAN_POINT('Ctrl Pts',(-19.4027402360246,-14.3877127193864,
114.955451726283)) ;
#165667=CARTESIAN_POINT('Ctrl Pts',(-19.392121494565,-14.4555593432216,
114.923108752279)) ;
#165668=CARTESIAN_POINT('Ctrl Pts',(-19.3183176631998,-14.455559363785,
114.947339830682)) ;
#165669=CARTESIAN_POINT('Ctrl Pts',(-19.2445138318345,-14.4555593843484,
114.971570909085)) ;
#165670=CARTESIAN_POINT('Ctrl Pts',(-19.2551325732941,-14.3877127605132,
115.003913883089)) ;
#165671=CARTESIAN_POINT('Ctrl Pts',(-19.1906766261937,-14.2212524561287,
114.77196540951)) ;
#165672=CARTESIAN_POINT('Ctrl Pts',(-19.2065492806211,-14.1649252203371,
114.820310954501)) ;
#165673=CARTESIAN_POINT('Ctrl Pts',(-19.280353116469,-14.1649251971047,
114.796079889752)) ;
#165674=CARTESIAN_POINT('Ctrl Pts',(-19.3541569523169,-14.1649251738723,
114.771848825002)) ;
#165675=CARTESIAN_POINT('Ctrl Pts',(-19.3382842978895,-14.2212524096639,
114.723503280012)) ;
#165676=CARTESIAN_POINT('Ctrl Pts',(-19.3224116434621,-14.2775796454555,
114.675157735021)) ;
#165677=CARTESIAN_POINT('Ctrl Pts',(-19.2486078076142,-14.2775796686879,
114.69938879977)) ;
#165678=CARTESIAN_POINT('Ctrl Pts',(-19.1748039717663,-14.2775796919203,
114.723619864519)) ;
#165679=CARTESIAN_POINT('Ctrl Pts',(-19.1906766261937,-14.2212524561287,
114.77196540951)) ;
#165680=CARTESIAN_POINT('Ctrl Pts',(-19.1431008734099,-13.9987538981264,
114.591734960995)) ;
#165681=CARTESIAN_POINT('Ctrl Pts',(-19.1630503294408,-13.9578771653023,
114.652497785746)) ;
#165682=CARTESIAN_POINT('Ctrl Pts',(-19.2368541686022,-13.9578771425154,
114.628266731089)) ;
#165683=CARTESIAN_POINT('Ctrl Pts',(-19.3106580077636,-13.9578771197285,
114.604035676433)) ;
#165684=CARTESIAN_POINT('Ctrl Pts',(-19.2907085517327,-13.9987538525526,
114.543272851682)) ;
#165685=CARTESIAN_POINT('Ctrl Pts',(-19.2707590957019,-14.0396305853768,
114.482510026931)) ;
#165686=CARTESIAN_POINT('Ctrl Pts',(-19.1969552565404,-14.0396306081637,
114.506741081588)) ;
#165687=CARTESIAN_POINT('Ctrl Pts',(-19.123151417379,-14.0396306309506,
114.530972136245)) ;
#165688=CARTESIAN_POINT('Ctrl Pts',(-19.1431008734099,-13.9987538981264,
114.591734960995)) ;
#165689=CARTESIAN_POINT('Ctrl Pts',(-19.1158102336092,-13.7338214529053,
114.473123572726)) ;
#165690=CARTESIAN_POINT('Ctrl Pts',(-19.138429846815,-13.7113815142411,
114.542019265248)) ;
#165691=CARTESIAN_POINT('Ctrl Pts',(-19.2122336887546,-13.7113814963311,
114.517788219053)) ;
#165692=CARTESIAN_POINT('Ctrl Pts',(-19.2860375306941,-13.7113814784212,
114.493557172857)) ;
#165693=CARTESIAN_POINT('Ctrl Pts',(-19.2634179174883,-13.7338214170854,
114.424661480336)) ;
#165694=CARTESIAN_POINT('Ctrl Pts',(-19.2407983042824,-13.7562613557496,
114.355765787815)) ;
#165695=CARTESIAN_POINT('Ctrl Pts',(-19.1669944623428,-13.7562613736596,
114.37999683401)) ;
#165696=CARTESIAN_POINT('Ctrl Pts',(-19.0931906204033,-13.7562613915695,
114.404227880205)) ;
#165697=CARTESIAN_POINT('Ctrl Pts',(-19.1158102336092,-13.7338214529053,
114.473123572726)) ;
#165698=CARTESIAN_POINT('Ctrl Pts',(-19.1118129583961,-13.4466916236415,
114.425526047976)) ;
#165699=CARTESIAN_POINT('Ctrl Pts',(-19.1354788504801,-13.4442666484752,
114.497608537013)) ;
#165700=CARTESIAN_POINT('Ctrl Pts',(-19.2092826939799,-13.4442666367421,
114.473377495571)) ;
#165701=CARTESIAN_POINT('Ctrl Pts',(-19.2830865374798,-13.4442666250089,
114.449146454128)) ;
#165702=CARTESIAN_POINT('Ctrl Pts',(-19.2594206453958,-13.4466916001752,
114.377063965091)) ;
#165703=CARTESIAN_POINT('Ctrl Pts',(-19.2357547533118,-13.4491165753415,
114.304981476054)) ;
#165704=CARTESIAN_POINT('Ctrl Pts',(-19.161950909812,-13.4491165870746,
114.329212517497)) ;
#165705=CARTESIAN_POINT('Ctrl Pts',(-19.0881470663121,-13.4491165988078,
114.353443558939)) ;
#165706=CARTESIAN_POINT('Ctrl Pts',(-19.1118129583961,-13.4466916236415,
114.425526047976)) ;
#165707=CARTESIAN_POINT('Ctrl Pts',(-19.1321594034187,-13.1565169960044,
114.451948862421)) ;
#165708=CARTESIAN_POINT('Ctrl Pts',(-19.1551759820499,-13.1743502694123,
114.522053647319)) ;
#165709=CARTESIAN_POINT('Ctrl Pts',(-19.2289798260042,-13.1743502645941,
114.49782260726)) ;
#165710=CARTESIAN_POINT('Ctrl Pts',(-19.3027836699584,-13.174350259776,
114.473591567202)) ;
#165711=CARTESIAN_POINT('Ctrl Pts',(-19.2797670913271,-13.156516986368,
114.403486782303)) ;
#165712=CARTESIAN_POINT('Ctrl Pts',(-19.2567505126958,-13.1386837129601,
114.333381997405)) ;
#165713=CARTESIAN_POINT('Ctrl Pts',(-19.1829466687416,-13.1386837177783,
114.357613037464)) ;
#165714=CARTESIAN_POINT('Ctrl Pts',(-19.1091428247873,-13.1386837225965,
114.381844077522)) ;
#165715=CARTESIAN_POINT('Ctrl Pts',(-19.1321594034187,-13.1565169960044,
114.451948862421)) ;
#165716=CARTESIAN_POINT('Ctrl Pts',(-19.1761811779931,-12.8855146893556,
114.550531779431)) ;
#165717=CARTESIAN_POINT('Ctrl Pts',(-19.1968930602221,-12.9222982070888,
114.613616830858)) ;
#165718=CARTESIAN_POINT('Ctrl Pts',(-19.2706969037714,-12.9222982069282,
114.589385789566)) ;
#165719=CARTESIAN_POINT('Ctrl Pts',(-19.3445007473207,-12.9222982067677,
114.565154748274)) ;
#165720=CARTESIAN_POINT('Ctrl Pts',(-19.3237888650918,-12.8855146890345,
114.502069696848)) ;
#165721=CARTESIAN_POINT('Ctrl Pts',(-19.3030769828629,-12.8487311713013,
114.438984645421)) ;
#165722=CARTESIAN_POINT('Ctrl Pts',(-19.2292731393135,-12.8487311714619,
114.463215686713)) ;
#165723=CARTESIAN_POINT('Ctrl Pts',(-19.1554692957642,-12.8487311716225,
114.487446728005)) ;
#165724=CARTESIAN_POINT('Ctrl Pts',(-19.1761811779931,-12.8855146893556,
114.550531779431)) ;
#165725=CARTESIAN_POINT('Ctrl Pts',(-19.2412304209422,-12.6534167842388,
114.713260927411)) ;
#165726=CARTESIAN_POINT('Ctrl Pts',(-19.25816354557,-12.7064619703102,114.764836492834)) ;
#165727=CARTESIAN_POINT('Ctrl Pts',(-19.3319673885266,-12.706461972049,
114.740605449737)) ;
#165728=CARTESIAN_POINT('Ctrl Pts',(-19.4057712314832,-12.7064619737879,
114.71637440664)) ;
#165729=CARTESIAN_POINT('Ctrl Pts',(-19.3888381068554,-12.6534167877166,
114.664798841216)) ;
#165730=CARTESIAN_POINT('Ctrl Pts',(-19.3719049822277,-12.6003716016452,
114.613223275793)) ;
#165731=CARTESIAN_POINT('Ctrl Pts',(-19.2981011392711,-12.6003715999064,
114.637454318891)) ;
#165732=CARTESIAN_POINT('Ctrl Pts',(-19.2242972963145,-12.6003715981675,
114.661685361988)) ;
#165733=CARTESIAN_POINT('Ctrl Pts',(-19.2412304209422,-12.6534167842388,
114.713260927411)) ;
#165734=CARTESIAN_POINT('Ctrl Pts',(-19.323368321488,-12.475742126735,114.928074488961)) ;
#165735=CARTESIAN_POINT('Ctrl Pts',(-19.3353229050844,-12.5412726842435,
114.964486221662)) ;
#165736=CARTESIAN_POINT('Ctrl Pts',(-19.4091267475277,-12.5412726859999,
114.940255177002)) ;
#165737=CARTESIAN_POINT('Ctrl Pts',(-19.4829305899709,-12.5412726877563,
114.916024132341)) ;
#165738=CARTESIAN_POINT('Ctrl Pts',(-19.4709760063745,-12.4757421302478,
114.87961239964)) ;
#165739=CARTESIAN_POINT('Ctrl Pts',(-19.4590214227781,-12.4102115727394,
114.843200666939)) ;
#165740=CARTESIAN_POINT('Ctrl Pts',(-19.3852175803349,-12.410211570983,
114.8674317116)) ;
#165741=CARTESIAN_POINT('Ctrl Pts',(-19.3114137378916,-12.4102115692266,
114.89166275626)) ;
#165742=CARTESIAN_POINT('Ctrl Pts',(-19.323368321488,-12.475742126735,114.928074488961)) ;
#165743=CARTESIAN_POINT('Ctrl Pts',(-19.4186665635696,-12.3646792210001,
115.18260181179)) ;
#165744=CARTESIAN_POINT('Ctrl Pts',(-19.4247236549107,-12.438062944576,
115.201050734672)) ;
#165745=CARTESIAN_POINT('Ctrl Pts',(-19.4985274977625,-12.4380629448186,
115.176819691256)) ;
#165746=CARTESIAN_POINT('Ctrl Pts',(-19.5723313406143,-12.4380629450611,
115.152588647839)) ;
#165747=CARTESIAN_POINT('Ctrl Pts',(-19.5662742492732,-12.3646792214852,
115.134139724957)) ;
#165748=CARTESIAN_POINT('Ctrl Pts',(-19.5602171579321,-12.2912954979092,
115.115690802074)) ;
#165749=CARTESIAN_POINT('Ctrl Pts',(-19.4864133150803,-12.2912954976667,
115.13992184549)) ;
#165750=CARTESIAN_POINT('Ctrl Pts',(-19.4126094722285,-12.2912954974242,
115.164152888907)) ;
#165751=CARTESIAN_POINT('Ctrl Pts',(-19.4186665635696,-12.3646792210001,
115.18260181179)) ;
#165752=CARTESIAN_POINT('Ctrl Pts',(-19.5188634349595,-12.33019827638,115.452501593325)) ;
#165753=CARTESIAN_POINT('Ctrl Pts',(-19.518663256346,-12.4060967099992,
115.451891881587)) ;
#165754=CARTESIAN_POINT('Ctrl Pts',(-19.5924671000764,-12.4060967096592,
115.427660840847)) ;
#165755=CARTESIAN_POINT('Ctrl Pts',(-19.6662709438068,-12.4060967093193,
115.403429800107)) ;
#165756=CARTESIAN_POINT('Ctrl Pts',(-19.6664711224204,-12.3301982757,115.404039511845)) ;
#165757=CARTESIAN_POINT('Ctrl Pts',(-19.6666713010339,-12.2542998420808,
115.404649223583)) ;
#165758=CARTESIAN_POINT('Ctrl Pts',(-19.5928674573034,-12.2542998424208,
115.428880264323)) ;
#165759=CARTESIAN_POINT('Ctrl Pts',(-19.519063613573,-12.2542998427607,
115.453111305064)) ;
#165760=CARTESIAN_POINT('Ctrl Pts',(-19.5188634349595,-12.33019827638,115.452501593325)) ;
#165761=CARTESIAN_POINT('Ctrl Pts',(-19.6194233101362,-12.3732244526573,
115.723247147594)) ;
#165762=CARTESIAN_POINT('Ctrl Pts',(-19.6129366875966,-12.4462297114867,
115.703489942071)) ;
#165763=CARTESIAN_POINT('Ctrl Pts',(-19.6867405329009,-12.4462297127272,
115.679258906124)) ;
#165764=CARTESIAN_POINT('Ctrl Pts',(-19.7605443782052,-12.4462297139677,
115.655027870178)) ;
#165765=CARTESIAN_POINT('Ctrl Pts',(-19.7670310007448,-12.3732244551383,
115.674785075701)) ;
#165766=CARTESIAN_POINT('Ctrl Pts',(-19.7735176232844,-12.300219196309,
115.694542281225)) ;
#165767=CARTESIAN_POINT('Ctrl Pts',(-19.6997137779801,-12.3002191950685,
115.718773317171)) ;
#165768=CARTESIAN_POINT('Ctrl Pts',(-19.6259099326758,-12.300219193828,
115.743004353118)) ;
#165769=CARTESIAN_POINT('Ctrl Pts',(-19.6194233101362,-12.3732244526573,
115.723247147594)) ;
#165770=CARTESIAN_POINT('Ctrl Pts',(-19.7127947734479,-12.4909980427198,
115.972246654781)) ;
#165771=CARTESIAN_POINT('Ctrl Pts',(-19.700511630848,-12.5558859351168,
115.93483418453)) ;
#165772=CARTESIAN_POINT('Ctrl Pts',(-19.7743154775138,-12.555885940904,
115.910603152731)) ;
#165773=CARTESIAN_POINT('Ctrl Pts',(-19.8481193241796,-12.5558859466913,
115.886372120931)) ;
#165774=CARTESIAN_POINT('Ctrl Pts',(-19.8604024667795,-12.4909980542943,
115.923784591182)) ;
#165775=CARTESIAN_POINT('Ctrl Pts',(-19.8726856093794,-12.4261101618973,
115.961197061433)) ;
#165776=CARTESIAN_POINT('Ctrl Pts',(-19.7988817627136,-12.4261101561101,
115.985428093232)) ;
#165777=CARTESIAN_POINT('Ctrl Pts',(-19.7250779160477,-12.4261101503228,
116.009659125032)) ;
#165778=CARTESIAN_POINT('Ctrl Pts',(-19.7127947734479,-12.4909980427198,
115.972246654781)) ;
#165779=CARTESIAN_POINT('Ctrl Pts',(-19.793610933256,-12.67497986033,116.182961362968)) ;
#165780=CARTESIAN_POINT('Ctrl Pts',(-19.7764005017003,-12.7271157689749,
116.130541165705)) ;
#165781=CARTESIAN_POINT('Ctrl Pts',(-19.8502043492699,-12.727115782205,
116.106310136658)) ;
#165782=CARTESIAN_POINT('Ctrl Pts',(-19.9240081968394,-12.7271157954351,
116.082079107611)) ;
#165783=CARTESIAN_POINT('Ctrl Pts',(-19.9412186283951,-12.6749798867901,
116.134499304874)) ;
#165784=CARTESIAN_POINT('Ctrl Pts',(-19.9584290599508,-12.6228439781452,
116.186919502137)) ;
#165785=CARTESIAN_POINT('Ctrl Pts',(-19.8846252123812,-12.6228439649152,
116.211150531184)) ;
#165786=CARTESIAN_POINT('Ctrl Pts',(-19.8108213648117,-12.6228439516851,
116.235381560231)) ;
#165787=CARTESIAN_POINT('Ctrl Pts',(-19.793610933256,-12.67497986033,116.182961362968)) ;
#165788=CARTESIAN_POINT('Ctrl Pts',(-19.8568164214443,-12.9129719673497,
116.339934873997)) ;
#165789=CARTESIAN_POINT('Ctrl Pts',(-19.8359033043558,-12.9485664184321,
116.276236894194)) ;
#165790=CARTESIAN_POINT('Ctrl Pts',(-19.909707151925,-12.9485664423294,
116.252005865145)) ;
#165791=CARTESIAN_POINT('Ctrl Pts',(-19.9835109994942,-12.9485664662267,
116.227774836097)) ;
#165792=CARTESIAN_POINT('Ctrl Pts',(-20.0044241165827,-12.9129720151443,
116.291472815901)) ;
#165793=CARTESIAN_POINT('Ctrl Pts',(-20.0253372336711,-12.8773775640619,
116.355170795705)) ;
#165794=CARTESIAN_POINT('Ctrl Pts',(-19.951533386102,-12.8773775401646,
116.379401824753)) ;
#165795=CARTESIAN_POINT('Ctrl Pts',(-19.8777295385328,-12.8773775162673,
116.403632853801)) ;
#165796=CARTESIAN_POINT('Ctrl Pts',(-19.8568164214443,-12.9129719673497,
116.339934873997)) ;
#165797=CARTESIAN_POINT('Ctrl Pts',(-19.8982594904765,-13.1860117694584,
116.43078023)) ;
#165798=CARTESIAN_POINT('Ctrl Pts',(-19.8751548018971,-13.2025937727261,
116.360407077191)) ;
#165799=CARTESIAN_POINT('Ctrl Pts',(-19.9489586478412,-13.2025938067603,
116.336176043193)) ;
#165800=CARTESIAN_POINT('Ctrl Pts',(-20.0227624937853,-13.2025938407946,
116.311945009195)) ;
#165801=CARTESIAN_POINT('Ctrl Pts',(-20.0458671823647,-13.1860118375269,
116.382318162004)) ;
#165802=CARTESIAN_POINT('Ctrl Pts',(-20.0689718709441,-13.1694298342593,
116.452691314813)) ;
#165803=CARTESIAN_POINT('Ctrl Pts',(-19.995168025,-13.169429800225,116.476922348811)) ;
#165804=CARTESIAN_POINT('Ctrl Pts',(-19.9213641790559,-13.1694297661908,
116.501153382809)) ;
#165805=CARTESIAN_POINT('Ctrl Pts',(-19.8982594904765,-13.1860117694584,
116.43078023)) ;
#165806=CARTESIAN_POINT('Ctrl Pts',(-19.9161358077784,-13.4763914936473,
116.449746710291)) ;
#165807=CARTESIAN_POINT('Ctrl Pts',(-19.8924837990799,-13.4727232020181,
116.377706508879)) ;
#165808=CARTESIAN_POINT('Ctrl Pts',(-19.9662876420239,-13.4727232458184,
116.353475465744)) ;
#165809=CARTESIAN_POINT('Ctrl Pts',(-20.040091484968,-13.4727232896187,
116.329244422608)) ;
#165810=CARTESIAN_POINT('Ctrl Pts',(-20.0637434936665,-13.4763915812479,
116.40128462402)) ;
#165811=CARTESIAN_POINT('Ctrl Pts',(-20.087395502365,-13.4800598728771,
116.473324825431)) ;
#165812=CARTESIAN_POINT('Ctrl Pts',(-20.0135916594209,-13.4800598290768,
116.497555868567)) ;
#165813=CARTESIAN_POINT('Ctrl Pts',(-19.9397878164769,-13.4800597852765,
116.521786911702)) ;
#165814=CARTESIAN_POINT('Ctrl Pts',(-19.9161358077784,-13.4763914936473,
116.449746710291)) ;
#165815=CARTESIAN_POINT('Ctrl Pts',(-19.9095920128141,-13.7633156829476,
116.394237436287)) ;
#165816=CARTESIAN_POINT('Ctrl Pts',(-19.887098792294,-13.7396092222064,
116.325726716888)) ;
#165817=CARTESIAN_POINT('Ctrl Pts',(-19.9609026306121,-13.7396092733025,
116.301495659662)) ;
#165818=CARTESIAN_POINT('Ctrl Pts',(-20.0347064689303,-13.7396093243987,
116.277264602437)) ;
#165819=CARTESIAN_POINT('Ctrl Pts',(-20.0571996894504,-13.7633157851398,
116.345775321837)) ;
#165820=CARTESIAN_POINT('Ctrl Pts',(-20.0796929099706,-13.787022245881,
116.414286041237)) ;
#165821=CARTESIAN_POINT('Ctrl Pts',(-20.0058890716524,-13.7870221947849,
116.438517098462)) ;
#165822=CARTESIAN_POINT('Ctrl Pts',(-19.9320852333342,-13.7870221436888,
116.462748155687)) ;
#165823=CARTESIAN_POINT('Ctrl Pts',(-19.9095920128141,-13.7633156829476,
116.394237436287)) ;
#165824=CARTESIAN_POINT('Ctrl Pts',(-19.8801111722998,-14.0239605605361,
116.269074441211)) ;
#165825=CARTESIAN_POINT('Ctrl Pts',(-19.8603756897852,-13.9820221332016,
116.208963346964)) ;
#165826=CARTESIAN_POINT('Ctrl Pts',(-19.9341795227265,-13.9820221845115,
116.184732273362)) ;
#165827=CARTESIAN_POINT('Ctrl Pts',(-20.0079833556679,-13.9820222358214,
116.16050119976)) ;
#165828=CARTESIAN_POINT('Ctrl Pts',(-20.0277188381826,-14.023960663156,
116.220612294007)) ;
#165829=CARTESIAN_POINT('Ctrl Pts',(-20.0474543206972,-14.0658990904905,
116.280723388254)) ;
#165830=CARTESIAN_POINT('Ctrl Pts',(-19.9736504877559,-14.0658990391806,
116.304954461856)) ;
#165831=CARTESIAN_POINT('Ctrl Pts',(-19.8998466548145,-14.0658989878706,
116.329185535458)) ;
#165832=CARTESIAN_POINT('Ctrl Pts',(-19.8801111722998,-14.0239605605361,
116.269074441211)) ;
#165833=CARTESIAN_POINT('Ctrl Pts',(-19.8302954553483,-14.2421936446632,
116.081819032021)) ;
#165834=CARTESIAN_POINT('Ctrl Pts',(-19.8147444706435,-14.1849578741807,
116.034453243106)) ;
#165835=CARTESIAN_POINT('Ctrl Pts',(-19.8885482976305,-14.1849579203882,
116.010222151368)) ;
#165836=CARTESIAN_POINT('Ctrl Pts',(-19.9623521246174,-14.1849579665956,
115.98599105963)) ;
#165837=CARTESIAN_POINT('Ctrl Pts',(-19.9779031093222,-14.2421937370781,
116.033356848544)) ;
#165838=CARTESIAN_POINT('Ctrl Pts',(-19.9934540940269,-14.2994295075606,
116.080722637459)) ;
#165839=CARTESIAN_POINT('Ctrl Pts',(-19.91965026704,-14.2994294613532,116.104953729197)) ;
#165840=CARTESIAN_POINT('Ctrl Pts',(-19.8458464400531,-14.2994294151457,
116.129184820935)) ;
#165841=CARTESIAN_POINT('Ctrl Pts',(-19.8302954553483,-14.2421936446632,
116.081819032021)) ;
#165842=CARTESIAN_POINT('Ctrl Pts',(-19.7649637327425,-14.4005934040497,
115.847505400487)) ;
#165843=CARTESIAN_POINT('Ctrl Pts',(-19.7546825121778,-14.3322159891563,
115.816190462997)) ;
#165844=CARTESIAN_POINT('Ctrl Pts',(-19.8284863340784,-14.3322160226317,
115.791959355766)) ;
#165845=CARTESIAN_POINT('Ctrl Pts',(-19.902290155979,-14.332216056107,115.767728248536)) ;
#165846=CARTESIAN_POINT('Ctrl Pts',(-19.9125713765437,-14.4005934710005,
115.799043186026)) ;
#165847=CARTESIAN_POINT('Ctrl Pts',(-19.9228525971083,-14.4689708858939,
115.830358123516)) ;
#165848=CARTESIAN_POINT('Ctrl Pts',(-19.8490487752077,-14.4689708524185,
115.854589230747)) ;
#165849=CARTESIAN_POINT('Ctrl Pts',(-19.7752449533071,-14.4689708189432,
115.878820337977)) ;
#165850=CARTESIAN_POINT('Ctrl Pts',(-19.7649637327425,-14.4005934040497,
115.847505400487)) ;
#165851=CARTESIAN_POINT('Ctrl Pts',(-19.6886669174365,-14.4895021228897,
115.579514611263)) ;
#165852=CARTESIAN_POINT('Ctrl Pts',(-19.6844341898727,-14.4148177682025,
115.566622407693)) ;
#165853=CARTESIAN_POINT('Ctrl Pts',(-19.7582380072419,-14.4148177835068,
115.542391286661)) ;
#165854=CARTESIAN_POINT('Ctrl Pts',(-19.8320418246112,-14.4148177988111,
115.518160165629)) ;
#165855=CARTESIAN_POINT('Ctrl Pts',(-19.836274552175,-14.4895021534983,
115.531052369199)) ;
#165856=CARTESIAN_POINT('Ctrl Pts',(-19.8405072797388,-14.5641865081855,
115.54394457277)) ;
#165857=CARTESIAN_POINT('Ctrl Pts',(-19.7667034623695,-14.5641864928812,
115.568175693802)) ;
#165858=CARTESIAN_POINT('Ctrl Pts',(-19.6928996450003,-14.5641864775769,
115.592406814834)) ;
#165859=CARTESIAN_POINT('Ctrl Pts',(-19.6886669174365,-14.4895021228897,
115.579514611263)) ;
#165860=CARTESIAN_POINT('Ctrl Pts',(-19.6086131782422,-14.5012817728617,
115.300312081332)) ;
#165861=CARTESIAN_POINT('Ctrl Pts',(-19.6106952959586,-14.425666653241,
115.306653877699)) ;
#165862=CARTESIAN_POINT('Ctrl Pts',(-19.6844991112022,-14.4256666452889,
115.282422750192)) ;
#165863=CARTESIAN_POINT('Ctrl Pts',(-19.7583029264457,-14.4256666373369,
115.258191622685)) ;
#165864=CARTESIAN_POINT('Ctrl Pts',(-19.7562208087292,-14.5012817569575,
115.251849826318)) ;
#165865=CARTESIAN_POINT('Ctrl Pts',(-19.7541386910127,-14.5768968765781,
115.245508029951)) ;
#165866=CARTESIAN_POINT('Ctrl Pts',(-19.6803348757692,-14.5768968845302,
115.269739157458)) ;
#165867=CARTESIAN_POINT('Ctrl Pts',(-19.6065310605257,-14.5768968924823,
115.293970284964)) ;
#165868=CARTESIAN_POINT('Ctrl Pts',(-19.6086131782422,-14.5012817728617,
115.300312081332)) ;
#165869=CARTESIAN_POINT('Ctrl Pts',(-19.5302683146018,-14.43501211062,115.026040039372)) ;
#165870=CARTESIAN_POINT('Ctrl Pts',(-19.5385607693486,-14.363912820796,
115.051297520427)) ;
#165871=CARTESIAN_POINT('Ctrl Pts',(-19.6123645843789,-14.3639127866614,
115.027066392271)) ;
#165872=CARTESIAN_POINT('Ctrl Pts',(-19.6861683994091,-14.3639127525269,
115.002835264114)) ;
#165873=CARTESIAN_POINT('Ctrl Pts',(-19.6778759446623,-14.4350120423509,
114.97757778306)) ;
#165874=CARTESIAN_POINT('Ctrl Pts',(-19.6695834899155,-14.506111332175,
114.952320302005)) ;
#165875=CARTESIAN_POINT('Ctrl Pts',(-19.5957796748852,-14.5061113663095,
114.976551430162)) ;
#165876=CARTESIAN_POINT('Ctrl Pts',(-19.521975859855,-14.5061114004441,
115.000782558318)) ;
#165877=CARTESIAN_POINT('Ctrl Pts',(-19.5302683146018,-14.43501211062,115.026040039372)) ;
#165878=CARTESIAN_POINT('Ctrl Pts',(-19.4613020602763,-14.2968843843662,
114.780704827686)) ;
#165879=CARTESIAN_POINT('Ctrl Pts',(-19.4751514840979,-14.2353253070851,
114.822887939996)) ;
#165880=CARTESIAN_POINT('Ctrl Pts',(-19.5489553020923,-14.2353252479564,
114.798656820868)) ;
#165881=CARTESIAN_POINT('Ctrl Pts',(-19.6227591200867,-14.2353251888277,
114.77442570174)) ;
#165882=CARTESIAN_POINT('Ctrl Pts',(-19.6089096962652,-14.2968842661087,
114.732242589431)) ;
#165883=CARTESIAN_POINT('Ctrl Pts',(-19.5950602724436,-14.3584433433898,
114.690059477121)) ;
#165884=CARTESIAN_POINT('Ctrl Pts',(-19.5212564544492,-14.3584434025185,
114.714290596249)) ;
#165885=CARTESIAN_POINT('Ctrl Pts',(-19.4474526364548,-14.3584434616473,
114.738521715376)) ;
#165886=CARTESIAN_POINT('Ctrl Pts',(-19.4613020602763,-14.2968843843662,
114.780704827686)) ;
#165887=CARTESIAN_POINT('Ctrl Pts',(-19.4062019880191,-14.0952651274861,
114.577384783976)) ;
#165888=CARTESIAN_POINT('Ctrl Pts',(-19.4246530089548,-14.0476919571474,
114.633583618702)) ;
#165889=CARTESIAN_POINT('Ctrl Pts',(-19.4984568320329,-14.0476918755957,
114.609352515058)) ;
#165890=CARTESIAN_POINT('Ctrl Pts',(-19.5722606551109,-14.047691794044,
114.585121411415)) ;
#165891=CARTESIAN_POINT('Ctrl Pts',(-19.5538096341753,-14.0952649643827,
114.528922576688)) ;
#165892=CARTESIAN_POINT('Ctrl Pts',(-19.5353586132396,-14.1428381347214,
114.472723741961)) ;
#165893=CARTESIAN_POINT('Ctrl Pts',(-19.4615547901615,-14.1428382162731,
114.496954845605)) ;
#165894=CARTESIAN_POINT('Ctrl Pts',(-19.3877509670834,-14.1428382978248,
114.521185949249)) ;
#165895=CARTESIAN_POINT('Ctrl Pts',(-19.4062019880191,-14.0952651274861,
114.577384783976)) ;
#165896=CARTESIAN_POINT('Ctrl Pts',(-19.3702132925559,-13.8453444760412,
114.432330882525)) ;
#165897=CARTESIAN_POINT('Ctrl Pts',(-19.3919372890595,-13.8151498849244,
114.498498672785)) ;
#165898=CARTESIAN_POINT('Ctrl Pts',(-19.4657411193459,-13.8151497867456,
114.474267591096)) ;
#165899=CARTESIAN_POINT('Ctrl Pts',(-19.5395449496322,-13.8151496885667,
114.450036509408)) ;
#165900=CARTESIAN_POINT('Ctrl Pts',(-19.5178209531287,-13.8453442796835,
114.383868719148)) ;
#165901=CARTESIAN_POINT('Ctrl Pts',(-19.4960969566251,-13.8755388708002,
114.317700928887)) ;
#165902=CARTESIAN_POINT('Ctrl Pts',(-19.4222931263387,-13.8755389689791,
114.341932010576)) ;
#165903=CARTESIAN_POINT('Ctrl Pts',(-19.3484892960523,-13.8755390671579,
114.366163092264)) ;
#165904=CARTESIAN_POINT('Ctrl Pts',(-19.3702132925559,-13.8453444760412,
114.432330882525)) ;
#165905=CARTESIAN_POINT('Ctrl Pts',(-19.356514093291,-13.5639203016943,
114.355047993229)) ;
#165906=CARTESIAN_POINT('Ctrl Pts',(-19.3799623708669,-13.5533288537195,
114.426467665453)) ;
#165907=CARTESIAN_POINT('Ctrl Pts',(-19.4537662097389,-13.5533287463832,
114.402236609915)) ;
#165908=CARTESIAN_POINT('Ctrl Pts',(-19.5275700486109,-13.5533286390469,
114.378005554377)) ;
#165909=CARTESIAN_POINT('Ctrl Pts',(-19.504121771035,-13.5639200870216,
114.306585882153)) ;
#165910=CARTESIAN_POINT('Ctrl Pts',(-19.4806734934592,-13.5745115349964,
114.235166209929)) ;
#165911=CARTESIAN_POINT('Ctrl Pts',(-19.4068696545872,-13.5745116423327,
114.259397265467)) ;
#165912=CARTESIAN_POINT('Ctrl Pts',(-19.3330658157152,-13.574511749669,
114.283628321005)) ;
#165913=CARTESIAN_POINT('Ctrl Pts',(-19.356514093291,-13.5639203016943,
114.355047993229)) ;
#165914=CARTESIAN_POINT('Ctrl Pts',(-19.3670894957072,-13.2722319962961,
114.351731726315)) ;
#165915=CARTESIAN_POINT('Ctrl Pts',(-19.3905693400295,-13.2819894198182,
114.423247545754)) ;
#165916=CARTESIAN_POINT('Ctrl Pts',(-19.4643731879902,-13.2819893125246,
114.399016517899)) ;
#165917=CARTESIAN_POINT('Ctrl Pts',(-19.538177035951,-13.281989205231,114.374785490044)) ;
#165918=CARTESIAN_POINT('Ctrl Pts',(-19.5146971916288,-13.2722317817088,
114.303269670605)) ;
#165919=CARTESIAN_POINT('Ctrl Pts',(-19.4912173473065,-13.2624743581867,
114.231753851165)) ;
#165920=CARTESIAN_POINT('Ctrl Pts',(-19.4174134993458,-13.2624744654803,
114.255984879021)) ;
#165921=CARTESIAN_POINT('Ctrl Pts',(-19.343609651385,-13.262474572774,114.280215906876)) ;
#165922=CARTESIAN_POINT('Ctrl Pts',(-19.3670894957072,-13.2722319962961,
114.351731726315)) ;
#165923=CARTESIAN_POINT('Ctrl Pts',(-19.4014893907637,-12.9927108288244,
114.421205255979)) ;
#165924=CARTESIAN_POINT('Ctrl Pts',(-19.4233327297624,-13.0219980101555,
114.487736544236)) ;
#165925=CARTESIAN_POINT('Ctrl Pts',(-19.4971365863264,-13.0219979113137,
114.463505542585)) ;
#165926=CARTESIAN_POINT('Ctrl Pts',(-19.5709404428904,-13.0219978124719,
114.439274540934)) ;
#165927=CARTESIAN_POINT('Ctrl Pts',(-19.5490971038917,-12.9927106311408,
114.372743252677)) ;
#165928=CARTESIAN_POINT('Ctrl Pts',(-19.527253764893,-12.9634234498097,
114.306211964419)) ;
#165929=CARTESIAN_POINT('Ctrl Pts',(-19.453449908329,-12.9634235486515,
114.330442966071)) ;
#165930=CARTESIAN_POINT('Ctrl Pts',(-19.379646051765,-12.9634236474933,
114.354673967722)) ;
#165931=CARTESIAN_POINT('Ctrl Pts',(-19.4014893907637,-12.9927108288244,
114.421205255979)) ;
#165932=CARTESIAN_POINT('Ctrl Pts',(-19.4584767230081,-12.7419081122581,
114.559249348352)) ;
#165933=CARTESIAN_POINT('Ctrl Pts',(-19.4771091783895,-12.7887491311702,
114.616000803142)) ;
#165934=CARTESIAN_POINT('Ctrl Pts',(-19.5509130422714,-12.78874904886,114.591769823781)) ;
#165935=CARTESIAN_POINT('Ctrl Pts',(-19.6247169061534,-12.7887489665498,
114.567538844419)) ;
#165936=CARTESIAN_POINT('Ctrl Pts',(-19.606084450772,-12.7419079476376,
114.510787389628)) ;
#165937=CARTESIAN_POINT('Ctrl Pts',(-19.5874519953906,-12.6950669287254,
114.454035934838)) ;
#165938=CARTESIAN_POINT('Ctrl Pts',(-19.5136481315087,-12.6950670110357,
114.4782669142)) ;
#165939=CARTESIAN_POINT('Ctrl Pts',(-19.4398442676267,-12.6950670933459,
114.502497893561)) ;
#165940=CARTESIAN_POINT('Ctrl Pts',(-19.4584767230081,-12.7419081122581,
114.559249348352)) ;
#165941=CARTESIAN_POINT('Ctrl Pts',(-19.5343623620457,-12.5402274188012,
114.754960677607)) ;
#165942=CARTESIAN_POINT('Ctrl Pts',(-19.5484574986284,-12.6012191381552,
114.797892191371)) ;
#165943=CARTESIAN_POINT('Ctrl Pts',(-19.6222613678262,-12.6012190780927,
114.773661228201)) ;
#165944=CARTESIAN_POINT('Ctrl Pts',(-19.6960652370241,-12.6012190180302,
114.74943026503)) ;
#165945=CARTESIAN_POINT('Ctrl Pts',(-19.6819701004414,-12.5402272986761,
114.706498751266)) ;
#165946=CARTESIAN_POINT('Ctrl Pts',(-19.6678749638587,-12.479235579322,
114.663567237502)) ;
#165947=CARTESIAN_POINT('Ctrl Pts',(-19.5940710946608,-12.4792356393845,
114.687798200673)) ;
#165948=CARTESIAN_POINT('Ctrl Pts',(-19.520267225463,-12.4792356994471,
114.712029163843)) ;
#165949=CARTESIAN_POINT('Ctrl Pts',(-19.5343623620457,-12.5402274188012,
114.754960677607)) ;
#165950=CARTESIAN_POINT('Ctrl Pts',(-19.624777106285,-12.4011175779625,
114.994845960025)) ;
#165951=CARTESIAN_POINT('Ctrl Pts',(-19.6333154990108,-12.4719130809355,
115.020852528492)) ;
#165952=CARTESIAN_POINT('Ctrl Pts',(-19.707119370965,-12.4719130465785,
114.996621573717)) ;
#165953=CARTESIAN_POINT('Ctrl Pts',(-19.7809232429191,-12.4719130122216,
114.972390618941)) ;
#165954=CARTESIAN_POINT('Ctrl Pts',(-19.7723848501933,-12.4011175092485,
114.946384050474)) ;
#165955=CARTESIAN_POINT('Ctrl Pts',(-19.7638464574675,-12.3303220062755,
114.920377482007)) ;
#165956=CARTESIAN_POINT('Ctrl Pts',(-19.6900425855133,-12.3303220406325,
114.944608436782)) ;
#165957=CARTESIAN_POINT('Ctrl Pts',(-19.6162387135592,-12.3303220749894,
114.968839391557)) ;
#165958=CARTESIAN_POINT('Ctrl Pts',(-19.624777106285,-12.4011175779625,
114.994845960025)) ;
#165959=CARTESIAN_POINT('Ctrl Pts',(-19.7234667624237,-12.3349520470046,
115.260072553625)) ;
#165960=CARTESIAN_POINT('Ctrl Pts',(-19.7258594391485,-12.4104731774987,
115.267360262672)) ;
#165961=CARTESIAN_POINT('Ctrl Pts',(-19.7996633114999,-12.4104731691892,
115.243129309107)) ;
#165962=CARTESIAN_POINT('Ctrl Pts',(-19.8734671838513,-12.4104731608796,
115.218898355542)) ;
#165963=CARTESIAN_POINT('Ctrl Pts',(-19.8710745071266,-12.3349520303855,
115.211610646495)) ;
#165964=CARTESIAN_POINT('Ctrl Pts',(-19.8686818304018,-12.2594308998913,
115.204322937447)) ;
#165965=CARTESIAN_POINT('Ctrl Pts',(-19.7948779580504,-12.2594309082008,
115.228553891012)) ;
#165966=CARTESIAN_POINT('Ctrl Pts',(-19.7210740856989,-12.2594309165104,
115.252784844578)) ;
#165967=CARTESIAN_POINT('Ctrl Pts',(-19.7234667624237,-12.3349520470046,
115.260072553625)) ;
#165968=CARTESIAN_POINT('Ctrl Pts',(-19.8252582804317,-12.346456548631,
115.534462410052)) ;
#165969=CARTESIAN_POINT('Ctrl Pts',(-19.8212853892728,-12.4212888141347,
115.522361626262)) ;
#165970=CARTESIAN_POINT('Ctrl Pts',(-19.8950892589879,-12.4212888296186,
115.498130664667)) ;
#165971=CARTESIAN_POINT('Ctrl Pts',(-19.9688931287029,-12.4212888451025,
115.473899703072)) ;
#165972=CARTESIAN_POINT('Ctrl Pts',(-19.9728660198618,-12.3464565795988,
115.486000486862)) ;
#165973=CARTESIAN_POINT('Ctrl Pts',(-19.9768389110207,-12.2716243140951,
115.498101270651)) ;
#165974=CARTESIAN_POINT('Ctrl Pts',(-19.9030350413057,-12.2716242986112,
115.522332232247)) ;
#165975=CARTESIAN_POINT('Ctrl Pts',(-19.8292311715906,-12.2716242831273,
115.546563193842)) ;
#165976=CARTESIAN_POINT('Ctrl Pts',(-19.8252582804317,-12.346456548631,
115.534462410052)) ;
#165977=CARTESIAN_POINT('Ctrl Pts',(-19.9219904763792,-12.4344867986536,
115.793753215516)) ;
#165978=CARTESIAN_POINT('Ctrl Pts',(-19.9119891025516,-12.5032854856229,
115.763290646093)) ;
#165979=CARTESIAN_POINT('Ctrl Pts',(-19.9857929683466,-12.5032855202655,
115.739059672558)) ;
#165980=CARTESIAN_POINT('Ctrl Pts',(-20.0595968341415,-12.503285554908,
115.714828699023)) ;
#165981=CARTESIAN_POINT('Ctrl Pts',(-20.0695982079691,-12.4344868679388,
115.745291268445)) ;
#165982=CARTESIAN_POINT('Ctrl Pts',(-20.0795995817966,-12.3656881809695,
115.775753837868)) ;
#165983=CARTESIAN_POINT('Ctrl Pts',(-20.0057957160017,-12.365688146327,
115.799984811403)) ;
#165984=CARTESIAN_POINT('Ctrl Pts',(-19.9319918502067,-12.3656881116844,
115.824215784938)) ;
#165985=CARTESIAN_POINT('Ctrl Pts',(-19.9219904763792,-12.4344867986536,
115.793753215516)) ;
#165986=CARTESIAN_POINT('Ctrl Pts',(-20.0087826519236,-12.5932721982848,
116.022595185583)) ;
#165987=CARTESIAN_POINT('Ctrl Pts',(-19.9934412072172,-12.6510887725529,
115.975867621727)) ;
#165988=CARTESIAN_POINT('Ctrl Pts',(-20.0672450674469,-12.6510888198682,
115.95163663124)) ;
#165989=CARTESIAN_POINT('Ctrl Pts',(-20.1410489276766,-12.6510888671835,
115.927405640754)) ;
#165990=CARTESIAN_POINT('Ctrl Pts',(-20.1563903723829,-12.5932722929155,
115.974133204611)) ;
#165991=CARTESIAN_POINT('Ctrl Pts',(-20.1717318170893,-12.5354557186474,
116.020860768468)) ;
#165992=CARTESIAN_POINT('Ctrl Pts',(-20.0979279568596,-12.5354556713321,
116.045091758954)) ;
#165993=CARTESIAN_POINT('Ctrl Pts',(-20.02412409663,-12.5354556240167,116.06932274944)) ;
#165994=CARTESIAN_POINT('Ctrl Pts',(-20.0087826519236,-12.5932721982848,
116.022595185583)) ;
#165995=CARTESIAN_POINT('Ctrl Pts',(-20.0794532739981,-12.8103924299054,
116.202472937064)) ;
#165996=CARTESIAN_POINT('Ctrl Pts',(-20.0598863895537,-12.8531370145114,
116.142875365397)) ;
#165997=CARTESIAN_POINT('Ctrl Pts',(-20.1336902439871,-12.8531370683972,
116.118644357256)) ;
#165998=CARTESIAN_POINT('Ctrl Pts',(-20.2074940984206,-12.8531371222829,
116.094413349116)) ;
#165999=CARTESIAN_POINT('Ctrl Pts',(-20.2270609828651,-12.810392537677,
116.154010920783)) ;
#166000=CARTESIAN_POINT('Ctrl Pts',(-20.2466278673096,-12.767647953071,
116.21360849245)) ;
#166001=CARTESIAN_POINT('Ctrl Pts',(-20.1728240128761,-12.7676478991852,
116.237839500591)) ;
#166002=CARTESIAN_POINT('Ctrl Pts',(-20.0990201584426,-12.7676478452995,
116.262070508731)) ;
#166003=CARTESIAN_POINT('Ctrl Pts',(-20.0794532739981,-12.8103924299054,
116.202472937064)) ;
#166004=CARTESIAN_POINT('Ctrl Pts',(-20.1303453815953,-13.0726323412443,
116.321870495346)) ;
#166005=CARTESIAN_POINT('Ctrl Pts',(-20.107932288737,-13.0971322435792,
116.253603831893)) ;
#166006=CARTESIAN_POINT('Ctrl Pts',(-20.1817361372741,-13.0971322955942,
116.229372805793)) ;
#166007=CARTESIAN_POINT('Ctrl Pts',(-20.2555399858112,-13.0971323476091,
116.205141779694)) ;
#166008=CARTESIAN_POINT('Ctrl Pts',(-20.2779530786695,-13.0726324452743,
116.273408443147)) ;
#166009=CARTESIAN_POINT('Ctrl Pts',(-20.3003661715278,-13.0481325429394,
116.3416751066)) ;
#166010=CARTESIAN_POINT('Ctrl Pts',(-20.2265623229907,-13.0481324909245,
116.3659061327)) ;
#166011=CARTESIAN_POINT('Ctrl Pts',(-20.1527584744536,-13.0481324389095,
116.3901371588)) ;
#166012=CARTESIAN_POINT('Ctrl Pts',(-20.1303453815953,-13.0726323412443,
116.321870495346)) ;
#166013=CARTESIAN_POINT('Ctrl Pts',(-20.1578525019935,-13.3588849654739,
116.370163901629)) ;
#166014=CARTESIAN_POINT('Ctrl Pts',(-20.1342191538104,-13.3634353466295,
116.298180537171)) ;
#166015=CARTESIAN_POINT('Ctrl Pts',(-20.2080229977771,-13.3634353921752,
116.27394949715)) ;
#166016=CARTESIAN_POINT('Ctrl Pts',(-20.2818268417438,-13.3634354377208,
116.24971845713)) ;
#166017=CARTESIAN_POINT('Ctrl Pts',(-20.3054601899268,-13.3588850565651,
116.321701821588)) ;
#166018=CARTESIAN_POINT('Ctrl Pts',(-20.3290935381099,-13.3543346754094,
116.393685186046)) ;
#166019=CARTESIAN_POINT('Ctrl Pts',(-20.2552896941432,-13.3543346298638,
116.417916226066)) ;
#166020=CARTESIAN_POINT('Ctrl Pts',(-20.1814858501765,-13.3543345843182,
116.442147266087)) ;
#166021=CARTESIAN_POINT('Ctrl Pts',(-20.1578525019935,-13.3588849654739,
116.370163901629)) ;
#166022=CARTESIAN_POINT('Ctrl Pts',(-20.1611723681104,-13.6479812710763,
116.344954804695)) ;
#166023=CARTESIAN_POINT('Ctrl Pts',(-20.1380024070174,-13.6323532637261,
116.274382842406)) ;
#166024=CARTESIAN_POINT('Ctrl Pts',(-20.2118062476732,-13.6323533009956,
116.250151792301)) ;
#166025=CARTESIAN_POINT('Ctrl Pts',(-20.285610088329,-13.632353338265,116.225920742195)) ;
#166026=CARTESIAN_POINT('Ctrl Pts',(-20.308780049422,-13.6479813456151,
116.296492704485)) ;
#166027=CARTESIAN_POINT('Ctrl Pts',(-20.331950010515,-13.6636093529653,
116.367064666774)) ;
#166028=CARTESIAN_POINT('Ctrl Pts',(-20.2581461698591,-13.6636093156958,
116.39129571688)) ;
#166029=CARTESIAN_POINT('Ctrl Pts',(-20.1843423292033,-13.6636092784264,
116.415526766985)) ;
#166030=CARTESIAN_POINT('Ctrl Pts',(-20.1611723681104,-13.6479812710763,
116.344954804695)) ;
#166031=CARTESIAN_POINT('Ctrl Pts',(-20.1407285861011,-13.9223253071587,
116.24714907814)) ;
#166032=CARTESIAN_POINT('Ctrl Pts',(-20.1196862628137,-13.8875179705717,
116.183057557135)) ;
#166033=CARTESIAN_POINT('Ctrl Pts',(-20.1934901017956,-13.8875179960034,
116.158826501931)) ;
#166034=CARTESIAN_POINT('Ctrl Pts',(-20.2672939407774,-13.8875180214352,
116.134595446728)) ;
#166035=CARTESIAN_POINT('Ctrl Pts',(-20.2883362640648,-13.9223253580222,
116.198686967732)) ;
#166036=CARTESIAN_POINT('Ctrl Pts',(-20.3093785873523,-13.9571326946092,
116.262778488737)) ;
#166037=CARTESIAN_POINT('Ctrl Pts',(-20.2355747483704,-13.9571326691774,
116.287009543941)) ;
#166038=CARTESIAN_POINT('Ctrl Pts',(-20.1617709093885,-13.9571326437457,
116.311240599144)) ;
#166039=CARTESIAN_POINT('Ctrl Pts',(-20.1407285861011,-13.9223253071587,
116.24714907814)) ;
#166040=CARTESIAN_POINT('Ctrl Pts',(-20.0987741035012,-14.1598247969233,
116.083922230041)) ;
#166041=CARTESIAN_POINT('Ctrl Pts',(-20.0813627450779,-14.1083816279705,
116.030890042007)) ;
#166042=CARTESIAN_POINT('Ctrl Pts',(-20.1551665838028,-14.1083816430256,
116.006658986021)) ;
#166043=CARTESIAN_POINT('Ctrl Pts',(-20.2289704225278,-14.1083816580807,
115.982427930034)) ;
#166044=CARTESIAN_POINT('Ctrl Pts',(-20.2463817809511,-14.1598248270335,
116.035460118068)) ;
#166045=CARTESIAN_POINT('Ctrl Pts',(-20.2637931393744,-14.2112679959863,
116.088492306103)) ;
#166046=CARTESIAN_POINT('Ctrl Pts',(-20.1899893006495,-14.2112679809312,
116.112723362089)) ;
#166047=CARTESIAN_POINT('Ctrl Pts',(-20.1161854619245,-14.2112679658761,
116.136954418075)) ;
#166048=CARTESIAN_POINT('Ctrl Pts',(-20.0987741035012,-14.1598247969233,
116.083922230041)) ;
#166049=CARTESIAN_POINT('Ctrl Pts',(-20.0388440499086,-14.3448019435796,
115.865824123426)) ;
#166050=CARTESIAN_POINT('Ctrl Pts',(-20.0263268379977,-14.2803646984367,
115.827698715844)) ;
#166051=CARTESIAN_POINT('Ctrl Pts',(-20.1001306778157,-14.2803647047343,
115.803467663186)) ;
#166052=CARTESIAN_POINT('Ctrl Pts',(-20.1739345176336,-14.2803647110319,
115.779236610529)) ;
#166053=CARTESIAN_POINT('Ctrl Pts',(-20.1864517295445,-14.3448019561748,
115.817362018112)) ;
#166054=CARTESIAN_POINT('Ctrl Pts',(-20.1989689414554,-14.4092392013176,
115.855487425695)) ;
#166055=CARTESIAN_POINT('Ctrl Pts',(-20.1251651016375,-14.40923919502,115.879718478352)) ;
#166056=CARTESIAN_POINT('Ctrl Pts',(-20.0513612618195,-14.4092391887224,
115.903949531009)) ;
#166057=CARTESIAN_POINT('Ctrl Pts',(-20.0388440499086,-14.3448019435796,
115.865824123426)) ;
#166058=CARTESIAN_POINT('Ctrl Pts',(-19.9663582699684,-14.4625579261475,
115.609608257701)) ;
#166059=CARTESIAN_POINT('Ctrl Pts',(-19.9596169228226,-14.3898012184393,
115.589075202144)) ;
#166060=CARTESIAN_POINT('Ctrl Pts',(-20.0334207640732,-14.3898012199962,
115.564844153851)) ;
#166061=CARTESIAN_POINT('Ctrl Pts',(-20.1072246053238,-14.3898012215531,
115.540613105557)) ;
#166062=CARTESIAN_POINT('Ctrl Pts',(-20.1139659524696,-14.4625579292612,
115.561146161114)) ;
#166063=CARTESIAN_POINT('Ctrl Pts',(-20.1207072996154,-14.5353146369693,
115.581679216671)) ;
#166064=CARTESIAN_POINT('Ctrl Pts',(-20.0469034583648,-14.5353146354125,
115.605910264964)) ;
#166065=CARTESIAN_POINT('Ctrl Pts',(-19.9730996171142,-14.5353146338556,
115.630141313258)) ;
#166066=CARTESIAN_POINT('Ctrl Pts',(-19.9663582699684,-14.4625579261475,
115.609608257701)) ;
#166067=CARTESIAN_POINT('Ctrl Pts',(-19.8873776134028,-14.5058691718866,
115.333726330134)) ;
#166068=CARTESIAN_POINT('Ctrl Pts',(-19.8868719421637,-14.4299792998369,
115.332186137181)) ;
#166069=CARTESIAN_POINT('Ctrl Pts',(-19.960675784752,-14.429979299475,115.307955092962)) ;
#166070=CARTESIAN_POINT('Ctrl Pts',(-20.0344796273404,-14.4299792991131,
115.283724048743)) ;
#166071=CARTESIAN_POINT('Ctrl Pts',(-20.0349852985795,-14.5058691711628,
115.285264241697)) ;
#166072=CARTESIAN_POINT('Ctrl Pts',(-20.0354909698187,-14.5817590432124,
115.28680443465)) ;
#166073=CARTESIAN_POINT('Ctrl Pts',(-19.9616871272303,-14.5817590435743,
115.311035478869)) ;
#166074=CARTESIAN_POINT('Ctrl Pts',(-19.887883284642,-14.5817590439362,
115.335266523088)) ;
#166075=CARTESIAN_POINT('Ctrl Pts',(-19.8873776134028,-14.5058691718866,
115.333726330134)) ;
#166076=CARTESIAN_POINT('Ctrl Pts',(-19.8074081898511,-14.471221053196,
115.054555605598)) ;
#166077=CARTESIAN_POINT('Ctrl Pts',(-19.8132226145073,-14.3976366078093,
115.072265404916)) ;
#166078=CARTESIAN_POINT('Ctrl Pts',(-19.8870264584312,-14.397636607939,
115.048034364765)) ;
#166079=CARTESIAN_POINT('Ctrl Pts',(-19.9608303023551,-14.3976366080687,
115.023803324613)) ;
#166080=CARTESIAN_POINT('Ctrl Pts',(-19.9550158776989,-14.4712210534553,
115.006093525296)) ;
#166081=CARTESIAN_POINT('Ctrl Pts',(-19.9492014530427,-14.5448054988419,
114.988383725979)) ;
#166082=CARTESIAN_POINT('Ctrl Pts',(-19.8753976091188,-14.5448054987123,
115.01261476613)) ;
#166083=CARTESIAN_POINT('Ctrl Pts',(-19.8015937651949,-14.5448054985826,
115.036845806281)) ;
#166084=CARTESIAN_POINT('Ctrl Pts',(-19.8074081898511,-14.471221053196,
115.054555605598)) ;
#166085=CARTESIAN_POINT('Ctrl Pts',(-19.7339488645536,-14.3613267795073,
114.795410318101)) ;
#166086=CARTESIAN_POINT('Ctrl Pts',(-19.7456340819167,-14.2953066789367,
114.831001604723)) ;
#166087=CARTESIAN_POINT('Ctrl Pts',(-19.8194379262271,-14.2953066805575,
114.806770565749)) ;
#166088=CARTESIAN_POINT('Ctrl Pts',(-19.8932417705375,-14.2953066821784,
114.782539526775)) ;
#166089=CARTESIAN_POINT('Ctrl Pts',(-19.8815565531744,-14.361326782749,
114.746948240154)) ;
#166090=CARTESIAN_POINT('Ctrl Pts',(-19.8698713358113,-14.4273468833197,
114.711356953532)) ;
#166091=CARTESIAN_POINT('Ctrl Pts',(-19.7960674915009,-14.4273468816988,
114.735587992506)) ;
#166092=CARTESIAN_POINT('Ctrl Pts',(-19.7222636471905,-14.4273468800779,
114.75981903148)) ;
#166093=CARTESIAN_POINT('Ctrl Pts',(-19.7339488645536,-14.3613267795073,
114.795410318101)) ;
#166094=CARTESIAN_POINT('Ctrl Pts',(-19.6723166521497,-14.1831445066676,
114.572116798133)) ;
#166095=CARTESIAN_POINT('Ctrl Pts',(-19.6890592182227,-14.1294690686809,
114.623111952935)) ;
#166096=CARTESIAN_POINT('Ctrl Pts',(-19.7628630622087,-14.1294690707301,
114.598880912973)) ;
#166097=CARTESIAN_POINT('Ctrl Pts',(-19.8366669061947,-14.1294690727794,
114.574649873011)) ;
#166098=CARTESIAN_POINT('Ctrl Pts',(-19.8199243401217,-14.1831445107661,
114.523654718209)) ;
#166099=CARTESIAN_POINT('Ctrl Pts',(-19.8031817740486,-14.2368199487529,
114.472659563407)) ;
#166100=CARTESIAN_POINT('Ctrl Pts',(-19.7293779300626,-14.2368199467036,
114.496890603369)) ;
#166101=CARTESIAN_POINT('Ctrl Pts',(-19.6555740860767,-14.2368199446543,
114.521121643331)) ;
#166102=CARTESIAN_POINT('Ctrl Pts',(-19.6723166521497,-14.1831445066676,
114.572116798133)) ;
#166103=CARTESIAN_POINT('Ctrl Pts',(-19.6282726005252,-13.9512771233317,
114.40260456507)) ;
#166104=CARTESIAN_POINT('Ctrl Pts',(-19.6488469329677,-13.9137135164908,
114.465270662026)) ;
#166105=CARTESIAN_POINT('Ctrl Pts',(-19.7226507763542,-13.9137135169973,
114.441039620238)) ;
#166106=CARTESIAN_POINT('Ctrl Pts',(-19.7964546197408,-13.9137135175038,
114.41680857845)) ;
#166107=CARTESIAN_POINT('Ctrl Pts',(-19.7758802872982,-13.9512771243447,
114.354142481495)) ;
#166108=CARTESIAN_POINT('Ctrl Pts',(-19.7553059548557,-13.9888407311855,
114.291476384539)) ;
#166109=CARTESIAN_POINT('Ctrl Pts',(-19.6815021114692,-13.988840730679,
114.315707426327)) ;
#166110=CARTESIAN_POINT('Ctrl Pts',(-19.6076982680827,-13.9888407301726,
114.339938468114)) ;
#166111=CARTESIAN_POINT('Ctrl Pts',(-19.6282726005252,-13.9512771233317,
114.40260456507)) ;
#166112=CARTESIAN_POINT('Ctrl Pts',(-19.6052474089062,-13.6804917592119,
114.29698357989)) ;
#166113=CARTESIAN_POINT('Ctrl Pts',(-19.6281940892339,-13.6617810820817,
114.366875465811)) ;
#166114=CARTESIAN_POINT('Ctrl Pts',(-19.7019979322277,-13.6617810784038,
114.342644422827)) ;
#166115=CARTESIAN_POINT('Ctrl Pts',(-19.7758017752214,-13.6617810747259,
114.318413379842)) ;
#166116=CARTESIAN_POINT('Ctrl Pts',(-19.7528550948936,-13.6804917518562,
114.248521493922)) ;
#166117=CARTESIAN_POINT('Ctrl Pts',(-19.7299084145659,-13.6992024289864,
114.178629608001)) ;
#166118=CARTESIAN_POINT('Ctrl Pts',(-19.6561045715721,-13.6992024326643,
114.202860650985)) ;
#166119=CARTESIAN_POINT('Ctrl Pts',(-19.5823007285784,-13.6992024363421,
114.227091693969)) ;
#166120=CARTESIAN_POINT('Ctrl Pts',(-19.6052474089062,-13.6804917592119,
114.29698357989)) ;
#166121=CARTESIAN_POINT('Ctrl Pts',(-19.6057961466648,-13.3916820675785,
114.263270356301)) ;
#166122=CARTESIAN_POINT('Ctrl Pts',(-19.6294701323659,-13.3931100750182,
114.335377497137)) ;
#166123=CARTESIAN_POINT('Ctrl Pts',(-19.7032739756634,-13.3931100660094,
114.311146455077)) ;
#166124=CARTESIAN_POINT('Ctrl Pts',(-19.7770778189608,-13.3931100570005,
114.286915413018)) ;
#166125=CARTESIAN_POINT('Ctrl Pts',(-19.7534038332597,-13.3916820495608,
114.214808272182)) ;
#166126=CARTESIAN_POINT('Ctrl Pts',(-19.7297298475586,-13.390254042121,
114.142701131346)) ;
#166127=CARTESIAN_POINT('Ctrl Pts',(-19.6559260042611,-13.3902540511299,
114.166932173406)) ;
#166128=CARTESIAN_POINT('Ctrl Pts',(-19.5821221609637,-13.3902540601387,
114.191163215465)) ;
#166129=CARTESIAN_POINT('Ctrl Pts',(-19.6057961466648,-13.3916820675785,
114.263270356301)) ;
#166130=CARTESIAN_POINT('Ctrl Pts',(-19.630746144009,-13.10326146677,114.303685809968)) ;
#166131=CARTESIAN_POINT('Ctrl Pts',(-19.6534487804468,-13.1248302660667,
114.372834377822)) ;
#166132=CARTESIAN_POINT('Ctrl Pts',(-19.7272526251537,-13.12483024999,114.348603340056)) ;
#166133=CARTESIAN_POINT('Ctrl Pts',(-19.8010564698606,-13.1248302339134,
114.32437230229)) ;
#166134=CARTESIAN_POINT('Ctrl Pts',(-19.7783538334228,-13.1032614346168,
114.255223734436)) ;
#166135=CARTESIAN_POINT('Ctrl Pts',(-19.755651196985,-13.0816926353201,
114.186075166582)) ;
#166136=CARTESIAN_POINT('Ctrl Pts',(-19.6818473522781,-13.0816926513967,
114.210306204348)) ;
#166137=CARTESIAN_POINT('Ctrl Pts',(-19.6080435075712,-13.0816926674734,
114.234537242114)) ;
#166138=CARTESIAN_POINT('Ctrl Pts',(-19.630746144009,-13.10326146677,114.303685809968)) ;
#166139=CARTESIAN_POINT('Ctrl Pts',(-19.6788883367903,-12.8385043736975,
114.414887005112)) ;
#166140=CARTESIAN_POINT('Ctrl Pts',(-19.6989956623995,-12.8785902983801,
114.476130675077)) ;
#166141=CARTESIAN_POINT('Ctrl Pts',(-19.772799509607,-12.8785902776547,
114.451899644927)) ;
#166142=CARTESIAN_POINT('Ctrl Pts',(-19.8466033568145,-12.8785902569293,
114.427668614778)) ;
#166143=CARTESIAN_POINT('Ctrl Pts',(-19.8264960312054,-12.8385043322466,
114.366424944813)) ;
#166144=CARTESIAN_POINT('Ctrl Pts',(-19.8063887055962,-12.7984184075639,
114.305181274849)) ;
#166145=CARTESIAN_POINT('Ctrl Pts',(-19.7325848583887,-12.7984184282893,
114.329412304998)) ;
#166146=CARTESIAN_POINT('Ctrl Pts',(-19.6587810111812,-12.7984184490148,
114.353643335148)) ;
#166147=CARTESIAN_POINT('Ctrl Pts',(-19.6788883367903,-12.8385043736975,
114.414887005112)) ;
#166148=CARTESIAN_POINT('Ctrl Pts',(-19.7478090515721,-12.6146172171064,
114.589262192695)) ;
#166149=CARTESIAN_POINT('Ctrl Pts',(-19.7638689510113,-12.6703934014124,
114.63817805577)) ;
#166150=CARTESIAN_POINT('Ctrl Pts',(-19.8376728018705,-12.6703933786195,
114.613947036742)) ;
#166151=CARTESIAN_POINT('Ctrl Pts',(-19.9114766527297,-12.6703933558266,
114.589716017715)) ;
#166152=CARTESIAN_POINT('Ctrl Pts',(-19.8954167532905,-12.6146171715207,
114.54080015464)) ;
#166153=CARTESIAN_POINT('Ctrl Pts',(-19.8793568538513,-12.5588409872148,
114.491884291566)) ;
#166154=CARTESIAN_POINT('Ctrl Pts',(-19.8055530029922,-12.5588410100077,
114.516115310593)) ;
#166155=CARTESIAN_POINT('Ctrl Pts',(-19.731749152133,-12.5588410328005,
114.54034632962)) ;
#166156=CARTESIAN_POINT('Ctrl Pts',(-19.7478090515721,-12.6146172171064,
114.589262192695)) ;
#166157=CARTESIAN_POINT('Ctrl Pts',(-19.8327892013851,-12.4490452703409,
114.812711060291)) ;
#166158=CARTESIAN_POINT('Ctrl Pts',(-19.8436711987224,-12.5164621248353,
114.845855869166)) ;
#166159=CARTESIAN_POINT('Ctrl Pts',(-19.9174750533839,-12.5164621055273,
114.82162486172)) ;
#166160=CARTESIAN_POINT('Ctrl Pts',(-19.9912789080454,-12.5164620862193,
114.797393854274)) ;
#166161=CARTESIAN_POINT('Ctrl Pts',(-19.9803969107081,-12.449045231725,
114.764249045399)) ;
#166162=CARTESIAN_POINT('Ctrl Pts',(-19.9695149133709,-12.3816283772306,
114.731104236523)) ;
#166163=CARTESIAN_POINT('Ctrl Pts',(-19.8957110587094,-12.3816283965386,
114.755335243969)) ;
#166164=CARTESIAN_POINT('Ctrl Pts',(-19.8219072040478,-12.3816284158465,
114.779566251415)) ;
#166165=CARTESIAN_POINT('Ctrl Pts',(-19.8327892013851,-12.4490452703409,
114.812711060291)) ;
#166166=CARTESIAN_POINT('Ctrl Pts',(-19.9292782242536,-12.3524023594542,
115.071032776141)) ;
#166167=CARTESIAN_POINT('Ctrl Pts',(-19.9341751641512,-12.4266644816829,
115.085948065929)) ;
#166168=CARTESIAN_POINT('Ctrl Pts',(-20.0079790229734,-12.4266644707959,
115.061717071156)) ;
#166169=CARTESIAN_POINT('Ctrl Pts',(-20.0817828817955,-12.4266644599088,
115.037486076383)) ;
#166170=CARTESIAN_POINT('Ctrl Pts',(-20.0768859418979,-12.3524023376801,
115.022570786595)) ;
#166171=CARTESIAN_POINT('Ctrl Pts',(-20.0719890020003,-12.2781402154514,
115.007655496807)) ;
#166172=CARTESIAN_POINT('Ctrl Pts',(-19.9981851431782,-12.2781402263384,
115.03188649158)) ;
#166173=CARTESIAN_POINT('Ctrl Pts',(-19.924381284356,-12.2781402372254,
115.056117486353)) ;
#166174=CARTESIAN_POINT('Ctrl Pts',(-19.9292782242536,-12.3524023594542,
115.071032776141)) ;
#166175=CARTESIAN_POINT('Ctrl Pts',(-20.02989329958,-12.3322917866331,115.342208218691)) ;
#166176=CARTESIAN_POINT('Ctrl Pts',(-20.0285025426279,-12.4080647606153,
115.337972198524)) ;
#166177=CARTESIAN_POINT('Ctrl Pts',(-20.1023064039529,-12.4080647636104,
115.313741211374)) ;
#166178=CARTESIAN_POINT('Ctrl Pts',(-20.1761102652779,-12.4080647666054,
115.289510224224)) ;
#166179=CARTESIAN_POINT('Ctrl Pts',(-20.17750102223,-12.3322917926232,115.293746244391)) ;
#166180=CARTESIAN_POINT('Ctrl Pts',(-20.1788917791821,-12.256518818641,
115.297982264558)) ;
#166181=CARTESIAN_POINT('Ctrl Pts',(-20.1050879178571,-12.256518815646,
115.322213251708)) ;
#166182=CARTESIAN_POINT('Ctrl Pts',(-20.0312840565321,-12.2565188126509,
115.346444238858)) ;
#166183=CARTESIAN_POINT('Ctrl Pts',(-20.02989329958,-12.3322917866331,115.342208218691)) ;
#166184=CARTESIAN_POINT('Ctrl Pts',(-20.1297073657354,-12.3899082998251,
115.610661574223)) ;
#166185=CARTESIAN_POINT('Ctrl Pts',(-20.1220816634719,-12.4617684939858,
115.587434916822)) ;
#166186=CARTESIAN_POINT('Ctrl Pts',(-20.1958855266358,-12.4617685151837,
115.563203935273)) ;
#166187=CARTESIAN_POINT('Ctrl Pts',(-20.2696893897997,-12.4617685363815,
115.538972953724)) ;
#166188=CARTESIAN_POINT('Ctrl Pts',(-20.2773150920632,-12.3899083422208,
115.562199611125)) ;
#166189=CARTESIAN_POINT('Ctrl Pts',(-20.2849407943267,-12.3180481480601,
115.585426268526)) ;
#166190=CARTESIAN_POINT('Ctrl Pts',(-20.2111369311628,-12.3180481268623,
115.609657250075)) ;
#166191=CARTESIAN_POINT('Ctrl Pts',(-20.1373330679989,-12.3180481056645,
115.633888231624)) ;
#166192=CARTESIAN_POINT('Ctrl Pts',(-20.1297073657354,-12.3899082998251,
115.610661574223)) ;
#166193=CARTESIAN_POINT('Ctrl Pts',(-20.2210035911202,-12.5204817202917,
115.853404760459)) ;
#166194=CARTESIAN_POINT('Ctrl Pts',(-20.2077238649911,-12.5833292491025,
115.812956858768)) ;
#166195=CARTESIAN_POINT('Ctrl Pts',(-20.2815277274735,-12.5833292901703,
115.788725875143)) ;
#166196=CARTESIAN_POINT('Ctrl Pts',(-20.3553315899559,-12.5833293312382,
115.764494891519)) ;
#166197=CARTESIAN_POINT('Ctrl Pts',(-20.3686113160851,-12.5204818024274,
115.804942793209)) ;
#166198=CARTESIAN_POINT('Ctrl Pts',(-20.3818910422142,-12.4576342736166,
115.8453906949)) ;
#166199=CARTESIAN_POINT('Ctrl Pts',(-20.3080871797318,-12.4576342325488,
115.869621678525)) ;
#166200=CARTESIAN_POINT('Ctrl Pts',(-20.2342833172493,-12.457634191481,
115.893852662149)) ;
#166201=CARTESIAN_POINT('Ctrl Pts',(-20.2210035911202,-12.5204817202917,
115.853404760459)) ;
#166202=CARTESIAN_POINT('Ctrl Pts',(-20.2992739009599,-12.7170079033734,
116.056135467332)) ;
#166203=CARTESIAN_POINT('Ctrl Pts',(-20.2812482485149,-12.7662262828423,
116.00123224001)) ;
#166204=CARTESIAN_POINT('Ctrl Pts',(-20.3550521086811,-12.7662263456653,
115.977001249331)) ;
#166205=CARTESIAN_POINT('Ctrl Pts',(-20.4288559688472,-12.7662264084883,
115.952770258651)) ;
#166206=CARTESIAN_POINT('Ctrl Pts',(-20.4468816212922,-12.7170080290195,
116.007673485972)) ;
#166207=CARTESIAN_POINT('Ctrl Pts',(-20.4649072737372,-12.6677896495507,
116.062576713293)) ;
#166208=CARTESIAN_POINT('Ctrl Pts',(-20.391103413571,-12.6677895867277,
116.086807703973)) ;
#166209=CARTESIAN_POINT('Ctrl Pts',(-20.3172995534049,-12.6677895239046,
116.111038694653)) ;
#166210=CARTESIAN_POINT('Ctrl Pts',(-20.2992739009599,-12.7170079033734,
116.056135467332)) ;
#166211=CARTESIAN_POINT('Ctrl Pts',(-20.3582578994183,-12.9615280720901,
116.200502710749)) ;
#166212=CARTESIAN_POINT('Ctrl Pts',(-20.3368182747409,-12.9937459693296,
116.135201074954)) ;
#166213=CARTESIAN_POINT('Ctrl Pts',(-20.410622129823,-12.9937460490588,
116.110970068789)) ;
#166214=CARTESIAN_POINT('Ctrl Pts',(-20.484425984905,-12.9937461287879,
116.086739062624)) ;
#166215=CARTESIAN_POINT('Ctrl Pts',(-20.5058656095824,-12.9615282315483,
116.152040698419)) ;
#166216=CARTESIAN_POINT('Ctrl Pts',(-20.5273052342599,-12.9293103343088,
116.217342334215)) ;
#166217=CARTESIAN_POINT('Ctrl Pts',(-20.4535013791778,-12.9293102545796,
116.241573340379)) ;
#166218=CARTESIAN_POINT('Ctrl Pts',(-20.3796975240957,-12.9293101748505,
116.265804346544)) ;
#166219=CARTESIAN_POINT('Ctrl Pts',(-20.3582578994183,-12.9615280720901,
116.200502710749)) ;
#166220=CARTESIAN_POINT('Ctrl Pts',(-20.3956758286965,-13.241668548695,
116.278772178116)) ;
#166221=CARTESIAN_POINT('Ctrl Pts',(-20.3723310699443,-13.2543754677215,
116.207667811464)) ;
#166222=CARTESIAN_POINT('Ctrl Pts',(-20.4461349183247,-13.2543755617733,
116.183436784887)) ;
#166223=CARTESIAN_POINT('Ctrl Pts',(-20.5199387667051,-13.2543756558251,
116.15920575831)) ;
#166224=CARTESIAN_POINT('Ctrl Pts',(-20.5432835254574,-13.2416687367986,
116.230310124962)) ;
#166225=CARTESIAN_POINT('Ctrl Pts',(-20.5666282842096,-13.228961817772,
116.301414491615)) ;
#166226=CARTESIAN_POINT('Ctrl Pts',(-20.4928244358292,-13.2289617237202,
116.325645518192)) ;
#166227=CARTESIAN_POINT('Ctrl Pts',(-20.4190205874488,-13.2289616296684,
116.349876544769)) ;
#166228=CARTESIAN_POINT('Ctrl Pts',(-20.3956758286965,-13.241668548695,
116.278772178116)) ;
#166229=CARTESIAN_POINT('Ctrl Pts',(-20.4087241002425,-13.5312927388049,
116.283231684985)) ;
#166230=CARTESIAN_POINT('Ctrl Pts',(-20.3851644865814,-13.5237974675911,
116.21147290502)) ;
#166231=CARTESIAN_POINT('Ctrl Pts',(-20.4589683268494,-13.5237975662632,
116.187241853734)) ;
#166232=CARTESIAN_POINT('Ctrl Pts',(-20.5327721671173,-13.5237976649353,
116.163010802447)) ;
#166233=CARTESIAN_POINT('Ctrl Pts',(-20.5563317807784,-13.5312929361492,
116.234769582413)) ;
#166234=CARTESIAN_POINT('Ctrl Pts',(-20.5798913944395,-13.538788207363,
116.306528362378)) ;
#166235=CARTESIAN_POINT('Ctrl Pts',(-20.5060875541715,-13.5387881086909,
116.330759413664)) ;
#166236=CARTESIAN_POINT('Ctrl Pts',(-20.4322837139035,-13.5387880100187,
116.35499046495)) ;
#166237=CARTESIAN_POINT('Ctrl Pts',(-20.4087241002425,-13.5312927388049,
116.283231684985)) ;
#166238=CARTESIAN_POINT('Ctrl Pts',(-20.397812395172,-13.8141856043051,
116.214533598902)) ;
#166239=CARTESIAN_POINT('Ctrl Pts',(-20.375713872965,-13.7869289146623,
116.147225067836)) ;
#166240=CARTESIAN_POINT('Ctrl Pts',(-20.4495177047382,-13.7869290108332,
116.122993990676)) ;
#166241=CARTESIAN_POINT('Ctrl Pts',(-20.5233215365114,-13.7869291070041,
116.098762913516)) ;
#166242=CARTESIAN_POINT('Ctrl Pts',(-20.5454200587184,-13.8141857966469,
116.166071444582)) ;
#166243=CARTESIAN_POINT('Ctrl Pts',(-20.5675185809255,-13.8414424862897,
116.233379975647)) ;
#166244=CARTESIAN_POINT('Ctrl Pts',(-20.4937147491523,-13.8414423901188,
116.257611052807)) ;
#166245=CARTESIAN_POINT('Ctrl Pts',(-20.4199109173791,-13.8414422939479,
116.281842129967)) ;
#166246=CARTESIAN_POINT('Ctrl Pts',(-20.397812395172,-13.8141856043051,
116.214533598902)) ;
#166247=CARTESIAN_POINT('Ctrl Pts',(-20.3642659620429,-14.0686273114668,
116.076918892834)) ;
#166248=CARTESIAN_POINT('Ctrl Pts',(-20.3452103378789,-14.0235664995227,
116.018878538292)) ;
#166249=CARTESIAN_POINT('Ctrl Pts',(-20.4190141615538,-14.0235665846011,
115.994647436466)) ;
#166250=CARTESIAN_POINT('Ctrl Pts',(-20.4928179852287,-14.0235666696795,
115.97041633464)) ;
#166251=CARTESIAN_POINT('Ctrl Pts',(-20.5118736093927,-14.0686274816236,
116.028456689182)) ;
#166252=CARTESIAN_POINT('Ctrl Pts',(-20.5309292335566,-14.1136882935678,
116.086497043723)) ;
#166253=CARTESIAN_POINT('Ctrl Pts',(-20.4571254098818,-14.1136882084894,
116.110728145549)) ;
#166254=CARTESIAN_POINT('Ctrl Pts',(-20.3833215862069,-14.113688123411,
116.134959247375)) ;
#166255=CARTESIAN_POINT('Ctrl Pts',(-20.3642659620429,-14.0686273114668,
116.076918892834)) ;
#166256=CARTESIAN_POINT('Ctrl Pts',(-20.3109843484247,-14.2772225776637,
115.879041201496)) ;
#166257=CARTESIAN_POINT('Ctrl Pts',(-20.2963568431874,-14.2175318931739,
115.834488182769)) ;
#166258=CARTESIAN_POINT('Ctrl Pts',(-20.3701606600124,-14.2175319594466,
115.81025706008)) ;
#166259=CARTESIAN_POINT('Ctrl Pts',(-20.4439644768373,-14.2175320257193,
115.78602593739)) ;
#166260=CARTESIAN_POINT('Ctrl Pts',(-20.4585919820747,-14.2772227102091,
115.830578956117)) ;
#166261=CARTESIAN_POINT('Ctrl Pts',(-20.473219487312,-14.3369133946989,
115.875131974844)) ;
#166262=CARTESIAN_POINT('Ctrl Pts',(-20.399415670487,-14.3369133284262,
115.899363097534)) ;
#166263=CARTESIAN_POINT('Ctrl Pts',(-20.325611853662,-14.3369132621536,
115.923594220223)) ;
#166264=CARTESIAN_POINT('Ctrl Pts',(-20.3109843484247,-14.2772225776637,
115.879041201496)) ;
#166265=CARTESIAN_POINT('Ctrl Pts',(-20.2431888087384,-14.4229662306659,
115.637203831171)) ;
#166266=CARTESIAN_POINT('Ctrl Pts',(-20.234004322962,-14.3530122150386,
115.609229371502)) ;
#166267=CARTESIAN_POINT('Ctrl Pts',(-20.3078081351379,-14.3530122565041,
115.584998234652)) ;
#166268=CARTESIAN_POINT('Ctrl Pts',(-20.3816119473137,-14.3530122979697,
115.560767097802)) ;
#166269=CARTESIAN_POINT('Ctrl Pts',(-20.3907964330902,-14.4229663135971,
115.588741557471)) ;
#166270=CARTESIAN_POINT('Ctrl Pts',(-20.3999809188666,-14.4929203292244,
115.61671601714)) ;
#166271=CARTESIAN_POINT('Ctrl Pts',(-20.3261771066907,-14.4929202877588,
115.640947153991)) ;
#166272=CARTESIAN_POINT('Ctrl Pts',(-20.2523732945149,-14.4929202462933,
115.665178290841)) ;
#166273=CARTESIAN_POINT('Ctrl Pts',(-20.2431888087384,-14.4229662306659,
115.637203831171)) ;
#166274=CARTESIAN_POINT('Ctrl Pts',(-20.165967360864,-14.4976749709137,
115.366562084077)) ;
#166275=CARTESIAN_POINT('Ctrl Pts',(-20.162893823781,-14.4224014624097,
115.357200588124)) ;
#166276=CARTESIAN_POINT('Ctrl Pts',(-20.2366976337292,-14.4224014756821,
115.332969444489)) ;
#166277=CARTESIAN_POINT('Ctrl Pts',(-20.3105014436775,-14.4224014889544,
115.308738300854)) ;
#166278=CARTESIAN_POINT('Ctrl Pts',(-20.3135749807605,-14.4976749974584,
115.318099796806)) ;
#166279=CARTESIAN_POINT('Ctrl Pts',(-20.3166485178435,-14.5729485059623,
115.327461292759)) ;
#166280=CARTESIAN_POINT('Ctrl Pts',(-20.2428447078953,-14.57294849269,115.351692436394)) ;
#166281=CARTESIAN_POINT('Ctrl Pts',(-20.169040897947,-14.5729484794176,
115.375923580029)) ;
#166282=CARTESIAN_POINT('Ctrl Pts',(-20.165967360864,-14.4976749709137,
115.366562084077)) ;
#166283=CARTESIAN_POINT('Ctrl Pts',(-20.0851494998397,-14.4944851703305,
115.084714178899)) ;
#166284=CARTESIAN_POINT('Ctrl Pts',(-20.0884522101337,-14.4193216059584,
115.094773703609)) ;
#166285=CARTESIAN_POINT('Ctrl Pts',(-20.1622560208923,-14.4193215903829,
115.070542562443)) ;
#166286=CARTESIAN_POINT('Ctrl Pts',(-20.2360598316509,-14.4193215748074,
115.046311421276)) ;
#166287=CARTESIAN_POINT('Ctrl Pts',(-20.232757121357,-14.4944851391795,
115.036251896566)) ;
#166288=CARTESIAN_POINT('Ctrl Pts',(-20.229454411063,-14.5696487035515,
115.026192371856)) ;
#166289=CARTESIAN_POINT('Ctrl Pts',(-20.1556506003044,-14.5696487191271,
115.050423513022)) ;
#166290=CARTESIAN_POINT('Ctrl Pts',(-20.0818467895458,-14.5696487347026,
115.074654654189)) ;
#166291=CARTESIAN_POINT('Ctrl Pts',(-20.0851494998397,-14.4944851703305,
115.084714178899)) ;
#166292=CARTESIAN_POINT('Ctrl Pts',(-20.0087955569206,-14.4147277655596,
114.816900333307)) ;
#166293=CARTESIAN_POINT('Ctrl Pts',(-20.0181634621253,-14.3450211180556,
114.845433463057)) ;
#166294=CARTESIAN_POINT('Ctrl Pts',(-20.091967275971,-14.3450210762549,
114.821202331292)) ;
#166295=CARTESIAN_POINT('Ctrl Pts',(-20.1657710898167,-14.3450210344541,
114.796971199528)) ;
#166296=CARTESIAN_POINT('Ctrl Pts',(-20.156403184612,-14.4147276819581,
114.768438069778)) ;
#166297=CARTESIAN_POINT('Ctrl Pts',(-20.1470352794072,-14.4844343294621,
114.739904940028)) ;
#166298=CARTESIAN_POINT('Ctrl Pts',(-20.0732314655615,-14.4844343712628,
114.764136071792)) ;
#166299=CARTESIAN_POINT('Ctrl Pts',(-19.9994276517158,-14.4844344130636,
114.788367203557)) ;
#166300=CARTESIAN_POINT('Ctrl Pts',(-20.0087955569206,-14.4147277655596,
114.816900333307)) ;
#166301=CARTESIAN_POINT('Ctrl Pts',(-19.9415785213677,-14.2631098096402,
114.576628280773)) ;
#166302=CARTESIAN_POINT('Ctrl Pts',(-19.9563887371762,-14.2038841179929,
114.621737810429)) ;
#166303=CARTESIAN_POINT('Ctrl Pts',(-20.0301925565596,-14.2038840550099,
114.597506695531)) ;
#166304=CARTESIAN_POINT('Ctrl Pts',(-20.103996375943,-14.203883992027,114.573275580634)) ;
#166305=CARTESIAN_POINT('Ctrl Pts',(-20.0891861601345,-14.2631096836743,
114.528166050978)) ;
#166306=CARTESIAN_POINT('Ctrl Pts',(-20.0743759443261,-14.3223353753216,
114.483056521323)) ;
#166307=CARTESIAN_POINT('Ctrl Pts',(-20.0005721249426,-14.3223354383045,
114.50728763622)) ;
#166308=CARTESIAN_POINT('Ctrl Pts',(-19.9267683055592,-14.3223355012875,
114.531518751117)) ;
#166309=CARTESIAN_POINT('Ctrl Pts',(-19.9415785213677,-14.2631098096402,
114.576628280773)) ;
#166310=CARTESIAN_POINT('Ctrl Pts',(-19.889902590895,-14.0515534840703,
114.38383900095)) ;
#166311=CARTESIAN_POINT('Ctrl Pts',(-19.9090752445563,-14.0070094522688,
114.442235812343)) ;
#166312=CARTESIAN_POINT('Ctrl Pts',(-19.9828790708446,-14.0070093747174,
114.418004718477)) ;
#166313=CARTESIAN_POINT('Ctrl Pts',(-20.056682897133,-14.007009297166,114.393773624611)) ;
#166314=CARTESIAN_POINT('Ctrl Pts',(-20.0375102434718,-14.0515533289676,
114.335376813219)) ;
#166315=CARTESIAN_POINT('Ctrl Pts',(-20.0183375898106,-14.0960973607691,
114.276980001827)) ;
#166316=CARTESIAN_POINT('Ctrl Pts',(-19.9445337635222,-14.0960974383204,
114.301211095692)) ;
#166317=CARTESIAN_POINT('Ctrl Pts',(-19.8707299372338,-14.0960975158718,
114.325442189558)) ;
#166318=CARTESIAN_POINT('Ctrl Pts',(-19.889902590895,-14.0515534840703,
114.38383900095)) ;
#166319=CARTESIAN_POINT('Ctrl Pts',(-19.8577995917922,-13.793288943793,
114.250462777897)) ;
#166320=CARTESIAN_POINT('Ctrl Pts',(-19.8799791098395,-13.7667090894671,
114.318018012925)) ;
#166321=CARTESIAN_POINT('Ctrl Pts',(-19.9537829439215,-13.7667090063188,
114.293786942797)) ;
#166322=CARTESIAN_POINT('Ctrl Pts',(-20.0275867780035,-13.7667089231704,
114.269555872669)) ;
#166323=CARTESIAN_POINT('Ctrl Pts',(-20.0054072599561,-13.7932887774963,
114.202000637641)) ;
#166324=CARTESIAN_POINT('Ctrl Pts',(-19.9832277419088,-13.8198686318222,
114.134445402614)) ;
#166325=CARTESIAN_POINT('Ctrl Pts',(-19.9094239078268,-13.8198687149705,
114.158676472742)) ;
#166326=CARTESIAN_POINT('Ctrl Pts',(-19.8356200737448,-13.8198687981189,
114.182907542869)) ;
#166327=CARTESIAN_POINT('Ctrl Pts',(-19.8577995917922,-13.793288943793,
114.250462777897)) ;
#166328=CARTESIAN_POINT('Ctrl Pts',(-19.8486859511613,-13.5095097704303,
114.187308101933)) ;
#166329=CARTESIAN_POINT('Ctrl Pts',(-19.8722676042901,-13.5027030390007,
114.259134014066)) ;
#166330=CARTESIAN_POINT('Ctrl Pts',(-19.946071445741,-13.5027029571053,
114.234902966383)) ;
#166331=CARTESIAN_POINT('Ctrl Pts',(-20.0198752871918,-13.50270287521,114.210671918699)) ;
#166332=CARTESIAN_POINT('Ctrl Pts',(-19.996293634063,-13.5095096066396,
114.138846006567)) ;
#166333=CARTESIAN_POINT('Ctrl Pts',(-19.9727119809342,-13.5163163380692,
114.067020094434)) ;
#166334=CARTESIAN_POINT('Ctrl Pts',(-19.8989081394833,-13.5163164199646,
114.091251142118)) ;
#166335=CARTESIAN_POINT('Ctrl Pts',(-19.8251042980325,-13.5163165018599,
114.115482189801)) ;
#166336=CARTESIAN_POINT('Ctrl Pts',(-19.8486859511613,-13.5095097704303,
114.187308101933)) ;
#166337=CARTESIAN_POINT('Ctrl Pts',(-19.8637427605227,-13.218674427129,
114.197696524742)) ;
#166338=CARTESIAN_POINT('Ctrl Pts',(-19.8870428101562,-13.2321633115492,
114.268664717921)) ;
#166339=CARTESIAN_POINT('Ctrl Pts',(-19.9608466580392,-13.2321632381837,
114.244433689829)) ;
#166340=CARTESIAN_POINT('Ctrl Pts',(-20.0346505059221,-13.2321631648182,
114.220202661737)) ;
#166341=CARTESIAN_POINT('Ctrl Pts',(-20.0113504562886,-13.2186742803981,
114.149234468558)) ;
#166342=CARTESIAN_POINT('Ctrl Pts',(-19.9880504066551,-13.2051853959779,
114.078266275379)) ;
#166343=CARTESIAN_POINT('Ctrl Pts',(-19.9142465587722,-13.2051854693434,
114.102497303471)) ;
#166344=CARTESIAN_POINT('Ctrl Pts',(-19.8404427108892,-13.2051855427089,
114.126728331563)) ;
#166345=CARTESIAN_POINT('Ctrl Pts',(-19.8637427605227,-13.218674427129,
114.197696524742)) ;
#166346=CARTESIAN_POINT('Ctrl Pts',(-19.9025785975589,-12.9425272619773,
114.280582549871)) ;
#166347=CARTESIAN_POINT('Ctrl Pts',(-19.9239349080404,-12.9753170489684,
114.345630427072)) ;
#166348=CARTESIAN_POINT('Ctrl Pts',(-19.9977387608683,-12.9753169887403,
114.321399414041)) ;
#166349=CARTESIAN_POINT('Ctrl Pts',(-20.0715426136962,-12.9753169285121,
114.297168401011)) ;
#166350=CARTESIAN_POINT('Ctrl Pts',(-20.0501863032146,-12.942527141521,
114.232120523809)) ;
#166351=CARTESIAN_POINT('Ctrl Pts',(-20.0288299927331,-12.9097373545299,
114.167072646608)) ;
#166352=CARTESIAN_POINT('Ctrl Pts',(-19.9550261399052,-12.9097374147581,
114.191303659639)) ;
#166353=CARTESIAN_POINT('Ctrl Pts',(-19.8812222870773,-12.9097374749862,
114.21553467267)) ;
#166354=CARTESIAN_POINT('Ctrl Pts',(-19.9025785975589,-12.9425272619773,
114.280582549871)) ;
#166355=CARTESIAN_POINT('Ctrl Pts',(-19.9637005352673,-12.6990701230285,
114.431122563372)) ;
#166356=CARTESIAN_POINT('Ctrl Pts',(-19.9815590200875,-12.7489081846955,
114.485516627788)) ;
#166357=CARTESIAN_POINT('Ctrl Pts',(-20.0553628755155,-12.748908142065,
114.461285622677)) ;
#166358=CARTESIAN_POINT('Ctrl Pts',(-20.1291667309434,-12.7489080994345,
114.437054617565)) ;
#166359=CARTESIAN_POINT('Ctrl Pts',(-20.1113082461232,-12.6990700377675,
114.382660553149)) ;
#166360=CARTESIAN_POINT('Ctrl Pts',(-20.0934497613029,-12.6492319761005,
114.328266488732)) ;
#166361=CARTESIAN_POINT('Ctrl Pts',(-20.019645905875,-12.649232018731,114.352497493844)) ;
#166362=CARTESIAN_POINT('Ctrl Pts',(-19.945842050447,-12.6492320613615,
114.376728498955)) ;
#166363=CARTESIAN_POINT('Ctrl Pts',(-19.9637005352673,-12.6990701230285,
114.431122563372)) ;
#166364=CARTESIAN_POINT('Ctrl Pts',(-20.0423283064488,-12.5091750901202,
114.635350522219)) ;
#166365=CARTESIAN_POINT('Ctrl Pts',(-20.0554534729284,-12.5723470280859,
114.675327662559)) ;
#166366=CARTESIAN_POINT('Ctrl Pts',(-20.1292573296924,-12.5723470007831,
114.651096661517)) ;
#166367=CARTESIAN_POINT('Ctrl Pts',(-20.2030611864563,-12.5723469734802,
114.626865660475)) ;
#166368=CARTESIAN_POINT('Ctrl Pts',(-20.1899360199767,-12.5091750355146,
114.586888520134)) ;
#166369=CARTESIAN_POINT('Ctrl Pts',(-20.1768108534972,-12.4460030975489,
114.546911379793)) ;
#166370=CARTESIAN_POINT('Ctrl Pts',(-20.1030069967332,-12.4460031248517,
114.571142380836)) ;
#166371=CARTESIAN_POINT('Ctrl Pts',(-20.0292031399693,-12.4460031521546,
114.595373381878)) ;
#166372=CARTESIAN_POINT('Ctrl Pts',(-20.0423283064488,-12.5091750901202,
114.635350522219)) ;
#166373=CARTESIAN_POINT('Ctrl Pts',(-20.1350384738347,-12.3826566850404,
114.882137699314)) ;
#166374=CARTESIAN_POINT('Ctrl Pts',(-20.1424469548967,-12.4547585599534,
114.904702738063)) ;
#166375=CARTESIAN_POINT('Ctrl Pts',(-20.2162508105127,-12.4547585482587,
114.880471733524)) ;
#166376=CARTESIAN_POINT('Ctrl Pts',(-20.2900546661287,-12.4547585365639,
114.856240728986)) ;
#166377=CARTESIAN_POINT('Ctrl Pts',(-20.2826461850667,-12.3826566616509,
114.833675690236)) ;
#166378=CARTESIAN_POINT('Ctrl Pts',(-20.2752377040047,-12.3105547867379,
114.811110651486)) ;
#166379=CARTESIAN_POINT('Ctrl Pts',(-20.2014338483887,-12.3105547984326,
114.835341656025)) ;
#166380=CARTESIAN_POINT('Ctrl Pts',(-20.1276299927727,-12.3105548101274,
114.859572660564)) ;
#166381=CARTESIAN_POINT('Ctrl Pts',(-20.1350384738347,-12.3826566850404,
114.882137699314)) ;
#166382=CARTESIAN_POINT('Ctrl Pts',(-20.2350090319357,-12.3310754563828,
115.151149980426)) ;
#166383=CARTESIAN_POINT('Ctrl Pts',(-20.2361827516347,-12.4068883304643,
115.154724941869)) ;
#166384=CARTESIAN_POINT('Ctrl Pts',(-20.309986605033,-12.406888329813,115.130493930576)) ;
#166385=CARTESIAN_POINT('Ctrl Pts',(-20.3837904584313,-12.4068883291616,
115.106262919282)) ;
#166386=CARTESIAN_POINT('Ctrl Pts',(-20.3826167387323,-12.3310754550801,
115.102687957839)) ;
#166387=CARTESIAN_POINT('Ctrl Pts',(-20.3814430190333,-12.2552625809986,
115.099112996395)) ;
#166388=CARTESIAN_POINT('Ctrl Pts',(-20.307639165635,-12.25526258165,115.123344007689)) ;
#166389=CARTESIAN_POINT('Ctrl Pts',(-20.2338353122368,-12.2552625823013,
115.147575018982)) ;
#166390=CARTESIAN_POINT('Ctrl Pts',(-20.2350090319357,-12.3310754563828,
115.151149980426)) ;
#166391=CARTESIAN_POINT('Ctrl Pts',(-20.3359195607843,-12.357364074466,
115.42305855361)) ;
#166392=CARTESIAN_POINT('Ctrl Pts',(-20.3307826681784,-12.4314561765023,
115.40741240803)) ;
#166393=CARTESIAN_POINT('Ctrl Pts',(-20.4045865188482,-12.4314561824614,
115.383181388426)) ;
#166394=CARTESIAN_POINT('Ctrl Pts',(-20.4783903695179,-12.4314561884204,
115.358950368822)) ;
#166395=CARTESIAN_POINT('Ctrl Pts',(-20.4835272621239,-12.3573640863842,
115.374596514401)) ;
#166396=CARTESIAN_POINT('Ctrl Pts',(-20.4886641547298,-12.2832719843479,
115.39024265998)) ;
#166397=CARTESIAN_POINT('Ctrl Pts',(-20.4148603040601,-12.2832719783889,
115.414473679585)) ;
#166398=CARTESIAN_POINT('Ctrl Pts',(-20.3410564533903,-12.2832719724298,
115.438704699189)) ;
#166399=CARTESIAN_POINT('Ctrl Pts',(-20.3359195607843,-12.357364074466,
115.42305855361)) ;
#166400=CARTESIAN_POINT('Ctrl Pts',(-20.4312001328524,-12.4589530543375,
115.677923655332)) ;
#166401=CARTESIAN_POINT('Ctrl Pts',(-20.4201340505478,-12.5260636075349,
115.644218154473)) ;
#166402=CARTESIAN_POINT('Ctrl Pts',(-20.4939378986042,-12.5260636163209,
115.619987126908)) ;
#166403=CARTESIAN_POINT('Ctrl Pts',(-20.5677417466605,-12.5260636251069,
115.595756099344)) ;
#166404=CARTESIAN_POINT('Ctrl Pts',(-20.5788078289651,-12.4589530719095,
115.629461600204)) ;
#166405=CARTESIAN_POINT('Ctrl Pts',(-20.5898739112697,-12.3918425187121,
115.663167101063)) ;
#166406=CARTESIAN_POINT('Ctrl Pts',(-20.5160700632133,-12.3918425099261,
115.687398128628)) ;
#166407=CARTESIAN_POINT('Ctrl Pts',(-20.442266215157,-12.3918425011401,
115.711629156192)) ;
#166408=CARTESIAN_POINT('Ctrl Pts',(-20.4312001328524,-12.4589530543375,
115.677923655332)) ;
#166409=CARTESIAN_POINT('Ctrl Pts',(-20.5157214281701,-12.6306888766498,
115.89970465667)) ;
#166410=CARTESIAN_POINT('Ctrl Pts',(-20.4994746267274,-12.6859095379068,
115.850219521061)) ;
#166411=CARTESIAN_POINT('Ctrl Pts',(-20.5732784720464,-12.6859095445597,
115.82598848516)) ;
#166412=CARTESIAN_POINT('Ctrl Pts',(-20.6470823173654,-12.6859095512127,
115.801757449258)) ;
#166413=CARTESIAN_POINT('Ctrl Pts',(-20.6633291188081,-12.6306888899557,
115.851242584866)) ;
#166414=CARTESIAN_POINT('Ctrl Pts',(-20.6795759202508,-12.5754682286988,
115.900727720475)) ;
#166415=CARTESIAN_POINT('Ctrl Pts',(-20.6057720749318,-12.5754682220458,
115.924958756377)) ;
#166416=CARTESIAN_POINT('Ctrl Pts',(-20.5319682296128,-12.5754682153929,
115.949189792279)) ;
#166417=CARTESIAN_POINT('Ctrl Pts',(-20.5157214281701,-12.6306888766498,
115.89970465667)) ;
#166418=CARTESIAN_POINT('Ctrl Pts',(-20.5826648508089,-12.8569331102211,
116.068310974654)) ;
#166419=CARTESIAN_POINT('Ctrl Pts',(-20.5624497196126,-12.8964388496988,
116.006738946817)) ;
#166420=CARTESIAN_POINT('Ctrl Pts',(-20.6362535636491,-12.8964388537721,
115.982507907009)) ;
#166421=CARTESIAN_POINT('Ctrl Pts',(-20.7100574076856,-12.8964388578454,
115.958276867201)) ;
#166422=CARTESIAN_POINT('Ctrl Pts',(-20.7302725388819,-12.8569331183677,
116.019848895037)) ;
#166423=CARTESIAN_POINT('Ctrl Pts',(-20.7504876700782,-12.81742737889,116.081420922874)) ;
#166424=CARTESIAN_POINT('Ctrl Pts',(-20.6766838260417,-12.8174273748167,
116.105651962682)) ;
#166425=CARTESIAN_POINT('Ctrl Pts',(-20.6028799820052,-12.8174273707434,
116.12988300249)) ;
#166426=CARTESIAN_POINT('Ctrl Pts',(-20.5826648508089,-12.8569331102211,
116.068310974654)) ;
#166427=CARTESIAN_POINT('Ctrl Pts',(-20.629281615088,-13.124308622433,116.174814524661)) ;
#166428=CARTESIAN_POINT('Ctrl Pts',(-20.6065153457123,-13.1452036324507,
116.105472141463)) ;
#166429=CARTESIAN_POINT('Ctrl Pts',(-20.6803191889954,-13.1452036323883,
116.08124109936)) ;
#166430=CARTESIAN_POINT('Ctrl Pts',(-20.7541230322785,-13.1452036323259,
116.057010057257)) ;
#166431=CARTESIAN_POINT('Ctrl Pts',(-20.7768893016542,-13.1243086223082,
116.126352440455)) ;
#166432=CARTESIAN_POINT('Ctrl Pts',(-20.7996555710298,-13.1034136122904,
116.195694823653)) ;
#166433=CARTESIAN_POINT('Ctrl Pts',(-20.7258517277467,-13.1034136123528,
116.219925865756)) ;
#166434=CARTESIAN_POINT('Ctrl Pts',(-20.6520478844636,-13.1034136124152,
116.244156907858)) ;
#166435=CARTESIAN_POINT('Ctrl Pts',(-20.629281615088,-13.124308622433,116.174814524661)) ;
#166436=CARTESIAN_POINT('Ctrl Pts',(-20.6523720977963,-13.4140118065031,
116.209521407609)) ;
#166437=CARTESIAN_POINT('Ctrl Pts',(-20.6286965490956,-13.4147080729357,
116.137409506245)) ;
#166438=CARTESIAN_POINT('Ctrl Pts',(-20.7025003924587,-13.414708069978,
116.113178464386)) ;
#166439=CARTESIAN_POINT('Ctrl Pts',(-20.7763042358217,-13.4147080670203,
116.088947422527)) ;
#166440=CARTESIAN_POINT('Ctrl Pts',(-20.7999797845225,-13.4140118005876,
116.16105932389)) ;
#166441=CARTESIAN_POINT('Ctrl Pts',(-20.8236553332232,-13.413315534155,
116.233171225254)) ;
#166442=CARTESIAN_POINT('Ctrl Pts',(-20.7498514898601,-13.4133155371127,
116.257402267113)) ;
#166443=CARTESIAN_POINT('Ctrl Pts',(-20.676047646497,-13.4133155400704,
116.281633308972)) ;
#166444=CARTESIAN_POINT('Ctrl Pts',(-20.6523720977963,-13.4140118065031,
116.209521407609)) ;
#166445=CARTESIAN_POINT('Ctrl Pts',(-20.6511480384506,-13.700942777731,
116.170554445295)) ;
#166446=CARTESIAN_POINT('Ctrl Pts',(-20.6282523177272,-13.6816044417709,
116.100817774118)) ;
#166447=CARTESIAN_POINT('Ctrl Pts',(-20.7020561614304,-13.6816044385339,
116.076586733294)) ;
#166448=CARTESIAN_POINT('Ctrl Pts',(-20.7758600051336,-13.6816044352969,
116.052355692471)) ;
#166449=CARTESIAN_POINT('Ctrl Pts',(-20.7987557258569,-13.700942771257,
116.122092363648)) ;
#166450=CARTESIAN_POINT('Ctrl Pts',(-20.8216514465802,-13.7202811072171,
116.191829034826)) ;
#166451=CARTESIAN_POINT('Ctrl Pts',(-20.747847602877,-13.7202811104541,
116.216060075649)) ;
#166452=CARTESIAN_POINT('Ctrl Pts',(-20.6740437591738,-13.7202811136911,
116.240291116472)) ;
#166453=CARTESIAN_POINT('Ctrl Pts',(-20.6511480384506,-13.700942777731,
116.170554445295)) ;
#166454=CARTESIAN_POINT('Ctrl Pts',(-20.6263783704797,-13.9707477592159,
116.059467822879)) ;
#166455=CARTESIAN_POINT('Ctrl Pts',(-20.605916023666,-13.9325402407103,
115.997142816043)) ;
#166456=CARTESIAN_POINT('Ctrl Pts',(-20.6797198673865,-13.9325402395383,
115.972911775272)) ;
#166457=CARTESIAN_POINT('Ctrl Pts',(-20.753523711107,-13.9325402383663,
115.948680734502)) ;
#166458=CARTESIAN_POINT('Ctrl Pts',(-20.7739860579206,-13.9707477568719,
116.011005741338)) ;
#166459=CARTESIAN_POINT('Ctrl Pts',(-20.7944484047343,-14.0089552753775,
116.073330748174)) ;
#166460=CARTESIAN_POINT('Ctrl Pts',(-20.7206445610138,-14.0089552765495,
116.097561788944)) ;
#166461=CARTESIAN_POINT('Ctrl Pts',(-20.6468407172933,-14.0089552777215,
116.121792829715)) ;
#166462=CARTESIAN_POINT('Ctrl Pts',(-20.6263783704797,-13.9707477592159,
116.059467822879)) ;
#166463=CARTESIAN_POINT('Ctrl Pts',(-20.5806731004674,-14.199353333197,
115.884809057481)) ;
#166464=CARTESIAN_POINT('Ctrl Pts',(-20.5641058076827,-14.1451271098491,
115.834347756825)) ;
#166465=CARTESIAN_POINT('Ctrl Pts',(-20.6379096506688,-14.1451271117169,
115.810116713818)) ;
#166466=CARTESIAN_POINT('Ctrl Pts',(-20.7117134936549,-14.1451271135848,
115.785885670811)) ;
#166467=CARTESIAN_POINT('Ctrl Pts',(-20.7282807864396,-14.1993533369326,
115.836346971466)) ;
#166468=CARTESIAN_POINT('Ctrl Pts',(-20.7448480792243,-14.2535795602805,
115.886808272121)) ;
#166469=CARTESIAN_POINT('Ctrl Pts',(-20.6710442362382,-14.2535795584127,
115.911039315129)) ;
#166470=CARTESIAN_POINT('Ctrl Pts',(-20.5972403932521,-14.2535795565448,
115.935270358136)) ;
#166471=CARTESIAN_POINT('Ctrl Pts',(-20.5806731004674,-14.199353333197,
115.884809057481)) ;
#166472=CARTESIAN_POINT('Ctrl Pts',(-20.5181371616778,-14.3720888987135,
115.6588933938)) ;
#166473=CARTESIAN_POINT('Ctrl Pts',(-20.5066456971274,-14.3057223139106,
115.623892247061)) ;
#166474=CARTESIAN_POINT('Ctrl Pts',(-20.5804495386208,-14.3057223178457,
115.599661199507)) ;
#166475=CARTESIAN_POINT('Ctrl Pts',(-20.6542533801142,-14.3057223217808,
115.575430151953)) ;
#166476=CARTESIAN_POINT('Ctrl Pts',(-20.6657448446646,-14.3720889065837,
115.610431298692)) ;
#166477=CARTESIAN_POINT('Ctrl Pts',(-20.677236309215,-14.4384554913866,
115.645432445431)) ;
#166478=CARTESIAN_POINT('Ctrl Pts',(-20.6034324677216,-14.4384554874515,
115.669663492985)) ;
#166479=CARTESIAN_POINT('Ctrl Pts',(-20.5296286262282,-14.4384554835164,
115.693894540539)) ;
#166480=CARTESIAN_POINT('Ctrl Pts',(-20.5181371616778,-14.3720888987135,
115.6588933938)) ;
#166481=CARTESIAN_POINT('Ctrl Pts',(-20.4439011849796,-14.4765884160959,
115.397333313055)) ;
#166482=CARTESIAN_POINT('Ctrl Pts',(-20.4383100272348,-14.4028287794428,
115.380303548956)) ;
#166483=CARTESIAN_POINT('Ctrl Pts',(-20.5121138665716,-14.4028287831727,
115.356072494834)) ;
#166484=CARTESIAN_POINT('Ctrl Pts',(-20.5859177059085,-14.4028287869026,
115.331841440712)) ;
#166485=CARTESIAN_POINT('Ctrl Pts',(-20.5915088636533,-14.4765884235558,
115.34887120481)) ;
#166486=CARTESIAN_POINT('Ctrl Pts',(-20.5971000213981,-14.5503480602089,
115.365900968908)) ;
#166487=CARTESIAN_POINT('Ctrl Pts',(-20.5232961820612,-14.550348056479,
115.390132023031)) ;
#166488=CARTESIAN_POINT('Ctrl Pts',(-20.4494923427243,-14.550348052749,
115.414363077153)) ;
#166489=CARTESIAN_POINT('Ctrl Pts',(-20.4439011849796,-14.4765884160959,
115.397333313055)) ;
#166490=CARTESIAN_POINT('Ctrl Pts',(-20.3640341320984,-14.5052820126098,
115.118610145838)) ;
#166491=CARTESIAN_POINT('Ctrl Pts',(-20.364745205464,-14.4294119228674,
115.120775960982)) ;
#166492=CARTESIAN_POINT('Ctrl Pts',(-20.4385490423595,-14.4294119227756,
115.096544899424)) ;
#166493=CARTESIAN_POINT('Ctrl Pts',(-20.512352879255,-14.4294119226838,
115.072313837865)) ;
#166494=CARTESIAN_POINT('Ctrl Pts',(-20.5116418058893,-14.5052820124263,
115.070148022721)) ;
#166495=CARTESIAN_POINT('Ctrl Pts',(-20.5109307325236,-14.5811521021687,
115.067982207577)) ;
#166496=CARTESIAN_POINT('Ctrl Pts',(-20.4371268956282,-14.5811521022605,
115.092213269135)) ;
#166497=CARTESIAN_POINT('Ctrl Pts',(-20.3633230587327,-14.5811521023523,
115.116444330694)) ;
#166498=CARTESIAN_POINT('Ctrl Pts',(-20.3640341320984,-14.5052820126098,
115.118610145838)) ;
#166499=CARTESIAN_POINT('Ctrl Pts',(-20.2851290429504,-14.4562719682351,
114.842865677127)) ;
#166500=CARTESIAN_POINT('Ctrl Pts',(-20.2920831949679,-14.3837141408082,
114.864046902673)) ;
#166501=CARTESIAN_POINT('Ctrl Pts',(-20.3658870298536,-14.383714132999,
114.839815834993)) ;
#166502=CARTESIAN_POINT('Ctrl Pts',(-20.4396908647393,-14.3837141251898,
114.815584767313)) ;
#166503=CARTESIAN_POINT('Ctrl Pts',(-20.4327367127217,-14.4562719526167,
114.794403541767)) ;
#166504=CARTESIAN_POINT('Ctrl Pts',(-20.4257825607042,-14.5288297800436,
114.77322231622)) ;
#166505=CARTESIAN_POINT('Ctrl Pts',(-20.3519787258185,-14.5288297878528,
114.7974533839)) ;
#166506=CARTESIAN_POINT('Ctrl Pts',(-20.2781748909328,-14.528829795662,
114.82168445158)) ;
#166507=CARTESIAN_POINT('Ctrl Pts',(-20.2851290429504,-14.4562719682351,
114.842865677127)) ;
#166508=CARTESIAN_POINT('Ctrl Pts',(-20.2133069531199,-14.3327513043896,
114.588610844516)) ;
#166509=CARTESIAN_POINT('Ctrl Pts',(-20.2260203578033,-14.2687127593662,
114.627333824599)) ;
#166510=CARTESIAN_POINT('Ctrl Pts',(-20.299824191333,-14.2687127399002,
114.603102752789)) ;
#166511=CARTESIAN_POINT('Ctrl Pts',(-20.3736280248627,-14.2687127204341,
114.578871680979)) ;
#166512=CARTESIAN_POINT('Ctrl Pts',(-20.3609146201792,-14.3327512654575,
114.540148700895)) ;
#166513=CARTESIAN_POINT('Ctrl Pts',(-20.3482012154958,-14.3967898104809,
114.501425720811)) ;
#166514=CARTESIAN_POINT('Ctrl Pts',(-20.2743973819661,-14.3967898299469,
114.525656792621)) ;
#166515=CARTESIAN_POINT('Ctrl Pts',(-20.2005935484364,-14.396789849413,
114.549887864432)) ;
#166516=CARTESIAN_POINT('Ctrl Pts',(-20.2133069531199,-14.3327513043896,
114.588610844516)) ;
#166517=CARTESIAN_POINT('Ctrl Pts',(-20.1547039197829,-14.1436492001557,
114.37463772925)) ;
#166518=CARTESIAN_POINT('Ctrl Pts',(-20.1722614774345,-14.0927211498799,
114.428115217844)) ;
#166519=CARTESIAN_POINT('Ctrl Pts',(-20.2460653110969,-14.0927211161122,
114.403884146439)) ;
#166520=CARTESIAN_POINT('Ctrl Pts',(-20.3198691447594,-14.0927210823444,
114.379653075033)) ;
#166521=CARTESIAN_POINT('Ctrl Pts',(-20.3023115871078,-14.1436491326202,
114.326175586438)) ;
#166522=CARTESIAN_POINT('Ctrl Pts',(-20.2847540294562,-14.194577182896,
114.272698097844)) ;
#166523=CARTESIAN_POINT('Ctrl Pts',(-20.2109501957937,-14.1945772166637,
114.29692916925)) ;
#166524=CARTESIAN_POINT('Ctrl Pts',(-20.1371463621312,-14.1945772504315,
114.321160240655)) ;
#166525=CARTESIAN_POINT('Ctrl Pts',(-20.1547039197829,-14.1436492001557,
114.37463772925)) ;
#166526=CARTESIAN_POINT('Ctrl Pts',(-20.1142261546022,-13.9025966993027,
114.215876145927)) ;
#166527=CARTESIAN_POINT('Ctrl Pts',(-20.1353692170321,-13.8684250728151,
114.280274503726)) ;
#166528=CARTESIAN_POINT('Ctrl Pts',(-20.2091730526184,-13.8684250241037,
114.25604343818)) ;
#166529=CARTESIAN_POINT('Ctrl Pts',(-20.2829768882046,-13.8684249753923,
114.231812372634)) ;
#166530=CARTESIAN_POINT('Ctrl Pts',(-20.2618338257748,-13.9025966018799,
114.167414014835)) ;
#166531=CARTESIAN_POINT('Ctrl Pts',(-20.240690763345,-13.9367682283676,
114.103015657035)) ;
#166532=CARTESIAN_POINT('Ctrl Pts',(-20.1668869277587,-13.936768277079,
114.127246722581)) ;
#166533=CARTESIAN_POINT('Ctrl Pts',(-20.0930830921724,-13.9367683257904,
114.151477788127)) ;
#166534=CARTESIAN_POINT('Ctrl Pts',(-20.1142261546022,-13.9025966993027,
114.215876145927)) ;
#166535=CARTESIAN_POINT('Ctrl Pts',(-20.095524871316,-13.6267191611602,
114.123431540438)) ;
#166536=CARTESIAN_POINT('Ctrl Pts',(-20.118738436967,-13.6117593942212,
114.194136317143)) ;
#166537=CARTESIAN_POINT('Ctrl Pts',(-20.1925422763569,-13.6117593320571,
114.169905263182)) ;
#166538=CARTESIAN_POINT('Ctrl Pts',(-20.2663461157468,-13.6117592698929,
114.145674209222)) ;
#166539=CARTESIAN_POINT('Ctrl Pts',(-20.2431325500958,-13.6267190368318,
114.074969432517)) ;
#166540=CARTESIAN_POINT('Ctrl Pts',(-20.2199189844448,-13.6416788037708,
114.004264655812)) ;
#166541=CARTESIAN_POINT('Ctrl Pts',(-20.1461151450549,-13.641678865935,
114.028495709773)) ;
#166542=CARTESIAN_POINT('Ctrl Pts',(-20.072311305665,-13.6416789280991,
114.052726763733)) ;
#166543=CARTESIAN_POINT('Ctrl Pts',(-20.095524871316,-13.6267191611602,
114.123431540438)) ;
#166544=CARTESIAN_POINT('Ctrl Pts',(-20.100701888957,-13.3360804435672,
114.103739360305)) ;
#166545=CARTESIAN_POINT('Ctrl Pts',(-20.1243213452086,-13.3413907563864,
114.175680414446)) ;
#166546=CARTESIAN_POINT('Ctrl Pts',(-20.1981251900942,-13.3413906849688,
114.151449377224)) ;
#166547=CARTESIAN_POINT('Ctrl Pts',(-20.2719290349799,-13.3413906135511,
114.127218340003)) ;
#166548=CARTESIAN_POINT('Ctrl Pts',(-20.2483095787283,-13.3360803007319,
114.055277285862)) ;
#166549=CARTESIAN_POINT('Ctrl Pts',(-20.2246901224767,-13.3307699879127,
113.983336231722)) ;
#166550=CARTESIAN_POINT('Ctrl Pts',(-20.1508862775911,-13.3307700593304,
114.007567268943)) ;
#166551=CARTESIAN_POINT('Ctrl Pts',(-20.0770824327054,-13.330770130748,
114.031798306165)) ;
#166552=CARTESIAN_POINT('Ctrl Pts',(-20.100701888957,-13.3360804435672,
114.103739360305)) ;
#166553=CARTESIAN_POINT('Ctrl Pts',(-20.1300970691021,-13.0512189530207,
114.157806062876)) ;
#166554=CARTESIAN_POINT('Ctrl Pts',(-20.1524323332958,-13.076425168365,
114.22583567536)) ;
#166555=CARTESIAN_POINT('Ctrl Pts',(-20.2262361848485,-13.0764250935319,
114.201604658445)) ;
#166556=CARTESIAN_POINT('Ctrl Pts',(-20.3000400364012,-13.0764250186989,
114.17737364153)) ;
#166557=CARTESIAN_POINT('Ctrl Pts',(-20.2777047722075,-13.0512188033546,
114.109344029046)) ;
#166558=CARTESIAN_POINT('Ctrl Pts',(-20.2553695080138,-13.0260125880103,
114.041314416562)) ;
#166559=CARTESIAN_POINT('Ctrl Pts',(-20.1815656564611,-13.0260126628434,
114.065545433477)) ;
#166560=CARTESIAN_POINT('Ctrl Pts',(-20.1077618049083,-13.0260127376764,
114.089776450392)) ;
#166561=CARTESIAN_POINT('Ctrl Pts',(-20.1300970691021,-13.0512189530207,
114.157806062876)) ;
#166562=CARTESIAN_POINT('Ctrl Pts',(-20.1824935961161,-12.7925464774136,
114.281896578911)) ;
#166563=CARTESIAN_POINT('Ctrl Pts',(-20.2019377404634,-12.835849054134,
114.341120306962)) ;
#166564=CARTESIAN_POINT('Ctrl Pts',(-20.2757415992436,-12.8358489831972,
114.316889312061)) ;
#166565=CARTESIAN_POINT('Ctrl Pts',(-20.3495454580238,-12.8358489122603,
114.29265831716)) ;
#166566=CARTESIAN_POINT('Ctrl Pts',(-20.3301013136765,-12.7925463355399,
114.233434589109)) ;
#166567=CARTESIAN_POINT('Ctrl Pts',(-20.3106571693291,-12.7492437588195,
114.174210861059)) ;
#166568=CARTESIAN_POINT('Ctrl Pts',(-20.2368533105489,-12.7492438297564,
114.19844185596)) ;
#166569=CARTESIAN_POINT('Ctrl Pts',(-20.1630494517688,-12.7492439006932,
114.222672850861)) ;
#166570=CARTESIAN_POINT('Ctrl Pts',(-20.1824935961161,-12.7925464774136,
114.281896578911)) ;
#166571=CARTESIAN_POINT('Ctrl Pts',(-20.2543021382623,-12.5795095572681,
114.465309293795)) ;
#166572=CARTESIAN_POINT('Ctrl Pts',(-20.2694915221364,-12.6377483614764,
114.511573708048)) ;
#166573=CARTESIAN_POINT('Ctrl Pts',(-20.3432953874626,-12.6377483026741,
114.487342733085)) ;
#166574=CARTESIAN_POINT('Ctrl Pts',(-20.4170992527888,-12.6377482438719,
114.463111758122)) ;
#166575=CARTESIAN_POINT('Ctrl Pts',(-20.4019098689147,-12.5795094396635,
114.41684734387)) ;
#166576=CARTESIAN_POINT('Ctrl Pts',(-20.3867204850407,-12.5212706354552,
114.370582929617)) ;
#166577=CARTESIAN_POINT('Ctrl Pts',(-20.3129166197145,-12.5212706942575,
114.39481390458)) ;
#166578=CARTESIAN_POINT('Ctrl Pts',(-20.2391127543883,-12.5212707530598,
114.419044879543)) ;
#166579=CARTESIAN_POINT('Ctrl Pts',(-20.2543021382623,-12.5795095572681,
114.465309293795)) ;
#166580=CARTESIAN_POINT('Ctrl Pts',(-20.3427409626681,-12.4247175389401,
114.698907771707)) ;
#166581=CARTESIAN_POINT('Ctrl Pts',(-20.3525184658105,-12.4938489762306,
114.72868847059)) ;
#166582=CARTESIAN_POINT('Ctrl Pts',(-20.4263223372475,-12.4938489356481,
114.70445751424)) ;
#166583=CARTESIAN_POINT('Ctrl Pts',(-20.5001262086845,-12.4938488950656,
114.680226557889)) ;
#166584=CARTESIAN_POINT('Ctrl Pts',(-20.4903487055421,-12.4247174577751,
114.650445859006)) ;
#166585=CARTESIAN_POINT('Ctrl Pts',(-20.4805712023998,-12.3555860204846,
114.620665160123)) ;
#166586=CARTESIAN_POINT('Ctrl Pts',(-20.4067673309628,-12.3555860610671,
114.644896116473)) ;
#166587=CARTESIAN_POINT('Ctrl Pts',(-20.3329634595258,-12.3555861016496,
114.669127072824)) ;
#166588=CARTESIAN_POINT('Ctrl Pts',(-20.3427409626681,-12.4247175389401,
114.698907771707)) ;
#166589=CARTESIAN_POINT('Ctrl Pts',(-20.4394881561563,-12.3430591277612,
114.958446225236)) ;
#166590=CARTESIAN_POINT('Ctrl Pts',(-20.4432522784755,-12.417991968948,
114.969911136438)) ;
#166591=CARTESIAN_POINT('Ctrl Pts',(-20.5170561530844,-12.4179919531806,
114.945680189749)) ;
#166592=CARTESIAN_POINT('Ctrl Pts',(-20.5908600276934,-12.4179919374132,
114.92144924306)) ;
#166593=CARTESIAN_POINT('Ctrl Pts',(-20.5870959053743,-12.3430590962263,
114.909984331859)) ;
#166594=CARTESIAN_POINT('Ctrl Pts',(-20.5833317830551,-12.2681262550395,
114.898519420657)) ;
#166595=CARTESIAN_POINT('Ctrl Pts',(-20.5095279084461,-12.2681262708069,
114.922750367346)) ;
#166596=CARTESIAN_POINT('Ctrl Pts',(-20.4357240338372,-12.2681262865743,
114.946981314035)) ;
#166597=CARTESIAN_POINT('Ctrl Pts',(-20.4394881561563,-12.3430591277612,
114.958446225236)) ;
#166598=CARTESIAN_POINT('Ctrl Pts',(-20.5412299493208,-12.3371678726539,
115.232716171247)) ;
#166599=CARTESIAN_POINT('Ctrl Pts',(-20.5386334836071,-12.4126223874774,
115.224807757656)) ;
#166600=CARTESIAN_POINT('Ctrl Pts',(-20.6124373596408,-12.4126223993309,
115.200576815306)) ;
#166601=CARTESIAN_POINT('Ctrl Pts',(-20.6862412356744,-12.4126224111843,
115.176345872957)) ;
#166602=CARTESIAN_POINT('Ctrl Pts',(-20.688837701388,-12.3371678963608,
115.184254286548)) ;
#166603=CARTESIAN_POINT('Ctrl Pts',(-20.6914341671017,-12.2617133815373,
115.192162700139)) ;
#166604=CARTESIAN_POINT('Ctrl Pts',(-20.6176302910681,-12.2617133696838,
115.216393642489)) ;
#166605=CARTESIAN_POINT('Ctrl Pts',(-20.5438264150345,-12.2617133578303,
115.240624584839)) ;
#166606=CARTESIAN_POINT('Ctrl Pts',(-20.5412299493208,-12.3371678726539,
115.232716171247)) ;
#166607=CARTESIAN_POINT('Ctrl Pts',(-20.6396317245463,-12.4090465693171,
115.497017252412)) ;
#166608=CARTESIAN_POINT('Ctrl Pts',(-20.630894174844,-12.4795937186109,
115.47040408789)) ;
#166609=CARTESIAN_POINT('Ctrl Pts',(-20.7046980492917,-12.4795937586664,
115.44617314071)) ;
#166610=CARTESIAN_POINT('Ctrl Pts',(-20.7785019237393,-12.4795937987218,
115.42194219353)) ;
#166611=CARTESIAN_POINT('Ctrl Pts',(-20.7872394734417,-12.409046649428,
115.448555358052)) ;
#166612=CARTESIAN_POINT('Ctrl Pts',(-20.795977023144,-12.3384995001342,
115.475168522574)) ;
#166613=CARTESIAN_POINT('Ctrl Pts',(-20.7221731486963,-12.3384994600787,
115.499399469754)) ;
#166614=CARTESIAN_POINT('Ctrl Pts',(-20.6483692742486,-12.3384994200233,
115.523630416934)) ;
#166615=CARTESIAN_POINT('Ctrl Pts',(-20.6396317245463,-12.4090465693171,
115.497017252412)) ;
#166616=CARTESIAN_POINT('Ctrl Pts',(-20.7292166921784,-12.5533759332391,
115.734353125795)) ;
#166617=CARTESIAN_POINT('Ctrl Pts',(-20.7149468386475,-12.6139509456652,
115.690889456467)) ;
#166618=CARTESIAN_POINT('Ctrl Pts',(-20.788750708927,-12.6139510114575,
115.666658496591)) ;
#166619=CARTESIAN_POINT('Ctrl Pts',(-20.8625545792065,-12.6139510772497,
115.642427536716)) ;
#166620=CARTESIAN_POINT('Ctrl Pts',(-20.8768244327374,-12.5533760648236,
115.685891206043)) ;
#166621=CARTESIAN_POINT('Ctrl Pts',(-20.8910942862683,-12.4928010523974,
115.729354875371)) ;
#166622=CARTESIAN_POINT('Ctrl Pts',(-20.8172904159888,-12.4928009866052,
115.753585835247)) ;
#166623=CARTESIAN_POINT('Ctrl Pts',(-20.7434865457093,-12.4928009208129,
115.777816795123)) ;
#166624=CARTESIAN_POINT('Ctrl Pts',(-20.7292166921784,-12.5533759332391,
115.734353125795)) ;
#166625=CARTESIAN_POINT('Ctrl Pts',(-20.8038057704106,-12.75934674632,115.926107924776)) ;
#166626=CARTESIAN_POINT('Ctrl Pts',(-20.7850403755029,-12.8056312692346,
115.868951561764)) ;
#166627=CARTESIAN_POINT('Ctrl Pts',(-20.8588442393246,-12.8056313554312,
115.844720582219)) ;
#166628=CARTESIAN_POINT('Ctrl Pts',(-20.9326481031462,-12.8056314416279,
115.820489602673)) ;
#166629=CARTESIAN_POINT('Ctrl Pts',(-20.9514134980538,-12.7593469187134,
115.877645965685)) ;
#166630=CARTESIAN_POINT('Ctrl Pts',(-20.9701788929615,-12.7130623957988,
115.934802328697)) ;
#166631=CARTESIAN_POINT('Ctrl Pts',(-20.8963750291398,-12.7130623096021,
115.959033308242)) ;
#166632=CARTESIAN_POINT('Ctrl Pts',(-20.8225711653182,-12.7130622234055,
115.983264287788)) ;
#166633=CARTESIAN_POINT('Ctrl Pts',(-20.8038057704106,-12.75934674632,115.926107924776)) ;
#166634=CARTESIAN_POINT('Ctrl Pts',(-20.8591055199317,-13.0122957598429,
116.059113603157)) ;
#166635=CARTESIAN_POINT('Ctrl Pts',(-20.8371845005619,-13.0409889610471,
115.99234571717)) ;
#166636=CARTESIAN_POINT('Ctrl Pts',(-20.910988356368,-13.0409890604734,
115.968114713211)) ;
#166637=CARTESIAN_POINT('Ctrl Pts',(-20.9847922121742,-13.0409891598997,
115.943883709251)) ;
#166638=CARTESIAN_POINT('Ctrl Pts',(-21.006713231544,-13.0122959586955,
116.010651595239)) ;
#166639=CARTESIAN_POINT('Ctrl Pts',(-21.0286342509138,-12.9836027574913,
116.077419481226)) ;
#166640=CARTESIAN_POINT('Ctrl Pts',(-20.9548303951076,-12.983602658065,
116.101650485186)) ;
#166641=CARTESIAN_POINT('Ctrl Pts',(-20.8810265393014,-12.9836025586387,
116.125881489145)) ;
#166642=CARTESIAN_POINT('Ctrl Pts',(-20.8591055199317,-13.0122957598429,
116.059113603157)) ;
#166643=CARTESIAN_POINT('Ctrl Pts',(-20.8919173958629,-13.2947806869138,
116.123563569553)) ;
#166644=CARTESIAN_POINT('Ctrl Pts',(-20.868407196844,-13.3037945330256,
116.051955298721)) ;
#166645=CARTESIAN_POINT('Ctrl Pts',(-20.9422110438593,-13.303794637043,
116.027724267986)) ;
#166646=CARTESIAN_POINT('Ctrl Pts',(-21.0160148908745,-13.3037947410603,
116.003493237251)) ;
#166647=CARTESIAN_POINT('Ctrl Pts',(-21.0395250898934,-13.2947808949484,
116.075101508083)) ;
#166648=CARTESIAN_POINT('Ctrl Pts',(-21.0630352889123,-13.2857670488366,
116.146709778915)) ;
#166649=CARTESIAN_POINT('Ctrl Pts',(-20.9892314418971,-13.2857669448193,
116.170940809651)) ;
#166650=CARTESIAN_POINT('Ctrl Pts',(-20.9154275948818,-13.2857668408019,
116.195171840386)) ;
#166651=CARTESIAN_POINT('Ctrl Pts',(-20.8919173958629,-13.2947806869138,
116.123563569553)) ;
#166652=CARTESIAN_POINT('Ctrl Pts',(-20.90055362823,-13.5857642149866,116.114420488259)) ;
#166653=CARTESIAN_POINT('Ctrl Pts',(-20.8771388082436,-13.5744758994453,
116.043102726506)) ;
#166654=CARTESIAN_POINT('Ctrl Pts',(-20.9509426466584,-13.574475999467,
116.018871669575)) ;
#166655=CARTESIAN_POINT('Ctrl Pts',(-21.0247464850732,-13.5744760994887,
115.994640612644)) ;
#166656=CARTESIAN_POINT('Ctrl Pts',(-21.0481613050596,-13.58576441503,116.065958374398)) ;
#166657=CARTESIAN_POINT('Ctrl Pts',(-21.0715761250459,-13.5970527305713,
116.137276136152)) ;
#166658=CARTESIAN_POINT('Ctrl Pts',(-20.9977722866311,-13.5970526305496,
116.161507193082)) ;
#166659=CARTESIAN_POINT('Ctrl Pts',(-20.9239684482163,-13.5970525305279,
116.185738250013)) ;
#166660=CARTESIAN_POINT('Ctrl Pts',(-20.90055362823,-13.5857642149866,116.114420488259)) ;
#166661=CARTESIAN_POINT('Ctrl Pts',(-20.8851305069006,-13.8655802602202,
116.031891050549)) ;
#166662=CARTESIAN_POINT('Ctrl Pts',(-20.8634929365054,-13.8347390280632,
115.965986504196)) ;
#166663=CARTESIAN_POINT('Ctrl Pts',(-20.9372967673917,-13.8347391156571,
115.941755424335)) ;
#166664=CARTESIAN_POINT('Ctrl Pts',(-21.011100598278,-13.834739203251,115.917524344474)) ;
#166665=CARTESIAN_POINT('Ctrl Pts',(-21.0327381686732,-13.865580435408,
115.983428890826)) ;
#166666=CARTESIAN_POINT('Ctrl Pts',(-21.0543757390685,-13.8964216675651,
116.049333437179)) ;
#166667=CARTESIAN_POINT('Ctrl Pts',(-20.9805719081821,-13.8964215799712,
116.07356451704)) ;
#166668=CARTESIAN_POINT('Ctrl Pts',(-20.9067680772958,-13.8964214923772,
116.097795596901)) ;
#166669=CARTESIAN_POINT('Ctrl Pts',(-20.8851305069006,-13.8655802602202,
116.031891050549)) ;
#166670=CARTESIAN_POINT('Ctrl Pts',(-20.8474026723801,-14.1129045177148,
115.881445598306)) ;
#166671=CARTESIAN_POINT('Ctrl Pts',(-20.8291018150253,-14.0647490921529,
115.825704141381)) ;
#166672=CARTESIAN_POINT('Ctrl Pts',(-20.9029056403244,-14.0647491613001,
115.801473044502)) ;
#166673=CARTESIAN_POINT('Ctrl Pts',(-20.9767094656234,-14.0647492304473,
115.777241947622)) ;
#166674=CARTESIAN_POINT('Ctrl Pts',(-20.9950103229782,-14.1129046560093,
115.832983404548)) ;
#166675=CARTESIAN_POINT('Ctrl Pts',(-21.0133111803329,-14.1610600815713,
115.888724861473)) ;
#166676=CARTESIAN_POINT('Ctrl Pts',(-20.9395073550338,-14.161060012424,
115.912955958352)) ;
#166677=CARTESIAN_POINT('Ctrl Pts',(-20.8657035297348,-14.1610599432768,
115.937187055231)) ;
#166678=CARTESIAN_POINT('Ctrl Pts',(-20.8474026723801,-14.1129045177148,
115.881445598306)) ;
#166679=CARTESIAN_POINT('Ctrl Pts',(-20.7913821624318,-14.3092608415155,
115.675523483977)) ;
#166680=CARTESIAN_POINT('Ctrl Pts',(-20.7776954169706,-14.2473238052157,
115.633835867297)) ;
#166681=CARTESIAN_POINT('Ctrl Pts',(-20.8514992385119,-14.2473238535572,
115.609604758972)) ;
#166682=CARTESIAN_POINT('Ctrl Pts',(-20.9253030600531,-14.2473239018987,
115.585373650647)) ;
#166683=CARTESIAN_POINT('Ctrl Pts',(-20.9389898055142,-14.3092609381985,
115.627061267327)) ;
#166684=CARTESIAN_POINT('Ctrl Pts',(-20.9526765509754,-14.3711979744983,
115.668748884008)) ;
#166685=CARTESIAN_POINT('Ctrl Pts',(-20.8788727294342,-14.3711979261568,
115.692979992333)) ;
#166686=CARTESIAN_POINT('Ctrl Pts',(-20.805068907893,-14.3711978778153,
115.717211100658)) ;
#166687=CARTESIAN_POINT('Ctrl Pts',(-20.7913821624318,-14.3092608415155,
115.675523483977)) ;
#166688=CARTESIAN_POINT('Ctrl Pts',(-20.721035507872,-14.4430503329775,
115.425718401597)) ;
#166689=CARTESIAN_POINT('Ctrl Pts',(-20.7129749835062,-14.3716785302195,
115.401167346437)) ;
#166690=CARTESIAN_POINT('Ctrl Pts',(-20.786778804069,-14.371678555561,115.376936235132)) ;
#166691=CARTESIAN_POINT('Ctrl Pts',(-20.8605826246318,-14.3716785809024,
115.352705123826)) ;
#166692=CARTESIAN_POINT('Ctrl Pts',(-20.8686431489976,-14.4430503836605,
115.377256178986)) ;
#166693=CARTESIAN_POINT('Ctrl Pts',(-20.8767036733634,-14.5144221864185,
115.401807234146)) ;
#166694=CARTESIAN_POINT('Ctrl Pts',(-20.8028998528006,-14.5144221610771,
115.426038345451)) ;
#166695=CARTESIAN_POINT('Ctrl Pts',(-20.7290960322378,-14.5144221357356,
115.450269456757)) ;
#166696=CARTESIAN_POINT('Ctrl Pts',(-20.721035507872,-14.4430503329775,
115.425718401597)) ;
#166697=CARTESIAN_POINT('Ctrl Pts',(-20.6429181303812,-14.5029681127336,
115.152436570148)) ;
#166698=CARTESIAN_POINT('Ctrl Pts',(-20.6410310401035,-14.4273052047568,
115.146688799011)) ;
#166699=CARTESIAN_POINT('Ctrl Pts',(-20.7148348614875,-14.427305209291,
115.122457690207)) ;
#166700=CARTESIAN_POINT('Ctrl Pts',(-20.7886386828715,-14.4273052138253,
115.098226581403)) ;
#166701=CARTESIAN_POINT('Ctrl Pts',(-20.7905257731491,-14.5029681218021,
115.10397435254)) ;
#166702=CARTESIAN_POINT('Ctrl Pts',(-20.7924128634268,-14.5786310297789,
115.109722123678)) ;
#166703=CARTESIAN_POINT('Ctrl Pts',(-20.7186090420428,-14.5786310252447,
115.133953232482)) ;
#166704=CARTESIAN_POINT('Ctrl Pts',(-20.6448052206588,-14.5786310207104,
115.158184341285)) ;
#166705=CARTESIAN_POINT('Ctrl Pts',(-20.6429181303812,-14.5029681127336,
115.152436570148)) ;
#166706=CARTESIAN_POINT('Ctrl Pts',(-20.5625765334162,-14.4854361051768,
114.872178149454)) ;
#166707=CARTESIAN_POINT('Ctrl Pts',(-20.5670316746526,-14.4108823854582,
114.885747792019)) ;
#166708=CARTESIAN_POINT('Ctrl Pts',(-20.6408354992009,-14.4108823726848,
114.861516692854)) ;
#166709=CARTESIAN_POINT('Ctrl Pts',(-20.7146393237493,-14.4108823599115,
114.837285593688)) ;
#166710=CARTESIAN_POINT('Ctrl Pts',(-20.7101841825129,-14.4854360796301,
114.823715951122)) ;
#166711=CARTESIAN_POINT('Ctrl Pts',(-20.7057290412765,-14.5599897993486,
114.810146308557)) ;
#166712=CARTESIAN_POINT('Ctrl Pts',(-20.6319252167282,-14.559989812122,
114.834377407723)) ;
#166713=CARTESIAN_POINT('Ctrl Pts',(-20.5581213921798,-14.5599898248954,
114.858608506888)) ;
#166714=CARTESIAN_POINT('Ctrl Pts',(-20.5625765334162,-14.4854361051768,
114.872178149454)) ;
#166715=CARTESIAN_POINT('Ctrl Pts',(-20.487126571455,-14.3912934817558,
114.606906973503)) ;
#166716=CARTESIAN_POINT('Ctrl Pts',(-20.4975902895172,-14.3231998086573,
114.638777771435)) ;
#166717=CARTESIAN_POINT('Ctrl Pts',(-20.5713941181967,-14.323199784148,
114.614546684851)) ;
#166718=CARTESIAN_POINT('Ctrl Pts',(-20.6451979468761,-14.3231997596387,
114.590315598268)) ;
#166719=CARTESIAN_POINT('Ctrl Pts',(-20.6347342288138,-14.3912934327372,
114.558444800337)) ;
#166720=CARTESIAN_POINT('Ctrl Pts',(-20.6242705107516,-14.4593871058357,
114.526574002406)) ;
#166721=CARTESIAN_POINT('Ctrl Pts',(-20.5504666820722,-14.459387130345,
114.550805088989)) ;
#166722=CARTESIAN_POINT('Ctrl Pts',(-20.4766628533928,-14.4593871548543,
114.575036175572)) ;
#166723=CARTESIAN_POINT('Ctrl Pts',(-20.487126571455,-14.3912934817558,
114.606906973503)) ;
#166724=CARTESIAN_POINT('Ctrl Pts',(-20.4224950432622,-14.2271892392871,
114.374541511787)) ;
#166725=CARTESIAN_POINT('Ctrl Pts',(-20.4382221279366,-14.1704502048887,
114.422443675001)) ;
#166726=CARTESIAN_POINT('Ctrl Pts',(-20.5120259612717,-14.1704501748707,
114.398212602598)) ;
#166727=CARTESIAN_POINT('Ctrl Pts',(-20.5858297946069,-14.1704501448526,
114.373981530195)) ;
#166728=CARTESIAN_POINT('Ctrl Pts',(-20.5701027099325,-14.227189179251,
114.326079366981)) ;
#166729=CARTESIAN_POINT('Ctrl Pts',(-20.5543756252582,-14.2839282136493,
114.278177203767)) ;
#166730=CARTESIAN_POINT('Ctrl Pts',(-20.480571791923,-14.2839282436673,
114.30240827617)) ;
#166731=CARTESIAN_POINT('Ctrl Pts',(-20.4067679585879,-14.2839282736854,
114.326639348572)) ;
#166732=CARTESIAN_POINT('Ctrl Pts',(-20.4224950432622,-14.2271892392871,
114.374541511787)) ;
#166733=CARTESIAN_POINT('Ctrl Pts',(-20.3743070729178,-14.0061849375035,
114.192428883395)) ;
#166734=CARTESIAN_POINT('Ctrl Pts',(-20.3941538224714,-13.9647911087946,
114.252878880981)) ;
#166735=CARTESIAN_POINT('Ctrl Pts',(-20.4679576599053,-13.9647910776001,
114.228647821063)) ;
#166736=CARTESIAN_POINT('Ctrl Pts',(-20.5417614973391,-13.9647910464057,
114.204416761144)) ;
#166737=CARTESIAN_POINT('Ctrl Pts',(-20.5219147477856,-14.0061848751146,
114.143966763558)) ;
#166738=CARTESIAN_POINT('Ctrl Pts',(-20.502067998232,-14.0475787038235,
114.083516765971)) ;
#166739=CARTESIAN_POINT('Ctrl Pts',(-20.4282641607982,-14.047578735018,
114.10774782589)) ;
#166740=CARTESIAN_POINT('Ctrl Pts',(-20.3544603233643,-14.0475787662124,
114.131978885808)) ;
#166741=CARTESIAN_POINT('Ctrl Pts',(-20.3743070729178,-14.0061849375035,
114.192428883395)) ;
#166742=CARTESIAN_POINT('Ctrl Pts',(-20.3463468419125,-13.7418695803109,
114.071733618865)) ;
#166743=CARTESIAN_POINT('Ctrl Pts',(-20.3689113162977,-13.7188682914606,
114.14046136761)) ;
#166744=CARTESIAN_POINT('Ctrl Pts',(-20.4427151573719,-13.7188682649132,
114.11623031878)) ;
#166745=CARTESIAN_POINT('Ctrl Pts',(-20.516518998446,-13.7188682383657,
114.091999269949)) ;
#166746=CARTESIAN_POINT('Ctrl Pts',(-20.4939545240607,-13.741869527216,
114.023271521203)) ;
#166747=CARTESIAN_POINT('Ctrl Pts',(-20.4713900496754,-13.7648708160662,
113.954543772457)) ;
#166748=CARTESIAN_POINT('Ctrl Pts',(-20.3975862086013,-13.7648708426137,
113.978774821288)) ;
#166749=CARTESIAN_POINT('Ctrl Pts',(-20.3237823675271,-13.7648708691611,
114.003005870119)) ;
#166750=CARTESIAN_POINT('Ctrl Pts',(-20.3463468419125,-13.7418695803109,
114.071733618865)) ;
#166751=CARTESIAN_POINT('Ctrl Pts',(-20.3416219830562,-13.4550293844737,
114.021913569137)) ;
#166752=CARTESIAN_POINT('Ctrl Pts',(-20.3652836693087,-13.4520215652615,
114.093983248047)) ;
#166753=CARTESIAN_POINT('Ctrl Pts',(-20.439087512752,-13.4520215454244,
114.069752206432)) ;
#166754=CARTESIAN_POINT('Ctrl Pts',(-20.5128913561953,-13.4520215255873,
114.045521164817)) ;
#166755=CARTESIAN_POINT('Ctrl Pts',(-20.4892296699427,-13.4550293447994,
113.973451485907)) ;
#166756=CARTESIAN_POINT('Ctrl Pts',(-20.4655679836902,-13.4580371640116,
113.901381806997)) ;
#166757=CARTESIAN_POINT('Ctrl Pts',(-20.3917641402469,-13.4580371838487,
113.925612848612)) ;
#166758=CARTESIAN_POINT('Ctrl Pts',(-20.3179602968036,-13.4580372036859,
113.949843890227)) ;
#166759=CARTESIAN_POINT('Ctrl Pts',(-20.3416219830562,-13.4550293844737,
114.021913569137)) ;
#166760=CARTESIAN_POINT('Ctrl Pts',(-20.3614601534258,-13.1635845721582,
114.04665004701)) ;
#166761=CARTESIAN_POINT('Ctrl Pts',(-20.3845110947562,-13.180922781359,
114.11685949526)) ;
#166762=CARTESIAN_POINT('Ctrl Pts',(-20.4583149391496,-13.1809227707576,
114.092628456539)) ;
#166763=CARTESIAN_POINT('Ctrl Pts',(-20.532118783543,-13.1809227601562,
114.068397417818)) ;
#166764=CARTESIAN_POINT('Ctrl Pts',(-20.5090678422126,-13.1635845509553,
113.998187969568)) ;
#166765=CARTESIAN_POINT('Ctrl Pts',(-20.4860169008822,-13.1462463417545,
113.927978521319)) ;
#166766=CARTESIAN_POINT('Ctrl Pts',(-20.4122130564889,-13.1462463523559,
113.95220956004)) ;
#166767=CARTESIAN_POINT('Ctrl Pts',(-20.3384092120955,-13.1462463629573,
113.976440598761)) ;
#166768=CARTESIAN_POINT('Ctrl Pts',(-20.3614601534258,-13.1635845721582,
114.04665004701)) ;
#166769=CARTESIAN_POINT('Ctrl Pts',(-20.4044535755017,-12.8938493439813,
114.142385565385)) ;
#166770=CARTESIAN_POINT('Ctrl Pts',(-20.4252657787376,-12.9300476003649,
114.205776178532)) ;
#166771=CARTESIAN_POINT('Ctrl Pts',(-20.499069623255,-12.9300475948517,
114.181545140189)) ;
#166772=CARTESIAN_POINT('Ctrl Pts',(-20.5728734677724,-12.9300475893384,
114.157314101845)) ;
#166773=CARTESIAN_POINT('Ctrl Pts',(-20.5520612645364,-12.8938493329547,
114.093923488698)) ;
#166774=CARTESIAN_POINT('Ctrl Pts',(-20.5312490613004,-12.857651076571,
114.030532875551)) ;
#166775=CARTESIAN_POINT('Ctrl Pts',(-20.4574452167831,-12.8576510820843,
114.054763913894)) ;
#166776=CARTESIAN_POINT('Ctrl Pts',(-20.3836413722657,-12.8576510875976,
114.078994952238)) ;
#166777=CARTESIAN_POINT('Ctrl Pts',(-20.4044535755017,-12.8938493439813,
114.142385565385)) ;
#166778=CARTESIAN_POINT('Ctrl Pts',(-20.4694496412937,-12.658475902558,
114.304658716124)) ;
#166779=CARTESIAN_POINT('Ctrl Pts',(-20.4864933769325,-12.7111646806542,
114.356571184894)) ;
#166780=CARTESIAN_POINT('Ctrl Pts',(-20.5602972205623,-12.7111646805121,
114.332340143848)) ;
#166781=CARTESIAN_POINT('Ctrl Pts',(-20.6341010641921,-12.7111646803699,
114.308109102801)) ;
#166782=CARTESIAN_POINT('Ctrl Pts',(-20.6170573285533,-12.6584759022737,
114.25619663403)) ;
#166783=CARTESIAN_POINT('Ctrl Pts',(-20.6000135929145,-12.6057871241775,
114.20428416526)) ;
#166784=CARTESIAN_POINT('Ctrl Pts',(-20.5262097492847,-12.6057871243196,
114.228515206307)) ;
#166785=CARTESIAN_POINT('Ctrl Pts',(-20.4524059056549,-12.6057871244618,
114.252746247354)) ;
#166786=CARTESIAN_POINT('Ctrl Pts',(-20.4694496412937,-12.658475902558,
114.304658716124)) ;
#166787=CARTESIAN_POINT('Ctrl Pts',(-20.5508406891179,-12.480124052921,
114.517369062638)) ;
#166788=CARTESIAN_POINT('Ctrl Pts',(-20.5629548634475,-12.545344547809,
114.554266882997)) ;
#166789=CARTESIAN_POINT('Ctrl Pts',(-20.6367587064007,-12.5453445488469,
114.530035839889)) ;
#166790=CARTESIAN_POINT('Ctrl Pts',(-20.7105625493539,-12.5453445498848,
114.505804796782)) ;
#166791=CARTESIAN_POINT('Ctrl Pts',(-20.6984483750243,-12.4801240549968,
114.468906976423)) ;
#166792=CARTESIAN_POINT('Ctrl Pts',(-20.6863342006947,-12.4149035601088,
114.432009156064)) ;
#166793=CARTESIAN_POINT('Ctrl Pts',(-20.6125303577415,-12.414903559071,
114.456240199172)) ;
#166794=CARTESIAN_POINT('Ctrl Pts',(-20.5387265147883,-12.4149035580331,
114.480471242279)) ;
#166795=CARTESIAN_POINT('Ctrl Pts',(-20.5508406891179,-12.480124052921,
114.517369062638)) ;
#166796=CARTESIAN_POINT('Ctrl Pts',(-20.6459051268629,-12.366810202119,
114.77115798259)) ;
#166797=CARTESIAN_POINT('Ctrl Pts',(-20.6521390295966,-12.4400414291151,
114.790145444413)) ;
#166798=CARTESIAN_POINT('Ctrl Pts',(-20.7259428719618,-12.4400414300861,
114.765914399515)) ;
#166799=CARTESIAN_POINT('Ctrl Pts',(-20.799746714327,-12.4400414310572,
114.741683354616)) ;
#166800=CARTESIAN_POINT('Ctrl Pts',(-20.7935128115933,-12.3668102040611,
114.722695892793)) ;
#166801=CARTESIAN_POINT('Ctrl Pts',(-20.7872789088596,-12.2935789770651,
114.70370843097)) ;
#166802=CARTESIAN_POINT('Ctrl Pts',(-20.7134750664944,-12.293578976094,
114.727939475869)) ;
#166803=CARTESIAN_POINT('Ctrl Pts',(-20.6396712241292,-12.293578975123,
114.752170520767)) ;
#166804=CARTESIAN_POINT('Ctrl Pts',(-20.6459051268629,-12.366810202119,
114.77115798259)) ;
#166805=CARTESIAN_POINT('Ctrl Pts',(-20.7458815806501,-12.3300613553443,
115.040439167001)) ;
#166806=CARTESIAN_POINT('Ctrl Pts',(-20.745872671566,-12.4059660659724,
115.040412031318)) ;
#166807=CARTESIAN_POINT('Ctrl Pts',(-20.8196765141725,-12.4059660657075,
115.016180987155)) ;
#166808=CARTESIAN_POINT('Ctrl Pts',(-20.8934803567791,-12.4059660654426,
114.991949942991)) ;
#166809=CARTESIAN_POINT('Ctrl Pts',(-20.8934892658632,-12.3300613548144,
114.991977078674)) ;
#166810=CARTESIAN_POINT('Ctrl Pts',(-20.8934981749473,-12.2541566441862,
114.992004214356)) ;
#166811=CARTESIAN_POINT('Ctrl Pts',(-20.8196943323408,-12.2541566444512,
115.01623525852)) ;
#166812=CARTESIAN_POINT('Ctrl Pts',(-20.7458904897342,-12.2541566447161,
115.040466302683)) ;
#166813=CARTESIAN_POINT('Ctrl Pts',(-20.7458815806501,-12.3300613553443,
115.040439167001)) ;
#166814=CARTESIAN_POINT('Ctrl Pts',(-20.8468477493283,-12.3711193571588,
115.312306178945)) ;
#166815=CARTESIAN_POINT('Ctrl Pts',(-20.8405264551882,-12.4442691147832,
115.293052536951)) ;
#166816=CARTESIAN_POINT('Ctrl Pts',(-20.9143302989252,-12.4442691147866,
115.268821496231)) ;
#166817=CARTESIAN_POINT('Ctrl Pts',(-20.9881341426622,-12.44426911479,115.24459045551)) ;
#166818=CARTESIAN_POINT('Ctrl Pts',(-20.9944554368023,-12.3711193571657,
115.263844097504)) ;
#166819=CARTESIAN_POINT('Ctrl Pts',(-21.0007767309424,-12.2979695995413,
115.283097739498)) ;
#166820=CARTESIAN_POINT('Ctrl Pts',(-20.9269728872054,-12.2979695995379,
115.307328780218)) ;
#166821=CARTESIAN_POINT('Ctrl Pts',(-20.8531690434684,-12.2979695995345,
115.331559820939)) ;
#166822=CARTESIAN_POINT('Ctrl Pts',(-20.8468477493283,-12.3711193571588,
115.312306178945)) ;
#166823=CARTESIAN_POINT('Ctrl Pts',(-20.9400118268714,-12.4860834955726,
115.560871243411)) ;
#166824=CARTESIAN_POINT('Ctrl Pts',(-20.927904670528,-12.5513121633835,
115.523994798755)) ;
#166825=CARTESIAN_POINT('Ctrl Pts',(-21.0017085151598,-12.5513121652031,
115.49976376076)) ;
#166826=CARTESIAN_POINT('Ctrl Pts',(-21.0755123597916,-12.5513121670227,
115.475532722765)) ;
#166827=CARTESIAN_POINT('Ctrl Pts',(-21.087619516135,-12.4860834992117,
115.512409167422)) ;
#166828=CARTESIAN_POINT('Ctrl Pts',(-21.0997266724784,-12.4208548314008,
115.549285612078)) ;
#166829=CARTESIAN_POINT('Ctrl Pts',(-21.0259228278466,-12.4208548295812,
115.573516650073)) ;
#166830=CARTESIAN_POINT('Ctrl Pts',(-20.9521189832147,-12.4208548277616,
115.597747688068)) ;
#166831=CARTESIAN_POINT('Ctrl Pts',(-20.9400118268714,-12.4860834955726,
115.560871243411)) ;
#166832=CARTESIAN_POINT('Ctrl Pts',(-21.0218131787759,-12.6694591781323,
115.774349736538)) ;
#166833=CARTESIAN_POINT('Ctrl Pts',(-21.0047147067805,-12.7219791159764,
115.72227054989)) ;
#166834=CARTESIAN_POINT('Ctrl Pts',(-21.0785185527964,-12.7219791238396,
115.698039516111)) ;
#166835=CARTESIAN_POINT('Ctrl Pts',(-21.1523223988123,-12.7219791317028,
115.673808482332)) ;
#166836=CARTESIAN_POINT('Ctrl Pts',(-21.1694208708077,-12.6694591938587,
115.72588766898)) ;
#166837=CARTESIAN_POINT('Ctrl Pts',(-21.1865193428031,-12.6169392560146,
115.777966855628)) ;
#166838=CARTESIAN_POINT('Ctrl Pts',(-21.1127154967872,-12.6169392481514,
115.802197889407)) ;
#166839=CARTESIAN_POINT('Ctrl Pts',(-21.0389116507713,-12.6169392402883,
115.826428923186)) ;
#166840=CARTESIAN_POINT('Ctrl Pts',(-21.0218131787759,-12.6694591781323,
115.774349736538)) ;
#166841=CARTESIAN_POINT('Ctrl Pts',(-21.0853187896977,-12.9054683696908,
115.932363519269)) ;
#166842=CARTESIAN_POINT('Ctrl Pts',(-21.0644942259678,-12.9415855764778,
115.868935258532)) ;
#166843=CARTESIAN_POINT('Ctrl Pts',(-21.1382980722319,-12.9415855922766,
115.844704225508)) ;
#166844=CARTESIAN_POINT('Ctrl Pts',(-21.212101918496,-12.9415856080754,
115.820473192485)) ;
#166845=CARTESIAN_POINT('Ctrl Pts',(-21.232926482226,-12.9054684012884,
115.883901453223)) ;
#166846=CARTESIAN_POINT('Ctrl Pts',(-21.2537510459559,-12.8693511945013,
115.947329713961)) ;
#166847=CARTESIAN_POINT('Ctrl Pts',(-21.1799471996917,-12.8693511787026,
115.971560746984)) ;
#166848=CARTESIAN_POINT('Ctrl Pts',(-21.1061433534276,-12.8693511629038,
115.995791780007)) ;
#166849=CARTESIAN_POINT('Ctrl Pts',(-21.0853187896977,-12.9054683696908,
115.932363519269)) ;
#166850=CARTESIAN_POINT('Ctrl Pts',(-21.1275223807036,-13.1783417993353,
116.025441846581)) ;
#166851=CARTESIAN_POINT('Ctrl Pts',(-21.1044548326585,-13.1954587831432,
115.955181817674)) ;
#166852=CARTESIAN_POINT('Ctrl Pts',(-21.1782586780653,-13.1954588083928,
115.93095078204)) ;
#166853=CARTESIAN_POINT('Ctrl Pts',(-21.252062523472,-13.1954588336424,
115.906719746405)) ;
#166854=CARTESIAN_POINT('Ctrl Pts',(-21.2751300715171,-13.1783418498345,
115.976979775312)) ;
#166855=CARTESIAN_POINT('Ctrl Pts',(-21.2981976195622,-13.1612248660266,
116.047239804219)) ;
#166856=CARTESIAN_POINT('Ctrl Pts',(-21.2243937741555,-13.161224840777,
116.071470839854)) ;
#166857=CARTESIAN_POINT('Ctrl Pts',(-21.1505899287487,-13.1612248155274,
116.095701875488)) ;
#166858=CARTESIAN_POINT('Ctrl Pts',(-21.1275223807036,-13.1783417993353,
116.025441846581)) ;
#166859=CARTESIAN_POINT('Ctrl Pts',(-21.1459730069986,-13.4677014527882,
116.046259246478)) ;
#166860=CARTESIAN_POINT('Ctrl Pts',(-21.1223160522397,-13.4646398279822,
115.974203979966)) ;
#166861=CARTESIAN_POINT('Ctrl Pts',(-21.1961198953758,-13.4646398615466,
115.949972937416)) ;
#166862=CARTESIAN_POINT('Ctrl Pts',(-21.269923738512,-13.464639895111,115.925741894866)) ;
#166863=CARTESIAN_POINT('Ctrl Pts',(-21.2935806932709,-13.4677015199171,
115.997797161377)) ;
#166864=CARTESIAN_POINT('Ctrl Pts',(-21.3172376480298,-13.4707631447231,
116.069852427888)) ;
#166865=CARTESIAN_POINT('Ctrl Pts',(-21.2434338048937,-13.4707631111587,
116.094083470438)) ;
#166866=CARTESIAN_POINT('Ctrl Pts',(-21.1696299617576,-13.4707630775943,
116.118314512989)) ;
#166867=CARTESIAN_POINT('Ctrl Pts',(-21.1459730069986,-13.4677014527882,
116.046259246478)) ;
#166868=CARTESIAN_POINT('Ctrl Pts',(-21.1402886926304,-13.7542094632266,
115.99348562837)) ;
#166869=CARTESIAN_POINT('Ctrl Pts',(-21.1177281868373,-13.7311394476093,
115.924769968664)) ;
#166870=CARTESIAN_POINT('Ctrl Pts',(-21.1915320264503,-13.7311394879972,
115.900538915382)) ;
#166871=CARTESIAN_POINT('Ctrl Pts',(-21.2653358660634,-13.7311395283851,
115.876307862101)) ;
#166872=CARTESIAN_POINT('Ctrl Pts',(-21.2878963718565,-13.7542095440024,
115.945023521808)) ;
#166873=CARTESIAN_POINT('Ctrl Pts',(-21.3104568776496,-13.7772795596197,
116.013739181515)) ;
#166874=CARTESIAN_POINT('Ctrl Pts',(-21.2366530380365,-13.7772795192318,
116.037970234796)) ;
#166875=CARTESIAN_POINT('Ctrl Pts',(-21.1628491984234,-13.7772794788439,
116.062201288077)) ;
#166876=CARTESIAN_POINT('Ctrl Pts',(-21.1402886926304,-13.7542094632266,
115.99348562837)) ;
#166877=CARTESIAN_POINT('Ctrl Pts',(-21.111182052806,-14.0177953901298,
115.869184389673)) ;
#166878=CARTESIAN_POINT('Ctrl Pts',(-21.091358617658,-13.976288401055,115.808805405729)) ;
#166879=CARTESIAN_POINT('Ctrl Pts',(-21.1651624521965,-13.9762884453848,
115.784574336992)) ;
#166880=CARTESIAN_POINT('Ctrl Pts',(-21.238966286735,-13.9762884897146,
115.760343268254)) ;
#166881=CARTESIAN_POINT('Ctrl Pts',(-21.258789721883,-14.0177954787893,
115.820722252198)) ;
#166882=CARTESIAN_POINT('Ctrl Pts',(-21.278613157031,-14.0593024678641,
115.881101236141)) ;
#166883=CARTESIAN_POINT('Ctrl Pts',(-21.2048093224926,-14.0593024235343,
115.905332304878)) ;
#166884=CARTESIAN_POINT('Ctrl Pts',(-21.131005487954,-14.0593023792045,
115.929563373616)) ;
#166885=CARTESIAN_POINT('Ctrl Pts',(-21.111182052806,-14.0177953901298,
115.869184389673)) ;
#166886=CARTESIAN_POINT('Ctrl Pts',(-21.0622744394062,-14.2358411050757,
115.684975992788)) ;
#166887=CARTESIAN_POINT('Ctrl Pts',(-21.0465664537973,-14.1790508956255,
115.63713200424)) ;
#166888=CARTESIAN_POINT('Ctrl Pts',(-21.1203702834702,-14.1790509350975,
115.612900920683)) ;
#166889=CARTESIAN_POINT('Ctrl Pts',(-21.194174113143,-14.1790509745695,
115.588669837125)) ;
#166890=CARTESIAN_POINT('Ctrl Pts',(-21.2098820987519,-14.2358411840197,
115.636513825673)) ;
#166891=CARTESIAN_POINT('Ctrl Pts',(-21.2255900843608,-14.2926313934699,
115.684357814221)) ;
#166892=CARTESIAN_POINT('Ctrl Pts',(-21.1517862546879,-14.2926313539979,
115.708588897779)) ;
#166893=CARTESIAN_POINT('Ctrl Pts',(-21.077982425015,-14.2926313145259,
115.732819981336)) ;
#166894=CARTESIAN_POINT('Ctrl Pts',(-21.0622744394062,-14.2358411050757,
115.684975992788)) ;
#166895=CARTESIAN_POINT('Ctrl Pts',(-20.9969244848175,-14.3973545116793,
115.450360447724)) ;
#166896=CARTESIAN_POINT('Ctrl Pts',(-20.9864923098944,-14.3292054144305,
115.418585727457)) ;
#166897=CARTESIAN_POINT('Ctrl Pts',(-21.0602961341888,-14.3292054449857,
115.394354627517)) ;
#166898=CARTESIAN_POINT('Ctrl Pts',(-21.1340999584832,-14.3292054755409,
115.370123527578)) ;
#166899=CARTESIAN_POINT('Ctrl Pts',(-21.1445321334063,-14.3973545727897,
115.401898247845)) ;
#166900=CARTESIAN_POINT('Ctrl Pts',(-21.1549643083294,-14.4655036700385,
115.433672968112)) ;
#166901=CARTESIAN_POINT('Ctrl Pts',(-21.081160484035,-14.4655036394833,
115.457904068052)) ;
#166902=CARTESIAN_POINT('Ctrl Pts',(-21.0073566597406,-14.4655036089281,
115.482135167991)) ;
#166903=CARTESIAN_POINT('Ctrl Pts',(-20.9969244848175,-14.3973545116793,
115.450360447724)) ;
#166904=CARTESIAN_POINT('Ctrl Pts',(-20.9210657871025,-14.487909543941,
115.183827051948)) ;
#166905=CARTESIAN_POINT('Ctrl Pts',(-20.9166489046695,-14.4133393487521,
115.170373942196)) ;
#166906=CARTESIAN_POINT('Ctrl Pts',(-20.9904527246687,-14.4133393631785,
115.146142829174)) ;
#166907=CARTESIAN_POINT('Ctrl Pts',(-21.0642565446678,-14.413339377605,
115.121911716152)) ;
#166908=CARTESIAN_POINT('Ctrl Pts',(-21.0686734271008,-14.4879095727939,
115.135364825905)) ;
#166909=CARTESIAN_POINT('Ctrl Pts',(-21.0730903095338,-14.5624797679828,
115.148817935657)) ;
#166910=CARTESIAN_POINT('Ctrl Pts',(-20.9992864895347,-14.5624797535563,
115.173049048679)) ;
#166911=CARTESIAN_POINT('Ctrl Pts',(-20.9254826695355,-14.5624797391299,
115.197280161701)) ;
#166912=CARTESIAN_POINT('Ctrl Pts',(-20.9210657871025,-14.487909543941,
115.183827051948)) ;
#166913=CARTESIAN_POINT('Ctrl Pts',(-20.8410002283841,-14.501998059837,
114.904561059631)) ;
#166914=CARTESIAN_POINT('Ctrl Pts',(-20.842899355212,-14.4263362561648,
114.910345495132)) ;
#166915=CARTESIAN_POINT('Ctrl Pts',(-20.9167031727645,-14.4263362496198,
114.886114374658)) ;
#166916=CARTESIAN_POINT('Ctrl Pts',(-20.9905069903171,-14.4263362430748,
114.861883254185)) ;
#166917=CARTESIAN_POINT('Ctrl Pts',(-20.9886078634892,-14.501998046747,
114.856098818683)) ;
#166918=CARTESIAN_POINT('Ctrl Pts',(-20.9867087366614,-14.5776598504192,
114.850314383182)) ;
#166919=CARTESIAN_POINT('Ctrl Pts',(-20.9129049191088,-14.5776598569642,
114.874545503655)) ;
#166920=CARTESIAN_POINT('Ctrl Pts',(-20.8391011015563,-14.5776598635092,
114.898776624129)) ;
#166921=CARTESIAN_POINT('Ctrl Pts',(-20.8410002283841,-14.501998059837,
114.904561059631)) ;
#166922=CARTESIAN_POINT('Ctrl Pts',(-20.7628140637106,-14.4383564825309,
114.63092278003)) ;
#166923=CARTESIAN_POINT('Ctrl Pts',(-20.7709091130621,-14.3670278101873,
114.65557899596)) ;
#166924=CARTESIAN_POINT('Ctrl Pts',(-20.8447129301326,-14.3670277794582,
114.631347874018)) ;
#166925=CARTESIAN_POINT('Ctrl Pts',(-20.918516747203,-14.3670277487292,
114.607116752076)) ;
#166926=CARTESIAN_POINT('Ctrl Pts',(-20.9104216978515,-14.4383564210728,
114.582460536145)) ;
#166927=CARTESIAN_POINT('Ctrl Pts',(-20.9023266485,-14.5096850934165,114.557804320215)) ;
#166928=CARTESIAN_POINT('Ctrl Pts',(-20.8285228314295,-14.5096851241455,
114.582035442157)) ;
#166929=CARTESIAN_POINT('Ctrl Pts',(-20.7547190143591,-14.5096851548746,
114.606266564099)) ;
#166930=CARTESIAN_POINT('Ctrl Pts',(-20.7628140637106,-14.4383564825309,
114.63092278003)) ;
#166931=CARTESIAN_POINT('Ctrl Pts',(-20.6932450307031,-14.3021834028963,
114.383646838591)) ;
#166932=CARTESIAN_POINT('Ctrl Pts',(-20.706940971323,-14.2402581580985,
114.425362465725)) ;
#166933=CARTESIAN_POINT('Ctrl Pts',(-20.7807447905397,-14.2402581030473,
114.40113135032)) ;
#166934=CARTESIAN_POINT('Ctrl Pts',(-20.8545486097562,-14.2402580479961,
114.376900234914)) ;
#166935=CARTESIAN_POINT('Ctrl Pts',(-20.8408526691363,-14.3021832927938,
114.33518460778)) ;
#166936=CARTESIAN_POINT('Ctrl Pts',(-20.8271567285164,-14.3641085375916,
114.293468980646)) ;
#166937=CARTESIAN_POINT('Ctrl Pts',(-20.7533529092998,-14.3641085926428,
114.317700096051)) ;
#166938=CARTESIAN_POINT('Ctrl Pts',(-20.6795490900832,-14.364108647694,
114.341931211457)) ;
#166939=CARTESIAN_POINT('Ctrl Pts',(-20.6932450307031,-14.3021834028963,
114.383646838591)) ;
#166940=CARTESIAN_POINT('Ctrl Pts',(-20.6374385512725,-14.1010124276425,
114.178000289426)) ;
#166941=CARTESIAN_POINT('Ctrl Pts',(-20.6557888301489,-14.0530410261757,
114.233892280025)) ;
#166942=CARTESIAN_POINT('Ctrl Pts',(-20.7295926537291,-14.0530409478965,
114.209661177911)) ;
#166943=CARTESIAN_POINT('Ctrl Pts',(-20.8033964773092,-14.0530408696173,
114.185430075796)) ;
#166944=CARTESIAN_POINT('Ctrl Pts',(-20.7850461984329,-14.101012271084,
114.129538085197)) ;
#166945=CARTESIAN_POINT('Ctrl Pts',(-20.7666959195565,-14.1489836725507,
114.073646094597)) ;
#166946=CARTESIAN_POINT('Ctrl Pts',(-20.6928920959764,-14.14898375083,114.097877196711)) ;
#166947=CARTESIAN_POINT('Ctrl Pts',(-20.6190882723962,-14.1489838291092,
114.122108298826)) ;
#166948=CARTESIAN_POINT('Ctrl Pts',(-20.6374385512725,-14.1010124276425,
114.178000289426)) ;
#166949=CARTESIAN_POINT('Ctrl Pts',(-20.6010815469782,-13.8533300885713,
114.031993487533)) ;
#166950=CARTESIAN_POINT('Ctrl Pts',(-20.622726691192,-13.822581157602,114.097921106379)) ;
#166951=CARTESIAN_POINT('Ctrl Pts',(-20.696530521615,-13.8225810627118,
114.073690025107)) ;
#166952=CARTESIAN_POINT('Ctrl Pts',(-20.770334352038,-13.8225809678216,
114.049458943834)) ;
#166953=CARTESIAN_POINT('Ctrl Pts',(-20.7486892078241,-13.8533298987908,
113.983531324988)) ;
#166954=CARTESIAN_POINT('Ctrl Pts',(-20.7270440636103,-13.8840788297601,
113.917603706141)) ;
#166955=CARTESIAN_POINT('Ctrl Pts',(-20.6532402331873,-13.8840789246503,
113.941834787413)) ;
#166956=CARTESIAN_POINT('Ctrl Pts',(-20.5794364027644,-13.8840790195405,
113.966065868686)) ;
#166957=CARTESIAN_POINT('Ctrl Pts',(-20.6010815469782,-13.8533300885713,
114.031993487533)) ;
#166958=CARTESIAN_POINT('Ctrl Pts',(-20.586642419132,-13.5731370136184,
113.952522413713)) ;
#166959=CARTESIAN_POINT('Ctrl Pts',(-20.6100618395561,-13.5619047330003,
114.023854191675)) ;
#166960=CARTESIAN_POINT('Ctrl Pts',(-20.6838656781738,-13.5619046275825,
113.999623135362)) ;
#166961=CARTESIAN_POINT('Ctrl Pts',(-20.7576695167915,-13.5619045221647,
113.975392079049)) ;
#166962=CARTESIAN_POINT('Ctrl Pts',(-20.7342500963673,-13.5731368027828,
113.904060301088)) ;
#166963=CARTESIAN_POINT('Ctrl Pts',(-20.7108306759432,-13.5843690834008,
113.832728523127)) ;
#166964=CARTESIAN_POINT('Ctrl Pts',(-20.6370268373256,-13.5843691888186,
113.856959579439)) ;
#166965=CARTESIAN_POINT('Ctrl Pts',(-20.5632229987079,-13.5843692942365,
113.881190635752)) ;
#166966=CARTESIAN_POINT('Ctrl Pts',(-20.586642419132,-13.5731370136184,
113.952522413713)) ;
#166967=CARTESIAN_POINT('Ctrl Pts',(-20.5964562900944,-13.2811248351023,
113.946846374768)) ;
#166968=CARTESIAN_POINT('Ctrl Pts',(-20.6199611334795,-13.2902630338005,
114.018438337316)) ;
#166969=CARTESIAN_POINT('Ctrl Pts',(-20.6937649811193,-13.2902629265376,
113.994207308483)) ;
#166970=CARTESIAN_POINT('Ctrl Pts',(-20.767568828759,-13.2902628192747,
113.969976279651)) ;
#166971=CARTESIAN_POINT('Ctrl Pts',(-20.7440639853739,-13.2811246205765,
113.898384317102)) ;
#166972=CARTESIAN_POINT('Ctrl Pts',(-20.7205591419887,-13.2719864218783,
113.826792354554)) ;
#166973=CARTESIAN_POINT('Ctrl Pts',(-20.646755294349,-13.2719865291412,
113.851023383387)) ;
#166974=CARTESIAN_POINT('Ctrl Pts',(-20.5729514467092,-13.2719866364041,
113.87525441222)) ;
#166975=CARTESIAN_POINT('Ctrl Pts',(-20.5964562900944,-13.2811248351023,
113.946846374768)) ;
#166976=CARTESIAN_POINT('Ctrl Pts',(-20.6302134446159,-13.0003515927813,
114.014286748923)) ;
#166977=CARTESIAN_POINT('Ctrl Pts',(-20.6521282105241,-13.0291058472193,
114.081035592042)) ;
#166978=CARTESIAN_POINT('Ctrl Pts',(-20.7259320669489,-13.029105747077,
114.056804589967)) ;
#166979=CARTESIAN_POINT('Ctrl Pts',(-20.7997359233737,-13.0291056469348,
114.032573587892)) ;
#166980=CARTESIAN_POINT('Ctrl Pts',(-20.7778211574655,-13.0003513924967,
113.965824744773)) ;
#166981=CARTESIAN_POINT('Ctrl Pts',(-20.7559063915572,-12.9715971380587,
113.899075901654)) ;
#166982=CARTESIAN_POINT('Ctrl Pts',(-20.6821025351324,-12.971597238201,
113.923306903729)) ;
#166983=CARTESIAN_POINT('Ctrl Pts',(-20.6082986787076,-12.9715973383433,
113.947537905805)) ;
#166984=CARTESIAN_POINT('Ctrl Pts',(-20.6302134446159,-13.0003515927813,
114.014286748923)) ;
#166985=CARTESIAN_POINT('Ctrl Pts',(-20.6868771702669,-12.7476820967297,
114.151219214788)) ;
#166986=CARTESIAN_POINT('Ctrl Pts',(-20.705606395181,-12.7941196142379,
114.208265414002)) ;
#166987=CARTESIAN_POINT('Ctrl Pts',(-20.7794102592639,-12.794119529764,
114.184034435252)) ;
#166988=CARTESIAN_POINT('Ctrl Pts',(-20.8532141233468,-12.7941194452901,
114.159803456503)) ;
#166989=CARTESIAN_POINT('Ctrl Pts',(-20.8344848984328,-12.7476819277819,
114.102757257289)) ;
#166990=CARTESIAN_POINT('Ctrl Pts',(-20.8157556735187,-12.7012444102737,
114.045711058075)) ;
#166991=CARTESIAN_POINT('Ctrl Pts',(-20.7419518094358,-12.7012444947476,
114.069942036824)) ;
#166992=CARTESIAN_POINT('Ctrl Pts',(-20.6681479453528,-12.7012445792215,
114.094173015574)) ;
#166993=CARTESIAN_POINT('Ctrl Pts',(-20.6868771702669,-12.7476820967297,
114.151219214788)) ;
#166994=CARTESIAN_POINT('Ctrl Pts',(-20.7618646026425,-12.5456564605608,
114.344400176223)) ;
#166995=CARTESIAN_POINT('Ctrl Pts',(-20.7761148264351,-12.6062676271749,
114.387804060677)) ;
#166996=CARTESIAN_POINT('Ctrl Pts',(-20.8499186963736,-12.6062675641062,
114.363573099762)) ;
#166997=CARTESIAN_POINT('Ctrl Pts',(-20.9237225663121,-12.6062675010375,
114.339342138848)) ;
#166998=CARTESIAN_POINT('Ctrl Pts',(-20.9094723425195,-12.5456563344234,
114.295938254394)) ;
#166999=CARTESIAN_POINT('Ctrl Pts',(-20.8952221187268,-12.4850451678094,
114.25253436994)) ;
#167000=CARTESIAN_POINT('Ctrl Pts',(-20.8214182487883,-12.4850452308781,
114.276765330855)) ;
#167001=CARTESIAN_POINT('Ctrl Pts',(-20.7476143788498,-12.4850452939468,
114.300996291769)) ;
#167002=CARTESIAN_POINT('Ctrl Pts',(-20.7618646026425,-12.5456564605608,
114.344400176223)) ;
#167003=CARTESIAN_POINT('Ctrl Pts',(-20.851984110481,-12.4041536111177,
114.583349964643)) ;
#167004=CARTESIAN_POINT('Ctrl Pts',(-20.8606991958322,-12.4747346832578,
114.609894710435)) ;
#167005=CARTESIAN_POINT('Ctrl Pts',(-20.9345030691503,-12.474734646304,
114.585663759814)) ;
#167006=CARTESIAN_POINT('Ctrl Pts',(-21.0083069424685,-12.4747346093502,
114.561432809193)) ;
#167007=CARTESIAN_POINT('Ctrl Pts',(-20.9995918571173,-12.4041535372102,
114.534888063401)) ;
#167008=CARTESIAN_POINT('Ctrl Pts',(-20.9908767717661,-12.3335724650701,
114.50834331761)) ;
#167009=CARTESIAN_POINT('Ctrl Pts',(-20.917072898448,-12.3335725020239,
114.532574268231)) ;
#167010=CARTESIAN_POINT('Ctrl Pts',(-20.8432690251298,-12.3335725389777,
114.556805218851)) ;
#167011=CARTESIAN_POINT('Ctrl Pts',(-20.851984110481,-12.4041536111177,
114.583349964643)) ;
#167012=CARTESIAN_POINT('Ctrl Pts',(-20.950708796806,-12.3358248594298,
114.848615416432)) ;
#167013=CARTESIAN_POINT('Ctrl Pts',(-20.9532774121855,-12.4112821257934,
114.856439006343)) ;
#167014=CARTESIAN_POINT('Ctrl Pts',(-21.0270812862604,-12.4112821160611,
114.832208058027)) ;
#167015=CARTESIAN_POINT('Ctrl Pts',(-21.1008851603352,-12.4112821063287,
114.807977109711)) ;
#167016=CARTESIAN_POINT('Ctrl Pts',(-21.0983165449557,-12.3358248399652,
114.8001535198)) ;
#167017=CARTESIAN_POINT('Ctrl Pts',(-21.0957479295762,-12.2603675736016,
114.79232992989)) ;
#167018=CARTESIAN_POINT('Ctrl Pts',(-21.0219440555014,-12.2603675833339,
114.816560878206)) ;
#167019=CARTESIAN_POINT('Ctrl Pts',(-20.9481401814265,-12.2603675930662,
114.840791826522)) ;
#167020=CARTESIAN_POINT('Ctrl Pts',(-20.950708796806,-12.3358248594298,
114.848615416432)) ;
#167021=CARTESIAN_POINT('Ctrl Pts',(-21.0521870092213,-12.3448661715,115.122173404757)) ;
#167022=CARTESIAN_POINT('Ctrl Pts',(-21.0484096856945,-12.4198057290159,
115.110668288568)) ;
#167023=CARTESIAN_POINT('Ctrl Pts',(-21.1222135578069,-12.41980574501,115.086437334275)) ;
#167024=CARTESIAN_POINT('Ctrl Pts',(-21.1960174299193,-12.4198057610042,
115.062206379981)) ;
#167025=CARTESIAN_POINT('Ctrl Pts',(-21.1997947534461,-12.3448662034884,
115.07371149617)) ;
#167026=CARTESIAN_POINT('Ctrl Pts',(-21.2035720769729,-12.2699266459725,
115.085216612359)) ;
#167027=CARTESIAN_POINT('Ctrl Pts',(-21.1297682048605,-12.2699266299783,
115.109447566652)) ;
#167028=CARTESIAN_POINT('Ctrl Pts',(-21.055964332748,-12.2699266139842,
115.133678520945)) ;
#167029=CARTESIAN_POINT('Ctrl Pts',(-21.0521870092213,-12.3448661715,115.122173404757)) ;
#167030=CARTESIAN_POINT('Ctrl Pts',(-21.1496243276175,-12.4312374679016,
115.383425842735)) ;
#167031=CARTESIAN_POINT('Ctrl Pts',(-21.1397735006215,-12.5002598101882,
115.353421814809)) ;
#167032=CARTESIAN_POINT('Ctrl Pts',(-21.213577368531,-12.5002598472916,
115.329190847715)) ;
#167033=CARTESIAN_POINT('Ctrl Pts',(-21.2873812364404,-12.5002598843951,
115.30495988062)) ;
#167034=CARTESIAN_POINT('Ctrl Pts',(-21.2972320634364,-12.4312375421085,
115.334963908546)) ;
#167035=CARTESIAN_POINT('Ctrl Pts',(-21.3070828904324,-12.3622151998219,
115.364967936471)) ;
#167036=CARTESIAN_POINT('Ctrl Pts',(-21.2332790225229,-12.3622151627184,
115.389198903566)) ;
#167037=CARTESIAN_POINT('Ctrl Pts',(-21.1594751546135,-12.362215125615,
115.413429870661)) ;
#167038=CARTESIAN_POINT('Ctrl Pts',(-21.1496243276175,-12.4312374679016,
115.383425842735)) ;
#167039=CARTESIAN_POINT('Ctrl Pts',(-21.2363589987988,-12.5874506151636,
115.612268295527)) ;
#167040=CARTESIAN_POINT('Ctrl Pts',(-21.2211688298052,-12.6456701044934,
115.566001493264)) ;
#167041=CARTESIAN_POINT('Ctrl Pts',(-21.2949726923912,-12.6456701572597,
115.541770509954)) ;
#167042=CARTESIAN_POINT('Ctrl Pts',(-21.3687765549771,-12.6456702100259,
115.517539526645)) ;
#167043=CARTESIAN_POINT('Ctrl Pts',(-21.3839667239706,-12.5874507206961,
115.563806328909)) ;
#167044=CARTESIAN_POINT('Ctrl Pts',(-21.3991568929642,-12.5292312313663,
115.610073131172)) ;
#167045=CARTESIAN_POINT('Ctrl Pts',(-21.3253530303783,-12.5292311786001,
115.634304114482)) ;
#167046=CARTESIAN_POINT('Ctrl Pts',(-21.2515491677923,-12.5292311258338,
115.658535097791)) ;
#167047=CARTESIAN_POINT('Ctrl Pts',(-21.2363589987988,-12.5874506151636,
115.612268295527)) ;
#167048=CARTESIAN_POINT('Ctrl Pts',(-21.3077549923188,-12.8034012905554,
115.794275144926)) ;
#167049=CARTESIAN_POINT('Ctrl Pts',(-21.2882906825649,-12.8466312900345,
115.734989999395)) ;
#167050=CARTESIAN_POINT('Ctrl Pts',(-21.3620945387581,-12.8466313512928,
115.710758996614)) ;
#167051=CARTESIAN_POINT('Ctrl Pts',(-21.4358983949512,-12.8466314125512,
115.686527993833)) ;
#167052=CARTESIAN_POINT('Ctrl Pts',(-21.455362704705,-12.8034014130721,
115.745813139364)) ;
#167053=CARTESIAN_POINT('Ctrl Pts',(-21.4748270144589,-12.760171413593,
115.805098284895)) ;
#167054=CARTESIAN_POINT('Ctrl Pts',(-21.4010231582657,-12.7601713523347,
115.829329287676)) ;
#167055=CARTESIAN_POINT('Ctrl Pts',(-21.3272193020726,-12.7601712910763,
115.853560290457)) ;
#167056=CARTESIAN_POINT('Ctrl Pts',(-21.3077549923188,-12.8034012905554,
115.794275144926)) ;
#167057=CARTESIAN_POINT('Ctrl Pts',(-21.3591929501021,-13.0643708673509,
115.91537665745)) ;
#167058=CARTESIAN_POINT('Ctrl Pts',(-21.336843717119,-13.0894456413712,
115.847304501069)) ;
#167059=CARTESIAN_POINT('Ctrl Pts',(-21.4106475668522,-13.0894457028003,
115.823073478613)) ;
#167060=CARTESIAN_POINT('Ctrl Pts',(-21.4844514165855,-13.0894457642295,
115.798842456156)) ;
#167061=CARTESIAN_POINT('Ctrl Pts',(-21.5068006495686,-13.0643709902092,
115.866914612537)) ;
#167062=CARTESIAN_POINT('Ctrl Pts',(-21.5291498825516,-13.0392962161889,
115.934986768918)) ;
#167063=CARTESIAN_POINT('Ctrl Pts',(-21.4553460328184,-13.0392961547597,
115.959217791375)) ;
#167064=CARTESIAN_POINT('Ctrl Pts',(-21.3815421830851,-13.0392960933306,
115.983448813831)) ;
#167065=CARTESIAN_POINT('Ctrl Pts',(-21.3591929501021,-13.0643708673509,
115.91537665745)) ;
#167066=CARTESIAN_POINT('Ctrl Pts',(-21.3874706338776,-13.3499213722247,
115.966045844109)) ;
#167067=CARTESIAN_POINT('Ctrl Pts',(-21.3638469150851,-13.355096833582,
115.894091809427)) ;
#167068=CARTESIAN_POINT('Ctrl Pts',(-21.4376507593288,-13.3550968897529,
115.869860770251)) ;
#167069=CARTESIAN_POINT('Ctrl Pts',(-21.5114546035725,-13.3550969459238,
115.845629731074)) ;
#167070=CARTESIAN_POINT('Ctrl Pts',(-21.5350783223649,-13.3499214845666,
115.917583765755)) ;
#167071=CARTESIAN_POINT('Ctrl Pts',(-21.5587020411574,-13.3447460232093,
115.989537800437)) ;
#167072=CARTESIAN_POINT('Ctrl Pts',(-21.4848981969137,-13.3447459670383,
116.013768839614)) ;
#167073=CARTESIAN_POINT('Ctrl Pts',(-21.41109435267,-13.3447459108674,116.037999878791)) ;
#167074=CARTESIAN_POINT('Ctrl Pts',(-21.3874706338776,-13.3499213722247,
115.966045844109)) ;
#167075=CARTESIAN_POINT('Ctrl Pts',(-21.391441344453,-13.6410985525755,
115.942581213302)) ;
#167076=CARTESIAN_POINT('Ctrl Pts',(-21.3682402719706,-13.6259514029626,
115.8719144909)) ;
#167077=CARTESIAN_POINT('Ctrl Pts',(-21.4420441121637,-13.625951448446,
115.847683439386)) ;
#167078=CARTESIAN_POINT('Ctrl Pts',(-21.5158479523567,-13.6259514939294,
115.823452387871)) ;
#167079=CARTESIAN_POINT('Ctrl Pts',(-21.5390490248392,-13.6410986435423,
115.894119110273)) ;
#167080=CARTESIAN_POINT('Ctrl Pts',(-21.5622500973216,-13.6562457931553,
115.964785832674)) ;
#167081=CARTESIAN_POINT('Ctrl Pts',(-21.4884462571285,-13.6562457476719,
115.989016884188)) ;
#167082=CARTESIAN_POINT('Ctrl Pts',(-21.4146424169355,-13.6562457021885,
116.013247935703)) ;
#167083=CARTESIAN_POINT('Ctrl Pts',(-21.391441344453,-13.6410985525755,
115.942581213302)) ;
#167084=CARTESIAN_POINT('Ctrl Pts',(-21.3717120179043,-13.9144130152127,
115.847175451564)) ;
#167085=CARTESIAN_POINT('Ctrl Pts',(-21.3505841798155,-13.8801596021724,
115.782823466471)) ;
#167086=CARTESIAN_POINT('Ctrl Pts',(-21.4243880174265,-13.8801596369213,
115.758592407092)) ;
#167087=CARTESIAN_POINT('Ctrl Pts',(-21.4981918550375,-13.8801596716703,
115.734361347713)) ;
#167088=CARTESIAN_POINT('Ctrl Pts',(-21.5193196931263,-13.9144130847105,
115.798713332805)) ;
#167089=CARTESIAN_POINT('Ctrl Pts',(-21.5404475312151,-13.9486664977508,
115.863065317898)) ;
#167090=CARTESIAN_POINT('Ctrl Pts',(-21.4666436936041,-13.9486664630018,
115.887296377277)) ;
#167091=CARTESIAN_POINT('Ctrl Pts',(-21.3928398559931,-13.9486664282529,
115.911527436656)) ;
#167092=CARTESIAN_POINT('Ctrl Pts',(-21.3717120179043,-13.9144130152127,
115.847175451564)) ;
#167093=CARTESIAN_POINT('Ctrl Pts',(-21.3303616828838,-14.1534993419982,
115.685759559863)) ;
#167094=CARTESIAN_POINT('Ctrl Pts',(-21.3128229753048,-14.1025003039047,
115.632339487033)) ;
#167095=CARTESIAN_POINT('Ctrl Pts',(-21.3866268120323,-14.1025003260636,
115.608108424963)) ;
#167096=CARTESIAN_POINT('Ctrl Pts',(-21.4604306487598,-14.1025003482225,
115.583877362893)) ;
#167097=CARTESIAN_POINT('Ctrl Pts',(-21.4779693563387,-14.153499386316,
115.637297435723)) ;
#167098=CARTESIAN_POINT('Ctrl Pts',(-21.4955080639176,-14.2044984244094,
115.690717508553)) ;
#167099=CARTESIAN_POINT('Ctrl Pts',(-21.4217042271901,-14.2044984022505,
115.714948570623)) ;
#167100=CARTESIAN_POINT('Ctrl Pts',(-21.3479003904626,-14.2044983800916,
115.739179632693)) ;
#167101=CARTESIAN_POINT('Ctrl Pts',(-21.3303616828838,-14.1534993419982,
115.685759559863)) ;
#167102=CARTESIAN_POINT('Ctrl Pts',(-21.2710083107908,-14.3398532357648,
115.469490040302)) ;
#167103=CARTESIAN_POINT('Ctrl Pts',(-21.2583217051769,-14.2757649069183,
115.430848687012)) ;
#167104=CARTESIAN_POINT('Ctrl Pts',(-21.3321255425352,-14.275764918267,
115.406617626863)) ;
#167105=CARTESIAN_POINT('Ctrl Pts',(-21.4059293798935,-14.2757649296157,
115.382386566715)) ;
#167106=CARTESIAN_POINT('Ctrl Pts',(-21.4186159855074,-14.3398532584622,
115.421027920004)) ;
#167107=CARTESIAN_POINT('Ctrl Pts',(-21.4313025911213,-14.4039415873087,
115.459669273294)) ;
#167108=CARTESIAN_POINT('Ctrl Pts',(-21.357498753763,-14.4039415759601,
115.483900333442)) ;
#167109=CARTESIAN_POINT('Ctrl Pts',(-21.2836949164047,-14.4039415646114,
115.508131393591)) ;
#167110=CARTESIAN_POINT('Ctrl Pts',(-21.2710083107908,-14.3398532357648,
115.469490040302)) ;
#167111=CARTESIAN_POINT('Ctrl Pts',(-21.1988659886176,-14.4601239905911,
115.214323564159)) ;
#167112=CARTESIAN_POINT('Ctrl Pts',(-21.1919307384879,-14.3875409587586,
115.193199911556)) ;
#167113=CARTESIAN_POINT('Ctrl Pts',(-21.2657345773112,-14.3875409624437,
115.168968855869)) ;
#167114=CARTESIAN_POINT('Ctrl Pts',(-21.3395384161345,-14.3875409661288,
115.144737800182)) ;
#167115=CARTESIAN_POINT('Ctrl Pts',(-21.3464736662642,-14.4601239979614,
115.165861452786)) ;
#167116=CARTESIAN_POINT('Ctrl Pts',(-21.3534089163939,-14.532707029794,
115.18698510539)) ;
#167117=CARTESIAN_POINT('Ctrl Pts',(-21.2796050775706,-14.5327070261088,
115.211216161076)) ;
#167118=CARTESIAN_POINT('Ctrl Pts',(-21.2058012387473,-14.5327070224237,
115.235447216763)) ;
#167119=CARTESIAN_POINT('Ctrl Pts',(-21.1988659886176,-14.4601239905911,
115.214323564159)) ;
#167120=CARTESIAN_POINT('Ctrl Pts',(-21.1193730346472,-14.5056532387337,
114.936603812244)) ;
#167121=CARTESIAN_POINT('Ctrl Pts',(-21.1187146887639,-14.4297812015044,
114.934598597057)) ;
#167122=CARTESIAN_POINT('Ctrl Pts',(-21.1925185297582,-14.4297812011716,
114.910367547982)) ;
#167123=CARTESIAN_POINT('Ctrl Pts',(-21.2663223707524,-14.4297812008388,
114.886136498908)) ;
#167124=CARTESIAN_POINT('Ctrl Pts',(-21.2669807166357,-14.5056532380682,
114.888141714096)) ;
#167125=CARTESIAN_POINT('Ctrl Pts',(-21.2676390625191,-14.5815252752975,
114.890146929283)) ;
#167126=CARTESIAN_POINT('Ctrl Pts',(-21.1938352215248,-14.5815252756303,
114.914377978358)) ;
#167127=CARTESIAN_POINT('Ctrl Pts',(-21.1200313805306,-14.5815252759631,
114.938609027432)) ;
#167128=CARTESIAN_POINT('Ctrl Pts',(-21.1193730346472,-14.5056532387337,
114.936603812244)) ;
#167129=CARTESIAN_POINT('Ctrl Pts',(-21.0400856818068,-14.4736304498916,
114.659861410865)) ;
#167130=CARTESIAN_POINT('Ctrl Pts',(-21.045691958151,-14.3998809483868,
114.676937224108)) ;
#167131=CARTESIAN_POINT('Ctrl Pts',(-21.1194958005253,-14.3998809471274,
114.652706179238)) ;
#167132=CARTESIAN_POINT('Ctrl Pts',(-21.1932996428997,-14.399880945868,
114.628475134367)) ;
#167133=CARTESIAN_POINT('Ctrl Pts',(-21.1876933665555,-14.4736304473727,
114.611399321123)) ;
#167134=CARTESIAN_POINT('Ctrl Pts',(-21.1820870902113,-14.5473799488775,
114.59432350788)) ;
#167135=CARTESIAN_POINT('Ctrl Pts',(-21.108283247837,-14.5473799501369,
114.61855455275)) ;
#167136=CARTESIAN_POINT('Ctrl Pts',(-21.0344794054626,-14.5473799513963,
114.642785597621)) ;
#167137=CARTESIAN_POINT('Ctrl Pts',(-21.0400856818068,-14.4736304498916,
114.659861410865)) ;
#167138=CARTESIAN_POINT('Ctrl Pts',(-20.9656884076386,-14.3649486844788,
114.397529024825)) ;
#167139=CARTESIAN_POINT('Ctrl Pts',(-20.9772377464687,-14.2986771390851,
114.432706447392)) ;
#167140=CARTESIAN_POINT('Ctrl Pts',(-21.0510415903523,-14.2986771395707,
114.408475407118)) ;
#167141=CARTESIAN_POINT('Ctrl Pts',(-21.1248454342359,-14.2986771400562,
114.384244366844)) ;
#167142=CARTESIAN_POINT('Ctrl Pts',(-21.1132960954058,-14.36494868545,114.349066944277)) ;
#167143=CARTESIAN_POINT('Ctrl Pts',(-21.1017467565757,-14.4312202308437,
114.31388952171)) ;
#167144=CARTESIAN_POINT('Ctrl Pts',(-21.0279429126921,-14.4312202303581,
114.338120561984)) ;
#167145=CARTESIAN_POINT('Ctrl Pts',(-20.9541390688086,-14.4312202298725,
114.362351602257)) ;
#167146=CARTESIAN_POINT('Ctrl Pts',(-20.9656884076386,-14.3649486844788,
114.397529024825)) ;
#167147=CARTESIAN_POINT('Ctrl Pts',(-20.9040908794189,-14.1895250687342,
114.174588389894)) ;
#167148=CARTESIAN_POINT('Ctrl Pts',(-20.9206896003898,-14.1354046364552,
114.225145415719)) ;
#167149=CARTESIAN_POINT('Ctrl Pts',(-20.9944934444827,-14.1354046385753,
114.200914376082)) ;
#167150=CARTESIAN_POINT('Ctrl Pts',(-21.0682972885756,-14.1354046406955,
114.176683336446)) ;
#167151=CARTESIAN_POINT('Ctrl Pts',(-21.0516985676048,-14.1895250729745,
114.126126310621)) ;
#167152=CARTESIAN_POINT('Ctrl Pts',(-21.0350998466339,-14.2436455052536,
114.075569284796)) ;
#167153=CARTESIAN_POINT('Ctrl Pts',(-20.9612960025409,-14.2436455031334,
114.099800324432)) ;
#167154=CARTESIAN_POINT('Ctrl Pts',(-20.887492158448,-14.2436455010133,
114.124031364069)) ;
#167155=CARTESIAN_POINT('Ctrl Pts',(-20.9040908794189,-14.1895250687342,
114.174588389894)) ;
#167156=CARTESIAN_POINT('Ctrl Pts',(-20.8593435984038,-13.9587919846541,
114.002862848148)) ;
#167157=CARTESIAN_POINT('Ctrl Pts',(-20.8798248430018,-13.9207033555361,
114.065245414496)) ;
#167158=CARTESIAN_POINT('Ctrl Pts',(-20.9536286868818,-13.9207033583064,
114.041014374211)) ;
#167159=CARTESIAN_POINT('Ctrl Pts',(-21.0274325307618,-13.9207033610767,
114.016783333927)) ;
#167160=CARTESIAN_POINT('Ctrl Pts',(-21.0069512861638,-13.9587919901947,
113.954400767579)) ;
#167161=CARTESIAN_POINT('Ctrl Pts',(-20.9864700415659,-13.9968806193127,
113.892018201231)) ;
#167162=CARTESIAN_POINT('Ctrl Pts',(-20.9126661976859,-13.9968806165424,
113.916249241516)) ;
#167163=CARTESIAN_POINT('Ctrl Pts',(-20.8388623538059,-13.9968806137721,
113.940480281801)) ;
#167164=CARTESIAN_POINT('Ctrl Pts',(-20.8593435984038,-13.9587919846541,
114.002862848148)) ;
#167165=CARTESIAN_POINT('Ctrl Pts',(-20.8356369939423,-13.6889251841896,
113.895181640807)) ;
#167166=CARTESIAN_POINT('Ctrl Pts',(-20.858537937481,-13.6696247434328,
113.964934219753)) ;
#167167=CARTESIAN_POINT('Ctrl Pts',(-20.9323417808698,-13.6696247444935,
113.940703177972)) ;
#167168=CARTESIAN_POINT('Ctrl Pts',(-21.0061456242587,-13.6696247455542,
113.916472136191)) ;
#167169=CARTESIAN_POINT('Ctrl Pts',(-20.9832446807201,-13.688925186311,
113.846719557246)) ;
#167170=CARTESIAN_POINT('Ctrl Pts',(-20.9603437371814,-13.7082256270677,
113.7769669783)) ;
#167171=CARTESIAN_POINT('Ctrl Pts',(-20.8865398937926,-13.708225626007,
113.801198020081)) ;
#167172=CARTESIAN_POINT('Ctrl Pts',(-20.8127360504037,-13.7082256249463,
113.825429061862)) ;
#167173=CARTESIAN_POINT('Ctrl Pts',(-20.8356369939423,-13.6889251841896,
113.895181640807)) ;
#167174=CARTESIAN_POINT('Ctrl Pts',(-20.8355656879003,-13.3992086458092,
113.859432886615)) ;
#167175=CARTESIAN_POINT('Ctrl Pts',(-20.8592405174172,-13.4001099249718,
113.931542597469)) ;
#167176=CARTESIAN_POINT('Ctrl Pts',(-20.9330443607297,-13.4001099216027,
113.907311555456)) ;
#167177=CARTESIAN_POINT('Ctrl Pts',(-21.0068482040421,-13.4001099182335,
113.883080513442)) ;
#167178=CARTESIAN_POINT('Ctrl Pts',(-20.9831733745252,-13.3992086390708,
113.810970802588)) ;
#167179=CARTESIAN_POINT('Ctrl Pts',(-20.9594985450083,-13.3983073599082,
113.738861091734)) ;
#167180=CARTESIAN_POINT('Ctrl Pts',(-20.8856947016959,-13.3983073632774,
113.763092133747)) ;
#167181=CARTESIAN_POINT('Ctrl Pts',(-20.8118908583834,-13.3983073666465,
113.787323175761)) ;
#167182=CARTESIAN_POINT('Ctrl Pts',(-20.8355656879003,-13.3992086458092,
113.859432886615)) ;
#167183=CARTESIAN_POINT('Ctrl Pts',(-20.8596153977637,-13.1124266878776,
113.89736040102)) ;
#167184=CARTESIAN_POINT('Ctrl Pts',(-20.8823763686297,-13.13335350732,113.966686645961)) ;
#167185=CARTESIAN_POINT('Ctrl Pts',(-20.9561802125574,-13.1333534995856,
113.942455605822)) ;
#167186=CARTESIAN_POINT('Ctrl Pts',(-21.029984056485,-13.1333534918511,
113.918224565682)) ;
#167187=CARTESIAN_POINT('Ctrl Pts',(-21.007223085619,-13.1124266724087,
113.848898320741)) ;
#167188=CARTESIAN_POINT('Ctrl Pts',(-20.984462114753,-13.0914998529662,
113.7795720758)) ;
#167189=CARTESIAN_POINT('Ctrl Pts',(-20.9106582708253,-13.0914998607007,
113.803803115939)) ;
#167190=CARTESIAN_POINT('Ctrl Pts',(-20.8368544268977,-13.0914998684351,
113.828034156079)) ;
#167191=CARTESIAN_POINT('Ctrl Pts',(-20.8596153977637,-13.1124266878776,
113.89736040102)) ;
#167192=CARTESIAN_POINT('Ctrl Pts',(-20.9073931832141,-12.8450096600115,
114.007218110877)) ;
#167193=CARTESIAN_POINT('Ctrl Pts',(-20.9275894252847,-12.8846394195873,
114.068732605881)) ;
#167194=CARTESIAN_POINT('Ctrl Pts',(-21.0013932711385,-12.8846394056337,
114.044501571608)) ;
#167195=CARTESIAN_POINT('Ctrl Pts',(-21.0751971169922,-12.8846393916802,
114.020270537335)) ;
#167196=CARTESIAN_POINT('Ctrl Pts',(-21.0550008749215,-12.8450096321044,
113.95875604233)) ;
#167197=CARTESIAN_POINT('Ctrl Pts',(-21.0348046328509,-12.8053798725287,
113.897241547326)) ;
#167198=CARTESIAN_POINT('Ctrl Pts',(-20.9610007869972,-12.8053798864822,
113.921472581599)) ;
#167199=CARTESIAN_POINT('Ctrl Pts',(-20.8871969411434,-12.8053799004358,
113.945703615872)) ;
#167200=CARTESIAN_POINT('Ctrl Pts',(-20.9073931832141,-12.8450096600115,
114.007218110877)) ;
#167201=CARTESIAN_POINT('Ctrl Pts',(-20.9754422866959,-12.6209217910559,
114.179130249146)) ;
#167202=CARTESIAN_POINT('Ctrl Pts',(-20.9916479840303,-12.6762550632743,
114.228490188886)) ;
#167203=CARTESIAN_POINT('Ctrl Pts',(-21.0654518325001,-12.6762550473825,
114.204259162581)) ;
#167204=CARTESIAN_POINT('Ctrl Pts',(-21.1392556809698,-12.6762550314906,
114.180028136276)) ;
#167205=CARTESIAN_POINT('Ctrl Pts',(-21.1230499836355,-12.6209217592723,
114.130668196536)) ;
#167206=CARTESIAN_POINT('Ctrl Pts',(-21.1068442863011,-12.5655884870539,
114.081308256797)) ;
#167207=CARTESIAN_POINT('Ctrl Pts',(-21.0330404378314,-12.5655885029457,
114.105539283102)) ;
#167208=CARTESIAN_POINT('Ctrl Pts',(-20.9592365893616,-12.5655885188375,
114.129770309407)) ;
#167209=CARTESIAN_POINT('Ctrl Pts',(-20.9754422866959,-12.6209217910559,
114.179130249146)) ;
#167210=CARTESIAN_POINT('Ctrl Pts',(-21.060116229982,-12.453038777336,114.401581870571)) ;
#167211=CARTESIAN_POINT('Ctrl Pts',(-21.0711669360117,-12.520173907181,
114.435240538705)) ;
#167212=CARTESIAN_POINT('Ctrl Pts',(-21.1449707877985,-12.5201738923226,
114.411009522503)) ;
#167213=CARTESIAN_POINT('Ctrl Pts',(-21.2187746395854,-12.5201738774643,
114.386778506302)) ;
#167214=CARTESIAN_POINT('Ctrl Pts',(-21.2077239335557,-12.4530387476193,
114.353119838167)) ;
#167215=CARTESIAN_POINT('Ctrl Pts',(-21.196673227526,-12.3859036177743,
114.319461170032)) ;
#167216=CARTESIAN_POINT('Ctrl Pts',(-21.1228693757392,-12.3859036326327,
114.343692186234)) ;
#167217=CARTESIAN_POINT('Ctrl Pts',(-21.0490655239523,-12.385903647491,
114.367923202436)) ;
#167218=CARTESIAN_POINT('Ctrl Pts',(-21.060116229982,-12.453038777336,114.401581870571)) ;
#167219=CARTESIAN_POINT('Ctrl Pts',(-21.1561433073425,-12.3543368017594,
114.658578252509)) ;
#167220=CARTESIAN_POINT('Ctrl Pts',(-21.1612396516993,-12.4284604690025,
114.67410089589)) ;
#167221=CARTESIAN_POINT('Ctrl Pts',(-21.23504350709,-12.4284604600379,114.649869890665)) ;
#167222=CARTESIAN_POINT('Ctrl Pts',(-21.3088473624807,-12.4284604510733,
114.62563888544)) ;
#167223=CARTESIAN_POINT('Ctrl Pts',(-21.3037510181239,-12.3543367838302,
114.610116242059)) ;
#167224=CARTESIAN_POINT('Ctrl Pts',(-21.2986546737672,-12.2802131165871,
114.594593598678)) ;
#167225=CARTESIAN_POINT('Ctrl Pts',(-21.2248508183765,-12.2802131255517,
114.618824603903)) ;
#167226=CARTESIAN_POINT('Ctrl Pts',(-21.1510469629858,-12.2802131345163,
114.643055609128)) ;
#167227=CARTESIAN_POINT('Ctrl Pts',(-21.1561433073425,-12.3543368017594,
114.658578252509)) ;
#167228=CARTESIAN_POINT('Ctrl Pts',(-21.2570400946613,-12.3316786589988,
114.930491348528)) ;
#167229=CARTESIAN_POINT('Ctrl Pts',(-21.2558318008147,-12.4074912166658,
114.926811081348)) ;
#167230=CARTESIAN_POINT('Ctrl Pts',(-21.3296356590554,-12.4074912185027,
114.902580084804)) ;
#167231=CARTESIAN_POINT('Ctrl Pts',(-21.403439517296,-12.4074912203397,
114.878349088259)) ;
#167232=CARTESIAN_POINT('Ctrl Pts',(-21.4046478111425,-12.3316786626727,
114.882029355439)) ;
#167233=CARTESIAN_POINT('Ctrl Pts',(-21.4058561049891,-12.2558661050058,
114.885709622619)) ;
#167234=CARTESIAN_POINT('Ctrl Pts',(-21.3320522467485,-12.2558661031688,
114.909940619164)) ;
#167235=CARTESIAN_POINT('Ctrl Pts',(-21.2582483885079,-12.2558661013318,
114.934171615708)) ;
#167236=CARTESIAN_POINT('Ctrl Pts',(-21.2570400946613,-12.3316786589988,
114.930491348528)) ;
#167237=CARTESIAN_POINT('Ctrl Pts',(-21.3572503237435,-12.3873927929882,
115.200059905244)) ;
#167238=CARTESIAN_POINT('Ctrl Pts',(-21.3497814966636,-12.4594256106333,
115.177311064172)) ;
#167239=CARTESIAN_POINT('Ctrl Pts',(-21.4235853573106,-12.4594256285176,
115.153080074957)) ;
#167240=CARTESIAN_POINT('Ctrl Pts',(-21.4973892179576,-12.4594256464019,
115.128849085742)) ;
#167241=CARTESIAN_POINT('Ctrl Pts',(-21.5048580450376,-12.3873928287568,
115.151597926814)) ;
#167242=CARTESIAN_POINT('Ctrl Pts',(-21.5123268721176,-12.3153600111117,
115.174346767886)) ;
#167243=CARTESIAN_POINT('Ctrl Pts',(-21.4385230114705,-12.3153599932274,
115.198577757101)) ;
#167244=CARTESIAN_POINT('Ctrl Pts',(-21.3647191508235,-12.3153599753431,
115.222808746316)) ;
#167245=CARTESIAN_POINT('Ctrl Pts',(-21.3572503237435,-12.3873927929882,
115.200059905244)) ;
#167246=CARTESIAN_POINT('Ctrl Pts',(-21.4488212057437,-12.5162741275779,
115.443632859608)) ;
#167247=CARTESIAN_POINT('Ctrl Pts',(-21.4356795074852,-12.5794124829248,
115.40360536838)) ;
#167248=CARTESIAN_POINT('Ctrl Pts',(-21.5094833678952,-12.5794125189228,
115.379374378443)) ;
#167249=CARTESIAN_POINT('Ctrl Pts',(-21.5832872283053,-12.5794125549208,
115.355143388506)) ;
#167250=CARTESIAN_POINT('Ctrl Pts',(-21.5964289265637,-12.5162741995739,
115.395170879734)) ;
#167251=CARTESIAN_POINT('Ctrl Pts',(-21.6095706248222,-12.453135844227,
115.435198370962)) ;
#167252=CARTESIAN_POINT('Ctrl Pts',(-21.5357667644122,-12.453135808229,
115.459429360899)) ;
#167253=CARTESIAN_POINT('Ctrl Pts',(-21.4619629040021,-12.453135772231,
115.483660350836)) ;
#167254=CARTESIAN_POINT('Ctrl Pts',(-21.4488212057437,-12.5162741275779,
115.443632859608)) ;
#167255=CARTESIAN_POINT('Ctrl Pts',(-21.5273021746152,-12.7104566542012,
115.647127915526)) ;
#167256=CARTESIAN_POINT('Ctrl Pts',(-21.5093975650024,-12.7601293026598,
115.592593364974)) ;
#167257=CARTESIAN_POINT('Ctrl Pts',(-21.5832014235926,-12.7601293584612,
115.568362369495)) ;
#167258=CARTESIAN_POINT('Ctrl Pts',(-21.6570052821828,-12.7601294142626,
115.544131374015)) ;
#167259=CARTESIAN_POINT('Ctrl Pts',(-21.6749098917956,-12.7104567658041,
115.598665924566)) ;
#167260=CARTESIAN_POINT('Ctrl Pts',(-21.6928145014084,-12.6607841173455,
115.653200475117)) ;
#167261=CARTESIAN_POINT('Ctrl Pts',(-21.6190106428182,-12.6607840615441,
115.677431470597)) ;
#167262=CARTESIAN_POINT('Ctrl Pts',(-21.5452067842279,-12.6607840057427,
115.701662466077)) ;
#167263=CARTESIAN_POINT('Ctrl Pts',(-21.5273021746152,-12.7104566542012,
115.647127915526)) ;
#167264=CARTESIAN_POINT('Ctrl Pts',(-21.5869697508136,-12.9544063196606,
115.793490670685)) ;
#167265=CARTESIAN_POINT('Ctrl Pts',(-21.5656053858241,-12.9871189134417,
115.728418263615)) ;
#167266=CARTESIAN_POINT('Ctrl Pts',(-21.6394092401113,-12.9871189862544,
115.704187255029)) ;
#167267=CARTESIAN_POINT('Ctrl Pts',(-21.7132130943986,-12.987119059067,
115.679956246443)) ;
#167268=CARTESIAN_POINT('Ctrl Pts',(-21.734577459388,-12.9544064652859,
115.745028653514)) ;
#167269=CARTESIAN_POINT('Ctrl Pts',(-21.7559418243775,-12.9216938715048,
115.810101060584)) ;
#167270=CARTESIAN_POINT('Ctrl Pts',(-21.6821379700903,-12.9216937986921,
115.83433206917)) ;
#167271=CARTESIAN_POINT('Ctrl Pts',(-21.608334115803,-12.9216937258795,
115.858563077756)) ;
#167272=CARTESIAN_POINT('Ctrl Pts',(-21.5869697508136,-12.9544063196606,
115.793490670685)) ;
#167273=CARTESIAN_POINT('Ctrl Pts',(-21.6248241880919,-13.2316631461472,
115.873367978984)) ;
#167274=CARTESIAN_POINT('Ctrl Pts',(-21.6015188760931,-13.2450660236381,
115.802383760619)) ;
#167275=CARTESIAN_POINT('Ctrl Pts',(-21.6753227243222,-13.2450661094682,
115.778152733581)) ;
#167276=CARTESIAN_POINT('Ctrl Pts',(-21.7491265725514,-13.2450661952983,
115.753921706544)) ;
#167277=CARTESIAN_POINT('Ctrl Pts',(-21.7724318845503,-13.2316633178074,
115.824905924908)) ;
#167278=CARTESIAN_POINT('Ctrl Pts',(-21.7957371965492,-13.2182604403165,
115.895890143273)) ;
#167279=CARTESIAN_POINT('Ctrl Pts',(-21.72193334832,-13.2182603544864,115.920121170311)) ;
#167280=CARTESIAN_POINT('Ctrl Pts',(-21.6481295000908,-13.2182602686563,
115.944352197349)) ;
#167281=CARTESIAN_POINT('Ctrl Pts',(-21.6248241880919,-13.2316631461472,
115.873367978984)) ;
#167282=CARTESIAN_POINT('Ctrl Pts',(-21.6387981022204,-13.5226486146427,
115.880466253006)) ;
#167283=CARTESIAN_POINT('Ctrl Pts',(-21.6152170567332,-13.5157554602217,
115.808642195042)) ;
#167284=CARTESIAN_POINT('Ctrl Pts',(-21.6890208974959,-13.5157555531286,
115.784411145263)) ;
#167285=CARTESIAN_POINT('Ctrl Pts',(-21.7628247382586,-13.5157556460354,
115.760180095483)) ;
#167286=CARTESIAN_POINT('Ctrl Pts',(-21.7864057837459,-13.5226488004565,
115.832004153447)) ;
#167287=CARTESIAN_POINT('Ctrl Pts',(-21.8099868292331,-13.5295419548775,
115.903828211411)) ;
#167288=CARTESIAN_POINT('Ctrl Pts',(-21.7361829884704,-13.5295418619706,
115.92805926119)) ;
#167289=CARTESIAN_POINT('Ctrl Pts',(-21.6623791477077,-13.5295417690637,
115.952290310969)) ;
#167290=CARTESIAN_POINT('Ctrl Pts',(-21.6387981022204,-13.5226486146427,
115.880466253006)) ;
#167291=CARTESIAN_POINT('Ctrl Pts',(-21.6284861294477,-13.8069296281822,
115.813488458912)) ;
#167292=CARTESIAN_POINT('Ctrl Pts',(-21.6063264693954,-13.7801790343967,
115.745993711753)) ;
#167293=CARTESIAN_POINT('Ctrl Pts',(-21.6801303018853,-13.7801791269532,
115.721762636776)) ;
#167294=CARTESIAN_POINT('Ctrl Pts',(-21.7539341343752,-13.7801792195097,
115.697531561799)) ;
#167295=CARTESIAN_POINT('Ctrl Pts',(-21.7760937944275,-13.8069298132952,
115.765026308958)) ;
#167296=CARTESIAN_POINT('Ctrl Pts',(-21.7982534544798,-13.8336804070807,
115.832521056117)) ;
#167297=CARTESIAN_POINT('Ctrl Pts',(-21.7244496219899,-13.8336803145242,
115.856752131094)) ;
#167298=CARTESIAN_POINT('Ctrl Pts',(-21.6506457895,-13.8336802219677,115.880983206071)) ;
#167299=CARTESIAN_POINT('Ctrl Pts',(-21.6284861294477,-13.8069296281822,
115.813488458912)) ;
#167300=CARTESIAN_POINT('Ctrl Pts',(-21.5954516704821,-14.0625497260425,
115.677400696328)) ;
#167301=CARTESIAN_POINT('Ctrl Pts',(-21.5762998168345,-14.0179135569207,
115.619067242248)) ;
#167302=CARTESIAN_POINT('Ctrl Pts',(-21.6501036412778,-14.017913640046,
115.594836142763)) ;
#167303=CARTESIAN_POINT('Ctrl Pts',(-21.7239074657211,-14.0179137231712,
115.570605043277)) ;
#167304=CARTESIAN_POINT('Ctrl Pts',(-21.7430593193686,-14.062549892293,
115.628938497357)) ;
#167305=CARTESIAN_POINT('Ctrl Pts',(-21.7622111730162,-14.1071860614148,
115.687271951437)) ;
#167306=CARTESIAN_POINT('Ctrl Pts',(-21.6884073485729,-14.1071859782896,
115.711503050923)) ;
#167307=CARTESIAN_POINT('Ctrl Pts',(-21.6146035241296,-14.1071858951643,
115.735734150408)) ;
#167308=CARTESIAN_POINT('Ctrl Pts',(-21.5954516704821,-14.0625497260425,
115.677400696328)) ;
#167309=CARTESIAN_POINT('Ctrl Pts',(-21.5427818566883,-14.2720262448878,
115.481481169144)) ;
#167310=CARTESIAN_POINT('Ctrl Pts',(-21.528013502307,-14.2126996245835,
115.436499146612)) ;
#167311=CARTESIAN_POINT('Ctrl Pts',(-21.6018173198018,-14.2126996903488,
115.412268025962)) ;
#167312=CARTESIAN_POINT('Ctrl Pts',(-21.6756211372967,-14.2126997561141,
115.388036905313)) ;
#167313=CARTESIAN_POINT('Ctrl Pts',(-21.690389491678,-14.2720263764183,
115.433018927845)) ;
#167314=CARTESIAN_POINT('Ctrl Pts',(-21.7051578460592,-14.3313529967226,
115.478000950378)) ;
#167315=CARTESIAN_POINT('Ctrl Pts',(-21.6313540285644,-14.3313529309573,
115.502232071027)) ;
#167316=CARTESIAN_POINT('Ctrl Pts',(-21.5575502110696,-14.331352865192,
115.526463191677)) ;
#167317=CARTESIAN_POINT('Ctrl Pts',(-21.5427818566883,-14.2720262448878,
115.481481169144)) ;
#167318=CARTESIAN_POINT('Ctrl Pts',(-21.4753425478091,-14.4199161330371,
115.240721116631)) ;
#167319=CARTESIAN_POINT('Ctrl Pts',(-21.4659923355475,-14.3501772641186,
115.212241880814)) ;
#167320=CARTESIAN_POINT('Ctrl Pts',(-21.5397961480427,-14.3501773061419,
115.188010744936)) ;
#167321=CARTESIAN_POINT('Ctrl Pts',(-21.613599960538,-14.3501773481651,
115.163779609059)) ;
#167322=CARTESIAN_POINT('Ctrl Pts',(-21.6229501727996,-14.4199162170836,
115.192258844876)) ;
#167323=CARTESIAN_POINT('Ctrl Pts',(-21.6323003850611,-14.489655086002,
115.220738080693)) ;
#167324=CARTESIAN_POINT('Ctrl Pts',(-21.5584965725659,-14.4896550439788,
115.244969216571)) ;
#167325=CARTESIAN_POINT('Ctrl Pts',(-21.4846927600706,-14.4896550019555,
115.269200352448)) ;
#167326=CARTESIAN_POINT('Ctrl Pts',(-21.4753425478091,-14.4199161330371,
115.240721116631)) ;
#167327=CARTESIAN_POINT('Ctrl Pts',(-21.397953128425,-14.496610258064,114.969417382177)) ;
#167328=CARTESIAN_POINT('Ctrl Pts',(-21.3947284182574,-14.4214134928077,
114.959595437408)) ;
#167329=CARTESIAN_POINT('Ctrl Pts',(-21.4685322281319,-14.4214135069691,
114.935364293548)) ;
#167330=CARTESIAN_POINT('Ctrl Pts',(-21.5423360380063,-14.4214135211306,
114.911133149688)) ;
#167331=CARTESIAN_POINT('Ctrl Pts',(-21.5455607481739,-14.496610286387,
114.920955094457)) ;
#167332=CARTESIAN_POINT('Ctrl Pts',(-21.5487854583414,-14.5718070516433,
114.930777039227)) ;
#167333=CARTESIAN_POINT('Ctrl Pts',(-21.474981648467,-14.5718070374819,
114.955008183087)) ;
#167334=CARTESIAN_POINT('Ctrl Pts',(-21.4011778385925,-14.5718070233204,
114.979239326947)) ;
#167335=CARTESIAN_POINT('Ctrl Pts',(-21.397953128425,-14.496610258064,114.969417382177)) ;
#167336=CARTESIAN_POINT('Ctrl Pts',(-21.3180584790138,-14.4958941579837,
114.690798167278)) ;
#167337=CARTESIAN_POINT('Ctrl Pts',(-21.3211368828269,-14.4206364931476,
114.700174490684)) ;
#167338=CARTESIAN_POINT('Ctrl Pts',(-21.3949406928266,-14.4206364783751,
114.675943347206)) ;
#167339=CARTESIAN_POINT('Ctrl Pts',(-21.4687445028263,-14.4206364636026,
114.651712203727)) ;
#167340=CARTESIAN_POINT('Ctrl Pts',(-21.4656660990133,-14.4958941284387,
114.642335880322)) ;
#167341=CARTESIAN_POINT('Ctrl Pts',(-21.4625876952002,-14.5711517932748,
114.632959556916)) ;
#167342=CARTESIAN_POINT('Ctrl Pts',(-21.3887838852004,-14.5711518080473,
114.657190700394)) ;
#167343=CARTESIAN_POINT('Ctrl Pts',(-21.3149800752007,-14.5711518228198,
114.681421843873)) ;
#167344=CARTESIAN_POINT('Ctrl Pts',(-21.3180584790138,-14.4958941579837,
114.690798167278)) ;
#167345=CARTESIAN_POINT('Ctrl Pts',(-21.2408257912765,-14.4180076226564,
114.419996127992)) ;
#167346=CARTESIAN_POINT('Ctrl Pts',(-21.2500367265787,-14.3480754910907,
114.448051152803)) ;
#167347=CARTESIAN_POINT('Ctrl Pts',(-21.3238405394614,-14.3480754488814,
114.423820018105)) ;
#167348=CARTESIAN_POINT('Ctrl Pts',(-21.3976443523441,-14.3480754066721,
114.399588883408)) ;
#167349=CARTESIAN_POINT('Ctrl Pts',(-21.388433417042,-14.4180075382377,
114.371533858597)) ;
#167350=CARTESIAN_POINT('Ctrl Pts',(-21.3792224817398,-14.4879396698034,
114.343478833786)) ;
#167351=CARTESIAN_POINT('Ctrl Pts',(-21.3054186688571,-14.4879397120127,
114.367709968483)) ;
#167352=CARTESIAN_POINT('Ctrl Pts',(-21.2316148559744,-14.4879397542221,
114.391941103181)) ;
#167353=CARTESIAN_POINT('Ctrl Pts',(-21.2408257912765,-14.4180076226564,
114.419996127992)) ;
#167354=CARTESIAN_POINT('Ctrl Pts',(-21.1734230549706,-14.2684543242656,
114.179245557719)) ;
#167355=CARTESIAN_POINT('Ctrl Pts',(-21.1880871641883,-14.2088592298977,
114.22391007036)) ;
#167356=CARTESIAN_POINT('Ctrl Pts',(-21.2618909823228,-14.2088591648377,
114.199678951658)) ;
#167357=CARTESIAN_POINT('Ctrl Pts',(-21.3356948004572,-14.2088590997777,
114.175447832957)) ;
#167358=CARTESIAN_POINT('Ctrl Pts',(-21.3210306912395,-14.2684541941456,
114.130783320317)) ;
#167359=CARTESIAN_POINT('Ctrl Pts',(-21.3063665820217,-14.3280492885136,
114.086118807677)) ;
#167360=CARTESIAN_POINT('Ctrl Pts',(-21.2325627638873,-14.3280493535736,
114.110349926378)) ;
#167361=CARTESIAN_POINT('Ctrl Pts',(-21.1587589457529,-14.3280494186336,
114.134581045079)) ;
#167362=CARTESIAN_POINT('Ctrl Pts',(-21.1734230549706,-14.2684543242656,
114.179245557719)) ;
#167363=CARTESIAN_POINT('Ctrl Pts',(-21.1211403104816,-14.0580103363769,
113.984528831462)) ;
#167364=CARTESIAN_POINT('Ctrl Pts',(-21.1402105735545,-14.0130186488343,
114.042613777743)) ;
#167365=CARTESIAN_POINT('Ctrl Pts',(-21.214014398683,-14.0130185675702,
114.018382680344)) ;
#167366=CARTESIAN_POINT('Ctrl Pts',(-21.2878182238116,-14.013018486306,
113.994151582946)) ;
#167367=CARTESIAN_POINT('Ctrl Pts',(-21.2687479607386,-14.0580101738486,
113.936066636665)) ;
#167368=CARTESIAN_POINT('Ctrl Pts',(-21.2496776976657,-14.1030018613912,
113.877981690384)) ;
#167369=CARTESIAN_POINT('Ctrl Pts',(-21.1758738725372,-14.1030019426553,
113.902212787783)) ;
#167370=CARTESIAN_POINT('Ctrl Pts',(-21.1020700474087,-14.1030020239195,
113.926443885181)) ;
#167371=CARTESIAN_POINT('Ctrl Pts',(-21.1211403104816,-14.0580103363769,
113.984528831462)) ;
#167372=CARTESIAN_POINT('Ctrl Pts',(-21.0885284661435,-13.8017355758307,
113.849734796424)) ;
#167373=CARTESIAN_POINT('Ctrl Pts',(-21.1106380366097,-13.7745688567898,
113.917076982543)) ;
#167374=CARTESIAN_POINT('Ctrl Pts',(-21.1844418696645,-13.7745687672832,
113.892845909287)) ;
#167375=CARTESIAN_POINT('Ctrl Pts',(-21.2582457027194,-13.7745686777767,
113.868614836031)) ;
#167376=CARTESIAN_POINT('Ctrl Pts',(-21.2361361322532,-13.8017353968177,
113.801272649912)) ;
#167377=CARTESIAN_POINT('Ctrl Pts',(-21.2140265617871,-13.8289021158586,
113.733930463793)) ;
#167378=CARTESIAN_POINT('Ctrl Pts',(-21.1402227287323,-13.8289022053652,
113.75816153705)) ;
#167379=CARTESIAN_POINT('Ctrl Pts',(-21.0664188956774,-13.8289022948717,
113.782392610306)) ;
#167380=CARTESIAN_POINT('Ctrl Pts',(-21.0885284661435,-13.8017355758307,
113.849734796424)) ;
#167381=CARTESIAN_POINT('Ctrl Pts',(-21.0786678337561,-13.5177911289146,
113.784214759022)) ;
#167382=CARTESIAN_POINT('Ctrl Pts',(-21.102233421415,-13.5104079472705,
113.85599173847)) ;
#167383=CARTESIAN_POINT('Ctrl Pts',(-21.1760372624413,-13.5104078579673,
113.831760689493)) ;
#167384=CARTESIAN_POINT('Ctrl Pts',(-21.2498411034676,-13.5104077686641,
113.807529640517)) ;
#167385=CARTESIAN_POINT('Ctrl Pts',(-21.2262755158087,-13.5177909503083,
113.735752661069)) ;
#167386=CARTESIAN_POINT('Ctrl Pts',(-21.2027099281497,-13.5251741319524,
113.663975681621)) ;
#167387=CARTESIAN_POINT('Ctrl Pts',(-21.1289060871234,-13.5251742212556,
113.688206730597)) ;
#167388=CARTESIAN_POINT('Ctrl Pts',(-21.0551022460972,-13.5251743105588,
113.712437779574)) ;
#167389=CARTESIAN_POINT('Ctrl Pts',(-21.0786678337561,-13.5177911289146,
113.784214759022)) ;
#167390=CARTESIAN_POINT('Ctrl Pts',(-21.0930193660603,-13.2272027816916,
113.79250094057)) ;
#167391=CARTESIAN_POINT('Ctrl Pts',(-21.1163514983344,-13.2400970018567,
113.863566852463)) ;
#167392=CARTESIAN_POINT('Ctrl Pts',(-21.1901553464802,-13.2400969198801,
113.839335825171)) ;
#167393=CARTESIAN_POINT('Ctrl Pts',(-21.2639591946259,-13.2400968379035,
113.815104797879)) ;
#167394=CARTESIAN_POINT('Ctrl Pts',(-21.2406270623518,-13.2272026177384,
113.744038885987)) ;
#167395=CARTESIAN_POINT('Ctrl Pts',(-21.2172949300776,-13.2143083975732,
113.672972974094)) ;
#167396=CARTESIAN_POINT('Ctrl Pts',(-21.1434910819319,-13.2143084795498,
113.697204001386)) ;
#167397=CARTESIAN_POINT('Ctrl Pts',(-21.0696872337862,-13.2143085615265,
113.721435028678)) ;
#167398=CARTESIAN_POINT('Ctrl Pts',(-21.0930193660603,-13.2272027816916,
113.79250094057)) ;
#167399=CARTESIAN_POINT('Ctrl Pts',(-21.1311631750796,-12.9503466746931,
113.873276997434)) ;
#167400=CARTESIAN_POINT('Ctrl Pts',(-21.152599925483,-12.9825901613467,
113.938569881838)) ;
#167401=CARTESIAN_POINT('Ctrl Pts',(-21.2264037793875,-12.9825900924411,
113.914338872086)) ;
#167402=CARTESIAN_POINT('Ctrl Pts',(-21.3002076332919,-12.9825900235354,
113.890107862335)) ;
#167403=CARTESIAN_POINT('Ctrl Pts',(-21.2787708828885,-12.9503465368818,
113.82481497793)) ;
#167404=CARTESIAN_POINT('Ctrl Pts',(-21.257334132485,-12.9181030502282,
113.759522093526)) ;
#167405=CARTESIAN_POINT('Ctrl Pts',(-21.1835302785805,-12.9181031191338,
113.783753103278)) ;
#167406=CARTESIAN_POINT('Ctrl Pts',(-21.1097264246761,-12.9181031880395,
113.80798411303)) ;
#167407=CARTESIAN_POINT('Ctrl Pts',(-21.1311631750796,-12.9503466746931,
113.873276997434)) ;
#167408=CARTESIAN_POINT('Ctrl Pts',(-21.1916208019657,-12.7057179827167,
114.021818954021)) ;
#167409=CARTESIAN_POINT('Ctrl Pts',(-21.2096056903535,-12.7550903667589,
114.076598023505)) ;
#167410=CARTESIAN_POINT('Ctrl Pts',(-21.2834095477442,-12.7550903161595,
114.052367024372)) ;
#167411=CARTESIAN_POINT('Ctrl Pts',(-21.3572134051349,-12.7550902655601,
114.028136025238)) ;
#167412=CARTESIAN_POINT('Ctrl Pts',(-21.3392285167472,-12.7057178815179,
113.973356955754)) ;
#167413=CARTESIAN_POINT('Ctrl Pts',(-21.3212436283594,-12.6563454974757,
113.91857788627)) ;
#167414=CARTESIAN_POINT('Ctrl Pts',(-21.2474397709687,-12.6563455480751,
113.942808885403)) ;
#167415=CARTESIAN_POINT('Ctrl Pts',(-21.173635913578,-12.6563455986745,
113.967039884536)) ;
#167416=CARTESIAN_POINT('Ctrl Pts',(-21.1916208019657,-12.7057179827167,
114.021818954021)) ;
#167417=CARTESIAN_POINT('Ctrl Pts',(-21.2699420517425,-12.5137879422887,
114.22504280419)) ;
#167418=CARTESIAN_POINT('Ctrl Pts',(-21.2832167372828,-12.5766355535095,
114.265475355653)) ;
#167419=CARTESIAN_POINT('Ctrl Pts',(-21.3570205964976,-12.5766355204259,
114.241244362076)) ;
#167420=CARTESIAN_POINT('Ctrl Pts',(-21.4308244557124,-12.5766354873422,
114.217013368499)) ;
#167421=CARTESIAN_POINT('Ctrl Pts',(-21.417549770172,-12.5137878761215,
114.176580817036)) ;
#167422=CARTESIAN_POINT('Ctrl Pts',(-21.4042750846316,-12.4509402649008,
114.136148265573)) ;
#167423=CARTESIAN_POINT('Ctrl Pts',(-21.3304712254169,-12.4509402979844,
114.16037925915)) ;
#167424=CARTESIAN_POINT('Ctrl Pts',(-21.2566673662021,-12.450940331068,
114.184610252727)) ;
#167425=CARTESIAN_POINT('Ctrl Pts',(-21.2699420517425,-12.5137879422887,
114.22504280419)) ;
#167426=CARTESIAN_POINT('Ctrl Pts',(-21.3620410862087,-12.3855428728414,
114.470083431169)) ;
#167427=CARTESIAN_POINT('Ctrl Pts',(-21.3696396280776,-12.4574400165938,
114.493227364683)) ;
#167428=CARTESIAN_POINT('Ctrl Pts',(-21.4434434869082,-12.4574400010847,
114.468996369935)) ;
#167429=CARTESIAN_POINT('Ctrl Pts',(-21.5172473457389,-12.4574399855756,
114.444765375188)) ;
#167430=CARTESIAN_POINT('Ctrl Pts',(-21.5096488038699,-12.3855428418231,
114.421621441674)) ;
#167431=CARTESIAN_POINT('Ctrl Pts',(-21.502050262001,-12.3136456980707,
114.39847750816)) ;
#167432=CARTESIAN_POINT('Ctrl Pts',(-21.4282464031703,-12.3136457135799,
114.422708502908)) ;
#167433=CARTESIAN_POINT('Ctrl Pts',(-21.3544425443397,-12.313645729089,
114.446939497655)) ;
#167434=CARTESIAN_POINT('Ctrl Pts',(-21.3620410862087,-12.3855428728414,
114.470083431169)) ;
#167435=CARTESIAN_POINT('Ctrl Pts',(-21.4620234613405,-12.3315373856839,
114.739072799255)) ;
#167436=CARTESIAN_POINT('Ctrl Pts',(-21.4633880246011,-12.4073146251765,
114.743229039594)) ;
#167437=CARTESIAN_POINT('Ctrl Pts',(-21.5371918812133,-12.4073146237206,
114.718998038089)) ;
#167438=CARTESIAN_POINT('Ctrl Pts',(-21.6109957378256,-12.4073146222647,
114.694767036585)) ;
#167439=CARTESIAN_POINT('Ctrl Pts',(-21.609631174565,-12.331537382772,114.690610796247)) ;
#167440=CARTESIAN_POINT('Ctrl Pts',(-21.6082666113044,-12.2557601432794,
114.686454555908)) ;
#167441=CARTESIAN_POINT('Ctrl Pts',(-21.5344627546922,-12.2557601447353,
114.710685557413)) ;
#167442=CARTESIAN_POINT('Ctrl Pts',(-21.4606588980799,-12.2557601461912,
114.734916558917)) ;
#167443=CARTESIAN_POINT('Ctrl Pts',(-21.4620234613405,-12.3315373856839,
114.739072799255)) ;
#167444=CARTESIAN_POINT('Ctrl Pts',(-21.5628393644424,-12.3551820249381,
115.010760483268)) ;
#167445=CARTESIAN_POINT('Ctrl Pts',(-21.557898953099,-12.4294230563163,
114.995712788115)) ;
#167446=CARTESIAN_POINT('Ctrl Pts',(-21.6317028069505,-12.4294230645316,
114.971481778201)) ;
#167447=CARTESIAN_POINT('Ctrl Pts',(-21.705506660802,-12.4294230727469,
114.947250768288)) ;
#167448=CARTESIAN_POINT('Ctrl Pts',(-21.7104470721454,-12.3551820413687,
114.962298463441)) ;
#167449=CARTESIAN_POINT('Ctrl Pts',(-21.7153874834888,-12.2809410099905,
114.977346158594)) ;
#167450=CARTESIAN_POINT('Ctrl Pts',(-21.6415836296373,-12.2809410017752,
115.001577168508)) ;
#167451=CARTESIAN_POINT('Ctrl Pts',(-21.5677797757859,-12.2809409935599,
115.025808178421)) ;
#167452=CARTESIAN_POINT('Ctrl Pts',(-21.5628393644424,-12.3551820249381,
115.010760483268)) ;
#167453=CARTESIAN_POINT('Ctrl Pts',(-21.659189028177,-12.4558831035982,
115.268554494791)) ;
#167454=CARTESIAN_POINT('Ctrl Pts',(-21.6482517146779,-12.5232058909048,
115.23524120307)) ;
#167455=CARTESIAN_POINT('Ctrl Pts',(-21.7220555646767,-12.52320590289,115.211010181422)) ;
#167456=CARTESIAN_POINT('Ctrl Pts',(-21.7958594146756,-12.5232059148753,
115.186779159775)) ;
#167457=CARTESIAN_POINT('Ctrl Pts',(-21.8067967281747,-12.4558831275687,
115.220092451495)) ;
#167458=CARTESIAN_POINT('Ctrl Pts',(-21.8177340416738,-12.3885603402622,
115.253405743216)) ;
#167459=CARTESIAN_POINT('Ctrl Pts',(-21.7439301916749,-12.3885603282769,
115.277636764863)) ;
#167460=CARTESIAN_POINT('Ctrl Pts',(-21.6701263416761,-12.3885603162917,
115.301867786511)) ;
#167461=CARTESIAN_POINT('Ctrl Pts',(-21.659189028177,-12.4558831035982,
115.268554494791)) ;
#167462=CARTESIAN_POINT('Ctrl Pts',(-21.743187461739,-12.6240117159259,
115.489136281723)) ;
#167463=CARTESIAN_POINT('Ctrl Pts',(-21.7270983492204,-12.6796964809936,
115.440131441313)) ;
#167464=CARTESIAN_POINT('Ctrl Pts',(-21.8009021966587,-12.6796964939069,
115.415900411867)) ;
#167465=CARTESIAN_POINT('Ctrl Pts',(-21.8747060440971,-12.6796965068202,
115.39166938242)) ;
#167466=CARTESIAN_POINT('Ctrl Pts',(-21.8907951566158,-12.6240117417526,
115.44067422283)) ;
#167467=CARTESIAN_POINT('Ctrl Pts',(-21.9068842691344,-12.568326976685,
115.489679063239)) ;
#167468=CARTESIAN_POINT('Ctrl Pts',(-21.833080421696,-12.5683269637716,
115.513910092686)) ;
#167469=CARTESIAN_POINT('Ctrl Pts',(-21.7592765742577,-12.5683269508583,
115.538141122132)) ;
#167470=CARTESIAN_POINT('Ctrl Pts',(-21.743187461739,-12.6240117159259,
115.489136281723)) ;
#167471=CARTESIAN_POINT('Ctrl Pts',(-21.8112843757368,-12.8504012275685,
115.660972680477)) ;
#167472=CARTESIAN_POINT('Ctrl Pts',(-21.7911521928067,-12.8903625364955,
115.599653299789)) ;
#167473=CARTESIAN_POINT('Ctrl Pts',(-21.8649560377389,-12.8903625457094,
115.575422262709)) ;
#167474=CARTESIAN_POINT('Ctrl Pts',(-21.9387598826711,-12.8903625549234,
115.551191225629)) ;
#167475=CARTESIAN_POINT('Ctrl Pts',(-21.9588920656012,-12.8504012459964,
115.612510606317)) ;
#167476=CARTESIAN_POINT('Ctrl Pts',(-21.9790242485314,-12.8104399370694,
115.673829987006)) ;
#167477=CARTESIAN_POINT('Ctrl Pts',(-21.9052204035992,-12.8104399278554,
115.698061024086)) ;
#167478=CARTESIAN_POINT('Ctrl Pts',(-21.831416558667,-12.8104399186415,
115.722292061166)) ;
#167479=CARTESIAN_POINT('Ctrl Pts',(-21.8112843757368,-12.8504012275685,
115.660972680477)) ;
#167480=CARTESIAN_POINT('Ctrl Pts',(-21.8582977807734,-13.116472804272,
115.768768866899)) ;
#167481=CARTESIAN_POINT('Ctrl Pts',(-21.8355851398991,-13.1379154690077,
115.699589827564)) ;
#167482=CARTESIAN_POINT('Ctrl Pts',(-21.9093889836109,-13.1379154738939,
115.675358786767)) ;
#167483=CARTESIAN_POINT('Ctrl Pts',(-21.9831928273227,-13.13791547878,115.651127745969)) ;
#167484=CARTESIAN_POINT('Ctrl Pts',(-22.0059054681969,-13.1164728140443,
115.720306785305)) ;
#167485=CARTESIAN_POINT('Ctrl Pts',(-22.0286181090711,-13.0950301493086,
115.789485824641)) ;
#167486=CARTESIAN_POINT('Ctrl Pts',(-21.9548142653594,-13.0950301444224,
115.813716865438)) ;
#167487=CARTESIAN_POINT('Ctrl Pts',(-21.8810104216476,-13.0950301395363,
115.837947906235)) ;
#167488=CARTESIAN_POINT('Ctrl Pts',(-21.8582977807734,-13.116472804272,
115.768768866899)) ;
#167489=CARTESIAN_POINT('Ctrl Pts',(-21.8820745506903,-13.4044926459014,
115.805724068696)) ;
#167490=CARTESIAN_POINT('Ctrl Pts',(-21.8584015173245,-13.4058558527326,
115.733619828702)) ;
#167491=CARTESIAN_POINT('Ctrl Pts',(-21.9322053606268,-13.4058558531923,
115.709388786657)) ;
#167492=CARTESIAN_POINT('Ctrl Pts',(-22.0060092039291,-13.405855853652,
115.685157744613)) ;
#167493=CARTESIAN_POINT('Ctrl Pts',(-22.0296822372949,-13.4044926468209,
115.757261984607)) ;
#167494=CARTESIAN_POINT('Ctrl Pts',(-22.0533552706608,-13.4031294399897,
115.829366224601)) ;
#167495=CARTESIAN_POINT('Ctrl Pts',(-21.9795514273585,-13.40312943953,115.853597266645)) ;
#167496=CARTESIAN_POINT('Ctrl Pts',(-21.9057475840562,-13.4031294390702,
115.877828308689)) ;
#167497=CARTESIAN_POINT('Ctrl Pts',(-21.8820745506903,-13.4044926459014,
115.805724068696)) ;
#167498=CARTESIAN_POINT('Ctrl Pts',(-21.8816087919377,-13.6930971947521,
115.768901188639)) ;
#167499=CARTESIAN_POINT('Ctrl Pts',(-21.8586656358087,-13.6743099521877,
115.699020036887)) ;
#167500=CARTESIAN_POINT('Ctrl Pts',(-21.9324694793602,-13.6743099497306,
115.674788995601)) ;
#167501=CARTESIAN_POINT('Ctrl Pts',(-22.0062733229118,-13.6743099472734,
115.650557954316)) ;
#167502=CARTESIAN_POINT('Ctrl Pts',(-22.0292164790407,-13.6930971898379,
115.720439106068)) ;
#167503=CARTESIAN_POINT('Ctrl Pts',(-22.0521596351697,-13.7118844324023,
115.79032025782)) ;
#167504=CARTESIAN_POINT('Ctrl Pts',(-21.9783557916181,-13.7118844348594,
115.814551299106)) ;
#167505=CARTESIAN_POINT('Ctrl Pts',(-21.9045519480666,-13.7118844373166,
115.838782340391)) ;
#167506=CARTESIAN_POINT('Ctrl Pts',(-21.8816087919377,-13.6930971947521,
115.768901188639)) ;
#167507=CARTESIAN_POINT('Ctrl Pts',(-21.8573708161065,-13.9640294815732,
115.659386725099)) ;
#167508=CARTESIAN_POINT('Ctrl Pts',(-21.8368246163992,-13.9262943650166,
115.596806315842)) ;
#167509=CARTESIAN_POINT('Ctrl Pts',(-21.9106284603522,-13.9262943620916,
115.572575275779)) ;
#167510=CARTESIAN_POINT('Ctrl Pts',(-21.9844323043051,-13.9262943591665,
115.548344235717)) ;
#167511=CARTESIAN_POINT('Ctrl Pts',(-22.0049785040124,-13.9640294757231,
115.610924644974)) ;
#167512=CARTESIAN_POINT('Ctrl Pts',(-22.0255247037197,-14.0017645922797,
115.673505054231)) ;
#167513=CARTESIAN_POINT('Ctrl Pts',(-21.9517208597667,-14.0017645952047,
115.697736094293)) ;
#167514=CARTESIAN_POINT('Ctrl Pts',(-21.8779170158137,-14.0017645981297,
115.721967134356)) ;
#167515=CARTESIAN_POINT('Ctrl Pts',(-21.8573708161065,-13.9640294815732,
115.659386725099)) ;
#167516=CARTESIAN_POINT('Ctrl Pts',(-21.8123589552263,-14.1931760928296,
115.486961111576)) ;
#167517=CARTESIAN_POINT('Ctrl Pts',(-21.7956567301436,-14.1393849019779,
115.436088828833)) ;
#167518=CARTESIAN_POINT('Ctrl Pts',(-21.8694605740056,-14.1393849008332,
115.411857788494)) ;
#167519=CARTESIAN_POINT('Ctrl Pts',(-21.9432644178677,-14.1393848996885,
115.387626748154)) ;
#167520=CARTESIAN_POINT('Ctrl Pts',(-21.9599666429505,-14.1931760905402,
115.438499030898)) ;
#167521=CARTESIAN_POINT('Ctrl Pts',(-21.9766688680333,-14.2469672813919,
115.489371313641)) ;
#167522=CARTESIAN_POINT('Ctrl Pts',(-21.9028650241712,-14.2469672825366,
115.513602353981)) ;
#167523=CARTESIAN_POINT('Ctrl Pts',(-21.8290611803091,-14.2469672836813,
115.53783339432)) ;
#167524=CARTESIAN_POINT('Ctrl Pts',(-21.8123589552263,-14.1931760928296,
115.486961111576)) ;
#167525=CARTESIAN_POINT('Ctrl Pts',(-21.7503610168771,-14.3676938142289,
115.262726512895)) ;
#167526=CARTESIAN_POINT('Ctrl Pts',(-21.7386959620902,-14.3016378950291,
115.227196638184)) ;
#167527=CARTESIAN_POINT('Ctrl Pts',(-21.8124998052628,-14.3016378958559,
115.202965595744)) ;
#167528=CARTESIAN_POINT('Ctrl Pts',(-21.8863036484354,-14.3016378966827,
115.178734553305)) ;
#167529=CARTESIAN_POINT('Ctrl Pts',(-21.8979687032223,-14.3676938158825,
115.214264428016)) ;
#167530=CARTESIAN_POINT('Ctrl Pts',(-21.9096337580092,-14.4337497350823,
115.249794302726)) ;
#167531=CARTESIAN_POINT('Ctrl Pts',(-21.8358299148366,-14.4337497342555,
115.274025345166)) ;
#167532=CARTESIAN_POINT('Ctrl Pts',(-21.762026071664,-14.4337497334287,
115.298256387605)) ;
#167533=CARTESIAN_POINT('Ctrl Pts',(-21.7503610168771,-14.3676938142289,
115.262726512895)) ;
#167534=CARTESIAN_POINT('Ctrl Pts',(-21.6763081582206,-14.4745465378171,
115.001681494378)) ;
#167535=CARTESIAN_POINT('Ctrl Pts',(-21.6705313272715,-14.4009329542059,
114.984086199513)) ;
#167536=CARTESIAN_POINT('Ctrl Pts',(-21.7443351688861,-14.4009329561401,
114.959855152328)) ;
#167537=CARTESIAN_POINT('Ctrl Pts',(-21.8181390105007,-14.4009329580743,
114.935624105143)) ;
#167538=CARTESIAN_POINT('Ctrl Pts',(-21.8239158414498,-14.4745465416855,
114.953219400009)) ;
#167539=CARTESIAN_POINT('Ctrl Pts',(-21.8296926723988,-14.5481601252968,
114.970814694874)) ;
#167540=CARTESIAN_POINT('Ctrl Pts',(-21.7558888307842,-14.5481601233625,
114.995045742059)) ;
#167541=CARTESIAN_POINT('Ctrl Pts',(-21.6820849891696,-14.5481601214283,
115.019276789244)) ;
#167542=CARTESIAN_POINT('Ctrl Pts',(-21.6763081582206,-14.4745465378171,
115.001681494378)) ;
#167543=CARTESIAN_POINT('Ctrl Pts',(-21.596449872518,-14.5056303399819,
114.722959733206)) ;
#167544=CARTESIAN_POINT('Ctrl Pts',(-21.5969750226913,-14.4297391365026,
114.72455925614)) ;
#167545=CARTESIAN_POINT('Ctrl Pts',(-21.6707788622314,-14.4297391368143,
114.700328202637)) ;
#167546=CARTESIAN_POINT('Ctrl Pts',(-21.7445827017715,-14.429739137126,
114.676097149134)) ;
#167547=CARTESIAN_POINT('Ctrl Pts',(-21.7440575515982,-14.5056303406052,
114.674497626199)) ;
#167548=CARTESIAN_POINT('Ctrl Pts',(-21.7435324014249,-14.5815215440845,
114.672898103265)) ;
#167549=CARTESIAN_POINT('Ctrl Pts',(-21.6697285618848,-14.5815215437728,
114.697129156768)) ;
#167550=CARTESIAN_POINT('Ctrl Pts',(-21.5959247223447,-14.5815215434611,
114.721360210271)) ;
#167551=CARTESIAN_POINT('Ctrl Pts',(-21.596449872518,-14.5056303399819,
114.722959733206)) ;
#167552=CARTESIAN_POINT('Ctrl Pts',(-21.5172133727287,-14.4584990503317,
114.446100755161)) ;
#167553=CARTESIAN_POINT('Ctrl Pts',(-21.5240068136617,-14.3857884203973,
114.466792480513)) ;
#167554=CARTESIAN_POINT('Ctrl Pts',(-21.5978106510323,-14.3857884151158,
114.442561420402)) ;
#167555=CARTESIAN_POINT('Ctrl Pts',(-21.6716144884028,-14.3857884098344,
114.41833036029)) ;
#167556=CARTESIAN_POINT('Ctrl Pts',(-21.6648210474699,-14.4584990397688,
114.397638634938)) ;
#167557=CARTESIAN_POINT('Ctrl Pts',(-21.6580276065369,-14.5312096697032,
114.376946909586)) ;
#167558=CARTESIAN_POINT('Ctrl Pts',(-21.5842237691663,-14.5312096749846,
114.401177969697)) ;
#167559=CARTESIAN_POINT('Ctrl Pts',(-21.5104199317957,-14.5312096802661,
114.425409029809)) ;
#167560=CARTESIAN_POINT('Ctrl Pts',(-21.5172133727287,-14.4584990503317,
114.446100755161)) ;
#167561=CARTESIAN_POINT('Ctrl Pts',(-21.4454184043166,-14.3375927241235,
114.192092160154)) ;
#167562=CARTESIAN_POINT('Ctrl Pts',(-21.4579655933527,-14.2732190066455,
114.230308873994)) ;
#167563=CARTESIAN_POINT('Ctrl Pts',(-21.5317694295724,-14.2732189929484,
114.206077810378)) ;
#167564=CARTESIAN_POINT('Ctrl Pts',(-21.6055732657922,-14.2732189792513,
114.181846746761)) ;
#167565=CARTESIAN_POINT('Ctrl Pts',(-21.5930260767561,-14.3375926967294,
114.143630032921)) ;
#167566=CARTESIAN_POINT('Ctrl Pts',(-21.58047888772,-14.4019664142074,114.105413319081)) ;
#167567=CARTESIAN_POINT('Ctrl Pts',(-21.5066750515002,-14.4019664279045,
114.129644382697)) ;
#167568=CARTESIAN_POINT('Ctrl Pts',(-21.4328712152804,-14.4019664416016,
114.153875446314)) ;
#167569=CARTESIAN_POINT('Ctrl Pts',(-21.4454184043166,-14.3375927241235,
114.192092160154)) ;
#167570=CARTESIAN_POINT('Ctrl Pts',(-21.3860672106349,-14.1494056626898,
113.975672837523)) ;
#167571=CARTESIAN_POINT('Ctrl Pts',(-21.4035142179222,-14.0980778114582,
114.02881360737)) ;
#167572=CARTESIAN_POINT('Ctrl Pts',(-21.4773180533873,-14.0980777847103,
114.004582541455)) ;
#167573=CARTESIAN_POINT('Ctrl Pts',(-21.5511218888525,-14.0980777579623,
113.98035147554)) ;
#167574=CARTESIAN_POINT('Ctrl Pts',(-21.5336748815651,-14.1494056091939,
113.927210705693)) ;
#167575=CARTESIAN_POINT('Ctrl Pts',(-21.5162278742778,-14.2007334604254,
113.874069935846)) ;
#167576=CARTESIAN_POINT('Ctrl Pts',(-21.4424240388127,-14.2007334871734,
113.898301001761)) ;
#167577=CARTESIAN_POINT('Ctrl Pts',(-21.3686202033475,-14.2007335139213,
113.922532067676)) ;
#167578=CARTESIAN_POINT('Ctrl Pts',(-21.3860672106349,-14.1494056626898,
113.975672837523)) ;
#167579=CARTESIAN_POINT('Ctrl Pts',(-21.345130013158,-13.9095500364901,
113.815534566818)) ;
#167580=CARTESIAN_POINT('Ctrl Pts',(-21.3661940068873,-13.8748947454948,
113.879692093934)) ;
#167581=CARTESIAN_POINT('Ctrl Pts',(-21.4399978437013,-13.874894705204,
113.855461032127)) ;
#167582=CARTESIAN_POINT('Ctrl Pts',(-21.5138016805153,-13.8748946649131,
113.831229970321)) ;
#167583=CARTESIAN_POINT('Ctrl Pts',(-21.492737686786,-13.9095499559084,
113.767072443205)) ;
#167584=CARTESIAN_POINT('Ctrl Pts',(-21.4716736930567,-13.9442052469036,
113.702914916089)) ;
#167585=CARTESIAN_POINT('Ctrl Pts',(-21.3978698562426,-13.9442052871945,
113.727145977895)) ;
#167586=CARTESIAN_POINT('Ctrl Pts',(-21.3240660194286,-13.9442053274854,
113.751377039702)) ;
#167587=CARTESIAN_POINT('Ctrl Pts',(-21.345130013158,-13.9095500364901,
113.815534566818)) ;
#167588=CARTESIAN_POINT('Ctrl Pts',(-21.3258230846178,-13.6354015229083,
113.721370608325)) ;
#167589=CARTESIAN_POINT('Ctrl Pts',(-21.3489970490078,-13.6198370471349,
113.791954765778)) ;
#167590=CARTESIAN_POINT('Ctrl Pts',(-21.4228008888894,-13.6198369951942,
113.767723713315)) ;
#167591=CARTESIAN_POINT('Ctrl Pts',(-21.496604728771,-13.6198369432535,
113.743492660852)) ;
#167592=CARTESIAN_POINT('Ctrl Pts',(-21.4734307643811,-13.6354014190268,
113.672908503398)) ;
#167593=CARTESIAN_POINT('Ctrl Pts',(-21.4502567999911,-13.6509658948002,
113.602324345945)) ;
#167594=CARTESIAN_POINT('Ctrl Pts',(-21.3764529601095,-13.6509659467409,
113.626555398408)) ;
#167595=CARTESIAN_POINT('Ctrl Pts',(-21.3026491202279,-13.6509659986816,
113.650786450871)) ;
#167596=CARTESIAN_POINT('Ctrl Pts',(-21.3258230846178,-13.6354015229083,
113.721370608325)) ;
#167597=CARTESIAN_POINT('Ctrl Pts',(-21.3302591662937,-13.3449945339553,
113.699428650571)) ;
#167598=CARTESIAN_POINT('Ctrl Pts',(-21.3538905068384,-13.3496833242157,
113.771405902157)) ;
#167599=CARTESIAN_POINT('Ctrl Pts',(-21.4276943513303,-13.3496832627429,
113.747174863736)) ;
#167600=CARTESIAN_POINT('Ctrl Pts',(-21.5014981958221,-13.3496832012701,
113.722943825315)) ;
#167601=CARTESIAN_POINT('Ctrl Pts',(-21.4778668552774,-13.3449944110097,
113.650966573729)) ;
#167602=CARTESIAN_POINT('Ctrl Pts',(-21.4542355147327,-13.3403056207493,
113.578989322142)) ;
#167603=CARTESIAN_POINT('Ctrl Pts',(-21.3804316702409,-13.3403056822221,
113.603220360563)) ;
#167604=CARTESIAN_POINT('Ctrl Pts',(-21.306627825749,-13.3403057436949,
113.627451398984)) ;
#167605=CARTESIAN_POINT('Ctrl Pts',(-21.3302591662937,-13.3449945339553,
113.699428650571)) ;
#167606=CARTESIAN_POINT('Ctrl Pts',(-21.3588254375783,-13.0600685836045,
113.75103011028)) ;
#167607=CARTESIAN_POINT('Ctrl Pts',(-21.3812291127916,-13.0846570049903,
113.8192680915)) ;
#167608=CARTESIAN_POINT('Ctrl Pts',(-21.4550329630849,-13.0846569392068,
113.795037070749)) ;
#167609=CARTESIAN_POINT('Ctrl Pts',(-21.5288368133782,-13.0846568734233,
113.770806049999)) ;
#167610=CARTESIAN_POINT('Ctrl Pts',(-21.5064331381649,-13.0600684520375,
113.702568068778)) ;
#167611=CARTESIAN_POINT('Ctrl Pts',(-21.4840294629517,-13.0354800306517,
113.634330087558)) ;
#167612=CARTESIAN_POINT('Ctrl Pts',(-21.4102256126584,-13.0354800964351,
113.658561108309)) ;
#167613=CARTESIAN_POINT('Ctrl Pts',(-21.3364217623651,-13.0354801622186,
113.68279212906)) ;
#167614=CARTESIAN_POINT('Ctrl Pts',(-21.3588254375783,-13.0600685836045,
113.75103011028)) ;
#167615=CARTESIAN_POINT('Ctrl Pts',(-21.4108808833159,-12.7987719757991,
113.873871369962)) ;
#167616=CARTESIAN_POINT('Ctrl Pts',(-21.4304218220357,-12.8416392533606,
113.933389917914)) ;
#167617=CARTESIAN_POINT('Ctrl Pts',(-21.5042256793353,-12.8416391878999,
113.909158918504)) ;
#167618=CARTESIAN_POINT('Ctrl Pts',(-21.5780295366349,-12.8416391224392,
113.884927919093)) ;
#167619=CARTESIAN_POINT('Ctrl Pts',(-21.5584885979151,-12.7987718448777,
113.825409371141)) ;
#167620=CARTESIAN_POINT('Ctrl Pts',(-21.5389476591953,-12.7559045673161,
113.765890823189)) ;
#167621=CARTESIAN_POINT('Ctrl Pts',(-21.4651438018957,-12.7559046327768,
113.790121822599)) ;
#167622=CARTESIAN_POINT('Ctrl Pts',(-21.3913399445961,-12.7559046982375,
113.81435282201)) ;
#167623=CARTESIAN_POINT('Ctrl Pts',(-21.4108808833159,-12.7987719757991,
113.873871369962)) ;
#167624=CARTESIAN_POINT('Ctrl Pts',(-21.4821786810617,-12.5848307790968,
114.055776077785)) ;
#167625=CARTESIAN_POINT('Ctrl Pts',(-21.4974995321701,-12.6426967262578,
114.102440919885)) ;
#167626=CARTESIAN_POINT('Ctrl Pts',(-21.571303395686,-12.6426966715405,
114.078209939408)) ;
#167627=CARTESIAN_POINT('Ctrl Pts',(-21.6451072592018,-12.6426966168232,
114.053978958931)) ;
#167628=CARTESIAN_POINT('Ctrl Pts',(-21.6297864080934,-12.5848306696622,
114.007314116831)) ;
#167629=CARTESIAN_POINT('Ctrl Pts',(-21.6144655569851,-12.5269647225012,
113.960649274732)) ;
#167630=CARTESIAN_POINT('Ctrl Pts',(-21.5406616934692,-12.5269647772185,
113.984880255209)) ;
#167631=CARTESIAN_POINT('Ctrl Pts',(-21.4668578299534,-12.5269648319358,
114.009111235686)) ;
#167632=CARTESIAN_POINT('Ctrl Pts',(-21.4821786810617,-12.5848307790968,
114.055776077785)) ;
#167633=CARTESIAN_POINT('Ctrl Pts',(-21.5695756033995,-12.428840573078,
114.286444660631)) ;
#167634=CARTESIAN_POINT('Ctrl Pts',(-21.5795521820823,-12.4976814923142,
114.31683171135)) ;
#167635=CARTESIAN_POINT('Ctrl Pts',(-21.6533560513287,-12.4976814537986,
114.292600748327)) ;
#167636=CARTESIAN_POINT('Ctrl Pts',(-21.7271599205752,-12.497681415283,
114.268369785305)) ;
#167637=CARTESIAN_POINT('Ctrl Pts',(-21.7171833418924,-12.4288404960468,
114.237982734586)) ;
#167638=CARTESIAN_POINT('Ctrl Pts',(-21.7072067632097,-12.3599995768106,
114.207595683868)) ;
#167639=CARTESIAN_POINT('Ctrl Pts',(-21.6334028939632,-12.3599996153262,
114.23182664689)) ;
#167640=CARTESIAN_POINT('Ctrl Pts',(-21.5595990247167,-12.3599996538418,
114.256057609913)) ;
#167641=CARTESIAN_POINT('Ctrl Pts',(-21.5695756033995,-12.428840573078,
114.286444660631)) ;
#167642=CARTESIAN_POINT('Ctrl Pts',(-21.6669221796403,-12.3440689509793,
114.547509032478)) ;
#167643=CARTESIAN_POINT('Ctrl Pts',(-21.6708501782994,-12.4189286311326,
114.559473084482)) ;
#167644=CARTESIAN_POINT('Ctrl Pts',(-21.7446540514633,-12.4189286151795,
114.535242133391)) ;
#167645=CARTESIAN_POINT('Ctrl Pts',(-21.8184579246271,-12.4189285992263,
114.5110111823)) ;
#167646=CARTESIAN_POINT('Ctrl Pts',(-21.8145299259679,-12.3440689190729,
114.499047130296)) ;
#167647=CARTESIAN_POINT('Ctrl Pts',(-21.8106019273088,-12.2692092389195,
114.487083078292)) ;
#167648=CARTESIAN_POINT('Ctrl Pts',(-21.736798054145,-12.2692092548727,
114.511314029383)) ;
#167649=CARTESIAN_POINT('Ctrl Pts',(-21.6629941809811,-12.2692092708259,
114.535544980474)) ;
#167650=CARTESIAN_POINT('Ctrl Pts',(-21.6669221796403,-12.3440689509793,
114.547509032478)) ;
#167651=CARTESIAN_POINT('Ctrl Pts',(-21.7687094216625,-12.3364316802486,
114.821900463108)) ;
#167652=CARTESIAN_POINT('Ctrl Pts',(-21.7662742013755,-12.4119346033566,
114.814483177004)) ;
#167653=CARTESIAN_POINT('Ctrl Pts',(-21.8400780763928,-12.4119346140826,
114.790252231559)) ;
#167654=CARTESIAN_POINT('Ctrl Pts',(-21.9138819514101,-12.4119346248087,
114.766021286114)) ;
#167655=CARTESIAN_POINT('Ctrl Pts',(-21.916317171697,-12.3364317017007,
114.773438572217)) ;
#167656=CARTESIAN_POINT('Ctrl Pts',(-21.918752391984,-12.2609287785927,
114.78085585832)) ;
#167657=CARTESIAN_POINT('Ctrl Pts',(-21.8449485169667,-12.2609287678666,
114.805086803766)) ;
#167658=CARTESIAN_POINT('Ctrl Pts',(-21.7711446419494,-12.2609287571406,
114.829317749211)) ;
#167659=CARTESIAN_POINT('Ctrl Pts',(-21.7687094216625,-12.3364316802486,
114.821900463108)) ;
#167660=CARTESIAN_POINT('Ctrl Pts',(-21.8668995311495,-12.4059134721985,
115.085690184209)) ;
#167661=CARTESIAN_POINT('Ctrl Pts',(-21.8583354753262,-12.4766756049436,
115.059605453997)) ;
#167662=CARTESIAN_POINT('Ctrl Pts',(-21.9321393490943,-12.4766756431297,
115.035374504746)) ;
#167663=CARTESIAN_POINT('Ctrl Pts',(-22.0059432228623,-12.4766756813157,
115.011143555496)) ;
#167664=CARTESIAN_POINT('Ctrl Pts',(-22.0145072786857,-12.4059135485707,
115.037228285708)) ;
#167665=CARTESIAN_POINT('Ctrl Pts',(-22.0230713345091,-12.3351514158256,
115.06331301592)) ;
#167666=CARTESIAN_POINT('Ctrl Pts',(-21.949267460741,-12.3351513776395,
115.087543965171)) ;
#167667=CARTESIAN_POINT('Ctrl Pts',(-21.8754635869729,-12.3351513394535,
115.111774914421)) ;
#167668=CARTESIAN_POINT('Ctrl Pts',(-21.8668995311495,-12.4059134721985,
115.085690184209)) ;
#167669=CARTESIAN_POINT('Ctrl Pts',(-21.9568607042708,-12.5482447968648,
115.324163533208)) ;
#167670=CARTESIAN_POINT('Ctrl Pts',(-21.9427385662062,-12.609174259838,
115.281149781333)) ;
#167671=CARTESIAN_POINT('Ctrl Pts',(-22.0165424363522,-12.6091743240943,
115.25691882105)) ;
#167672=CARTESIAN_POINT('Ctrl Pts',(-22.0903463064982,-12.6091743883507,
115.232687860767)) ;
#167673=CARTESIAN_POINT('Ctrl Pts',(-22.1044684445627,-12.5482449253774,
115.275701612643)) ;
#167674=CARTESIAN_POINT('Ctrl Pts',(-22.1185905826272,-12.4873154624041,
115.318715364518)) ;
#167675=CARTESIAN_POINT('Ctrl Pts',(-22.0447867124812,-12.4873153981478,
115.342946324801)) ;
#167676=CARTESIAN_POINT('Ctrl Pts',(-21.9709828423353,-12.4873153338915,
115.367177285083)) ;
#167677=CARTESIAN_POINT('Ctrl Pts',(-21.9568607042708,-12.5482447968648,
115.324163533208)) ;
#167678=CARTESIAN_POINT('Ctrl Pts',(-22.0318603212468,-12.7523234032848,
115.517213231457)) ;
#167679=CARTESIAN_POINT('Ctrl Pts',(-22.0132133823266,-12.7990945462317,
115.460417666269)) ;
#167680=CARTESIAN_POINT('Ctrl Pts',(-22.0870172463905,-12.7990946317952,
115.436186687461)) ;
#167681=CARTESIAN_POINT('Ctrl Pts',(-22.1608211104543,-12.7990947173587,
115.411955708654)) ;
#167682=CARTESIAN_POINT('Ctrl Pts',(-22.1794680493745,-12.7523235744117,
115.468751273841)) ;
#167683=CARTESIAN_POINT('Ctrl Pts',(-22.1981149882947,-12.7055524314648,
115.525546839029)) ;
#167684=CARTESIAN_POINT('Ctrl Pts',(-22.1243111242308,-12.7055523459013,
115.549777817836)) ;
#167685=CARTESIAN_POINT('Ctrl Pts',(-22.050507260167,-12.7055522603379,
115.574008796644)) ;
#167686=CARTESIAN_POINT('Ctrl Pts',(-22.0318603212468,-12.7523234032848,
115.517213231457)) ;
#167687=CARTESIAN_POINT('Ctrl Pts',(-22.0879198570419,-13.0044659647124,
115.652477656322)) ;
#167688=CARTESIAN_POINT('Ctrl Pts',(-22.066065668734,-13.0337028196908,
115.585913326992)) ;
#167689=CARTESIAN_POINT('Ctrl Pts',(-22.1398695249688,-13.0337029200477,
115.561682324338)) ;
#167690=CARTESIAN_POINT('Ctrl Pts',(-22.2136733812036,-13.0337030204046,
115.537451321685)) ;
#167691=CARTESIAN_POINT('Ctrl Pts',(-22.2355275695115,-13.0044661654261,
115.604015651014)) ;
#167692=CARTESIAN_POINT('Ctrl Pts',(-22.2573817578194,-12.9752293104477,
115.670579980344)) ;
#167693=CARTESIAN_POINT('Ctrl Pts',(-22.1835779015846,-12.9752292100908,
115.694810982998)) ;
#167694=CARTESIAN_POINT('Ctrl Pts',(-22.1097740453498,-12.9752291097339,
115.719041985652)) ;
#167695=CARTESIAN_POINT('Ctrl Pts',(-22.0879198570419,-13.0044659647124,
115.652477656322)) ;
#167696=CARTESIAN_POINT('Ctrl Pts',(-22.1214488600341,-13.2877069321833,
115.718954843121)) ;
#167697=CARTESIAN_POINT('Ctrl Pts',(-22.0979587435142,-13.2972126814731,
115.647407740385)) ;
#167698=CARTESIAN_POINT('Ctrl Pts',(-22.1717625908651,-13.2972127876648,
115.623176710672)) ;
#167699=CARTESIAN_POINT('Ctrl Pts',(-22.245566438216,-13.2972128938564,
115.598945680959)) ;
#167700=CARTESIAN_POINT('Ctrl Pts',(-22.269056554736,-13.2877071445666,
115.670492783696)) ;
#167701=CARTESIAN_POINT('Ctrl Pts',(-22.2925466712559,-13.2782013952768,
115.742039886433)) ;
#167702=CARTESIAN_POINT('Ctrl Pts',(-22.218742823905,-13.2782012890852,
115.766270916145)) ;
#167703=CARTESIAN_POINT('Ctrl Pts',(-22.1449389765541,-13.2782011828935,
115.790501945858)) ;
#167704=CARTESIAN_POINT('Ctrl Pts',(-22.1214488600341,-13.2877069321833,
115.718954843121)) ;
#167705=CARTESIAN_POINT('Ctrl Pts',(-22.1306963457754,-13.5768962487208,
115.71190010407)) ;
#167706=CARTESIAN_POINT('Ctrl Pts',(-22.1072546120684,-13.5662255723237,
115.640500367543)) ;
#167707=CARTESIAN_POINT('Ctrl Pts',(-22.1810584505935,-13.5662256764684,
115.616269310949)) ;
#167708=CARTESIAN_POINT('Ctrl Pts',(-22.2548622891185,-13.5662257806131,
115.592038254354)) ;
#167709=CARTESIAN_POINT('Ctrl Pts',(-22.2783040228256,-13.5768964570101,
115.66343799088)) ;
#167710=CARTESIAN_POINT('Ctrl Pts',(-22.3017457565327,-13.5875671334072,
115.734837727407)) ;
#167711=CARTESIAN_POINT('Ctrl Pts',(-22.2279419180076,-13.5875670292625,
115.759068784001)) ;
#167712=CARTESIAN_POINT('Ctrl Pts',(-22.1541380794825,-13.5875669251178,
115.783299840596)) ;
#167713=CARTESIAN_POINT('Ctrl Pts',(-22.1306963457754,-13.5768962487208,
115.71190010407)) ;
#167714=CARTESIAN_POINT('Ctrl Pts',(-22.1159420679376,-13.8582071770573,
115.631296548337)) ;
#167715=CARTESIAN_POINT('Ctrl Pts',(-22.0942331444257,-13.8278804219563,
115.565174672)) ;
#167716=CARTESIAN_POINT('Ctrl Pts',(-22.1680369749167,-13.8278805144787,
115.540943590935)) ;
#167717=CARTESIAN_POINT('Ctrl Pts',(-22.2418408054076,-13.8278806070012,
115.516712509869)) ;
#167718=CARTESIAN_POINT('Ctrl Pts',(-22.2635497289195,-13.8582073621022,
115.582834386206)) ;
#167719=CARTESIAN_POINT('Ctrl Pts',(-22.2852586524313,-13.8885341172032,
115.648956262542)) ;
#167720=CARTESIAN_POINT('Ctrl Pts',(-22.2114548219404,-13.8885340246808,
115.673187343608)) ;
#167721=CARTESIAN_POINT('Ctrl Pts',(-22.1376509914495,-13.8885339321583,
115.697418424673)) ;
#167722=CARTESIAN_POINT('Ctrl Pts',(-22.1159420679376,-13.8582071770573,
115.631296548337)) ;
#167723=CARTESIAN_POINT('Ctrl Pts',(-22.0788832137679,-14.1061445299723,
115.482974778229)) ;
#167724=CARTESIAN_POINT('Ctrl Pts',(-22.0604625649498,-14.0584618505827,
115.426868455962)) ;
#167725=CARTESIAN_POINT('Ctrl Pts',(-22.134266389145,-14.0584619253186,
115.40263735572)) ;
#167726=CARTESIAN_POINT('Ctrl Pts',(-22.20807021334,-14.0584620000544,115.378406255479)) ;
#167727=CARTESIAN_POINT('Ctrl Pts',(-22.2264908621581,-14.106144679444,
115.434512577746)) ;
#167728=CARTESIAN_POINT('Ctrl Pts',(-22.2449115109762,-14.1538273588336,
115.490618900013)) ;
#167729=CARTESIAN_POINT('Ctrl Pts',(-22.1711076867811,-14.1538272840978,
115.514850000255)) ;
#167730=CARTESIAN_POINT('Ctrl Pts',(-22.097303862586,-14.1538272093619,
115.539081100496)) ;
#167731=CARTESIAN_POINT('Ctrl Pts',(-22.0788832137679,-14.1061445299723,
115.482974778229)) ;
#167732=CARTESIAN_POINT('Ctrl Pts',(-22.02325368044,-14.3044364274605,115.278182501201)) ;
#167733=CARTESIAN_POINT('Ctrl Pts',(-22.0094209261797,-14.2428379118998,
115.236050165413)) ;
#167734=CARTESIAN_POINT('Ctrl Pts',(-22.0832247460729,-14.2428379649648,
115.211819052068)) ;
#167735=CARTESIAN_POINT('Ctrl Pts',(-22.157028565966,-14.2428380180299,
115.187587938724)) ;
#167736=CARTESIAN_POINT('Ctrl Pts',(-22.1708613202263,-14.3044365335905,
115.229720274512)) ;
#167737=CARTESIAN_POINT('Ctrl Pts',(-22.1846940744866,-14.3660350491512,
115.271852610301)) ;
#167738=CARTESIAN_POINT('Ctrl Pts',(-22.1108902545935,-14.3660349960862,
115.296083723645)) ;
#167739=CARTESIAN_POINT('Ctrl Pts',(-22.0370864347003,-14.3660349430211,
115.32031483699)) ;
#167740=CARTESIAN_POINT('Ctrl Pts',(-22.02325368044,-14.3044364274605,115.278182501201)) ;
#167741=CARTESIAN_POINT('Ctrl Pts',(-21.9534860382684,-14.4399899755949,
115.030260894437)) ;
#167742=CARTESIAN_POINT('Ctrl Pts',(-21.9452364473927,-14.3688346755136,
115.005133973366)) ;
#167743=CARTESIAN_POINT('Ctrl Pts',(-22.0190402654135,-14.3688347045207,
114.980902854319)) ;
#167744=CARTESIAN_POINT('Ctrl Pts',(-22.0928440834343,-14.3688347335278,
114.956671735271)) ;
#167745=CARTESIAN_POINT('Ctrl Pts',(-22.10109367431,-14.4399900336091,114.981798656342)) ;
#167746=CARTESIAN_POINT('Ctrl Pts',(-22.1093432651856,-14.5111453336905,
115.006925577413)) ;
#167747=CARTESIAN_POINT('Ctrl Pts',(-22.0355394471648,-14.5111453046834,
115.03115669646)) ;
#167748=CARTESIAN_POINT('Ctrl Pts',(-21.961735629144,-14.5111452756763,
115.055387815508)) ;
#167749=CARTESIAN_POINT('Ctrl Pts',(-21.9534860382684,-14.4399899755949,
115.030260894437)) ;
#167750=CARTESIAN_POINT('Ctrl Pts',(-21.8748683527051,-14.5025588290042,
114.755160393342)) ;
#167751=CARTESIAN_POINT('Ctrl Pts',(-21.8728327619573,-14.4269270667857,
114.748960313873)) ;
#167752=CARTESIAN_POINT('Ctrl Pts',(-21.9466365811031,-14.4269270722705,
114.724729198252)) ;
#167753=CARTESIAN_POINT('Ctrl Pts',(-22.0204404002489,-14.4269270777552,
114.700498082631)) ;
#167754=CARTESIAN_POINT('Ctrl Pts',(-22.0224759909966,-14.5025588399736,
114.7066981621)) ;
#167755=CARTESIAN_POINT('Ctrl Pts',(-22.0245115817444,-14.5781906021921,
114.71289824157)) ;
#167756=CARTESIAN_POINT('Ctrl Pts',(-21.9507077625986,-14.5781905967074,
114.737129357191)) ;
#167757=CARTESIAN_POINT('Ctrl Pts',(-21.8769039434528,-14.5781905912227,
114.761360472812)) ;
#167758=CARTESIAN_POINT('Ctrl Pts',(-21.8748683527051,-14.5025588290042,
114.755160393342)) ;
#167759=CARTESIAN_POINT('Ctrl Pts',(-21.7947021537826,-14.4867545034676,
114.475532312766)) ;
#167760=CARTESIAN_POINT('Ctrl Pts',(-21.7989943291188,-14.4121117686934,
114.488605587658)) ;
#167761=CARTESIAN_POINT('Ctrl Pts',(-21.8727981510333,-14.4121117549338,
114.46437448047)) ;
#167762=CARTESIAN_POINT('Ctrl Pts',(-21.9466019729478,-14.4121117411741,
114.440143373282)) ;
#167763=CARTESIAN_POINT('Ctrl Pts',(-21.9423097976117,-14.4867544759483,
114.42707009839)) ;
#167764=CARTESIAN_POINT('Ctrl Pts',(-21.9380176222755,-14.5613972107224,
114.413996823498)) ;
#167765=CARTESIAN_POINT('Ctrl Pts',(-21.864213800361,-14.5613972244821,
114.438227930686)) ;
#167766=CARTESIAN_POINT('Ctrl Pts',(-21.7904099784465,-14.5613972382417,
114.462459037874)) ;
#167767=CARTESIAN_POINT('Ctrl Pts',(-21.7947021537826,-14.4867545034676,
114.475532312766)) ;
#167768=CARTESIAN_POINT('Ctrl Pts',(-21.7193075294336,-14.395053842158,
114.210551242128)) ;
#167769=CARTESIAN_POINT('Ctrl Pts',(-21.7296015565806,-14.3267009786415,
114.241905189105)) ;
#167770=CARTESIAN_POINT('Ctrl Pts',(-21.8034053823653,-14.3267009501932,
114.217674093705)) ;
#167771=CARTESIAN_POINT('Ctrl Pts',(-21.8772092081501,-14.3267009217449,
114.193442998305)) ;
#167772=CARTESIAN_POINT('Ctrl Pts',(-21.866915181003,-14.3950537852614,
114.162089051328)) ;
#167773=CARTESIAN_POINT('Ctrl Pts',(-21.856621153856,-14.463406648778,114.130735104351)) ;
#167774=CARTESIAN_POINT('Ctrl Pts',(-21.7828173280713,-14.4634066772262,
114.154966199751)) ;
#167775=CARTESIAN_POINT('Ctrl Pts',(-21.7090135022865,-14.4634067056745,
114.179197295151)) ;
#167776=CARTESIAN_POINT('Ctrl Pts',(-21.7193075294336,-14.395053842158,
114.210551242128)) ;
#167777=CARTESIAN_POINT('Ctrl Pts',(-21.6543128388828,-14.2332235226471,
113.977125631216)) ;
#167778=CARTESIAN_POINT('Ctrl Pts',(-21.6698942629534,-14.1760661182545,
114.02458413594)) ;
#167779=CARTESIAN_POINT('Ctrl Pts',(-21.7436980937312,-14.1760660813659,
114.000353055749)) ;
#167780=CARTESIAN_POINT('Ctrl Pts',(-21.8175019245091,-14.1760660444773,
113.976121975557)) ;
#167781=CARTESIAN_POINT('Ctrl Pts',(-21.8019205004385,-14.2332234488699,
113.928663470833)) ;
#167782=CARTESIAN_POINT('Ctrl Pts',(-21.786339076368,-14.2903808532625,
113.881204966109)) ;
#167783=CARTESIAN_POINT('Ctrl Pts',(-21.7125352455901,-14.2903808901511,
113.905436046301)) ;
#167784=CARTESIAN_POINT('Ctrl Pts',(-21.6387314148122,-14.2903809270397,
113.929667126492)) ;
#167785=CARTESIAN_POINT('Ctrl Pts',(-21.6543128388828,-14.2332235226471,
113.977125631216)) ;
#167786=CARTESIAN_POINT('Ctrl Pts',(-21.605413342524,-14.0127300062097,
113.792696033333)) ;
#167787=CARTESIAN_POINT('Ctrl Pts',(-21.6251670568667,-13.9708810531426,
113.852862660857)) ;
#167788=CARTESIAN_POINT('Ctrl Pts',(-21.6989708926631,-13.9708810143348,
113.828631595951)) ;
#167789=CARTESIAN_POINT('Ctrl Pts',(-21.7727747284595,-13.9708809755269,
113.804400531044)) ;
#167790=CARTESIAN_POINT('Ctrl Pts',(-21.7530210141168,-14.0127299285939,
113.744233903521)) ;
#167791=CARTESIAN_POINT('Ctrl Pts',(-21.7332672997741,-14.054578881661,
113.684067275997)) ;
#167792=CARTESIAN_POINT('Ctrl Pts',(-21.6594634639777,-14.0545789204688,
113.708298340903)) ;
#167793=CARTESIAN_POINT('Ctrl Pts',(-21.5856596281813,-14.0545789592767,
113.732529405809)) ;
#167794=CARTESIAN_POINT('Ctrl Pts',(-21.605413342524,-14.0127300062097,
113.792696033333)) ;
#167795=CARTESIAN_POINT('Ctrl Pts',(-21.5768555726489,-13.7497867225439,
113.670246591571)) ;
#167796=CARTESIAN_POINT('Ctrl Pts',(-21.5993671606262,-13.7262335262759,
113.738813257035)) ;
#167797=CARTESIAN_POINT('Ctrl Pts',(-21.6731710007795,-13.7262334907042,
113.7145822054)) ;
#167798=CARTESIAN_POINT('Ctrl Pts',(-21.7469748409328,-13.7262334551324,
113.690351153764)) ;
#167799=CARTESIAN_POINT('Ctrl Pts',(-21.7244632529556,-13.7497866514004,
113.6217844883)) ;
#167800=CARTESIAN_POINT('Ctrl Pts',(-21.7019516649783,-13.7733398476684,
113.553217822836)) ;
#167801=CARTESIAN_POINT('Ctrl Pts',(-21.628147824825,-13.7733398832402,
113.577448874471)) ;
#167802=CARTESIAN_POINT('Ctrl Pts',(-21.5543439846717,-13.7733399188119,
113.601679926107)) ;
#167803=CARTESIAN_POINT('Ctrl Pts',(-21.5768555726489,-13.7497867225439,
113.670246591571)) ;
#167804=CARTESIAN_POINT('Ctrl Pts',(-21.5715836653068,-13.4618226176213,
113.618571162712)) ;
#167805=CARTESIAN_POINT('Ctrl Pts',(-21.5952346989203,-13.4583403895165,
113.690608395545)) ;
#167806=CARTESIAN_POINT('Ctrl Pts',(-21.6690385421918,-13.458340362269,
113.666377353407)) ;
#167807=CARTESIAN_POINT('Ctrl Pts',(-21.7428423854632,-13.4583403350215,
113.642146311268)) ;
#167808=CARTESIAN_POINT('Ctrl Pts',(-21.7191913518496,-13.4618225631264,
113.570109078435)) ;
#167809=CARTESIAN_POINT('Ctrl Pts',(-21.6955403182359,-13.4653047912312,
113.498071845602)) ;
#167810=CARTESIAN_POINT('Ctrl Pts',(-21.6217364749645,-13.4653048184787,
113.52230288774)) ;
#167811=CARTESIAN_POINT('Ctrl Pts',(-21.5479326316931,-13.4653048457262,
113.546533929879)) ;
#167812=CARTESIAN_POINT('Ctrl Pts',(-21.5715836653068,-13.4618226176213,
113.618571162712)) ;
#167813=CARTESIAN_POINT('Ctrl Pts',(-21.5903574401915,-13.1741720910159,
113.64057286247)) ;
#167814=CARTESIAN_POINT('Ctrl Pts',(-21.6134611754768,-13.1907692085376,
113.710943112796)) ;
#167815=CARTESIAN_POINT('Ctrl Pts',(-21.6872650205988,-13.1907691874801,
113.686712076294)) ;
#167816=CARTESIAN_POINT('Ctrl Pts',(-21.7610688657208,-13.1907691664227,
113.662481039792)) ;
#167817=CARTESIAN_POINT('Ctrl Pts',(-21.7379651304355,-13.1741720489011,
113.592110789466)) ;
#167818=CARTESIAN_POINT('Ctrl Pts',(-21.7148613951501,-13.1575749313794,
113.52174053914)) ;
#167819=CARTESIAN_POINT('Ctrl Pts',(-21.6410575500281,-13.1575749524368,
113.545971575642)) ;
#167820=CARTESIAN_POINT('Ctrl Pts',(-21.5672537049062,-13.1575749734943,
113.570202612144)) ;
#167821=CARTESIAN_POINT('Ctrl Pts',(-21.5903574401915,-13.1741720910159,
113.64057286247)) ;
#167822=CARTESIAN_POINT('Ctrl Pts',(-21.6331211640016,-12.9003777795887,
113.735179592382)) ;
#167823=CARTESIAN_POINT('Ctrl Pts',(-21.654011633631,-12.9361179634059,
113.798808592458)) ;
#167824=CARTESIAN_POINT('Ctrl Pts',(-21.7278154791519,-12.9361179523589,
113.774577557172)) ;
#167825=CARTESIAN_POINT('Ctrl Pts',(-21.8016193246729,-12.9361179413118,
113.750346521885)) ;
#167826=CARTESIAN_POINT('Ctrl Pts',(-21.7807288550435,-12.9003777574947,
113.686717521809)) ;
#167827=CARTESIAN_POINT('Ctrl Pts',(-21.759838385414,-12.8646375736775,
113.623088521733)) ;
#167828=CARTESIAN_POINT('Ctrl Pts',(-21.6860345398931,-12.8646375847245,
113.64731955702)) ;
#167829=CARTESIAN_POINT('Ctrl Pts',(-21.6122306943722,-12.8646375957715,
113.671550592306)) ;
#167830=CARTESIAN_POINT('Ctrl Pts',(-21.6331211640016,-12.9003777795887,
113.735179592382)) ;
#167831=CARTESIAN_POINT('Ctrl Pts',(-21.6969659859909,-12.6657294356323,
113.89428002861)) ;
#167832=CARTESIAN_POINT('Ctrl Pts',(-21.7141616319594,-12.7179077722526,
113.946655191865)) ;
#167833=CARTESIAN_POINT('Ctrl Pts',(-21.7879654770538,-12.7179077672934,
113.922424155279)) ;
#167834=CARTESIAN_POINT('Ctrl Pts',(-21.8617693221483,-12.7179077623343,
113.898193118693)) ;
#167835=CARTESIAN_POINT('Ctrl Pts',(-21.8445736761798,-12.665729425714,
113.845817955438)) ;
#167836=CARTESIAN_POINT('Ctrl Pts',(-21.8273780302113,-12.6135510890938,
113.793442792184)) ;
#167837=CARTESIAN_POINT('Ctrl Pts',(-21.7535741851169,-12.6135510940529,
113.81767382877)) ;
#167838=CARTESIAN_POINT('Ctrl Pts',(-21.6797703400225,-12.6135510990121,
113.841904865355)) ;
#167839=CARTESIAN_POINT('Ctrl Pts',(-21.6969659859909,-12.6657294356323,
113.89428002861)) ;
#167840=CARTESIAN_POINT('Ctrl Pts',(-21.778661308746,-12.4838951882172,
114.107573907655)) ;
#167841=CARTESIAN_POINT('Ctrl Pts',(-21.7909137057025,-12.5488490680583,
114.144892731903)) ;
#167842=CARTESIAN_POINT('Ctrl Pts',(-21.8647175496609,-12.5488490674887,
114.120661691857)) ;
#167843=CARTESIAN_POINT('Ctrl Pts',(-21.9385213936193,-12.5488490669192,
114.096430651811)) ;
#167844=CARTESIAN_POINT('Ctrl Pts',(-21.9262689966628,-12.4838951870781,
114.059111827563)) ;
#167845=CARTESIAN_POINT('Ctrl Pts',(-21.9140165997062,-12.418941307237,
114.021793003316)) ;
#167846=CARTESIAN_POINT('Ctrl Pts',(-21.8402127557478,-12.4189413078066,
114.046024043362)) ;
#167847=CARTESIAN_POINT('Ctrl Pts',(-21.7664089117894,-12.4189413083761,
114.070255083408)) ;
#167848=CARTESIAN_POINT('Ctrl Pts',(-21.778661308746,-12.4838951882172,
114.107573907655)) ;
#167849=CARTESIAN_POINT('Ctrl Pts',(-21.8724459100831,-12.3696269961183,
114.357853657507)) ;
#167850=CARTESIAN_POINT('Ctrl Pts',(-21.8788999247854,-12.4426568392055,
114.377511544911)) ;
#167851=CARTESIAN_POINT('Ctrl Pts',(-21.9527037677865,-12.4426568397969,
114.353280501949)) ;
#167852=CARTESIAN_POINT('Ctrl Pts',(-22.0265076107875,-12.4426568403884,
114.329049458987)) ;
#167853=CARTESIAN_POINT('Ctrl Pts',(-22.0200535960851,-12.3696269973012,
114.309391571583)) ;
#167854=CARTESIAN_POINT('Ctrl Pts',(-22.0135995813828,-12.2965971542141,
114.289733684178)) ;
#167855=CARTESIAN_POINT('Ctrl Pts',(-21.9397957383818,-12.2965971536226,
114.31396472714)) ;
#167856=CARTESIAN_POINT('Ctrl Pts',(-21.8659918953808,-12.2965971530311,
114.338195770102)) ;
#167857=CARTESIAN_POINT('Ctrl Pts',(-21.8724459100831,-12.3696269961183,
114.357853657507)) ;
#167858=CARTESIAN_POINT('Ctrl Pts',(-21.9730577437289,-12.3300023799241,
114.628793507168)) ;
#167859=CARTESIAN_POINT('Ctrl Pts',(-21.973230577012,-12.4059080645877,
114.629319929397)) ;
#167860=CARTESIAN_POINT('Ctrl Pts',(-22.0470344193771,-12.4059080646803,
114.605088884498)) ;
#167861=CARTESIAN_POINT('Ctrl Pts',(-22.1208382617422,-12.4059080647729,
114.580857839599)) ;
#167862=CARTESIAN_POINT('Ctrl Pts',(-22.1206654284592,-12.3300023801093,
114.58033141737)) ;
#167863=CARTESIAN_POINT('Ctrl Pts',(-22.120492595176,-12.2540966954457,
114.579804995141)) ;
#167864=CARTESIAN_POINT('Ctrl Pts',(-22.0466887528109,-12.2540966953531,
114.60403604004)) ;
#167865=CARTESIAN_POINT('Ctrl Pts',(-21.9728849104458,-12.2540966952605,
114.628267084938)) ;
#167866=CARTESIAN_POINT('Ctrl Pts',(-21.9730577437289,-12.3300023799241,
114.628793507168)) ;
#167867=CARTESIAN_POINT('Ctrl Pts',(-22.0736203367957,-12.3684199778557,
114.899625493982)) ;
#167868=CARTESIAN_POINT('Ctrl Pts',(-22.0675051364082,-12.4417552779972,
114.88099958023)) ;
#167869=CARTESIAN_POINT('Ctrl Pts',(-22.1413089789616,-12.4417552770606,
114.856768535904)) ;
#167870=CARTESIAN_POINT('Ctrl Pts',(-22.215112821515,-12.441755276124,114.832537491579)) ;
#167871=CARTESIAN_POINT('Ctrl Pts',(-22.2212280219025,-12.3684199759825,
114.851163405331)) ;
#167872=CARTESIAN_POINT('Ctrl Pts',(-22.2273432222899,-12.2950846758409,
114.869789319083)) ;
#167873=CARTESIAN_POINT('Ctrl Pts',(-22.1535393797365,-12.2950846767775,
114.894020363408)) ;
#167874=CARTESIAN_POINT('Ctrl Pts',(-22.0797355371831,-12.2950846777141,
114.918251407734)) ;
#167875=CARTESIAN_POINT('Ctrl Pts',(-22.0736203367957,-12.3684199778557,
114.899625493982)) ;
#167876=CARTESIAN_POINT('Ctrl Pts',(-22.168037726153,-12.4825669571575,
115.151626856521)) ;
#167877=CARTESIAN_POINT('Ctrl Pts',(-22.1560567891196,-12.5480396537864,
115.115134855438)) ;
#167878=CARTESIAN_POINT('Ctrl Pts',(-22.2298606326288,-12.5480396536061,
115.090903814024)) ;
#167879=CARTESIAN_POINT('Ctrl Pts',(-22.303664476138,-12.5480396534258,
115.06667277261)) ;
#167880=CARTESIAN_POINT('Ctrl Pts',(-22.3156454131713,-12.4825669567968,
115.103164773693)) ;
#167881=CARTESIAN_POINT('Ctrl Pts',(-22.3276263502047,-12.4170942601679,
115.139656774775)) ;
#167882=CARTESIAN_POINT('Ctrl Pts',(-22.2538225066955,-12.4170942603482,
115.163887816189)) ;
#167883=CARTESIAN_POINT('Ctrl Pts',(-22.1800186631863,-12.4170942605285,
115.188118857604)) ;
#167884=CARTESIAN_POINT('Ctrl Pts',(-22.168037726153,-12.4825669571575,
115.151626856521)) ;
#167885=CARTESIAN_POINT('Ctrl Pts',(-22.2495860805879,-12.6630281231511,
115.364618342181)) ;
#167886=CARTESIAN_POINT('Ctrl Pts',(-22.2326259100458,-12.7159956192618,
115.312960399306)) ;
#167887=CARTESIAN_POINT('Ctrl Pts',(-22.3064297544898,-12.7159956220205,
115.288729360739)) ;
#167888=CARTESIAN_POINT('Ctrl Pts',(-22.3802335989338,-12.7159956247792,
115.264498322172)) ;
#167889=CARTESIAN_POINT('Ctrl Pts',(-22.3971937694758,-12.6630281286685,
115.316156265047)) ;
#167890=CARTESIAN_POINT('Ctrl Pts',(-22.4141539400179,-12.6100606325577,
115.367814207921)) ;
#167891=CARTESIAN_POINT('Ctrl Pts',(-22.3403500955739,-12.610060629799,
115.392045246488)) ;
#167892=CARTESIAN_POINT('Ctrl Pts',(-22.2665462511299,-12.6100606270403,
115.416276285055)) ;
#167893=CARTESIAN_POINT('Ctrl Pts',(-22.2495860805879,-12.6630281231511,
115.364618342181)) ;
#167894=CARTESIAN_POINT('Ctrl Pts',(-22.3138854050452,-12.898267035054,
115.524940420666)) ;
#167895=CARTESIAN_POINT('Ctrl Pts',(-22.293145904255,-12.9348862826856,
115.461771247767)) ;
#167896=CARTESIAN_POINT('Ctrl Pts',(-22.3669497493675,-12.9348862916205,
115.437540211236)) ;
#167897=CARTESIAN_POINT('Ctrl Pts',(-22.44075359448,-12.9348863005553,115.413309174706)) ;
#167898=CARTESIAN_POINT('Ctrl Pts',(-22.4614930952703,-12.8982670529237,
115.476478347604)) ;
#167899=CARTESIAN_POINT('Ctrl Pts',(-22.4822325960606,-12.8616478052921,
115.539647520503)) ;
#167900=CARTESIAN_POINT('Ctrl Pts',(-22.4084287509481,-12.8616477963572,
115.563878557034)) ;
#167901=CARTESIAN_POINT('Ctrl Pts',(-22.3346249058356,-12.8616477874224,
115.588109593565)) ;
#167902=CARTESIAN_POINT('Ctrl Pts',(-22.3138854050452,-12.898267035054,
115.524940420666)) ;
#167903=CARTESIAN_POINT('Ctrl Pts',(-22.3565804412161,-13.1692444185093,
115.619663390432)) ;
#167904=CARTESIAN_POINT('Ctrl Pts',(-22.3335607360355,-13.1869963126333,
115.549549082981)) ;
#167905=CARTESIAN_POINT('Ctrl Pts',(-22.4073645807767,-13.186996328282,
115.525318045319)) ;
#167906=CARTESIAN_POINT('Ctrl Pts',(-22.4811684255178,-13.1869963439306,
115.501087007657)) ;
#167907=CARTESIAN_POINT('Ctrl Pts',(-22.5041881306984,-13.1692444498067,
115.571201315108)) ;
#167908=CARTESIAN_POINT('Ctrl Pts',(-22.527207835879,-13.1514925556827,
115.641315622559)) ;
#167909=CARTESIAN_POINT('Ctrl Pts',(-22.4534039911379,-13.1514925400341,
115.665546660221)) ;
#167910=CARTESIAN_POINT('Ctrl Pts',(-22.3796001463967,-13.1514925243854,
115.689777697883)) ;
#167911=CARTESIAN_POINT('Ctrl Pts',(-22.3565804412161,-13.1692444185093,
115.619663390432)) ;
#167912=CARTESIAN_POINT('Ctrl Pts',(-22.3758900582822,-13.4593682561925,
115.642974281355)) ;
#167913=CARTESIAN_POINT('Ctrl Pts',(-22.3522233784854,-13.4568887930797,
115.570889393765)) ;
#167914=CARTESIAN_POINT('Ctrl Pts',(-22.4260272218503,-13.4568888172156,
115.546658351912)) ;
#167915=CARTESIAN_POINT('Ctrl Pts',(-22.4998310652151,-13.4568888413516,
115.522427310058)) ;
#167916=CARTESIAN_POINT('Ctrl Pts',(-22.5234977450119,-13.4593683044645,
115.594512197648)) ;
#167917=CARTESIAN_POINT('Ctrl Pts',(-22.5471644248086,-13.4618477675773,
115.666597085238)) ;
#167918=CARTESIAN_POINT('Ctrl Pts',(-22.4733605814438,-13.4618477434414,
115.690828127091)) ;
#167919=CARTESIAN_POINT('Ctrl Pts',(-22.399556738079,-13.4618477193054,
115.715059168945)) ;
#167920=CARTESIAN_POINT('Ctrl Pts',(-22.3758900582822,-13.4593682561925,
115.642974281355)) ;
#167921=CARTESIAN_POINT('Ctrl Pts',(-22.3707818364666,-13.7466998259824,
115.591894004533)) ;
#167922=CARTESIAN_POINT('Ctrl Pts',(-22.3481725681148,-13.7241548771273,
115.523029821762)) ;
#167923=CARTESIAN_POINT('Ctrl Pts',(-22.4219764086385,-13.7241549087659,
115.498798771254)) ;
#167924=CARTESIAN_POINT('Ctrl Pts',(-22.4957802491622,-13.7241549404046,
115.474567720747)) ;
#167925=CARTESIAN_POINT('Ctrl Pts',(-22.5183895175141,-13.7466998892598,
115.543431903518)) ;
#167926=CARTESIAN_POINT('Ctrl Pts',(-22.5409987858659,-13.7692448381149,
115.612296086289)) ;
#167927=CARTESIAN_POINT('Ctrl Pts',(-22.4671949453422,-13.7692448064763,
115.636527136796)) ;
#167928=CARTESIAN_POINT('Ctrl Pts',(-22.3933911048185,-13.7692447748376,
115.660758187303)) ;
#167929=CARTESIAN_POINT('Ctrl Pts',(-22.3707818364666,-13.7466998259824,
115.591894004533)) ;
#167930=CARTESIAN_POINT('Ctrl Pts',(-22.3425575296485,-14.0096322945866,
115.470512365556)) ;
#167931=CARTESIAN_POINT('Ctrl Pts',(-22.3226190812992,-13.9686968355008,
115.409783069735)) ;
#167932=CARTESIAN_POINT('Ctrl Pts',(-22.396422917929,-13.9686968703367,
115.385552007367)) ;
#167933=CARTESIAN_POINT('Ctrl Pts',(-22.4702267545589,-13.9686969051726,
115.361320945)) ;
#167934=CARTESIAN_POINT('Ctrl Pts',(-22.4901652029082,-14.0096323642584,
115.422050240821)) ;
#167935=CARTESIAN_POINT('Ctrl Pts',(-22.5101036512575,-14.0505678233442,
115.482779536643)) ;
#167936=CARTESIAN_POINT('Ctrl Pts',(-22.4362998146277,-14.0505677885083,
115.50701059901)) ;
#167937=CARTESIAN_POINT('Ctrl Pts',(-22.3624959779978,-14.0505677536723,
115.531241661378)) ;
#167938=CARTESIAN_POINT('Ctrl Pts',(-22.3425575296485,-14.0096322945866,
115.470512365556)) ;
#167939=CARTESIAN_POINT('Ctrl Pts',(-22.2939191122543,-14.2308164989726,
115.286886571348)) ;
#167940=CARTESIAN_POINT('Ctrl Pts',(-22.2780819245253,-14.1743789457168,
115.238649053812)) ;
#167941=CARTESIAN_POINT('Ctrl Pts',(-22.3518857564706,-14.1743789796015,
115.214417977176)) ;
#167942=CARTESIAN_POINT('Ctrl Pts',(-22.4256895884157,-14.1743790134861,
115.19018690054)) ;
#167943=CARTESIAN_POINT('Ctrl Pts',(-22.4415267761447,-14.2308165667419,
115.238424418076)) ;
#167944=CARTESIAN_POINT('Ctrl Pts',(-22.4573639638737,-14.2872541199976,
115.286661935612)) ;
#167945=CARTESIAN_POINT('Ctrl Pts',(-22.3835601319285,-14.287254086113,
115.310893012248)) ;
#167946=CARTESIAN_POINT('Ctrl Pts',(-22.3097562999833,-14.2872540522283,
115.335124088884)) ;
#167947=CARTESIAN_POINT('Ctrl Pts',(-22.2939191122543,-14.2308164989726,
115.286886571348)) ;
#167948=CARTESIAN_POINT('Ctrl Pts',(-22.2288101941412,-14.3939170940553,
115.052972439355)) ;
#167949=CARTESIAN_POINT('Ctrl Pts',(-22.2182325563075,-14.3260101541607,
115.020754662367)) ;
#167950=CARTESIAN_POINT('Ctrl Pts',(-22.2920363830491,-14.3260101812409,
114.996523569882)) ;
#167951=CARTESIAN_POINT('Ctrl Pts',(-22.3658402097907,-14.3260102083211,
114.972292477396)) ;
#167952=CARTESIAN_POINT('Ctrl Pts',(-22.3764178476244,-14.3939171482158,
115.004510254384)) ;
#167953=CARTESIAN_POINT('Ctrl Pts',(-22.386995485458,-14.4618240881105,
115.036728031371)) ;
#167954=CARTESIAN_POINT('Ctrl Pts',(-22.3131916587164,-14.4618240610302,
115.060959123857)) ;
#167955=CARTESIAN_POINT('Ctrl Pts',(-22.2393878319748,-14.46182403395,115.085190216342)) ;
#167956=CARTESIAN_POINT('Ctrl Pts',(-22.2288101941412,-14.3939170940553,
115.052972439355)) ;
#167957=CARTESIAN_POINT('Ctrl Pts',(-22.1536104156,-14.4862563732453,114.788647345672)) ;
#167958=CARTESIAN_POINT('Ctrl Pts',(-22.1489978393131,-14.411804800515,
114.774598183824)) ;
#167959=CARTESIAN_POINT('Ctrl Pts',(-22.2228016623764,-14.4118048137988,
114.750367080135)) ;
#167960=CARTESIAN_POINT('Ctrl Pts',(-22.2966054854396,-14.4118048270827,
114.726135976446)) ;
#167961=CARTESIAN_POINT('Ctrl Pts',(-22.3012180617265,-14.486256399813,
114.740185138294)) ;
#167962=CARTESIAN_POINT('Ctrl Pts',(-22.3058306380133,-14.5607079725433,
114.754234300141)) ;
#167963=CARTESIAN_POINT('Ctrl Pts',(-22.2320268149501,-14.5607079592595,
114.77846540383)) ;
#167964=CARTESIAN_POINT('Ctrl Pts',(-22.1582229918869,-14.5607079459756,
114.802696507519)) ;
#167965=CARTESIAN_POINT('Ctrl Pts',(-22.1536104156,-14.4862563732453,114.788647345672)) ;
#167966=CARTESIAN_POINT('Ctrl Pts',(-22.0731223082853,-14.5025873133897,
114.507882396618)) ;
#167967=CARTESIAN_POINT('Ctrl Pts',(-22.0748593506673,-14.4268872889833,
114.513173148907)) ;
#167968=CARTESIAN_POINT('Ctrl Pts',(-22.1486631705148,-14.4268872836565,
114.488942035423)) ;
#167969=CARTESIAN_POINT('Ctrl Pts',(-22.2224669903623,-14.4268872783298,
114.464710921939)) ;
#167970=CARTESIAN_POINT('Ctrl Pts',(-22.2207299479803,-14.5025873027362,
114.45942016965)) ;
#167971=CARTESIAN_POINT('Ctrl Pts',(-22.2189929055983,-14.5782873271426,
114.454129417361)) ;
#167972=CARTESIAN_POINT('Ctrl Pts',(-22.1451890857508,-14.5782873324694,
114.478360530845)) ;
#167973=CARTESIAN_POINT('Ctrl Pts',(-22.0713852659033,-14.5782873377961,
114.502591644329)) ;
#167974=CARTESIAN_POINT('Ctrl Pts',(-22.0731223082853,-14.5025873133897,
114.507882396618)) ;
#167975=CARTESIAN_POINT('Ctrl Pts',(-21.9952150839896,-14.4415569455837,
114.235304068453)) ;
#167976=CARTESIAN_POINT('Ctrl Pts',(-22.0031240160095,-14.3700086479268,
114.259393400862)) ;
#167977=CARTESIAN_POINT('Ctrl Pts',(-22.0769278353894,-14.370008620797,
114.235162285954)) ;
#167978=CARTESIAN_POINT('Ctrl Pts',(-22.1507316547692,-14.3700085936673,
114.210931171046)) ;
#167979=CARTESIAN_POINT('Ctrl Pts',(-22.1428227227493,-14.4415568913242,
114.186841838637)) ;
#167980=CARTESIAN_POINT('Ctrl Pts',(-22.1349137907294,-14.5131051889812,
114.162752506228)) ;
#167981=CARTESIAN_POINT('Ctrl Pts',(-22.0611099713496,-14.5131052161109,
114.186983621136)) ;
#167982=CARTESIAN_POINT('Ctrl Pts',(-21.9873061519697,-14.5131052432407,
114.211214736044)) ;
#167983=CARTESIAN_POINT('Ctrl Pts',(-21.9952150839896,-14.4415569455837,
114.235304068453)) ;
#167984=CARTESIAN_POINT('Ctrl Pts',(-21.9247229138988,-14.3059463498269,
113.984884763739)) ;
#167985=CARTESIAN_POINT('Ctrl Pts',(-21.9383038334394,-14.2437611215803,
114.026250055128)) ;
#167986=CARTESIAN_POINT('Ctrl Pts',(-22.0121076538114,-14.2437610699902,
114.002018943242)) ;
#167987=CARTESIAN_POINT('Ctrl Pts',(-22.0859114741834,-14.2437610184,113.977787831356)) ;
#167988=CARTESIAN_POINT('Ctrl Pts',(-22.0723305546428,-14.3059462466466,
113.936422539967)) ;
#167989=CARTESIAN_POINT('Ctrl Pts',(-22.0587496351021,-14.3681314748932,
113.895057248578)) ;
#167990=CARTESIAN_POINT('Ctrl Pts',(-21.9849458147301,-14.3681315264833,
113.919288360464)) ;
#167991=CARTESIAN_POINT('Ctrl Pts',(-21.9111419943582,-14.3681315780735,
113.94351947235)) ;
#167992=CARTESIAN_POINT('Ctrl Pts',(-21.9247229138988,-14.3059463498269,
113.984884763739)) ;
#167993=CARTESIAN_POINT('Ctrl Pts',(-21.8690302313287,-14.1081523204692,
113.779936751177)) ;
#167994=CARTESIAN_POINT('Ctrl Pts',(-21.8872499276746,-14.0596861997997,
113.835431008341)) ;
#167995=CARTESIAN_POINT('Ctrl Pts',(-21.9610537522494,-14.0596861267513,
113.811199909255)) ;
#167996=CARTESIAN_POINT('Ctrl Pts',(-22.0348575768242,-14.059686053703,
113.78696881017)) ;
#167997=CARTESIAN_POINT('Ctrl Pts',(-22.0166378804783,-14.1081521743725,
113.731474553006)) ;
#167998=CARTESIAN_POINT('Ctrl Pts',(-21.9984181841324,-14.1566182950421,
113.675980295843)) ;
#167999=CARTESIAN_POINT('Ctrl Pts',(-21.9246143595576,-14.1566183680904,
113.700211394928)) ;
#168000=CARTESIAN_POINT('Ctrl Pts',(-21.8508105349828,-14.1566184411388,
113.724442494013)) ;
#168001=CARTESIAN_POINT('Ctrl Pts',(-21.8690302313287,-14.1081523204692,
113.779936751177)) ;
#168002=CARTESIAN_POINT('Ctrl Pts',(-21.8317929609378,-13.8605107481474,
113.631055122176)) ;
#168003=CARTESIAN_POINT('Ctrl Pts',(-21.8533727983839,-13.8292631951763,
113.69678382707)) ;
#168004=CARTESIAN_POINT('Ctrl Pts',(-21.9271766290347,-13.8292631042665,
113.672552746491)) ;
#168005=CARTESIAN_POINT('Ctrl Pts',(-22.0009804596855,-13.8292630133566,
113.648321665912)) ;
#168006=CARTESIAN_POINT('Ctrl Pts',(-21.9794006222394,-13.8605105663277,
113.582592961019)) ;
#168007=CARTESIAN_POINT('Ctrl Pts',(-21.9578207847933,-13.8917581192987,
113.516864256125)) ;
#168008=CARTESIAN_POINT('Ctrl Pts',(-21.8840169541425,-13.8917582102086,
113.541095336704)) ;
#168009=CARTESIAN_POINT('Ctrl Pts',(-21.8102131234917,-13.8917583011184,
113.565326417282)) ;
#168010=CARTESIAN_POINT('Ctrl Pts',(-21.8317929609378,-13.8605107481474,
113.631055122176)) ;
#168011=CARTESIAN_POINT('Ctrl Pts',(-21.8167817419917,-13.5802159839548,
113.549772204603)) ;
#168012=CARTESIAN_POINT('Ctrl Pts',(-21.840177115245,-13.5684914929652,
113.621030738711)) ;
#168013=CARTESIAN_POINT('Ctrl Pts',(-21.9139809537407,-13.5684913902422,
113.596799682027)) ;
#168014=CARTESIAN_POINT('Ctrl Pts',(-21.9877847922365,-13.5684912875191,
113.572568625343)) ;
#168015=CARTESIAN_POINT('Ctrl Pts',(-21.9643894189832,-13.5802157785087,
113.501310091235)) ;
#168016=CARTESIAN_POINT('Ctrl Pts',(-21.94099404573,-13.5919402694983,113.430051557127)) ;
#168017=CARTESIAN_POINT('Ctrl Pts',(-21.8671902072343,-13.5919403722214,
113.454282613811)) ;
#168018=CARTESIAN_POINT('Ctrl Pts',(-21.7933863687385,-13.5919404749444,
113.478513670495)) ;
#168019=CARTESIAN_POINT('Ctrl Pts',(-21.8167817419917,-13.5802159839548,
113.549772204603)) ;
#168020=CARTESIAN_POINT('Ctrl Pts',(-21.8259670175883,-13.2888355614903,
113.542253086016)) ;
#168021=CARTESIAN_POINT('Ctrl Pts',(-21.8494900051154,-13.2974368879024,
113.613900312663)) ;
#168022=CARTESIAN_POINT('Ctrl Pts',(-21.9232938524342,-13.2974367821204,
113.589669282852)) ;
#168023=CARTESIAN_POINT('Ctrl Pts',(-21.997097699753,-13.2974366763383,
113.565438253042)) ;
#168024=CARTESIAN_POINT('Ctrl Pts',(-21.973574712226,-13.2888353499262,
113.493791026395)) ;
#168025=CARTESIAN_POINT('Ctrl Pts',(-21.9500517246989,-13.2802340235141,
113.422143799749)) ;
#168026=CARTESIAN_POINT('Ctrl Pts',(-21.87624787738,-13.2802341292962,113.446374829559)) ;
#168027=CARTESIAN_POINT('Ctrl Pts',(-21.8024440300612,-13.2802342350782,
113.47060585937)) ;
#168028=CARTESIAN_POINT('Ctrl Pts',(-21.8259670175883,-13.2888355614903,
113.542253086016)) ;
#168029=CARTESIAN_POINT('Ctrl Pts',(-21.8589580647777,-13.0084923611293,
113.607479583454)) ;
#168030=CARTESIAN_POINT('Ctrl Pts',(-21.8809417628856,-13.0366789477102,
113.674438382918)) ;
#168031=CARTESIAN_POINT('Ctrl Pts',(-21.9547456189426,-13.0366788478173,
113.650207379723)) ;
#168032=CARTESIAN_POINT('Ctrl Pts',(-22.0285494749996,-13.0366787479245,
113.625976376527)) ;
#168033=CARTESIAN_POINT('Ctrl Pts',(-22.0065657768918,-13.0084921613435,
113.559017577064)) ;
#168034=CARTESIAN_POINT('Ctrl Pts',(-21.9845820787839,-12.9803055747626,
113.4920587776)) ;
#168035=CARTESIAN_POINT('Ctrl Pts',(-21.9107782227269,-12.9803056746555,
113.516289780796)) ;
#168036=CARTESIAN_POINT('Ctrl Pts',(-21.8369743666699,-12.9803057745484,
113.540520783991)) ;
#168037=CARTESIAN_POINT('Ctrl Pts',(-21.8589580647777,-13.0084923611293,
113.607479583454)) ;
#168038=CARTESIAN_POINT('Ctrl Pts',(-21.9147410221325,-12.7552927085919,
113.741839536219)) ;
#168039=CARTESIAN_POINT('Ctrl Pts',(-21.9335982548626,-12.8011984065865,
113.799275626608)) ;
#168040=CARTESIAN_POINT('Ctrl Pts',(-22.0074021188863,-12.8011983205869,
113.775044647678)) ;
#168041=CARTESIAN_POINT('Ctrl Pts',(-22.0812059829101,-12.8011982345872,
113.750813668748)) ;
#168042=CARTESIAN_POINT('Ctrl Pts',(-22.06234875018,-12.7552925365926,113.693377578359)) ;
#168043=CARTESIAN_POINT('Ctrl Pts',(-22.0434915174499,-12.709386838598,
113.635941487971)) ;
#168044=CARTESIAN_POINT('Ctrl Pts',(-21.9696876534261,-12.7093869245976,
113.660172466901)) ;
#168045=CARTESIAN_POINT('Ctrl Pts',(-21.8958837894024,-12.7093870105973,
113.68440344583)) ;
#168046=CARTESIAN_POINT('Ctrl Pts',(-21.9147410221325,-12.7552927085919,
113.741839536219)) ;
#168047=CARTESIAN_POINT('Ctrl Pts',(-21.9895561849059,-12.5504983058309,
113.934322640531)) ;
#168048=CARTESIAN_POINT('Ctrl Pts',(-22.0039503096504,-12.6107700146374,
113.978164824106)) ;
#168049=CARTESIAN_POINT('Ctrl Pts',(-22.0777541799352,-12.6107699496328,
113.953933864246)) ;
#168050=CARTESIAN_POINT('Ctrl Pts',(-22.1515580502199,-12.6107698846282,
113.929702904386)) ;
#168051=CARTESIAN_POINT('Ctrl Pts',(-22.1371639254754,-12.5504981758217,
113.885860720812)) ;
#168052=CARTESIAN_POINT('Ctrl Pts',(-22.1227698007308,-12.4902264670152,
113.842018537237)) ;
#168053=CARTESIAN_POINT('Ctrl Pts',(-22.048965930446,-12.4902265320198,
113.866249497097)) ;
#168054=CARTESIAN_POINT('Ctrl Pts',(-21.9751620601613,-12.4902265970244,
113.890480456957)) ;
#168055=CARTESIAN_POINT('Ctrl Pts',(-21.9895561849059,-12.5504983058309,
113.934322640531)) ;
#168056=CARTESIAN_POINT('Ctrl Pts',(-22.0795106288401,-12.4070470358761,
114.17271722211)) ;
#168057=CARTESIAN_POINT('Ctrl Pts',(-22.0883824289903,-12.477423987992,
114.199739295954)) ;
#168058=CARTESIAN_POINT('Ctrl Pts',(-22.1621863031239,-12.4774239490789,
114.175508347817)) ;
#168059=CARTESIAN_POINT('Ctrl Pts',(-22.2359901772575,-12.4774239101657,
114.15127739968)) ;
#168060=CARTESIAN_POINT('Ctrl Pts',(-22.2271183771075,-12.4070469580498,
114.124255325836)) ;
#168061=CARTESIAN_POINT('Ctrl Pts',(-22.2182465769573,-12.336670005934,
114.097233251992)) ;
#168062=CARTESIAN_POINT('Ctrl Pts',(-22.1444427028237,-12.3366700448471,
114.121464200129)) ;
#168063=CARTESIAN_POINT('Ctrl Pts',(-22.07063882869,-12.3366700837602,114.145695148265)) ;
#168064=CARTESIAN_POINT('Ctrl Pts',(-22.0795106288401,-12.4070470358761,
114.17271722211)) ;
#168065=CARTESIAN_POINT('Ctrl Pts',(-22.1777882055102,-12.336806735375,
114.436722224739)) ;
#168066=CARTESIAN_POINT('Ctrl Pts',(-22.180542808377,-12.4121923869935,
114.445112302616)) ;
#168067=CARTESIAN_POINT('Ctrl Pts',(-22.2543466838533,-12.4121923758419,
114.420881358569)) ;
#168068=CARTESIAN_POINT('Ctrl Pts',(-22.3281505593297,-12.4121923646903,
114.396650414522)) ;
#168069=CARTESIAN_POINT('Ctrl Pts',(-22.325395956463,-12.3368067130718,
114.388260336645)) ;
#168070=CARTESIAN_POINT('Ctrl Pts',(-22.3226413535963,-12.2614210614532,
114.379870258768)) ;
#168071=CARTESIAN_POINT('Ctrl Pts',(-22.2488374781199,-12.2614210726048,
114.404101202815)) ;
#168072=CARTESIAN_POINT('Ctrl Pts',(-22.1750336026435,-12.2614210837564,
114.428332146862)) ;
#168073=CARTESIAN_POINT('Ctrl Pts',(-22.1777882055102,-12.336806735375,
114.436722224739)) ;
#168074=CARTESIAN_POINT('Ctrl Pts',(-22.2791750260875,-12.343454815208,
114.710038652952)) ;
#168075=CARTESIAN_POINT('Ctrl Pts',(-22.2755896110811,-12.4184892364302,
114.69911805927)) ;
#168076=CARTESIAN_POINT('Ctrl Pts',(-22.3493934851188,-12.4184892524871,
114.674887110841)) ;
#168077=CARTESIAN_POINT('Ctrl Pts',(-22.4231973591565,-12.418489268544,
114.650656162412)) ;
#168078=CARTESIAN_POINT('Ctrl Pts',(-22.4267827741629,-12.3434548473218,
114.661576756094)) ;
#168079=CARTESIAN_POINT('Ctrl Pts',(-22.4303681891693,-12.2684204260996,
114.672497349776)) ;
#168080=CARTESIAN_POINT('Ctrl Pts',(-22.3565643151316,-12.2684204100427,
114.696728298206)) ;
#168081=CARTESIAN_POINT('Ctrl Pts',(-22.282760441094,-12.2684203939858,
114.720959246635)) ;
#168082=CARTESIAN_POINT('Ctrl Pts',(-22.2791750260875,-12.343454815208,
114.710038652952)) ;
#168083=CARTESIAN_POINT('Ctrl Pts',(-22.3767867804856,-12.4274004694333,
114.971842801054)) ;
#168084=CARTESIAN_POINT('Ctrl Pts',(-22.3671156303644,-12.4966868092395,
114.942386040042)) ;
#168085=CARTESIAN_POINT('Ctrl Pts',(-22.4409195004905,-12.4966868487172,
114.918155079699)) ;
#168086=CARTESIAN_POINT('Ctrl Pts',(-22.5147233706166,-12.496686888195,
114.893924119355)) ;
#168087=CARTESIAN_POINT('Ctrl Pts',(-22.5243945207378,-12.4274005483888,
114.923380880368)) ;
#168088=CARTESIAN_POINT('Ctrl Pts',(-22.534065670859,-12.3581142085826,
114.95283764138)) ;
#168089=CARTESIAN_POINT('Ctrl Pts',(-22.460261800733,-12.3581141691049,
114.977068601723)) ;
#168090=CARTESIAN_POINT('Ctrl Pts',(-22.3864579306068,-12.3581141296271,
115.001299562066)) ;
#168091=CARTESIAN_POINT('Ctrl Pts',(-22.3767867804856,-12.4274004694333,
114.971842801054)) ;
#168092=CARTESIAN_POINT('Ctrl Pts',(-22.4641882116034,-12.5821548538746,
115.202603030469)) ;
#168093=CARTESIAN_POINT('Ctrl Pts',(-22.4491338350531,-12.6407407748519,
115.156749830222)) ;
#168094=CARTESIAN_POINT('Ctrl Pts',(-22.5229376995646,-12.6407408319528,
115.132518852778)) ;
#168095=CARTESIAN_POINT('Ctrl Pts',(-22.5967415640761,-12.6407408890538,
115.108287875333)) ;
#168096=CARTESIAN_POINT('Ctrl Pts',(-22.6117959406265,-12.5821549680765,
115.15414107558)) ;
#168097=CARTESIAN_POINT('Ctrl Pts',(-22.6268503171768,-12.5235690470992,
115.199994275827)) ;
#168098=CARTESIAN_POINT('Ctrl Pts',(-22.5530464526653,-12.5235689899983,
115.224225253271)) ;
#168099=CARTESIAN_POINT('Ctrl Pts',(-22.4792425881538,-12.5235689328973,
115.248456230715)) ;
#168100=CARTESIAN_POINT('Ctrl Pts',(-22.4641882116034,-12.5821548538746,
115.202603030469)) ;
#168101=CARTESIAN_POINT('Ctrl Pts',(-22.5360152755925,-12.7965584285917,
115.385946401626)) ;
#168102=CARTESIAN_POINT('Ctrl Pts',(-22.5166564652332,-12.8402632676504,
115.326982590391)) ;
#168103=CARTESIAN_POINT('Ctrl Pts',(-22.5904603231125,-12.8402633354297,
115.302751592746)) ;
#168104=CARTESIAN_POINT('Ctrl Pts',(-22.6642641809918,-12.8402634032089,
115.278520595101)) ;
#168105=CARTESIAN_POINT('Ctrl Pts',(-22.683622991351,-12.7965585641502,
115.337484406336)) ;
#168106=CARTESIAN_POINT('Ctrl Pts',(-22.7029818017103,-12.7528537250914,
115.39644821757)) ;
#168107=CARTESIAN_POINT('Ctrl Pts',(-22.6291779438311,-12.7528536573122,
115.420679215215)) ;
#168108=CARTESIAN_POINT('Ctrl Pts',(-22.5553740859518,-12.752853589533,
115.444910212861)) ;
#168109=CARTESIAN_POINT('Ctrl Pts',(-22.5360152755925,-12.7965584285917,
115.385946401626)) ;
#168110=CARTESIAN_POINT('Ctrl Pts',(-22.587997010465,-13.0557769277784,
115.508794067491)) ;
#168111=CARTESIAN_POINT('Ctrl Pts',(-22.5657137741848,-13.0814494476449,
115.440922926611)) ;
#168112=CARTESIAN_POINT('Ctrl Pts',(-22.6395176251257,-13.0814495182785,
115.416691907832)) ;
#168113=CARTESIAN_POINT('Ctrl Pts',(-22.7133214760666,-13.0814495889122,
115.392460889054)) ;
#168114=CARTESIAN_POINT('Ctrl Pts',(-22.7356047123469,-13.0557770690457,
115.460332029934)) ;
#168115=CARTESIAN_POINT('Ctrl Pts',(-22.7578879486272,-13.0301045491793,
115.528203170815)) ;
#168116=CARTESIAN_POINT('Ctrl Pts',(-22.6840840976862,-13.0301044785456,
115.552434189593)) ;
#168117=CARTESIAN_POINT('Ctrl Pts',(-22.6102802467453,-13.030104407912,
115.576665208371)) ;
#168118=CARTESIAN_POINT('Ctrl Pts',(-22.587997010465,-13.0557769277784,
115.508794067491)) ;
#168119=CARTESIAN_POINT('Ctrl Pts',(-22.6170289999404,-13.3412469909538,
115.561709527004)) ;
#168120=CARTESIAN_POINT('Ctrl Pts',(-22.593419786976,-13.3470269436932,
115.489799674927)) ;
#168121=CARTESIAN_POINT('Ctrl Pts',(-22.6672236316055,-13.3470270098198,
115.465568636925)) ;
#168122=CARTESIAN_POINT('Ctrl Pts',(-22.7410274762349,-13.3470270759464,
115.441337598923)) ;
#168123=CARTESIAN_POINT('Ctrl Pts',(-22.7646366891993,-13.341247123207,
115.513247451)) ;
#168124=CARTESIAN_POINT('Ctrl Pts',(-22.7882459021636,-13.3354671704675,
115.585157303077)) ;
#168125=CARTESIAN_POINT('Ctrl Pts',(-22.7144420575342,-13.335467104341,
115.609388341079)) ;
#168126=CARTESIAN_POINT('Ctrl Pts',(-22.6406382129048,-13.3354670382144,
115.633619379081)) ;
#168127=CARTESIAN_POINT('Ctrl Pts',(-22.6170289999404,-13.3412469909538,
115.561709527004)) ;
#168128=CARTESIAN_POINT('Ctrl Pts',(-22.6217619532277,-13.6316256256215,
115.540686913954)) ;
#168129=CARTESIAN_POINT('Ctrl Pts',(-22.5985198370732,-13.6171399155478,
115.469895179372)) ;
#168130=CARTESIAN_POINT('Ctrl Pts',(-22.6723236766946,-13.6171399723523,
115.445664126116)) ;
#168131=CARTESIAN_POINT('Ctrl Pts',(-22.7461275163159,-13.6171400291567,
115.42143307286)) ;
#168132=CARTESIAN_POINT('Ctrl Pts',(-22.7693696324704,-13.6316257392305,
115.492224807443)) ;
#168133=CARTESIAN_POINT('Ctrl Pts',(-22.7926117486249,-13.6461114493042,
115.563016542025)) ;
#168134=CARTESIAN_POINT('Ctrl Pts',(-22.7188079090035,-13.6461113924997,
115.587247595281)) ;
#168135=CARTESIAN_POINT('Ctrl Pts',(-22.6450040693822,-13.6461113356952,
115.611478648537)) ;
#168136=CARTESIAN_POINT('Ctrl Pts',(-22.6217619532277,-13.6316256256215,
115.540686913954)) ;
#168137=CARTESIAN_POINT('Ctrl Pts',(-22.6026935421642,-13.9070076933881,
115.447135113786)) ;
#168138=CARTESIAN_POINT('Ctrl Pts',(-22.5814815681784,-13.8732725053054,
115.382526864519)) ;
#168139=CARTESIAN_POINT('Ctrl Pts',(-22.6552854044309,-13.8732725490148,
115.358295801002)) ;
#168140=CARTESIAN_POINT('Ctrl Pts',(-22.7290892406833,-13.8732725927241,
115.334064737485)) ;
#168141=CARTESIAN_POINT('Ctrl Pts',(-22.7503012146691,-13.9070077808067,
115.398672986752)) ;
#168142=CARTESIAN_POINT('Ctrl Pts',(-22.7715131886548,-13.9407429688894,
115.463281236019)) ;
#168143=CARTESIAN_POINT('Ctrl Pts',(-22.6977093524024,-13.9407429251801,
115.487512299536)) ;
#168144=CARTESIAN_POINT('Ctrl Pts',(-22.6239055161499,-13.9407428814708,
115.511743363053)) ;
#168145=CARTESIAN_POINT('Ctrl Pts',(-22.6026935421642,-13.9070076933881,
115.447135113786)) ;
#168146=CARTESIAN_POINT('Ctrl Pts',(-22.561780007704,-14.1476875757229,
115.286985040181)) ;
#168147=CARTESIAN_POINT('Ctrl Pts',(-22.5441277753165,-14.0970962848469,
115.233219189277)) ;
#168148=CARTESIAN_POINT('Ctrl Pts',(-22.6179316101862,-14.0970963139386,
115.208988121549)) ;
#168149=CARTESIAN_POINT('Ctrl Pts',(-22.691735445056,-14.0970963430303,
115.18475705382)) ;
#168150=CARTESIAN_POINT('Ctrl Pts',(-22.7093876774435,-14.1476876339063,
115.238522904724)) ;
#168151=CARTESIAN_POINT('Ctrl Pts',(-22.7270399098311,-14.1982789247823,
115.292288755627)) ;
#168152=CARTESIAN_POINT('Ctrl Pts',(-22.6532360749613,-14.1982788956906,
115.316519823355)) ;
#168153=CARTESIAN_POINT('Ctrl Pts',(-22.5794322400915,-14.1982788665989,
115.340750891084)) ;
#168154=CARTESIAN_POINT('Ctrl Pts',(-22.561780007704,-14.1476875757229,
115.286985040181)) ;
#168155=CARTESIAN_POINT('Ctrl Pts',(-22.5030326356716,-14.3351652655006,
115.072661970802)) ;
#168156=CARTESIAN_POINT('Ctrl Pts',(-22.4901879000911,-14.2714071859544,
115.033538979335)) ;
#168157=CARTESIAN_POINT('Ctrl Pts',(-22.5639917349384,-14.2714072026928,
115.009307911538)) ;
#168158=CARTESIAN_POINT('Ctrl Pts',(-22.6377955697856,-14.2714072194312,
114.985076843741)) ;
#168159=CARTESIAN_POINT('Ctrl Pts',(-22.6506403053661,-14.3351652989775,
115.024199835208)) ;
#168160=CARTESIAN_POINT('Ctrl Pts',(-22.6634850409466,-14.3989233785238,
115.063322826674)) ;
#168161=CARTESIAN_POINT('Ctrl Pts',(-22.5896812060994,-14.3989233617854,
115.087553894471)) ;
#168162=CARTESIAN_POINT('Ctrl Pts',(-22.5158773712521,-14.3989233450469,
115.111784962268)) ;
#168163=CARTESIAN_POINT('Ctrl Pts',(-22.5030326356716,-14.3351652655006,
115.072661970802)) ;
#168164=CARTESIAN_POINT('Ctrl Pts',(-22.431285724249,-14.4575099619995,
114.818736284685)) ;
#168165=CARTESIAN_POINT('Ctrl Pts',(-22.4241636182106,-14.3851129420045,
114.797043499313)) ;
#168166=CARTESIAN_POINT('Ctrl Pts',(-22.4979674542533,-14.38511294846,114.772812435157)) ;
#168167=CARTESIAN_POINT('Ctrl Pts',(-22.5717712902961,-14.3851129549154,
114.748581371002)) ;
#168168=CARTESIAN_POINT('Ctrl Pts',(-22.5788933963345,-14.4575099749105,
114.770274156374)) ;
#168169=CARTESIAN_POINT('Ctrl Pts',(-22.586015502373,-14.5299069949055,
114.791966941746)) ;
#168170=CARTESIAN_POINT('Ctrl Pts',(-22.5122116663302,-14.52990698845,114.816198005902)) ;
#168171=CARTESIAN_POINT('Ctrl Pts',(-22.4384078302875,-14.5299069819946,
114.840429070058)) ;
#168172=CARTESIAN_POINT('Ctrl Pts',(-22.431285724249,-14.4575099619995,
114.818736284685)) ;
#168173=CARTESIAN_POINT('Ctrl Pts',(-22.3517910412139,-14.5055206620573,
114.54096052116)) ;
#168174=CARTESIAN_POINT('Ctrl Pts',(-22.3509465715137,-14.4296611949973,
114.538388403003)) ;
#168175=CARTESIAN_POINT('Ctrl Pts',(-22.424750410142,-14.4296611947843,
114.514157346723)) ;
#168176=CARTESIAN_POINT('Ctrl Pts',(-22.4985542487703,-14.4296611945714,
114.489926290442)) ;
#168177=CARTESIAN_POINT('Ctrl Pts',(-22.4993987184705,-14.5055206616315,
114.492498408599)) ;
#168178=CARTESIAN_POINT('Ctrl Pts',(-22.5002431881708,-14.5813801286916,
114.495070526755)) ;
#168179=CARTESIAN_POINT('Ctrl Pts',(-22.4264393495425,-14.5813801289045,
114.519301583036)) ;
#168180=CARTESIAN_POINT('Ctrl Pts',(-22.3526355109141,-14.5813801291174,
114.543532639316)) ;
#168181=CARTESIAN_POINT('Ctrl Pts',(-22.3517910412139,-14.5055206620573,
114.54096052116)) ;
#168182=CARTESIAN_POINT('Ctrl Pts',(-22.2722771348599,-14.4754288487564,
114.263452537845)) ;
#168183=CARTESIAN_POINT('Ctrl Pts',(-22.2777143862475,-14.4015565166022,
114.280013528463)) ;
#168184=CARTESIAN_POINT('Ctrl Pts',(-22.3515182267516,-14.4015565138437,
114.255782477895)) ;
#168185=CARTESIAN_POINT('Ctrl Pts',(-22.4253220672556,-14.4015565110851,
114.231551427328)) ;
#168186=CARTESIAN_POINT('Ctrl Pts',(-22.419884815868,-14.4754288432393,
114.214990436711)) ;
#168187=CARTESIAN_POINT('Ctrl Pts',(-22.4144475644804,-14.5493011753935,
114.198429446093)) ;
#168188=CARTESIAN_POINT('Ctrl Pts',(-22.3406437239764,-14.5493011781521,
114.222660496661)) ;
#168189=CARTESIAN_POINT('Ctrl Pts',(-22.2668398834723,-14.5493011809106,
114.246891547228)) ;
#168190=CARTESIAN_POINT('Ctrl Pts',(-22.2722771348599,-14.4754288487564,
114.263452537845)) ;
#168191=CARTESIAN_POINT('Ctrl Pts',(-22.1980599297582,-14.3696969300058,
114.00189324141)) ;
#168192=CARTESIAN_POINT('Ctrl Pts',(-22.2094224709354,-14.3030961668257,
114.036501708568)) ;
#168193=CARTESIAN_POINT('Ctrl Pts',(-22.2832263134077,-14.3030961645972,
114.012270663996)) ;
#168194=CARTESIAN_POINT('Ctrl Pts',(-22.35703015588,-14.3030961623686,113.988039619424)) ;
#168195=CARTESIAN_POINT('Ctrl Pts',(-22.3456676147028,-14.3696969255486,
113.953431152266)) ;
#168196=CARTESIAN_POINT('Ctrl Pts',(-22.3343050735257,-14.4362976887287,
113.918822685108)) ;
#168197=CARTESIAN_POINT('Ctrl Pts',(-22.2605012310534,-14.4362976909572,
113.94305372968)) ;
#168198=CARTESIAN_POINT('Ctrl Pts',(-22.1866973885811,-14.4362976931858,
113.967284774253)) ;
#168199=CARTESIAN_POINT('Ctrl Pts',(-22.1980599297582,-14.3696969300058,
114.00189324141)) ;
#168200=CARTESIAN_POINT('Ctrl Pts',(-22.1356986945465,-14.1954536297215,
113.776452902693)) ;
#168201=CARTESIAN_POINT('Ctrl Pts',(-22.1521674655351,-14.1409200386093,
113.826614121888)) ;
#168202=CARTESIAN_POINT('Ctrl Pts',(-22.2259713091281,-14.1409200387787,
113.802383080729)) ;
#168203=CARTESIAN_POINT('Ctrl Pts',(-22.2997751527211,-14.1409200389481,
113.77815203957)) ;
#168204=CARTESIAN_POINT('Ctrl Pts',(-22.2833063817325,-14.1954536300603,
113.727990820375)) ;
#168205=CARTESIAN_POINT('Ctrl Pts',(-22.266837610744,-14.2499872211724,
113.677829601181)) ;
#168206=CARTESIAN_POINT('Ctrl Pts',(-22.193033767151,-14.249987221003,113.70206064234)) ;
#168207=CARTESIAN_POINT('Ctrl Pts',(-22.119229923558,-14.2499872208336,
113.726291683498)) ;
#168208=CARTESIAN_POINT('Ctrl Pts',(-22.1356986945465,-14.1954536297215,
113.776452902693)) ;
#168209=CARTESIAN_POINT('Ctrl Pts',(-22.0904372209487,-13.9663067477415,
113.603202833569)) ;
#168210=CARTESIAN_POINT('Ctrl Pts',(-22.1108234263171,-13.9276927071092,
113.665295925763)) ;
#168211=CARTESIAN_POINT('Ctrl Pts',(-22.1846272702145,-13.9276927095559,
113.641064885531)) ;
#168212=CARTESIAN_POINT('Ctrl Pts',(-22.2584311141118,-13.9276927120025,
113.6168338453)) ;
#168213=CARTESIAN_POINT('Ctrl Pts',(-22.2380449087434,-13.9663067526349,
113.554740753105)) ;
#168214=CARTESIAN_POINT('Ctrl Pts',(-22.217658703375,-14.0049207932672,
113.492647660911)) ;
#168215=CARTESIAN_POINT('Ctrl Pts',(-22.1438548594777,-14.0049207908205,
113.516878701143)) ;
#168216=CARTESIAN_POINT('Ctrl Pts',(-22.0700510155803,-14.0049207883739,
113.541109741375)) ;
#168217=CARTESIAN_POINT('Ctrl Pts',(-22.0904372209487,-13.9663067477415,
113.603202833569)) ;
#168218=CARTESIAN_POINT('Ctrl Pts',(-22.0660586940401,-13.6964880977043,
113.493367442293)) ;
#168219=CARTESIAN_POINT('Ctrl Pts',(-22.088914009386,-13.6766583743927,
113.562981045083)) ;
#168220=CARTESIAN_POINT('Ctrl Pts',(-22.1627178530358,-13.6766583775101,
113.538750004097)) ;
#168221=CARTESIAN_POINT('Ctrl Pts',(-22.2365216966856,-13.6766583806274,
113.514518963111)) ;
#168222=CARTESIAN_POINT('Ctrl Pts',(-22.2136663813398,-13.696488103939,
113.444905360321)) ;
#168223=CARTESIAN_POINT('Ctrl Pts',(-22.1908110659939,-13.7163178272505,
113.375291757531)) ;
#168224=CARTESIAN_POINT('Ctrl Pts',(-22.1170072223441,-13.7163178241332,
113.399522798517)) ;
#168225=CARTESIAN_POINT('Ctrl Pts',(-22.0432033786943,-13.7163178210159,
113.423753839503)) ;
#168226=CARTESIAN_POINT('Ctrl Pts',(-22.0660586940401,-13.6964880977043,
113.493367442293)) ;
#168227=CARTESIAN_POINT('Ctrl Pts',(-22.0652380838038,-13.4086720240795,
113.455542704925)) ;
#168228=CARTESIAN_POINT('Ctrl Pts',(-22.0889152773064,-13.4089104896533,
113.527659616002)) ;
#168229=CARTESIAN_POINT('Ctrl Pts',(-22.1627191206271,-13.4089104912241,
113.503428574014)) ;
#168230=CARTESIAN_POINT('Ctrl Pts',(-22.2365229639478,-13.408910492795,
113.479197532026)) ;
#168231=CARTESIAN_POINT('Ctrl Pts',(-22.2128457704452,-13.4086720272212,
113.407080620949)) ;
#168232=CARTESIAN_POINT('Ctrl Pts',(-22.1891685769426,-13.4084335616475,
113.334963709871)) ;
#168233=CARTESIAN_POINT('Ctrl Pts',(-22.1153647336219,-13.4084335600766,
113.359194751859)) ;
#168234=CARTESIAN_POINT('Ctrl Pts',(-22.0415608903012,-13.4084335585058,
113.383425793848)) ;
#168235=CARTESIAN_POINT('Ctrl Pts',(-22.0652380838038,-13.4086720240795,
113.455542704925)) ;
#168236=CARTESIAN_POINT('Ctrl Pts',(-22.0887502249899,-13.1198463580562,
113.49161061441)) ;
#168237=CARTESIAN_POINT('Ctrl Pts',(-22.11155604208,-13.1402531049797,113.561073453608)) ;
#168238=CARTESIAN_POINT('Ctrl Pts',(-22.1853598855831,-13.1402531026116,
113.536842412175)) ;
#168239=CARTESIAN_POINT('Ctrl Pts',(-22.2591637290863,-13.1402531002435,
113.512611370743)) ;
#168240=CARTESIAN_POINT('Ctrl Pts',(-22.2363579119963,-13.1198463533199,
113.443148531545)) ;
#168241=CARTESIAN_POINT('Ctrl Pts',(-22.2135520949062,-13.0994396063964,
113.373685692348)) ;
#168242=CARTESIAN_POINT('Ctrl Pts',(-22.139748251403,-13.0994396087645,
113.39791673378)) ;
#168243=CARTESIAN_POINT('Ctrl Pts',(-22.0659444078998,-13.0994396111326,
113.422147775213)) ;
#168244=CARTESIAN_POINT('Ctrl Pts',(-22.0887502249899,-13.1198463580562,
113.49161061441)) ;
#168245=CARTESIAN_POINT('Ctrl Pts',(-22.1354479268997,-12.8536440540051,
113.598479641973)) ;
#168246=CARTESIAN_POINT('Ctrl Pts',(-22.1557581310016,-12.8926679376459,
113.660341246762)) ;
#168247=CARTESIAN_POINT('Ctrl Pts',(-22.2295619753836,-12.8926679313973,
113.636110208007)) ;
#168248=CARTESIAN_POINT('Ctrl Pts',(-22.3033658197655,-12.8926679251486,
113.611879169251)) ;
#168249=CARTESIAN_POINT('Ctrl Pts',(-22.2830556156637,-12.8536440415079,
113.550017564462)) ;
#168250=CARTESIAN_POINT('Ctrl Pts',(-22.2627454115618,-12.8146201578671,
113.488155959672)) ;
#168251=CARTESIAN_POINT('Ctrl Pts',(-22.1889415671798,-12.8146201641158,
113.512386998428)) ;
#168252=CARTESIAN_POINT('Ctrl Pts',(-22.1151377227978,-12.8146201703644,
113.536618037184)) ;
#168253=CARTESIAN_POINT('Ctrl Pts',(-22.1354479268997,-12.8536440540051,
113.598479641973)) ;
#168254=CARTESIAN_POINT('Ctrl Pts',(-22.2034506138866,-12.6260691585523,
113.769947386255)) ;
#168255=CARTESIAN_POINT('Ctrl Pts',(-22.2197801294508,-12.6810405314409,
113.819684456192)) ;
#168256=CARTESIAN_POINT('Ctrl Pts',(-22.2935839760765,-12.6810405208292,
113.79545342427)) ;
#168257=CARTESIAN_POINT('Ctrl Pts',(-22.3673878227021,-12.6810405102175,
113.771222392348)) ;
#168258=CARTESIAN_POINT('Ctrl Pts',(-22.3510583071379,-12.6260691373289,
113.721485322411)) ;
#168259=CARTESIAN_POINT('Ctrl Pts',(-22.3347287915737,-12.5710977644403,
113.671748252474)) ;
#168260=CARTESIAN_POINT('Ctrl Pts',(-22.2609249449481,-12.571097775052,
113.695979284396)) ;
#168261=CARTESIAN_POINT('Ctrl Pts',(-22.1871210983224,-12.5710977856637,
113.720210316318)) ;
#168262=CARTESIAN_POINT('Ctrl Pts',(-22.2034506138866,-12.6260691585523,
113.769947386255)) ;
#168263=CARTESIAN_POINT('Ctrl Pts',(-22.2875987666924,-12.4569456938658,
113.990878373043)) ;
#168264=CARTESIAN_POINT('Ctrl Pts',(-22.2988084284199,-12.5238051277268,
114.025021194409)) ;
#168265=CARTESIAN_POINT('Ctrl Pts',(-22.3726122776629,-12.5238051170314,
114.000790170459)) ;
#168266=CARTESIAN_POINT('Ctrl Pts',(-22.446416126906,-12.523805106336,113.976559146509)) ;
#168267=CARTESIAN_POINT('Ctrl Pts',(-22.4352064651785,-12.4569456724751,
113.942416325143)) ;
#168268=CARTESIAN_POINT('Ctrl Pts',(-22.423996803451,-12.3900862386142,
113.908273503778)) ;
#168269=CARTESIAN_POINT('Ctrl Pts',(-22.3501929542079,-12.3900862493095,
113.932504527728)) ;
#168270=CARTESIAN_POINT('Ctrl Pts',(-22.2763891049649,-12.3900862600049,
113.956735551678)) ;
#168271=CARTESIAN_POINT('Ctrl Pts',(-22.2875987666924,-12.4569456938658,
113.990878373043)) ;
#168272=CARTESIAN_POINT('Ctrl Pts',(-22.3834860536271,-12.3560371763605,
114.247407246605)) ;
#168273=CARTESIAN_POINT('Ctrl Pts',(-22.388752146054,-12.4300391766208,
114.263446915039)) ;
#168274=CARTESIAN_POINT('Ctrl Pts',(-22.4625559985964,-12.43003916942,114.239215901139)) ;
#168275=CARTESIAN_POINT('Ctrl Pts',(-22.5363598511387,-12.4300391622191,
114.214984887238)) ;
#168276=CARTESIAN_POINT('Ctrl Pts',(-22.5310937587119,-12.3560371619588,
114.198945218804)) ;
#168277=CARTESIAN_POINT('Ctrl Pts',(-22.525827666285,-12.2820351616984,
114.182905550369)) ;
#168278=CARTESIAN_POINT('Ctrl Pts',(-22.4520238137426,-12.2820351688993,
114.20713656427)) ;
#168279=CARTESIAN_POINT('Ctrl Pts',(-22.3782199612002,-12.2820351761001,
114.23136757817)) ;
#168280=CARTESIAN_POINT('Ctrl Pts',(-22.3834860536271,-12.3560371763605,
114.247407246605)) ;
#168281=CARTESIAN_POINT('Ctrl Pts',(-22.4840972968736,-12.3312869891021,
114.51853287169)) ;
#168282=CARTESIAN_POINT('Ctrl Pts',(-22.4830771493672,-12.407123602134,
114.515425667706)) ;
#168283=CARTESIAN_POINT('Ctrl Pts',(-22.5568810044093,-12.4071236031691,
114.49119466142)) ;
#168284=CARTESIAN_POINT('Ctrl Pts',(-22.6306848594514,-12.4071236042042,
114.466963655133)) ;
#168285=CARTESIAN_POINT('Ctrl Pts',(-22.6317050069579,-12.3312869911723,
114.470070859117)) ;
#168286=CARTESIAN_POINT('Ctrl Pts',(-22.6327251544643,-12.2554503781403,
114.473178063101)) ;
#168287=CARTESIAN_POINT('Ctrl Pts',(-22.5589212994222,-12.2554503771052,
114.497409069387)) ;
#168288=CARTESIAN_POINT('Ctrl Pts',(-22.4851174443801,-12.2554503760701,
114.521640075674)) ;
#168289=CARTESIAN_POINT('Ctrl Pts',(-22.4840972968736,-12.3312869891021,
114.51853287169)) ;
#168290=CARTESIAN_POINT('Ctrl Pts',(-22.5844346669737,-12.384579728798,
114.788494098103)) ;
#168291=CARTESIAN_POINT('Ctrl Pts',(-22.5771451839705,-12.4568056181836,
114.766291509953)) ;
#168292=CARTESIAN_POINT('Ctrl Pts',(-22.6509490416241,-12.4568056323219,
114.74206051162)) ;
#168293=CARTESIAN_POINT('Ctrl Pts',(-22.7247528992776,-12.4568056464601,
114.717829513288)) ;
#168294=CARTESIAN_POINT('Ctrl Pts',(-22.7320423822809,-12.3845797570745,
114.740032101438)) ;
#168295=CARTESIAN_POINT('Ctrl Pts',(-22.7393318652841,-12.3123538676888,
114.762234689588)) ;
#168296=CARTESIAN_POINT('Ctrl Pts',(-22.6655280076305,-12.3123538535506,
114.78646568792)) ;
#168297=CARTESIAN_POINT('Ctrl Pts',(-22.5917241499769,-12.3123538394123,
114.810696686253)) ;
#168298=CARTESIAN_POINT('Ctrl Pts',(-22.5844346669737,-12.384579728798,
114.788494098103)) ;
#168299=CARTESIAN_POINT('Ctrl Pts',(-22.6765292835833,-12.5118388251457,
115.033574716962)) ;
#168300=CARTESIAN_POINT('Ctrl Pts',(-22.6635323516411,-12.5752838792253,
114.993988160397)) ;
#168301=CARTESIAN_POINT('Ctrl Pts',(-22.7373362097494,-12.5752839097083,
114.96975716345)) ;
#168302=CARTESIAN_POINT('Ctrl Pts',(-22.8111400678576,-12.5752839401913,
114.945526166502)) ;
#168303=CARTESIAN_POINT('Ctrl Pts',(-22.8241369997999,-12.5118388861117,
114.985112723066)) ;
#168304=CARTESIAN_POINT('Ctrl Pts',(-22.8371339317421,-12.448393832032,
115.024699279631)) ;
#168305=CARTESIAN_POINT('Ctrl Pts',(-22.7633300736338,-12.4483938015491,
115.048930276579)) ;
#168306=CARTESIAN_POINT('Ctrl Pts',(-22.6895262155256,-12.4483937710661,
115.073161273526)) ;
#168307=CARTESIAN_POINT('Ctrl Pts',(-22.6765292835833,-12.5118388251457,
115.033574716962)) ;
#168308=CARTESIAN_POINT('Ctrl Pts',(-22.7552676475542,-12.7038857020727,
115.237944156855)) ;
#168309=CARTESIAN_POINT('Ctrl Pts',(-22.7374881961524,-12.7540141068732,
115.183790817835)) ;
#168310=CARTESIAN_POINT('Ctrl Pts',(-22.8112920529231,-12.7540141550584,
115.159559816814)) ;
#168311=CARTESIAN_POINT('Ctrl Pts',(-22.8850959096938,-12.7540142032436,
115.135328815792)) ;
#168312=CARTESIAN_POINT('Ctrl Pts',(-22.9028753610955,-12.7038857984431,
115.189482154812)) ;
#168313=CARTESIAN_POINT('Ctrl Pts',(-22.9206548124973,-12.6537573936426,
115.243635493831)) ;
#168314=CARTESIAN_POINT('Ctrl Pts',(-22.8468509557266,-12.6537573454574,
115.267866494853)) ;
#168315=CARTESIAN_POINT('Ctrl Pts',(-22.7730470989559,-12.6537572972722,
115.292097495875)) ;
#168316=CARTESIAN_POINT('Ctrl Pts',(-22.7552676475542,-12.7038857020727,
115.237944156855)) ;
#168317=CARTESIAN_POINT('Ctrl Pts',(-22.8155921978644,-12.9467051649881,
115.386282575257)) ;
#168318=CARTESIAN_POINT('Ctrl Pts',(-22.7943078394483,-12.9799528972862,
115.321453855131)) ;
#168319=CARTESIAN_POINT('Ctrl Pts',(-22.868111692756,-12.9799529618983,
115.297222843561)) ;
#168320=CARTESIAN_POINT('Ctrl Pts',(-22.9419155460636,-12.9799530265103,
115.272991831992)) ;
#168321=CARTESIAN_POINT('Ctrl Pts',(-22.9631999044797,-12.9467052942123,
115.337820552117)) ;
#168322=CARTESIAN_POINT('Ctrl Pts',(-22.9844842628957,-12.9134575619143,
115.402649272243)) ;
#168323=CARTESIAN_POINT('Ctrl Pts',(-22.9106804095881,-12.9134574973022,
115.426880283813)) ;
#168324=CARTESIAN_POINT('Ctrl Pts',(-22.8368765562805,-12.9134574326901,
115.451111295382)) ;
#168325=CARTESIAN_POINT('Ctrl Pts',(-22.8155921978644,-12.9467051649881,
115.386282575257)) ;
#168326=CARTESIAN_POINT('Ctrl Pts',(-22.854117195054,-13.2232753780377,
115.468204454967)) ;
#168327=CARTESIAN_POINT('Ctrl Pts',(-22.8308452016767,-13.237261879662,
115.397321719593)) ;
#168328=CARTESIAN_POINT('Ctrl Pts',(-22.9046490496905,-13.237261957473,
115.373090691899)) ;
#168329=CARTESIAN_POINT('Ctrl Pts',(-22.9784528977043,-13.237262035284,
115.348859664205)) ;
#168330=CARTESIAN_POINT('Ctrl Pts',(-23.0017248910816,-13.2232755336597,
115.419742399579)) ;
#168331=CARTESIAN_POINT('Ctrl Pts',(-23.0249968844588,-13.2092890320355,
115.490625134953)) ;
#168332=CARTESIAN_POINT('Ctrl Pts',(-22.9511930364451,-13.2092889542245,
115.514856162647)) ;
#168333=CARTESIAN_POINT('Ctrl Pts',(-22.8773891884313,-13.2092888764135,
115.539087190341)) ;
#168334=CARTESIAN_POINT('Ctrl Pts',(-22.854117195054,-13.2232753780377,
115.468204454967)) ;
#168335=CARTESIAN_POINT('Ctrl Pts',(-22.8687874098863,-13.5141286997517,
115.477425109878)) ;
#168336=CARTESIAN_POINT('Ctrl Pts',(-22.8451911742884,-13.5078290678433,
115.405554785151)) ;
#168337=CARTESIAN_POINT('Ctrl Pts',(-22.9189950154969,-13.5078291537003,
115.381323736729)) ;
#168338=CARTESIAN_POINT('Ctrl Pts',(-22.9927988567055,-13.5078292395572,
115.357092688308)) ;
#168339=CARTESIAN_POINT('Ctrl Pts',(-23.0163950923034,-13.5141288714655,
115.428963013036)) ;
#168340=CARTESIAN_POINT('Ctrl Pts',(-23.0399913279013,-13.5204285033738,
115.500833337763)) ;
#168341=CARTESIAN_POINT('Ctrl Pts',(-22.9661874866927,-13.5204284175169,
115.525064386185)) ;
#168342=CARTESIAN_POINT('Ctrl Pts',(-22.8923836454841,-13.52042833166,115.549295434606)) ;
#168343=CARTESIAN_POINT('Ctrl Pts',(-22.8687874098863,-13.5141286997517,
115.477425109878)) ;
#168344=CARTESIAN_POINT('Ctrl Pts',(-22.8592321322332,-13.7984771926956,
115.412815935399)) ;
#168345=CARTESIAN_POINT('Ctrl Pts',(-22.8370032864545,-13.7723162248091,
115.345110459558)) ;
#168346=CARTESIAN_POINT('Ctrl Pts',(-22.9108071199101,-13.7723163117777,
115.320879387523)) ;
#168347=CARTESIAN_POINT('Ctrl Pts',(-22.9846109533657,-13.7723163987464,
115.296648315487)) ;
#168348=CARTESIAN_POINT('Ctrl Pts',(-23.0068397991444,-13.7984773666329,
115.364353791328)) ;
#168349=CARTESIAN_POINT('Ctrl Pts',(-23.0290686449232,-13.8246383345194,
115.432059267169)) ;
#168350=CARTESIAN_POINT('Ctrl Pts',(-22.9552648114676,-13.8246382475507,
115.456290339205)) ;
#168351=CARTESIAN_POINT('Ctrl Pts',(-22.881460978012,-13.8246381605821,
115.48052141124)) ;
#168352=CARTESIAN_POINT('Ctrl Pts',(-22.8592321322332,-13.7984771926956,
115.412815935399)) ;
#168353=CARTESIAN_POINT('Ctrl Pts',(-22.8267505858683,-14.0556517682192,
115.278338405061)) ;
#168354=CARTESIAN_POINT('Ctrl Pts',(-22.8074924148263,-14.0114975765456,
115.219681125259)) ;
#168355=CARTESIAN_POINT('Ctrl Pts',(-22.8812962403663,-14.011497656322,
115.195450029114)) ;
#168356=CARTESIAN_POINT('Ctrl Pts',(-22.9551000659063,-14.0114977360984,
115.171218932969)) ;
#168357=CARTESIAN_POINT('Ctrl Pts',(-22.9743582369483,-14.055651927772,
115.22987621277)) ;
#168358=CARTESIAN_POINT('Ctrl Pts',(-22.9936164079904,-14.0998061194455,
115.288533492572)) ;
#168359=CARTESIAN_POINT('Ctrl Pts',(-22.9198125824504,-14.0998060396691,
115.312764588717)) ;
#168360=CARTESIAN_POINT('Ctrl Pts',(-22.8460087569104,-14.0998059598928,
115.336995684862)) ;
#168361=CARTESIAN_POINT('Ctrl Pts',(-22.8267505858683,-14.0556517682192,
115.278338405061)) ;
#168362=CARTESIAN_POINT('Ctrl Pts',(-22.7749229736523,-14.2658619034502,
115.085168032102)) ;
#168363=CARTESIAN_POINT('Ctrl Pts',(-22.7599858265449,-14.206967241119,
115.03967189408)) ;
#168364=CARTESIAN_POINT('Ctrl Pts',(-22.8337896452694,-14.2069673051098,
115.015440777175)) ;
#168365=CARTESIAN_POINT('Ctrl Pts',(-22.9075934639938,-14.2069673691006,
114.991209660271)) ;
#168366=CARTESIAN_POINT('Ctrl Pts',(-22.9225306111012,-14.2658620314317,
115.036705798294)) ;
#168367=CARTESIAN_POINT('Ctrl Pts',(-22.9374677582085,-14.3247566937629,
115.082201936316)) ;
#168368=CARTESIAN_POINT('Ctrl Pts',(-22.8636639394841,-14.3247566297721,
115.10643305322)) ;
#168369=CARTESIAN_POINT('Ctrl Pts',(-22.7898601207596,-14.3247565657813,
115.130664170125)) ;
#168370=CARTESIAN_POINT('Ctrl Pts',(-22.7749229736523,-14.2658619034502,
115.085168032102)) ;
#168371=CARTESIAN_POINT('Ctrl Pts',(-22.7073801962301,-14.4169100671748,
114.843829194715)) ;
#168372=CARTESIAN_POINT('Ctrl Pts',(-22.6978734686817,-14.3473831262014,
114.814873238548)) ;
#168373=CARTESIAN_POINT('Ctrl Pts',(-22.7716772818824,-14.3473831682741,
114.790642104819)) ;
#168374=CARTESIAN_POINT('Ctrl Pts',(-22.8454810950831,-14.3473832103469,
114.76641097109)) ;
#168375=CARTESIAN_POINT('Ctrl Pts',(-22.8549878226315,-14.4169101513204,
114.795366927258)) ;
#168376=CARTESIAN_POINT('Ctrl Pts',(-22.8644945501799,-14.4864370922939,
114.824322883424)) ;
#168377=CARTESIAN_POINT('Ctrl Pts',(-22.7906907369792,-14.4864370502211,
114.848554017153)) ;
#168378=CARTESIAN_POINT('Ctrl Pts',(-22.7168869237785,-14.4864370081483,
114.872785150882)) ;
#168379=CARTESIAN_POINT('Ctrl Pts',(-22.7073801962301,-14.4169100671748,
114.843829194715)) ;
#168380=CARTESIAN_POINT('Ctrl Pts',(-22.6304186927666,-14.4953742453793,
114.573953875057)) ;
#168381=CARTESIAN_POINT('Ctrl Pts',(-22.6270049111093,-14.4202668072197,
114.563556049018)) ;
#168382=CARTESIAN_POINT('Ctrl Pts',(-22.7008087213179,-14.4202668221935,
114.539324906176)) ;
#168383=CARTESIAN_POINT('Ctrl Pts',(-22.7746125315266,-14.4202668371673,
114.515093763334)) ;
#168384=CARTESIAN_POINT('Ctrl Pts',(-22.7780263131839,-14.495374275327,
114.525491589373)) ;
#168385=CARTESIAN_POINT('Ctrl Pts',(-22.7814400948412,-14.5704817134867,
114.535889415412)) ;
#168386=CARTESIAN_POINT('Ctrl Pts',(-22.7076362846326,-14.5704816985128,
114.560120558254)) ;
#168387=CARTESIAN_POINT('Ctrl Pts',(-22.6338324744239,-14.570481683539,
114.584351701096)) ;
#168388=CARTESIAN_POINT('Ctrl Pts',(-22.6304186927666,-14.4953742453793,
114.573953875057)) ;
#168389=CARTESIAN_POINT('Ctrl Pts',(-22.550396983414,-14.4969828286805,
114.294883066469)) ;
#168390=CARTESIAN_POINT('Ctrl Pts',(-22.553296213992,-14.4216525600046,
114.303713657114)) ;
#168391=CARTESIAN_POINT('Ctrl Pts',(-22.6271000238928,-14.4216525461531,
114.279482513335)) ;
#168392=CARTESIAN_POINT('Ctrl Pts',(-22.7009038337936,-14.4216525323015,
114.255251369555)) ;
#168393=CARTESIAN_POINT('Ctrl Pts',(-22.6980046032156,-14.4969828009775,
114.24642077891)) ;
#168394=CARTESIAN_POINT('Ctrl Pts',(-22.6951053726376,-14.5723130696534,
114.237590188265)) ;
#168395=CARTESIAN_POINT('Ctrl Pts',(-22.6213015627367,-14.5723130835049,
114.261821332045)) ;
#168396=CARTESIAN_POINT('Ctrl Pts',(-22.5474977528359,-14.5723130973564,
114.286052475824)) ;
#168397=CARTESIAN_POINT('Ctrl Pts',(-22.550396983414,-14.4969828286805,
114.294883066469)) ;
#168398=CARTESIAN_POINT('Ctrl Pts',(-22.4731667198219,-14.421551875411,
114.024183632776)) ;
#168399=CARTESIAN_POINT('Ctrl Pts',(-22.4821960521994,-14.3513763125925,
114.051685524413)) ;
#168400=CARTESIAN_POINT('Ctrl Pts',(-22.555999864463,-14.3513762706419,
114.02745438783)) ;
#168401=CARTESIAN_POINT('Ctrl Pts',(-22.6298036767266,-14.3513762286912,
114.003223251247)) ;
#168402=CARTESIAN_POINT('Ctrl Pts',(-22.6207743443492,-14.4215517915098,
113.97572135961)) ;
#168403=CARTESIAN_POINT('Ctrl Pts',(-22.6117450119717,-14.4917273543283,
113.948219467973)) ;
#168404=CARTESIAN_POINT('Ctrl Pts',(-22.5379411997081,-14.491727396279,
113.972450604555)) ;
#168405=CARTESIAN_POINT('Ctrl Pts',(-22.4641373874444,-14.4917274382296,
113.996681741138)) ;
#168406=CARTESIAN_POINT('Ctrl Pts',(-22.4731667198219,-14.421551875411,
114.024183632776)) ;
#168407=CARTESIAN_POINT('Ctrl Pts',(-22.4051586069589,-14.2735000710325,
113.781463265939)) ;
#168408=CARTESIAN_POINT('Ctrl Pts',(-22.4196856428359,-14.213556255384,
113.825710275356)) ;
#168409=CARTESIAN_POINT('Ctrl Pts',(-22.4934894600971,-14.2135561892348,
113.801479153994)) ;
#168410=CARTESIAN_POINT('Ctrl Pts',(-22.5672932773583,-14.2135561230857,
113.777248032633)) ;
#168411=CARTESIAN_POINT('Ctrl Pts',(-22.5527662414813,-14.2734999387342,
113.733001023217)) ;
#168412=CARTESIAN_POINT('Ctrl Pts',(-22.5382392056042,-14.3334437543827,
113.6887540138)) ;
#168413=CARTESIAN_POINT('Ctrl Pts',(-22.4644353883431,-14.3334438205319,
113.712985135162)) ;
#168414=CARTESIAN_POINT('Ctrl Pts',(-22.3906315710819,-14.3334438866811,
113.737216256523)) ;
#168415=CARTESIAN_POINT('Ctrl Pts',(-22.4051586069589,-14.2735000710325,
113.781463265939)) ;
#168416=CARTESIAN_POINT('Ctrl Pts',(-22.3524264112535,-14.0646532706665,
113.585402345504)) ;
#168417=CARTESIAN_POINT('Ctrl Pts',(-22.3713901641002,-14.019201123048,
113.643162878901)) ;
#168418=CARTESIAN_POINT('Ctrl Pts',(-22.4451939882553,-14.0192010389841,
113.618931778537)) ;
#168419=CARTESIAN_POINT('Ctrl Pts',(-22.5189978124103,-14.0192009549201,
113.594700678174)) ;
#168420=CARTESIAN_POINT('Ctrl Pts',(-22.5000340595636,-14.0646531025386,
113.536940144777)) ;
#168421=CARTESIAN_POINT('Ctrl Pts',(-22.4810703067168,-14.110105250157,
113.47917961138)) ;
#168422=CARTESIAN_POINT('Ctrl Pts',(-22.4072664825617,-14.110105334221,
113.503410711744)) ;
#168423=CARTESIAN_POINT('Ctrl Pts',(-22.3334626584067,-14.1101054182849,
113.527641812108)) ;
#168424=CARTESIAN_POINT('Ctrl Pts',(-22.3524264112535,-14.0646532706665,
113.585402345504)) ;
#168425=CARTESIAN_POINT('Ctrl Pts',(-22.3192033937915,-13.8091818841456,
113.448713324322)) ;
#168426=CARTESIAN_POINT('Ctrl Pts',(-22.3412495726263,-13.7814979528365,
113.515862429858)) ;
#168427=CARTESIAN_POINT('Ctrl Pts',(-22.4150534048702,-13.7814978588796,
113.491631354132)) ;
#168428=CARTESIAN_POINT('Ctrl Pts',(-22.4888572371141,-13.7814977649226,
113.467400278406)) ;
#168429=CARTESIAN_POINT('Ctrl Pts',(-22.4668110582793,-13.8091816962316,
113.400251172869)) ;
#168430=CARTESIAN_POINT('Ctrl Pts',(-22.4447648794445,-13.8368656275406,
113.333102067333)) ;
#168431=CARTESIAN_POINT('Ctrl Pts',(-22.3709610472006,-13.8368657214976,
113.357333143059)) ;
#168432=CARTESIAN_POINT('Ctrl Pts',(-22.2971572149566,-13.8368658154546,
113.381564218785)) ;
#168433=CARTESIAN_POINT('Ctrl Pts',(-22.3192033937915,-13.8091818841456,
113.448713324322)) ;
#168434=CARTESIAN_POINT('Ctrl Pts',(-22.3086900686666,-13.5266904596517,
113.381322855657)) ;
#168435=CARTESIAN_POINT('Ctrl Pts',(-22.3322350932624,-13.5186880514058,
113.453037203464)) ;
#168436=CARTESIAN_POINT('Ctrl Pts',(-22.406038933809,-13.5186879553988,
113.428806153027)) ;
#168437=CARTESIAN_POINT('Ctrl Pts',(-22.4798427743556,-13.5186878593918,
113.404575102589)) ;
#168438=CARTESIAN_POINT('Ctrl Pts',(-22.4562977497598,-13.5266902676377,
113.332860754782)) ;
#168439=CARTESIAN_POINT('Ctrl Pts',(-22.432752725164,-13.5346926758837,
113.261146406975)) ;
#168440=CARTESIAN_POINT('Ctrl Pts',(-22.3589488846175,-13.5346927718906,
113.285377457413)) ;
#168441=CARTESIAN_POINT('Ctrl Pts',(-22.2851450440709,-13.5346928678976,
113.30960850785)) ;
#168442=CARTESIAN_POINT('Ctrl Pts',(-22.3086900686666,-13.5266904596517,
113.381322855657)) ;
#168443=CARTESIAN_POINT('Ctrl Pts',(-22.3223045121506,-13.2352604395114,
113.387274613305)) ;
#168444=CARTESIAN_POINT('Ctrl Pts',(-22.3456693500622,-13.2475929455495,
113.458440141433)) ;
#168445=CARTESIAN_POINT('Ctrl Pts',(-22.4194731984143,-13.2475928562787,
113.434209114769)) ;
#168446=CARTESIAN_POINT('Ctrl Pts',(-22.4932770467663,-13.2475927670079,
113.409978088106)) ;
#168447=CARTESIAN_POINT('Ctrl Pts',(-22.4699122088548,-13.2352602609698,
113.338812559978)) ;
#168448=CARTESIAN_POINT('Ctrl Pts',(-22.4465473709432,-13.2229277549316,
113.26764703185)) ;
#168449=CARTESIAN_POINT('Ctrl Pts',(-22.3727435225911,-13.2229278442025,
113.291878058513)) ;
#168450=CARTESIAN_POINT('Ctrl Pts',(-22.2989396742391,-13.2229279334733,
113.316109085177)) ;
#168451=CARTESIAN_POINT('Ctrl Pts',(-22.3223045121506,-13.2352604395114,
113.387274613305)) ;
#168452=CARTESIAN_POINT('Ctrl Pts',(-22.360045558316,-12.9567404114365,
113.466682888076)) ;
#168453=CARTESIAN_POINT('Ctrl Pts',(-22.3815461871748,-12.9885373907524,
113.532170336082)) ;
#168454=CARTESIAN_POINT('Ctrl Pts',(-22.4553500418253,-12.9885373153284,
113.507939328603)) ;
#168455=CARTESIAN_POINT('Ctrl Pts',(-22.5291538964759,-12.9885372399044,
113.483708321124)) ;
#168456=CARTESIAN_POINT('Ctrl Pts',(-22.5076532676171,-12.9567402605885,
113.418220873118)) ;
#168457=CARTESIAN_POINT('Ctrl Pts',(-22.4861526387583,-12.9249432812726,
113.352733425112)) ;
#168458=CARTESIAN_POINT('Ctrl Pts',(-22.4123487841078,-12.9249433566966,
113.376964432591)) ;
#168459=CARTESIAN_POINT('Ctrl Pts',(-22.3385449294572,-12.9249434321206,
113.401195440071)) ;
#168460=CARTESIAN_POINT('Ctrl Pts',(-22.360045558316,-12.9567404114365,
113.466682888076)) ;
#168461=CARTESIAN_POINT('Ctrl Pts',(-22.4196665993384,-12.7122106250869,
113.612854579177)) ;
#168462=CARTESIAN_POINT('Ctrl Pts',(-22.437769996859,-12.7611284974195,
113.667994608535)) ;
#168463=CARTESIAN_POINT('Ctrl Pts',(-22.5115738559352,-12.7611284394827,
113.643763614535)) ;
#168464=CARTESIAN_POINT('Ctrl Pts',(-22.5853777150113,-12.7611283815459,
113.619532620536)) ;
#168465=CARTESIAN_POINT('Ctrl Pts',(-22.5672743174907,-12.7122105092134,
113.564392591178)) ;
#168466=CARTESIAN_POINT('Ctrl Pts',(-22.5491709199701,-12.6632926368809,
113.509252561821)) ;
#168467=CARTESIAN_POINT('Ctrl Pts',(-22.4753670608939,-12.6632926948177,
113.533483555821)) ;
#168468=CARTESIAN_POINT('Ctrl Pts',(-22.4015632018178,-12.6632927527544,
113.55771454982)) ;
#168469=CARTESIAN_POINT('Ctrl Pts',(-22.4196665993384,-12.7122106250869,
113.612854579177)) ;
#168470=CARTESIAN_POINT('Ctrl Pts',(-22.4976345852883,-12.5182289407429,
113.814941278565)) ;
#168471=CARTESIAN_POINT('Ctrl Pts',(-22.5110539521442,-12.5807644314872,
113.855814506146)) ;
#168472=CARTESIAN_POINT('Ctrl Pts',(-22.5848578136224,-12.5807643929597,
113.831583519462)) ;
#168473=CARTESIAN_POINT('Ctrl Pts',(-22.6586616751006,-12.5807643544323,
113.807352532779)) ;
#168474=CARTESIAN_POINT('Ctrl Pts',(-22.6452423082446,-12.518228863688,
113.766479305198)) ;
#168475=CARTESIAN_POINT('Ctrl Pts',(-22.6318229413887,-12.4556933729437,
113.725606077618)) ;
#168476=CARTESIAN_POINT('Ctrl Pts',(-22.5580190799105,-12.4556934114712,
113.749837064301)) ;
#168477=CARTESIAN_POINT('Ctrl Pts',(-22.4842152184323,-12.4556934499986,
113.774068050984)) ;
#168478=CARTESIAN_POINT('Ctrl Pts',(-22.4976345852883,-12.5182289407429,
113.814941278565)) ;
#168479=CARTESIAN_POINT('Ctrl Pts',(-22.5895023142545,-12.3880154836096,
114.059257743448)) ;
#168480=CARTESIAN_POINT('Ctrl Pts',(-22.5972623678869,-12.4597373427525,
114.082893615912)) ;
#168481=CARTESIAN_POINT('Ctrl Pts',(-22.6710662293981,-12.4597373239449,
114.058662629329)) ;
#168482=CARTESIAN_POINT('Ctrl Pts',(-22.7448700909092,-12.4597373051373,
114.034431642746)) ;
#168483=CARTESIAN_POINT('Ctrl Pts',(-22.7371100372769,-12.3880154459944,
114.010795770283)) ;
#168484=CARTESIAN_POINT('Ctrl Pts',(-22.7293499836445,-12.3162935868514,
113.987159897819)) ;
#168485=CARTESIAN_POINT('Ctrl Pts',(-22.6555461221333,-12.316293605659,
114.011390884402)) ;
#168486=CARTESIAN_POINT('Ctrl Pts',(-22.5817422606221,-12.3162936244666,
114.035621870985)) ;
#168487=CARTESIAN_POINT('Ctrl Pts',(-22.5895023142545,-12.3880154836096,
114.059257743448)) ;
#168488=CARTESIAN_POINT('Ctrl Pts',(-22.6895136884931,-12.3319594983171,
114.328282716118)) ;
#168489=CARTESIAN_POINT('Ctrl Pts',(-22.6910391558902,-12.4077044418995,
114.332929044665)) ;
#168490=CARTESIAN_POINT('Ctrl Pts',(-22.7648430152365,-12.407704439621,
114.308698051488)) ;
#168491=CARTESIAN_POINT('Ctrl Pts',(-22.8386468745828,-12.4077044373425,
114.284467058311)) ;
#168492=CARTESIAN_POINT('Ctrl Pts',(-22.8371214071857,-12.33195949376,114.279820729764)) ;
#168493=CARTESIAN_POINT('Ctrl Pts',(-22.8355959397885,-12.2562145501775,
114.275174401218)) ;
#168494=CARTESIAN_POINT('Ctrl Pts',(-22.7617920804422,-12.2562145524561,
114.299405394395)) ;
#168495=CARTESIAN_POINT('Ctrl Pts',(-22.6879882210959,-12.2562145547346,
114.323636387572)) ;
#168496=CARTESIAN_POINT('Ctrl Pts',(-22.6895136884931,-12.3319594983171,
114.328282716118)) ;
#168497=CARTESIAN_POINT('Ctrl Pts',(-22.7899870488057,-12.3535606969818,
114.599060850757)) ;
#168498=CARTESIAN_POINT('Ctrl Pts',(-22.7852289860199,-12.4279116529158,
114.584568560083)) ;
#168499=CARTESIAN_POINT('Ctrl Pts',(-22.8590328429792,-12.4279116627694,
114.560337559636)) ;
#168500=CARTESIAN_POINT('Ctrl Pts',(-22.9328366999386,-12.427911672623,
114.536106559189)) ;
#168501=CARTESIAN_POINT('Ctrl Pts',(-22.9375947627244,-12.3535607166891,
114.550598849862)) ;
#168502=CARTESIAN_POINT('Ctrl Pts',(-22.9423528255101,-12.2792097607552,
114.565091140536)) ;
#168503=CARTESIAN_POINT('Ctrl Pts',(-22.8685489685508,-12.2792097509015,
114.589322140983)) ;
#168504=CARTESIAN_POINT('Ctrl Pts',(-22.7947451115915,-12.2792097410479,
114.61355314143)) ;
#168505=CARTESIAN_POINT('Ctrl Pts',(-22.7899870488057,-12.3535606969818,
114.599060850757)) ;
#168506=CARTESIAN_POINT('Ctrl Pts',(-22.8861512888301,-12.451253883518,
114.856463511096)) ;
#168507=CARTESIAN_POINT('Ctrl Pts',(-22.8754061618611,-12.5188965599117,
114.823735588756)) ;
#168508=CARTESIAN_POINT('Ctrl Pts',(-22.9492100150156,-12.5188965769681,
114.79950457672)) ;
#168509=CARTESIAN_POINT('Ctrl Pts',(-23.0230138681702,-12.5188965940245,
114.775273564684)) ;
#168510=CARTESIAN_POINT('Ctrl Pts',(-23.0337589951393,-12.4512539176309,
114.808001487025)) ;
#168511=CARTESIAN_POINT('Ctrl Pts',(-23.0445041221084,-12.3836112412372,
114.840729409365)) ;
#168512=CARTESIAN_POINT('Ctrl Pts',(-22.9707002689538,-12.3836112241808,
114.864960421401)) ;
#168513=CARTESIAN_POINT('Ctrl Pts',(-22.8968964157992,-12.3836112071243,
114.889191433437)) ;
#168514=CARTESIAN_POINT('Ctrl Pts',(-22.8861512888301,-12.451253883518,
114.856463511096)) ;
#168515=CARTESIAN_POINT('Ctrl Pts',(-22.9710997816442,-12.618326669095,
115.079730072994)) ;
#168516=CARTESIAN_POINT('Ctrl Pts',(-22.9551410288214,-12.6744063613934,
115.031122287354)) ;
#168517=CARTESIAN_POINT('Ctrl Pts',(-23.0289448782623,-12.6744063803127,
115.006891264007)) ;
#168518=CARTESIAN_POINT('Ctrl Pts',(-23.1027487277032,-12.6744063992319,
114.98266024066)) ;
#168519=CARTESIAN_POINT('Ctrl Pts',(-23.118707480526,-12.6183267069335,
115.0312680263)) ;
#168520=CARTESIAN_POINT('Ctrl Pts',(-23.1346662333488,-12.5622470146351,
115.07987581194)) ;
#168521=CARTESIAN_POINT('Ctrl Pts',(-23.0608623839079,-12.5622469957158,
115.104106835287)) ;
#168522=CARTESIAN_POINT('Ctrl Pts',(-22.987058534467,-12.5622469767965,
115.128337858634)) ;
#168523=CARTESIAN_POINT('Ctrl Pts',(-22.9710997816442,-12.618326669095,
115.079730072994)) ;
#168524=CARTESIAN_POINT('Ctrl Pts',(-23.0396705642867,-12.8433532834822,
115.253021743051)) ;
#168525=CARTESIAN_POINT('Ctrl Pts',(-23.0196356089412,-12.883805650216,
115.191998502051)) ;
#168526=CARTESIAN_POINT('Ctrl Pts',(-23.0934394551956,-12.8838056661619,
115.167767468999)) ;
#168527=CARTESIAN_POINT('Ctrl Pts',(-23.16724330145,-12.8838056821078,115.143536435946)) ;
#168528=CARTESIAN_POINT('Ctrl Pts',(-23.1872782567955,-12.843353315374,
115.204559676946)) ;
#168529=CARTESIAN_POINT('Ctrl Pts',(-23.207313212141,-12.8029009486403,
115.265582917945)) ;
#168530=CARTESIAN_POINT('Ctrl Pts',(-23.1335093658866,-12.8029009326944,
115.289813950998)) ;
#168531=CARTESIAN_POINT('Ctrl Pts',(-23.0597055196322,-12.8029009167485,
115.314044984051)) ;
#168532=CARTESIAN_POINT('Ctrl Pts',(-23.0396705642867,-12.8433532834822,
115.253021743051)) ;
#168533=CARTESIAN_POINT('Ctrl Pts',(-23.0873467114543,-13.1083703127966,
115.362848501741)) ;
#168534=CARTESIAN_POINT('Ctrl Pts',(-23.0646848738263,-13.1303789495469,
115.293824201028)) ;
#168535=CARTESIAN_POINT('Ctrl Pts',(-23.1384887180983,-13.1303789610419,
115.269593161937)) ;
#168536=CARTESIAN_POINT('Ctrl Pts',(-23.2122925623702,-13.130378972537,
115.245362122846)) ;
#168537=CARTESIAN_POINT('Ctrl Pts',(-23.2349543999982,-13.1083703357867,
115.314386423559)) ;
#168538=CARTESIAN_POINT('Ctrl Pts',(-23.2576162376261,-13.0863616990364,
115.383410724271)) ;
#168539=CARTESIAN_POINT('Ctrl Pts',(-23.1838123933542,-13.0863616875414,
115.407641763362)) ;
#168540=CARTESIAN_POINT('Ctrl Pts',(-23.1100085490823,-13.0863616760463,
115.431872802453)) ;
#168541=CARTESIAN_POINT('Ctrl Pts',(-23.0873467114543,-13.1083703127966,
115.362848501741)) ;
#168542=CARTESIAN_POINT('Ctrl Pts',(-23.1118506671336,-13.3973093025061,
115.401868284808)) ;
#168543=CARTESIAN_POINT('Ctrl Pts',(-23.0881805683991,-13.3991753907739,
115.329772983313)) ;
#168544=CARTESIAN_POINT('Ctrl Pts',(-23.1619844116872,-13.399175395662,
115.305541941225)) ;
#168545=CARTESIAN_POINT('Ctrl Pts',(-23.2357882549754,-13.39917540055,115.281310899138)) ;
#168546=CARTESIAN_POINT('Ctrl Pts',(-23.2594583537099,-13.3973093122823,
115.353406200633)) ;
#168547=CARTESIAN_POINT('Ctrl Pts',(-23.2831284524444,-13.3954432240146,
115.425501502128)) ;
#168548=CARTESIAN_POINT('Ctrl Pts',(-23.2093246091562,-13.3954432191265,
115.449732544215)) ;
#168549=CARTESIAN_POINT('Ctrl Pts',(-23.1355207658681,-13.3954432142384,
115.473963586303)) ;
#168550=CARTESIAN_POINT('Ctrl Pts',(-23.1118506671336,-13.3973093025061,
115.401868284808)) ;
#168551=CARTESIAN_POINT('Ctrl Pts',(-23.1119807889645,-13.685052446536,
115.366993485152)) ;
#168552=CARTESIAN_POINT('Ctrl Pts',(-23.0889961755581,-13.666829482395,
115.296986061293)) ;
#168553=CARTESIAN_POINT('Ctrl Pts',(-23.1628000187813,-13.6668294834514,
115.272755019008)) ;
#168554=CARTESIAN_POINT('Ctrl Pts',(-23.2366038620046,-13.6668294845077,
115.248523976722)) ;
#168555=CARTESIAN_POINT('Ctrl Pts',(-23.2595884754109,-13.6850524486487,
115.318531400582)) ;
#168556=CARTESIAN_POINT('Ctrl Pts',(-23.2825730888173,-13.7032754127896,
115.388538824441)) ;
#168557=CARTESIAN_POINT('Ctrl Pts',(-23.2087692455941,-13.7032754117333,
115.412769866726)) ;
#168558=CARTESIAN_POINT('Ctrl Pts',(-23.1349654023708,-13.7032754106769,
115.437000909011)) ;
#168559=CARTESIAN_POINT('Ctrl Pts',(-23.1119807889645,-13.685052446536,
115.366993485152)) ;
#168560=CARTESIAN_POINT('Ctrl Pts',(-23.0885048309624,-13.9562925901238,
115.259878332445)) ;
#168561=CARTESIAN_POINT('Ctrl Pts',(-23.0678620146304,-13.9191017880253,
115.197003644556)) ;
#168562=CARTESIAN_POINT('Ctrl Pts',(-23.1416658583648,-13.9191017857383,
115.172772603827)) ;
#168563=CARTESIAN_POINT('Ctrl Pts',(-23.2154697020991,-13.9191017834513,
115.148541563099)) ;
#168564=CARTESIAN_POINT('Ctrl Pts',(-23.236112518431,-13.9562925855498,
115.211416250988)) ;
#168565=CARTESIAN_POINT('Ctrl Pts',(-23.2567553347629,-13.9934833876483,
115.274290938878)) ;
#168566=CARTESIAN_POINT('Ctrl Pts',(-23.1829514910286,-13.9934833899353,
115.298521979606)) ;
#168567=CARTESIAN_POINT('Ctrl Pts',(-23.1091476472943,-13.9934833922223,
115.322753020334)) ;
#168568=CARTESIAN_POINT('Ctrl Pts',(-23.0885048309624,-13.9562925901238,
115.259878332445)) ;
#168569=CARTESIAN_POINT('Ctrl Pts',(-23.0439896792581,-14.1872893194723,
115.088901502234)) ;
#168570=CARTESIAN_POINT('Ctrl Pts',(-23.0271571303233,-14.1339131286007,
115.037632274036)) ;
#168571=CARTESIAN_POINT('Ctrl Pts',(-23.1009609744752,-14.1339131262424,
115.013401234579)) ;
#168572=CARTESIAN_POINT('Ctrl Pts',(-23.1747648186271,-14.1339131238842,
114.989170195123)) ;
#168573=CARTESIAN_POINT('Ctrl Pts',(-23.1915973675619,-14.1872893147558,
115.040439423321)) ;
#168574=CARTESIAN_POINT('Ctrl Pts',(-23.2084299164967,-14.2406655056274,
115.091708651519)) ;
#168575=CARTESIAN_POINT('Ctrl Pts',(-23.1346260723448,-14.2406655079856,
115.115939690975)) ;
#168576=CARTESIAN_POINT('Ctrl Pts',(-23.0608222281929,-14.2406655103439,
115.140170730432)) ;
#168577=CARTESIAN_POINT('Ctrl Pts',(-23.0439896792581,-14.1872893194723,
115.088901502234)) ;
#168578=CARTESIAN_POINT('Ctrl Pts',(-22.9823604254838,-14.3636852679792,
114.865766334949)) ;
#168579=CARTESIAN_POINT('Ctrl Pts',(-22.9705395949471,-14.2979128675593,
114.829761992371)) ;
#168580=CARTESIAN_POINT('Ctrl Pts',(-23.0443434390419,-14.2979128665308,
114.805530952741)) ;
#168581=CARTESIAN_POINT('Ctrl Pts',(-23.1181472831367,-14.2979128655022,
114.78129991311)) ;
#168582=CARTESIAN_POINT('Ctrl Pts',(-23.1299681136734,-14.3636852659222,
114.817304255688)) ;
#168583=CARTESIAN_POINT('Ctrl Pts',(-23.1417889442101,-14.4294576663421,
114.853308598265)) ;
#168584=CARTESIAN_POINT('Ctrl Pts',(-23.0679851001154,-14.4294576673706,
114.877539637896)) ;
#168585=CARTESIAN_POINT('Ctrl Pts',(-22.9941812560206,-14.4294576683991,
114.901770677526)) ;
#168586=CARTESIAN_POINT('Ctrl Pts',(-22.9823604254838,-14.3636852679792,
114.865766334949)) ;
#168587=CARTESIAN_POINT('Ctrl Pts',(-22.908524900711,-14.4725504618335,
114.605368957616)) ;
#168588=CARTESIAN_POINT('Ctrl Pts',(-22.9025772469157,-14.3990795841732,
114.587253363822)) ;
#168589=CARTESIAN_POINT('Ctrl Pts',(-22.9763810901088,-14.3990795846932,
114.563022321445)) ;
#168590=CARTESIAN_POINT('Ctrl Pts',(-23.0501849333019,-14.3990795852131,
114.538791279068)) ;
#168591=CARTESIAN_POINT('Ctrl Pts',(-23.0561325870972,-14.4725504628734,
114.556906872862)) ;
#168592=CARTESIAN_POINT('Ctrl Pts',(-23.0620802408925,-14.5460213405337,
114.575022466657)) ;
#168593=CARTESIAN_POINT('Ctrl Pts',(-22.9882763976994,-14.5460213400138,
114.599253509034)) ;
#168594=CARTESIAN_POINT('Ctrl Pts',(-22.9144725545063,-14.5460213394938,
114.623484551411)) ;
#168595=CARTESIAN_POINT('Ctrl Pts',(-22.908524900711,-14.4725504618335,
114.605368957616)) ;
#168596=CARTESIAN_POINT('Ctrl Pts',(-22.8289915160444,-14.505767100085,
114.327744641728)) ;
#168597=CARTESIAN_POINT('Ctrl Pts',(-22.8293207368645,-14.4298697296846,
114.328747395323)) ;
#168598=CARTESIAN_POINT('Ctrl Pts',(-22.903124578711,-14.429869730049,114.304516348845)) ;
#168599=CARTESIAN_POINT('Ctrl Pts',(-22.9769284205575,-14.4298697304134,
114.280285302366)) ;
#168600=CARTESIAN_POINT('Ctrl Pts',(-22.9765991997374,-14.5057671008138,
114.279282548771)) ;
#168601=CARTESIAN_POINT('Ctrl Pts',(-22.9762699789173,-14.5816644712143,
114.278279795176)) ;
#168602=CARTESIAN_POINT('Ctrl Pts',(-22.9024661370708,-14.5816644708498,
114.302510841654)) ;
#168603=CARTESIAN_POINT('Ctrl Pts',(-22.8286622952243,-14.5816644704854,
114.326741888133)) ;
#168604=CARTESIAN_POINT('Ctrl Pts',(-22.8289915160444,-14.505767100085,
114.327744641728)) ;
#168605=CARTESIAN_POINT('Ctrl Pts',(-22.7496283707013,-14.461184023194,
114.050502355121)) ;
#168606=CARTESIAN_POINT('Ctrl Pts',(-22.7562345239439,-14.388288943336,
114.070623632217)) ;
#168607=CARTESIAN_POINT('Ctrl Pts',(-22.8300383639314,-14.3882889407252,
114.046392580076)) ;
#168608=CARTESIAN_POINT('Ctrl Pts',(-22.9038422039188,-14.3882889381144,
114.022161527935)) ;
#168609=CARTESIAN_POINT('Ctrl Pts',(-22.8972360506762,-14.4611840179724,
114.002040250839)) ;
#168610=CARTESIAN_POINT('Ctrl Pts',(-22.8906298974336,-14.5340790978304,
113.981918973743)) ;
#168611=CARTESIAN_POINT('Ctrl Pts',(-22.8168260574461,-14.5340791004412,
114.006150025884)) ;
#168612=CARTESIAN_POINT('Ctrl Pts',(-22.7430222174587,-14.534079103052,
114.030381078025)) ;
#168613=CARTESIAN_POINT('Ctrl Pts',(-22.7496283707013,-14.461184023194,
114.050502355121)) ;
#168614=CARTESIAN_POINT('Ctrl Pts',(-22.6772956319986,-14.3417566878776,
113.794723577592)) ;
#168615=CARTESIAN_POINT('Ctrl Pts',(-22.6896957697514,-14.2770945733709,
113.832492396787)) ;
#168616=CARTESIAN_POINT('Ctrl Pts',(-22.7634996081967,-14.2770945642116,
113.808261339949)) ;
#168617=CARTESIAN_POINT('Ctrl Pts',(-22.837303446642,-14.2770945550524,
113.784030283111)) ;
#168618=CARTESIAN_POINT('Ctrl Pts',(-22.8249033088892,-14.3417566695591,
113.746261463916)) ;
#168619=CARTESIAN_POINT('Ctrl Pts',(-22.8125031711365,-14.4064187840659,
113.708492644721)) ;
#168620=CARTESIAN_POINT('Ctrl Pts',(-22.7386993326912,-14.4064187932251,
113.732723701559)) ;
#168621=CARTESIAN_POINT('Ctrl Pts',(-22.6648954942459,-14.4064188023844,
113.756954758397)) ;
#168622=CARTESIAN_POINT('Ctrl Pts',(-22.6772956319986,-14.3417566878776,
113.794723577592)) ;
#168623=CARTESIAN_POINT('Ctrl Pts',(-22.6178545187857,-14.1564991842471,
113.578251720131)) ;
#168624=CARTESIAN_POINT('Ctrl Pts',(-22.6351559129392,-14.104678506832,
113.630948975651)) ;
#168625=CARTESIAN_POINT('Ctrl Pts',(-22.7089597507266,-14.1046784883743,
113.60671791681)) ;
#168626=CARTESIAN_POINT('Ctrl Pts',(-22.7827635885141,-14.1046784699167,
113.582486857968)) ;
#168627=CARTESIAN_POINT('Ctrl Pts',(-22.7654621943605,-14.1564991473318,
113.529789602448)) ;
#168628=CARTESIAN_POINT('Ctrl Pts',(-22.748160800207,-14.208319824747,113.477092346927)) ;
#168629=CARTESIAN_POINT('Ctrl Pts',(-22.6743569624196,-14.2083198432046,
113.501323405769)) ;
#168630=CARTESIAN_POINT('Ctrl Pts',(-22.6005531246321,-14.2083198616622,
113.52555446461)) ;
#168631=CARTESIAN_POINT('Ctrl Pts',(-22.6178545187857,-14.1564991842471,
113.578251720131)) ;
#168632=CARTESIAN_POINT('Ctrl Pts',(-22.5761478520901,-13.9178865274089,
113.415717840721)) ;
#168633=CARTESIAN_POINT('Ctrl Pts',(-22.5971209446297,-13.8826509917796,
113.479598497267)) ;
#168634=CARTESIAN_POINT('Ctrl Pts',(-22.6709247828783,-13.8826509615156,
113.45536743983)) ;
#168635=CARTESIAN_POINT('Ctrl Pts',(-22.744728621127,-13.8826509312515,
113.431136382393)) ;
#168636=CARTESIAN_POINT('Ctrl Pts',(-22.7237555285874,-13.9178864668808,
113.367255725847)) ;
#168637=CARTESIAN_POINT('Ctrl Pts',(-22.7027824360478,-13.9531220025101,
113.303375069301)) ;
#168638=CARTESIAN_POINT('Ctrl Pts',(-22.6289785977992,-13.9531220327742,
113.327606126738)) ;
#168639=CARTESIAN_POINT('Ctrl Pts',(-22.5551747595505,-13.9531220630382,
113.351837184175)) ;
#168640=CARTESIAN_POINT('Ctrl Pts',(-22.5761478520901,-13.9178865274089,
113.415717840721)) ;
#168641=CARTESIAN_POINT('Ctrl Pts',(-22.5561014124412,-13.643415658276,
113.31916524184)) ;
#168642=CARTESIAN_POINT('Ctrl Pts',(-22.579238957361,-13.6272927364366,
113.389638471276)) ;
#168643=CARTESIAN_POINT('Ctrl Pts',(-22.6530427977317,-13.627292694101,
113.365407420303)) ;
#168644=CARTESIAN_POINT('Ctrl Pts',(-22.7268466381025,-13.6272926517654,
113.34117636933)) ;
#168645=CARTESIAN_POINT('Ctrl Pts',(-22.7037090931827,-13.6434155736048,
113.270703139894)) ;
#168646=CARTESIAN_POINT('Ctrl Pts',(-22.6805715482629,-13.6595384954442,
113.200229910458)) ;
#168647=CARTESIAN_POINT('Ctrl Pts',(-22.6067677078921,-13.6595385377798,
113.224460961431)) ;
#168648=CARTESIAN_POINT('Ctrl Pts',(-22.5329638675213,-13.6595385801154,
113.248692012404)) ;
#168649=CARTESIAN_POINT('Ctrl Pts',(-22.5561014124412,-13.643415658276,
113.31916524184)) ;
#168650=CARTESIAN_POINT('Ctrl Pts',(-22.5598524729045,-13.3531854263633,
113.295142705237)) ;
#168651=CARTESIAN_POINT('Ctrl Pts',(-22.5834950317507,-13.3573028544331,
113.367154125775)) ;
#168652=CARTESIAN_POINT('Ctrl Pts',(-22.6572988758986,-13.3573028025058,
113.342923086306)) ;
#168653=CARTESIAN_POINT('Ctrl Pts',(-22.7311027200465,-13.3573027505784,
113.318692046837)) ;
#168654=CARTESIAN_POINT('Ctrl Pts',(-22.7074601612002,-13.3531853225086,
113.2466806263)) ;
#168655=CARTESIAN_POINT('Ctrl Pts',(-22.683817602354,-13.3490678944388,
113.174669205762)) ;
#168656=CARTESIAN_POINT('Ctrl Pts',(-22.6100137582061,-13.3490679463661,
113.198900245231)) ;
#168657=CARTESIAN_POINT('Ctrl Pts',(-22.5362099140582,-13.3490679982935,
113.2231312847)) ;
#168658=CARTESIAN_POINT('Ctrl Pts',(-22.5598524729045,-13.3531854263633,
113.295142705237)) ;
#168659=CARTESIAN_POINT('Ctrl Pts',(-22.5878485384446,-13.0673885224611,
113.344945022211)) ;
#168660=CARTESIAN_POINT('Ctrl Pts',(-22.6103045670656,-13.0914657876093,
113.413342463295)) ;
#168661=CARTESIAN_POINT('Ctrl Pts',(-22.6841084163441,-13.0914657299476,
113.389111439454)) ;
#168662=CARTESIAN_POINT('Ctrl Pts',(-22.7579122656227,-13.0914656722859,
113.364880415613)) ;
#168663=CARTESIAN_POINT('Ctrl Pts',(-22.7354562370017,-13.0673884071377,
113.296482974528)) ;
#168664=CARTESIAN_POINT('Ctrl Pts',(-22.7130002083808,-13.0433111419895,
113.228085533443)) ;
#168665=CARTESIAN_POINT('Ctrl Pts',(-22.6391963591022,-13.0433111996512,
113.252316557285)) ;
#168666=CARTESIAN_POINT('Ctrl Pts',(-22.5653925098236,-13.0433112573129,
113.276547581126)) ;
#168667=CARTESIAN_POINT('Ctrl Pts',(-22.5878485384446,-13.0673885224611,
113.344945022211)) ;
#168668=CARTESIAN_POINT('Ctrl Pts',(-22.6389570341485,-12.8066409255768,
113.465116760669)) ;
#168669=CARTESIAN_POINT('Ctrl Pts',(-22.6586117821665,-12.8489579270799,
113.524981953187)) ;
#168670=CARTESIAN_POINT('Ctrl Pts',(-22.7324156375432,-12.8489578695406,
113.50075094792)) ;
#168671=CARTESIAN_POINT('Ctrl Pts',(-22.8062194929197,-12.8489578120014,
113.476519942652)) ;
#168672=CARTESIAN_POINT('Ctrl Pts',(-22.7865647449017,-12.8066408104982,
113.416654750134)) ;
#168673=CARTESIAN_POINT('Ctrl Pts',(-22.7669099968836,-12.7643238089951,
113.356789557615)) ;
#168674=CARTESIAN_POINT('Ctrl Pts',(-22.693106141507,-12.7643238665344,
113.381020562883)) ;
#168675=CARTESIAN_POINT('Ctrl Pts',(-22.6193022861304,-12.7643239240736,
113.405251568151)) ;
#168676=CARTESIAN_POINT('Ctrl Pts',(-22.6389570341485,-12.8066409255768,
113.465116760669)) ;
#168677=CARTESIAN_POINT('Ctrl Pts',(-22.7097903100766,-12.5904014103484,
113.645526694695)) ;
#168678=CARTESIAN_POINT('Ctrl Pts',(-22.7252592148691,-12.6478767369269,
113.692642484262)) ;
#168679=CARTESIAN_POINT('Ctrl Pts',(-22.7990630761565,-12.6478766870741,
113.668411496998)) ;
#168680=CARTESIAN_POINT('Ctrl Pts',(-22.872866937444,-12.6478766372212,
113.644180509733)) ;
#168681=CARTESIAN_POINT('Ctrl Pts',(-22.8573980326515,-12.5904013106426,
113.597064720167)) ;
#168682=CARTESIAN_POINT('Ctrl Pts',(-22.8419291278591,-12.5329259840641,
113.5499489306)) ;
#168683=CARTESIAN_POINT('Ctrl Pts',(-22.7681252665716,-12.5329260339169,
113.574179917864)) ;
#168684=CARTESIAN_POINT('Ctrl Pts',(-22.6943214052842,-12.5329260837698,
113.598410905129)) ;
#168685=CARTESIAN_POINT('Ctrl Pts',(-22.7097903100766,-12.5904014103484,
113.645526694695)) ;
#168686=CARTESIAN_POINT('Ctrl Pts',(-22.7973377104979,-12.4318423089519,
113.876458241546)) ;
#168687=CARTESIAN_POINT('Ctrl Pts',(-22.807456155429,-12.500471718984,113.907277393848)) ;
#168688=CARTESIAN_POINT('Ctrl Pts',(-22.8812600228401,-12.5004716824447,
113.883046425235)) ;
#168689=CARTESIAN_POINT('Ctrl Pts',(-22.9550638902512,-12.5004716459054,
113.858815456623)) ;
#168690=CARTESIAN_POINT('Ctrl Pts',(-22.94494544532,-12.4318422358733,113.827996304321)) ;
#168691=CARTESIAN_POINT('Ctrl Pts',(-22.9348270003888,-12.3632128258413,
113.797177152019)) ;
#168692=CARTESIAN_POINT('Ctrl Pts',(-22.8610231329778,-12.3632128623805,
113.821408120632)) ;
#168693=CARTESIAN_POINT('Ctrl Pts',(-22.7872192655667,-12.3632128989198,
113.845639089245)) ;
#168694=CARTESIAN_POINT('Ctrl Pts',(-22.7973377104979,-12.4318423089519,
113.876458241546)) ;
#168695=CARTESIAN_POINT('Ctrl Pts',(-22.8940411989731,-12.3456712150683,
114.135732174982)) ;
#168696=CARTESIAN_POINT('Ctrl Pts',(-22.8981525025119,-12.4204161323536,
114.148254543946)) ;
#168697=CARTESIAN_POINT('Ctrl Pts',(-22.9719563736072,-12.4204161168077,
114.124023586555)) ;
#168698=CARTESIAN_POINT('Ctrl Pts',(-23.0457602447025,-12.4204161012619,
114.099792629164)) ;
#168699=CARTESIAN_POINT('Ctrl Pts',(-23.0416489411638,-12.3456711839767,
114.0872702602)) ;
#168700=CARTESIAN_POINT('Ctrl Pts',(-23.037537637625,-12.2709262666914,
114.074747891236)) ;
#168701=CARTESIAN_POINT('Ctrl Pts',(-22.9637337665296,-12.2709262822373,
114.098978848627)) ;
#168702=CARTESIAN_POINT('Ctrl Pts',(-22.8899298954343,-12.2709262977831,
114.123209806018)) ;
#168703=CARTESIAN_POINT('Ctrl Pts',(-22.8940411989731,-12.3456712150683,
114.135732174982)) ;
#168704=CARTESIAN_POINT('Ctrl Pts',(-22.9953415992751,-12.3353742164119,
114.408800882689)) ;
#168705=CARTESIAN_POINT('Ctrl Pts',(-22.9931205397198,-12.4109469942247,
114.402035895503)) ;
#168706=CARTESIAN_POINT('Ctrl Pts',(-23.0669244128859,-12.4109470032869,
114.377804944419)) ;
#168707=CARTESIAN_POINT('Ctrl Pts',(-23.1407282860521,-12.410947012349,
114.353573993335)) ;
#168708=CARTESIAN_POINT('Ctrl Pts',(-23.1429493456074,-12.3353742345363,
114.360338980522)) ;
#168709=CARTESIAN_POINT('Ctrl Pts',(-23.1451704051626,-12.2598014567236,
114.367103967708)) ;
#168710=CARTESIAN_POINT('Ctrl Pts',(-23.0713665319965,-12.2598014476614,
114.391334918792)) ;
#168711=CARTESIAN_POINT('Ctrl Pts',(-22.9975626588303,-12.2598014385992,
114.415565869876)) ;
#168712=CARTESIAN_POINT('Ctrl Pts',(-22.9953415992751,-12.3353742164119,
114.408800882689)) ;
#168713=CARTESIAN_POINT('Ctrl Pts',(-23.0941945934012,-12.402733699683,
114.674438282461)) ;
#168714=CARTESIAN_POINT('Ctrl Pts',(-23.0858023223332,-12.473714122898,
114.648876780817)) ;
#168715=CARTESIAN_POINT('Ctrl Pts',(-23.1596061950238,-12.4737141587005,
114.624645828285)) ;
#168716=CARTESIAN_POINT('Ctrl Pts',(-23.2334100677144,-12.473714194503,
114.600414875753)) ;
#168717=CARTESIAN_POINT('Ctrl Pts',(-23.2418023387824,-12.402733771288,
114.625976377397)) ;
#168718=CARTESIAN_POINT('Ctrl Pts',(-23.2501946098504,-12.331753348073,
114.651537879041)) ;
#168719=CARTESIAN_POINT('Ctrl Pts',(-23.1763907371598,-12.3317533122705,
114.675768831573)) ;
#168720=CARTESIAN_POINT('Ctrl Pts',(-23.1025868644692,-12.331753276468,
114.699999784105)) ;
#168721=CARTESIAN_POINT('Ctrl Pts',(-23.0941945934012,-12.402733699683,
114.674438282461)) ;
#168722=CARTESIAN_POINT('Ctrl Pts',(-23.1845580290586,-12.5432714498278,
114.914111547974)) ;
#168723=CARTESIAN_POINT('Ctrl Pts',(-23.1705803992153,-12.6045444668254,
114.871537944772)) ;
#168724=CARTESIAN_POINT('Ctrl Pts',(-23.244384268865,-12.6045445287426,
114.847306982978)) ;
#168725=CARTESIAN_POINT('Ctrl Pts',(-23.3181881385147,-12.6045445906598,
114.823076021184)) ;
#168726=CARTESIAN_POINT('Ctrl Pts',(-23.332165768358,-12.5432715736621,
114.865649624386)) ;
#168727=CARTESIAN_POINT('Ctrl Pts',(-23.3461433982013,-12.4819985566645,
114.908223227588)) ;
#168728=CARTESIAN_POINT('Ctrl Pts',(-23.2723395285516,-12.4819984947474,
114.932454189382)) ;
#168729=CARTESIAN_POINT('Ctrl Pts',(-23.1985356589018,-12.4819984328302,
114.956685151176)) ;
#168730=CARTESIAN_POINT('Ctrl Pts',(-23.1845580290586,-12.5432714498278,
114.914111547974)) ;
#168731=CARTESIAN_POINT('Ctrl Pts',(-23.2601807339086,-12.7462375607508,
115.108986544249)) ;
#168732=CARTESIAN_POINT('Ctrl Pts',(-23.2416365667801,-12.7934303811122,
115.052504005331)) ;
#168733=CARTESIAN_POINT('Ctrl Pts',(-23.3154404307945,-12.7934304650843,
115.028273026373)) ;
#168734=CARTESIAN_POINT('Ctrl Pts',(-23.3892442948089,-12.7934305490564,
115.004042047414)) ;
#168735=CARTESIAN_POINT('Ctrl Pts',(-23.4077884619374,-12.746237728695,
115.060524586332)) ;
#168736=CARTESIAN_POINT('Ctrl Pts',(-23.4263326290658,-12.6990449083337,
115.11700712525)) ;
#168737=CARTESIAN_POINT('Ctrl Pts',(-23.3525287650514,-12.6990448243616,
115.141238104209)) ;
#168738=CARTESIAN_POINT('Ctrl Pts',(-23.278724901037,-12.6990447403895,
115.165469083167)) ;
#168739=CARTESIAN_POINT('Ctrl Pts',(-23.2601807339086,-12.7462375607508,
115.108986544249)) ;
#168740=CARTESIAN_POINT('Ctrl Pts',(-23.3166354321301,-12.9968255702811,
115.245531849597)) ;
#168741=CARTESIAN_POINT('Ctrl Pts',(-23.2948551085598,-13.0265927652578,
115.179192500334)) ;
#168742=CARTESIAN_POINT('Ctrl Pts',(-23.368658965033,-13.0265928649381,
115.154961498407)) ;
#168743=CARTESIAN_POINT('Ctrl Pts',(-23.4424628215062,-13.0265929646183,
115.130730496479)) ;
#168744=CARTESIAN_POINT('Ctrl Pts',(-23.4642431450764,-12.9968257696416,
115.197069845742)) ;
#168745=CARTESIAN_POINT('Ctrl Pts',(-23.4860234686466,-12.9670585746648,
115.263409195005)) ;
#168746=CARTESIAN_POINT('Ctrl Pts',(-23.4122196121735,-12.9670584749846,
115.287640196933)) ;
#168747=CARTESIAN_POINT('Ctrl Pts',(-23.3384157557003,-12.9670583753043,
115.31187119886)) ;
#168748=CARTESIAN_POINT('Ctrl Pts',(-23.3166354321301,-12.9968255702811,
115.245531849597)) ;
#168749=CARTESIAN_POINT('Ctrl Pts',(-23.3507793496113,-13.2777710794654,
115.314086325876)) ;
#168750=CARTESIAN_POINT('Ctrl Pts',(-23.3273163717843,-13.2879677234676,
115.242621883247)) ;
#168751=CARTESIAN_POINT('Ctrl Pts',(-23.4011202195342,-13.2879678309871,
115.21839085475)) ;
#168752=CARTESIAN_POINT('Ctrl Pts',(-23.474924067284,-13.2879679385065,
115.194159826252)) ;
#168753=CARTESIAN_POINT('Ctrl Pts',(-23.498387045111,-13.2777712945044,
115.26562426888)) ;
#168754=CARTESIAN_POINT('Ctrl Pts',(-23.521850022938,-13.2675746505022,
115.337088711509)) ;
#168755=CARTESIAN_POINT('Ctrl Pts',(-23.4480461751882,-13.2675745429828,
115.361319740006)) ;
#168756=CARTESIAN_POINT('Ctrl Pts',(-23.3742423274384,-13.2675744354633,
115.385550768504)) ;
#168757=CARTESIAN_POINT('Ctrl Pts',(-23.3507793496113,-13.2777710794654,
115.314086325876)) ;
#168758=CARTESIAN_POINT('Ctrl Pts',(-23.3608646469754,-13.5692121151867,
115.309310772099)) ;
#168759=CARTESIAN_POINT('Ctrl Pts',(-23.3373971099136,-13.5590766136152,
115.23783244276)) ;
#168760=CARTESIAN_POINT('Ctrl Pts',(-23.4112009485982,-13.5590767201184,
115.213601386652)) ;
#168761=CARTESIAN_POINT('Ctrl Pts',(-23.4850047872827,-13.5590768266217,
115.189370330543)) ;
#168762=CARTESIAN_POINT('Ctrl Pts',(-23.5084723243445,-13.5692123281932,
115.260848659881)) ;
#168763=CARTESIAN_POINT('Ctrl Pts',(-23.5319398614064,-13.5793478297647,
115.332326989219)) ;
#168764=CARTESIAN_POINT('Ctrl Pts',(-23.4581360227218,-13.5793477232615,
115.356558045328)) ;
#168765=CARTESIAN_POINT('Ctrl Pts',(-23.3843321840373,-13.5793476167582,
115.380789101437)) ;
#168766=CARTESIAN_POINT('Ctrl Pts',(-23.3608646469754,-13.5692121151867,
115.309310772099)) ;
#168767=CARTESIAN_POINT('Ctrl Pts',(-23.3467205470048,-13.8503430324929,
115.230657743514)) ;
#168768=CARTESIAN_POINT('Ctrl Pts',(-23.3249414773231,-13.8205648157971,
115.164322213335)) ;
#168769=CARTESIAN_POINT('Ctrl Pts',(-23.3987453076205,-13.8205649121888,
115.140091131681)) ;
#168770=CARTESIAN_POINT('Ctrl Pts',(-23.4725491379179,-13.8205650085804,
115.115860050026)) ;
#168771=CARTESIAN_POINT('Ctrl Pts',(-23.4943282075997,-13.8503432252762,
115.182195580204)) ;
#168772=CARTESIAN_POINT('Ctrl Pts',(-23.5161072772814,-13.880121441972,
115.248531110382)) ;
#168773=CARTESIAN_POINT('Ctrl Pts',(-23.442303446984,-13.8801213455804,
115.272762192037)) ;
#168774=CARTESIAN_POINT('Ctrl Pts',(-23.3684996166866,-13.8801212491888,
115.296993273692)) ;
#168775=CARTESIAN_POINT('Ctrl Pts',(-23.3467205470048,-13.8503430324929,
115.230657743514)) ;
#168776=CARTESIAN_POINT('Ctrl Pts',(-23.3104950812117,-14.0986233529731,
115.085011079683)) ;
#168777=CARTESIAN_POINT('Ctrl Pts',(-23.2919434103993,-14.0514664875456,
115.028505685671)) ;
#168778=CARTESIAN_POINT('Ctrl Pts',(-23.3657472337263,-14.0514665673178,
115.004274582785)) ;
#168779=CARTESIAN_POINT('Ctrl Pts',(-23.4395510570533,-14.05146664709,114.9800434799)) ;
#168780=CARTESIAN_POINT('Ctrl Pts',(-23.4581027278657,-14.0986235125175,
115.036548873912)) ;
#168781=CARTESIAN_POINT('Ctrl Pts',(-23.4766543986781,-14.145780377945,
115.093054267924)) ;
#168782=CARTESIAN_POINT('Ctrl Pts',(-23.4028505753511,-14.1457802981728,
115.11728537081)) ;
#168783=CARTESIAN_POINT('Ctrl Pts',(-23.3290467520241,-14.1457802184006,
115.141516473695)) ;
#168784=CARTESIAN_POINT('Ctrl Pts',(-23.3104950812117,-14.0986233529731,
115.085011079683)) ;
#168785=CARTESIAN_POINT('Ctrl Pts',(-23.2552110709686,-14.2995832696182,
114.881140254992)) ;
#168786=CARTESIAN_POINT('Ctrl Pts',(-23.2412255998243,-14.2383253097085,
114.838542768335)) ;
#168787=CARTESIAN_POINT('Ctrl Pts',(-23.315029418276,-14.2383253669594,
114.8143116506)) ;
#168788=CARTESIAN_POINT('Ctrl Pts',(-23.3888332367278,-14.2383254242103,
114.790080532865)) ;
#168789=CARTESIAN_POINT('Ctrl Pts',(-23.402818707872,-14.29958338412,114.832678019522)) ;
#168790=CARTESIAN_POINT('Ctrl Pts',(-23.4168041790163,-14.3608413440297,
114.875275506179)) ;
#168791=CARTESIAN_POINT('Ctrl Pts',(-23.3430003605645,-14.3608412867788,
114.899506623914)) ;
#168792=CARTESIAN_POINT('Ctrl Pts',(-23.2691965421128,-14.3608412295279,
114.923737741649)) ;
#168793=CARTESIAN_POINT('Ctrl Pts',(-23.2552110709686,-14.2995832696182,
114.881140254992)) ;
#168794=CARTESIAN_POINT('Ctrl Pts',(-23.1854571810787,-14.4373031232107,
114.633125479994)) ;
#168795=CARTESIAN_POINT('Ctrl Pts',(-23.1770564137006,-14.3663375815008,
114.607538099809)) ;
#168796=CARTESIAN_POINT('Ctrl Pts',(-23.2508602299918,-14.3663376133963,
114.583306975493)) ;
#168797=CARTESIAN_POINT('Ctrl Pts',(-23.3246640462829,-14.3663376452917,
114.559075851177)) ;
#168798=CARTESIAN_POINT('Ctrl Pts',(-23.3330648136609,-14.4373031870016,
114.584663231363)) ;
#168799=CARTESIAN_POINT('Ctrl Pts',(-23.341465581039,-14.5082687287115,
114.610250611548)) ;
#168800=CARTESIAN_POINT('Ctrl Pts',(-23.2676617647479,-14.5082686968161,
114.634481735864)) ;
#168801=CARTESIAN_POINT('Ctrl Pts',(-23.1938579484568,-14.5082686649206,
114.65871286018)) ;
#168802=CARTESIAN_POINT('Ctrl Pts',(-23.1854571810787,-14.4373031232107,
114.633125479994)) ;
#168803=CARTESIAN_POINT('Ctrl Pts',(-23.1076519671601,-14.5016051754735,
114.360797992838)) ;
#168804=CARTESIAN_POINT('Ctrl Pts',(-23.1054022061001,-14.4260436157556,
114.353945585335)) ;
#168805=CARTESIAN_POINT('Ctrl Pts',(-23.1792060223591,-14.4260436229732,
114.329714460921)) ;
#168806=CARTESIAN_POINT('Ctrl Pts',(-23.2530098386182,-14.4260436301907,
114.305483336507)) ;
#168807=CARTESIAN_POINT('Ctrl Pts',(-23.2552595996782,-14.5016051899087,
114.31233574401)) ;
#168808=CARTESIAN_POINT('Ctrl Pts',(-23.2575093607382,-14.5771667496267,
114.319188151513)) ;
#168809=CARTESIAN_POINT('Ctrl Pts',(-23.1837055444792,-14.5771667424091,
114.343419275927)) ;
#168810=CARTESIAN_POINT('Ctrl Pts',(-23.1099017282202,-14.5771667351915,
114.367650400341)) ;
#168811=CARTESIAN_POINT('Ctrl Pts',(-23.1076519671601,-14.5016051754735,
114.360797992838)) ;
#168812=CARTESIAN_POINT('Ctrl Pts',(-23.0272520332699,-14.4885235205326,
114.080367454721)) ;
#168813=CARTESIAN_POINT('Ctrl Pts',(-23.031347792647,-14.4137610040608,
114.092842478479)) ;
#168814=CARTESIAN_POINT('Ctrl Pts',(-23.1051516115704,-14.4137609891403,
114.06861136218)) ;
#168815=CARTESIAN_POINT('Ctrl Pts',(-23.1789554304938,-14.4137609742198,
114.044380245882)) ;
#168816=CARTESIAN_POINT('Ctrl Pts',(-23.1748596711167,-14.4885234906916,
114.031905222124)) ;
#168817=CARTESIAN_POINT('Ctrl Pts',(-23.1707639117397,-14.5632860071634,
114.019430198366)) ;
#168818=CARTESIAN_POINT('Ctrl Pts',(-23.0969600928162,-14.5632860220839,
114.043661314664)) ;
#168819=CARTESIAN_POINT('Ctrl Pts',(-23.0231562738928,-14.5632860370044,
114.067892430963)) ;
#168820=CARTESIAN_POINT('Ctrl Pts',(-23.0272520332699,-14.4885235205326,
114.080367454721)) ;
#168821=CARTESIAN_POINT('Ctrl Pts',(-22.9514685700045,-14.3988909925641,
113.814136978792)) ;
#168822=CARTESIAN_POINT('Ctrl Pts',(-22.9615943154396,-14.3302736656516,
113.844978367012)) ;
#168823=CARTESIAN_POINT('Ctrl Pts',(-23.0353981384749,-14.3302736334562,
113.820747263238)) ;
#168824=CARTESIAN_POINT('Ctrl Pts',(-23.1092019615102,-14.3302736012609,
113.796516159463)) ;
#168825=CARTESIAN_POINT('Ctrl Pts',(-23.0990762160752,-14.3988909281734,
113.765674771244)) ;
#168826=CARTESIAN_POINT('Ctrl Pts',(-23.0889504706401,-14.4675082550859,
113.734833383024)) ;
#168827=CARTESIAN_POINT('Ctrl Pts',(-23.0151466476048,-14.4675082872812,
113.759064486798)) ;
#168828=CARTESIAN_POINT('Ctrl Pts',(-22.9413428245695,-14.4675083194766,
113.783295590572)) ;
#168829=CARTESIAN_POINT('Ctrl Pts',(-22.9514685700045,-14.3988909925641,
113.814136978792)) ;
#168830=CARTESIAN_POINT('Ctrl Pts',(-22.8859156809784,-14.2382785177405,
113.578895834363)) ;
#168831=CARTESIAN_POINT('Ctrl Pts',(-22.9013699117956,-14.1807709154062,
113.625966929132)) ;
#168832=CARTESIAN_POINT('Ctrl Pts',(-22.9751737403754,-14.180770872992,
113.601735842246)) ;
#168833=CARTESIAN_POINT('Ctrl Pts',(-23.0489775689551,-14.1807708305777,
113.577504755359)) ;
#168834=CARTESIAN_POINT('Ctrl Pts',(-23.0335233381379,-14.2382784329119,
113.53043366059)) ;
#168835=CARTESIAN_POINT('Ctrl Pts',(-23.0180691073207,-14.2957860352462,
113.483362565821)) ;
#168836=CARTESIAN_POINT('Ctrl Pts',(-22.9442652787409,-14.2957860776604,
113.507593652707)) ;
#168837=CARTESIAN_POINT('Ctrl Pts',(-22.8704614501611,-14.2957861200747,
113.531824739594)) ;
#168838=CARTESIAN_POINT('Ctrl Pts',(-22.8859156809784,-14.2382785177405,
113.578895834363)) ;
#168839=CARTESIAN_POINT('Ctrl Pts',(-22.8366909878539,-14.0201835577284,
113.393629387852)) ;
#168840=CARTESIAN_POINT('Ctrl Pts',(-22.8563366770582,-13.9778166138277,
113.453466988439)) ;
#168841=CARTESIAN_POINT('Ctrl Pts',(-22.9301405109221,-13.9778165664169,
113.429235917646)) ;
#168842=CARTESIAN_POINT('Ctrl Pts',(-23.003944344786,-13.9778165190061,
113.405004846854)) ;
#168843=CARTESIAN_POINT('Ctrl Pts',(-22.9842986555816,-14.0201834629068,
113.345167246267)) ;
#168844=CARTESIAN_POINT('Ctrl Pts',(-22.9646529663773,-14.0625504068075,
113.28532964568)) ;
#168845=CARTESIAN_POINT('Ctrl Pts',(-22.8908491325134,-14.0625504542183,
113.309560716472)) ;
#168846=CARTESIAN_POINT('Ctrl Pts',(-22.8170452986496,-14.0625505016291,
113.333791787265)) ;
#168847=CARTESIAN_POINT('Ctrl Pts',(-22.8366909878539,-14.0201835577284,
113.393629387852)) ;
#168848=CARTESIAN_POINT('Ctrl Pts',(-22.8074315802463,-13.7575805640437,
113.268949038296)) ;
#168849=CARTESIAN_POINT('Ctrl Pts',(-22.829885948188,-13.7334844884055,
113.337341420952)) ;
#168850=CARTESIAN_POINT('Ctrl Pts',(-22.9036897872937,-13.7334844436557,
113.313110366126)) ;
#168851=CARTESIAN_POINT('Ctrl Pts',(-22.9774936263994,-13.7334843989059,
113.288879311299)) ;
#168852=CARTESIAN_POINT('Ctrl Pts',(-22.9550392584577,-13.7575804745442,
113.220486928643)) ;
#168853=CARTESIAN_POINT('Ctrl Pts',(-22.9325848905159,-13.7816765501825,
113.152094545987)) ;
#168854=CARTESIAN_POINT('Ctrl Pts',(-22.8587810514102,-13.7816765949322,
113.176325600813)) ;
#168855=CARTESIAN_POINT('Ctrl Pts',(-22.7849772123045,-13.781676639682,
113.20055665564)) ;
#168856=CARTESIAN_POINT('Ctrl Pts',(-22.8074315802463,-13.7575805640437,
113.268949038296)) ;
#168857=CARTESIAN_POINT('Ctrl Pts',(-22.8014281414069,-13.4715356144856,
113.215234575554)) ;
#168858=CARTESIAN_POINT('Ctrl Pts',(-22.8250688612617,-13.467375361388,
113.287240394559)) ;
#168859=CARTESIAN_POINT('Ctrl Pts',(-22.8988727043007,-13.4673753229371,
113.263009351712)) ;
#168860=CARTESIAN_POINT('Ctrl Pts',(-22.9726765473396,-13.4673752844861,
113.238778308866)) ;
#168861=CARTESIAN_POINT('Ctrl Pts',(-22.9490358274848,-13.4715355375837,
113.166772489861)) ;
#168862=CARTESIAN_POINT('Ctrl Pts',(-22.92539510763,-13.4756957906813,113.094766670856)) ;
#168863=CARTESIAN_POINT('Ctrl Pts',(-22.8515912645911,-13.4756958291323,
113.118997713702)) ;
#168864=CARTESIAN_POINT('Ctrl Pts',(-22.7777874215521,-13.4756958675833,
113.143228756549)) ;
#168865=CARTESIAN_POINT('Ctrl Pts',(-22.8014281414069,-13.4715356144856,
113.215234575554)) ;
#168866=CARTESIAN_POINT('Ctrl Pts',(-22.8195788653586,-13.1815808813972,
113.235079702884)) ;
#168867=CARTESIAN_POINT('Ctrl Pts',(-22.8427214378284,-13.1976597435624,
113.30556824517)) ;
#168868=CARTESIAN_POINT('Ctrl Pts',(-22.9165252835433,-13.1976597143198,
113.281337210474)) ;
#168869=CARTESIAN_POINT('Ctrl Pts',(-22.9903291292582,-13.1976596850772,
113.257106175778)) ;
#168870=CARTESIAN_POINT('Ctrl Pts',(-22.9671865567883,-13.1815808229121,
113.186617633492)) ;
#168871=CARTESIAN_POINT('Ctrl Pts',(-22.9440439843185,-13.1655019607469,
113.116129091206)) ;
#168872=CARTESIAN_POINT('Ctrl Pts',(-22.8702401386036,-13.1655019899895,
113.140360125902)) ;
#168873=CARTESIAN_POINT('Ctrl Pts',(-22.7964362928887,-13.1655020192321,
113.164591160598)) ;
#168874=CARTESIAN_POINT('Ctrl Pts',(-22.8195788653586,-13.1815808813972,
113.235079702884)) ;
#168875=CARTESIAN_POINT('Ctrl Pts',(-22.8617885311853,-12.9071949482228,
113.328012511746)) ;
#168876=CARTESIAN_POINT('Ctrl Pts',(-22.8827563840684,-12.9424572144763,
113.391877208875)) ;
#168877=CARTESIAN_POINT('Ctrl Pts',(-22.9565602306879,-12.9424571966172,
113.367646176935)) ;
#168878=CARTESIAN_POINT('Ctrl Pts',(-23.0303640773074,-12.9424571787581,
113.343415144994)) ;
#168879=CARTESIAN_POINT('Ctrl Pts',(-23.0093962244244,-12.9071949125046,
113.279550447865)) ;
#168880=CARTESIAN_POINT('Ctrl Pts',(-22.9884283715413,-12.8719326462511,
113.215685750736)) ;
#168881=CARTESIAN_POINT('Ctrl Pts',(-22.9146245249218,-12.8719326641102,
113.239916782676)) ;
#168882=CARTESIAN_POINT('Ctrl Pts',(-22.8408206783023,-12.8719326819694,
113.264147814617)) ;
#168883=CARTESIAN_POINT('Ctrl Pts',(-22.8617885311853,-12.9071949482228,
113.328012511746)) ;
#168884=CARTESIAN_POINT('Ctrl Pts',(-22.9249619978587,-12.6718251326146,
113.485139268914)) ;
#168885=CARTESIAN_POINT('Ctrl Pts',(-22.9422806312259,-12.723574947821,
113.537889032084)) ;
#168886=CARTESIAN_POINT('Ctrl Pts',(-23.0160844779008,-12.7235749374657,
113.513658000312)) ;
#168887=CARTESIAN_POINT('Ctrl Pts',(-23.0898883245757,-12.7235749271105,
113.48942696854)) ;
#168888=CARTESIAN_POINT('Ctrl Pts',(-23.0725696912085,-12.6718251119041,
113.43667720537)) ;
#168889=CARTESIAN_POINT('Ctrl Pts',(-23.0552510578412,-12.6200752966978,
113.3839274422)) ;
#168890=CARTESIAN_POINT('Ctrl Pts',(-22.9814472111664,-12.620075307053,
113.408158473972)) ;
#168891=CARTESIAN_POINT('Ctrl Pts',(-22.9076433644914,-12.6200753174082,
113.432389505744)) ;
#168892=CARTESIAN_POINT('Ctrl Pts',(-22.9249619978587,-12.6718251326146,
113.485139268914)) ;
#168893=CARTESIAN_POINT('Ctrl Pts',(-23.0059942336063,-12.4884732056212,
113.696495324864)) ;
#168894=CARTESIAN_POINT('Ctrl Pts',(-23.0184146037982,-12.553103678643,
113.734325768607)) ;
#168895=CARTESIAN_POINT('Ctrl Pts',(-23.0922184494783,-12.5531036749217,
113.710094733805)) ;
#168896=CARTESIAN_POINT('Ctrl Pts',(-23.1660222951584,-12.5531036712005,
113.685863699003)) ;
#168897=CARTESIAN_POINT('Ctrl Pts',(-23.1536019249665,-12.4884731981787,
113.64803325526)) ;
#168898=CARTESIAN_POINT('Ctrl Pts',(-23.1411815547745,-12.4238427251569,
113.610202811517)) ;
#168899=CARTESIAN_POINT('Ctrl Pts',(-23.0673777090945,-12.4238427288782,
113.634433846319)) ;
#168900=CARTESIAN_POINT('Ctrl Pts',(-22.9935738634144,-12.4238427325995,
113.658664881121)) ;
#168901=CARTESIAN_POINT('Ctrl Pts',(-23.0059942336063,-12.4884732056212,
113.696495324864)) ;
#168902=CARTESIAN_POINT('Ctrl Pts',(-23.1000078654876,-12.3715751089405,
113.947282082598)) ;
#168903=CARTESIAN_POINT('Ctrl Pts',(-23.1066182036233,-12.4444657268571,
113.967416106029)) ;
#168904=CARTESIAN_POINT('Ctrl Pts',(-23.1804220477466,-12.4444657266469,
113.943185066485)) ;
#168905=CARTESIAN_POINT('Ctrl Pts',(-23.2542258918699,-12.4444657264366,
113.918954026941)) ;
#168906=CARTESIAN_POINT('Ctrl Pts',(-23.2476155537342,-12.3715751085199,
113.89882000351)) ;
#168907=CARTESIAN_POINT('Ctrl Pts',(-23.2410052155985,-12.2986844906033,
113.878685980079)) ;
#168908=CARTESIAN_POINT('Ctrl Pts',(-23.1672013714752,-12.2986844908136,
113.902917019623)) ;
#168909=CARTESIAN_POINT('Ctrl Pts',(-23.0933975273519,-12.2986844910239,
113.927148059167)) ;
#168910=CARTESIAN_POINT('Ctrl Pts',(-23.1000078654876,-12.3715751089405,
113.947282082598)) ;
#168911=CARTESIAN_POINT('Ctrl Pts',(-23.2003199061484,-12.3301226383043,
114.217388478731)) ;
#168912=CARTESIAN_POINT('Ctrl Pts',(-23.2006687533814,-12.4060167548224,
114.218451011093)) ;
#168913=CARTESIAN_POINT('Ctrl Pts',(-23.2744725964053,-12.4060167550604,
114.1942199682)) ;
#168914=CARTESIAN_POINT('Ctrl Pts',(-23.3482764394292,-12.4060167552985,
114.169988925308)) ;
#168915=CARTESIAN_POINT('Ctrl Pts',(-23.3479275921962,-12.3301226387804,
114.168926392946)) ;
#168916=CARTESIAN_POINT('Ctrl Pts',(-23.3475787449632,-12.2542285222622,
114.167863860585)) ;
#168917=CARTESIAN_POINT('Ctrl Pts',(-23.2737749019393,-12.2542285220242,
114.192094903477)) ;
#168918=CARTESIAN_POINT('Ctrl Pts',(-23.1999710589154,-12.2542285217862,
114.216325946369)) ;
#168919=CARTESIAN_POINT('Ctrl Pts',(-23.2003199061484,-12.3301226383043,
114.217388478731)) ;
#168920=CARTESIAN_POINT('Ctrl Pts',(-23.3007380070665,-12.3662578527564,
114.487855727773)) ;
#168921=CARTESIAN_POINT('Ctrl Pts',(-23.2948077898911,-12.4397415757967,
114.469793243034)) ;
#168922=CARTESIAN_POINT('Ctrl Pts',(-23.3686116323531,-12.4397415751055,
114.44556219843)) ;
#168923=CARTESIAN_POINT('Ctrl Pts',(-23.4424154748152,-12.4397415744144,
114.421331153827)) ;
#168924=CARTESIAN_POINT('Ctrl Pts',(-23.4483456919906,-12.366257851374,
114.439393638566)) ;
#168925=CARTESIAN_POINT('Ctrl Pts',(-23.454275909166,-12.2927741283337,
114.457456123305)) ;
#168926=CARTESIAN_POINT('Ctrl Pts',(-23.3804720667039,-12.2927741290249,
114.481687167909)) ;
#168927=CARTESIAN_POINT('Ctrl Pts',(-23.3066682242419,-12.2927741297161,
114.505918212512)) ;
#168928=CARTESIAN_POINT('Ctrl Pts',(-23.3007380070665,-12.3662578527564,
114.487855727773)) ;
#168929=CARTESIAN_POINT('Ctrl Pts',(-23.3952053708607,-12.4776432814408,
114.740115458462)) ;
#168930=CARTESIAN_POINT('Ctrl Pts',(-23.3834038459423,-12.5434578807603,
114.704169917668)) ;
#168931=CARTESIAN_POINT('Ctrl Pts',(-23.4572076885097,-12.5434578790229,
114.679938873385)) ;
#168932=CARTESIAN_POINT('Ctrl Pts',(-23.5310115310771,-12.5434578772856,
114.655707829103)) ;
#168933=CARTESIAN_POINT('Ctrl Pts',(-23.5428130559955,-12.477643277966,
114.691653369897)) ;
#168934=CARTESIAN_POINT('Ctrl Pts',(-23.5546145809139,-12.4118286786465,
114.727598910691)) ;
#168935=CARTESIAN_POINT('Ctrl Pts',(-23.4808107383465,-12.4118286803839,
114.751829954974)) ;
#168936=CARTESIAN_POINT('Ctrl Pts',(-23.4070068957792,-12.4118286821212,
114.776060999257)) ;
#168937=CARTESIAN_POINT('Ctrl Pts',(-23.3952053708607,-12.4776432814408,
114.740115458462)) ;
#168938=CARTESIAN_POINT('Ctrl Pts',(-23.4777530924333,-12.6576066827307,
114.955900577125)) ;
#168939=CARTESIAN_POINT('Ctrl Pts',(-23.460907482304,-12.71095179343,114.904591566696)) ;
#168940=CARTESIAN_POINT('Ctrl Pts',(-23.5347113257398,-12.7109517930547,
114.880360525058)) ;
#168941=CARTESIAN_POINT('Ctrl Pts',(-23.6085151691756,-12.7109517926794,
114.856129483421)) ;
#168942=CARTESIAN_POINT('Ctrl Pts',(-23.6253607793049,-12.6576066819802,
114.907438493849)) ;
#168943=CARTESIAN_POINT('Ctrl Pts',(-23.6422063894341,-12.604261571281,
114.958747504278)) ;
#168944=CARTESIAN_POINT('Ctrl Pts',(-23.5684025459984,-12.6042615716562,
114.982978545915)) ;
#168945=CARTESIAN_POINT('Ctrl Pts',(-23.4945987025626,-12.6042615720315,
115.007209587553)) ;
#168946=CARTESIAN_POINT('Ctrl Pts',(-23.4777530924333,-12.6576066827307,
114.955900577125)) ;
#168947=CARTESIAN_POINT('Ctrl Pts',(-23.5422559394209,-12.8904240369604,
115.117024877862)) ;
#168948=CARTESIAN_POINT('Ctrl Pts',(-23.5216131954621,-12.9275904125638,
115.054150410526)) ;
#168949=CARTESIAN_POINT('Ctrl Pts',(-23.5954170395086,-12.9275904154763,
115.029919370748)) ;
#168950=CARTESIAN_POINT('Ctrl Pts',(-23.6692208835552,-12.9275904183888,
115.005688330971)) ;
#168951=CARTESIAN_POINT('Ctrl Pts',(-23.689863627514,-12.8904240427854,
115.068562798306)) ;
#168952=CARTESIAN_POINT('Ctrl Pts',(-23.7105063714728,-12.853257667182,
115.131437265642)) ;
#168953=CARTESIAN_POINT('Ctrl Pts',(-23.6367025274263,-12.8532576642695,
115.15566830542)) ;
#168954=CARTESIAN_POINT('Ctrl Pts',(-23.5628986833797,-12.853257661357,
115.179899345197)) ;
#168955=CARTESIAN_POINT('Ctrl Pts',(-23.5422559394209,-12.8904240369604,
115.117024877862)) ;
#168956=CARTESIAN_POINT('Ctrl Pts',(-23.5857808510703,-13.1612401483887,
115.214177425736)) ;
#168957=CARTESIAN_POINT('Ctrl Pts',(-23.5628018590313,-13.1795510816038,
115.144187123799)) ;
#168958=CARTESIAN_POINT('Ctrl Pts',(-23.6366057032453,-13.1795510898929,
115.119956084532)) ;
#168959=CARTESIAN_POINT('Ctrl Pts',(-23.7104095474593,-13.1795510981819,
115.095725045265)) ;
#168960=CARTESIAN_POINT('Ctrl Pts',(-23.7333885394984,-13.1612401649668,
115.165715347201)) ;
#168961=CARTESIAN_POINT('Ctrl Pts',(-23.7563675315375,-13.1429292317516,
115.235705649138)) ;
#168962=CARTESIAN_POINT('Ctrl Pts',(-23.6825636873234,-13.1429292234626,
115.259936688406)) ;
#168963=CARTESIAN_POINT('Ctrl Pts',(-23.6087598431094,-13.1429292151735,
115.284167727673)) ;
#168964=CARTESIAN_POINT('Ctrl Pts',(-23.5857808510703,-13.1612401483887,
115.214177425736)) ;
#168965=CARTESIAN_POINT('Ctrl Pts',(-23.6057316422003,-13.4512163582634,
115.239436705029)) ;
#168966=CARTESIAN_POINT('Ctrl Pts',(-23.5820609538197,-13.4493066869731,
115.167339607776)) ;
#168967=CARTESIAN_POINT('Ctrl Pts',(-23.6558647972831,-13.4493067026551,
115.143108566222)) ;
#168968=CARTESIAN_POINT('Ctrl Pts',(-23.7296686407465,-13.4493067183372,
115.118877524669)) ;
#168969=CARTESIAN_POINT('Ctrl Pts',(-23.7533393291271,-13.4512163896275,
115.190974621922)) ;
#168970=CARTESIAN_POINT('Ctrl Pts',(-23.7770100175077,-13.4531260609178,
115.263071719175)) ;
#168971=CARTESIAN_POINT('Ctrl Pts',(-23.7032061740443,-13.4531260452357,
115.287302760728)) ;
#168972=CARTESIAN_POINT('Ctrl Pts',(-23.6294023305809,-13.4531260295536,
115.311533802282)) ;
#168973=CARTESIAN_POINT('Ctrl Pts',(-23.6057316422003,-13.4512163582634,
115.239436705029)) ;
#168974=CARTESIAN_POINT('Ctrl Pts',(-23.6013424516955,-13.7384260494091,
115.190608267416)) ;
#168975=CARTESIAN_POINT('Ctrl Pts',(-23.5786776934113,-13.7164599573725,
115.121575071076)) ;
#168976=CARTESIAN_POINT('Ctrl Pts',(-23.6524815348966,-13.7164599797673,
115.097344023498)) ;
#168977=CARTESIAN_POINT('Ctrl Pts',(-23.726285376382,-13.7164600021621,
115.073112975919)) ;
#168978=CARTESIAN_POINT('Ctrl Pts',(-23.7489501346663,-13.7384260941987,
115.142146172259)) ;
#168979=CARTESIAN_POINT('Ctrl Pts',(-23.7716148929505,-13.7603921862353,
115.211179368599)) ;
#168980=CARTESIAN_POINT('Ctrl Pts',(-23.6978110514652,-13.7603921638405,
115.235410416177)) ;
#168981=CARTESIAN_POINT('Ctrl Pts',(-23.6240072099798,-13.7603921414456,
115.259641463756)) ;
#168982=CARTESIAN_POINT('Ctrl Pts',(-23.6013424516955,-13.7384260494091,
115.190608267416)) ;
#168983=CARTESIAN_POINT('Ctrl Pts',(-23.5737147002099,-14.0027479972631,
115.070987295502)) ;
#168984=CARTESIAN_POINT('Ctrl Pts',(-23.5536801496635,-13.9622948022858,
115.009965287708)) ;
#168985=CARTESIAN_POINT('Ctrl Pts',(-23.6274839879841,-13.962294829201,
114.985734230491)) ;
#168986=CARTESIAN_POINT('Ctrl Pts',(-23.7012878263047,-13.9622948561163,
114.961503173273)) ;
#168987=CARTESIAN_POINT('Ctrl Pts',(-23.7213223768512,-14.0027480510937,
115.022525181066)) ;
#168988=CARTESIAN_POINT('Ctrl Pts',(-23.7413569273976,-14.0432012460711,
115.08354718886)) ;
#168989=CARTESIAN_POINT('Ctrl Pts',(-23.667553089077,-14.0432012191558,
115.107778246078)) ;
#168990=CARTESIAN_POINT('Ctrl Pts',(-23.5937492507564,-14.0432011922405,
115.132009303295)) ;
#168991=CARTESIAN_POINT('Ctrl Pts',(-23.5737147002099,-14.0027479972631,
115.070987295502)) ;
#168992=CARTESIAN_POINT('Ctrl Pts',(-23.5256807526921,-14.2248634912547,
114.889270709179)) ;
#168993=CARTESIAN_POINT('Ctrl Pts',(-23.5097038108168,-14.1688437545673,
114.840607522861)) ;
#168994=CARTESIAN_POINT('Ctrl Pts',(-23.583507645237,-14.1688437816251,
114.816376453763)) ;
#168995=CARTESIAN_POINT('Ctrl Pts',(-23.6573114796572,-14.168843808683,
114.792145384665)) ;
#168996=CARTESIAN_POINT('Ctrl Pts',(-23.6732884215325,-14.2248635453705,
114.840808570983)) ;
#168997=CARTESIAN_POINT('Ctrl Pts',(-23.6892653634078,-14.2808832820579,
114.889471757302)) ;
#168998=CARTESIAN_POINT('Ctrl Pts',(-23.6154615289876,-14.2808832550001,
114.913702826399)) ;
#168999=CARTESIAN_POINT('Ctrl Pts',(-23.5416576945674,-14.2808832279422,
114.937933895497)) ;
#169000=CARTESIAN_POINT('Ctrl Pts',(-23.5256807526921,-14.2248634912547,
114.889270709179)) ;
#169001=CARTESIAN_POINT('Ctrl Pts',(-23.461215966023,-14.3897502001773,
114.657418556327)) ;
#169002=CARTESIAN_POINT('Ctrl Pts',(-23.4504514511971,-14.3221371212432,
114.624631581955)) ;
#169003=CARTESIAN_POINT('Ctrl Pts',(-23.5242552811751,-14.3221371438564,
114.600400499327)) ;
#169004=CARTESIAN_POINT('Ctrl Pts',(-23.5980591111531,-14.3221371664696,
114.576169416699)) ;
#169005=CARTESIAN_POINT('Ctrl Pts',(-23.6088236259791,-14.3897502454037,
114.608956391071)) ;
#169006=CARTESIAN_POINT('Ctrl Pts',(-23.619588140805,-14.4573633243378,
114.641743365443)) ;
#169007=CARTESIAN_POINT('Ctrl Pts',(-23.545784310827,-14.4573633017246,
114.665974448071)) ;
#169008=CARTESIAN_POINT('Ctrl Pts',(-23.471980480849,-14.4573632791114,
114.690205530699)) ;
#169009=CARTESIAN_POINT('Ctrl Pts',(-23.461215966023,-14.3897502001773,
114.657418556327)) ;
#169010=CARTESIAN_POINT('Ctrl Pts',(-23.3857401849695,-14.4847583322739,
114.392013776167)) ;
#169011=CARTESIAN_POINT('Ctrl Pts',(-23.3809646627516,-14.4104140333925,
114.377468307136)) ;
#169012=CARTESIAN_POINT('Ctrl Pts',(-23.4547684885272,-14.4104140454356,
114.353237211708)) ;
#169013=CARTESIAN_POINT('Ctrl Pts',(-23.5285723143027,-14.4104140574787,
114.32900611628)) ;
#169014=CARTESIAN_POINT('Ctrl Pts',(-23.5333478365205,-14.4847583563601,
114.343551585311)) ;
#169015=CARTESIAN_POINT('Ctrl Pts',(-23.5381233587383,-14.5591026552415,
114.358097054342)) ;
#169016=CARTESIAN_POINT('Ctrl Pts',(-23.4643195329628,-14.5591026431984,
114.38232814977)) ;
#169017=CARTESIAN_POINT('Ctrl Pts',(-23.3905157071873,-14.5591026311553,
114.406559245198)) ;
#169018=CARTESIAN_POINT('Ctrl Pts',(-23.3857401849695,-14.4847583322739,
114.392013776167)) ;
#169019=CARTESIAN_POINT('Ctrl Pts',(-23.3057972119039,-14.5032991769,114.113141625194)) ;
#169020=CARTESIAN_POINT('Ctrl Pts',(-23.3073283222928,-14.4275531479525,
114.117805141659)) ;
#169021=CARTESIAN_POINT('Ctrl Pts',(-23.3811321453339,-14.4275531440522,
114.093574037902)) ;
#169022=CARTESIAN_POINT('Ctrl Pts',(-23.454935968375,-14.427553140152,114.069342934146)) ;
#169023=CARTESIAN_POINT('Ctrl Pts',(-23.4534048579861,-14.5032991690996,
114.064679417681)) ;
#169024=CARTESIAN_POINT('Ctrl Pts',(-23.4518737475972,-14.5790451980471,
114.060015901216)) ;
#169025=CARTESIAN_POINT('Ctrl Pts',(-23.3780699245561,-14.5790452019473,
114.084247004972)) ;
#169026=CARTESIAN_POINT('Ctrl Pts',(-23.304266101515,-14.5790452058476,
114.108478108729)) ;
#169027=CARTESIAN_POINT('Ctrl Pts',(-23.3057972119039,-14.5032991769,114.113141625194)) ;
#169028=CARTESIAN_POINT('Ctrl Pts',(-23.2272555357364,-14.4441301859155,
113.838399442431)) ;
#169029=CARTESIAN_POINT('Ctrl Pts',(-23.2350073561252,-14.3724053611762,
113.862010238012)) ;
#169030=CARTESIAN_POINT('Ctrl Pts',(-23.3088111777221,-14.3724053372545,
113.837779129857)) ;
#169031=CARTESIAN_POINT('Ctrl Pts',(-23.382614999319,-14.3724053133327,
113.813548021702)) ;
#169032=CARTESIAN_POINT('Ctrl Pts',(-23.3748631789302,-14.444130138072,
113.789937226121)) ;
#169033=CARTESIAN_POINT('Ctrl Pts',(-23.3671113585414,-14.5158549628113,
113.76632643054)) ;
#169034=CARTESIAN_POINT('Ctrl Pts',(-23.2933075369445,-14.5158549867331,
113.790557538695)) ;
#169035=CARTESIAN_POINT('Ctrl Pts',(-23.2195037153477,-14.5158550106548,
113.81478864685)) ;
#169036=CARTESIAN_POINT('Ctrl Pts',(-23.2272555357364,-14.4441301859155,
113.838399442431)) ;
#169037=CARTESIAN_POINT('Ctrl Pts',(-23.1569464450254,-14.3114937407021,
113.588802208014)) ;
#169038=CARTESIAN_POINT('Ctrl Pts',(-23.1703517418229,-14.2489252476856,
113.629632580692)) ;
#169039=CARTESIAN_POINT('Ctrl Pts',(-23.2441555643269,-14.2489252018326,
113.6054014753)) ;
#169040=CARTESIAN_POINT('Ctrl Pts',(-23.317959386831,-14.2489251559797,
113.581170369907)) ;
#169041=CARTESIAN_POINT('Ctrl Pts',(-23.3045540900335,-14.3114936489961,
113.54033999723)) ;
#169042=CARTESIAN_POINT('Ctrl Pts',(-23.2911487932361,-14.3740621420126,
113.499509624552)) ;
#169043=CARTESIAN_POINT('Ctrl Pts',(-23.217344970732,-14.3740621878656,
113.523740729944)) ;
#169044=CARTESIAN_POINT('Ctrl Pts',(-23.143541148228,-14.3740622337185,
113.547971835337)) ;
#169045=CARTESIAN_POINT('Ctrl Pts',(-23.1569464450254,-14.3114937407021,
113.588802208014)) ;
#169046=CARTESIAN_POINT('Ctrl Pts',(-23.1004490169695,-14.114774307687,
113.381241689025)) ;
#169047=CARTESIAN_POINT('Ctrl Pts',(-23.118552366844,-14.0658491597741,
113.43638157348)) ;
#169048=CARTESIAN_POINT('Ctrl Pts',(-23.1923561925365,-14.0658490924885,
113.412150477799)) ;
#169049=CARTESIAN_POINT('Ctrl Pts',(-23.2661600182289,-14.0658490252028,
113.387919382118)) ;
#169050=CARTESIAN_POINT('Ctrl Pts',(-23.2480566683545,-14.1147741731156,
113.332779497664)) ;
#169051=CARTESIAN_POINT('Ctrl Pts',(-23.22995331848,-14.1636993210285,113.277639613209)) ;
#169052=CARTESIAN_POINT('Ctrl Pts',(-23.1561494927875,-14.1636993883142,
113.30187070889)) ;
#169053=CARTESIAN_POINT('Ctrl Pts',(-23.082345667095,-14.1636994555999,
113.326101804571)) ;
#169054=CARTESIAN_POINT('Ctrl Pts',(-23.1004490169695,-14.114774307687,
113.381241689025)) ;
#169055=CARTESIAN_POINT('Ctrl Pts',(-23.062667902268,-13.8682921869894,
113.230716909827)) ;
#169056=CARTESIAN_POINT('Ctrl Pts',(-23.0841688593971,-13.8365043277557,
113.296205357889)) ;
#169057=CARTESIAN_POINT('Ctrl Pts',(-23.1579726905666,-13.8365042424835,
113.271974278891)) ;
#169058=CARTESIAN_POINT('Ctrl Pts',(-23.2317765217361,-13.8365041572113,
113.247743199892)) ;
#169059=CARTESIAN_POINT('Ctrl Pts',(-23.210275564607,-13.868292016445,113.182254751829)) ;
#169060=CARTESIAN_POINT('Ctrl Pts',(-23.1887746074778,-13.9000798756787,
113.116766303766)) ;
#169061=CARTESIAN_POINT('Ctrl Pts',(-23.1149707763083,-13.9000799609509,
113.140997382765)) ;
#169062=CARTESIAN_POINT('Ctrl Pts',(-23.0411669451388,-13.9000800462231,
113.165228461764)) ;
#169063=CARTESIAN_POINT('Ctrl Pts',(-23.062667902268,-13.8682921869894,
113.230716909827)) ;
#169064=CARTESIAN_POINT('Ctrl Pts',(-23.046982381011,-13.5896536678714,
113.147496899994)) ;
#169065=CARTESIAN_POINT('Ctrl Pts',(-23.0703432142598,-13.5772729173919,
113.218650230723)) ;
#169066=CARTESIAN_POINT('Ctrl Pts',(-23.1441470526942,-13.5772728198901,
113.194419173852)) ;
#169067=CARTESIAN_POINT('Ctrl Pts',(-23.2179508911286,-13.5772727223883,
113.170188116981)) ;
#169068=CARTESIAN_POINT('Ctrl Pts',(-23.1945900578798,-13.5896534728677,
113.099034786252)) ;
#169069=CARTESIAN_POINT('Ctrl Pts',(-23.1712292246311,-13.6020342233472,
113.027881455524)) ;
#169070=CARTESIAN_POINT('Ctrl Pts',(-23.0974253861966,-13.6020343208491,
113.052112512395)) ;
#169071=CARTESIAN_POINT('Ctrl Pts',(-23.0236215477622,-13.6020344183509,
113.076343569266)) ;
#169072=CARTESIAN_POINT('Ctrl Pts',(-23.046982381011,-13.5896536678714,
113.147496899994)) ;
#169073=CARTESIAN_POINT('Ctrl Pts',(-23.0553081301007,-13.2982167701219,
113.137350825504)) ;
#169074=CARTESIAN_POINT('Ctrl Pts',(-23.0788565858859,-13.3061648042617,
113.209075624288)) ;
#169075=CARTESIAN_POINT('Ctrl Pts',(-23.1526604327469,-13.3061647018305,
113.184844593083)) ;
#169076=CARTESIAN_POINT('Ctrl Pts',(-23.2264642796078,-13.3061645993992,
113.160613561877)) ;
#169077=CARTESIAN_POINT('Ctrl Pts',(-23.2029158238225,-13.2982165652594,
113.088888763094)) ;
#169078=CARTESIAN_POINT('Ctrl Pts',(-23.1793673680372,-13.2902685311196,
113.01716396431)) ;
#169079=CARTESIAN_POINT('Ctrl Pts',(-23.1055635211763,-13.2902686335509,
113.041394995515)) ;
#169080=CARTESIAN_POINT('Ctrl Pts',(-23.0317596743153,-13.2902687359821,
113.06562602672)) ;
#169081=CARTESIAN_POINT('Ctrl Pts',(-23.0553081301007,-13.2982167701219,
113.137350825504)) ;
#169082=CARTESIAN_POINT('Ctrl Pts',(-23.0878545163832,-13.0155927262678,
113.201000676988)) ;
#169083=CARTESIAN_POINT('Ctrl Pts',(-23.1098994771013,-13.0432841492844,
113.268146072441)) ;
#169084=CARTESIAN_POINT('Ctrl Pts',(-23.183703332692,-13.0432840507906,
113.243915067826)) ;
#169085=CARTESIAN_POINT('Ctrl Pts',(-23.2575071882827,-13.0432839522968,
113.21968406321)) ;
#169086=CARTESIAN_POINT('Ctrl Pts',(-23.2354622275647,-13.0155925292803,
113.152538667757)) ;
#169087=CARTESIAN_POINT('Ctrl Pts',(-23.2134172668467,-12.9879011062637,
113.085393272303)) ;
#169088=CARTESIAN_POINT('Ctrl Pts',(-23.1396134112559,-12.9879012047575,
113.109624276918)) ;
#169089=CARTESIAN_POINT('Ctrl Pts',(-23.0658095556652,-12.9879013032513,
113.133855281534)) ;
#169090=CARTESIAN_POINT('Ctrl Pts',(-23.0878545163832,-13.0155927262678,
113.201000676988)) ;
#169091=CARTESIAN_POINT('Ctrl Pts',(-23.1427829186928,-12.7625129426041,
113.33292942976)) ;
#169092=CARTESIAN_POINT('Ctrl Pts',(-23.1617573175269,-12.8079141772025,
113.390722389181)) ;
#169093=CARTESIAN_POINT('Ctrl Pts',(-23.235561181146,-12.8079140912617,
113.366491409019)) ;
#169094=CARTESIAN_POINT('Ctrl Pts',(-23.3093650447651,-12.8079140053209,
113.342260428856)) ;
#169095=CARTESIAN_POINT('Ctrl Pts',(-23.290390645931,-12.7625127707225,
113.284467469435)) ;
#169096=CARTESIAN_POINT('Ctrl Pts',(-23.2714162470969,-12.7171115361241,
113.226674510015)) ;
#169097=CARTESIAN_POINT('Ctrl Pts',(-23.1976123834778,-12.7171116220649,
113.250905490177)) ;
#169098=CARTESIAN_POINT('Ctrl Pts',(-23.1238085198587,-12.7171117080057,
113.275136470339)) ;
#169099=CARTESIAN_POINT('Ctrl Pts',(-23.1427829186928,-12.7625129426041,
113.33292942976)) ;
#169100=CARTESIAN_POINT('Ctrl Pts',(-23.2173049964885,-12.5553594059935,
113.524403018202)) ;
#169101=CARTESIAN_POINT('Ctrl Pts',(-23.231839369238,-12.6152904005215,
113.568672374581)) ;
#169102=CARTESIAN_POINT('Ctrl Pts',(-23.3056432394893,-12.6152903344179,
113.54444141462)) ;
#169103=CARTESIAN_POINT('Ctrl Pts',(-23.3794471097407,-12.6152902683143,
113.520210454658)) ;
#169104=CARTESIAN_POINT('Ctrl Pts',(-23.3649127369912,-12.5553592737864,
113.475941098278)) ;
#169105=CARTESIAN_POINT('Ctrl Pts',(-23.3503783642417,-12.4954282792585,
113.431671741899)) ;
#169106=CARTESIAN_POINT('Ctrl Pts',(-23.2765744939903,-12.4954283453621,
113.45590270186)) ;
#169107=CARTESIAN_POINT('Ctrl Pts',(-23.202770623739,-12.4954284114656,
113.480133661822)) ;
#169108=CARTESIAN_POINT('Ctrl Pts',(-23.2173049964885,-12.5553594059935,
113.524403018202)) ;
#169109=CARTESIAN_POINT('Ctrl Pts',(-23.3068806905073,-12.4101759250027,
113.761668971239)) ;
#169110=CARTESIAN_POINT('Ctrl Pts',(-23.3159187908398,-12.4803322250042,
113.789197568645)) ;
#169111=CARTESIAN_POINT('Ctrl Pts',(-23.3897226654383,-12.4803321844946,
113.764966621924)) ;
#169112=CARTESIAN_POINT('Ctrl Pts',(-23.4635265400367,-12.4803321439849,
113.740735675203)) ;
#169113=CARTESIAN_POINT('Ctrl Pts',(-23.4544884397042,-12.4101758439834,
113.713207077797)) ;
#169114=CARTESIAN_POINT('Ctrl Pts',(-23.4454503393718,-12.3400195439819,
113.685678480392)) ;
#169115=CARTESIAN_POINT('Ctrl Pts',(-23.3716464647733,-12.3400195844916,
113.709909427113)) ;
#169116=CARTESIAN_POINT('Ctrl Pts',(-23.2978425901748,-12.3400196250012,
113.734140373834)) ;
#169117=CARTESIAN_POINT('Ctrl Pts',(-23.3068806905073,-12.4101759250027,
113.761668971239)) ;
#169118=CARTESIAN_POINT('Ctrl Pts',(-23.405005780283,-12.3376963152453,
114.025199960178)) ;
#169119=CARTESIAN_POINT('Ctrl Pts',(-23.4079377709915,-12.4130169374688,
114.034130332859)) ;
#169120=CARTESIAN_POINT('Ctrl Pts',(-23.4817416473952,-12.4130169250925,
114.009899391637)) ;
#169121=CARTESIAN_POINT('Ctrl Pts',(-23.5555455237989,-12.4130169127163,
113.985668450414)) ;
#169122=CARTESIAN_POINT('Ctrl Pts',(-23.5526135330904,-12.3376962904928,
113.976738077733)) ;
#169123=CARTESIAN_POINT('Ctrl Pts',(-23.5496815423819,-12.2623756682694,
113.967807705051)) ;
#169124=CARTESIAN_POINT('Ctrl Pts',(-23.4758776659782,-12.2623756806456,
113.992038646274)) ;
#169125=CARTESIAN_POINT('Ctrl Pts',(-23.4020737895745,-12.2623756930219,
114.016269587496)) ;
#169126=CARTESIAN_POINT('Ctrl Pts',(-23.405005780283,-12.3376963152453,
114.025199960178)) ;
#169127=CARTESIAN_POINT('Ctrl Pts',(-23.5066801809222,-12.3422639933637,
114.299298215706)) ;
#169128=CARTESIAN_POINT('Ctrl Pts',(-23.5032543515753,-12.4173784848516,
114.28886369427)) ;
#169129=CARTESIAN_POINT('Ctrl Pts',(-23.577058226874,-12.4173785007626,
114.264632749682)) ;
#169130=CARTESIAN_POINT('Ctrl Pts',(-23.6508621021727,-12.4173785166736,
114.240401805094)) ;
#169131=CARTESIAN_POINT('Ctrl Pts',(-23.6542879315196,-12.3422640251856,
114.25083632653)) ;
#169132=CARTESIAN_POINT('Ctrl Pts',(-23.6577137608664,-12.2671495336977,
114.261270847965)) ;
#169133=CARTESIAN_POINT('Ctrl Pts',(-23.5839098855678,-12.2671495177867,
114.285501792553)) ;
#169134=CARTESIAN_POINT('Ctrl Pts',(-23.5101060102691,-12.2671495018757,
114.309732737142)) ;
#169135=CARTESIAN_POINT('Ctrl Pts',(-23.5066801809222,-12.3422639933637,
114.299298215706)) ;
#169136=CARTESIAN_POINT('Ctrl Pts',(-23.6043850261139,-12.4243537888734,
114.561410934724)) ;
#169137=CARTESIAN_POINT('Ctrl Pts',(-23.5948667124673,-12.4938495197523,
114.532419689052)) ;
#169138=CARTESIAN_POINT('Ctrl Pts',(-23.6686705841451,-12.4938495605533,
114.508188733435)) ;
#169139=CARTESIAN_POINT('Ctrl Pts',(-23.7424744558228,-12.4938496013543,
114.483957777818)) ;
#169140=CARTESIAN_POINT('Ctrl Pts',(-23.7519927694694,-12.4243538704754,
114.51294902349)) ;
#169141=CARTESIAN_POINT('Ctrl Pts',(-23.761511083116,-12.3548581395965,
114.541940269163)) ;
#169142=CARTESIAN_POINT('Ctrl Pts',(-23.6877072114382,-12.3548580987955,
114.56617122478)) ;
#169143=CARTESIAN_POINT('Ctrl Pts',(-23.6139033397605,-12.3548580579945,
114.590402180397)) ;
#169144=CARTESIAN_POINT('Ctrl Pts',(-23.6043850261139,-12.4243537888734,
114.561410934724)) ;
#169145=CARTESIAN_POINT('Ctrl Pts',(-23.6917800294508,-12.5764990896273,
114.7923054574)) ;
#169146=CARTESIAN_POINT('Ctrl Pts',(-23.6768761024066,-12.6354761389067,
114.746910502209)) ;
#169147=CARTESIAN_POINT('Ctrl Pts',(-23.7506799687729,-12.6354761997948,
114.722679530414)) ;
#169148=CARTESIAN_POINT('Ctrl Pts',(-23.8244838351391,-12.6354762606829,
114.698448558619)) ;
#169149=CARTESIAN_POINT('Ctrl Pts',(-23.8393877621834,-12.5764992114035,
114.74384351381)) ;
#169150=CARTESIAN_POINT('Ctrl Pts',(-23.8542916892276,-12.5175221621241,
114.789238469001)) ;
#169151=CARTESIAN_POINT('Ctrl Pts',(-23.7804878228613,-12.517522101236,
114.813469440796)) ;
#169152=CARTESIAN_POINT('Ctrl Pts',(-23.7066839564951,-12.5175220403479,
114.837700412591)) ;
#169153=CARTESIAN_POINT('Ctrl Pts',(-23.6917800294508,-12.5764990896273,
114.7923054574)) ;
#169154=CARTESIAN_POINT('Ctrl Pts',(-23.7643708740628,-12.7898749801387,
114.977872887432)) ;
#169155=CARTESIAN_POINT('Ctrl Pts',(-23.7451115981193,-12.8340435200322,
114.91921224211)) ;
#169156=CARTESIAN_POINT('Ctrl Pts',(-23.8189154574709,-12.834043593478,
114.894981248949)) ;
#169157=CARTESIAN_POINT('Ctrl Pts',(-23.8927193168225,-12.8340436669238,
114.870750255788)) ;
#169158=CARTESIAN_POINT('Ctrl Pts',(-23.9119785927659,-12.7898751270303,
114.92941090111)) ;
#169159=CARTESIAN_POINT('Ctrl Pts',(-23.9312378687094,-12.7457065871368,
114.988071546433)) ;
#169160=CARTESIAN_POINT('Ctrl Pts',(-23.8574340093578,-12.745706513691,
115.012302539593)) ;
#169161=CARTESIAN_POINT('Ctrl Pts',(-23.7836301500062,-12.7457064402452,
115.036533532754)) ;
#169162=CARTESIAN_POINT('Ctrl Pts',(-23.7643708740628,-12.7898749801387,
114.977872887432)) ;
#169163=CARTESIAN_POINT('Ctrl Pts',(-23.8170503352041,-13.0489854290901,
115.102740722146)) ;
#169164=CARTESIAN_POINT('Ctrl Pts',(-23.7948202389745,-13.0751301371368,
115.035031437426)) ;
#169165=CARTESIAN_POINT('Ctrl Pts',(-23.8686240908392,-13.0751302144171,
115.010800421462)) ;
#169166=CARTESIAN_POINT('Ctrl Pts',(-23.942427942704,-13.0751302916973,
114.986569405497)) ;
#169167=CARTESIAN_POINT('Ctrl Pts',(-23.9646580389336,-13.0489855836505,
115.054278690217)) ;
#169168=CARTESIAN_POINT('Ctrl Pts',(-23.9868881351632,-13.0228408756037,
115.121987974937)) ;
#169169=CARTESIAN_POINT('Ctrl Pts',(-23.9130842832985,-13.0228407983235,
115.146218990902)) ;
#169170=CARTESIAN_POINT('Ctrl Pts',(-23.8392804314337,-13.0228407210433,
115.170450006866)) ;
#169171=CARTESIAN_POINT('Ctrl Pts',(-23.8170503352041,-13.0489854290901,
115.102740722146)) ;
#169172=CARTESIAN_POINT('Ctrl Pts',(-23.8466050136932,-13.3335116646803,
115.157315047406)) ;
#169173=CARTESIAN_POINT('Ctrl Pts',(-23.8230112672121,-13.3398303944034,
115.085452303904)) ;
#169174=CARTESIAN_POINT('Ctrl Pts',(-23.8968151122376,-13.3398304688619,
115.061221267108)) ;
#169175=CARTESIAN_POINT('Ctrl Pts',(-23.970618957263,-13.3398305433204,
115.036990230313)) ;
#169176=CARTESIAN_POINT('Ctrl Pts',(-23.994212703744,-13.3335118135973,
115.108852973814)) ;
#169177=CARTESIAN_POINT('Ctrl Pts',(-24.0178064502251,-13.3271930838743,
115.180715717316)) ;
#169178=CARTESIAN_POINT('Ctrl Pts',(-23.9440026051996,-13.3271930094158,
115.204946754112)) ;
#169179=CARTESIAN_POINT('Ctrl Pts',(-23.8701987601742,-13.3271929349573,
115.229177790907)) ;
#169180=CARTESIAN_POINT('Ctrl Pts',(-23.8466050136932,-13.3335116646803,
115.157315047406)) ;
#169181=CARTESIAN_POINT('Ctrl Pts',(-23.8520217309769,-13.6230727255243,
115.138490203622)) ;
#169182=CARTESIAN_POINT('Ctrl Pts',(-23.8287451419027,-13.6091838535946,
115.06759347028)) ;
#169183=CARTESIAN_POINT('Ctrl Pts',(-23.9025489811084,-13.6091839202508,
115.043362415759)) ;
#169184=CARTESIAN_POINT('Ctrl Pts',(-23.9763528203141,-13.6091839869071,
115.019131361237)) ;
#169185=CARTESIAN_POINT('Ctrl Pts',(-23.9996294093884,-13.6230728588367,
115.090028094579)) ;
#169186=CARTESIAN_POINT('Ctrl Pts',(-24.0229059984626,-13.6369617307664,
115.160924827921)) ;
#169187=CARTESIAN_POINT('Ctrl Pts',(-23.9491021592569,-13.6369616641102,
115.185155882443)) ;
#169188=CARTESIAN_POINT('Ctrl Pts',(-23.8752983200512,-13.6369615974539,
115.209386936964)) ;
#169189=CARTESIAN_POINT('Ctrl Pts',(-23.8520217309769,-13.6230727255243,
115.138490203622)) ;
#169190=CARTESIAN_POINT('Ctrl Pts',(-23.8336611247372,-13.8991091738745,
115.047105108385)) ;
#169191=CARTESIAN_POINT('Ctrl Pts',(-23.8123650030025,-13.8659263158171,
114.982240558852)) ;
#169192=CARTESIAN_POINT('Ctrl Pts',(-23.8861688379437,-13.8659263690519,
114.958009491342)) ;
#169193=CARTESIAN_POINT('Ctrl Pts',(-23.959972672885,-13.8659264222868,
114.933778423831)) ;
#169194=CARTESIAN_POINT('Ctrl Pts',(-23.9812687946197,-13.8991092803442,
114.998642973364)) ;
#169195=CARTESIAN_POINT('Ctrl Pts',(-24.0025649163544,-13.9322921384017,
115.063507522897)) ;
#169196=CARTESIAN_POINT('Ctrl Pts',(-23.9287610814131,-13.9322920851668,
115.087738590407)) ;
#169197=CARTESIAN_POINT('Ctrl Pts',(-23.8549572464718,-13.9322920319319,
115.111969657918)) ;
#169198=CARTESIAN_POINT('Ctrl Pts',(-23.8336611247372,-13.8991091738745,
115.047105108385)) ;
#169199=CARTESIAN_POINT('Ctrl Pts',(-23.7933725279164,-14.1412745978093,
114.888849693188)) ;
#169200=CARTESIAN_POINT('Ctrl Pts',(-23.7755925026804,-14.0911330408888,
114.834694606088)) ;
#169201=CARTESIAN_POINT('Ctrl Pts',(-23.8493963354353,-14.0911330778526,
114.810463531918)) ;
#169202=CARTESIAN_POINT('Ctrl Pts',(-23.9232001681903,-14.0911331148164,
114.786232457749)) ;
#169203=CARTESIAN_POINT('Ctrl Pts',(-23.9409801934264,-14.141274671737,
114.840387544848)) ;
#169204=CARTESIAN_POINT('Ctrl Pts',(-23.9587602186625,-14.1914162286575,
114.894542631948)) ;
#169205=CARTESIAN_POINT('Ctrl Pts',(-23.8849563859075,-14.1914161916937,
114.918773706118)) ;
#169206=CARTESIAN_POINT('Ctrl Pts',(-23.8111525531525,-14.1914161547299,
114.943004780288)) ;
#169207=CARTESIAN_POINT('Ctrl Pts',(-23.7933725279164,-14.1412745978093,
114.888849693188)) ;
#169208=CARTESIAN_POINT('Ctrl Pts',(-23.7346974692278,-14.3313662237517,
114.67454342391)) ;
#169209=CARTESIAN_POINT('Ctrl Pts',(-23.7217237245287,-14.2678756388728,
114.635027491642)) ;
#169210=CARTESIAN_POINT('Ctrl Pts',(-23.7955275572489,-14.2678756602265,
114.610796417367)) ;
#169211=CARTESIAN_POINT('Ctrl Pts',(-23.8693313899692,-14.2678756815801,
114.586565343091)) ;
#169212=CARTESIAN_POINT('Ctrl Pts',(-23.8823051346683,-14.331366266459,
114.626081275358)) ;
#169213=CARTESIAN_POINT('Ctrl Pts',(-23.8952788793673,-14.3948568513378,
114.665597207626)) ;
#169214=CARTESIAN_POINT('Ctrl Pts',(-23.8214750466471,-14.3948568299842,
114.689828281901)) ;
#169215=CARTESIAN_POINT('Ctrl Pts',(-23.7476712139269,-14.3948568086305,
114.714059356177)) ;
#169216=CARTESIAN_POINT('Ctrl Pts',(-23.7346974692278,-14.3313662237517,
114.67454342391)) ;
#169217=CARTESIAN_POINT('Ctrl Pts',(-23.6635924763443,-14.4547660222928,
114.422764378375)) ;
#169218=CARTESIAN_POINT('Ctrl Pts',(-23.6562923933097,-14.3825637894308,
114.400529503979)) ;
#169219=CARTESIAN_POINT('Ctrl Pts',(-23.7300962264647,-14.3825637991791,
114.376298431027)) ;
#169220=CARTESIAN_POINT('Ctrl Pts',(-23.8039000596197,-14.3825638089273,
114.352067358076)) ;
#169221=CARTESIAN_POINT('Ctrl Pts',(-23.8112001426543,-14.4547660417892,
114.374302232472)) ;
#169222=CARTESIAN_POINT('Ctrl Pts',(-23.8185002256888,-14.5269682746512,
114.396537106869)) ;
#169223=CARTESIAN_POINT('Ctrl Pts',(-23.7446963925338,-14.526968264903,
114.42076817982)) ;
#169224=CARTESIAN_POINT('Ctrl Pts',(-23.6708925593788,-14.5269682551548,
114.444999252771)) ;
#169225=CARTESIAN_POINT('Ctrl Pts',(-23.6635924763443,-14.4547660222928,
114.422764378375)) ;
#169226=CARTESIAN_POINT('Ctrl Pts',(-23.5843592342863,-14.5053328691454,
114.145839565311)) ;
#169227=CARTESIAN_POINT('Ctrl Pts',(-23.5833169453667,-14.4294900381805,
114.142664921913)) ;
#169228=CARTESIAN_POINT('Ctrl Pts',(-23.6571207810576,-14.4294900382422,
114.118433856685)) ;
#169229=CARTESIAN_POINT('Ctrl Pts',(-23.7309246167484,-14.4294900383039,
114.094202791458)) ;
#169230=CARTESIAN_POINT('Ctrl Pts',(-23.731966905668,-14.5053328692688,
114.097377434856)) ;
#169231=CARTESIAN_POINT('Ctrl Pts',(-23.7330091945875,-14.5811757002337,
114.100552078255)) ;
#169232=CARTESIAN_POINT('Ctrl Pts',(-23.6592053588967,-14.581175700172,
114.124783143482)) ;
#169233=CARTESIAN_POINT('Ctrl Pts',(-23.5854015232058,-14.5811757001103,
114.14901420871)) ;
#169234=CARTESIAN_POINT('Ctrl Pts',(-23.5843592342863,-14.5053328691454,
114.145839565311)) ;
#169235=CARTESIAN_POINT('Ctrl Pts',(-23.5043319156258,-14.4771328889757,
113.866567081809)) ;
#169236=CARTESIAN_POINT('Ctrl Pts',(-23.5096110710499,-14.4031442032382,
113.882646537764)) ;
#169237=CARTESIAN_POINT('Ctrl Pts',(-23.5834149094567,-14.4031441988983,
113.858415480808)) ;
#169238=CARTESIAN_POINT('Ctrl Pts',(-23.6572187478634,-14.4031441945584,
113.834184423853)) ;
#169239=CARTESIAN_POINT('Ctrl Pts',(-23.6519395924393,-14.4771328802959,
113.818104967899)) ;
#169240=CARTESIAN_POINT('Ctrl Pts',(-23.6466604370152,-14.5511215660333,
113.802025511944)) ;
#169241=CARTESIAN_POINT('Ctrl Pts',(-23.5728565986085,-14.5511215703732,
113.8262565689)) ;
#169242=CARTESIAN_POINT('Ctrl Pts',(-23.4990527602017,-14.5511215747131,
113.850487625855)) ;
#169243=CARTESIAN_POINT('Ctrl Pts',(-23.5043319156258,-14.4771328889757,
113.866567081809)) ;
#169244=CARTESIAN_POINT('Ctrl Pts',(-23.4303264176823,-14.3740575561619,
113.605870865708)) ;
#169245=CARTESIAN_POINT('Ctrl Pts',(-23.4415111093854,-14.3071548458452,
113.639937632206)) ;
#169246=CARTESIAN_POINT('Ctrl Pts',(-23.5153149498543,-14.307154840074,
113.615706581531)) ;
#169247=CARTESIAN_POINT('Ctrl Pts',(-23.5891187903231,-14.3071548343027,
113.591475530857)) ;
#169248=CARTESIAN_POINT('Ctrl Pts',(-23.5779340986201,-14.3740575446194,
113.557408764359)) ;
#169249=CARTESIAN_POINT('Ctrl Pts',(-23.5667494069171,-14.4409602549361,
113.523341997861)) ;
#169250=CARTESIAN_POINT('Ctrl Pts',(-23.4929455664482,-14.4409602607073,
113.547573048536)) ;
#169251=CARTESIAN_POINT('Ctrl Pts',(-23.4191417259793,-14.4409602664786,
113.57180409921)) ;
#169252=CARTESIAN_POINT('Ctrl Pts',(-23.4303264176823,-14.3740575561619,
113.605870865708)) ;
#169253=CARTESIAN_POINT('Ctrl Pts',(-23.367255733875,-14.2012582823737,
113.378139757424)) ;
#169254=CARTESIAN_POINT('Ctrl Pts',(-23.3835987072137,-14.1463204404916,
113.427917817362)) ;
#169255=CARTESIAN_POINT('Ctrl Pts',(-23.4574025498353,-14.1463204373001,
113.403686773245)) ;
#169256=CARTESIAN_POINT('Ctrl Pts',(-23.531206392457,-14.1463204341086,
113.379455729128)) ;
#169257=CARTESIAN_POINT('Ctrl Pts',(-23.5148634191183,-14.2012582759907,
113.329677669189)) ;
#169258=CARTESIAN_POINT('Ctrl Pts',(-23.4985204457796,-14.2561961178728,
113.27989960925)) ;
#169259=CARTESIAN_POINT('Ctrl Pts',(-23.4247166031579,-14.2561961210643,
113.304130653368)) ;
#169260=CARTESIAN_POINT('Ctrl Pts',(-23.3509127605363,-14.2561961242558,
113.328361697485)) ;
#169261=CARTESIAN_POINT('Ctrl Pts',(-23.367255733875,-14.2012582823737,
113.378139757424)) ;
#169262=CARTESIAN_POINT('Ctrl Pts',(-23.3214527143622,-13.9726608385018,
113.203153689332)) ;
#169263=CARTESIAN_POINT('Ctrl Pts',(-23.341752719975,-13.9336031304971,
113.264984231032)) ;
#169264=CARTESIAN_POINT('Ctrl Pts',(-23.4155565634811,-13.9336031304968,
113.240753189609)) ;
#169265=CARTESIAN_POINT('Ctrl Pts',(-23.4893604069873,-13.9336031304964,
113.216522148185)) ;
#169266=CARTESIAN_POINT('Ctrl Pts',(-23.4690604013745,-13.9726608385011,
113.154691606486)) ;
#169267=CARTESIAN_POINT('Ctrl Pts',(-23.4487603957618,-14.0117185465058,
113.092861064786)) ;
#169268=CARTESIAN_POINT('Ctrl Pts',(-23.3749565522556,-14.0117185465062,
113.117092106209)) ;
#169269=CARTESIAN_POINT('Ctrl Pts',(-23.3011527087495,-14.0117185465065,
113.141323147633)) ;
#169270=CARTESIAN_POINT('Ctrl Pts',(-23.3214527143622,-13.9726608385018,
113.203153689332)) ;
#169271=CARTESIAN_POINT('Ctrl Pts',(-23.2965488105759,-13.7058102020006,
113.091988324737)) ;
#169272=CARTESIAN_POINT('Ctrl Pts',(-23.3193487242451,-13.6853276622156,
113.161433182971)) ;
#169273=CARTESIAN_POINT('Ctrl Pts',(-23.3931525679122,-13.685327664635,
113.137202142038)) ;
#169274=CARTESIAN_POINT('Ctrl Pts',(-23.4669564115793,-13.6853276670543,
113.112971101105)) ;
#169275=CARTESIAN_POINT('Ctrl Pts',(-23.4441564979102,-13.7058102068394,
113.04352624287)) ;
#169276=CARTESIAN_POINT('Ctrl Pts',(-23.421356584241,-13.7262927466244,
112.974081384636)) ;
#169277=CARTESIAN_POINT('Ctrl Pts',(-23.3475527405739,-13.726292744205,
112.998312425569)) ;
#169278=CARTESIAN_POINT('Ctrl Pts',(-23.2737488969068,-13.7262927417856,
113.022543466502)) ;
#169279=CARTESIAN_POINT('Ctrl Pts',(-23.2965488105759,-13.7058102020006,
113.091988324737)) ;
#169280=CARTESIAN_POINT('Ctrl Pts',(-23.2950095776943,-13.4160016672544,
113.051687295608)) ;
#169281=CARTESIAN_POINT('Ctrl Pts',(-23.318688002029,-13.4157263085417,
113.123807955567)) ;
#169282=CARTESIAN_POINT('Ctrl Pts',(-23.3924918454245,-13.4157263119192,
113.099576913806)) ;
#169283=CARTESIAN_POINT('Ctrl Pts',(-23.4662956888199,-13.4157263152968,
113.075345872045)) ;
#169284=CARTESIAN_POINT('Ctrl Pts',(-23.4426172644851,-13.4160016740095,
113.003225212087)) ;
#169285=CARTESIAN_POINT('Ctrl Pts',(-23.4189388401504,-13.4162770327222,
112.931104552128)) ;
#169286=CARTESIAN_POINT('Ctrl Pts',(-23.345134996755,-13.4162770293446,
112.955335593889)) ;
#169287=CARTESIAN_POINT('Ctrl Pts',(-23.2713311533596,-13.4162770259671,
112.979566635649)) ;
#169288=CARTESIAN_POINT('Ctrl Pts',(-23.2950095776943,-13.4160016672544,
113.051687295608)) ;
#169289=CARTESIAN_POINT('Ctrl Pts',(-23.3177569881887,-13.1285751860039,
113.085639842079)) ;
#169290=CARTESIAN_POINT('Ctrl Pts',(-23.3406129860406,-13.1483696405658,
113.155255523698)) ;
#169291=CARTESIAN_POINT('Ctrl Pts',(-23.4144168292376,-13.1483696423267,
113.131024481333)) ;
#169292=CARTESIAN_POINT('Ctrl Pts',(-23.4882206724346,-13.1483696440876,
113.106793438967)) ;
#169293=CARTESIAN_POINT('Ctrl Pts',(-23.4653646745826,-13.1285751895257,
113.037177757348)) ;
#169294=CARTESIAN_POINT('Ctrl Pts',(-23.4425086767307,-13.1087807349637,
112.967562075729)) ;
#169295=CARTESIAN_POINT('Ctrl Pts',(-23.3687048335338,-13.1087807332029,
112.991793118094)) ;
#169296=CARTESIAN_POINT('Ctrl Pts',(-23.2949009903368,-13.108780731442,
113.016024160459)) ;
#169297=CARTESIAN_POINT('Ctrl Pts',(-23.3177569881887,-13.1285751860039,
113.085639842079)) ;
#169298=CARTESIAN_POINT('Ctrl Pts',(-23.3638473343004,-12.8607655160009,
113.19057058285)) ;
#169299=CARTESIAN_POINT('Ctrl Pts',(-23.3842522246996,-12.8992892822013,
113.252720586712)) ;
#169300=CARTESIAN_POINT('Ctrl Pts',(-23.4580560681807,-12.8992892809573,
113.228489545212)) ;
#169301=CARTESIAN_POINT('Ctrl Pts',(-23.5318599116619,-12.8992892797133,
113.204258503713)) ;
#169302=CARTESIAN_POINT('Ctrl Pts',(-23.5114550212627,-12.8607655135129,
113.14210849985)) ;
#169303=CARTESIAN_POINT('Ctrl Pts',(-23.4910501308634,-12.8222417473126,
113.079958495988)) ;
#169304=CARTESIAN_POINT('Ctrl Pts',(-23.4172462873823,-12.8222417485565,
113.104189537488)) ;
#169305=CARTESIAN_POINT('Ctrl Pts',(-23.3434424439011,-12.8222417498005,
113.128420578987)) ;
#169306=CARTESIAN_POINT('Ctrl Pts',(-23.3638473343004,-12.8607655160009,
113.19057058285)) ;
#169307=CARTESIAN_POINT('Ctrl Pts',(-23.4313745687069,-12.6316532711116,
113.360568411281)) ;
#169308=CARTESIAN_POINT('Ctrl Pts',(-23.4478325750678,-12.686231857174,
113.410696843313)) ;
#169309=CARTESIAN_POINT('Ctrl Pts',(-23.5216364200498,-12.6862318515475,
113.386465806385)) ;
#169310=CARTESIAN_POINT('Ctrl Pts',(-23.5954402650319,-12.6862318459211,
113.362234769457)) ;
#169311=CARTESIAN_POINT('Ctrl Pts',(-23.5789822586709,-12.6316532598588,
113.312106337425)) ;
#169312=CARTESIAN_POINT('Ctrl Pts',(-23.56252425231,-12.5770746737964,113.261977905393)) ;
#169313=CARTESIAN_POINT('Ctrl Pts',(-23.488720407328,-12.5770746794228,
113.286208942321)) ;
#169314=CARTESIAN_POINT('Ctrl Pts',(-23.4149165623459,-12.5770746850493,
113.310439979249)) ;
#169315=CARTESIAN_POINT('Ctrl Pts',(-23.4313745687069,-12.6316532711116,
113.360568411281)) ;
#169316=CARTESIAN_POINT('Ctrl Pts',(-23.5152154328115,-12.460718041819,
113.580530422711)) ;
#169317=CARTESIAN_POINT('Ctrl Pts',(-23.5265758928896,-12.5273111609863,
113.615132551369)) ;
#169318=CARTESIAN_POINT('Ctrl Pts',(-23.6003797399565,-12.5273111540266,
113.590901520791)) ;
#169319=CARTESIAN_POINT('Ctrl Pts',(-23.6741835870235,-12.5273111470668,
113.566670490213)) ;
#169320=CARTESIAN_POINT('Ctrl Pts',(-23.6628231269454,-12.4607180278995,
113.532068361556)) ;
#169321=CARTESIAN_POINT('Ctrl Pts',(-23.6514626668674,-12.3941249087322,
113.497466232898)) ;
#169322=CARTESIAN_POINT('Ctrl Pts',(-23.5776588198004,-12.394124915692,
113.521697263476)) ;
#169323=CARTESIAN_POINT('Ctrl Pts',(-23.5038549727334,-12.3941249226517,
113.545928294054)) ;
#169324=CARTESIAN_POINT('Ctrl Pts',(-23.5152154328115,-12.460718041819,
113.580530422711)) ;
#169325=CARTESIAN_POINT('Ctrl Pts',(-23.6105283082249,-12.3580087732105,
113.83543283703)) ;
#169326=CARTESIAN_POINT('Ctrl Pts',(-23.6159828998831,-12.4318697519678,
113.85204664352)) ;
#169327=CARTESIAN_POINT('Ctrl Pts',(-23.6897867494488,-12.4318697467782,
113.827815620553)) ;
#169328=CARTESIAN_POINT('Ctrl Pts',(-23.7635905990146,-12.4318697415885,
113.803584597586)) ;
#169329=CARTESIAN_POINT('Ctrl Pts',(-23.7581360073565,-12.3580087628311,
113.786970791096)) ;
#169330=CARTESIAN_POINT('Ctrl Pts',(-23.7526814156984,-12.2841477840738,
113.770356984606)) ;
#169331=CARTESIAN_POINT('Ctrl Pts',(-23.6788775661326,-12.2841477892635,
113.794588007573)) ;
#169332=CARTESIAN_POINT('Ctrl Pts',(-23.6050737165668,-12.2841477944531,
113.81881903054)) ;
#169333=CARTESIAN_POINT('Ctrl Pts',(-23.6105283082249,-12.3580087732105,
113.83543283703)) ;
#169334=CARTESIAN_POINT('Ctrl Pts',(-23.711289186048,-12.3309308762199,
114.106935761208)) ;
#169335=CARTESIAN_POINT('Ctrl Pts',(-23.7104488970533,-12.4067892276866,
114.104376377047)) ;
#169336=CARTESIAN_POINT('Ctrl Pts',(-23.7842527491276,-12.4067892280987,
114.08014536172)) ;
#169337=CARTESIAN_POINT('Ctrl Pts',(-23.8580566012019,-12.4067892285108,
114.055914346394)) ;
#169338=CARTESIAN_POINT('Ctrl Pts',(-23.8588968901966,-12.330930877044,
114.058473730555)) ;
#169339=CARTESIAN_POINT('Ctrl Pts',(-23.8597371791913,-12.2550725255773,
114.061033114716)) ;
#169340=CARTESIAN_POINT('Ctrl Pts',(-23.7859333271171,-12.2550725251652,
114.085264130043)) ;
#169341=CARTESIAN_POINT('Ctrl Pts',(-23.7121294750428,-12.2550725247531,
114.109495145369)) ;
#169342=CARTESIAN_POINT('Ctrl Pts',(-23.711289186048,-12.3309308762199,
114.106935761208)) ;
#169343=CARTESIAN_POINT('Ctrl Pts',(-23.811392388045,-12.3817530522947,
114.376315180334)) ;
#169344=CARTESIAN_POINT('Ctrl Pts',(-23.8042965762851,-12.4541728296822,
114.354702483328)) ;
#169345=CARTESIAN_POINT('Ctrl Pts',(-23.878100430679,-12.454172840125,114.330471475067)) ;
#169346=CARTESIAN_POINT('Ctrl Pts',(-23.9519042850728,-12.4541728505679,
114.306240466806)) ;
#169347=CARTESIAN_POINT('Ctrl Pts',(-23.9590000968328,-12.3817530731804,
114.327853163812)) ;
#169348=CARTESIAN_POINT('Ctrl Pts',(-23.9660959085927,-12.3093332957928,
114.349465860818)) ;
#169349=CARTESIAN_POINT('Ctrl Pts',(-23.8922920541988,-12.30933328535,114.373696869079)) ;
#169350=CARTESIAN_POINT('Ctrl Pts',(-23.818488199805,-12.3093332749072,
114.39792787734)) ;
#169351=CARTESIAN_POINT('Ctrl Pts',(-23.811392388045,-12.3817530522947,
114.376315180334)) ;
#169352=CARTESIAN_POINT('Ctrl Pts',(-23.9039028684115,-12.506826084586,
114.622631137675)) ;
#169353=CARTESIAN_POINT('Ctrl Pts',(-23.8910714153864,-12.5706179101752,
114.583548602984)) ;
#169354=CARTESIAN_POINT('Ctrl Pts',(-23.9648752707621,-12.5706179343356,
114.559317597713)) ;
#169355=CARTESIAN_POINT('Ctrl Pts',(-24.0386791261378,-12.5706179584961,
114.535086592443)) ;
#169356=CARTESIAN_POINT('Ctrl Pts',(-24.0515105791629,-12.5068261329069,
114.574169127134)) ;
#169357=CARTESIAN_POINT('Ctrl Pts',(-24.0643420321881,-12.4430343073178,
114.613251661825)) ;
#169358=CARTESIAN_POINT('Ctrl Pts',(-23.9905381768124,-12.4430342831573,
114.637482667096)) ;
#169359=CARTESIAN_POINT('Ctrl Pts',(-23.9167343214367,-12.4430342589969,
114.661713672366)) ;
#169360=CARTESIAN_POINT('Ctrl Pts',(-23.9039028684115,-12.506826084586,
114.622631137675)) ;
#169361=CARTESIAN_POINT('Ctrl Pts',(-23.9831660419676,-12.6970626230436,
114.828592893483)) ;
#169362=CARTESIAN_POINT('Ctrl Pts',(-23.9655157499272,-12.7476645000542,
114.774832952836)) ;
#169363=CARTESIAN_POINT('Ctrl Pts',(-24.0393196046863,-12.7476645399719,
114.750601945687)) ;
#169364=CARTESIAN_POINT('Ctrl Pts',(-24.1131234594454,-12.7476645798895,
114.726370938538)) ;
#169365=CARTESIAN_POINT('Ctrl Pts',(-24.1307737514858,-12.6970627028788,
114.780130879185)) ;
#169366=CARTESIAN_POINT('Ctrl Pts',(-24.1484240435262,-12.6464608258682,
114.833890819833)) ;
#169367=CARTESIAN_POINT('Ctrl Pts',(-24.0746201887671,-12.6464607859506,
114.858121826981)) ;
#169368=CARTESIAN_POINT('Ctrl Pts',(-24.000816334008,-12.646460746033,114.88235283413)) ;
#169369=CARTESIAN_POINT('Ctrl Pts',(-23.9831660419676,-12.6970626230436,
114.828592893483)) ;
#169370=CARTESIAN_POINT('Ctrl Pts',(-24.0443887911562,-12.9398196291384,
114.979493433224)) ;
#169371=CARTESIAN_POINT('Ctrl Pts',(-24.0231745362282,-12.9735460220805,
114.91487823685)) ;
#169372=CARTESIAN_POINT('Ctrl Pts',(-24.0969783885857,-12.9735460788729,
114.890647222387)) ;
#169373=CARTESIAN_POINT('Ctrl Pts',(-24.1707822409432,-12.9735461356652,
114.866416207923)) ;
#169374=CARTESIAN_POINT('Ctrl Pts',(-24.1919964958711,-12.9398197427232,
114.931031404297)) ;
#169375=CARTESIAN_POINT('Ctrl Pts',(-24.2132107507992,-12.9060933497811,
114.995646600671)) ;
#169376=CARTESIAN_POINT('Ctrl Pts',(-24.1394068984417,-12.9060932929888,
115.019877615135)) ;
#169377=CARTESIAN_POINT('Ctrl Pts',(-24.0656030460843,-12.9060932361964,
115.044108629598)) ;
#169378=CARTESIAN_POINT('Ctrl Pts',(-24.0443887911562,-12.9398196291384,
114.979493433224)) ;
#169379=CARTESIAN_POINT('Ctrl Pts',(-24.0834950036509,-13.2163226304817,
115.063123342648)) ;
#169380=CARTESIAN_POINT('Ctrl Pts',(-24.060253892529,-13.2307930159817,
114.992334669498)) ;
#169381=CARTESIAN_POINT('Ctrl Pts',(-24.134057740261,-13.2307930864604,
114.968103640946)) ;
#169382=CARTESIAN_POINT('Ctrl Pts',(-24.207861587993,-13.2307931569392,
114.943872612394)) ;
#169383=CARTESIAN_POINT('Ctrl Pts',(-24.2311026991149,-13.2163227714392,
115.014661285543)) ;
#169384=CARTESIAN_POINT('Ctrl Pts',(-24.2543438102368,-13.2018523859393,
115.085449958693)) ;
#169385=CARTESIAN_POINT('Ctrl Pts',(-24.1805399625048,-13.2018523154605,
115.109680987245)) ;
#169386=CARTESIAN_POINT('Ctrl Pts',(-24.1067361147728,-13.2018522449817,
115.133912015797)) ;
#169387=CARTESIAN_POINT('Ctrl Pts',(-24.0834950036509,-13.2163226304817,
115.063123342648)) ;
#169388=CARTESIAN_POINT('Ctrl Pts',(-24.0987740331511,-13.5056990228868,
115.074368143953)) ;
#169389=CARTESIAN_POINT('Ctrl Pts',(-24.0751629373277,-13.4999868027269,
115.00245255722)) ;
#169390=CARTESIAN_POINT('Ctrl Pts',(-24.1489667789724,-13.4999868805839,
114.978221510127)) ;
#169391=CARTESIAN_POINT('Ctrl Pts',(-24.2227706206172,-13.499986958441,
114.953990463034)) ;
#169392=CARTESIAN_POINT('Ctrl Pts',(-24.2463817164407,-13.5056991786008,
115.025906049768)) ;
#169393=CARTESIAN_POINT('Ctrl Pts',(-24.2699928122642,-13.5114113987607,
115.097821636502)) ;
#169394=CARTESIAN_POINT('Ctrl Pts',(-24.1961889706194,-13.5114113209037,
115.122052683594)) ;
#169395=CARTESIAN_POINT('Ctrl Pts',(-24.1223851289746,-13.5114112430466,
115.146283730687)) ;
#169396=CARTESIAN_POINT('Ctrl Pts',(-24.0987740331511,-13.5056990228868,
115.074368143953)) ;
#169397=CARTESIAN_POINT('Ctrl Pts',(-24.0898176525087,-13.7916926696265,
115.011429383632)) ;
#169398=CARTESIAN_POINT('Ctrl Pts',(-24.067535226085,-13.7660050582146,
114.943560709675)) ;
#169399=CARTESIAN_POINT('Ctrl Pts',(-24.1413390603976,-13.7660051397553,
114.91932964025)) ;
#169400=CARTESIAN_POINT('Ctrl Pts',(-24.2151428947103,-13.766005221296,
114.895098570825)) ;
#169401=CARTESIAN_POINT('Ctrl Pts',(-24.2374253211339,-13.791692832708,
114.962967244781)) ;
#169402=CARTESIAN_POINT('Ctrl Pts',(-24.2597077475576,-13.81738044412,115.030835918738)) ;
#169403=CARTESIAN_POINT('Ctrl Pts',(-24.185903913245,-13.8173803625793,
115.055066988163)) ;
#169404=CARTESIAN_POINT('Ctrl Pts',(-24.1121000789324,-13.8173802810385,
115.079298057588)) ;
#169405=CARTESIAN_POINT('Ctrl Pts',(-24.0898176525087,-13.7916926696265,
115.011429383632)) ;
#169406=CARTESIAN_POINT('Ctrl Pts',(-24.0580663785572,-14.0485418604028,
114.879359386084)) ;
#169407=CARTESIAN_POINT('Ctrl Pts',(-24.0387000607933,-14.0048845368929,
114.820372708696)) ;
#169408=CARTESIAN_POINT('Ctrl Pts',(-24.1125038876702,-14.0048846120398,
114.796141616622)) ;
#169409=CARTESIAN_POINT('Ctrl Pts',(-24.1863077145469,-14.0048846871867,
114.771910524549)) ;
#169410=CARTESIAN_POINT('Ctrl Pts',(-24.2056740323108,-14.0485420106967,
114.830897201937)) ;
#169411=CARTESIAN_POINT('Ctrl Pts',(-24.2250403500747,-14.0921993342066,
114.889883879324)) ;
#169412=CARTESIAN_POINT('Ctrl Pts',(-24.1512365231979,-14.0921992590597,
114.914114971398)) ;
#169413=CARTESIAN_POINT('Ctrl Pts',(-24.0774326963211,-14.0921991839128,
114.938346063471)) ;
#169414=CARTESIAN_POINT('Ctrl Pts',(-24.0580663785572,-14.0485418604028,
114.879359386084)) ;
#169415=CARTESIAN_POINT('Ctrl Pts',(-24.0066666727784,-14.2607963084926,
114.687415370563)) ;
#169416=CARTESIAN_POINT('Ctrl Pts',(-23.9915929582829,-14.2022566312554,
114.641503270218)) ;
#169417=CARTESIAN_POINT('Ctrl Pts',(-24.0653967783519,-14.2022566928803,
114.617272157409)) ;
#169418=CARTESIAN_POINT('Ctrl Pts',(-24.1392005984209,-14.2022567545052,
114.5930410446)) ;
#169419=CARTESIAN_POINT('Ctrl Pts',(-24.1542743129165,-14.2607964317425,
114.638953144946)) ;
#169420=CARTESIAN_POINT('Ctrl Pts',(-24.169348027412,-14.3193361089797,
114.684865245291)) ;
#169421=CARTESIAN_POINT('Ctrl Pts',(-24.095544207343,-14.3193360473548,
114.7090963581)) ;
#169422=CARTESIAN_POINT('Ctrl Pts',(-24.021740387274,-14.3193359857299,
114.733327470909)) ;
#169423=CARTESIAN_POINT('Ctrl Pts',(-24.0066666727784,-14.2607963084926,
114.687415370563)) ;
#169424=CARTESIAN_POINT('Ctrl Pts',(-23.9395888105032,-14.4133855037132,
114.447558126479)) ;
#169425=CARTESIAN_POINT('Ctrl Pts',(-23.9299116484695,-14.3441068413642,
114.418083054295)) ;
#169426=CARTESIAN_POINT('Ctrl Pts',(-24.0037154628795,-14.3441068827324,
114.39385192425)) ;
#169427=CARTESIAN_POINT('Ctrl Pts',(-24.0775192772894,-14.3441069241007,
114.369620794205)) ;
#169428=CARTESIAN_POINT('Ctrl Pts',(-24.0871964393232,-14.4133855864497,
114.399095866389)) ;
#169429=CARTESIAN_POINT('Ctrl Pts',(-24.096873601357,-14.4826642487988,
114.428570938573)) ;
#169430=CARTESIAN_POINT('Ctrl Pts',(-24.023069786947,-14.4826642074306,
114.452802068618)) ;
#169431=CARTESIAN_POINT('Ctrl Pts',(-23.949265972537,-14.4826641660623,
114.477033198663)) ;
#169432=CARTESIAN_POINT('Ctrl Pts',(-23.9395888105032,-14.4133855037132,
114.447558126479)) ;
#169433=CARTESIAN_POINT('Ctrl Pts',(-23.8629281001325,-14.4941554742073,
114.178638574649)) ;
#169434=CARTESIAN_POINT('Ctrl Pts',(-23.8593218801757,-14.4191362246067,
114.16765461255)) ;
#169435=CARTESIAN_POINT('Ctrl Pts',(-23.9331256912243,-14.4191362402107,
114.143423472266)) ;
#169436=CARTESIAN_POINT('Ctrl Pts',(-24.0069295022728,-14.4191362558146,
114.119192331982)) ;
#169437=CARTESIAN_POINT('Ctrl Pts',(-24.0105357222296,-14.4941555054153,
114.130176294082)) ;
#169438=CARTESIAN_POINT('Ctrl Pts',(-24.0141419421864,-14.5691747550159,
114.141160256181)) ;
#169439=CARTESIAN_POINT('Ctrl Pts',(-23.9403381311378,-14.5691747394119,
114.165391396465)) ;
#169440=CARTESIAN_POINT('Ctrl Pts',(-23.8665343200893,-14.5691747238079,
114.189622536749)) ;
#169441=CARTESIAN_POINT('Ctrl Pts',(-23.8629281001325,-14.4941554742073,
114.178638574649)) ;
#169442=CARTESIAN_POINT('Ctrl Pts',(-23.7825672394954,-14.4980202636657,
113.898384946366)) ;
#169443=CARTESIAN_POINT('Ctrl Pts',(-23.7853004615776,-14.4226207212898,
113.906709901897)) ;
#169444=CARTESIAN_POINT('Ctrl Pts',(-23.859104271779,-14.4226207084362,
113.882478759033)) ;
#169445=CARTESIAN_POINT('Ctrl Pts',(-23.9329080819803,-14.4226206955826,
113.858247616169)) ;
#169446=CARTESIAN_POINT('Ctrl Pts',(-23.9301748598981,-14.4980202379585,
113.849922660638)) ;
#169447=CARTESIAN_POINT('Ctrl Pts',(-23.9274416378159,-14.5734197803344,
113.841597705107)) ;
#169448=CARTESIAN_POINT('Ctrl Pts',(-23.8536378276146,-14.573419793188,
113.865828847971)) ;
#169449=CARTESIAN_POINT('Ctrl Pts',(-23.7798340174132,-14.5734198060416,
113.890059990835)) ;
#169450=CARTESIAN_POINT('Ctrl Pts',(-23.7825672394954,-14.4980202636657,
113.898384946366)) ;
#169451=CARTESIAN_POINT('Ctrl Pts',(-23.7052727096048,-14.4245044594768,
113.627527308844)) ;
#169452=CARTESIAN_POINT('Ctrl Pts',(-23.7141395064161,-14.3541263042152,
113.654534143371)) ;
#169453=CARTESIAN_POINT('Ctrl Pts',(-23.7879433185797,-14.3541262631264,
113.630303006484)) ;
#169454=CARTESIAN_POINT('Ctrl Pts',(-23.8617471307432,-14.3541262220375,
113.606071869596)) ;
#169455=CARTESIAN_POINT('Ctrl Pts',(-23.8528803339319,-14.4245043772991,
113.579065035068)) ;
#169456=CARTESIAN_POINT('Ctrl Pts',(-23.8440135371206,-14.4948825325607,
113.552058200541)) ;
#169457=CARTESIAN_POINT('Ctrl Pts',(-23.770209724957,-14.4948825736496,
113.576289337429)) ;
#169458=CARTESIAN_POINT('Ctrl Pts',(-23.6964059127935,-14.4948826147384,
113.600520474317)) ;
#169459=CARTESIAN_POINT('Ctrl Pts',(-23.7052727096048,-14.4245044594768,
113.627527308844)) ;
#169460=CARTESIAN_POINT('Ctrl Pts',(-23.6372016675347,-14.279297376843,
113.384786368389)) ;
#169461=CARTESIAN_POINT('Ctrl Pts',(-23.6515666761006,-14.2189530105724,
113.428539868789)) ;
#169462=CARTESIAN_POINT('Ctrl Pts',(-23.7253704927677,-14.2189529442762,
113.404308745619)) ;
#169463=CARTESIAN_POINT('Ctrl Pts',(-23.7991743094348,-14.2189528779799,
113.380077622448)) ;
#169464=CARTESIAN_POINT('Ctrl Pts',(-23.7848093008689,-14.2792972442505,
113.336324122048)) ;
#169465=CARTESIAN_POINT('Ctrl Pts',(-23.770444292303,-14.3396416105211,
113.292570621647)) ;
#169466=CARTESIAN_POINT('Ctrl Pts',(-23.696640475636,-14.3396416768173,
113.316801744818)) ;
#169467=CARTESIAN_POINT('Ctrl Pts',(-23.6228366589689,-14.3396417431136,
113.341032867988)) ;
#169468=CARTESIAN_POINT('Ctrl Pts',(-23.6372016675347,-14.279297376843,
113.384786368389)) ;
#169469=CARTESIAN_POINT('Ctrl Pts',(-23.583741652297,-14.0713598205673,
113.186374509989)) ;
#169470=CARTESIAN_POINT('Ctrl Pts',(-23.6025966694698,-14.0254428843111,
113.24380385212)) ;
#169471=CARTESIAN_POINT('Ctrl Pts',(-23.6764004928724,-14.0254427985769,
113.219572749465)) ;
#169472=CARTESIAN_POINT('Ctrl Pts',(-23.750204316275,-14.0254427128428,
113.19534164681)) ;
#169473=CARTESIAN_POINT('Ctrl Pts',(-23.7313492991022,-14.0713596490991,
113.137912304678)) ;
#169474=CARTESIAN_POINT('Ctrl Pts',(-23.7124942819294,-14.1172765853553,
113.080482962546)) ;
#169475=CARTESIAN_POINT('Ctrl Pts',(-23.6386904585268,-14.1172766710895,
113.104714065202)) ;
#169476=CARTESIAN_POINT('Ctrl Pts',(-23.5648866351242,-14.1172767568236,
113.128945167857)) ;
#169477=CARTESIAN_POINT('Ctrl Pts',(-23.583741652297,-14.0713598205673,
113.186374509989)) ;
#169478=CARTESIAN_POINT('Ctrl Pts',(-23.5499741300626,-13.8176789860274,
113.048124711497)) ;
#169479=CARTESIAN_POINT('Ctrl Pts',(-23.5719472275288,-13.7894049725344,
113.115051223061)) ;
#169480=CARTESIAN_POINT('Ctrl Pts',(-23.6457510590017,-13.7894048748747,
113.090820144986)) ;
#169481=CARTESIAN_POINT('Ctrl Pts',(-23.7195548904747,-13.789404777215,
113.066589066912)) ;
#169482=CARTESIAN_POINT('Ctrl Pts',(-23.6975817930084,-13.8176787907079,
112.999662555348)) ;
#169483=CARTESIAN_POINT('Ctrl Pts',(-23.6756086955422,-13.8459528042009,
112.932736043785)) ;
#169484=CARTESIAN_POINT('Ctrl Pts',(-23.6018048640693,-13.8459529018606,
112.95696712186)) ;
#169485=CARTESIAN_POINT('Ctrl Pts',(-23.5280010325963,-13.8459529995203,
112.981198199934)) ;
#169486=CARTESIAN_POINT('Ctrl Pts',(-23.5499741300626,-13.8176789860274,
113.048124711497)) ;
#169487=CARTESIAN_POINT('Ctrl Pts',(-23.5387047936549,-13.5347545509982,
112.97830483339)) ;
#169488=CARTESIAN_POINT('Ctrl Pts',(-23.5622320126425,-13.526191139526,
113.049964948284)) ;
#169489=CARTESIAN_POINT('Ctrl Pts',(-23.6360358527796,-13.5261910386332,
113.0257338966)) ;
#169490=CARTESIAN_POINT('Ctrl Pts',(-23.7098396929168,-13.5261909377405,
113.001502844915)) ;
#169491=CARTESIAN_POINT('Ctrl Pts',(-23.6863124739292,-13.5347543492127,
112.929842730021)) ;
#169492=CARTESIAN_POINT('Ctrl Pts',(-23.6627852549415,-13.5433177606849,
112.858182615127)) ;
#169493=CARTESIAN_POINT('Ctrl Pts',(-23.5889814148044,-13.5433178615776,
112.882413666812)) ;
#169494=CARTESIAN_POINT('Ctrl Pts',(-23.5151775746673,-13.5433179624704,
112.906644718497)) ;
#169495=CARTESIAN_POINT('Ctrl Pts',(-23.5387047936549,-13.5347545509982,
112.97830483339)) ;
#169496=CARTESIAN_POINT('Ctrl Pts',(-23.5516559483396,-13.2436560304018,
112.982285898806)) ;
#169497=CARTESIAN_POINT('Ctrl Pts',(-23.575048090854,-13.2554035564965,
113.05353459247)) ;
#169498=CARTESIAN_POINT('Ctrl Pts',(-23.6488519392539,-13.2554034608617,
113.029303565953)) ;
#169499=CARTESIAN_POINT('Ctrl Pts',(-23.7226557876538,-13.2554033652269,
113.005072539435)) ;
#169500=CARTESIAN_POINT('Ctrl Pts',(-23.6992636451394,-13.2436558391322,
112.93382384577)) ;
#169501=CARTESIAN_POINT('Ctrl Pts',(-23.675871502625,-13.2319083130375,
112.862575152106)) ;
#169502=CARTESIAN_POINT('Ctrl Pts',(-23.6020676542251,-13.2319084086723,
112.886806178624)) ;
#169503=CARTESIAN_POINT('Ctrl Pts',(-23.5282638058252,-13.2319085043071,
112.911037205141)) ;
#169504=CARTESIAN_POINT('Ctrl Pts',(-23.5516559483396,-13.2436560304018,
112.982285898806)) ;
#169505=CARTESIAN_POINT('Ctrl Pts',(-23.5885583255177,-12.9652204672347,
113.059240112295)) ;
#169506=CARTESIAN_POINT('Ctrl Pts',(-23.6101425833914,-12.9964254468849,
113.124982280943)) ;
#169507=CARTESIAN_POINT('Ctrl Pts',(-23.6839464388598,-12.9964253637305,
113.100751275955)) ;
#169508=CARTESIAN_POINT('Ctrl Pts',(-23.7577502943282,-12.996425280576,
113.076520270967)) ;
#169509=CARTESIAN_POINT('Ctrl Pts',(-23.7361660364545,-12.9652203009257,
113.010778102319)) ;
#169510=CARTESIAN_POINT('Ctrl Pts',(-23.7145817785808,-12.9340153212755,
112.94503593367)) ;
#169511=CARTESIAN_POINT('Ctrl Pts',(-23.6407779231125,-12.93401540443,112.969266938659)) ;
#169512=CARTESIAN_POINT('Ctrl Pts',(-23.5669740676441,-12.9340154875845,
112.993497943647)) ;
#169513=CARTESIAN_POINT('Ctrl Pts',(-23.5885583255177,-12.9652204672347,
113.059240112295)) ;
#169514=CARTESIAN_POINT('Ctrl Pts',(-23.6475911503442,-12.7189935301929,
113.203572736331)) ;
#169515=CARTESIAN_POINT('Ctrl Pts',(-23.6658203545754,-12.7674367069974,
113.259095952798)) ;
#169516=CARTESIAN_POINT('Ctrl Pts',(-23.7396242152506,-12.7674366419676,
113.234864963669)) ;
#169517=CARTESIAN_POINT('Ctrl Pts',(-23.8134280759257,-12.7674365769377,
113.210633974539)) ;
#169518=CARTESIAN_POINT('Ctrl Pts',(-23.7951988716945,-12.7189934001331,
113.155110758072)) ;
#169519=CARTESIAN_POINT('Ctrl Pts',(-23.7769696674633,-12.6705502233285,
113.099587541605)) ;
#169520=CARTESIAN_POINT('Ctrl Pts',(-23.7031658067881,-12.6705502883584,
113.123818530734)) ;
#169521=CARTESIAN_POINT('Ctrl Pts',(-23.629361946113,-12.6705503533883,
113.148049519863)) ;
#169522=CARTESIAN_POINT('Ctrl Pts',(-23.6475911503442,-12.7189935301929,
113.203572736331)) ;
#169523=CARTESIAN_POINT('Ctrl Pts',(-23.7252965328095,-12.5228013953796,
113.404766433141)) ;
#169524=CARTESIAN_POINT('Ctrl Pts',(-23.738862230298,-12.585015703863,113.446085360385)) ;
#169525=CARTESIAN_POINT('Ctrl Pts',(-23.812666093898,-12.5850156600089,
113.421854380164)) ;
#169526=CARTESIAN_POINT('Ctrl Pts',(-23.8864699574979,-12.5850156161548,
113.397623399943)) ;
#169527=CARTESIAN_POINT('Ctrl Pts',(-23.8729042600094,-12.5228013076713,
113.356304472699)) ;
#169528=CARTESIAN_POINT('Ctrl Pts',(-23.8593385625208,-12.4605869991879,
113.314985545455)) ;
#169529=CARTESIAN_POINT('Ctrl Pts',(-23.7855346989208,-12.460587043042,
113.339216525676)) ;
#169530=CARTESIAN_POINT('Ctrl Pts',(-23.7117308353209,-12.4605870868961,
113.363447505897)) ;
#169531=CARTESIAN_POINT('Ctrl Pts',(-23.7252965328095,-12.5228013953796,
113.404766433141)) ;
#169532=CARTESIAN_POINT('Ctrl Pts',(-23.8167981675552,-12.3908781186536,
113.647994834552)) ;
#169533=CARTESIAN_POINT('Ctrl Pts',(-23.8247297631087,-12.462397411453,
113.672153196211)) ;
#169534=CARTESIAN_POINT('Ctrl Pts',(-23.8985336273289,-12.4623973889088,
113.647922217879)) ;
#169535=CARTESIAN_POINT('Ctrl Pts',(-23.9723374915491,-12.4623973663647,
113.623691239548)) ;
#169536=CARTESIAN_POINT('Ctrl Pts',(-23.9644058959957,-12.3908780735653,
113.599532877889)) ;
#169537=CARTESIAN_POINT('Ctrl Pts',(-23.9564743004422,-12.3193587807659,
113.575374516231)) ;
#169538=CARTESIAN_POINT('Ctrl Pts',(-23.882670436222,-12.3193588033101,
113.599605494562)) ;
#169539=CARTESIAN_POINT('Ctrl Pts',(-23.8088665720018,-12.3193588258542,
113.623836472894)) ;
#169540=CARTESIAN_POINT('Ctrl Pts',(-23.8167981675552,-12.3908781186536,
113.647994834552)) ;
#169541=CARTESIAN_POINT('Ctrl Pts',(-23.9162161601881,-12.3325103501403,
113.915369597383)) ;
#169542=CARTESIAN_POINT('Ctrl Pts',(-23.9179516544004,-12.4082131688575,
113.92065563394)) ;
#169543=CARTESIAN_POINT('Ctrl Pts',(-23.9917555172703,-12.4082131654103,
113.896424651495)) ;
#169544=CARTESIAN_POINT('Ctrl Pts',(-24.0655593801402,-12.4082131619632,
113.872193669051)) ;
#169545=CARTESIAN_POINT('Ctrl Pts',(-24.0638238859279,-12.332510343246,
113.866907632493)) ;
#169546=CARTESIAN_POINT('Ctrl Pts',(-24.0620883917157,-12.2568075245288,
113.861621595936)) ;
#169547=CARTESIAN_POINT('Ctrl Pts',(-23.9882845288458,-12.2568075279759,
113.885852578381)) ;
#169548=CARTESIAN_POINT('Ctrl Pts',(-23.9144806659759,-12.2568075314231,
113.910083560825)) ;
#169549=CARTESIAN_POINT('Ctrl Pts',(-23.9162161601881,-12.3325103501403,
113.915369597383)) ;
#169550=CARTESIAN_POINT('Ctrl Pts',(-24.017451872201,-12.3519340314614,
114.188217872385)) ;
#169551=CARTESIAN_POINT('Ctrl Pts',(-24.0128562086239,-12.4263955875959,
114.174220223673)) ;
#169552=CARTESIAN_POINT('Ctrl Pts',(-24.0866600683682,-12.4263955990476,
114.149989231708)) ;
#169553=CARTESIAN_POINT('Ctrl Pts',(-24.1604639281124,-12.4263956104993,
114.125758239743)) ;
#169554=CARTESIAN_POINT('Ctrl Pts',(-24.1650595916895,-12.3519340543648,
114.139755888456)) ;
#169555=CARTESIAN_POINT('Ctrl Pts',(-24.1696552552667,-12.2774724982303,
114.153753537168)) ;
#169556=CARTESIAN_POINT('Ctrl Pts',(-24.0958513955224,-12.2774724867786,
114.177984529133)) ;
#169557=CARTESIAN_POINT('Ctrl Pts',(-24.0220475357782,-12.2774724753269,
114.202215521098)) ;
#169558=CARTESIAN_POINT('Ctrl Pts',(-24.017451872201,-12.3519340314614,
114.188217872385)) ;
#169559=CARTESIAN_POINT('Ctrl Pts',(-24.113519984847,-12.4474402254027,
114.445443546699)) ;
#169560=CARTESIAN_POINT('Ctrl Pts',(-24.1029419026619,-12.5153461039576,
114.413224416014)) ;
#169561=CARTESIAN_POINT('Ctrl Pts',(-24.1767457586865,-12.5153461252544,
114.38899341272)) ;
#169562=CARTESIAN_POINT('Ctrl Pts',(-24.250549614711,-12.5153461465513,
114.364762409425)) ;
#169563=CARTESIAN_POINT('Ctrl Pts',(-24.2611276968961,-12.4474402679963,
114.39698154011)) ;
#169564=CARTESIAN_POINT('Ctrl Pts',(-24.2717057790811,-12.3795343894413,
114.429200670795)) ;
#169565=CARTESIAN_POINT('Ctrl Pts',(-24.1979019230565,-12.3795343681445,
114.45343167409)) ;
#169566=CARTESIAN_POINT('Ctrl Pts',(-24.124098067032,-12.3795343468477,
114.477662677384)) ;
#169567=CARTESIAN_POINT('Ctrl Pts',(-24.113519984847,-12.4474402254027,
114.445443546699)) ;
#169568=CARTESIAN_POINT('Ctrl Pts',(-24.1988643834179,-12.6124878626438,
114.669923303231)) ;
#169569=CARTESIAN_POINT('Ctrl Pts',(-24.1830452149199,-12.6689727866278,
114.621740669115)) ;
#169570=CARTESIAN_POINT('Ctrl Pts',(-24.2568490666953,-12.6689728121277,
114.597509652878)) ;
#169571=CARTESIAN_POINT('Ctrl Pts',(-24.3306529184707,-12.6689728376277,
114.573278636642)) ;
#169572=CARTESIAN_POINT('Ctrl Pts',(-24.3464720869687,-12.6124879136438,
114.621461270758)) ;
#169573=CARTESIAN_POINT('Ctrl Pts',(-24.3622912554668,-12.5560029896598,
114.669643904875)) ;
#169574=CARTESIAN_POINT('Ctrl Pts',(-24.2884874036914,-12.5560029641598,
114.693874921111)) ;
#169575=CARTESIAN_POINT('Ctrl Pts',(-24.214683551916,-12.5560029386599,
114.718105937348)) ;
#169576=CARTESIAN_POINT('Ctrl Pts',(-24.1988643834179,-12.6124878626438,
114.669923303231)) ;
#169577=CARTESIAN_POINT('Ctrl Pts',(-24.2679912812749,-12.8359789539693,
114.844917416136)) ;
#169578=CARTESIAN_POINT('Ctrl Pts',(-24.2480571471312,-12.8769447916209,
114.78420126043)) ;
#169579=CARTESIAN_POINT('Ctrl Pts',(-24.3218609949561,-12.8769448154243,
114.759970232161)) ;
#169580=CARTESIAN_POINT('Ctrl Pts',(-24.395664842781,-12.8769448392277,
114.735739203891)) ;
#169581=CARTESIAN_POINT('Ctrl Pts',(-24.4155989769246,-12.8359790015761,
114.796455359597)) ;
#169582=CARTESIAN_POINT('Ctrl Pts',(-24.4355331110683,-12.7950131639245,
114.857171515303)) ;
#169583=CARTESIAN_POINT('Ctrl Pts',(-24.3617292632435,-12.7950131401211,
114.881402543573)) ;
#169584=CARTESIAN_POINT('Ctrl Pts',(-24.2879254154186,-12.7950131163177,
114.905633571842)) ;
#169585=CARTESIAN_POINT('Ctrl Pts',(-24.2679912812749,-12.8359789539693,
114.844917416136)) ;
#169586=CARTESIAN_POINT('Ctrl Pts',(-24.3163387004766,-13.1004046039055,
114.956742952325)) ;
#169587=CARTESIAN_POINT('Ctrl Pts',(-24.2937318355072,-13.1229691360916,
114.887886089619)) ;
#169588=CARTESIAN_POINT('Ctrl Pts',(-24.3675356805423,-13.1229691554338,
114.863655052853)) ;
#169589=CARTESIAN_POINT('Ctrl Pts',(-24.4413395255774,-13.1229691747759,
114.839424016087)) ;
#169590=CARTESIAN_POINT('Ctrl Pts',(-24.4639463905468,-13.1004046425898,
114.908280878792)) ;
#169591=CARTESIAN_POINT('Ctrl Pts',(-24.4865532555163,-13.0778401104037,
114.977137741498)) ;
#169592=CARTESIAN_POINT('Ctrl Pts',(-24.4127494104811,-13.0778400910615,
115.001368778264)) ;
#169593=CARTESIAN_POINT('Ctrl Pts',(-24.338945565446,-13.0778400717194,
115.02559981503)) ;
#169594=CARTESIAN_POINT('Ctrl Pts',(-24.3163387004766,-13.1004046039055,
114.956742952325)) ;
#169595=CARTESIAN_POINT('Ctrl Pts',(-24.3415133892028,-13.3877822848103,
114.997954547246)) ;
#169596=CARTESIAN_POINT('Ctrl Pts',(-24.3178484788146,-13.3903147860949,
114.925875048769)) ;
#169597=CARTESIAN_POINT('Ctrl Pts',(-24.3916523221406,-13.3903147988625,
114.901644006797)) ;
#169598=CARTESIAN_POINT('Ctrl Pts',(-24.4654561654666,-13.3903148116302,
114.877412964825)) ;
#169599=CARTESIAN_POINT('Ctrl Pts',(-24.4891210758549,-13.3877823103455,
114.949492463302)) ;
#169600=CARTESIAN_POINT('Ctrl Pts',(-24.5127859862431,-13.3852498090609,
115.021571961778)) ;
#169601=CARTESIAN_POINT('Ctrl Pts',(-24.438982142917,-13.3852497962932,
115.04580300375)) ;
#169602=CARTESIAN_POINT('Ctrl Pts',(-24.365178299591,-13.3852497835256,
115.070034045722)) ;
#169603=CARTESIAN_POINT('Ctrl Pts',(-24.3415133892028,-13.3877822848103,
114.997954547246)) ;
#169604=CARTESIAN_POINT('Ctrl Pts',(-24.3423651713577,-13.6773386169807,
114.965081433948)) ;
#169605=CARTESIAN_POINT('Ctrl Pts',(-24.3193390920628,-13.6596563698358,
114.894947711785)) ;
#169606=CARTESIAN_POINT('Ctrl Pts',(-24.3931429348365,-13.659656376027,
114.870716668131)) ;
#169607=CARTESIAN_POINT('Ctrl Pts',(-24.4669467776103,-13.6596563822181,
114.846485624477)) ;
#169608=CARTESIAN_POINT('Ctrl Pts',(-24.4899728569052,-13.6773386293631,
114.916619346639)) ;
#169609=CARTESIAN_POINT('Ctrl Pts',(-24.5129989362001,-13.695020876508,
114.986753068802)) ;
#169610=CARTESIAN_POINT('Ctrl Pts',(-24.4391950934264,-13.6950208703168,
115.010984112456)) ;
#169611=CARTESIAN_POINT('Ctrl Pts',(-24.3653912506526,-13.6950208641256,
115.03521515611)) ;
#169612=CARTESIAN_POINT('Ctrl Pts',(-24.3423651713577,-13.6773386169807,
114.965081433948)) ;
#169613=CARTESIAN_POINT('Ctrl Pts',(-24.3196433120407,-13.9481535278235,
114.860433233373)) ;
#169614=CARTESIAN_POINT('Ctrl Pts',(-24.2989026954842,-13.9115346180425,
114.797260661859)) ;
#169615=CARTESIAN_POINT('Ctrl Pts',(-24.3727065385483,-13.9115346192683,
114.773029619089)) ;
#169616=CARTESIAN_POINT('Ctrl Pts',(-24.4465103816125,-13.9115346204941,
114.74879857632)) ;
#169617=CARTESIAN_POINT('Ctrl Pts',(-24.467250998169,-13.948153530275,114.811971147834)) ;
#169618=CARTESIAN_POINT('Ctrl Pts',(-24.4879916147256,-13.984772440056,
114.875143719347)) ;
#169619=CARTESIAN_POINT('Ctrl Pts',(-24.4141877716614,-13.9847724388302,
114.899374762117)) ;
#169620=CARTESIAN_POINT('Ctrl Pts',(-24.3403839285972,-13.9847724376044,
114.923605804887)) ;
#169621=CARTESIAN_POINT('Ctrl Pts',(-24.3196433120407,-13.9481535278235,
114.860433233373)) ;
#169622=CARTESIAN_POINT('Ctrl Pts',(-24.2756541802911,-14.1811353756388,
114.690976851647)) ;
#169623=CARTESIAN_POINT('Ctrl Pts',(-24.2586883222684,-14.1281930358969,
114.639301585507)) ;
#169624=CARTESIAN_POINT('Ctrl Pts',(-24.3324921660103,-14.1281930344687,
114.615070544802)) ;
#169625=CARTESIAN_POINT('Ctrl Pts',(-24.4062960097522,-14.1281930330404,
114.590839504097)) ;
#169626=CARTESIAN_POINT('Ctrl Pts',(-24.4232618677749,-14.1811353727823,
114.642514770237)) ;
#169627=CARTESIAN_POINT('Ctrl Pts',(-24.4402277257976,-14.2340777125242,
114.694190036376)) ;
#169628=CARTESIAN_POINT('Ctrl Pts',(-24.3664238820557,-14.2340777139524,
114.718421077082)) ;
#169629=CARTESIAN_POINT('Ctrl Pts',(-24.2926200383138,-14.2340777153806,
114.742652117787)) ;
#169630=CARTESIAN_POINT('Ctrl Pts',(-24.2756541802911,-14.1811353756388,
114.690976851647)) ;
#169631=CARTESIAN_POINT('Ctrl Pts',(-24.21454103563,-14.3592804603128,114.469454230547)) ;
#169632=CARTESIAN_POINT('Ctrl Pts',(-24.2025496065343,-14.2938199374356,
114.432930272264)) ;
#169633=CARTESIAN_POINT('Ctrl Pts',(-24.2763534508764,-14.2938199356805,
114.408699233387)) ;
#169634=CARTESIAN_POINT('Ctrl Pts',(-24.3501572952184,-14.2938199339254,
114.384468194509)) ;
#169635=CARTESIAN_POINT('Ctrl Pts',(-24.362148724314,-14.3592804568026,
114.420992152792)) ;
#169636=CARTESIAN_POINT('Ctrl Pts',(-24.3741401534097,-14.4247409796798,
114.457516111074)) ;
#169637=CARTESIAN_POINT('Ctrl Pts',(-24.3003363090677,-14.4247409814349,
114.481747149952)) ;
#169638=CARTESIAN_POINT('Ctrl Pts',(-24.2265324647257,-14.4247409831899,
114.505978188829)) ;
#169639=CARTESIAN_POINT('Ctrl Pts',(-24.21454103563,-14.3592804603128,114.469454230547)) ;
#169640=CARTESIAN_POINT('Ctrl Pts',(-24.1405314237191,-14.4707867328028,
114.208317405989)) ;
#169641=CARTESIAN_POINT('Ctrl Pts',(-24.1344295829411,-14.3974420670784,
114.189732183463)) ;
#169642=CARTESIAN_POINT('Ctrl Pts',(-24.2082334270705,-14.3974420666518,
114.165501143937)) ;
#169643=CARTESIAN_POINT('Ctrl Pts',(-24.2820372711998,-14.3974420662252,
114.141270104412)) ;
#169644=CARTESIAN_POINT('Ctrl Pts',(-24.2881391119777,-14.4707867319496,
114.159855326938)) ;
#169645=CARTESIAN_POINT('Ctrl Pts',(-24.2942409527556,-14.5441313976739,
114.178440549464)) ;
#169646=CARTESIAN_POINT('Ctrl Pts',(-24.2204371086263,-14.5441313981005,
114.20267158899)) ;
#169647=CARTESIAN_POINT('Ctrl Pts',(-24.146633264497,-14.5441313985271,
114.226902628515)) ;
#169648=CARTESIAN_POINT('Ctrl Pts',(-24.1405314237191,-14.4707867328028,
114.208317405989)) ;
#169649=CARTESIAN_POINT('Ctrl Pts',(-24.0613460516658,-14.5057904984994,
113.931879153805)) ;
#169650=CARTESIAN_POINT('Ctrl Pts',(-24.0614939657,-14.429894649573,113.932329676088)) ;
#169651=CARTESIAN_POINT('Ctrl Pts',(-24.1352978090977,-14.4298946498541,
113.908098634334)) ;
#169652=CARTESIAN_POINT('Ctrl Pts',(-24.2091016524954,-14.4298946501351,
113.88386759258)) ;
#169653=CARTESIAN_POINT('Ctrl Pts',(-24.2089537384612,-14.5057904990616,
113.883417070297)) ;
#169654=CARTESIAN_POINT('Ctrl Pts',(-24.208805824427,-14.581686347988,113.882966548014)) ;
#169655=CARTESIAN_POINT('Ctrl Pts',(-24.1350019810292,-14.5816863477069,
113.907197589767)) ;
#169656=CARTESIAN_POINT('Ctrl Pts',(-24.0611981376315,-14.5816863474258,
113.931428631521)) ;
#169657=CARTESIAN_POINT('Ctrl Pts',(-24.0613460516658,-14.5057904984994,
113.931879153805)) ;
#169658=CARTESIAN_POINT('Ctrl Pts',(-23.981949761782,-14.4636194148643,
113.654568691097)) ;
#169659=CARTESIAN_POINT('Ctrl Pts',(-23.9883761002209,-14.3905570608512,
113.67414228118)) ;
#169660=CARTESIAN_POINT('Ctrl Pts',(-24.062179942285,-14.3905570601267,
113.649911235364)) ;
#169661=CARTESIAN_POINT('Ctrl Pts',(-24.135983784349,-14.3905570594022,
113.625680189548)) ;
#169662=CARTESIAN_POINT('Ctrl Pts',(-24.1295574459101,-14.4636194134152,
113.606106599465)) ;
#169663=CARTESIAN_POINT('Ctrl Pts',(-24.1231311074711,-14.5366817674283,
113.586533009382)) ;
#169664=CARTESIAN_POINT('Ctrl Pts',(-24.0493272654071,-14.5366817681528,
113.610764055198)) ;
#169665=CARTESIAN_POINT('Ctrl Pts',(-23.9755234233431,-14.5366817688773,
113.634995101014)) ;
#169666=CARTESIAN_POINT('Ctrl Pts',(-23.981949761782,-14.4636194148643,
113.654568691097)) ;
#169667=CARTESIAN_POINT('Ctrl Pts',(-23.9092977046696,-14.3461280489561,
113.397794692953)) ;
#169668=CARTESIAN_POINT('Ctrl Pts',(-23.9215407074399,-14.2811630148822,
113.435084904191)) ;
#169669=CARTESIAN_POINT('Ctrl Pts',(-23.9953445480101,-14.2811630098894,
113.410853853825)) ;
#169670=CARTESIAN_POINT('Ctrl Pts',(-24.0691483885803,-14.2811630048965,
113.386622803459)) ;
#169671=CARTESIAN_POINT('Ctrl Pts',(-24.05690538581,-14.3461280389704,113.349332592221)) ;
#169672=CARTESIAN_POINT('Ctrl Pts',(-24.0446623830397,-14.4110930730442,
113.312042380983)) ;
#169673=CARTESIAN_POINT('Ctrl Pts',(-23.9708585424695,-14.4110930780371,
113.336273431349)) ;
#169674=CARTESIAN_POINT('Ctrl Pts',(-23.8970547018993,-14.41109308303,113.360504481715)) ;
#169675=CARTESIAN_POINT('Ctrl Pts',(-23.9092977046696,-14.3461280489561,
113.397794692953)) ;
#169676=CARTESIAN_POINT('Ctrl Pts',(-23.8494456096459,-14.1630186070769,
113.180123238634)) ;
#169677=CARTESIAN_POINT('Ctrl Pts',(-23.8666173455508,-14.1107446176607,
113.232425575869)) ;
#169678=CARTESIAN_POINT('Ctrl Pts',(-23.940421185266,-14.1107446061865,
113.208194522899)) ;
#169679=CARTESIAN_POINT('Ctrl Pts',(-24.0142250249813,-14.1107445947124,
113.183963469929)) ;
#169680=CARTESIAN_POINT('Ctrl Pts',(-23.9970532890764,-14.1630185841287,
113.131661132695)) ;
#169681=CARTESIAN_POINT('Ctrl Pts',(-23.9798815531715,-14.215292573545,
113.07935879546)) ;
#169682=CARTESIAN_POINT('Ctrl Pts',(-23.9060777134563,-14.2152925850191,
113.10358984843)) ;
#169683=CARTESIAN_POINT('Ctrl Pts',(-23.832273873741,-14.2152925964932,
113.1278209014)) ;
#169684=CARTESIAN_POINT('Ctrl Pts',(-23.8494456096459,-14.1630186070769,
113.180123238634)) ;
#169685=CARTESIAN_POINT('Ctrl Pts',(-23.8069643592986,-13.9239936072657,
113.01499355577)) ;
#169686=CARTESIAN_POINT('Ctrl Pts',(-23.8278669143801,-13.8883328136029,
113.078659366449)) ;
#169687=CARTESIAN_POINT('Ctrl Pts',(-23.9016707537285,-13.8883327903774,
113.054428312361)) ;
#169688=CARTESIAN_POINT('Ctrl Pts',(-23.9754745930768,-13.8883327671519,
113.030197258274)) ;
#169689=CARTESIAN_POINT('Ctrl Pts',(-23.9545720379952,-13.9239935608147,
112.966531447595)) ;
#169690=CARTESIAN_POINT('Ctrl Pts',(-23.9336694829136,-13.9596543544774,
112.902865636916)) ;
#169691=CARTESIAN_POINT('Ctrl Pts',(-23.8598656435653,-13.9596543777029,
112.927096691003)) ;
#169692=CARTESIAN_POINT('Ctrl Pts',(-23.7860618042169,-13.9596544009284,
112.951327745091)) ;
#169693=CARTESIAN_POINT('Ctrl Pts',(-23.8069643592986,-13.9239936072657,
113.01499355577)) ;
#169694=CARTESIAN_POINT('Ctrl Pts',(-23.7864462608402,-13.6520857920573,
112.917251285057)) ;
#169695=CARTESIAN_POINT('Ctrl Pts',(-23.8095408056918,-13.6353584241277,
112.987593543021)) ;
#169696=CARTESIAN_POINT('Ctrl Pts',(-23.8833446466771,-13.6353583920573,
112.96336249392)) ;
#169697=CARTESIAN_POINT('Ctrl Pts',(-23.9571484876624,-13.635358359987,
112.939131444818)) ;
#169698=CARTESIAN_POINT('Ctrl Pts',(-23.9340539428108,-13.6520857279166,
112.868789186854)) ;
#169699=CARTESIAN_POINT('Ctrl Pts',(-23.9109593979592,-13.6688130958462,
112.79844692889)) ;
#169700=CARTESIAN_POINT('Ctrl Pts',(-23.8371555569739,-13.6688131279166,
112.822677977992)) ;
#169701=CARTESIAN_POINT('Ctrl Pts',(-23.7633517159886,-13.668813159987,
112.846909027093)) ;
#169702=CARTESIAN_POINT('Ctrl Pts',(-23.7864462608402,-13.6520857920573,
112.917251285057)) ;
#169703=CARTESIAN_POINT('Ctrl Pts',(-23.7894943758897,-13.3607989189298,
112.890930631403)) ;
#169704=CARTESIAN_POINT('Ctrl Pts',(-23.8131463729172,-13.3643850289944,
112.962970798943)) ;
#169705=CARTESIAN_POINT('Ctrl Pts',(-23.8869502167856,-13.3643849861059,
112.938739758623)) ;
#169706=CARTESIAN_POINT('Ctrl Pts',(-23.9607540606539,-13.3643849432174,
112.914508718302)) ;
#169707=CARTESIAN_POINT('Ctrl Pts',(-23.9371020636264,-13.3607988331528,
112.842468550762)) ;
#169708=CARTESIAN_POINT('Ctrl Pts',(-23.9134500665988,-13.3572127230881,
112.770428383222)) ;
#169709=CARTESIAN_POINT('Ctrl Pts',(-23.8396462227305,-13.3572127659766,
112.794659423543)) ;
#169710=CARTESIAN_POINT('Ctrl Pts',(-23.7658423788621,-13.3572128088652,
112.818890463863)) ;
#169711=CARTESIAN_POINT('Ctrl Pts',(-23.7894943758897,-13.3607989189298,
112.890930631403)) ;
#169712=CARTESIAN_POINT('Ctrl Pts',(-23.8167514278251,-13.0758433976518,
112.938634896679)) ;
#169713=CARTESIAN_POINT('Ctrl Pts',(-23.8392651657168,-13.0993300266372,
113.007208110689)) ;
#169714=CARTESIAN_POINT('Ctrl Pts',(-23.9130690138605,-13.0993299787843,
112.982977083391)) ;
#169715=CARTESIAN_POINT('Ctrl Pts',(-23.9868728620042,-13.0993299309314,
112.958746056093)) ;
#169716=CARTESIAN_POINT('Ctrl Pts',(-23.9643591241125,-13.075843301946,
112.890172842083)) ;
#169717=CARTESIAN_POINT('Ctrl Pts',(-23.9418453862208,-13.0523566729605,
112.821599628073)) ;
#169718=CARTESIAN_POINT('Ctrl Pts',(-23.8680415380771,-13.0523567208134,
112.845830655371)) ;
#169719=CARTESIAN_POINT('Ctrl Pts',(-23.7942376899334,-13.0523567686663,
112.870061682669)) ;
#169720=CARTESIAN_POINT('Ctrl Pts',(-23.8167514278251,-13.0758433976518,
112.938634896679)) ;
#169721=CARTESIAN_POINT('Ctrl Pts',(-23.8671295596071,-12.8137701829539,
113.056567674092)) ;
#169722=CARTESIAN_POINT('Ctrl Pts',(-23.8868933516135,-12.8555883335488,
113.116764996813)) ;
#169723=CARTESIAN_POINT('Ctrl Pts',(-23.9606972050676,-12.8555882837421,
113.092533985689)) ;
#169724=CARTESIAN_POINT('Ctrl Pts',(-24.0345010585216,-12.8555882339354,
113.068302974566)) ;
#169725=CARTESIAN_POINT('Ctrl Pts',(-24.0147372665152,-12.8137700833405,
113.008105651844)) ;
#169726=CARTESIAN_POINT('Ctrl Pts',(-23.9949734745088,-12.7719519327456,
112.947908329123)) ;
#169727=CARTESIAN_POINT('Ctrl Pts',(-23.9211696210548,-12.7719519825523,
112.972139340247)) ;
#169728=CARTESIAN_POINT('Ctrl Pts',(-23.8473657676007,-12.771952032359,
112.99637035137)) ;
#169729=CARTESIAN_POINT('Ctrl Pts',(-23.8671295596071,-12.8137701829539,
113.056567674092)) ;
#169730=CARTESIAN_POINT('Ctrl Pts',(-23.9380620209041,-12.5948352961054,
113.237023873309)) ;
#169731=CARTESIAN_POINT('Ctrl Pts',(-23.9536386278267,-12.6519997752805,
113.284467706048)) ;
#169732=CARTESIAN_POINT('Ctrl Pts',(-24.0274424873426,-12.6519997298115,
113.260236713388)) ;
#169733=CARTESIAN_POINT('Ctrl Pts',(-24.1012463468584,-12.6519996843424,
113.236005720728)) ;
#169734=CARTESIAN_POINT('Ctrl Pts',(-24.0856697399359,-12.5948352051674,
113.188561887988)) ;
#169735=CARTESIAN_POINT('Ctrl Pts',(-24.0700931330132,-12.5376707259923,
113.141118055248)) ;
#169736=CARTESIAN_POINT('Ctrl Pts',(-23.9962892734974,-12.5376707714613,
113.165349047909)) ;
#169737=CARTESIAN_POINT('Ctrl Pts',(-23.9224854139815,-12.5376708169303,
113.189580040569)) ;
#169738=CARTESIAN_POINT('Ctrl Pts',(-23.9380620209041,-12.5948352961054,
113.237023873309)) ;
#169739=CARTESIAN_POINT('Ctrl Pts',(-24.0241344799407,-12.4363827345609,
113.463912936618)) ;
#169740=CARTESIAN_POINT('Ctrl Pts',(-24.034454027819,-12.5046923403289,
113.495344615851)) ;
#169741=CARTESIAN_POINT('Ctrl Pts',(-24.1082578922502,-12.5046923075435,
113.471113638162)) ;
#169742=CARTESIAN_POINT('Ctrl Pts',(-24.1820617566815,-12.5046922747581,
113.446882660473)) ;
#169743=CARTESIAN_POINT('Ctrl Pts',(-24.1717422088033,-12.4363826689901,
113.415450981241)) ;
#169744=CARTESIAN_POINT('Ctrl Pts',(-24.1614226609251,-12.368073063222,
113.384019302008)) ;
#169745=CARTESIAN_POINT('Ctrl Pts',(-24.0876187964938,-12.3680730960074,
113.408250279697)) ;
#169746=CARTESIAN_POINT('Ctrl Pts',(-24.0138149320625,-12.3680731287928,
113.432481257386)) ;
#169747=CARTESIAN_POINT('Ctrl Pts',(-24.0241344799407,-12.4363827345609,
113.463912936618)) ;
#169748=CARTESIAN_POINT('Ctrl Pts',(-24.1211715621355,-12.3469185629382,
113.723977397692)) ;
#169749=CARTESIAN_POINT('Ctrl Pts',(-24.1254657239507,-12.4215734203002,
113.737056723317)) ;
#169750=CARTESIAN_POINT('Ctrl Pts',(-24.1992695926889,-12.4215734050828,
113.712825758746)) ;
#169751=CARTESIAN_POINT('Ctrl Pts',(-24.2730734614271,-12.4215733898654,
113.688594794176)) ;
#169752=CARTESIAN_POINT('Ctrl Pts',(-24.2687792996119,-12.3469185325034,
113.675515468551)) ;
#169753=CARTESIAN_POINT('Ctrl Pts',(-24.2644851377967,-12.2722636751415,
113.662436142925)) ;
#169754=CARTESIAN_POINT('Ctrl Pts',(-24.1906812690584,-12.2722636903589,
113.686667107496)) ;
#169755=CARTESIAN_POINT('Ctrl Pts',(-24.1168774003202,-12.2722637055763,
113.710898072066)) ;
#169756=CARTESIAN_POINT('Ctrl Pts',(-24.1211715621355,-12.3469185629382,
113.723977397692)) ;
#169757=CARTESIAN_POINT('Ctrl Pts',(-24.2227254729925,-12.3346897142696,
113.997726976907)) ;
#169758=CARTESIAN_POINT('Ctrl Pts',(-24.2206716932284,-12.410307219777,
113.991471496858)) ;
#169759=CARTESIAN_POINT('Ctrl Pts',(-24.2944755645646,-12.4103072275808,
113.967240540201)) ;
#169760=CARTESIAN_POINT('Ctrl Pts',(-24.3682794359007,-12.4103072353845,
113.943009583543)) ;
#169761=CARTESIAN_POINT('Ctrl Pts',(-24.3703332156647,-12.3346897298771,
113.949265063591)) ;
#169762=CARTESIAN_POINT('Ctrl Pts',(-24.3723869954288,-12.2590722243697,
113.95552054364)) ;
#169763=CARTESIAN_POINT('Ctrl Pts',(-24.2985831240927,-12.259072216566,
113.979751500297)) ;
#169764=CARTESIAN_POINT('Ctrl Pts',(-24.2247792527566,-12.2590722087622,
114.003982456955)) ;
#169765=CARTESIAN_POINT('Ctrl Pts',(-24.2227254729925,-12.3346897142696,
113.997726976907)) ;
#169766=CARTESIAN_POINT('Ctrl Pts',(-24.3213836615378,-12.3996707792268,
114.262894713048)) ;
#169767=CARTESIAN_POINT('Ctrl Pts',(-24.3131699295231,-12.470861286488,
114.237877012443)) ;
#169768=CARTESIAN_POINT('Ctrl Pts',(-24.3869738006343,-12.4708613194526,
114.2136460551)) ;
#169769=CARTESIAN_POINT('Ctrl Pts',(-24.4607776717455,-12.4708613524172,
114.189415097757)) ;
#169770=CARTESIAN_POINT('Ctrl Pts',(-24.4689914037601,-12.3996708451561,
114.214432798363)) ;
#169771=CARTESIAN_POINT('Ctrl Pts',(-24.4772051357748,-12.3284803378949,
114.239450498968)) ;
#169772=CARTESIAN_POINT('Ctrl Pts',(-24.4034012646637,-12.3284803049303,
114.263681456311)) ;
#169773=CARTESIAN_POINT('Ctrl Pts',(-24.3295973935525,-12.3284802719657,
114.287912413654)) ;
#169774=CARTESIAN_POINT('Ctrl Pts',(-24.3213836615378,-12.3996707792268,
114.262894713048)) ;
#169775=CARTESIAN_POINT('Ctrl Pts',(-24.4121011317654,-12.5380776390174,
114.503646698879)) ;
#169776=CARTESIAN_POINT('Ctrl Pts',(-24.3982776140999,-12.5997094329327,
114.461542496421)) ;
#169777=CARTESIAN_POINT('Ctrl Pts',(-24.4720814828292,-12.5997094914945,
114.437311531823)) ;
#169778=CARTESIAN_POINT('Ctrl Pts',(-24.5458853515585,-12.5997095500564,
114.413080567226)) ;
#169779=CARTESIAN_POINT('Ctrl Pts',(-24.559708869224,-12.5380777561411,
114.455184769684)) ;
#169780=CARTESIAN_POINT('Ctrl Pts',(-24.5735323868896,-12.4764459622258,
114.497288972142)) ;
#169781=CARTESIAN_POINT('Ctrl Pts',(-24.4997285181602,-12.476445903664,
114.52151993674)) ;
#169782=CARTESIAN_POINT('Ctrl Pts',(-24.4259246494309,-12.4764458451021,
114.545750901337)) ;
#169783=CARTESIAN_POINT('Ctrl Pts',(-24.4121011317654,-12.5380776390174,
114.503646698879)) ;
#169784=CARTESIAN_POINT('Ctrl Pts',(-24.488256946051,-12.739380812412,114.700140077213)) ;
#169785=CARTESIAN_POINT('Ctrl Pts',(-24.4698300851511,-12.7870487344557,
114.644014834082)) ;
#169786=CARTESIAN_POINT('Ctrl Pts',(-24.5436339488168,-12.7870488154654,
114.619783854061)) ;
#169787=CARTESIAN_POINT('Ctrl Pts',(-24.6174378124824,-12.7870488964751,
114.59555287404)) ;
#169788=CARTESIAN_POINT('Ctrl Pts',(-24.6358646733823,-12.7393809744314,
114.651678117172)) ;
#169789=CARTESIAN_POINT('Ctrl Pts',(-24.6542915342823,-12.6917130523877,
114.707803360304)) ;
#169790=CARTESIAN_POINT('Ctrl Pts',(-24.5804876706166,-12.691712971378,
114.732034340324)) ;
#169791=CARTESIAN_POINT('Ctrl Pts',(-24.506683806951,-12.6917128903682,
114.756265320345)) ;
#169792=CARTESIAN_POINT('Ctrl Pts',(-24.488256946051,-12.739380812412,114.700140077213)) ;
#169793=CARTESIAN_POINT('Ctrl Pts',(-24.5454206194932,-12.9893867745162,
114.838765803688)) ;
#169794=CARTESIAN_POINT('Ctrl Pts',(-24.5237099602011,-13.0196703754918,
114.772638640544)) ;
#169795=CARTESIAN_POINT('Ctrl Pts',(-24.59751381674,-13.0196704733174,114.748407638817)) ;
#169796=CARTESIAN_POINT('Ctrl Pts',(-24.671317673279,-13.019670571143,114.724176637089)) ;
#169797=CARTESIAN_POINT('Ctrl Pts',(-24.6930283325711,-12.9893869701674,
114.790303800233)) ;
#169798=CARTESIAN_POINT('Ctrl Pts',(-24.7147389918632,-12.9591033691919,
114.856430963377)) ;
#169799=CARTESIAN_POINT('Ctrl Pts',(-24.6409351353243,-12.9591032713663,
114.880661965104)) ;
#169800=CARTESIAN_POINT('Ctrl Pts',(-24.5671312787853,-12.9591031735407,
114.904892966831)) ;
#169801=CARTESIAN_POINT('Ctrl Pts',(-24.5454206194932,-12.9893867745162,
114.838765803688)) ;
#169802=CARTESIAN_POINT('Ctrl Pts',(-24.5802165214264,-13.2694171615401,
114.909351828959)) ;
#169803=CARTESIAN_POINT('Ctrl Pts',(-24.5567770069868,-13.2801946819997,
114.837958852016)) ;
#169804=CARTESIAN_POINT('Ctrl Pts',(-24.6305808550088,-13.2801947890163,
114.813727824347)) ;
#169805=CARTESIAN_POINT('Ctrl Pts',(-24.7043847030307,-13.2801948960329,
114.789496796678)) ;
#169806=CARTESIAN_POINT('Ctrl Pts',(-24.7278242174703,-13.2694173755733,
114.860889773621)) ;
#169807=CARTESIAN_POINT('Ctrl Pts',(-24.7512637319099,-13.2586398551137,
114.932282750565)) ;
#169808=CARTESIAN_POINT('Ctrl Pts',(-24.677459883888,-13.2586397480971,
114.956513778234)) ;
#169809=CARTESIAN_POINT('Ctrl Pts',(-24.603656035866,-13.2586396410806,
114.980744805903)) ;
#169810=CARTESIAN_POINT('Ctrl Pts',(-24.5802165214264,-13.2694171615401,
114.909351828959)) ;
#169811=CARTESIAN_POINT('Ctrl Pts',(-24.5909392079198,-13.5619468890867,
114.906377302558)) ;
#169812=CARTESIAN_POINT('Ctrl Pts',(-24.5674535497162,-13.5523172456924,
114.834843779161)) ;
#169813=CARTESIAN_POINT('Ctrl Pts',(-24.6412573886373,-13.5523173531236,
114.810612723773)) ;
#169814=CARTESIAN_POINT('Ctrl Pts',(-24.7150612275583,-13.5523174605549,
114.786381668384)) ;
#169815=CARTESIAN_POINT('Ctrl Pts',(-24.7385468857619,-13.5619471039492,
114.85791519178)) ;
#169816=CARTESIAN_POINT('Ctrl Pts',(-24.7620325439655,-13.5715767473435,
114.929448715177)) ;
#169817=CARTESIAN_POINT('Ctrl Pts',(-24.6882287050445,-13.5715766399123,
114.953679770565)) ;
#169818=CARTESIAN_POINT('Ctrl Pts',(-24.6144248661234,-13.5715765324811,
114.977910825954)) ;
#169819=CARTESIAN_POINT('Ctrl Pts',(-24.5909392079198,-13.5619468890867,
114.906377302558)) ;
#169820=CARTESIAN_POINT('Ctrl Pts',(-24.5776432777125,-13.8411213292838,
114.83064171812)) ;
#169821=CARTESIAN_POINT('Ctrl Pts',(-24.5557804108624,-13.8119862931275,
114.764050955339)) ;
#169822=CARTESIAN_POINT('Ctrl Pts',(-24.6295842411457,-13.8119863923944,
114.739819873641)) ;
#169823=CARTESIAN_POINT('Ctrl Pts',(-24.7033880714288,-13.8119864916613,
114.715588791943)) ;
#169824=CARTESIAN_POINT('Ctrl Pts',(-24.7252509382789,-13.8411215278176,
114.782179554724)) ;
#169825=CARTESIAN_POINT('Ctrl Pts',(-24.7471138051289,-13.870256563974,
114.848770317504)) ;
#169826=CARTESIAN_POINT('Ctrl Pts',(-24.6733099748457,-13.8702564647071,
114.873001399203)) ;
#169827=CARTESIAN_POINT('Ctrl Pts',(-24.5995061445625,-13.8702563654402,
114.897232480901)) ;
#169828=CARTESIAN_POINT('Ctrl Pts',(-24.5776432777125,-13.8411213292838,
114.83064171812)) ;
#169829=CARTESIAN_POINT('Ctrl Pts',(-24.5417994729014,-14.0928083771544,
114.685855733235)) ;
#169830=CARTESIAN_POINT('Ctrl Pts',(-24.5231432551102,-14.0460580395473,
114.629031906056)) ;
#169831=CARTESIAN_POINT('Ctrl Pts',(-24.5969470779918,-14.0460581223417,
114.604800801814)) ;
#169832=CARTESIAN_POINT('Ctrl Pts',(-24.6707509008735,-14.0460582051361,
114.580569697572)) ;
#169833=CARTESIAN_POINT('Ctrl Pts',(-24.6894071186647,-14.0928085427432,
114.637393524751)) ;
#169834=CARTESIAN_POINT('Ctrl Pts',(-24.7080633364559,-14.1395588803503,
114.694217351929)) ;
#169835=CARTESIAN_POINT('Ctrl Pts',(-24.6342595135742,-14.1395587975559,
114.718448456171)) ;
#169836=CARTESIAN_POINT('Ctrl Pts',(-24.5604556906926,-14.1395587147615,
114.742679560413)) ;
#169837=CARTESIAN_POINT('Ctrl Pts',(-24.5417994729014,-14.0928083771544,
114.685855733235)) ;
#169838=CARTESIAN_POINT('Ctrl Pts',(-24.4870105886222,-14.2946225939457,
114.483569102264)) ;
#169839=CARTESIAN_POINT('Ctrl Pts',(-24.4728844270664,-14.2337123839225,
114.4405430954)) ;
#169840=CARTESIAN_POINT('Ctrl Pts',(-24.5466882445676,-14.2337124445756,
114.41631197477)) ;
#169841=CARTESIAN_POINT('Ctrl Pts',(-24.6204920620688,-14.2337125052288,
114.39208085414)) ;
#169842=CARTESIAN_POINT('Ctrl Pts',(-24.6346182236247,-14.2946227152521,
114.435106861004)) ;
#169843=CARTESIAN_POINT('Ctrl Pts',(-24.6487443851805,-14.3555329252753,
114.478132867868)) ;
#169844=CARTESIAN_POINT('Ctrl Pts',(-24.5749405676793,-14.3555328646222,
114.502363988498)) ;
#169845=CARTESIAN_POINT('Ctrl Pts',(-24.5011367501781,-14.355532803969,
114.526595109128)) ;
#169846=CARTESIAN_POINT('Ctrl Pts',(-24.4870105886222,-14.2946225939457,
114.483569102264)) ;
#169847=CARTESIAN_POINT('Ctrl Pts',(-24.4178592615303,-14.4342154714355,
114.237501249069)) ;
#169848=CARTESIAN_POINT('Ctrl Pts',(-24.4092733028564,-14.3634681415102,
114.211349806201)) ;
#169849=CARTESIAN_POINT('Ctrl Pts',(-24.483077117361,-14.3634681764234,
114.187118676444)) ;
#169850=CARTESIAN_POINT('Ctrl Pts',(-24.5568809318657,-14.3634682113365,
114.162887546687)) ;
#169851=CARTESIAN_POINT('Ctrl Pts',(-24.5654668905395,-14.4342155412618,
114.189038989554)) ;
#169852=CARTESIAN_POINT('Ctrl Pts',(-24.5740528492134,-14.5049628711871,
114.215190432422)) ;
#169853=CARTESIAN_POINT('Ctrl Pts',(-24.5002490347088,-14.5049628362739,
114.239421562179)) ;
#169854=CARTESIAN_POINT('Ctrl Pts',(-24.4264452202042,-14.5049628013607,
114.263652691936)) ;
#169855=CARTESIAN_POINT('Ctrl Pts',(-24.4178592615303,-14.4342154714355,
114.237501249069)) ;
#169856=CARTESIAN_POINT('Ctrl Pts',(-24.3396042038614,-14.5009486089819,
113.96352975376)) ;
#169857=CARTESIAN_POINT('Ctrl Pts',(-24.3372058944274,-14.4254353908754,
113.956224891987)) ;
#169858=CARTESIAN_POINT('Ctrl Pts',(-24.4110097089487,-14.4254353992881,
113.93199376228)) ;
#169859=CARTESIAN_POINT('Ctrl Pts',(-24.4848135234698,-14.4254354077009,
113.907762632573)) ;
#169860=CARTESIAN_POINT('Ctrl Pts',(-24.4872118329038,-14.5009486258073,
113.915067494347)) ;
#169861=CARTESIAN_POINT('Ctrl Pts',(-24.4896101423378,-14.5764618439138,
113.92237235612)) ;
#169862=CARTESIAN_POINT('Ctrl Pts',(-24.4158063278166,-14.5764618355011,
113.946603485826)) ;
#169863=CARTESIAN_POINT('Ctrl Pts',(-24.3420025132954,-14.5764618270883,
113.970834615533)) ;
#169864=CARTESIAN_POINT('Ctrl Pts',(-24.3396042038614,-14.5009486089819,
113.96352975376)) ;
#169865=CARTESIAN_POINT('Ctrl Pts',(-24.2597681290623,-14.4900601303297,
113.68508815172)) ;
#169866=CARTESIAN_POINT('Ctrl Pts',(-24.2636701688541,-14.4151940072696,
113.69697313704)) ;
#169867=CARTESIAN_POINT('Ctrl Pts',(-24.3374739851644,-14.4151939916633,
113.672742012783)) ;
#169868=CARTESIAN_POINT('Ctrl Pts',(-24.4112778014747,-14.4151939760569,
113.648510888525)) ;
#169869=CARTESIAN_POINT('Ctrl Pts',(-24.4073757616829,-14.490060099117,
113.636625903205)) ;
#169870=CARTESIAN_POINT('Ctrl Pts',(-24.4034737218912,-14.564926222177,
113.624740917885)) ;
#169871=CARTESIAN_POINT('Ctrl Pts',(-24.3296699055809,-14.5649262377834,
113.648972042142)) ;
#169872=CARTESIAN_POINT('Ctrl Pts',(-24.2558660892706,-14.5649262533898,
113.6732031664)) ;
#169873=CARTESIAN_POINT('Ctrl Pts',(-24.2597681290623,-14.4900601303297,
113.68508815172)) ;
#169874=CARTESIAN_POINT('Ctrl Pts',(-24.1834123171793,-14.4021465802023,
113.416932198274)) ;
#169875=CARTESIAN_POINT('Ctrl Pts',(-24.1933877112254,-14.3333051056759,
113.447315640572)) ;
#169876=CARTESIAN_POINT('Ctrl Pts',(-24.2671915319703,-14.3333050707066,
113.423084529822)) ;
#169877=CARTESIAN_POINT('Ctrl Pts',(-24.3409953527152,-14.3333050357374,
113.398853419072)) ;
#169878=CARTESIAN_POINT('Ctrl Pts',(-24.3310199586691,-14.4021465102638,
113.368469976773)) ;
#169879=CARTESIAN_POINT('Ctrl Pts',(-24.321044564623,-14.4709879847903,
113.338086534475)) ;
#169880=CARTESIAN_POINT('Ctrl Pts',(-24.2472407438781,-14.4709880197595,
113.362317645225)) ;
#169881=CARTESIAN_POINT('Ctrl Pts',(-24.1734369231332,-14.4709880547288,
113.386548755976)) ;
#169882=CARTESIAN_POINT('Ctrl Pts',(-24.1834123171793,-14.4021465802023,
113.416932198274)) ;
#169883=CARTESIAN_POINT('Ctrl Pts',(-24.1178153865265,-14.2443882215466,
113.181766630605)) ;
#169884=CARTESIAN_POINT('Ctrl Pts',(-24.1331176094938,-14.1864574930971,
113.228374734188)) ;
#169885=CARTESIAN_POINT('Ctrl Pts',(-24.206921435554,-14.1864574444021,
113.204143639628)) ;
#169886=CARTESIAN_POINT('Ctrl Pts',(-24.2807252616142,-14.1864573957072,
113.179912545067)) ;
#169887=CARTESIAN_POINT('Ctrl Pts',(-24.2654230386468,-14.2443881241568,
113.133304441483)) ;
#169888=CARTESIAN_POINT('Ctrl Pts',(-24.2501208156794,-14.3023188526063,
113.0866963379)) ;
#169889=CARTESIAN_POINT('Ctrl Pts',(-24.1763169896193,-14.3023189013012,
113.110927432461)) ;
#169890=CARTESIAN_POINT('Ctrl Pts',(-24.1025131635591,-14.3023189499961,
113.135158527022)) ;
#169891=CARTESIAN_POINT('Ctrl Pts',(-24.1178153865265,-14.2443882215466,
113.181766630605)) ;
#169892=CARTESIAN_POINT('Ctrl Pts',(-24.0676784811312,-14.0257063779415,
112.993394903444)) ;
#169893=CARTESIAN_POINT('Ctrl Pts',(-24.0872425216887,-13.9829558305902,
113.052983815574)) ;
#169894=CARTESIAN_POINT('Ctrl Pts',(-24.1610463541072,-13.9829557770323,
113.028752740379)) ;
#169895=CARTESIAN_POINT('Ctrl Pts',(-24.2348501865257,-13.9829557234744,
113.004521665184)) ;
#169896=CARTESIAN_POINT('Ctrl Pts',(-24.2152861459681,-14.0257062708258,
112.944932753054)) ;
#169897=CARTESIAN_POINT('Ctrl Pts',(-24.1957221054106,-14.0684568181771,
112.885343840924)) ;
#169898=CARTESIAN_POINT('Ctrl Pts',(-24.1219182729921,-14.068456871735,
112.909574916119)) ;
#169899=CARTESIAN_POINT('Ctrl Pts',(-24.0481144405737,-14.0684569252929,
112.933805991313)) ;
#169900=CARTESIAN_POINT('Ctrl Pts',(-24.0676784811312,-14.0257063779415,
112.993394903444)) ;
#169901=CARTESIAN_POINT('Ctrl Pts',(-24.0381389778697,-13.7667943185538,
112.86824672277)) ;
#169902=CARTESIAN_POINT('Ctrl Pts',(-24.0605227986181,-13.7420568683352,
112.936424230282)) ;
#169903=CARTESIAN_POINT('Ctrl Pts',(-24.1343266364055,-13.7420568128391,
112.91219317144)) ;
#169904=CARTESIAN_POINT('Ctrl Pts',(-24.2081304741928,-13.7420567573429,
112.887962112598)) ;
#169905=CARTESIAN_POINT('Ctrl Pts',(-24.1857466534444,-13.7667942075616,
112.819784605086)) ;
#169906=CARTESIAN_POINT('Ctrl Pts',(-24.1633628326959,-13.7915316577803,
112.751607097573)) ;
#169907=CARTESIAN_POINT('Ctrl Pts',(-24.0895589949086,-13.7915317132764,
112.775838156415)) ;
#169908=CARTESIAN_POINT('Ctrl Pts',(-24.0157551571213,-13.7915317687725,
112.800069215258)) ;
#169909=CARTESIAN_POINT('Ctrl Pts',(-24.0381389778697,-13.7667943185538,
112.86824672277)) ;
#169910=CARTESIAN_POINT('Ctrl Pts',(-24.0313067339811,-13.4796298971122,
112.81179860376)) ;
#169911=CARTESIAN_POINT('Ctrl Pts',(-24.0549391608204,-13.4749049518927,
112.883779163764)) ;
#169912=CARTESIAN_POINT('Ctrl Pts',(-24.1287430036364,-13.4749049038309,
112.859548120238)) ;
#169913=CARTESIAN_POINT('Ctrl Pts',(-24.2025468464523,-13.474904855769,
112.835317076712)) ;
#169914=CARTESIAN_POINT('Ctrl Pts',(-24.178914419613,-13.4796298009885,
112.763336516709)) ;
#169915=CARTESIAN_POINT('Ctrl Pts',(-24.1552819927736,-13.4843547462079,
112.691355956706)) ;
#169916=CARTESIAN_POINT('Ctrl Pts',(-24.0814781499577,-13.4843547942698,
112.715587000231)) ;
#169917=CARTESIAN_POINT('Ctrl Pts',(-24.0076743071417,-13.4843548423316,
112.739818043757)) ;
#169918=CARTESIAN_POINT('Ctrl Pts',(-24.0313067339811,-13.4796298971122,
112.81179860376)) ;
#169919=CARTESIAN_POINT('Ctrl Pts',(-24.0487404996973,-13.1904267551927,
112.829580265168)) ;
#169920=CARTESIAN_POINT('Ctrl Pts',(-24.0719222496774,-13.2058873743104,
112.900188136033)) ;
#169921=CARTESIAN_POINT('Ctrl Pts',(-24.1457260959883,-13.2058873346672,
112.875957103152)) ;
#169922=CARTESIAN_POINT('Ctrl Pts',(-24.2195299422992,-13.205887295024,
112.851726070272)) ;
#169923=CARTESIAN_POINT('Ctrl Pts',(-24.1963481923192,-13.1904266759062,
112.781118199406)) ;
#169924=CARTESIAN_POINT('Ctrl Pts',(-24.1731664423392,-13.1749660567885,
112.710510328541)) ;
#169925=CARTESIAN_POINT('Ctrl Pts',(-24.0993625960283,-13.1749660964317,
112.734741361422)) ;
#169926=CARTESIAN_POINT('Ctrl Pts',(-24.0255587497174,-13.1749661360749,
112.758972394302)) ;
#169927=CARTESIAN_POINT('Ctrl Pts',(-24.0487404996973,-13.1904267551927,
112.829580265168)) ;
#169928=CARTESIAN_POINT('Ctrl Pts',(-24.0902477017721,-12.9149395489465,
112.920337621988)) ;
#169929=CARTESIAN_POINT('Ctrl Pts',(-24.1113047035226,-12.9496591977343,
112.98447385237)) ;
#169930=CARTESIAN_POINT('Ctrl Pts',(-24.1851085515239,-12.9496591712855,
112.960242824638)) ;
#169931=CARTESIAN_POINT('Ctrl Pts',(-24.2589123995253,-12.9496591448368,
112.936011796906)) ;
#169932=CARTESIAN_POINT('Ctrl Pts',(-24.2378553977748,-12.914939496049,
112.871875566525)) ;
#169933=CARTESIAN_POINT('Ctrl Pts',(-24.2167983960244,-12.8802198472613,
112.807739336143)) ;
#169934=CARTESIAN_POINT('Ctrl Pts',(-24.142994548023,-12.88021987371,112.831970363875)) ;
#169935=CARTESIAN_POINT('Ctrl Pts',(-24.0691907000217,-12.8802199001588,
112.856201391607)) ;
#169936=CARTESIAN_POINT('Ctrl Pts',(-24.0902477017721,-12.9149395489465,
112.920337621988)) ;
#169937=CARTESIAN_POINT('Ctrl Pts',(-24.1529087502765,-12.6780026906519,
113.075870610028)) ;
#169938=CARTESIAN_POINT('Ctrl Pts',(-24.1703532645626,-12.7293185102392,
113.129003786334)) ;
#169939=CARTESIAN_POINT('Ctrl Pts',(-24.2441571130729,-12.7293184935026,
113.104772760153)) ;
#169940=CARTESIAN_POINT('Ctrl Pts',(-24.3179609615833,-12.729318476766,
113.080541733971)) ;
#169941=CARTESIAN_POINT('Ctrl Pts',(-24.3005164472972,-12.6780026571787,
113.027408557665)) ;
#169942=CARTESIAN_POINT('Ctrl Pts',(-24.2830719330111,-12.6266868375913,
112.974275381359)) ;
#169943=CARTESIAN_POINT('Ctrl Pts',(-24.2092680845008,-12.6266868543279,
112.998506407541)) ;
#169944=CARTESIAN_POINT('Ctrl Pts',(-24.1354642359904,-12.6266868710645,
113.022737433722)) ;
#169945=CARTESIAN_POINT('Ctrl Pts',(-24.1529087502765,-12.6780026906519,
113.075870610028)) ;
#169946=CARTESIAN_POINT('Ctrl Pts',(-24.2335276358452,-12.492912372698,
113.285956395486)) ;
#169947=CARTESIAN_POINT('Ctrl Pts',(-24.2461033083903,-12.5572296336134,
113.324259865286)) ;
#169948=CARTESIAN_POINT('Ctrl Pts',(-24.3199071561044,-12.5572296258791,
113.300028836679)) ;
#169949=CARTESIAN_POINT('Ctrl Pts',(-24.3937110038185,-12.5572296181447,
113.275797808072)) ;
#169950=CARTESIAN_POINT('Ctrl Pts',(-24.3811353312734,-12.4929123572293,
113.237494338272)) ;
#169951=CARTESIAN_POINT('Ctrl Pts',(-24.3685596587283,-12.4285950963139,
113.199190868472)) ;
#169952=CARTESIAN_POINT('Ctrl Pts',(-24.2947558110142,-12.4285951040482,
113.223421897078)) ;
#169953=CARTESIAN_POINT('Ctrl Pts',(-24.2209519633001,-12.4285951117825,
113.247652925685)) ;
#169954=CARTESIAN_POINT('Ctrl Pts',(-24.2335276358452,-12.492912372698,
113.285956395486)) ;
#169955=CARTESIAN_POINT('Ctrl Pts',(-24.3270570352882,-12.3740385950698,
113.535339725245)) ;
#169956=CARTESIAN_POINT('Ctrl Pts',(-24.3338554351378,-12.446753464716,
113.55604655444)) ;
#169957=CARTESIAN_POINT('Ctrl Pts',(-24.4076592812388,-12.4467534627922,
113.53181552092)) ;
#169958=CARTESIAN_POINT('Ctrl Pts',(-24.4814631273398,-12.4467534608683,
113.5075844874)) ;
#169959=CARTESIAN_POINT('Ctrl Pts',(-24.4746647274902,-12.374038591222,
113.486877658205)) ;
#169960=CARTESIAN_POINT('Ctrl Pts',(-24.4678663276405,-12.3013237215758,
113.46617082901)) ;
#169961=CARTESIAN_POINT('Ctrl Pts',(-24.3940624815395,-12.3013237234996,
113.49040186253)) ;
#169962=CARTESIAN_POINT('Ctrl Pts',(-24.3202586354385,-12.3013237254235,
113.51463289605)) ;
#169963=CARTESIAN_POINT('Ctrl Pts',(-24.3270570352882,-12.3740385950698,
113.535339725245)) ;
#169964=CARTESIAN_POINT('Ctrl Pts',(-24.4275571229869,-12.3302346237977,
113.80591117555)) ;
#169965=CARTESIAN_POINT('Ctrl Pts',(-24.4280835159596,-12.406117742521,
113.807514483671)) ;
#169966=CARTESIAN_POINT('Ctrl Pts',(-24.5018873603174,-12.4061177428899,
113.783283444841)) ;
#169967=CARTESIAN_POINT('Ctrl Pts',(-24.5756912046753,-12.4061177432587,
113.759052406012)) ;
#169968=CARTESIAN_POINT('Ctrl Pts',(-24.5751648117025,-12.3302346245354,
113.757449097891)) ;
#169969=CARTESIAN_POINT('Ctrl Pts',(-24.5746384187298,-12.2543515058121,
113.755845789771)) ;
#169970=CARTESIAN_POINT('Ctrl Pts',(-24.5008345743719,-12.2543515054432,
113.7800768286)) ;
#169971=CARTESIAN_POINT('Ctrl Pts',(-24.4270307300141,-12.2543515050743,
113.80430786743)) ;
#169972=CARTESIAN_POINT('Ctrl Pts',(-24.4275571229869,-12.3302346237977,
113.80591117555)) ;
#169973=CARTESIAN_POINT('Ctrl Pts',(-24.5279557593141,-12.3639942142519,
114.076366355261)) ;
#169974=CARTESIAN_POINT('Ctrl Pts',(-24.5222038772141,-12.4376333996041,
114.058847050435)) ;
#169975=CARTESIAN_POINT('Ctrl Pts',(-24.5960077204063,-12.4376333997196,
114.034616008055)) ;
#169976=CARTESIAN_POINT('Ctrl Pts',(-24.6698115635986,-12.4376333998351,
114.010384965676)) ;
#169977=CARTESIAN_POINT('Ctrl Pts',(-24.6755634456986,-12.3639942144829,
114.027904270502)) ;
#169978=CARTESIAN_POINT('Ctrl Pts',(-24.6813153277986,-12.2903550291307,
114.045423575328)) ;
#169979=CARTESIAN_POINT('Ctrl Pts',(-24.6075114846064,-12.2903550290152,
114.069654617708)) ;
#169980=CARTESIAN_POINT('Ctrl Pts',(-24.5337076414141,-12.2903550288997,
114.093885660087)) ;
#169981=CARTESIAN_POINT('Ctrl Pts',(-24.5279557593141,-12.3639942142519,
114.076366355261)) ;
#169982=CARTESIAN_POINT('Ctrl Pts',(-24.6232350266706,-12.4744699305646,
114.330862780655)) ;
#169983=CARTESIAN_POINT('Ctrl Pts',(-24.6115600779504,-12.5405049323792,
114.295302770537)) ;
#169984=CARTESIAN_POINT('Ctrl Pts',(-24.6853639204602,-12.5405049308727,
114.271071726079)) ;
#169985=CARTESIAN_POINT('Ctrl Pts',(-24.7591677629699,-12.5405049293662,
114.24684068162)) ;
#169986=CARTESIAN_POINT('Ctrl Pts',(-24.7708427116901,-12.4744699275516,
114.282400691739)) ;
#169987=CARTESIAN_POINT('Ctrl Pts',(-24.7825176604102,-12.408434925737,
114.317960701857)) ;
#169988=CARTESIAN_POINT('Ctrl Pts',(-24.7087138179005,-12.4084349272435,
114.342191746315)) ;
#169989=CARTESIAN_POINT('Ctrl Pts',(-24.6349099753908,-12.40843492875,114.366422790774)) ;
#169990=CARTESIAN_POINT('Ctrl Pts',(-24.6232350266706,-12.4744699305646,
114.330862780655)) ;
#169991=CARTESIAN_POINT('Ctrl Pts',(-24.7051121876909,-12.6502203530517,
114.545089149363)) ;
#169992=CARTESIAN_POINT('Ctrl Pts',(-24.6884304701762,-12.7040802804882,
114.494279329336)) ;
#169993=CARTESIAN_POINT('Ctrl Pts',(-24.7622343128994,-12.7040802781189,
114.470048285528)) ;
#169994=CARTESIAN_POINT('Ctrl Pts',(-24.8360381556225,-12.7040802757496,
114.44581724172)) ;
#169995=CARTESIAN_POINT('Ctrl Pts',(-24.8527198731372,-12.6502203483131,
114.496627061747)) ;
#169996=CARTESIAN_POINT('Ctrl Pts',(-24.8694015906519,-12.5963604208767,
114.547436881774)) ;
#169997=CARTESIAN_POINT('Ctrl Pts',(-24.7955977479287,-12.596360423246,
114.571667925582)) ;
#169998=CARTESIAN_POINT('Ctrl Pts',(-24.7217939052056,-12.5963604256153,
114.59589896939)) ;
#169999=CARTESIAN_POINT('Ctrl Pts',(-24.7051121876909,-12.6502203530517,
114.545089149363)) ;
#170000=CARTESIAN_POINT('Ctrl Pts',(-24.7708093325559,-12.8831101738135,
114.709574205269)) ;
#170001=CARTESIAN_POINT('Ctrl Pts',(-24.7502524566444,-12.9207872316337,
114.64696127806)) ;
#170002=CARTESIAN_POINT('Ctrl Pts',(-24.8240562999475,-12.9207872305233,
114.622730236018)) ;
#170003=CARTESIAN_POINT('Ctrl Pts',(-24.8978601432505,-12.9207872294128,
114.598499193976)) ;
#170004=CARTESIAN_POINT('Ctrl Pts',(-24.9184170191621,-12.8831101715926,
114.661112121185)) ;
#170005=CARTESIAN_POINT('Ctrl Pts',(-24.9389738950736,-12.8454331137723,
114.723725048394)) ;
#170006=CARTESIAN_POINT('Ctrl Pts',(-24.8651700517706,-12.8454331148828,
114.747956090436)) ;
#170007=CARTESIAN_POINT('Ctrl Pts',(-24.7913662084675,-12.8454331159932,
114.772187132478)) ;
#170008=CARTESIAN_POINT('Ctrl Pts',(-24.7708093325559,-12.8831101738135,
114.709574205269)) ;
#170009=CARTESIAN_POINT('Ctrl Pts',(-24.8149023489856,-13.1530763913863,
114.808480864834)) ;
#170010=CARTESIAN_POINT('Ctrl Pts',(-24.7919690280488,-13.1719578711027,
114.738629669587)) ;
#170011=CARTESIAN_POINT('Ctrl Pts',(-24.865772871781,-13.1719578734333,
114.714398628852)) ;
#170012=CARTESIAN_POINT('Ctrl Pts',(-24.9395767155132,-13.1719578757638,
114.690167588117)) ;
#170013=CARTESIAN_POINT('Ctrl Pts',(-24.96251003645,-13.1530763960474,114.760018783364)) ;
#170014=CARTESIAN_POINT('Ctrl Pts',(-24.9854433573868,-13.134194916331,
114.829869978612)) ;
#170015=CARTESIAN_POINT('Ctrl Pts',(-24.9116395136546,-13.1341949140004,
114.854101019347)) ;
#170016=CARTESIAN_POINT('Ctrl Pts',(-24.8378356699223,-13.1341949116699,
114.878332060081)) ;
#170017=CARTESIAN_POINT('Ctrl Pts',(-24.8149023489856,-13.1530763913863,
114.808480864834)) ;
#170018=CARTESIAN_POINT('Ctrl Pts',(-24.8355728558331,-13.4431032907692,
114.835890910938)) ;
#170019=CARTESIAN_POINT('Ctrl Pts',(-24.8118983223279,-13.4417610754161,
114.763782101914)) ;
#170020=CARTESIAN_POINT('Ctrl Pts',(-24.8857021658435,-13.4417610837383,
114.73955106052)) ;
#170021=CARTESIAN_POINT('Ctrl Pts',(-24.9595060093591,-13.4417610920606,
114.715320019125)) ;
#170022=CARTESIAN_POINT('Ctrl Pts',(-24.9831805428643,-13.4431033074138,
114.787428828149)) ;
#170023=CARTESIAN_POINT('Ctrl Pts',(-25.0068550763695,-13.4444455227669,
114.859537637173)) ;
#170024=CARTESIAN_POINT('Ctrl Pts',(-24.9330512328539,-13.4444455144446,
114.883768678568)) ;
#170025=CARTESIAN_POINT('Ctrl Pts',(-24.8592473893383,-13.4444455061224,
114.907999719962)) ;
#170026=CARTESIAN_POINT('Ctrl Pts',(-24.8355728558331,-13.4431032907692,
114.835890910938)) ;
#170027=CARTESIAN_POINT('Ctrl Pts',(-24.8318678122467,-13.7301505723016,
114.789212778357)) ;
#170028=CARTESIAN_POINT('Ctrl Pts',(-24.8091500394405,-13.7087638139034,
114.720018108166)) ;
#170029=CARTESIAN_POINT('Ctrl Pts',(-24.8829538817403,-13.7087638278677,
114.695787063069)) ;
#170030=CARTESIAN_POINT('Ctrl Pts',(-24.9567577240401,-13.7087638418319,
114.671556017971)) ;
#170031=CARTESIAN_POINT('Ctrl Pts',(-24.9794754968464,-13.7301506002301,
114.740750688162)) ;
#170032=CARTESIAN_POINT('Ctrl Pts',(-25.0021932696526,-13.7515373586284,
114.809945358352)) ;
#170033=CARTESIAN_POINT('Ctrl Pts',(-24.9283894273528,-13.7515373446641,
114.83417640345)) ;
#170034=CARTESIAN_POINT('Ctrl Pts',(-24.854585585053,-13.7515373306999,
114.858407448548)) ;
#170035=CARTESIAN_POINT('Ctrl Pts',(-24.8318678122467,-13.7301505723016,
114.789212778357)) ;
#170036=CARTESIAN_POINT('Ctrl Pts',(-24.8049151957928,-13.9953629945928,
114.671655667574)) ;
#170037=CARTESIAN_POINT('Ctrl Pts',(-24.7847802406744,-13.9554274129798,
114.610327843468)) ;
#170038=CARTESIAN_POINT('Ctrl Pts',(-24.8585840806476,-13.9554274317702,
114.586096791283)) ;
#170039=CARTESIAN_POINT('Ctrl Pts',(-24.9323879206208,-13.9554274505607,
114.561865739099)) ;
#170040=CARTESIAN_POINT('Ctrl Pts',(-24.9525228757392,-13.9953630321736,
114.623193563205)) ;
#170041=CARTESIAN_POINT('Ctrl Pts',(-24.9726578308576,-14.0352986137866,
114.684521387312)) ;
#170042=CARTESIAN_POINT('Ctrl Pts',(-24.8988539908844,-14.0352985949962,
114.708752439496)) ;
#170043=CARTESIAN_POINT('Ctrl Pts',(-24.8250501509112,-14.0352985762058,
114.732983491681)) ;
#170044=CARTESIAN_POINT('Ctrl Pts',(-24.8049151957928,-13.9953629945928,
114.671655667574)) ;
#170045=CARTESIAN_POINT('Ctrl Pts',(-24.7574454109872,-14.2191243988368,
114.491650052615)) ;
#170046=CARTESIAN_POINT('Ctrl Pts',(-24.7413286926604,-14.1635077763497,
114.442561129583)) ;
#170047=CARTESIAN_POINT('Ctrl Pts',(-24.8151325294779,-14.1635077969098,
114.418330067787)) ;
#170048=CARTESIAN_POINT('Ctrl Pts',(-24.8889363662954,-14.16350781747,114.394099005991)) ;
#170049=CARTESIAN_POINT('Ctrl Pts',(-24.9050530846223,-14.2191244399571,
114.443187929023)) ;
#170050=CARTESIAN_POINT('Ctrl Pts',(-24.9211698029491,-14.2747410624442,
114.492276852054)) ;
#170051=CARTESIAN_POINT('Ctrl Pts',(-24.8473659661316,-14.2747410418841,
114.51650791385)) ;
#170052=CARTESIAN_POINT('Ctrl Pts',(-24.7735621293141,-14.2747410213239,
114.540738975646)) ;
#170053=CARTESIAN_POINT('Ctrl Pts',(-24.7574454109872,-14.2191243988368,
114.491650052615)) ;
#170054=CARTESIAN_POINT('Ctrl Pts',(-24.6930620100319,-14.3863702551061,
114.259889607909)) ;
#170055=CARTESIAN_POINT('Ctrl Pts',(-24.6821550649487,-14.318995498507,
114.226668813785)) ;
#170056=CARTESIAN_POINT('Ctrl Pts',(-24.7559588974035,-14.3189955173641,
114.202437738701)) ;
#170057=CARTESIAN_POINT('Ctrl Pts',(-24.8297627298584,-14.3189955362211,
114.178206663618)) ;
#170058=CARTESIAN_POINT('Ctrl Pts',(-24.8406696749416,-14.3863702928201,
114.211427457741)) ;
#170059=CARTESIAN_POINT('Ctrl Pts',(-24.8515766200249,-14.4537450494192,
114.244648251865)) ;
#170060=CARTESIAN_POINT('Ctrl Pts',(-24.77777278757,-14.4537450305621,114.268879326949)) ;
#170061=CARTESIAN_POINT('Ctrl Pts',(-24.7039689551151,-14.4537450117051,
114.293110402033)) ;
#170062=CARTESIAN_POINT('Ctrl Pts',(-24.6930620100319,-14.3863702551061,
114.259889607909)) ;
#170063=CARTESIAN_POINT('Ctrl Pts',(-24.6182341661136,-14.4829184358348,
113.996662475295)) ;
#170064=CARTESIAN_POINT('Ctrl Pts',(-24.6132666839143,-14.408705819493,
113.981532326927)) ;
#170065=CARTESIAN_POINT('Ctrl Pts',(-24.6870705129792,-14.4087058298003,
113.957301241518)) ;
#170066=CARTESIAN_POINT('Ctrl Pts',(-24.7608743420441,-14.4087058401076,
113.933070156109)) ;
#170067=CARTESIAN_POINT('Ctrl Pts',(-24.7658418242435,-14.4829184564494,
113.948200304477)) ;
#170068=CARTESIAN_POINT('Ctrl Pts',(-24.7708093064428,-14.5571310727912,
113.963330452846)) ;
#170069=CARTESIAN_POINT('Ctrl Pts',(-24.6970054773779,-14.5571310624839,
113.987561538255)) ;
#170070=CARTESIAN_POINT('Ctrl Pts',(-24.623201648313,-14.5571310521766,
114.011792623664)) ;
#170071=CARTESIAN_POINT('Ctrl Pts',(-24.6182341661136,-14.4829184358348,
113.996662475295)) ;
#170072=CARTESIAN_POINT('Ctrl Pts',(-24.5380341001339,-14.5038609743369,
113.716865195632)) ;
#170073=CARTESIAN_POINT('Ctrl Pts',(-24.5393939069206,-14.4280787626501,
113.721006948789)) ;
#170074=CARTESIAN_POINT('Ctrl Pts',(-24.613197732782,-14.4280787598768,
113.696775853622)) ;
#170075=CARTESIAN_POINT('Ctrl Pts',(-24.6870015586434,-14.4280787571034,
113.672544758456)) ;
#170076=CARTESIAN_POINT('Ctrl Pts',(-24.6856417518568,-14.5038609687901,
113.668403005299)) ;
#170077=CARTESIAN_POINT('Ctrl Pts',(-24.6842819450701,-14.5796431804768,
113.664261252142)) ;
#170078=CARTESIAN_POINT('Ctrl Pts',(-24.6104781192086,-14.5796431832502,
113.688492347308)) ;
#170079=CARTESIAN_POINT('Ctrl Pts',(-24.5366742933472,-14.5796431860236,
113.712723442475)) ;
#170080=CARTESIAN_POINT('Ctrl Pts',(-24.5380341001339,-14.5038609743369,
113.716865195632)) ;
#170081=CARTESIAN_POINT('Ctrl Pts',(-24.4595898163493,-14.4469649885374,
113.442529411797)) ;
#170082=CARTESIAN_POINT('Ctrl Pts',(-24.4671610719166,-14.3750457551338,
113.465590235879)) ;
#170083=CARTESIAN_POINT('Ctrl Pts',(-24.5409648962975,-14.3750457349022,
113.441359136204)) ;
#170084=CARTESIAN_POINT('Ctrl Pts',(-24.6147687206784,-14.3750457146707,
113.417128036528)) ;
#170085=CARTESIAN_POINT('Ctrl Pts',(-24.6071974651112,-14.4469649480743,
113.394067212446)) ;
#170086=CARTESIAN_POINT('Ctrl Pts',(-24.5996262095439,-14.5188841814779,
113.371006388363)) ;
#170087=CARTESIAN_POINT('Ctrl Pts',(-24.525822385163,-14.5188842017095,
113.395237488039)) ;
#170088=CARTESIAN_POINT('Ctrl Pts',(-24.452018560782,-14.518884221941,113.419468587715)) ;
#170089=CARTESIAN_POINT('Ctrl Pts',(-24.4595898163493,-14.4469649885374,
113.442529411797)) ;
#170090=CARTESIAN_POINT('Ctrl Pts',(-24.3888589686452,-14.3162777489947,
113.191599288438)) ;
#170091=CARTESIAN_POINT('Ctrl Pts',(-24.4021139128791,-14.2533785894399,
113.231971711301)) ;
#170092=CARTESIAN_POINT('Ctrl Pts',(-24.4759177374634,-14.2533785490254,
113.207740612244)) ;
#170093=CARTESIAN_POINT('Ctrl Pts',(-24.5497215620477,-14.253378508611,
113.183509513188)) ;
#170094=CARTESIAN_POINT('Ctrl Pts',(-24.5364666178138,-14.3162776681657,
113.143137090325)) ;
#170095=CARTESIAN_POINT('Ctrl Pts',(-24.5232116735799,-14.3791768277205,
113.102764667462)) ;
#170096=CARTESIAN_POINT('Ctrl Pts',(-24.4494078489956,-14.379176868135,
113.126995766519)) ;
#170097=CARTESIAN_POINT('Ctrl Pts',(-24.3756040244114,-14.3791769085495,
113.151226865575)) ;
#170098=CARTESIAN_POINT('Ctrl Pts',(-24.3888589686452,-14.3162777489947,
113.191599288438)) ;
#170099=CARTESIAN_POINT('Ctrl Pts',(-24.3319214311833,-14.1213118802641,
112.982718459293)) ;
#170100=CARTESIAN_POINT('Ctrl Pts',(-24.3499044990959,-14.0719335115926,
113.037491984146)) ;
#170101=CARTESIAN_POINT('Ctrl Pts',(-24.4237083262045,-14.0719334508548,
113.013260892779)) ;
#170102=CARTESIAN_POINT('Ctrl Pts',(-24.4975121533131,-14.0719333901169,
112.989029801411)) ;
#170103=CARTESIAN_POINT('Ctrl Pts',(-24.4795290854005,-14.1213117587884,
112.934256276558)) ;
#170104=CARTESIAN_POINT('Ctrl Pts',(-24.4615460174878,-14.1706901274599,
112.879482751705)) ;
#170105=CARTESIAN_POINT('Ctrl Pts',(-24.3877421903792,-14.1706901881977,
112.903713843072)) ;
#170106=CARTESIAN_POINT('Ctrl Pts',(-24.3139383632706,-14.1706902489356,
112.92794493444)) ;
#170107=CARTESIAN_POINT('Ctrl Pts',(-24.3319214311833,-14.1213118802641,
112.982718459293)) ;
#170108=CARTESIAN_POINT('Ctrl Pts',(-24.2934703508109,-13.8756723338256,
112.83009751122)) ;
#170109=CARTESIAN_POINT('Ctrl Pts',(-24.3148987517297,-13.8433718742573,
112.895364964646)) ;
#170110=CARTESIAN_POINT('Ctrl Pts',(-24.3887025835186,-13.8433717952861,
112.871133887534)) ;
#170111=CARTESIAN_POINT('Ctrl Pts',(-24.4625064153074,-13.8433717163149,
112.846902810421)) ;
#170112=CARTESIAN_POINT('Ctrl Pts',(-24.4410780143885,-13.8756721758832,
112.781635356995)) ;
#170113=CARTESIAN_POINT('Ctrl Pts',(-24.4196496134697,-13.9079726354515,
112.716367903568)) ;
#170114=CARTESIAN_POINT('Ctrl Pts',(-24.3458457816808,-13.9079727144228,
112.740598980681)) ;
#170115=CARTESIAN_POINT('Ctrl Pts',(-24.272041949892,-13.907972793394,112.764830057793)) ;
#170116=CARTESIAN_POINT('Ctrl Pts',(-24.2934703508109,-13.8756723338256,
112.83009751122)) ;
#170117=CARTESIAN_POINT('Ctrl Pts',(-24.2771743617304,-13.597140902686,
112.744958189465)) ;
#170118=CARTESIAN_POINT('Ctrl Pts',(-24.3005063726652,-13.584239435371,
112.816023731974)) ;
#170119=CARTESIAN_POINT('Ctrl Pts',(-24.3743102111448,-13.5842393431877,
112.791792675241)) ;
#170120=CARTESIAN_POINT('Ctrl Pts',(-24.4481140496243,-13.5842392510044,
112.767561618507)) ;
#170121=CARTESIAN_POINT('Ctrl Pts',(-24.4247820386894,-13.5971407183194,
112.696496075998)) ;
#170122=CARTESIAN_POINT('Ctrl Pts',(-24.4014500277545,-13.6100421856345,
112.625430533489)) ;
#170123=CARTESIAN_POINT('Ctrl Pts',(-24.327646189275,-13.6100422778178,
112.649661590222)) ;
#170124=CARTESIAN_POINT('Ctrl Pts',(-24.2538423507955,-13.6100423700011,
112.673892646956)) ;
#170125=CARTESIAN_POINT('Ctrl Pts',(-24.2771743617304,-13.597140902686,
112.744958189465)) ;
#170126=CARTESIAN_POINT('Ctrl Pts',(-24.2847732062642,-13.3072582096283,
112.732779234924)) ;
#170127=CARTESIAN_POINT('Ctrl Pts',(-24.3083395158188,-13.3145766205793,
112.804558413309)) ;
#170128=CARTESIAN_POINT('Ctrl Pts',(-24.3821433622311,-13.3145765231922,
112.780327380737)) ;
#170129=CARTESIAN_POINT('Ctrl Pts',(-24.4559472086434,-13.3145764258051,
112.756096348166)) ;
#170130=CARTESIAN_POINT('Ctrl Pts',(-24.4323808990888,-13.3072580148542,
112.684317169781)) ;
#170131=CARTESIAN_POINT('Ctrl Pts',(-24.4088145895342,-13.2999396039032,
112.612537991397)) ;
#170132=CARTESIAN_POINT('Ctrl Pts',(-24.335010743122,-13.2999397012903,
112.636769023968)) ;
#170133=CARTESIAN_POINT('Ctrl Pts',(-24.2612068967096,-13.2999397986774,
112.66100005654)) ;
#170134=CARTESIAN_POINT('Ctrl Pts',(-24.2847732062642,-13.3072582096283,
112.732779234924)) ;
#170135=CARTESIAN_POINT('Ctrl Pts',(-24.3165545058404,-13.023884652308,
112.794080029736)) ;
#170136=CARTESIAN_POINT('Ctrl Pts',(-24.3386710351731,-13.0509977629016,
112.861443411571)) ;
#170137=CARTESIAN_POINT('Ctrl Pts',(-24.412474890052,-13.0509976674412,
112.837212404788)) ;
#170138=CARTESIAN_POINT('Ctrl Pts',(-24.486278744931,-13.0509975719808,
112.812981398004)) ;
#170139=CARTESIAN_POINT('Ctrl Pts',(-24.4641622155983,-13.0238844613873,
112.745618016169)) ;
#170140=CARTESIAN_POINT('Ctrl Pts',(-24.4420456862657,-12.9967713507938,
112.678254634333)) ;
#170141=CARTESIAN_POINT('Ctrl Pts',(-24.3682418313867,-12.9967714462542,
112.702485641117)) ;
#170142=CARTESIAN_POINT('Ctrl Pts',(-24.2944379765078,-12.9967715417145,
112.7267166479)) ;
#170143=CARTESIAN_POINT('Ctrl Pts',(-24.3165545058404,-13.023884652308,
112.794080029736)) ;
#170144=CARTESIAN_POINT('Ctrl Pts',(-24.3710194266415,-12.7690113233817,
112.924503192536)) ;
#170145=CARTESIAN_POINT('Ctrl Pts',(-24.3900997882587,-12.8139584952445,
112.982618897456)) ;
#170146=CARTESIAN_POINT('Ctrl Pts',(-24.4639036512443,-12.813958410504,
112.958387915364)) ;
#170147=CARTESIAN_POINT('Ctrl Pts',(-24.5377075142299,-12.8139583257634,
112.934156933272)) ;
#170148=CARTESIAN_POINT('Ctrl Pts',(-24.5186271526127,-12.7690111539007,
112.876041228353)) ;
#170149=CARTESIAN_POINT('Ctrl Pts',(-24.4995467909954,-12.7240639820379,
112.817925523433)) ;
#170150=CARTESIAN_POINT('Ctrl Pts',(-24.4257429280098,-12.7240640667784,
112.842156505525)) ;
#170151=CARTESIAN_POINT('Ctrl Pts',(-24.3519390650242,-12.724064151519,
112.866387487617)) ;
#170152=CARTESIAN_POINT('Ctrl Pts',(-24.3710194266415,-12.7690113233817,
112.924503192536)) ;
#170153=CARTESIAN_POINT('Ctrl Pts',(-24.4450008074729,-12.5606194771078,
113.114364621987)) ;
#170154=CARTESIAN_POINT('Ctrl Pts',(-24.4596781905624,-12.6201819472302,
113.159069564768)) ;
#170155=CARTESIAN_POINT('Ctrl Pts',(-24.533482060381,-12.6201818809856,
113.134838603488)) ;
#170156=CARTESIAN_POINT('Ctrl Pts',(-24.6072859301996,-12.620181814741,
113.110607642208)) ;
#170157=CARTESIAN_POINT('Ctrl Pts',(-24.5926085471101,-12.5606193446187,
113.065902699427)) ;
#170158=CARTESIAN_POINT('Ctrl Pts',(-24.5779311640206,-12.5010568744963,
113.021197756646)) ;
#170159=CARTESIAN_POINT('Ctrl Pts',(-24.504127294202,-12.5010569407409,
113.045428717926)) ;
#170160=CARTESIAN_POINT('Ctrl Pts',(-24.4303234243834,-12.5010570069855,
113.069659679205)) ;
#170161=CARTESIAN_POINT('Ctrl Pts',(-24.4450008074729,-12.5606194771078,
113.114364621987)) ;
#170162=CARTESIAN_POINT('Ctrl Pts',(-24.5338650383482,-12.413760463827,
113.349590588029)) ;
#170163=CARTESIAN_POINT('Ctrl Pts',(-24.5430932310349,-12.4836640016496,
113.377698176085)) ;
#170164=CARTESIAN_POINT('Ctrl Pts',(-24.6168971056564,-12.4836639599655,
113.353467229434)) ;
#170165=CARTESIAN_POINT('Ctrl Pts',(-24.690700980278,-12.4836639182814,
113.329236282783)) ;
#170166=CARTESIAN_POINT('Ctrl Pts',(-24.6814727875913,-12.4137603804588,
113.301128694728)) ;
#170167=CARTESIAN_POINT('Ctrl Pts',(-24.6722445949046,-12.3438568426362,
113.273021106673)) ;
#170168=CARTESIAN_POINT('Ctrl Pts',(-24.5984407202831,-12.3438568843203,
113.297252053324)) ;
#170169=CARTESIAN_POINT('Ctrl Pts',(-24.5246368456615,-12.3438569260044,
113.321482999974)) ;
#170170=CARTESIAN_POINT('Ctrl Pts',(-24.5338650383482,-12.413760463827,
113.349590588029)) ;
#170171=CARTESIAN_POINT('Ctrl Pts',(-24.6321826857904,-12.3386970972896,
113.613568979409)) ;
#170172=CARTESIAN_POINT('Ctrl Pts',(-24.6352945524771,-12.4139449164538,
113.623047225329)) ;
#170173=CARTESIAN_POINT('Ctrl Pts',(-24.7090984293634,-12.4139449029389,
113.598816285577)) ;
#170174=CARTESIAN_POINT('Ctrl Pts',(-24.7829023062498,-12.4139448894239,
113.574585345824)) ;
#170175=CARTESIAN_POINT('Ctrl Pts',(-24.7797904395631,-12.3386970702597,
113.565107099904)) ;
#170176=CARTESIAN_POINT('Ctrl Pts',(-24.7766785728765,-12.2634492510955,
113.555628853984)) ;
#170177=CARTESIAN_POINT('Ctrl Pts',(-24.7028746959902,-12.2634492646105,
113.579859793736)) ;
#170178=CARTESIAN_POINT('Ctrl Pts',(-24.6290708191038,-12.2634492781254,
113.604090733489)) ;
#170179=CARTESIAN_POINT('Ctrl Pts',(-24.6321826857904,-12.3386970972896,
113.613568979409)) ;
#170180=CARTESIAN_POINT('Ctrl Pts',(-24.7334826748307,-12.3409867725706,
113.886661565323)) ;
#170181=CARTESIAN_POINT('Ctrl Pts',(-24.730260281677,-12.4161865646984,
113.876846677773)) ;
#170182=CARTESIAN_POINT('Ctrl Pts',(-24.8040641580606,-12.4161865800311,
113.852615736489)) ;
#170183=CARTESIAN_POINT('Ctrl Pts',(-24.8778680344442,-12.4161865953639,
113.828384795205)) ;
#170184=CARTESIAN_POINT('Ctrl Pts',(-24.8810904275978,-12.3409868032361,
113.838199682755)) ;
#170185=CARTESIAN_POINT('Ctrl Pts',(-24.8843128207515,-12.2657870111083,
113.848014570306)) ;
#170186=CARTESIAN_POINT('Ctrl Pts',(-24.8105089443679,-12.2657869957756,
113.87224551159)) ;
#170187=CARTESIAN_POINT('Ctrl Pts',(-24.7367050679843,-12.2657869804429,
113.896476452874)) ;
#170188=CARTESIAN_POINT('Ctrl Pts',(-24.7334826748307,-12.3409867725706,
113.886661565323)) ;
#170189=CARTESIAN_POINT('Ctrl Pts',(-24.8314366572385,-12.4204578395528,
114.149527864238)) ;
#170190=CARTESIAN_POINT('Ctrl Pts',(-24.8221048881669,-12.4902214392955,
114.121104803336)) ;
#170191=CARTESIAN_POINT('Ctrl Pts',(-24.8959087613574,-12.4902214812087,
114.096873852327)) ;
#170192=CARTESIAN_POINT('Ctrl Pts',(-24.9697126345479,-12.4902215231219,
114.072642901317)) ;
#170193=CARTESIAN_POINT('Ctrl Pts',(-24.9790444036195,-12.4204579233792,
114.101065962219)) ;
#170194=CARTESIAN_POINT('Ctrl Pts',(-24.9883761726911,-12.3506943236366,
114.129489023121)) ;
#170195=CARTESIAN_POINT('Ctrl Pts',(-24.9145722995006,-12.3506942817234,
114.15371997413)) ;
#170196=CARTESIAN_POINT('Ctrl Pts',(-24.8407684263101,-12.3506942398102,
114.17795092514)) ;
#170197=CARTESIAN_POINT('Ctrl Pts',(-24.8314366572385,-12.4204578395528,
114.149527864238)) ;
#170198=CARTESIAN_POINT('Ctrl Pts',(-24.9196367729375,-12.5714299256093,
114.382700587259)) ;
#170199=CARTESIAN_POINT('Ctrl Pts',(-24.9048671068876,-12.6307574701192,
114.337714569493)) ;
#170200=CARTESIAN_POINT('Ctrl Pts',(-24.9786709746415,-12.6307575336333,
114.313483601925)) ;
#170201=CARTESIAN_POINT('Ctrl Pts',(-25.0524748423954,-12.6307575971475,
114.289252634356)) ;
#170202=CARTESIAN_POINT('Ctrl Pts',(-25.0672445084453,-12.5714300526376,
114.334238652123)) ;
#170203=CARTESIAN_POINT('Ctrl Pts',(-25.0820141744952,-12.5121025081277,
114.379224669889)) ;
#170204=CARTESIAN_POINT('Ctrl Pts',(-25.0082103067413,-12.5121024446135,
114.403455637457)) ;
#170205=CARTESIAN_POINT('Ctrl Pts',(-24.9344064389874,-12.5121023810993,
114.427686605026)) ;
#170206=CARTESIAN_POINT('Ctrl Pts',(-24.9196367729375,-12.5714299256093,
114.382700587259)) ;
#170207=CARTESIAN_POINT('Ctrl Pts',(-24.9924945178044,-12.7828129113163,
114.56917762335)) ;
#170208=CARTESIAN_POINT('Ctrl Pts',(-24.9733491898405,-12.8274711161602,
114.510864045317)) ;
#170209=CARTESIAN_POINT('Ctrl Pts',(-25.0471530506454,-12.82747119449,114.486633056583)) ;
#170210=CARTESIAN_POINT('Ctrl Pts',(-25.1209569114504,-12.8274712728199,
114.46240206785)) ;
#170211=CARTESIAN_POINT('Ctrl Pts',(-25.1401022394143,-12.782813067976,
114.520715645882)) ;
#170212=CARTESIAN_POINT('Ctrl Pts',(-25.1592475673782,-12.7381548631321,
114.579029223915)) ;
#170213=CARTESIAN_POINT('Ctrl Pts',(-25.0854437065732,-12.7381547848022,
114.603260212648)) ;
#170214=CARTESIAN_POINT('Ctrl Pts',(-25.0116398457683,-12.7381547064724,
114.627491201382)) ;
#170215=CARTESIAN_POINT('Ctrl Pts',(-24.9924945178044,-12.7828129113163,
114.56917762335)) ;
#170216=CARTESIAN_POINT('Ctrl Pts',(-25.0456977654746,-13.0396896566704,
114.695776913012)) ;
#170217=CARTESIAN_POINT('Ctrl Pts',(-25.023542631379,-13.0664804040034,
114.628295951028)) ;
#170218=CARTESIAN_POINT('Ctrl Pts',(-25.0973464844517,-13.0664804892966,
114.604064938743)) ;
#170219=CARTESIAN_POINT('Ctrl Pts',(-25.1711503375243,-13.0664805745898,
114.579833926458)) ;
#170220=CARTESIAN_POINT('Ctrl Pts',(-25.1933054716199,-13.0396898272568,
114.647314888442)) ;
#170221=CARTESIAN_POINT('Ctrl Pts',(-25.2154606057155,-13.0128990799238,
114.714795850425)) ;
#170222=CARTESIAN_POINT('Ctrl Pts',(-25.1416567526428,-13.0128989946306,
114.739026862711)) ;
#170223=CARTESIAN_POINT('Ctrl Pts',(-25.0678528995702,-13.0128989093375,
114.763257874996)) ;
#170224=CARTESIAN_POINT('Ctrl Pts',(-25.0456977654746,-13.0396896566704,
114.695776913012)) ;
#170225=CARTESIAN_POINT('Ctrl Pts',(-25.0761544983611,-13.3246405733811,
114.752976375053)) ;
#170226=CARTESIAN_POINT('Ctrl Pts',(-25.0525753762368,-13.3315770270648,
114.681158175154)) ;
#170227=CARTESIAN_POINT('Ctrl Pts',(-25.1263792216785,-13.331577110356,
114.656927139626)) ;
#170228=CARTESIAN_POINT('Ctrl Pts',(-25.2001830671202,-13.3315771936471,
114.632696104099)) ;
#170229=CARTESIAN_POINT('Ctrl Pts',(-25.2237621892446,-13.3246407399634,
114.704514303997)) ;
#170230=CARTESIAN_POINT('Ctrl Pts',(-25.2473413113689,-13.3177042862798,
114.776332503896)) ;
#170231=CARTESIAN_POINT('Ctrl Pts',(-25.1735374659272,-13.3177042029886,
114.800563539424)) ;
#170232=CARTESIAN_POINT('Ctrl Pts',(-25.0997336204854,-13.3177041196975,
114.824794574952)) ;
#170233=CARTESIAN_POINT('Ctrl Pts',(-25.0761544983611,-13.3246405733811,
114.752976375053)) ;
#170234=CARTESIAN_POINT('Ctrl Pts',(-25.0822716580922,-13.6149949699245,
114.736205333748)) ;
#170235=CARTESIAN_POINT('Ctrl Pts',(-25.0589624399057,-13.6016695488901,
114.665209217564)) ;
#170236=CARTESIAN_POINT('Ctrl Pts',(-25.1327662787753,-13.6016696242958,
114.640978162019)) ;
#170237=CARTESIAN_POINT('Ctrl Pts',(-25.2065701176448,-13.6016696997014,
114.616747106473)) ;
#170238=CARTESIAN_POINT('Ctrl Pts',(-25.2298793358313,-13.6149951207358,
114.687743222656)) ;
#170239=CARTESIAN_POINT('Ctrl Pts',(-25.2531885540178,-13.6283205417703,
114.758739338839)) ;
#170240=CARTESIAN_POINT('Ctrl Pts',(-25.1793847151483,-13.6283204663646,
114.782970394385)) ;
#170241=CARTESIAN_POINT('Ctrl Pts',(-25.1055808762787,-13.6283203909589,
114.807201449931)) ;
#170242=CARTESIAN_POINT('Ctrl Pts',(-25.0822716580922,-13.6149949699245,
114.736205333748)) ;
#170243=CARTESIAN_POINT('Ctrl Pts',(-25.06454635551,-13.8916396903177,114.646761857288)) ;
#170244=CARTESIAN_POINT('Ctrl Pts',(-25.043173102537,-13.8589788645426,
114.58166237863)) ;
#170245=CARTESIAN_POINT('Ctrl Pts',(-25.1169769363613,-13.8589789264578,
114.557431307717)) ;
#170246=CARTESIAN_POINT('Ctrl Pts',(-25.1907807701857,-13.858978988373,
114.533200236805)) ;
#170247=CARTESIAN_POINT('Ctrl Pts',(-25.2121540231587,-13.891639814148,
114.598299715463)) ;
#170248=CARTESIAN_POINT('Ctrl Pts',(-25.2335272761317,-13.9243006399231,
114.663399194122)) ;
#170249=CARTESIAN_POINT('Ctrl Pts',(-25.1597234423074,-13.9243005780079,
114.687630265035)) ;
#170250=CARTESIAN_POINT('Ctrl Pts',(-25.085919608483,-13.9243005160927,
114.711861335947)) ;
#170251=CARTESIAN_POINT('Ctrl Pts',(-25.06454635551,-13.8916396903177,114.646761857288)) ;
#170252=CARTESIAN_POINT('Ctrl Pts',(-25.0249777077505,-14.1343825887975,
114.490801908801)) ;
#170253=CARTESIAN_POINT('Ctrl Pts',(-25.0070681267458,-14.0847239411806,
114.436252215942)) ;
#170254=CARTESIAN_POINT('Ctrl Pts',(-25.0808719574157,-14.0847239865753,
114.412021135421)) ;
#170255=CARTESIAN_POINT('Ctrl Pts',(-25.1546757880855,-14.0847240319701,
114.387790054901)) ;
#170256=CARTESIAN_POINT('Ctrl Pts',(-25.1725853690902,-14.134382679587,
114.44233974776)) ;
#170257=CARTESIAN_POINT('Ctrl Pts',(-25.1904949500949,-14.1840413272039,
114.49688944062)) ;
#170258=CARTESIAN_POINT('Ctrl Pts',(-25.116691119425,-14.1840412818091,
114.521120521141)) ;
#170259=CARTESIAN_POINT('Ctrl Pts',(-25.0428872887551,-14.1840412364144,
114.545351601661)) ;
#170260=CARTESIAN_POINT('Ctrl Pts',(-25.0249777077505,-14.1343825887975,
114.490801908801)) ;
#170261=CARTESIAN_POINT('Ctrl Pts',(-24.9668445289914,-14.3263844089833,
114.278154012734)) ;
#170262=CARTESIAN_POINT('Ctrl Pts',(-24.9537029589574,-14.2632443878997,
114.238126911786)) ;
#170263=CARTESIAN_POINT('Ctrl Pts',(-25.0275067888665,-14.263244415508,
114.213895828948)) ;
#170264=CARTESIAN_POINT('Ctrl Pts',(-25.1013106187757,-14.2632444431164,
114.189664746111)) ;
#170265=CARTESIAN_POINT('Ctrl Pts',(-25.1144521888096,-14.3263844642,114.229691847058)) ;
#170266=CARTESIAN_POINT('Ctrl Pts',(-25.1275937588436,-14.3895244852836,
114.269718948005)) ;
#170267=CARTESIAN_POINT('Ctrl Pts',(-25.0537899289344,-14.3895244576753,
114.293950030843)) ;
#170268=CARTESIAN_POINT('Ctrl Pts',(-24.9799860990254,-14.3895244300669,
114.318181113681)) ;
#170269=CARTESIAN_POINT('Ctrl Pts',(-24.9668445289914,-14.3263844089833,
114.278154012734)) ;
#170270=CARTESIAN_POINT('Ctrl Pts',(-24.8957621143126,-14.4524065463604,
114.026303661662)) ;
#170271=CARTESIAN_POINT('Ctrl Pts',(-24.8882951456828,-14.3803719566858,
114.003560480852)) ;
#170272=CARTESIAN_POINT('Ctrl Pts',(-24.9620989760419,-14.3803719694669,
113.979329399385)) ;
#170273=CARTESIAN_POINT('Ctrl Pts',(-25.035902806401,-14.3803719822481,
113.955098317918)) ;
#170274=CARTESIAN_POINT('Ctrl Pts',(-25.0433697750307,-14.4524065719227,
113.977841498727)) ;
#170275=CARTESIAN_POINT('Ctrl Pts',(-25.0508367436604,-14.5244411615974,
114.000584679537)) ;
#170276=CARTESIAN_POINT('Ctrl Pts',(-24.9770329133014,-14.5244411488162,
114.024815761004)) ;
#170277=CARTESIAN_POINT('Ctrl Pts',(-24.9032290829423,-14.5244411360351,
114.049046842471)) ;
#170278=CARTESIAN_POINT('Ctrl Pts',(-24.8957621143126,-14.4524065463604,
114.026303661662)) ;
#170279=CARTESIAN_POINT('Ctrl Pts',(-24.8165686904461,-14.5048820459499,
113.749467211737)) ;
#170280=CARTESIAN_POINT('Ctrl Pts',(-24.8153570946285,-14.4290737092712,
113.745776887015)) ;
#170281=CARTESIAN_POINT('Ctrl Pts',(-24.8891609275668,-14.4290737099999,
113.721545813404)) ;
#170282=CARTESIAN_POINT('Ctrl Pts',(-24.9629647605052,-14.4290737107285,
113.697314739792)) ;
#170283=CARTESIAN_POINT('Ctrl Pts',(-24.9641763563227,-14.5048820474072,
113.701005064514)) ;
#170284=CARTESIAN_POINT('Ctrl Pts',(-24.9653879521404,-14.5806903840858,
113.704695389236)) ;
#170285=CARTESIAN_POINT('Ctrl Pts',(-24.891584119202,-14.5806903833572,
113.728926462847)) ;
#170286=CARTESIAN_POINT('Ctrl Pts',(-24.8177802862637,-14.5806903826285,
113.753157536459)) ;
#170287=CARTESIAN_POINT('Ctrl Pts',(-24.8165686904461,-14.5048820459499,
113.749467211737)) ;
#170288=CARTESIAN_POINT('Ctrl Pts',(-24.7369131556287,-14.4792643387988,
113.471526923201)) ;
#170289=CARTESIAN_POINT('Ctrl Pts',(-24.7419924769914,-14.4051302441696,
113.48699771704)) ;
#170290=CARTESIAN_POINT('Ctrl Pts',(-24.8157963123699,-14.4051302376983,
113.462766650861)) ;
#170291=CARTESIAN_POINT('Ctrl Pts',(-24.8896001477485,-14.405130231227,
113.438535584683)) ;
#170292=CARTESIAN_POINT('Ctrl Pts',(-24.8845208263858,-14.4792643258562,
113.423064790844)) ;
#170293=CARTESIAN_POINT('Ctrl Pts',(-24.8794415050231,-14.5533984204853,
113.407593997005)) ;
#170294=CARTESIAN_POINT('Ctrl Pts',(-24.8056376696446,-14.5533984269566,
113.431825063184)) ;
#170295=CARTESIAN_POINT('Ctrl Pts',(-24.731833834266,-14.5533984334279,
113.456056129363)) ;
#170296=CARTESIAN_POINT('Ctrl Pts',(-24.7369131556287,-14.4792643387988,
113.471526923201)) ;
#170297=CARTESIAN_POINT('Ctrl Pts',(-24.6622449881226,-14.3777623982077,
113.208611229877)) ;
#170298=CARTESIAN_POINT('Ctrl Pts',(-24.6732800440833,-14.3106033154662,
113.242222230191)) ;
#170299=CARTESIAN_POINT('Ctrl Pts',(-24.7470838825016,-14.3106033061414,
113.217991173271)) ;
#170300=CARTESIAN_POINT('Ctrl Pts',(-24.8208877209198,-14.3106032968165,
113.193760116351)) ;
#170301=CARTESIAN_POINT('Ctrl Pts',(-24.8098526649591,-14.377762379558,
113.160149116037)) ;
#170302=CARTESIAN_POINT('Ctrl Pts',(-24.7988176089984,-14.4449214622994,
113.126538115723)) ;
#170303=CARTESIAN_POINT('Ctrl Pts',(-24.7250137705801,-14.4449214716243,
113.150769172643)) ;
#170304=CARTESIAN_POINT('Ctrl Pts',(-24.6512099321618,-14.4449214809491,
113.175000229563)) ;
#170305=CARTESIAN_POINT('Ctrl Pts',(-24.6622449881226,-14.3777623982077,
113.208611229877)) ;
#170306=CARTESIAN_POINT('Ctrl Pts',(-24.59913585455,-14.2077004202751,112.980968522228)) ;
#170307=CARTESIAN_POINT('Ctrl Pts',(-24.6153271901671,-14.1523145589373,
113.030284718282)) ;
#170308=CARTESIAN_POINT('Ctrl Pts',(-24.6891310310512,-14.1523145504394,
113.006053668872)) ;
#170309=CARTESIAN_POINT('Ctrl Pts',(-24.7629348719354,-14.1523145419415,
112.981822619462)) ;
#170310=CARTESIAN_POINT('Ctrl Pts',(-24.7467435363182,-14.2077004032793,
112.932506423408)) ;
#170311=CARTESIAN_POINT('Ctrl Pts',(-24.7305522007011,-14.2630862646171,
112.883190227354)) ;
#170312=CARTESIAN_POINT('Ctrl Pts',(-24.656748359817,-14.2630862731151,
112.907421276764)) ;
#170313=CARTESIAN_POINT('Ctrl Pts',(-24.5829445189329,-14.263086281613,
112.931652326173)) ;
#170314=CARTESIAN_POINT('Ctrl Pts',(-24.59913585455,-14.2077004202751,112.980968522228)) ;
#170315=CARTESIAN_POINT('Ctrl Pts',(-24.5525713605202,-13.980362420234,
112.803591412359)) ;
#170316=CARTESIAN_POINT('Ctrl Pts',(-24.5727742599949,-13.9407671671798,
112.865126184531)) ;
#170317=CARTESIAN_POINT('Ctrl Pts',(-24.6465781027262,-13.9407671625387,
112.840895140748)) ;
#170318=CARTESIAN_POINT('Ctrl Pts',(-24.7203819454574,-13.9407671578977,
112.816664096964)) ;
#170319=CARTESIAN_POINT('Ctrl Pts',(-24.7001790459827,-13.980362410952,
112.755129324791)) ;
#170320=CARTESIAN_POINT('Ctrl Pts',(-24.679976146508,-14.0199576640062,
112.693594552618)) ;
#170321=CARTESIAN_POINT('Ctrl Pts',(-24.6061723037767,-14.0199576686472,
112.717825596402)) ;
#170322=CARTESIAN_POINT('Ctrl Pts',(-24.5323684610455,-14.0199576732883,
112.742056640186)) ;
#170323=CARTESIAN_POINT('Ctrl Pts',(-24.5525713605202,-13.980362420234,
112.803591412359)) ;
#170324=CARTESIAN_POINT('Ctrl Pts',(-24.5269666018519,-13.7128487430244,
112.690103143311)) ;
#170325=CARTESIAN_POINT('Ctrl Pts',(-24.5497224381023,-13.6918738812675,
112.759413748897)) ;
#170326=CARTESIAN_POINT('Ctrl Pts',(-24.6235262815752,-13.6918738808366,
112.735182707372)) ;
#170327=CARTESIAN_POINT('Ctrl Pts',(-24.697330125048,-13.6918738804057,
112.710951665847)) ;
#170328=CARTESIAN_POINT('Ctrl Pts',(-24.6745742887976,-13.7128487421626,
112.641641060262)) ;
#170329=CARTESIAN_POINT('Ctrl Pts',(-24.6518184525471,-13.7338236039195,
112.572330454676)) ;
#170330=CARTESIAN_POINT('Ctrl Pts',(-24.5780146090743,-13.7338236043504,
112.596561496201)) ;
#170331=CARTESIAN_POINT('Ctrl Pts',(-24.5042107656014,-13.7338236047813,
112.620792537726)) ;
#170332=CARTESIAN_POINT('Ctrl Pts',(-24.5269666018519,-13.7128487430244,
112.690103143311)) ;
#170333=CARTESIAN_POINT('Ctrl Pts',(-24.5248000668453,-13.4250762896625,
112.648103876864)) ;
#170334=CARTESIAN_POINT('Ctrl Pts',(-24.5484737092852,-13.4241646281582,
112.720209971964)) ;
#170335=CARTESIAN_POINT('Ctrl Pts',(-24.6222775527583,-13.424164630414,
112.69597893044)) ;
#170336=CARTESIAN_POINT('Ctrl Pts',(-24.6960813962314,-13.4241646326699,
112.671747888916)) ;
#170337=CARTESIAN_POINT('Ctrl Pts',(-24.6724077537915,-13.4250762941742,
112.599641793815)) ;
#170338=CARTESIAN_POINT('Ctrl Pts',(-24.6487341113515,-13.4259879556785,
112.527535698715)) ;
#170339=CARTESIAN_POINT('Ctrl Pts',(-24.5749302678784,-13.4259879534226,
112.551766740239)) ;
#170340=CARTESIAN_POINT('Ctrl Pts',(-24.5011264244053,-13.4259879511667,
112.575997781763)) ;
#170341=CARTESIAN_POINT('Ctrl Pts',(-24.5248000668453,-13.4250762896625,
112.648103876864)) ;
#170342=CARTESIAN_POINT('Ctrl Pts',(-24.5467181523936,-13.1369898154444,
112.679497598363)) ;
#170343=CARTESIAN_POINT('Ctrl Pts',(-24.5696282907065,-13.1561933535751,
112.749278183058)) ;
#170344=CARTESIAN_POINT('Ctrl Pts',(-24.6434321338206,-13.1561933570076,
112.725047140441)) ;
#170345=CARTESIAN_POINT('Ctrl Pts',(-24.7172359769348,-13.15619336044,112.700816097823)) ;
#170346=CARTESIAN_POINT('Ctrl Pts',(-24.6943258386219,-13.1369898223093,
112.631035513128)) ;
#170347=CARTESIAN_POINT('Ctrl Pts',(-24.6714157003091,-13.1177862841786,
112.561254928433)) ;
#170348=CARTESIAN_POINT('Ctrl Pts',(-24.597611857195,-13.1177862807461,
112.585485971051)) ;
#170349=CARTESIAN_POINT('Ctrl Pts',(-24.5238080140808,-13.1177862773137,
112.609717013668)) ;
#170350=CARTESIAN_POINT('Ctrl Pts',(-24.5467181523936,-13.1369898154444,
112.679497598363)) ;
#170351=CARTESIAN_POINT('Ctrl Pts',(-24.5926693672663,-12.8663855366991,
112.783721838426)) ;
#170352=CARTESIAN_POINT('Ctrl Pts',(-24.6131442990518,-12.9045144387046,
112.846085176993)) ;
#170353=CARTESIAN_POINT('Ctrl Pts',(-24.6869481421206,-12.9045144401406,
112.821854134237)) ;
#170354=CARTESIAN_POINT('Ctrl Pts',(-24.7607519851895,-12.9045144415766,
112.797623091482)) ;
#170355=CARTESIAN_POINT('Ctrl Pts',(-24.7402770534039,-12.8663855395711,
112.735259752915)) ;
#170356=CARTESIAN_POINT('Ctrl Pts',(-24.7198021216184,-12.8282566375656,
112.672896414349)) ;
#170357=CARTESIAN_POINT('Ctrl Pts',(-24.6459982785496,-12.8282566361296,
112.697127457104)) ;
#170358=CARTESIAN_POINT('Ctrl Pts',(-24.5721944354807,-12.8282566346936,
112.72135849986)) ;
#170359=CARTESIAN_POINT('Ctrl Pts',(-24.5926693672663,-12.8663855366991,
112.783721838426)) ;
#170360=CARTESIAN_POINT('Ctrl Pts',(-24.6589432293647,-12.6384940512534,
112.950297607118)) ;
#170361=CARTESIAN_POINT('Ctrl Pts',(-24.6755506105844,-12.6925911695923,
113.000881010742)) ;
#170362=CARTESIAN_POINT('Ctrl Pts',(-24.7493544541457,-12.6925911686239,
112.976649969486)) ;
#170363=CARTESIAN_POINT('Ctrl Pts',(-24.823158297707,-12.6925911676555,
112.952418928231)) ;
#170364=CARTESIAN_POINT('Ctrl Pts',(-24.8065509164873,-12.6384940493165,
112.901835524607)) ;
#170365=CARTESIAN_POINT('Ctrl Pts',(-24.7899435352676,-12.5843969309776,
112.851252120983)) ;
#170366=CARTESIAN_POINT('Ctrl Pts',(-24.7161396917063,-12.584396931946,
112.875483162238)) ;
#170367=CARTESIAN_POINT('Ctrl Pts',(-24.642335848145,-12.5843969329144,
112.899714203494)) ;
#170368=CARTESIAN_POINT('Ctrl Pts',(-24.6589432293647,-12.6384940512534,
112.950297607118)) ;
#170369=CARTESIAN_POINT('Ctrl Pts',(-24.7426000968426,-12.4647340958094,
113.169559327226)) ;
#170370=CARTESIAN_POINT('Ctrl Pts',(-24.7541259248004,-12.5310434351584,
113.20466513962)) ;
#170371=CARTESIAN_POINT('Ctrl Pts',(-24.8279297698228,-12.5310434317377,
113.180434102815)) ;
#170372=CARTESIAN_POINT('Ctrl Pts',(-24.9017336148452,-12.5310434283171,
113.156203066009)) ;
#170373=CARTESIAN_POINT('Ctrl Pts',(-24.8902077868874,-12.4647340889681,
113.121097253616)) ;
#170374=CARTESIAN_POINT('Ctrl Pts',(-24.8786819589297,-12.3984247496191,
113.085991441223)) ;
#170375=CARTESIAN_POINT('Ctrl Pts',(-24.8048781139073,-12.3984247530398,
113.110222478028)) ;
#170376=CARTESIAN_POINT('Ctrl Pts',(-24.7310742688849,-12.3984247564605,
113.134453514833)) ;
#170377=CARTESIAN_POINT('Ctrl Pts',(-24.7426000968426,-12.4647340958094,
113.169559327226)) ;
#170378=CARTESIAN_POINT('Ctrl Pts',(-24.8376583123465,-12.3600064377204,
113.423696409434)) ;
#170379=CARTESIAN_POINT('Ctrl Pts',(-24.8432960062769,-12.4337245690079,
113.440867915738)) ;
#170380=CARTESIAN_POINT('Ctrl Pts',(-24.917099853265,-12.4337245657129,
113.41663688492)) ;
#170381=CARTESIAN_POINT('Ctrl Pts',(-24.9909037002531,-12.4337245624179,
113.392405854102)) ;
#170382=CARTESIAN_POINT('Ctrl Pts',(-24.9852660063225,-12.3600064311304,
113.375234347797)) ;
#170383=CARTESIAN_POINT('Ctrl Pts',(-24.979628312392,-12.286288299843,113.358062841493)) ;
#170384=CARTESIAN_POINT('Ctrl Pts',(-24.905824465404,-12.286288303138,113.382293872311)) ;
#170385=CARTESIAN_POINT('Ctrl Pts',(-24.8320206184159,-12.286288306433,
113.406524903129)) ;
#170386=CARTESIAN_POINT('Ctrl Pts',(-24.8376583123465,-12.3600064377204,
113.423696409434)) ;
#170387=CARTESIAN_POINT('Ctrl Pts',(-24.9384569987699,-12.3305764766961,
113.695274669522)) ;
#170388=CARTESIAN_POINT('Ctrl Pts',(-24.9377981669915,-12.4064564353267,
113.69326797459)) ;
#170389=CARTESIAN_POINT('Ctrl Pts',(-25.0116020162607,-12.4064564352426,
113.66903695072)) ;
#170390=CARTESIAN_POINT('Ctrl Pts',(-25.08540586553,-12.4064564351584,113.64480592685)) ;
#170391=CARTESIAN_POINT('Ctrl Pts',(-25.0860646973084,-12.3305764765278,
113.646812621782)) ;
#170392=CARTESIAN_POINT('Ctrl Pts',(-25.0867235290868,-12.2546965178971,
113.648819316715)) ;
#170393=CARTESIAN_POINT('Ctrl Pts',(-25.0129196798176,-12.2546965179813,
113.673050340585)) ;
#170394=CARTESIAN_POINT('Ctrl Pts',(-24.9391158305484,-12.2546965180655,
113.697281364455)) ;
#170395=CARTESIAN_POINT('Ctrl Pts',(-24.9384569987699,-12.3305764766961,
113.695274669522)) ;
#170396=CARTESIAN_POINT('Ctrl Pts',(-25.0387364603478,-12.3793274592069,
113.965169521633)) ;
#170397=CARTESIAN_POINT('Ctrl Pts',(-25.0318103813017,-12.4519136571081,
113.944073802906)) ;
#170398=CARTESIAN_POINT('Ctrl Pts',(-25.1056142329247,-12.4519136645641,
113.919842786205)) ;
#170399=CARTESIAN_POINT('Ctrl Pts',(-25.1794180845476,-12.4519136720201,
113.895611769504)) ;
#170400=CARTESIAN_POINT('Ctrl Pts',(-25.1863441635937,-12.379327474119,
113.916707488231)) ;
#170401=CARTESIAN_POINT('Ctrl Pts',(-25.1932702426397,-12.3067412762178,
113.937803206958)) ;
#170402=CARTESIAN_POINT('Ctrl Pts',(-25.1194663910168,-12.3067412687618,
113.962034223658)) ;
#170403=CARTESIAN_POINT('Ctrl Pts',(-25.0456625393938,-12.3067412613058,
113.986265240359)) ;
#170404=CARTESIAN_POINT('Ctrl Pts',(-25.0387364603478,-12.3793274592069,
113.965169521633)) ;
#170405=CARTESIAN_POINT('Ctrl Pts',(-25.1313553076052,-12.5020990421703,
114.211888040928)) ;
#170406=CARTESIAN_POINT('Ctrl Pts',(-25.1186847142816,-12.5662179845147,
114.173295458733)) ;
#170407=CARTESIAN_POINT('Ctrl Pts',(-25.192488566993,-12.5662180028208,
114.149064445347)) ;
#170408=CARTESIAN_POINT('Ctrl Pts',(-25.2662924197043,-12.5662180211268,
114.124833431961)) ;
#170409=CARTESIAN_POINT('Ctrl Pts',(-25.2789630130279,-12.5020990787824,
114.163426014156)) ;
#170410=CARTESIAN_POINT('Ctrl Pts',(-25.2916336063514,-12.4379801364379,
114.20201859635)) ;
#170411=CARTESIAN_POINT('Ctrl Pts',(-25.21782975364,-12.4379801181319,114.226249609736)) ;
#170412=CARTESIAN_POINT('Ctrl Pts',(-25.1440259009287,-12.4379800998258,
114.250480623122)) ;
#170413=CARTESIAN_POINT('Ctrl Pts',(-25.1313553076052,-12.5020990421703,
114.211888040928)) ;
#170414=CARTESIAN_POINT('Ctrl Pts',(-25.2111527874365,-12.6906392671464,
114.419456391341)) ;
#170415=CARTESIAN_POINT('Ctrl Pts',(-25.1936266344623,-12.7416870715668,
114.366074558063)) ;
#170416=CARTESIAN_POINT('Ctrl Pts',(-25.2674304872085,-12.7416871035792,
114.341843544783)) ;
#170417=CARTESIAN_POINT('Ctrl Pts',(-25.3412343399546,-12.7416871355915,
114.317612531503)) ;
#170418=CARTESIAN_POINT('Ctrl Pts',(-25.3587604929287,-12.6906393311711,
114.370994364781)) ;
#170419=CARTESIAN_POINT('Ctrl Pts',(-25.3762866459028,-12.6395915267507,
114.424376198059)) ;
#170420=CARTESIAN_POINT('Ctrl Pts',(-25.3024827931567,-12.6395914947383,
114.448607211339)) ;
#170421=CARTESIAN_POINT('Ctrl Pts',(-25.2286789404106,-12.639591462726,
114.472838224619)) ;
#170422=CARTESIAN_POINT('Ctrl Pts',(-25.2111527874365,-12.6906392671464,
114.419456391341)) ;
#170423=CARTESIAN_POINT('Ctrl Pts',(-25.2729365333473,-12.9321841999642,
114.572061782235)) ;
#170424=CARTESIAN_POINT('Ctrl Pts',(-25.25180746659,-12.9664415034876,114.507706055091)) ;
#170425=CARTESIAN_POINT('Ctrl Pts',(-25.3256113176767,-12.9664415511475,
114.483475036757)) ;
#170426=CARTESIAN_POINT('Ctrl Pts',(-25.3994151687633,-12.9664415988073,
114.459244018423)) ;
#170427=CARTESIAN_POINT('Ctrl Pts',(-25.4205442355206,-12.9321842952839,
114.523599745566)) ;
#170428=CARTESIAN_POINT('Ctrl Pts',(-25.4416733022779,-12.8979269917605,
114.58795547271)) ;
#170429=CARTESIAN_POINT('Ctrl Pts',(-25.3678694511913,-12.8979269441006,
114.612186491044)) ;
#170430=CARTESIAN_POINT('Ctrl Pts',(-25.2940656001046,-12.8979268964408,
114.636417509379)) ;
#170431=CARTESIAN_POINT('Ctrl Pts',(-25.2729365333473,-12.9321841999642,
114.572061782235)) ;
#170432=CARTESIAN_POINT('Ctrl Pts',(-25.3126916179783,-13.2070342064579,
114.657780243976)) ;
#170433=CARTESIAN_POINT('Ctrl Pts',(-25.2894883187306,-13.2221513251204,
114.58710673949)) ;
#170434=CARTESIAN_POINT('Ctrl Pts',(-25.3632921660642,-13.2221513851254,
114.562875709725)) ;
#170435=CARTESIAN_POINT('Ctrl Pts',(-25.4370960133978,-13.2221514451304,
114.538644679959)) ;
#170436=CARTESIAN_POINT('Ctrl Pts',(-25.4602993126456,-13.2070343264679,
114.609318184445)) ;
#170437=CARTESIAN_POINT('Ctrl Pts',(-25.4835026118934,-13.1919172078054,
114.679991688931)) ;
#170438=CARTESIAN_POINT('Ctrl Pts',(-25.4096987645597,-13.1919171478004,
114.704222718696)) ;
#170439=CARTESIAN_POINT('Ctrl Pts',(-25.3358949172261,-13.1919170877954,
114.728453748462)) ;
#170440=CARTESIAN_POINT('Ctrl Pts',(-25.3126916179783,-13.2070342064579,
114.657780243976)) ;
#170441=CARTESIAN_POINT('Ctrl Pts',(-25.3287288342473,-13.4981307625057,
114.671102244044)) ;
#170442=CARTESIAN_POINT('Ctrl Pts',(-25.30510729808,-13.4929460625343,114.599154857553)) ;
#170443=CARTESIAN_POINT('Ctrl Pts',(-25.3789111400793,-13.492946132437,
114.57492381154)) ;
#170444=CARTESIAN_POINT('Ctrl Pts',(-25.4527149820785,-13.4929462023397,
114.550692765527)) ;
#170445=CARTESIAN_POINT('Ctrl Pts',(-25.4763365182457,-13.4981309023111,
114.622640152017)) ;
#170446=CARTESIAN_POINT('Ctrl Pts',(-25.499958054413,-13.5033156022825,
114.694587538508)) ;
#170447=CARTESIAN_POINT('Ctrl Pts',(-25.4261542124138,-13.5033155323798,
114.718818584521)) ;
#170448=CARTESIAN_POINT('Ctrl Pts',(-25.3523503704145,-13.5033154624771,
114.743049630534)) ;
#170449=CARTESIAN_POINT('Ctrl Pts',(-25.3287288342473,-13.4981307625057,
114.671102244044)) ;
#170450=CARTESIAN_POINT('Ctrl Pts',(-25.3205785524251,-13.7819922849582,
114.610954054946)) ;
#170451=CARTESIAN_POINT('Ctrl Pts',(-25.2982228761858,-13.7569816324817,
114.542862273677)) ;
#170452=CARTESIAN_POINT('Ctrl Pts',(-25.3720267117804,-13.7569817049211,
114.518631208156)) ;
#170453=CARTESIAN_POINT('Ctrl Pts',(-25.4458305473751,-13.7569817773604,
114.494400142636)) ;
#170454=CARTESIAN_POINT('Ctrl Pts',(-25.4681862236144,-13.7819924298369,
114.562491923905)) ;
#170455=CARTESIAN_POINT('Ctrl Pts',(-25.4905418998538,-13.8070030823134,
114.630583705174)) ;
#170456=CARTESIAN_POINT('Ctrl Pts',(-25.4167380642591,-13.807003009874,
114.654814770694)) ;
#170457=CARTESIAN_POINT('Ctrl Pts',(-25.3429342286645,-13.8070029374347,
114.679045836215)) ;
#170458=CARTESIAN_POINT('Ctrl Pts',(-25.3205785524251,-13.7819922849582,
114.610954054946)) ;
#170459=CARTESIAN_POINT('Ctrl Pts',(-25.2893677697261,-14.041794726603,
114.480288046438)) ;
#170460=CARTESIAN_POINT('Ctrl Pts',(-25.2698952365706,-13.9986090894959,
114.420977853969)) ;
#170461=CARTESIAN_POINT('Ctrl Pts',(-25.3436990649528,-13.998609159369,
114.39674676648)) ;
#170462=CARTESIAN_POINT('Ctrl Pts',(-25.4175028933349,-13.998609229242,
114.372515678992)) ;
#170463=CARTESIAN_POINT('Ctrl Pts',(-25.4369754264904,-14.0417948663491,
114.431825871461)) ;
#170464=CARTESIAN_POINT('Ctrl Pts',(-25.4564479596458,-14.0849805034562,
114.49113606393)) ;
#170465=CARTESIAN_POINT('Ctrl Pts',(-25.3826441312637,-14.0849804335832,
114.515367151419)) ;
#170466=CARTESIAN_POINT('Ctrl Pts',(-25.3088403028815,-14.0849803637101,
114.539598238908)) ;
#170467=CARTESIAN_POINT('Ctrl Pts',(-25.2893677697261,-14.041794726603,
114.480288046438)) ;
#170468=CARTESIAN_POINT('Ctrl Pts',(-25.2384611579753,-14.255449164482,
114.289862963828)) ;
#170469=CARTESIAN_POINT('Ctrl Pts',(-25.2232464047646,-14.197284228839,
114.243521282191)) ;
#170470=CARTESIAN_POINT('Ctrl Pts',(-25.2970502265122,-14.197284287096,
114.219290174495)) ;
#170471=CARTESIAN_POINT('Ctrl Pts',(-25.3708540482598,-14.197284345353,
114.195059066798)) ;
#170472=CARTESIAN_POINT('Ctrl Pts',(-25.3860688014705,-14.2554492809961,
114.241400748435)) ;
#170473=CARTESIAN_POINT('Ctrl Pts',(-25.4012835546813,-14.3136142166391,
114.287742430073)) ;
#170474=CARTESIAN_POINT('Ctrl Pts',(-25.3274797329337,-14.3136141583821,
114.311973537769)) ;
#170475=CARTESIAN_POINT('Ctrl Pts',(-25.2536759111861,-14.313614100125,
114.336204645465)) ;
#170476=CARTESIAN_POINT('Ctrl Pts',(-25.2384611579753,-14.255449164482,
114.289862963828)) ;
#170477=CARTESIAN_POINT('Ctrl Pts',(-25.1715626825997,-14.4102492008634,
114.050454773655)) ;
#170478=CARTESIAN_POINT('Ctrl Pts',(-25.161733771036,-14.3411914994799,
114.0205174968)) ;
#170479=CARTESIAN_POINT('Ctrl Pts',(-25.2355375868551,-14.3411915397154,
113.996286371046)) ;
#170480=CARTESIAN_POINT('Ctrl Pts',(-25.3093414026742,-14.3411915799509,
113.972055245292)) ;
#170481=CARTESIAN_POINT('Ctrl Pts',(-25.3191703142378,-14.4102492813345,
114.001992522148)) ;
#170482=CARTESIAN_POINT('Ctrl Pts',(-25.3289992258014,-14.4793069827181,
114.031929799003)) ;
#170483=CARTESIAN_POINT('Ctrl Pts',(-25.2551954099824,-14.4793069424825,
114.056160924757)) ;
#170484=CARTESIAN_POINT('Ctrl Pts',(-25.1813915941633,-14.479306902247,
114.080392050511)) ;
#170485=CARTESIAN_POINT('Ctrl Pts',(-25.1715626825997,-14.4102492008634,
114.050454773655)) ;
#170486=CARTESIAN_POINT('Ctrl Pts',(-25.0954032709923,-14.4927425304254,
113.7832103655)) ;
#170487=CARTESIAN_POINT('Ctrl Pts',(-25.0916071708474,-14.4178249477771,
113.771648058903)) ;
#170488=CARTESIAN_POINT('Ctrl Pts',(-25.1654109832459,-14.4178249636249,
113.747416922731)) ;
#170489=CARTESIAN_POINT('Ctrl Pts',(-25.2392147956444,-14.4178249794727,
113.723185786558)) ;
#170490=CARTESIAN_POINT('Ctrl Pts',(-25.2430108957893,-14.4927425621209,
113.734748093156)) ;
#170491=CARTESIAN_POINT('Ctrl Pts',(-25.2468069959341,-14.5676601447692,
113.746310399753)) ;
#170492=CARTESIAN_POINT('Ctrl Pts',(-25.1730031835356,-14.5676601289214,
113.770541535925)) ;
#170493=CARTESIAN_POINT('Ctrl Pts',(-25.0991993711371,-14.5676601130736,
113.794772672097)) ;
#170494=CARTESIAN_POINT('Ctrl Pts',(-25.0954032709923,-14.4927425304254,
113.7832103655)) ;
#170495=CARTESIAN_POINT('Ctrl Pts',(-25.0150521907154,-14.4990616510816,
113.502979825597)) ;
#170496=CARTESIAN_POINT('Ctrl Pts',(-25.0175947209408,-14.4235929848165,
113.510723964445)) ;
#170497=CARTESIAN_POINT('Ctrl Pts',(-25.0913985319841,-14.4235929732871,
113.486492824145)) ;
#170498=CARTESIAN_POINT('Ctrl Pts',(-25.1652023430274,-14.4235929617576,
113.462261683846)) ;
#170499=CARTESIAN_POINT('Ctrl Pts',(-25.162659812802,-14.4990616280226,
113.454517544997)) ;
#170500=CARTESIAN_POINT('Ctrl Pts',(-25.1601172825766,-14.5745302942877,
113.446773406148)) ;
#170501=CARTESIAN_POINT('Ctrl Pts',(-25.0863134715333,-14.5745303058172,
113.471004546448)) ;
#170502=CARTESIAN_POINT('Ctrl Pts',(-25.01250966049,-14.5745303173466,113.495235686748)) ;
#170503=CARTESIAN_POINT('Ctrl Pts',(-25.0150521907154,-14.4990616510816,
113.502979825597)) ;
#170504=CARTESIAN_POINT('Ctrl Pts',(-24.9375447991963,-14.4278621718276,
113.231466674976)) ;
#170505=CARTESIAN_POINT('Ctrl Pts',(-24.9462355998666,-14.3572534635398,
113.257937453626)) ;
#170506=CARTESIAN_POINT('Ctrl Pts',(-25.0200394123353,-14.357253423911,
113.233706317668)) ;
#170507=CARTESIAN_POINT('Ctrl Pts',(-25.0938432248041,-14.3572533842822,
113.20947518171)) ;
#170508=CARTESIAN_POINT('Ctrl Pts',(-25.0851524241338,-14.4278620925699,
113.18300440306)) ;
#170509=CARTESIAN_POINT('Ctrl Pts',(-25.0764616234635,-14.4984708008576,
113.15653362441)) ;
#170510=CARTESIAN_POINT('Ctrl Pts',(-25.0026578109947,-14.4984708404865,
113.180764760368)) ;
#170511=CARTESIAN_POINT('Ctrl Pts',(-24.928853998526,-14.4984708801153,
113.204995896326)) ;
#170512=CARTESIAN_POINT('Ctrl Pts',(-24.9375447991963,-14.4278621718276,
113.231466674976)) ;
#170513=CARTESIAN_POINT('Ctrl Pts',(-24.8688494001846,-14.2839264835508,
112.986674234856)) ;
#170514=CARTESIAN_POINT('Ctrl Pts',(-24.8830847973271,-14.2232622888904,
113.030032959772)) ;
#170515=CARTESIAN_POINT('Ctrl Pts',(-24.9568886138432,-14.2232622233179,
113.005801836142)) ;
#170516=CARTESIAN_POINT('Ctrl Pts',(-25.0306924303592,-14.2232621577455,
112.981570712511)) ;
#170517=CARTESIAN_POINT('Ctrl Pts',(-25.0164570332166,-14.2839263524059,
112.938211987594)) ;
#170518=CARTESIAN_POINT('Ctrl Pts',(-25.0022216360741,-14.3445905470663,
112.894853262678)) ;
#170519=CARTESIAN_POINT('Ctrl Pts',(-24.928417819558,-14.3445906126388,
112.919084386308)) ;
#170520=CARTESIAN_POINT('Ctrl Pts',(-24.854614003042,-14.3445906782112,
112.943315509939)) ;
#170521=CARTESIAN_POINT('Ctrl Pts',(-24.8688494001846,-14.2839264835508,
112.986674234856)) ;
#170522=CARTESIAN_POINT('Ctrl Pts',(-24.815043038472,-14.0776636855761,
112.787261502365)) ;
#170523=CARTESIAN_POINT('Ctrl Pts',(-24.8337912269029,-14.0313099788708,
112.844365461409)) ;
#170524=CARTESIAN_POINT('Ctrl Pts',(-24.9075950498521,-14.0313098927161,
112.820134357373)) ;
#170525=CARTESIAN_POINT('Ctrl Pts',(-24.9813988728013,-14.0313098065613,
112.795903253336)) ;
#170526=CARTESIAN_POINT('Ctrl Pts',(-24.9626506843704,-14.0776635132666,
112.738799294292)) ;
#170527=CARTESIAN_POINT('Ctrl Pts',(-24.9439024959395,-14.1240172199719,
112.681695335248)) ;
#170528=CARTESIAN_POINT('Ctrl Pts',(-24.8700986729903,-14.1240173061266,
112.705926439284)) ;
#170529=CARTESIAN_POINT('Ctrl Pts',(-24.7962948500411,-14.1240173922814,
112.730157543321)) ;
#170530=CARTESIAN_POINT('Ctrl Pts',(-24.815043038472,-14.0776636855761,
112.787261502365)) ;
#170531=CARTESIAN_POINT('Ctrl Pts',(-24.7807407303966,-13.825817961869,
112.647479206348)) ;
#170532=CARTESIAN_POINT('Ctrl Pts',(-24.8026420004503,-13.7969788395993,
112.714186943252)) ;
#170533=CARTESIAN_POINT('Ctrl Pts',(-24.8764458313452,-13.7969787399069,
112.689955863417)) ;
#170534=CARTESIAN_POINT('Ctrl Pts',(-24.95024966224,-13.7969786402144,112.665724783582)) ;
#170535=CARTESIAN_POINT('Ctrl Pts',(-24.9283483921862,-13.8258177624841,
112.599017046678)) ;
#170536=CARTESIAN_POINT('Ctrl Pts',(-24.9064471221324,-13.8546568847537,
112.532309309774)) ;
#170537=CARTESIAN_POINT('Ctrl Pts',(-24.8326432912376,-13.8546569844462,
112.556540389609)) ;
#170538=CARTESIAN_POINT('Ctrl Pts',(-24.7588394603428,-13.8546570841386,
112.580771469444)) ;
#170539=CARTESIAN_POINT('Ctrl Pts',(-24.7807407303966,-13.825817961869,
112.647479206348)) ;
#170540=CARTESIAN_POINT('Ctrl Pts',(-24.7687598363281,-13.5431962708422,
112.575457209354)) ;
#170541=CARTESIAN_POINT('Ctrl Pts',(-24.7922654208681,-13.5340457388908,
112.647051429285)) ;
#170542=CARTESIAN_POINT('Ctrl Pts',(-24.8660692605831,-13.5340456342861,
112.622820376315)) ;
#170543=CARTESIAN_POINT('Ctrl Pts',(-24.9398731002982,-13.5340455296813,
112.598589323345)) ;
#170544=CARTESIAN_POINT('Ctrl Pts',(-24.9163675157582,-13.5431960616327,
112.526995103414)) ;
#170545=CARTESIAN_POINT('Ctrl Pts',(-24.8928619312182,-13.5523465935841,
112.455400883483)) ;
#170546=CARTESIAN_POINT('Ctrl Pts',(-24.8190580915032,-13.5523466981889,
112.479631936453)) ;
#170547=CARTESIAN_POINT('Ctrl Pts',(-24.7452542517881,-13.5523468027936,
112.503862989423)) ;
#170548=CARTESIAN_POINT('Ctrl Pts',(-24.7687598363281,-13.5431962708422,
112.575457209354)) ;
#170549=CARTESIAN_POINT('Ctrl Pts',(-24.7809665685125,-13.2523620051609,
112.577212862889)) ;
#170550=CARTESIAN_POINT('Ctrl Pts',(-24.8043879898163,-13.2635030369063,
112.648550735123)) ;
#170551=CARTESIAN_POINT('Ctrl Pts',(-24.878191838198,-13.2635029359697,
112.62431970855)) ;
#170552=CARTESIAN_POINT('Ctrl Pts',(-24.9519956865798,-13.2635028350331,
112.600088681977)) ;
#170553=CARTESIAN_POINT('Ctrl Pts',(-24.9285742652759,-13.2523618032878,
112.528750809743)) ;
#170554=CARTESIAN_POINT('Ctrl Pts',(-24.9051528439722,-13.2412207715424,
112.457412937509)) ;
#170555=CARTESIAN_POINT('Ctrl Pts',(-24.8313489955904,-13.241220872479,
112.481643964082)) ;
#170556=CARTESIAN_POINT('Ctrl Pts',(-24.7575451472087,-13.2412209734156,
112.505874990655)) ;
#170557=CARTESIAN_POINT('Ctrl Pts',(-24.7809665685125,-13.2523620051609,
112.577212862889)) ;
#170558=CARTESIAN_POINT('Ctrl Pts',(-24.8172568115443,-12.972854005055,
112.652243647584)) ;
#170559=CARTESIAN_POINT('Ctrl Pts',(-24.8389143107608,-13.0035262645876,
112.718208897662)) ;
#170560=CARTESIAN_POINT('Ctrl Pts',(-24.9127181667632,-13.0035261755681,
112.6939778943)) ;
#170561=CARTESIAN_POINT('Ctrl Pts',(-24.9865220227656,-13.0035260865486,
112.669746890938)) ;
#170562=CARTESIAN_POINT('Ctrl Pts',(-24.9648645235491,-12.9728538270159,
112.603781640861)) ;
#170563=CARTESIAN_POINT('Ctrl Pts',(-24.9432070243326,-12.9421815674833,
112.537816390783)) ;
#170564=CARTESIAN_POINT('Ctrl Pts',(-24.8694031683302,-12.9421816565028,
112.562047394144)) ;
#170565=CARTESIAN_POINT('Ctrl Pts',(-24.7955993123278,-12.9421817455224,
112.586278397506)) ;
#170566=CARTESIAN_POINT('Ctrl Pts',(-24.8172568115443,-12.972854005055,
112.652243647584)) ;
#170567=CARTESIAN_POINT('Ctrl Pts',(-24.8754805907761,-12.7260422771964,
112.794217709271)) ;
#170568=CARTESIAN_POINT('Ctrl Pts',(-24.8938372765157,-12.7739923813095,
112.850129213994)) ;
#170569=CARTESIAN_POINT('Ctrl Pts',(-24.9676411385468,-12.7739923097986,
112.825898228995)) ;
#170570=CARTESIAN_POINT('Ctrl Pts',(-25.041445000578,-12.7739922382878,
112.801667243996)) ;
#170571=CARTESIAN_POINT('Ctrl Pts',(-25.0230883148385,-12.7260421341746,
112.745755739273)) ;
#170572=CARTESIAN_POINT('Ctrl Pts',(-25.0047316290989,-12.6780920300614,
112.68984423455)) ;
#170573=CARTESIAN_POINT('Ctrl Pts',(-24.9309277670678,-12.6780921015723,
112.714075219549)) ;
#170574=CARTESIAN_POINT('Ctrl Pts',(-24.8571239050366,-12.6780921730832,
112.738306204548)) ;
#170575=CARTESIAN_POINT('Ctrl Pts',(-24.8754805907761,-12.7260422771964,
112.794217709271)) ;
#170576=CARTESIAN_POINT('Ctrl Pts',(-24.9530612233143,-12.5272823112894,
112.994865114969)) ;
#170577=CARTESIAN_POINT('Ctrl Pts',(-24.9667668683183,-12.5891820336003,
113.03661029991)) ;
#170578=CARTESIAN_POINT('Ctrl Pts',(-25.0405707337368,-12.5891819848851,
113.012379325228)) ;
#170579=CARTESIAN_POINT('Ctrl Pts',(-25.1143745991552,-12.58918193617,112.988148350546)) ;
#170580=CARTESIAN_POINT('Ctrl Pts',(-25.1006689541512,-12.5272822138591,
112.946403165605)) ;
#170581=CARTESIAN_POINT('Ctrl Pts',(-25.0869633091472,-12.4653824915483,
112.904657980664)) ;
#170582=CARTESIAN_POINT('Ctrl Pts',(-25.0131594437287,-12.4653825402634,
112.928888955346)) ;
#170583=CARTESIAN_POINT('Ctrl Pts',(-24.9393555783103,-12.4653825889786,
112.953119930028)) ;
#170584=CARTESIAN_POINT('Ctrl Pts',(-24.9530612233143,-12.5272823112894,
112.994865114969)) ;
#170585=CARTESIAN_POINT('Ctrl Pts',(-25.043926335439,-12.3938739809445,
113.23628572976)) ;
#170586=CARTESIAN_POINT('Ctrl Pts',(-25.0520397402365,-12.4651813337181,
113.26099785322)) ;
#170587=CARTESIAN_POINT('Ctrl Pts',(-25.1258436071122,-12.4651813074342,
113.236766882977)) ;
#170588=CARTESIAN_POINT('Ctrl Pts',(-25.1996474739879,-12.4651812811503,
113.212535912733)) ;
#170589=CARTESIAN_POINT('Ctrl Pts',(-25.1915340691904,-12.3938739283766,
113.187823789273)) ;
#170590=CARTESIAN_POINT('Ctrl Pts',(-25.1834206643929,-12.322566575603,
113.163111665812)) ;
#170591=CARTESIAN_POINT('Ctrl Pts',(-25.1096167975172,-12.3225666018869,
113.187342636056)) ;
#170592=CARTESIAN_POINT('Ctrl Pts',(-25.0358129306415,-12.3225666281708,
113.211573606299)) ;
#170593=CARTESIAN_POINT('Ctrl Pts',(-25.043926335439,-12.3938739809445,
113.23628572976)) ;
#170594=CARTESIAN_POINT('Ctrl Pts',(-25.1433950034912,-12.3331330123649,
113.503738250658)) ;
#170595=CARTESIAN_POINT('Ctrl Pts',(-25.1453107042945,-12.4087892430706,
113.509573167594)) ;
#170596=CARTESIAN_POINT('Ctrl Pts',(-25.2191145700333,-12.408789238365,
113.485342193888)) ;
#170597=CARTESIAN_POINT('Ctrl Pts',(-25.2929184357722,-12.4087892336594,
113.461111220182)) ;
#170598=CARTESIAN_POINT('Ctrl Pts',(-25.2910027349689,-12.3331330029537,
113.455276303246)) ;
#170599=CARTESIAN_POINT('Ctrl Pts',(-25.2890870341656,-12.257476772248,
113.44944138631)) ;
#170600=CARTESIAN_POINT('Ctrl Pts',(-25.2152831684267,-12.2574767769536,
113.473672360017)) ;
#170601=CARTESIAN_POINT('Ctrl Pts',(-25.1414793026879,-12.2574767816592,
113.497903333723)) ;
#170602=CARTESIAN_POINT('Ctrl Pts',(-25.1433950034912,-12.3331330123649,
113.503738250658)) ;
#170603=CARTESIAN_POINT('Ctrl Pts',(-25.2443302602174,-12.3500900604043,
113.775797196118)) ;
#170604=CARTESIAN_POINT('Ctrl Pts',(-25.2399335184134,-12.4246766699504,
113.76240543124)) ;
#170605=CARTESIAN_POINT('Ctrl Pts',(-25.3137373815055,-12.4246766830339,
113.738174449473)) ;
#170606=CARTESIAN_POINT('Ctrl Pts',(-25.3875412445977,-12.4246766961173,
113.713943467705)) ;
#170607=CARTESIAN_POINT('Ctrl Pts',(-25.3919379864017,-12.3500900865712,
113.727335232583)) ;
#170608=CARTESIAN_POINT('Ctrl Pts',(-25.3963347282057,-12.2755034770251,
113.740726997461)) ;
#170609=CARTESIAN_POINT('Ctrl Pts',(-25.3225308651136,-12.2755034639416,
113.764957979228)) ;
#170610=CARTESIAN_POINT('Ctrl Pts',(-25.2487270020214,-12.2755034508582,
113.789188960996)) ;
#170611=CARTESIAN_POINT('Ctrl Pts',(-25.2443302602174,-12.3500900604043,
113.775797196118)) ;
#170612=CARTESIAN_POINT('Ctrl Pts',(-25.3412640091243,-12.4439523224458,
114.035430164998)) ;
#170613=CARTESIAN_POINT('Ctrl Pts',(-25.3308294983348,-12.5120989674076,
114.003648329789)) ;
#170614=CARTESIAN_POINT('Ctrl Pts',(-25.4046333568467,-12.5120989925412,
113.979417334071)) ;
#170615=CARTESIAN_POINT('Ctrl Pts',(-25.4784372153586,-12.5120990176749,
113.955186338353)) ;
#170616=CARTESIAN_POINT('Ctrl Pts',(-25.4888717261481,-12.4439523727131,
113.986968173562)) ;
#170617=CARTESIAN_POINT('Ctrl Pts',(-25.4993062369376,-12.3758057277512,
114.01875000877)) ;
#170618=CARTESIAN_POINT('Ctrl Pts',(-25.4255023784257,-12.3758057026176,
114.042981004488)) ;
#170619=CARTESIAN_POINT('Ctrl Pts',(-25.3516985199137,-12.3758056774839,
114.067212000207)) ;
#170620=CARTESIAN_POINT('Ctrl Pts',(-25.3412640091243,-12.4439523224458,
114.035430164998)) ;
#170621=CARTESIAN_POINT('Ctrl Pts',(-25.4269581595394,-12.607738556858,
114.260951876422)) ;
#170622=CARTESIAN_POINT('Ctrl Pts',(-25.411258848313,-12.6645527953263,
114.213134308381)) ;
#170623=CARTESIAN_POINT('Ctrl Pts',(-25.485062702167,-12.6645528262529,
114.188903298476)) ;
#170624=CARTESIAN_POINT('Ctrl Pts',(-25.558866556021,-12.6645528571796,
114.16467228857)) ;
#170625=CARTESIAN_POINT('Ctrl Pts',(-25.5745658672475,-12.6077386187113,
114.212489856611)) ;
#170626=CARTESIAN_POINT('Ctrl Pts',(-25.5902651784739,-12.5509243802431,
114.260307424651)) ;
#170627=CARTESIAN_POINT('Ctrl Pts',(-25.5164613246199,-12.5509243493165,
114.284538434557)) ;
#170628=CARTESIAN_POINT('Ctrl Pts',(-25.4426574707659,-12.5509243183898,
114.308769444462)) ;
#170629=CARTESIAN_POINT('Ctrl Pts',(-25.4269581595394,-12.607738556858,
114.260951876422)) ;
#170630=CARTESIAN_POINT('Ctrl Pts',(-25.4961702874896,-12.8282760815645,
114.436439976788)) ;
#170631=CARTESIAN_POINT('Ctrl Pts',(-25.4763456274778,-12.8697778180786,
114.376057261829)) ;
#170632=CARTESIAN_POINT('Ctrl Pts',(-25.5501494771654,-12.8697778506645,
114.351826239234)) ;
#170633=CARTESIAN_POINT('Ctrl Pts',(-25.6239533268531,-12.8697778832504,
114.327595216638)) ;
#170634=CARTESIAN_POINT('Ctrl Pts',(-25.6437779868649,-12.8282761467363,
114.387977931597)) ;
#170635=CARTESIAN_POINT('Ctrl Pts',(-25.6636026468767,-12.7867744102223,
114.448360646555)) ;
#170636=CARTESIAN_POINT('Ctrl Pts',(-25.589798797189,-12.7867743776364,
114.472591669151)) ;
#170637=CARTESIAN_POINT('Ctrl Pts',(-25.5159949475014,-12.7867743450505,
114.496822691746)) ;
#170638=CARTESIAN_POINT('Ctrl Pts',(-25.4961702874896,-12.8282760815645,
114.436439976788)) ;
#170639=CARTESIAN_POINT('Ctrl Pts',(-25.5453502164331,-13.0924261676405,
114.550696842166)) ;
#170640=CARTESIAN_POINT('Ctrl Pts',(-25.5227969254224,-13.1155471529824,
114.48200315727)) ;
#170641=CARTESIAN_POINT('Ctrl Pts',(-25.5966007713147,-13.1155471809982,
114.457772123114)) ;
#170642=CARTESIAN_POINT('Ctrl Pts',(-25.6704046172069,-13.1155472090139,
114.433541088958)) ;
#170643=CARTESIAN_POINT('Ctrl Pts',(-25.6929579082176,-13.092426223672,
114.502234773854)) ;
#170644=CARTESIAN_POINT('Ctrl Pts',(-25.7155111992283,-13.06930523833,114.57092845875)) ;
#170645=CARTESIAN_POINT('Ctrl Pts',(-25.641707353336,-13.0693052103143,
114.595159492906)) ;
#170646=CARTESIAN_POINT('Ctrl Pts',(-25.5679035074438,-13.0693051822985,
114.619390527062)) ;
#170647=CARTESIAN_POINT('Ctrl Pts',(-25.5453502164331,-13.0924261676405,
114.550696842166)) ;
#170648=CARTESIAN_POINT('Ctrl Pts',(-25.5711878044013,-13.3792544087802,
114.593953694912)) ;
#170649=CARTESIAN_POINT('Ctrl Pts',(-25.5475296838539,-13.3823829246599,
114.52189487736)) ;
#170650=CARTESIAN_POINT('Ctrl Pts',(-25.6213335272747,-13.3823829459244,
114.497663835676)) ;
#170651=CARTESIAN_POINT('Ctrl Pts',(-25.6951373706955,-13.3823829671888,
114.473432793993)) ;
#170652=CARTESIAN_POINT('Ctrl Pts',(-25.7187954912429,-13.3792544513091,
114.545491611545)) ;
#170653=CARTESIAN_POINT('Ctrl Pts',(-25.7424536117902,-13.3761259354293,
114.617550429098)) ;
#170654=CARTESIAN_POINT('Ctrl Pts',(-25.6686497683694,-13.3761259141649,
114.641781470781)) ;
#170655=CARTESIAN_POINT('Ctrl Pts',(-25.5948459249486,-13.3761258929005,
114.666012512465)) ;
#170656=CARTESIAN_POINT('Ctrl Pts',(-25.5711878044013,-13.3792544087802,
114.593953694912)) ;
#170657=CARTESIAN_POINT('Ctrl Pts',(-25.572740914633,-13.6698091146606,
114.563123414499)) ;
#170658=CARTESIAN_POINT('Ctrl Pts',(-25.5496743867624,-13.6526542862593,
114.492866492629)) ;
#170659=CARTESIAN_POINT('Ctrl Pts',(-25.6234782290232,-13.6526542988554,
114.468635447412)) ;
#170660=CARTESIAN_POINT('Ctrl Pts',(-25.697282071284,-13.6526543114514,
114.444404402195)) ;
#170661=CARTESIAN_POINT('Ctrl Pts',(-25.7203485991545,-13.6698091398527,
114.514661324065)) ;
#170662=CARTESIAN_POINT('Ctrl Pts',(-25.7434151270251,-13.686963968254,
114.584918245935)) ;
#170663=CARTESIAN_POINT('Ctrl Pts',(-25.6696112847643,-13.686963955658,
114.609149291152)) ;
#170664=CARTESIAN_POINT('Ctrl Pts',(-25.5958074425035,-13.6869639430619,
114.633380336369)) ;
#170665=CARTESIAN_POINT('Ctrl Pts',(-25.572740914633,-13.6698091146606,
114.563123414499)) ;
#170666=CARTESIAN_POINT('Ctrl Pts',(-25.5505747674364,-13.9412445098837,
114.460172921106)) ;
#170667=CARTESIAN_POINT('Ctrl Pts',(-25.5297546025764,-13.9051106030385,
114.396758058401)) ;
#170668=CARTESIAN_POINT('Ctrl Pts',(-25.6035584448034,-13.9051106090347,
114.372527013081)) ;
#170669=CARTESIAN_POINT('Ctrl Pts',(-25.6773622870305,-13.905110615031,
114.348295967762)) ;
#170670=CARTESIAN_POINT('Ctrl Pts',(-25.6981824518905,-13.9412445218762,
114.411710830467)) ;
#170671=CARTESIAN_POINT('Ctrl Pts',(-25.7190026167506,-13.9773784287214,
114.475125693173)) ;
#170672=CARTESIAN_POINT('Ctrl Pts',(-25.6451987745235,-13.9773784227252,
114.499356738492)) ;
#170673=CARTESIAN_POINT('Ctrl Pts',(-25.5713949322964,-13.9773784167289,
114.523587783811)) ;
#170674=CARTESIAN_POINT('Ctrl Pts',(-25.5505747674364,-13.9412445098837,
114.460172921106)) ;
#170675=CARTESIAN_POINT('Ctrl Pts',(-25.5073811967448,-14.1747166899893,
114.293293093269)) ;
#170676=CARTESIAN_POINT('Ctrl Pts',(-25.4902767699507,-14.1222263839683,
114.241195769094)) ;
#170677=CARTESIAN_POINT('Ctrl Pts',(-25.5640806127003,-14.1222263855747,
114.216964725366)) ;
#170678=CARTESIAN_POINT('Ctrl Pts',(-25.6378844554499,-14.122226387181,
114.192733681639)) ;
#170679=CARTESIAN_POINT('Ctrl Pts',(-25.654988882244,-14.1747166932021,
114.244831005813)) ;
#170680=CARTESIAN_POINT('Ctrl Pts',(-25.672093309038,-14.2272069992232,
114.296928329988)) ;
#170681=CARTESIAN_POINT('Ctrl Pts',(-25.5982894662884,-14.2272069976168,
114.321159373716)) ;
#170682=CARTESIAN_POINT('Ctrl Pts',(-25.5244856235388,-14.2272069960104,
114.345390417444)) ;
#170683=CARTESIAN_POINT('Ctrl Pts',(-25.5073811967448,-14.1747166899893,
114.293293093269)) ;
#170684=CARTESIAN_POINT('Ctrl Pts',(-25.4463048591916,-14.355514528968,
114.071666128729)) ;
#170685=CARTESIAN_POINT('Ctrl Pts',(-25.4341763419453,-14.2903204554486,
114.034724622094)) ;
#170686=CARTESIAN_POINT('Ctrl Pts',(-25.5079801857457,-14.2903204543728,
114.010493581567)) ;
#170687=CARTESIAN_POINT('Ctrl Pts',(-25.581784029546,-14.290320453297,113.98626254104)) ;
#170688=CARTESIAN_POINT('Ctrl Pts',(-25.5939125467923,-14.3555145268165,
114.023204047674)) ;
#170689=CARTESIAN_POINT('Ctrl Pts',(-25.6060410640385,-14.4207086003359,
114.060145554309)) ;
#170690=CARTESIAN_POINT('Ctrl Pts',(-25.5322372202382,-14.4207086014117,
114.084376594836)) ;
#170691=CARTESIAN_POINT('Ctrl Pts',(-25.4584333764379,-14.4207086024875,
114.108607635363)) ;
#170692=CARTESIAN_POINT('Ctrl Pts',(-25.4463048591916,-14.355514528968,
114.071666128729)) ;
#170693=CARTESIAN_POINT('Ctrl Pts',(-25.3732239530328,-14.4682461385157,
113.813679160758)) ;
#170694=CARTESIAN_POINT('Ctrl Pts',(-25.3669130070119,-14.3950833007867,
113.794457037381)) ;
#170695=CARTESIAN_POINT('Ctrl Pts',(-25.4407168514207,-14.3950832998909,
113.770225998707)) ;
#170696=CARTESIAN_POINT('Ctrl Pts',(-25.5145206958295,-14.395083298995,
113.745994960033)) ;
#170697=CARTESIAN_POINT('Ctrl Pts',(-25.5208316418504,-14.468246136724,
113.76521708341)) ;
#170698=CARTESIAN_POINT('Ctrl Pts',(-25.5271425878713,-14.5414089744529,
113.784439206786)) ;
#170699=CARTESIAN_POINT('Ctrl Pts',(-25.4533387434625,-14.5414089753487,
113.80867024546)) ;
#170700=CARTESIAN_POINT('Ctrl Pts',(-25.3795348990537,-14.5414089762446,
113.832901284134)) ;
#170701=CARTESIAN_POINT('Ctrl Pts',(-25.3732239530328,-14.4682461385157,
113.813679160758)) ;
#170702=CARTESIAN_POINT('Ctrl Pts',(-25.2933869167422,-14.5059599121584,
113.534915352588)) ;
#170703=CARTESIAN_POINT('Ctrl Pts',(-25.2933783368985,-14.4300548891346,
113.534889219716)) ;
#170704=CARTESIAN_POINT('Ctrl Pts',(-25.3671821811493,-14.4300548892677,
113.510658180561)) ;
#170705=CARTESIAN_POINT('Ctrl Pts',(-25.4409860254001,-14.4300548894008,
113.486427141406)) ;
#170706=CARTESIAN_POINT('Ctrl Pts',(-25.4409946052437,-14.5059599124246,
113.486453274277)) ;
#170707=CARTESIAN_POINT('Ctrl Pts',(-25.4410031850873,-14.5818649354484,
113.486479407148)) ;
#170708=CARTESIAN_POINT('Ctrl Pts',(-25.3671993408365,-14.5818649353153,
113.510710446304)) ;
#170709=CARTESIAN_POINT('Ctrl Pts',(-25.2933954965857,-14.5818649351822,
113.534941485459)) ;
#170710=CARTESIAN_POINT('Ctrl Pts',(-25.2933869167422,-14.5059599121584,
113.534915352588)) ;
#170711=CARTESIAN_POINT('Ctrl Pts',(-25.2143421603494,-14.4658731530402,
113.258876232179)) ;
#170712=CARTESIAN_POINT('Ctrl Pts',(-25.2205830584677,-14.3926562072765,
113.27788500087)) ;
#170713=CARTESIAN_POINT('Ctrl Pts',(-25.2943869020412,-14.3926562077147,
113.253653959652)) ;
#170714=CARTESIAN_POINT('Ctrl Pts',(-25.3681907456146,-14.3926562081529,
113.229422918433)) ;
#170715=CARTESIAN_POINT('Ctrl Pts',(-25.3619498474963,-14.4658731539167,
113.210414149742)) ;
#170716=CARTESIAN_POINT('Ctrl Pts',(-25.355708949378,-14.5390900996804,
113.191405381051)) ;
#170717=CARTESIAN_POINT('Ctrl Pts',(-25.2819051058046,-14.5390900992422,
113.215636422269)) ;
#170718=CARTESIAN_POINT('Ctrl Pts',(-25.2081012622311,-14.539090098804,
113.239867463488)) ;
#170719=CARTESIAN_POINT('Ctrl Pts',(-25.2143421603494,-14.4658731530402,
113.258876232179)) ;
#170720=CARTESIAN_POINT('Ctrl Pts',(-25.1412442200855,-14.3505784504634,
113.000683869835)) ;
#170721=CARTESIAN_POINT('Ctrl Pts',(-25.153334124402,-14.2853046871927,
113.037507767757)) ;
#170722=CARTESIAN_POINT('Ctrl Pts',(-25.2271379667205,-14.2853046856717,
113.013276722716)) ;
#170723=CARTESIAN_POINT('Ctrl Pts',(-25.300941809039,-14.2853046841507,
112.989045677675)) ;
#170724=CARTESIAN_POINT('Ctrl Pts',(-25.2888519047224,-14.3505784474213,
112.952221779753)) ;
#170725=CARTESIAN_POINT('Ctrl Pts',(-25.2767620004059,-14.4158522106919,
112.915397881831)) ;
#170726=CARTESIAN_POINT('Ctrl Pts',(-25.2029581580874,-14.4158522122129,
112.939628926871)) ;
#170727=CARTESIAN_POINT('Ctrl Pts',(-25.129154315769,-14.415852213734,112.963859971912)) ;
#170728=CARTESIAN_POINT('Ctrl Pts',(-25.1412442200855,-14.3505784504634,
113.000683869835)) ;
#170729=CARTESIAN_POINT('Ctrl Pts',(-25.0807965149899,-14.1680509006919,
112.781046396121)) ;
#170730=CARTESIAN_POINT('Ctrl Pts',(-25.0978599658701,-14.1154268840112,
112.833018914517)) ;
#170731=CARTESIAN_POINT('Ctrl Pts',(-25.1716638070098,-14.1154268771774,
112.808787865886)) ;
#170732=CARTESIAN_POINT('Ctrl Pts',(-25.2454676481495,-14.1154268703437,
112.784556817255)) ;
#170733=CARTESIAN_POINT('Ctrl Pts',(-25.2284041972694,-14.1680508870244,
112.732584298859)) ;
#170734=CARTESIAN_POINT('Ctrl Pts',(-25.2113407463893,-14.220674903705,
112.680611780463)) ;
#170735=CARTESIAN_POINT('Ctrl Pts',(-25.1375369052496,-14.2206749105388,
112.704842829094)) ;
#170736=CARTESIAN_POINT('Ctrl Pts',(-25.0637330641098,-14.2206749173726,
112.729073877726)) ;
#170737=CARTESIAN_POINT('Ctrl Pts',(-25.0807965149899,-14.1680509006919,
112.781046396121)) ;
#170738=CARTESIAN_POINT('Ctrl Pts',(-25.0381542588277,-13.9327426687889,
112.615783480832)) ;
#170739=CARTESIAN_POINT('Ctrl Pts',(-25.0589520128571,-13.8964722980425,
112.679130084212)) ;
#170740=CARTESIAN_POINT('Ctrl Pts',(-25.1327558537343,-13.8964722840852,
112.654899034782)) ;
#170741=CARTESIAN_POINT('Ctrl Pts',(-25.2065596946115,-13.896472270128,
112.630667985351)) ;
#170742=CARTESIAN_POINT('Ctrl Pts',(-25.1857619405821,-13.9327426408744,
112.56732138197)) ;
#170743=CARTESIAN_POINT('Ctrl Pts',(-25.1649641865527,-13.9690130116207,
112.50397477859)) ;
#170744=CARTESIAN_POINT('Ctrl Pts',(-25.0911603456755,-13.969013025578,
112.528205828021)) ;
#170745=CARTESIAN_POINT('Ctrl Pts',(-25.0173565047983,-13.9690130395352,
112.552436877452)) ;
#170746=CARTESIAN_POINT('Ctrl Pts',(-25.0381542588277,-13.9327426687889,
112.615783480832)) ;
#170747=CARTESIAN_POINT('Ctrl Pts',(-25.01675443207,-13.660519783253,112.515187651297)) ;
#170748=CARTESIAN_POINT('Ctrl Pts',(-25.0398093319936,-13.6432040400609,
112.58540915702)) ;
#170749=CARTESIAN_POINT('Ctrl Pts',(-25.1136131735509,-13.6432040175434,
112.56117810966)) ;
#170750=CARTESIAN_POINT('Ctrl Pts',(-25.1874170151081,-13.643203995026,
112.536947062301)) ;
#170751=CARTESIAN_POINT('Ctrl Pts',(-25.1643621151845,-13.6605197382181,
112.466725556578)) ;
#170752=CARTESIAN_POINT('Ctrl Pts',(-25.1413072152608,-13.6778354814103,
112.396504050855)) ;
#170753=CARTESIAN_POINT('Ctrl Pts',(-25.0675033737036,-13.6778355039277,
112.420735098215)) ;
#170754=CARTESIAN_POINT('Ctrl Pts',(-24.9936995321464,-13.6778355264452,
112.444966145574)) ;
#170755=CARTESIAN_POINT('Ctrl Pts',(-25.01675443207,-13.660519783253,112.515187651297)) ;
#170756=CARTESIAN_POINT('Ctrl Pts',(-25.0191170090691,-13.3693405601706,
112.486775760889)) ;
#170757=CARTESIAN_POINT('Ctrl Pts',(-25.0427772853919,-13.3723302960764,
112.558841145632)) ;
#170758=CARTESIAN_POINT('Ctrl Pts',(-25.1165811290148,-13.3723302632285,
112.534610104564)) ;
#170759=CARTESIAN_POINT('Ctrl Pts',(-25.1903849726377,-13.3723302303806,
112.510379063496)) ;
#170760=CARTESIAN_POINT('Ctrl Pts',(-25.1667246963149,-13.3693404944748,
112.438313678754)) ;
#170761=CARTESIAN_POINT('Ctrl Pts',(-25.143064419992,-13.3663507585691,
112.366248294011)) ;
#170762=CARTESIAN_POINT('Ctrl Pts',(-25.0692605763692,-13.366350791417,
112.390479335079)) ;
#170763=CARTESIAN_POINT('Ctrl Pts',(-24.9954567327463,-13.3663508242649,
112.414710376146)) ;
#170764=CARTESIAN_POINT('Ctrl Pts',(-25.0191170090691,-13.3693405601706,
112.486775760889)) ;
#170765=CARTESIAN_POINT('Ctrl Pts',(-25.0457464324794,-13.0834454323783,
112.532499973071)) ;
#170766=CARTESIAN_POINT('Ctrl Pts',(-25.0683137612795,-13.1064007088209,
112.601236416157)) ;
#170767=CARTESIAN_POINT('Ctrl Pts',(-25.1421176083962,-13.1064006698969,
112.577005385731)) ;
#170768=CARTESIAN_POINT('Ctrl Pts',(-25.2159214555129,-13.1064006309729,
112.552774355305)) ;
#170769=CARTESIAN_POINT('Ctrl Pts',(-25.1933541267128,-13.0834453545303,
112.484037912218)) ;
#170770=CARTESIAN_POINT('Ctrl Pts',(-25.1707867979127,-13.0604900780877,
112.415301469132)) ;
#170771=CARTESIAN_POINT('Ctrl Pts',(-25.096982950796,-13.0604901170117,
112.439532499558)) ;
#170772=CARTESIAN_POINT('Ctrl Pts',(-25.0231791036793,-13.0604901559357,
112.463763529984)) ;
#170773=CARTESIAN_POINT('Ctrl Pts',(-25.0457464324794,-13.0834454323783,
112.532499973071)) ;
#170774=CARTESIAN_POINT('Ctrl Pts',(-25.0953927384069,-12.8212149019315,
112.648303528621)) ;
#170775=CARTESIAN_POINT('Ctrl Pts',(-25.1152590939034,-12.8625120463937,
112.708813242983)) ;
#170776=CARTESIAN_POINT('Ctrl Pts',(-25.1890629454817,-12.8625120051449,
112.684582226146)) ;
#170777=CARTESIAN_POINT('Ctrl Pts',(-25.26286679706,-12.8625119638961,112.660351209309)) ;
#170778=CARTESIAN_POINT('Ctrl Pts',(-25.2430004415635,-12.8212148194339,
112.599841494947)) ;
#170779=CARTESIAN_POINT('Ctrl Pts',(-25.223134086067,-12.7799176749718,
112.539331780585)) ;
#170780=CARTESIAN_POINT('Ctrl Pts',(-25.1493302344887,-12.7799177162206,
112.563562797422)) ;
#170781=CARTESIAN_POINT('Ctrl Pts',(-25.0755263829104,-12.7799177574694,
112.587793814259)) ;
#170782=CARTESIAN_POINT('Ctrl Pts',(-25.0953927384069,-12.8212149019315,
112.648303528621)) ;
#170783=CARTESIAN_POINT('Ctrl Pts',(-25.1654351503245,-12.6012650290221,
112.826176017049)) ;
#170784=CARTESIAN_POINT('Ctrl Pts',(-25.1811738053442,-12.6579784616352,
112.874113421929)) ;
#170785=CARTESIAN_POINT('Ctrl Pts',(-25.2549776620693,-12.6579784230308,
112.849882420768)) ;
#170786=CARTESIAN_POINT('Ctrl Pts',(-25.3287815187944,-12.6579783844264,
112.825651419607)) ;
#170787=CARTESIAN_POINT('Ctrl Pts',(-25.3130428637748,-12.6012649518134,
112.777714014728)) ;
#170788=CARTESIAN_POINT('Ctrl Pts',(-25.2973042087551,-12.5445515192003,
112.729776609848)) ;
#170789=CARTESIAN_POINT('Ctrl Pts',(-25.22350035203,-12.5445515578047,112.754007611009)) ;
#170790=CARTESIAN_POINT('Ctrl Pts',(-25.1496964953049,-12.5445515964091,
112.77823861217)) ;
#170791=CARTESIAN_POINT('Ctrl Pts',(-25.1654351503245,-12.6012650290221,
112.826176017049)) ;
#170792=CARTESIAN_POINT('Ctrl Pts',(-25.2517211384274,-12.4396335453714,
113.053457862825)) ;
#170793=CARTESIAN_POINT('Ctrl Pts',(-25.2621934935828,-12.5077139487023,
113.085354968207)) ;
#170794=CARTESIAN_POINT('Ctrl Pts',(-25.3359973555674,-12.5077139189152,
113.061123983066)) ;
#170795=CARTESIAN_POINT('Ctrl Pts',(-25.4098012175519,-12.5077138891282,
113.036892997925)) ;
#170796=CARTESIAN_POINT('Ctrl Pts',(-25.3993288623965,-12.4396334857973,
113.004995892543)) ;
#170797=CARTESIAN_POINT('Ctrl Pts',(-25.3888565072411,-12.3715530824664,
112.973098787161)) ;
#170798=CARTESIAN_POINT('Ctrl Pts',(-25.3150526452566,-12.3715531122535,
112.997329772302)) ;
#170799=CARTESIAN_POINT('Ctrl Pts',(-25.241248783272,-12.3715531420405,
113.021560757443)) ;
#170800=CARTESIAN_POINT('Ctrl Pts',(-25.2517211384274,-12.4396335453714,
113.053457862825)) ;
#170801=CARTESIAN_POINT('Ctrl Pts',(-25.3485498372979,-12.3483868402897,
113.31290023935)) ;
#170802=CARTESIAN_POINT('Ctrl Pts',(-25.3530112255867,-12.4229364888091,
113.32648890968)) ;
#170803=CARTESIAN_POINT('Ctrl Pts',(-25.4268150918738,-12.4229364744478,
113.302257937644)) ;
#170804=CARTESIAN_POINT('Ctrl Pts',(-25.5006189581609,-12.4229364600866,
113.278026965608)) ;
#170805=CARTESIAN_POINT('Ctrl Pts',(-25.4961575698721,-12.3483868115671,
113.264438295278)) ;
#170806=CARTESIAN_POINT('Ctrl Pts',(-25.4916961815832,-12.2738371630477,
113.250849624949)) ;
#170807=CARTESIAN_POINT('Ctrl Pts',(-25.4178923152961,-12.2738371774089,
113.275080596985)) ;
#170808=CARTESIAN_POINT('Ctrl Pts',(-25.344088449009,-12.2738371917702,
113.299311569021)) ;
#170809=CARTESIAN_POINT('Ctrl Pts',(-25.3485498372979,-12.3483868402897,
113.31290023935)) ;
#170810=CARTESIAN_POINT('Ctrl Pts',(-25.4498951527532,-12.3339887574785,
113.58607265207)) ;
#170811=CARTESIAN_POINT('Ctrl Pts',(-25.4480221295144,-12.4096519181944,
113.580367727088)) ;
#170812=CARTESIAN_POINT('Ctrl Pts',(-25.5218259985408,-12.4096519246285,
113.556136763396)) ;
#170813=CARTESIAN_POINT('Ctrl Pts',(-25.5956298675672,-12.4096519310626,
113.531905799703)) ;
#170814=CARTESIAN_POINT('Ctrl Pts',(-25.597502890806,-12.3339887703467,
113.537610724685)) ;
#170815=CARTESIAN_POINT('Ctrl Pts',(-25.5993759140449,-12.2583256096307,
113.543315649667)) ;
#170816=CARTESIAN_POINT('Ctrl Pts',(-25.5255720450185,-12.2583256031966,
113.56754661336)) ;
#170817=CARTESIAN_POINT('Ctrl Pts',(-25.4517681759921,-12.2583255967626,
113.591777577052)) ;
#170818=CARTESIAN_POINT('Ctrl Pts',(-25.4498951527532,-12.3339887574785,
113.58607265207)) ;
#170819=CARTESIAN_POINT('Ctrl Pts',(-25.5487281653842,-12.3966946761742,
113.851770969332)) ;
#170820=CARTESIAN_POINT('Ctrl Pts',(-25.5406832866208,-12.4680894419109,
113.827267568358)) ;
#170821=CARTESIAN_POINT('Ctrl Pts',(-25.6144871558984,-12.4680894717794,
113.80303660543)) ;
#170822=CARTESIAN_POINT('Ctrl Pts',(-25.6882910251759,-12.4680895016479,
113.778805642503)) ;
#170823=CARTESIAN_POINT('Ctrl Pts',(-25.6963359039393,-12.3966947359113,
113.803309043476)) ;
#170824=CARTESIAN_POINT('Ctrl Pts',(-25.7043807827027,-12.3252999701746,
113.82781244445)) ;
#170825=CARTESIAN_POINT('Ctrl Pts',(-25.6305769134251,-12.3252999403061,
113.852043407378)) ;
#170826=CARTESIAN_POINT('Ctrl Pts',(-25.5567730441475,-12.3252999104375,
113.876274370305)) ;
#170827=CARTESIAN_POINT('Ctrl Pts',(-25.5487281653842,-12.3966946761742,
113.851770969332)) ;
#170828=CARTESIAN_POINT('Ctrl Pts',(-25.6400647909922,-12.5338429010278,
114.094279498921)) ;
#170829=CARTESIAN_POINT('Ctrl Pts',(-25.6263698061829,-12.5957672263305,
114.052566786713)) ;
#170830=CARTESIAN_POINT('Ctrl Pts',(-25.7001736738541,-12.5957672815326,
114.028335818893)) ;
#170831=CARTESIAN_POINT('Ctrl Pts',(-25.7739775415252,-12.5957673367347,
114.004104851072)) ;
#170832=CARTESIAN_POINT('Ctrl Pts',(-25.7876725263345,-12.533843011432,
114.04581756328)) ;
#170833=CARTESIAN_POINT('Ctrl Pts',(-25.8013675111438,-12.4719186861293,
114.087530275488)) ;
#170834=CARTESIAN_POINT('Ctrl Pts',(-25.7275636434727,-12.4719186309272,
114.111761243309)) ;
#170835=CARTESIAN_POINT('Ctrl Pts',(-25.6537597758015,-12.4719185757251,
114.135992211129)) ;
#170836=CARTESIAN_POINT('Ctrl Pts',(-25.6400647909922,-12.5338429010278,
114.094279498921)) ;
#170837=CARTESIAN_POINT('Ctrl Pts',(-25.7162744596763,-12.7326606979156,
114.291115372328)) ;
#170838=CARTESIAN_POINT('Ctrl Pts',(-25.6979689798409,-12.780794213553,
114.235359836244)) ;
#170839=CARTESIAN_POINT('Ctrl Pts',(-25.7717728428061,-12.7807942904156,
114.21112885409)) ;
#170840=CARTESIAN_POINT('Ctrl Pts',(-25.8455767057714,-12.7807943672782,
114.186897871936)) ;
#170841=CARTESIAN_POINT('Ctrl Pts',(-25.8638821856068,-12.7326608516408,
114.24265340802)) ;
#170842=CARTESIAN_POINT('Ctrl Pts',(-25.8821876654422,-12.6845273360034,
114.298408944103)) ;
#170843=CARTESIAN_POINT('Ctrl Pts',(-25.8083838024769,-12.6845272591408,
114.322639926257)) ;
#170844=CARTESIAN_POINT('Ctrl Pts',(-25.7345799395117,-12.6845271822782,
114.346870908411)) ;
#170845=CARTESIAN_POINT('Ctrl Pts',(-25.7162744596763,-12.7326606979156,
114.291115372328)) ;
#170846=CARTESIAN_POINT('Ctrl Pts',(-25.774069178511,-12.9811862243396,
114.431686787132)) ;
#170847=CARTESIAN_POINT('Ctrl Pts',(-25.7524356589921,-13.0120391573078,
114.365794579227)) ;
#170848=CARTESIAN_POINT('Ctrl Pts',(-25.8262395153994,-13.0120392516688,
114.341563577098)) ;
#170849=CARTESIAN_POINT('Ctrl Pts',(-25.9000433718066,-13.0120393460298,
114.31733257497)) ;
#170850=CARTESIAN_POINT('Ctrl Pts',(-25.9216768913254,-12.9811864130616,
114.383224782875)) ;
#170851=CARTESIAN_POINT('Ctrl Pts',(-25.9433104108443,-12.9503334800935,
114.44911699078)) ;
#170852=CARTESIAN_POINT('Ctrl Pts',(-25.8695065544371,-12.9503333857324,
114.473347992909)) ;
#170853=CARTESIAN_POINT('Ctrl Pts',(-25.7957026980299,-12.9503332913714,
114.497578995037)) ;
#170854=CARTESIAN_POINT('Ctrl Pts',(-25.774069178511,-12.9811862243396,
114.431686787132)) ;
#170855=CARTESIAN_POINT('Ctrl Pts',(-25.8095884902637,-13.260918115125,
114.504434976696)) ;
#170856=CARTESIAN_POINT('Ctrl Pts',(-25.7861766587316,-13.2722865612631,
114.433126317383)) ;
#170857=CARTESIAN_POINT('Ctrl Pts',(-25.8599805069678,-13.2722866661501,
114.408895290367)) ;
#170858=CARTESIAN_POINT('Ctrl Pts',(-25.9337843552041,-13.2722867710372,
114.384664263351)) ;
#170859=CARTESIAN_POINT('Ctrl Pts',(-25.9571961867363,-13.2609183248991,
114.455972922664)) ;
#170860=CARTESIAN_POINT('Ctrl Pts',(-25.9806080182684,-13.249549878761,
114.527281581977)) ;
#170861=CARTESIAN_POINT('Ctrl Pts',(-25.9068041700321,-13.249549773874,
114.551512608993)) ;
#170862=CARTESIAN_POINT('Ctrl Pts',(-25.8330003217958,-13.249549668987,
114.575743636009)) ;
#170863=CARTESIAN_POINT('Ctrl Pts',(-25.8095884902637,-13.260918115125,
114.504434976696)) ;
#170864=CARTESIAN_POINT('Ctrl Pts',(-25.8210548218699,-13.5531074788782,
114.503769138301)) ;
#170865=CARTESIAN_POINT('Ctrl Pts',(-25.7975442428386,-13.5440933427765,
114.432159710076)) ;
#170866=CARTESIAN_POINT('Ctrl Pts',(-25.8713480820835,-13.5440934499071,
114.407928655674)) ;
#170867=CARTESIAN_POINT('Ctrl Pts',(-25.9451519213283,-13.5440935570377,
114.383697601272)) ;
#170868=CARTESIAN_POINT('Ctrl Pts',(-25.9686625003595,-13.5531076931393,
114.455307029496)) ;
#170869=CARTESIAN_POINT('Ctrl Pts',(-25.9921730793908,-13.5621218292409,
114.526916457721)) ;
#170870=CARTESIAN_POINT('Ctrl Pts',(-25.9183692401459,-13.5621217221104,
114.551147512123)) ;
#170871=CARTESIAN_POINT('Ctrl Pts',(-25.8445654009011,-13.5621216149798,
114.575378566526)) ;
#170872=CARTESIAN_POINT('Ctrl Pts',(-25.8210548218699,-13.5531074788782,
114.503769138301)) ;
#170873=CARTESIAN_POINT('Ctrl Pts',(-25.808372018338,-13.8336246591284,
114.429796254132)) ;
#170874=CARTESIAN_POINT('Ctrl Pts',(-25.7864435705866,-13.8050124160848,
114.363005742518)) ;
#170875=CARTESIAN_POINT('Ctrl Pts',(-25.8602474010713,-13.805012516226,
114.338774661433)) ;
#170876=CARTESIAN_POINT('Ctrl Pts',(-25.934051231556,-13.8050126163672,
114.314543580349)) ;
#170877=CARTESIAN_POINT('Ctrl Pts',(-25.9559796793074,-13.8336248594109,
114.381334091963)) ;
#170878=CARTESIAN_POINT('Ctrl Pts',(-25.9779081270588,-13.8622371024545,
114.448124603577)) ;
#170879=CARTESIAN_POINT('Ctrl Pts',(-25.9041042965741,-13.8622370023133,
114.472355684662)) ;
#170880=CARTESIAN_POINT('Ctrl Pts',(-25.8303004660894,-13.8622369021721,
114.496586765746)) ;
#170881=CARTESIAN_POINT('Ctrl Pts',(-25.808372018338,-13.8336246591284,
114.429796254132)) ;
#170882=CARTESIAN_POINT('Ctrl Pts',(-25.7733597736157,-14.0853767704005,
114.287716933633)) ;
#170883=CARTESIAN_POINT('Ctrl Pts',(-25.7545765163614,-14.0391458019482,
114.230506164792)) ;
#170884=CARTESIAN_POINT('Ctrl Pts',(-25.8283803390502,-14.0391458872152,
114.206275059963)) ;
#170885=CARTESIAN_POINT('Ctrl Pts',(-25.9021841617389,-14.0391459724823,
114.182043955133)) ;
#170886=CARTESIAN_POINT('Ctrl Pts',(-25.9209674189931,-14.0853769409346,
114.239254723973)) ;
#170887=CARTESIAN_POINT('Ctrl Pts',(-25.9397506762473,-14.131607909387,
114.296465492813)) ;
#170888=CARTESIAN_POINT('Ctrl Pts',(-25.8659468535586,-14.1316078241199,
114.320696597643)) ;
#170889=CARTESIAN_POINT('Ctrl Pts',(-25.7921430308699,-14.1316077388528,
114.344927702473)) ;
#170890=CARTESIAN_POINT('Ctrl Pts',(-25.7733597736157,-14.0853767704005,
114.287716933633)) ;
#170891=CARTESIAN_POINT('Ctrl Pts',(-25.7186373576974,-14.2903978532202,
114.085351542632)) ;
#170892=CARTESIAN_POINT('Ctrl Pts',(-25.7043849358257,-14.2297838798409,
114.041940967275)) ;
#170893=CARTESIAN_POINT('Ctrl Pts',(-25.7781887527212,-14.2297839428811,
114.0177098448)) ;
#170894=CARTESIAN_POINT('Ctrl Pts',(-25.8519925696167,-14.2297840059213,
113.993478722325)) ;
#170895=CARTESIAN_POINT('Ctrl Pts',(-25.8662449914884,-14.2903979793006,
114.036889297682)) ;
#170896=CARTESIAN_POINT('Ctrl Pts',(-25.8804974133601,-14.3510119526798,
114.080299873038)) ;
#170897=CARTESIAN_POINT('Ctrl Pts',(-25.8066935964646,-14.3510118896396,
114.104530995513)) ;
#170898=CARTESIAN_POINT('Ctrl Pts',(-25.7328897795691,-14.3510118265994,
114.128762117988)) ;
#170899=CARTESIAN_POINT('Ctrl Pts',(-25.7186373576974,-14.2903978532202,
114.085351542632)) ;
#170900=CARTESIAN_POINT('Ctrl Pts',(-25.6501353567778,-14.430884933304,
113.841453445767)) ;
#170901=CARTESIAN_POINT('Ctrl Pts',(-25.6413738678537,-14.36037249955,113.814767366167)) ;
#170902=CARTESIAN_POINT('Ctrl Pts',(-25.7151776811438,-14.3603725370538,
113.790536232711)) ;
#170903=CARTESIAN_POINT('Ctrl Pts',(-25.7889814944339,-14.3603725745575,
113.766305099254)) ;
#170904=CARTESIAN_POINT('Ctrl Pts',(-25.797742983358,-14.4308850083114,
113.792991178854)) ;
#170905=CARTESIAN_POINT('Ctrl Pts',(-25.8065044722821,-14.5013974420654,
113.819677258453)) ;
#170906=CARTESIAN_POINT('Ctrl Pts',(-25.732700658992,-14.5013974045617,
113.84390839191)) ;
#170907=CARTESIAN_POINT('Ctrl Pts',(-25.6588968457018,-14.501397367058,
113.868139525366)) ;
#170908=CARTESIAN_POINT('Ctrl Pts',(-25.6501353567778,-14.430884933304,
113.841453445767)) ;
#170909=CARTESIAN_POINT('Ctrl Pts',(-25.5722582992266,-14.5000545452193,
113.568712686133)) ;
#170910=CARTESIAN_POINT('Ctrl Pts',(-25.5696561821823,-14.4246071586731,
113.560787059388)) ;
#170911=CARTESIAN_POINT('Ctrl Pts',(-25.643459994712,-14.4246071686467,
113.536555923616)) ;
#170912=CARTESIAN_POINT('Ctrl Pts',(-25.7172638072416,-14.4246071786203,
113.512324787843)) ;
#170913=CARTESIAN_POINT('Ctrl Pts',(-25.7198659242859,-14.5000545651665,
113.520250414587)) ;
#170914=CARTESIAN_POINT('Ctrl Pts',(-25.7224680413302,-14.5755019517128,
113.528176041332)) ;
#170915=CARTESIAN_POINT('Ctrl Pts',(-25.6486642288005,-14.5755019417391,
113.552407177104)) ;
#170916=CARTESIAN_POINT('Ctrl Pts',(-25.5748604162709,-14.5755019317655,
113.576638312877)) ;
#170917=CARTESIAN_POINT('Ctrl Pts',(-25.5722582992266,-14.5000545452193,
113.568712686133)) ;
#170918=CARTESIAN_POINT('Ctrl Pts',(-25.492125647743,-14.4915166284975,
113.289248825608)) ;
#170919=CARTESIAN_POINT('Ctrl Pts',(-25.4958466642941,-14.4165522893736,
113.300582443476)) ;
#170920=CARTESIAN_POINT('Ctrl Pts',(-25.5696504784892,-14.4165522733908,
113.276351312775)) ;
#170921=CARTESIAN_POINT('Ctrl Pts',(-25.6434542926842,-14.4165522574081,
113.252120182075)) ;
#170922=CARTESIAN_POINT('Ctrl Pts',(-25.6397332761331,-14.491516596532,
113.240786564208)) ;
#170923=CARTESIAN_POINT('Ctrl Pts',(-25.636012259582,-14.566480935656,113.229452946341)) ;
#170924=CARTESIAN_POINT('Ctrl Pts',(-25.5622084453869,-14.5664809516387,
113.253684077041)) ;
#170925=CARTESIAN_POINT('Ctrl Pts',(-25.4884046311919,-14.5664809676215,
113.277915207741)) ;
#170926=CARTESIAN_POINT('Ctrl Pts',(-25.492125647743,-14.4915166284975,
113.289248825608)) ;
#170927=CARTESIAN_POINT('Ctrl Pts',(-25.4155369746647,-14.4057133919849,
113.020376417355)) ;
#170928=CARTESIAN_POINT('Ctrl Pts',(-25.4253474075907,-14.3366264116548,
113.050257414847)) ;
#170929=CARTESIAN_POINT('Ctrl Pts',(-25.499151226059,-14.3366263740412,
113.026026297163)) ;
#170930=CARTESIAN_POINT('Ctrl Pts',(-25.5729550445272,-14.3366263364276,
113.001795179478)) ;
#170931=CARTESIAN_POINT('Ctrl Pts',(-25.5631446116012,-14.4057133167577,
112.971914181986)) ;
#170932=CARTESIAN_POINT('Ctrl Pts',(-25.5533341786752,-14.4748002970877,
112.942033184493)) ;
#170933=CARTESIAN_POINT('Ctrl Pts',(-25.479530360207,-14.4748003347014,
112.966264302178)) ;
#170934=CARTESIAN_POINT('Ctrl Pts',(-25.4057265417387,-14.474800372315,
112.990495419862)) ;
#170935=CARTESIAN_POINT('Ctrl Pts',(-25.4155369746647,-14.4057133919849,
113.020376417355)) ;
#170936=CARTESIAN_POINT('Ctrl Pts',(-25.3495488251331,-14.2496052022137,
112.783991163958)) ;
#170937=CARTESIAN_POINT('Ctrl Pts',(-25.3647136799672,-14.1913134689692,
112.83018086653)) ;
#170938=CARTESIAN_POINT('Ctrl Pts',(-25.4385175039201,-14.1913134155293,
112.805949765551)) ;
#170939=CARTESIAN_POINT('Ctrl Pts',(-25.512321327873,-14.1913133620894,
112.781718664571)) ;
#170940=CARTESIAN_POINT('Ctrl Pts',(-25.4971564730389,-14.2496050953339,
112.735528961999)) ;
#170941=CARTESIAN_POINT('Ctrl Pts',(-25.4819916182047,-14.3078968285784,
112.689339259427)) ;
#170942=CARTESIAN_POINT('Ctrl Pts',(-25.4081877942518,-14.3078968820183,
112.713570360406)) ;
#170943=CARTESIAN_POINT('Ctrl Pts',(-25.3343839702989,-14.3078969354582,
112.737801461386)) ;
#170944=CARTESIAN_POINT('Ctrl Pts',(-25.3495488251331,-14.2496052022137,
112.783991163958)) ;
#170945=CARTESIAN_POINT('Ctrl Pts',(-25.2990932542373,-14.0337448610519,
112.594839446854)) ;
#170946=CARTESIAN_POINT('Ctrl Pts',(-25.3185378072279,-13.9904362158164,
112.654064419341)) ;
#170947=CARTESIAN_POINT('Ctrl Pts',(-25.3923416376092,-13.9904361538178,
112.629833337941)) ;
#170948=CARTESIAN_POINT('Ctrl Pts',(-25.4661454679905,-13.9904360918192,
112.605602256542)) ;
#170949=CARTESIAN_POINT('Ctrl Pts',(-25.4467009149999,-14.0337447370547,
112.546377284055)) ;
#170950=CARTESIAN_POINT('Ctrl Pts',(-25.4272563620092,-14.0770533822902,
112.487152311568)) ;
#170951=CARTESIAN_POINT('Ctrl Pts',(-25.353452531628,-14.0770534442888,
112.511383392968)) ;
#170952=CARTESIAN_POINT('Ctrl Pts',(-25.2796487012467,-14.0770535062874,
112.535614474367)) ;
#170953=CARTESIAN_POINT('Ctrl Pts',(-25.2990932542373,-14.0337448610519,
112.594839446854)) ;
#170954=CARTESIAN_POINT('Ctrl Pts',(-25.2686792913389,-13.774289830103,
112.466801754916)) ;
#170955=CARTESIAN_POINT('Ctrl Pts',(-25.2910092781579,-13.7490307967716,
112.534815293139)) ;
#170956=CARTESIAN_POINT('Ctrl Pts',(-25.3648131149332,-13.7490307328435,
112.510584231214)) ;
#170957=CARTESIAN_POINT('Ctrl Pts',(-25.4386169517085,-13.7490306689154,
112.48635316929)) ;
#170958=CARTESIAN_POINT('Ctrl Pts',(-25.4162869648896,-13.7742897022469,
112.418339631067)) ;
#170959=CARTESIAN_POINT('Ctrl Pts',(-25.3939569780706,-13.7995487355784,
112.350326092844)) ;
#170960=CARTESIAN_POINT('Ctrl Pts',(-25.3201531412953,-13.7995487995064,
112.374557154769)) ;
#170961=CARTESIAN_POINT('Ctrl Pts',(-25.24634930452,-13.7995488634345,112.398788216693)) ;
#170962=CARTESIAN_POINT('Ctrl Pts',(-25.2686792913389,-13.774289830103,
112.466801754916)) ;
#170963=CARTESIAN_POINT('Ctrl Pts',(-25.2612500837139,-13.4875484100679,
112.408546039972)) ;
#170964=CARTESIAN_POINT('Ctrl Pts',(-25.284870016536,-13.4822714043299,
112.480488545396)) ;
#170965=CARTESIAN_POINT('Ctrl Pts',(-25.3586738590323,-13.4822713469427,
112.456257500897)) ;
#170966=CARTESIAN_POINT('Ctrl Pts',(-25.4324777015287,-13.4822712895556,
112.432026456398)) ;
#170967=CARTESIAN_POINT('Ctrl Pts',(-25.4088577687066,-13.4875482952936,
112.360083950974)) ;
#170968=CARTESIAN_POINT('Ctrl Pts',(-25.3852378358846,-13.4928253010316,
112.28814144555)) ;
#170969=CARTESIAN_POINT('Ctrl Pts',(-25.3114339933882,-13.4928253584187,
112.312372490049)) ;
#170970=CARTESIAN_POINT('Ctrl Pts',(-25.2376301508919,-13.4928254158059,
112.336603534548)) ;
#170971=CARTESIAN_POINT('Ctrl Pts',(-25.2612500837139,-13.4875484100679,
112.408546039972)) ;
#170972=CARTESIAN_POINT('Ctrl Pts',(-25.2779813826279,-13.1987144632943,
112.424247332912)) ;
#170973=CARTESIAN_POINT('Ctrl Pts',(-25.3011983723262,-13.2135962190273,
112.494962538468)) ;
#170974=CARTESIAN_POINT('Ctrl Pts',(-25.3750022191492,-13.2135961694435,
112.470731507147)) ;
#170975=CARTESIAN_POINT('Ctrl Pts',(-25.4488060659722,-13.2135961198597,
112.446500475826)) ;
#170976=CARTESIAN_POINT('Ctrl Pts',(-25.4255890762739,-13.1987143641267,
112.375785270271)) ;
#170977=CARTESIAN_POINT('Ctrl Pts',(-25.4023720865755,-13.1838326083937,
112.305070064715)) ;
#170978=CARTESIAN_POINT('Ctrl Pts',(-25.3285682397525,-13.1838326579775,
112.329301096036)) ;
#170979=CARTESIAN_POINT('Ctrl Pts',(-25.2547643929295,-13.1838327075613,
112.353532127357)) ;
#170980=CARTESIAN_POINT('Ctrl Pts',(-25.2779813826279,-13.1987144632943,
112.424247332912)) ;
#170981=CARTESIAN_POINT('Ctrl Pts',(-25.3186803797673,-12.9229602452279,
112.512616871207)) ;
#170982=CARTESIAN_POINT('Ctrl Pts',(-25.3398275683234,-12.9571183444642,
112.577027796252)) ;
#170983=CARTESIAN_POINT('Ctrl Pts',(-25.4136314177794,-12.9571183085152,
112.552796772951)) ;
#170984=CARTESIAN_POINT('Ctrl Pts',(-25.4874352672354,-12.9571182725662,
112.528565749649)) ;
#170985=CARTESIAN_POINT('Ctrl Pts',(-25.4662880786793,-12.9229601733299,
112.464154824605)) ;
#170986=CARTESIAN_POINT('Ctrl Pts',(-25.4451408901232,-12.8888020740936,
112.399743899561)) ;
#170987=CARTESIAN_POINT('Ctrl Pts',(-25.3713370406672,-12.8888021100426,
112.423974922862)) ;
#170988=CARTESIAN_POINT('Ctrl Pts',(-25.2975331912112,-12.8888021459916,
112.448205946163)) ;
#170989=CARTESIAN_POINT('Ctrl Pts',(-25.3186803797673,-12.9229602452279,
112.512616871207)) ;
#170990=CARTESIAN_POINT('Ctrl Pts',(-25.3810378795507,-12.6836290013039,
112.667065868669)) ;
#170991=CARTESIAN_POINT('Ctrl Pts',(-25.3985974186503,-12.7345497889164,
112.720549392164)) ;
#170992=CARTESIAN_POINT('Ctrl Pts',(-25.4724012689758,-12.7345497658022,
112.696318371512)) ;
#170993=CARTESIAN_POINT('Ctrl Pts',(-25.5462051193014,-12.734549742688,
112.672087350859)) ;
#170994=CARTESIAN_POINT('Ctrl Pts',(-25.5286455802018,-12.6836289550754,
112.618603827363)) ;
#170995=CARTESIAN_POINT('Ctrl Pts',(-25.5110860411021,-12.6327081674629,
112.565120303868)) ;
#170996=CARTESIAN_POINT('Ctrl Pts',(-25.4372821907766,-12.6327081905771,
112.58935132452)) ;
#170997=CARTESIAN_POINT('Ctrl Pts',(-25.3634783404511,-12.6327082136913,
112.613582345173)) ;
#170998=CARTESIAN_POINT('Ctrl Pts',(-25.3810378795507,-12.6836290013039,
112.667065868669)) ;
#170999=CARTESIAN_POINT('Ctrl Pts',(-25.4612408939245,-12.4971808863818,
112.875902607548)) ;
#171000=CARTESIAN_POINT('Ctrl Pts',(-25.4739605108467,-12.5611972883497,
112.914644508854)) ;
#171001=CARTESIAN_POINT('Ctrl Pts',(-25.5477643607026,-12.5611972760957,
112.890413486771)) ;
#171002=CARTESIAN_POINT('Ctrl Pts',(-25.6215682105584,-12.5611972638417,
112.866182464688)) ;
#171003=CARTESIAN_POINT('Ctrl Pts',(-25.6088485936362,-12.4971808618738,
112.827440563381)) ;
#171004=CARTESIAN_POINT('Ctrl Pts',(-25.596128976714,-12.4331644599059,
112.788698662075)) ;
#171005=CARTESIAN_POINT('Ctrl Pts',(-25.5223251268581,-12.4331644721599,
112.812929684158)) ;
#171006=CARTESIAN_POINT('Ctrl Pts',(-25.4485212770022,-12.4331644844139,
112.837160706241)) ;
#171007=CARTESIAN_POINT('Ctrl Pts',(-25.4612408939245,-12.4971808863818,
112.875902607548)) ;
#171008=CARTESIAN_POINT('Ctrl Pts',(-25.5540720154026,-12.3766482309411,
113.123307400288)) ;
#171009=CARTESIAN_POINT('Ctrl Pts',(-25.5610604027361,-12.4491772372763,
113.144592900868)) ;
#171010=CARTESIAN_POINT('Ctrl Pts',(-25.6348642513686,-12.4491772329469,
113.120361875059)) ;
#171011=CARTESIAN_POINT('Ctrl Pts',(-25.7086681000012,-12.4491772286174,
113.09613084925)) ;
#171012=CARTESIAN_POINT('Ctrl Pts',(-25.7016797126678,-12.3766482222823,
113.07484534867)) ;
#171013=CARTESIAN_POINT('Ctrl Pts',(-25.6946913253343,-12.3041192159472,
113.05355984809)) ;
#171014=CARTESIAN_POINT('Ctrl Pts',(-25.6208874767018,-12.3041192202766,
113.077790873899)) ;
#171015=CARTESIAN_POINT('Ctrl Pts',(-25.5470836280692,-12.304119224606,
113.102021899709)) ;
#171016=CARTESIAN_POINT('Ctrl Pts',(-25.5540720154026,-12.3766482309411,
113.123307400288)) ;
#171017=CARTESIAN_POINT('Ctrl Pts',(-25.6548077636956,-12.3303160635296,
113.394473806366)) ;
#171018=CARTESIAN_POINT('Ctrl Pts',(-25.6555106525389,-12.406190350598,
113.396614692547)) ;
#171019=CARTESIAN_POINT('Ctrl Pts',(-25.7293144987663,-12.4061903509704,
113.372383659411)) ;
#171020=CARTESIAN_POINT('Ctrl Pts',(-25.8031183449935,-12.4061903513427,
113.348152626276)) ;
#171021=CARTESIAN_POINT('Ctrl Pts',(-25.8024154561502,-12.3303160642744,
113.346011740096)) ;
#171022=CARTESIAN_POINT('Ctrl Pts',(-25.8017125673069,-12.254441777206,
113.343870853916)) ;
#171023=CARTESIAN_POINT('Ctrl Pts',(-25.7279087210796,-12.2544417768337,
113.368101887051)) ;
#171024=CARTESIAN_POINT('Ctrl Pts',(-25.6541048748523,-12.2544417764613,
113.392332920186)) ;
#171025=CARTESIAN_POINT('Ctrl Pts',(-25.6548077636956,-12.3303160635296,
113.394473806366)) ;
#171026=CARTESIAN_POINT('Ctrl Pts',(-25.7551087146694,-12.3620878034078,
113.664686262464)) ;
#171027=CARTESIAN_POINT('Ctrl Pts',(-25.7495393610477,-12.4358572257211,
113.647722910032)) ;
#171028=CARTESIAN_POINT('Ctrl Pts',(-25.8233432057987,-12.435857227174,
113.6234918724)) ;
#171029=CARTESIAN_POINT('Ctrl Pts',(-25.8971470505497,-12.4358572286269,
113.599260834769)) ;
#171030=CARTESIAN_POINT('Ctrl Pts',(-25.9027164041715,-12.3620878063136,
113.616224187201)) ;
#171031=CARTESIAN_POINT('Ctrl Pts',(-25.9082857577932,-12.2883183840004,
113.633187539633)) ;
#171032=CARTESIAN_POINT('Ctrl Pts',(-25.8344819130422,-12.2883183825475,
113.657418577265)) ;
#171033=CARTESIAN_POINT('Ctrl Pts',(-25.7606780682912,-12.2883183810946,
113.681649614896)) ;
#171034=CARTESIAN_POINT('Ctrl Pts',(-25.7551087146694,-12.3620878034078,
113.664686262464)) ;
#171035=CARTESIAN_POINT('Ctrl Pts',(-25.8501668503569,-12.4693107333451,
113.918717660534)) ;
#171036=CARTESIAN_POINT('Ctrl Pts',(-25.8386861551213,-12.5357038324563,
113.883749315246)) ;
#171037=CARTESIAN_POINT('Ctrl Pts',(-25.9124899984294,-12.5357038327128,
113.859518273219)) ;
#171038=CARTESIAN_POINT('Ctrl Pts',(-25.9862938417375,-12.5357038329694,
113.835287231193)) ;
#171039=CARTESIAN_POINT('Ctrl Pts',(-25.9977745369731,-12.4693107338582,
113.87025557648)) ;
#171040=CARTESIAN_POINT('Ctrl Pts',(-26.0092552322087,-12.402917634747,
113.905223921768)) ;
#171041=CARTESIAN_POINT('Ctrl Pts',(-25.9354513889006,-12.4029176344904,
113.929454963794)) ;
#171042=CARTESIAN_POINT('Ctrl Pts',(-25.8616475455925,-12.4029176342339,
113.953686005821)) ;
#171043=CARTESIAN_POINT('Ctrl Pts',(-25.8501668503569,-12.4693107333451,
113.918717660534)) ;
#171044=CARTESIAN_POINT('Ctrl Pts',(-25.9334232704776,-12.645191135036,
114.136742805122)) ;
#171045=CARTESIAN_POINT('Ctrl Pts',(-25.9168475822572,-12.6994019736038,
114.086255933222)) ;
#171046=CARTESIAN_POINT('Ctrl Pts',(-25.9906514249747,-12.6994019715653,
114.062024889397)) ;
#171047=CARTESIAN_POINT('Ctrl Pts',(-26.0644552676921,-12.6994019695268,
114.037793845571)) ;
#171048=CARTESIAN_POINT('Ctrl Pts',(-26.0810309559125,-12.6451911309591,
114.088280717471)) ;
#171049=CARTESIAN_POINT('Ctrl Pts',(-26.0976066441328,-12.5909802923914,
114.138767589371)) ;
#171050=CARTESIAN_POINT('Ctrl Pts',(-26.0238028014154,-12.5909802944298,
114.162998633196)) ;
#171051=CARTESIAN_POINT('Ctrl Pts',(-25.9499989586979,-12.5909802964683,
114.187229677022)) ;
#171052=CARTESIAN_POINT('Ctrl Pts',(-25.9334232704776,-12.645191135036,
114.136742805122)) ;
#171053=CARTESIAN_POINT('Ctrl Pts',(-25.999272047211,-12.8761323945115,
114.301835536524)) ;
#171054=CARTESIAN_POINT('Ctrl Pts',(-25.9788076787168,-12.9142969383445,
114.239504371944)) ;
#171055=CARTESIAN_POINT('Ctrl Pts',(-26.0526115216438,-12.9142969355883,
114.215273328757)) ;
#171056=CARTESIAN_POINT('Ctrl Pts',(-26.1264153645708,-12.9142969328321,
114.191042285569)) ;
#171057=CARTESIAN_POINT('Ctrl Pts',(-26.1468797330649,-12.8761323889991,
114.253373450149)) ;
#171058=CARTESIAN_POINT('Ctrl Pts',(-26.1673441015591,-12.8379678451661,
114.31570461473)) ;
#171059=CARTESIAN_POINT('Ctrl Pts',(-26.0935402586321,-12.8379678479223,
114.339935657917)) ;
#171060=CARTESIAN_POINT('Ctrl Pts',(-26.0197364157051,-12.8379678506785,
114.364166701105)) ;
#171061=CARTESIAN_POINT('Ctrl Pts',(-25.999272047211,-12.8761323945115,
114.301835536524)) ;
#171062=CARTESIAN_POINT('Ctrl Pts',(-26.0439639830932,-13.1443073603244,
114.40267311779)) ;
#171063=CARTESIAN_POINT('Ctrl Pts',(-26.0210791556646,-13.1638021990363,
114.332969625858)) ;
#171064=CARTESIAN_POINT('Ctrl Pts',(-26.0948829990038,-13.16380219707,114.308738583926)) ;
#171065=CARTESIAN_POINT('Ctrl Pts',(-26.1686868423429,-13.1638021951038,
114.284507541994)) ;
#171066=CARTESIAN_POINT('Ctrl Pts',(-26.1915716697714,-13.1443073563919,
114.354211033926)) ;
#171067=CARTESIAN_POINT('Ctrl Pts',(-26.2144564971999,-13.12481251768,114.423914525858)) ;
#171068=CARTESIAN_POINT('Ctrl Pts',(-26.1406526538608,-13.1248125196462,
114.44814556779)) ;
#171069=CARTESIAN_POINT('Ctrl Pts',(-26.0668488105217,-13.1248125216125,
114.472376609722)) ;
#171070=CARTESIAN_POINT('Ctrl Pts',(-26.0439639830932,-13.1443073603244,
114.40267311779)) ;
#171071=CARTESIAN_POINT('Ctrl Pts',(-26.0654214447628,-13.4354170804365,
114.432316659204)) ;
#171072=CARTESIAN_POINT('Ctrl Pts',(-26.0417435519583,-13.4346128293488,
114.360197618186)) ;
#171073=CARTESIAN_POINT('Ctrl Pts',(-26.1155473954861,-13.4346128319822,
114.335966576829)) ;
#171074=CARTESIAN_POINT('Ctrl Pts',(-26.189351239014,-13.4346128346157,
114.311735535472)) ;
#171075=CARTESIAN_POINT('Ctrl Pts',(-26.2130291318185,-13.4354170857033,
114.383854576489)) ;
#171076=CARTESIAN_POINT('Ctrl Pts',(-26.2367070246231,-13.436221336791,
114.455973617507)) ;
#171077=CARTESIAN_POINT('Ctrl Pts',(-26.1629031810952,-13.4362213341576,
114.480204658864)) ;
#171078=CARTESIAN_POINT('Ctrl Pts',(-26.0890993375674,-13.4362213315242,
114.504435700221)) ;
#171079=CARTESIAN_POINT('Ctrl Pts',(-26.0654214447628,-13.4354170804365,
114.432316659204)) ;
#171080=CARTESIAN_POINT('Ctrl Pts',(-26.0623510035417,-13.7221366616439,
114.38765243736)) ;
#171081=CARTESIAN_POINT('Ctrl Pts',(-26.0395838511607,-13.7013113003572,
114.318307364811)) ;
#171082=CARTESIAN_POINT('Ctrl Pts',(-26.1133876940889,-13.7013113073341,
114.294076321627)) ;
#171083=CARTESIAN_POINT('Ctrl Pts',(-26.1871915370171,-13.7013113143109,
114.269845278443)) ;
#171084=CARTESIAN_POINT('Ctrl Pts',(-26.2099586893981,-13.7221366755976,
114.339190350992)) ;
#171085=CARTESIAN_POINT('Ctrl Pts',(-26.2327258417792,-13.7429620368844,
114.408535423541)) ;
#171086=CARTESIAN_POINT('Ctrl Pts',(-26.158921998851,-13.7429620299075,
114.432766466724)) ;
#171087=CARTESIAN_POINT('Ctrl Pts',(-26.0851181559228,-13.7429620229307,
114.456997509908)) ;
#171088=CARTESIAN_POINT('Ctrl Pts',(-26.0623510035417,-13.7221366616439,
114.38765243736)) ;
#171089=CARTESIAN_POINT('Ctrl Pts',(-26.0360612678888,-13.9882040306806,
114.272122330666)) ;
#171090=CARTESIAN_POINT('Ctrl Pts',(-26.0158303614321,-13.948770536174,
114.210502254101)) ;
#171091=CARTESIAN_POINT('Ctrl Pts',(-26.0896342028091,-13.9487705477941,
114.186271206193)) ;
#171092=CARTESIAN_POINT('Ctrl Pts',(-26.1634380441861,-13.9487705594142,
114.162040158284)) ;
#171093=CARTESIAN_POINT('Ctrl Pts',(-26.1836689506428,-13.9882040539209,
114.223660234849)) ;
#171094=CARTESIAN_POINT('Ctrl Pts',(-26.2038998570996,-14.0276375484275,
114.285280311414)) ;
#171095=CARTESIAN_POINT('Ctrl Pts',(-26.1300960157226,-14.0276375368073,
114.309511359322)) ;
#171096=CARTESIAN_POINT('Ctrl Pts',(-26.0562921743456,-14.0276375251872,
114.333742407231)) ;
#171097=CARTESIAN_POINT('Ctrl Pts',(-26.0360612678888,-13.9882040306806,
114.272122330666)) ;
#171098=CARTESIAN_POINT('Ctrl Pts',(-25.9891697623435,-14.2132831582582,
114.093901493958)) ;
#171099=CARTESIAN_POINT('Ctrl Pts',(-25.9729161073915,-14.1580769970448,
114.044395483879)) ;
#171100=CARTESIAN_POINT('Ctrl Pts',(-26.0467199463987,-14.1580770113055,
114.020164428752)) ;
#171101=CARTESIAN_POINT('Ctrl Pts',(-26.1205237854058,-14.1580770255661,
113.995933373626)) ;
#171102=CARTESIAN_POINT('Ctrl Pts',(-26.1367774403579,-14.2132831867795,
114.045439383705)) ;
#171103=CARTESIAN_POINT('Ctrl Pts',(-26.1530310953099,-14.2684893479928,
114.094945393784)) ;
#171104=CARTESIAN_POINT('Ctrl Pts',(-26.0792272563027,-14.2684893337322,
114.119176448911)) ;
#171105=CARTESIAN_POINT('Ctrl Pts',(-26.0054234172956,-14.2684893194715,
114.143407504037)) ;
#171106=CARTESIAN_POINT('Ctrl Pts',(-25.9891697623435,-14.2132831582582,
114.093901493958)) ;
#171107=CARTESIAN_POINT('Ctrl Pts',(-25.9251466069735,-14.3825130038358,
113.863210711069)) ;
#171108=CARTESIAN_POINT('Ctrl Pts',(-25.9140780038205,-14.3154103550948,
113.829497532359)) ;
#171109=CARTESIAN_POINT('Ctrl Pts',(-25.9878818390175,-14.3154103696642,
113.805266465627)) ;
#171110=CARTESIAN_POINT('Ctrl Pts',(-26.0616856742145,-14.3154103842335,
113.781035398895)) ;
#171111=CARTESIAN_POINT('Ctrl Pts',(-26.0727542773675,-14.3825130329745,
113.814748577605)) ;
#171112=CARTESIAN_POINT('Ctrl Pts',(-26.0838228805205,-14.4496156817154,
113.848461756315)) ;
#171113=CARTESIAN_POINT('Ctrl Pts',(-26.0100190453235,-14.4496156671461,
113.872692823047)) ;
#171114=CARTESIAN_POINT('Ctrl Pts',(-25.9362152101265,-14.4496156525767,
113.896923889778)) ;
#171115=CARTESIAN_POINT('Ctrl Pts',(-25.9251466069735,-14.3825130038358,
113.863210711069)) ;
#171116=CARTESIAN_POINT('Ctrl Pts',(-25.8506582051535,-14.4810713491466,
113.601065674823)) ;
#171117=CARTESIAN_POINT('Ctrl Pts',(-25.8455042079974,-14.4069908889082,
113.585367431789)) ;
#171118=CARTESIAN_POINT('Ctrl Pts',(-25.9193080402583,-14.4069908973545,
113.561136356115)) ;
#171119=CARTESIAN_POINT('Ctrl Pts',(-25.9931118725193,-14.4069909058008,
113.53690528044)) ;
#171120=CARTESIAN_POINT('Ctrl Pts',(-25.9982658696754,-14.4810713660392,
113.552603523474)) ;
#171121=CARTESIAN_POINT('Ctrl Pts',(-26.0034198668315,-14.5551518262776,
113.568301766508)) ;
#171122=CARTESIAN_POINT('Ctrl Pts',(-25.9296160345705,-14.5551518178313,
113.592532842183)) ;
#171123=CARTESIAN_POINT('Ctrl Pts',(-25.8558122023096,-14.555151809385,
113.616763917857)) ;
#171124=CARTESIAN_POINT('Ctrl Pts',(-25.8506582051535,-14.4810713491466,
113.601065674823)) ;
#171125=CARTESIAN_POINT('Ctrl Pts',(-25.770453573245,-14.5044054817918,
113.321227426534)) ;
#171126=CARTESIAN_POINT('Ctrl Pts',(-25.7716275560046,-14.4285885279282,
113.324803189491)) ;
#171127=CARTESIAN_POINT('Ctrl Pts',(-25.8454313850184,-14.4285885262166,
113.300572103926)) ;
#171128=CARTESIAN_POINT('Ctrl Pts',(-25.9192352140321,-14.4285885245051,
113.276341018362)) ;
#171129=CARTESIAN_POINT('Ctrl Pts',(-25.9180612312726,-14.5044054783686,
113.272765255405)) ;
#171130=CARTESIAN_POINT('Ctrl Pts',(-25.9168872485131,-14.5802224322322,
113.269189492448)) ;
#171131=CARTESIAN_POINT('Ctrl Pts',(-25.8430834194993,-14.5802224339438,
113.293420578013)) ;
#171132=CARTESIAN_POINT('Ctrl Pts',(-25.7692795904855,-14.5802224356554,
113.317651663578)) ;
#171133=CARTESIAN_POINT('Ctrl Pts',(-25.770453573245,-14.5044054817918,
113.321227426534)) ;
#171134=CARTESIAN_POINT('Ctrl Pts',(-25.6917906589482,-14.4496129795719,
113.046187296342)) ;
#171135=CARTESIAN_POINT('Ctrl Pts',(-25.6991919532336,-14.377512086332,
113.068730445599)) ;
#171136=CARTESIAN_POINT('Ctrl Pts',(-25.7729957803867,-14.3775120696296,
113.044499354366)) ;
#171137=CARTESIAN_POINT('Ctrl Pts',(-25.8467996075397,-14.3775120529272,
113.020268263134)) ;
#171138=CARTESIAN_POINT('Ctrl Pts',(-25.8393983132543,-14.449612946167,
112.997725113878)) ;
#171139=CARTESIAN_POINT('Ctrl Pts',(-25.8319970189689,-14.5217138394069,
112.975181964621)) ;
#171140=CARTESIAN_POINT('Ctrl Pts',(-25.7581931918158,-14.5217138561093,
112.999413055854)) ;
#171141=CARTESIAN_POINT('Ctrl Pts',(-25.6843893646628,-14.5217138728117,
113.023644147086)) ;
#171142=CARTESIAN_POINT('Ctrl Pts',(-25.6917906589482,-14.4496129795719,
113.046187296342)) ;
#171143=CARTESIAN_POINT('Ctrl Pts',(-25.6207924323353,-14.3209948065222,
112.79446435437)) ;
#171144=CARTESIAN_POINT('Ctrl Pts',(-25.6338954260901,-14.2577695417982,
112.83437396041)) ;
#171145=CARTESIAN_POINT('Ctrl Pts',(-25.7076992529809,-14.257769507085,
112.810142868379)) ;
#171146=CARTESIAN_POINT('Ctrl Pts',(-25.7815030798717,-14.2577694723718,
112.785911776348)) ;
#171147=CARTESIAN_POINT('Ctrl Pts',(-25.7684000861169,-14.3209947370958,
112.746002170308)) ;
#171148=CARTESIAN_POINT('Ctrl Pts',(-25.7552970923621,-14.3842200018198,
112.706092564267)) ;
#171149=CARTESIAN_POINT('Ctrl Pts',(-25.6814932654713,-14.384220036533,
112.730323656298)) ;
#171150=CARTESIAN_POINT('Ctrl Pts',(-25.6076894385805,-14.3842200712462,
112.754554748329)) ;
#171151=CARTESIAN_POINT('Ctrl Pts',(-25.6207924323353,-14.3209948065222,
112.79446435437)) ;
#171152=CARTESIAN_POINT('Ctrl Pts',(-25.5633709290415,-14.1276267553148,
112.584095959637)) ;
#171153=CARTESIAN_POINT('Ctrl Pts',(-25.5812359055684,-14.0778104825488,
112.638509797017)) ;
#171154=CARTESIAN_POINT('Ctrl Pts',(-25.6550397342676,-14.077810428769,
112.614278710494)) ;
#171155=CARTESIAN_POINT('Ctrl Pts',(-25.7288435629669,-14.0778103749893,
112.590047623971)) ;
#171156=CARTESIAN_POINT('Ctrl Pts',(-25.71097858644,-14.1276266477552,112.535633786592)) ;
#171157=CARTESIAN_POINT('Ctrl Pts',(-25.6931136099132,-14.1774429205212,
112.481219949212)) ;
#171158=CARTESIAN_POINT('Ctrl Pts',(-25.6193097812139,-14.177442974301,
112.505451035735)) ;
#171159=CARTESIAN_POINT('Ctrl Pts',(-25.5455059525147,-14.1774430280807,
112.529682122257)) ;
#171160=CARTESIAN_POINT('Ctrl Pts',(-25.5633709290415,-14.1276267553148,
112.584095959637)) ;
#171161=CARTESIAN_POINT('Ctrl Pts',(-25.5243599004901,-13.88341485216,112.429801042865)) ;
#171162=CARTESIAN_POINT('Ctrl Pts',(-25.5457084250049,-13.8505765249219,
112.494825205497)) ;
#171163=CARTESIAN_POINT('Ctrl Pts',(-25.6195122576543,-13.8505764535514,
112.470594131005)) ;
#171164=CARTESIAN_POINT('Ctrl Pts',(-25.6933160903036,-13.850576382181,
112.446363056514)) ;
#171165=CARTESIAN_POINT('Ctrl Pts',(-25.6719675657889,-13.8834147094192,
112.381338893882)) ;
#171166=CARTESIAN_POINT('Ctrl Pts',(-25.6506190412741,-13.9162530366573,
112.31631473125)) ;
#171167=CARTESIAN_POINT('Ctrl Pts',(-25.5768152086248,-13.9162531080278,
112.340545805741)) ;
#171168=CARTESIAN_POINT('Ctrl Pts',(-25.5030113759754,-13.9162531793982,
112.364776880233)) ;
#171169=CARTESIAN_POINT('Ctrl Pts',(-25.5243599004901,-13.88341485216,112.429801042865)) ;
#171170=CARTESIAN_POINT('Ctrl Pts',(-25.5073970747293,-13.605636693064,
112.342636129513)) ;
#171171=CARTESIAN_POINT('Ctrl Pts',(-25.5306954589167,-13.5921442428259,
112.413599250237)) ;
#171172=CARTESIAN_POINT('Ctrl Pts',(-25.6044992975363,-13.5921441578331,
112.38936819393)) ;
#171173=CARTESIAN_POINT('Ctrl Pts',(-25.6783031361559,-13.5921440728403,
112.365137137623)) ;
#171174=CARTESIAN_POINT('Ctrl Pts',(-25.6550047519685,-13.6056365230784,
112.294174016899)) ;
#171175=CARTESIAN_POINT('Ctrl Pts',(-25.631706367781,-13.6191289733166,
112.223210896175)) ;
#171176=CARTESIAN_POINT('Ctrl Pts',(-25.5579025291614,-13.6191290583094,
112.247441952482)) ;
#171177=CARTESIAN_POINT('Ctrl Pts',(-25.4840986905419,-13.6191291433021,
112.271673008789)) ;
#171178=CARTESIAN_POINT('Ctrl Pts',(-25.5073970747293,-13.605636693064,
112.342636129513)) ;
#171179=CARTESIAN_POINT('Ctrl Pts',(-25.5142052747166,-13.3159385103922,
112.328067762604)) ;
#171180=CARTESIAN_POINT('Ctrl Pts',(-25.5377925942813,-13.3226522577716,
112.399910933968)) ;
#171181=CARTESIAN_POINT('Ctrl Pts',(-25.6115964402047,-13.3226521665054,
112.375679899907)) ;
#171182=CARTESIAN_POINT('Ctrl Pts',(-25.685400286128,-13.3226520752392,
112.351448865846)) ;
#171183=CARTESIAN_POINT('Ctrl Pts',(-25.6618129665633,-13.3159383278597,
112.279605694482)) ;
#171184=CARTESIAN_POINT('Ctrl Pts',(-25.6382256469986,-13.3092245804803,
112.207762523118)) ;
#171185=CARTESIAN_POINT('Ctrl Pts',(-25.5644218010753,-13.3092246717465,
112.231993557178)) ;
#171186=CARTESIAN_POINT('Ctrl Pts',(-25.4906179551519,-13.3092247630127,
112.256224591239)) ;
#171187=CARTESIAN_POINT('Ctrl Pts',(-25.5142052747166,-13.3159385103922,
112.328067762604)) ;
#171188=CARTESIAN_POINT('Ctrl Pts',(-25.5456617971205,-13.0300093756574,
112.388107483979)) ;
#171189=CARTESIAN_POINT('Ctrl Pts',(-25.5678278490325,-13.0566953178852,
112.45562170353)) ;
#171190=CARTESIAN_POINT('Ctrl Pts',(-25.6416317032956,-13.0566952256386,
112.43139069487)) ;
#171191=CARTESIAN_POINT('Ctrl Pts',(-25.7154355575587,-13.0566951333921,
112.407159686211)) ;
#171192=CARTESIAN_POINT('Ctrl Pts',(-25.6932695056467,-13.0300091911643,
112.33964546666)) ;
#171193=CARTESIAN_POINT('Ctrl Pts',(-25.6711034537346,-13.0033232489365,
112.27213124711)) ;
#171194=CARTESIAN_POINT('Ctrl Pts',(-25.5972995994715,-13.003323341183,
112.296362255769)) ;
#171195=CARTESIAN_POINT('Ctrl Pts',(-25.5234957452084,-13.0033234334296,
112.320593264428)) ;
#171196=CARTESIAN_POINT('Ctrl Pts',(-25.5456617971205,-13.0300093756574,
112.388107483979)) ;
#171197=CARTESIAN_POINT('Ctrl Pts',(-25.5990739293158,-12.7764992730081,
112.515654295035)) ;
#171198=CARTESIAN_POINT('Ctrl Pts',(-25.6182700989793,-12.820923286975,
112.574122732496)) ;
#171199=CARTESIAN_POINT('Ctrl Pts',(-25.6920739609603,-12.8209232050731,
112.549891747345)) ;
#171200=CARTESIAN_POINT('Ctrl Pts',(-25.7658778229413,-12.8209231231712,
112.525660762193)) ;
#171201=CARTESIAN_POINT('Ctrl Pts',(-25.7466816532778,-12.7764991092043,
112.467192324731)) ;
#171202=CARTESIAN_POINT('Ctrl Pts',(-25.7274854836142,-12.7320750952375,
112.40872388727)) ;
#171203=CARTESIAN_POINT('Ctrl Pts',(-25.6536816216332,-12.7320751771394,
112.432954872422)) ;
#171204=CARTESIAN_POINT('Ctrl Pts',(-25.5798777596522,-12.7320752590413,
112.457185857574)) ;
#171205=CARTESIAN_POINT('Ctrl Pts',(-25.5990739293158,-12.7764992730081,
112.515654295035)) ;
#171206=CARTESIAN_POINT('Ctrl Pts',(-25.6727778832843,-12.5655360581605,
112.704525516889)) ;
#171207=CARTESIAN_POINT('Ctrl Pts',(-25.6875936661384,-12.6247539701097,
112.749652002979)) ;
#171208=CARTESIAN_POINT('Ctrl Pts',(-25.7613975352215,-12.6247539044987,
112.725421039459)) ;
#171209=CARTESIAN_POINT('Ctrl Pts',(-25.8352014043047,-12.6247538388877,
112.701190075939)) ;
#171210=CARTESIAN_POINT('Ctrl Pts',(-25.8203856214506,-12.5655359269385,
112.656063589849)) ;
#171211=CARTESIAN_POINT('Ctrl Pts',(-25.8055698385965,-12.5063180149893,
112.610937103759)) ;
#171212=CARTESIAN_POINT('Ctrl Pts',(-25.7317659695133,-12.5063180806004,
112.635168067279)) ;
#171213=CARTESIAN_POINT('Ctrl Pts',(-25.6579621004302,-12.5063181462114,
112.659399030798)) ;
#171214=CARTESIAN_POINT('Ctrl Pts',(-25.6727778832843,-12.5655360581605,
112.704525516889)) ;
#171215=CARTESIAN_POINT('Ctrl Pts',(-25.7612652883096,-12.4169761529621,
112.938629023383)) ;
#171216=CARTESIAN_POINT('Ctrl Pts',(-25.7706577740588,-12.4866530449287,
112.967237021576)) ;
#171217=CARTESIAN_POINT('Ctrl Pts',(-25.8444616482445,-12.4866530028469,
112.943006073598)) ;
#171218=CARTESIAN_POINT('Ctrl Pts',(-25.9182655224302,-12.4866529607651,
112.91877512562)) ;
#171219=CARTESIAN_POINT('Ctrl Pts',(-25.908873036681,-12.4169760687985,
112.890167127427)) ;
#171220=CARTESIAN_POINT('Ctrl Pts',(-25.8994805509318,-12.3472991768318,
112.861559129234)) ;
#171221=CARTESIAN_POINT('Ctrl Pts',(-25.8256766767461,-12.3472992189136,
112.885790077212)) ;
#171222=CARTESIAN_POINT('Ctrl Pts',(-25.7518728025604,-12.3472992609954,
112.91002102519)) ;
#171223=CARTESIAN_POINT('Ctrl Pts',(-25.7612652883096,-12.4169761529621,
112.938629023383)) ;
#171224=CARTESIAN_POINT('Ctrl Pts',(-25.8595188377888,-12.339692635442,
113.20236799913)) ;
#171225=CARTESIAN_POINT('Ctrl Pts',(-25.8628006300689,-12.4148681964576,
113.212363810995)) ;
#171226=CARTESIAN_POINT('Ctrl Pts',(-25.9366045069881,-12.4148681820189,
113.188132871343)) ;
#171227=CARTESIAN_POINT('Ctrl Pts',(-26.0104083839073,-12.4148681675802,
113.16390193169)) ;
#171228=CARTESIAN_POINT('Ctrl Pts',(-26.0071265916272,-12.3396926065646,
113.153906119825)) ;
#171229=CARTESIAN_POINT('Ctrl Pts',(-26.0038447993471,-12.264517045549,
113.14391030796)) ;
#171230=CARTESIAN_POINT('Ctrl Pts',(-25.9300409224279,-12.2645170599877,
113.168141247613)) ;
#171231=CARTESIAN_POINT('Ctrl Pts',(-25.8562370455087,-12.2645170744263,
113.192372187265)) ;
#171232=CARTESIAN_POINT('Ctrl Pts',(-25.8595188377888,-12.339692635442,
113.20236799913)) ;
#171233=CARTESIAN_POINT('Ctrl Pts',(-25.9607682026483,-12.3399218128255,
113.475325729361)) ;
#171234=CARTESIAN_POINT('Ctrl Pts',(-25.9577191084769,-12.4151926619622,
113.466038682576)) ;
#171235=CARTESIAN_POINT('Ctrl Pts',(-26.0315229853345,-12.4151926765907,
113.441807742736)) ;
#171236=CARTESIAN_POINT('Ctrl Pts',(-26.1053268621922,-12.4151926912192,
113.417576802896)) ;
#171237=CARTESIAN_POINT('Ctrl Pts',(-26.1083759563636,-12.3399218420826,
113.426863849681)) ;
#171238=CARTESIAN_POINT('Ctrl Pts',(-26.1114250505351,-12.2646509929459,
113.436150896466)) ;
#171239=CARTESIAN_POINT('Ctrl Pts',(-26.0376211736774,-12.2646509783174,
113.460381836306)) ;
#171240=CARTESIAN_POINT('Ctrl Pts',(-25.9638172968198,-12.2646509636889,
113.484612776146)) ;
#171241=CARTESIAN_POINT('Ctrl Pts',(-25.9607682026483,-12.3399218128255,
113.475325729361)) ;
#171242=CARTESIAN_POINT('Ctrl Pts',(-26.0587509812645,-12.4170982893213,
113.738337027537)) ;
#171243=CARTESIAN_POINT('Ctrl Pts',(-26.0495896106153,-12.4870926783877,
113.710432972791)) ;
#171244=CARTESIAN_POINT('Ctrl Pts',(-26.1233934847273,-12.4870927205449,
113.686202024588)) ;
#171245=CARTESIAN_POINT('Ctrl Pts',(-26.1971973588393,-12.4870927627021,
113.661971076385)) ;
#171246=CARTESIAN_POINT('Ctrl Pts',(-26.2063587294884,-12.4170983736357,
113.689875131132)) ;
#171247=CARTESIAN_POINT('Ctrl Pts',(-26.2155201001376,-12.3471039845693,
113.717779185878)) ;
#171248=CARTESIAN_POINT('Ctrl Pts',(-26.1417162260256,-12.3471039424121,
113.742010134081)) ;
#171249=CARTESIAN_POINT('Ctrl Pts',(-26.0679123519136,-12.3471039002549,
113.766241082284)) ;
#171250=CARTESIAN_POINT('Ctrl Pts',(-26.0587509812645,-12.4170982893213,
113.738337027537)) ;
#171251=CARTESIAN_POINT('Ctrl Pts',(-26.1473630413061,-12.5661915214183,
113.972745351393)) ;
#171252=CARTESIAN_POINT('Ctrl Pts',(-26.1327357424787,-12.6258811352282,
113.928192961293)) ;
#171253=CARTESIAN_POINT('Ctrl Pts',(-26.2065396113906,-12.6258812005672,
113.903961997252)) ;
#171254=CARTESIAN_POINT('Ctrl Pts',(-26.2803434803025,-12.6258812659061,
113.879731033211)) ;
#171255=CARTESIAN_POINT('Ctrl Pts',(-26.2949707791298,-12.5661916520963,
113.92428342331)) ;
#171256=CARTESIAN_POINT('Ctrl Pts',(-26.3095980779572,-12.5065020382865,
113.968835813409)) ;
#171257=CARTESIAN_POINT('Ctrl Pts',(-26.2357942090453,-12.5065019729475,
113.993066777451)) ;
#171258=CARTESIAN_POINT('Ctrl Pts',(-26.1619903401334,-12.5065019076085,
114.017297741492)) ;
#171259=CARTESIAN_POINT('Ctrl Pts',(-26.1473630413061,-12.5661915214183,
113.972745351393)) ;
#171260=CARTESIAN_POINT('Ctrl Pts',(-26.2207601261338,-12.7760910985915,
114.160853377573)) ;
#171261=CARTESIAN_POINT('Ctrl Pts',(-26.2017200658351,-12.8212153371298,
114.102860427963)) ;
#171262=CARTESIAN_POINT('Ctrl Pts',(-26.2755239277867,-12.8212154191497,
114.078629442721)) ;
#171263=CARTESIAN_POINT('Ctrl Pts',(-26.3493277897383,-12.8212155011696,
114.05439845748)) ;
#171264=CARTESIAN_POINT('Ctrl Pts',(-26.368367850037,-12.7760912626314,
114.11239140709)) ;
#171265=CARTESIAN_POINT('Ctrl Pts',(-26.3874079103356,-12.7309670240931,
114.1703843567)) ;
#171266=CARTESIAN_POINT('Ctrl Pts',(-26.3136040483841,-12.7309669420732,
114.194615341941)) ;
#171267=CARTESIAN_POINT('Ctrl Pts',(-26.2398001864325,-12.7309668600532,
114.218846327183)) ;
#171268=CARTESIAN_POINT('Ctrl Pts',(-26.2207601261338,-12.7760910985915,
114.160853377573)) ;
#171269=CARTESIAN_POINT('Ctrl Pts',(-26.274697438766,-13.0327329322163,
114.289584630443)) ;
#171270=CARTESIAN_POINT('Ctrl Pts',(-26.2525986608536,-13.0600070239695,
114.222275320409)) ;
#171271=CARTESIAN_POINT('Ctrl Pts',(-26.3264025147417,-13.0600071142797,
114.198044310608)) ;
#171272=CARTESIAN_POINT('Ctrl Pts',(-26.4002063686298,-13.0600072045899,
114.173813300806)) ;
#171273=CARTESIAN_POINT('Ctrl Pts',(-26.4223051465423,-13.0327331128366,
114.241122610841)) ;
#171274=CARTESIAN_POINT('Ctrl Pts',(-26.4444039244547,-13.0054590210833,
114.308431920875)) ;
#171275=CARTESIAN_POINT('Ctrl Pts',(-26.3706000705666,-13.0054589307732,
114.332662930677)) ;
#171276=CARTESIAN_POINT('Ctrl Pts',(-26.2967962166784,-13.005458840463,
114.356893940478)) ;
#171277=CARTESIAN_POINT('Ctrl Pts',(-26.274697438766,-13.0327329322163,
114.289584630443)) ;
#171278=CARTESIAN_POINT('Ctrl Pts',(-26.3056984325726,-13.3169814944794,
114.34847609993)) ;
#171279=CARTESIAN_POINT('Ctrl Pts',(-26.2821371567087,-13.3244510016564,
114.276712256991)) ;
#171280=CARTESIAN_POINT('Ctrl Pts',(-26.3559410025772,-13.3244510916003,
114.252481222763)) ;
#171281=CARTESIAN_POINT('Ctrl Pts',(-26.4297448484457,-13.3244511815443,
114.228250188535)) ;
#171282=CARTESIAN_POINT('Ctrl Pts',(-26.4533061243096,-13.3169816743673,
114.300014031474)) ;
#171283=CARTESIAN_POINT('Ctrl Pts',(-26.4768674001734,-13.3095121671903,
114.371777874413)) ;
#171284=CARTESIAN_POINT('Ctrl Pts',(-26.4030635543049,-13.3095120772463,
114.396008908641)) ;
#171285=CARTESIAN_POINT('Ctrl Pts',(-26.3292597084365,-13.3095119873024,
114.420239942869)) ;
#171286=CARTESIAN_POINT('Ctrl Pts',(-26.3056984325726,-13.3169814944794,
114.34847609993)) ;
#171287=CARTESIAN_POINT('Ctrl Pts',(-26.3125024381578,-13.6065319682423,
114.333907323218)) ;
#171288=CARTESIAN_POINT('Ctrl Pts',(-26.2891610497531,-13.593796615994,
114.262813221903)) ;
#171289=CARTESIAN_POINT('Ctrl Pts',(-26.3629648883744,-13.5937966997554,
114.238582165601)) ;
#171290=CARTESIAN_POINT('Ctrl Pts',(-26.4367687269956,-13.5937967835168,
114.214351109299)) ;
#171291=CARTESIAN_POINT('Ctrl Pts',(-26.4601101154003,-13.6065321357651,
114.285445210614)) ;
#171292=CARTESIAN_POINT('Ctrl Pts',(-26.483451503805,-13.6192674880133,
114.35653931193)) ;
#171293=CARTESIAN_POINT('Ctrl Pts',(-26.4096476651838,-13.6192674042519,
114.380770368232)) ;
#171294=CARTESIAN_POINT('Ctrl Pts',(-26.3358438265625,-13.6192673204905,
114.405001424534)) ;
#171295=CARTESIAN_POINT('Ctrl Pts',(-26.3125024381578,-13.6065319682423,
114.333907323218)) ;
#171296=CARTESIAN_POINT('Ctrl Pts',(-26.2953957023122,-13.8845186470045,
114.246262443011)) ;
#171297=CARTESIAN_POINT('Ctrl Pts',(-26.2739487735497,-13.8523553116745,
114.180938559947)) ;
#171298=CARTESIAN_POINT('Ctrl Pts',(-26.3477526064039,-13.852355381399,
114.156707486079)) ;
#171299=CARTESIAN_POINT('Ctrl Pts',(-26.4215564392581,-13.8523554511235,
114.132476412212)) ;
#171300=CARTESIAN_POINT('Ctrl Pts',(-26.4430033680206,-13.8845187864536,
114.197800295276)) ;
#171301=CARTESIAN_POINT('Ctrl Pts',(-26.464450296783,-13.9166821217837,
114.263124178339)) ;
#171302=CARTESIAN_POINT('Ctrl Pts',(-26.3906464639288,-13.9166820520591,
114.287355252207)) ;
#171303=CARTESIAN_POINT('Ctrl Pts',(-26.3168426310747,-13.9166819823346,
114.311586326074)) ;
#171304=CARTESIAN_POINT('Ctrl Pts',(-26.2953957023122,-13.8845186470045,
114.246262443011)) ;
#171305=CARTESIAN_POINT('Ctrl Pts',(-26.2564785433818,-14.1277890814299,
114.092378152371)) ;
#171306=CARTESIAN_POINT('Ctrl Pts',(-26.2384479066427,-14.0785921493268,
114.037459743464)) ;
#171307=CARTESIAN_POINT('Ctrl Pts',(-26.3122517354857,-14.0785922024829,
114.013228657379)) ;
#171308=CARTESIAN_POINT('Ctrl Pts',(-26.3860555643286,-14.0785922556391,
113.988997571294)) ;
#171309=CARTESIAN_POINT('Ctrl Pts',(-26.4040862010677,-14.1277891877422,
114.043915980201)) ;
#171310=CARTESIAN_POINT('Ctrl Pts',(-26.4221168378068,-14.1769861198453,
114.098834389108)) ;
#171311=CARTESIAN_POINT('Ctrl Pts',(-26.3483130089639,-14.1769860666892,
114.123065475193)) ;
#171312=CARTESIAN_POINT('Ctrl Pts',(-26.2745091801209,-14.1769860135331,
114.147296561278)) ;
#171313=CARTESIAN_POINT('Ctrl Pts',(-26.2564785433818,-14.1277890814299,
114.092378152371)) ;
#171314=CARTESIAN_POINT('Ctrl Pts',(-26.1989157065957,-14.3214999944636,
113.88150015982)) ;
#171315=CARTESIAN_POINT('Ctrl Pts',(-26.1856123717527,-14.2587034430882,
113.840980349568)) ;
#171316=CARTESIAN_POINT('Ctrl Pts',(-26.2594161990129,-14.2587034768352,
113.816749258662)) ;
#171317=CARTESIAN_POINT('Ctrl Pts',(-26.3332200262729,-14.2587035105822,
113.792518167755)) ;
#171318=CARTESIAN_POINT('Ctrl Pts',(-26.3465233611159,-14.3215000619577,
113.833037978008)) ;
#171319=CARTESIAN_POINT('Ctrl Pts',(-26.3598266959589,-14.3842966133332,
113.873557788261)) ;
#171320=CARTESIAN_POINT('Ctrl Pts',(-26.2860228686988,-14.3842965795861,
113.897788879167)) ;
#171321=CARTESIAN_POINT('Ctrl Pts',(-26.2122190414387,-14.3842965458391,
113.922019970073)) ;
#171322=CARTESIAN_POINT('Ctrl Pts',(-26.1989157065957,-14.3214999944636,
113.88150015982)) ;
#171323=CARTESIAN_POINT('Ctrl Pts',(-26.1278964756566,-14.4499114443817,
113.629724275749)) ;
#171324=CARTESIAN_POINT('Ctrl Pts',(-26.1202654228016,-14.3780538242765,
113.606481321047)) ;
#171325=CARTESIAN_POINT('Ctrl Pts',(-26.1940692503916,-14.37805384036,113.582250231146)) ;
#171326=CARTESIAN_POINT('Ctrl Pts',(-26.2678730779816,-14.3780538564435,
113.558019141244)) ;
#171327=CARTESIAN_POINT('Ctrl Pts',(-26.2755041308367,-14.4499114765488,
113.581262095946)) ;
#171328=CARTESIAN_POINT('Ctrl Pts',(-26.2831351836917,-14.521769096654,
113.604505050649)) ;
#171329=CARTESIAN_POINT('Ctrl Pts',(-26.2093313561017,-14.5217690805705,
113.62873614055)) ;
#171330=CARTESIAN_POINT('Ctrl Pts',(-26.1355275285117,-14.521769064487,
113.652967230451)) ;
#171331=CARTESIAN_POINT('Ctrl Pts',(-26.1278964756566,-14.4499114443817,
113.629724275749)) ;
#171332=CARTESIAN_POINT('Ctrl Pts',(-26.0490886415224,-14.5043711676863,
113.354180073168)) ;
#171333=CARTESIAN_POINT('Ctrl Pts',(-26.0476832870499,-14.4286019200682,
113.34989959105)) ;
#171334=CARTESIAN_POINT('Ctrl Pts',(-26.1214871167149,-14.4286019216996,
113.325668507468)) ;
#171335=CARTESIAN_POINT('Ctrl Pts',(-26.1952909463798,-14.4286019233309,
113.301437423887)) ;
#171336=CARTESIAN_POINT('Ctrl Pts',(-26.1966963008522,-14.504371170949,
113.305717906005)) ;
#171337=CARTESIAN_POINT('Ctrl Pts',(-26.1981016553247,-14.5801404185671,
113.309998388123)) ;
#171338=CARTESIAN_POINT('Ctrl Pts',(-26.1242978256598,-14.5801404169357,
113.334229471704)) ;
#171339=CARTESIAN_POINT('Ctrl Pts',(-26.0504939959948,-14.5801404153043,
113.358460555286)) ;
#171340=CARTESIAN_POINT('Ctrl Pts',(-26.0490886415224,-14.5043711676863,
113.354180073168)) ;
#171341=CARTESIAN_POINT('Ctrl Pts',(-25.9693316672278,-14.481209763182,
113.075913353523)) ;
#171342=CARTESIAN_POINT('Ctrl Pts',(-25.9742242882722,-14.4069431255803,
113.090815488511)) ;
#171343=CARTESIAN_POINT('Ctrl Pts',(-26.0480281205744,-14.4069431170847,
113.066584412962)) ;
#171344=CARTESIAN_POINT('Ctrl Pts',(-26.1218319528766,-14.4069431085892,
113.042353337413)) ;
#171345=CARTESIAN_POINT('Ctrl Pts',(-26.1169393318322,-14.4812097461908,
113.027451202425)) ;
#171346=CARTESIAN_POINT('Ctrl Pts',(-26.1120467107878,-14.5554763837924,
113.012549067438)) ;
#171347=CARTESIAN_POINT('Ctrl Pts',(-26.0382428784855,-14.555476392288,
113.036780142987)) ;
#171348=CARTESIAN_POINT('Ctrl Pts',(-25.9644390461833,-14.5554764007836,
113.061011218535)) ;
#171349=CARTESIAN_POINT('Ctrl Pts',(-25.9693316672278,-14.481209763182,
113.075913353523)) ;
#171350=CARTESIAN_POINT('Ctrl Pts',(-25.8943302897143,-14.3816923411007,
112.811938342538)) ;
#171351=CARTESIAN_POINT('Ctrl Pts',(-25.9052024989069,-14.3142615616255,
112.845053338047)) ;
#171352=CARTESIAN_POINT('Ctrl Pts',(-25.9790063348074,-14.3142615481585,
112.820822273458)) ;
#171353=CARTESIAN_POINT('Ctrl Pts',(-26.052810170708,-14.3142615346915,
112.796591208869)) ;
#171354=CARTESIAN_POINT('Ctrl Pts',(-26.0419379615153,-14.3816923141668,
112.76347621336)) ;
#171355=CARTESIAN_POINT('Ctrl Pts',(-26.0310657523227,-14.449123093642,
112.730361217852)) ;
#171356=CARTESIAN_POINT('Ctrl Pts',(-25.9572619164222,-14.449123107109,
112.754592282441)) ;
#171357=CARTESIAN_POINT('Ctrl Pts',(-25.8834580805216,-14.4491231205759,
112.778823347029)) ;
#171358=CARTESIAN_POINT('Ctrl Pts',(-25.8943302897143,-14.3816923411007,
112.811938342538)) ;
#171359=CARTESIAN_POINT('Ctrl Pts',(-25.8307713706495,-14.2134896291755,
112.582919254125)) ;
#171360=CARTESIAN_POINT('Ctrl Pts',(-25.8468311156039,-14.1577013578714,
112.63183464641)) ;
#171361=CARTESIAN_POINT('Ctrl Pts',(-25.9206349546597,-14.1577013437741,
112.607603591431)) ;
#171362=CARTESIAN_POINT('Ctrl Pts',(-25.9944387937155,-14.1577013296769,
112.583372536453)) ;
#171363=CARTESIAN_POINT('Ctrl Pts',(-25.9783790487612,-14.2134896009809,
112.534457144168)) ;
#171364=CARTESIAN_POINT('Ctrl Pts',(-25.9623193038068,-14.269277872285,
112.485541751884)) ;
#171365=CARTESIAN_POINT('Ctrl Pts',(-25.888515464751,-14.2692778863823,
112.509772806863)) ;
#171366=CARTESIAN_POINT('Ctrl Pts',(-25.8147116256952,-14.2692779004795,
112.534003861841)) ;
#171367=CARTESIAN_POINT('Ctrl Pts',(-25.8307713706495,-14.2134896291755,
112.582919254125)) ;
#171368=CARTESIAN_POINT('Ctrl Pts',(-25.7835794301014,-13.9864989351748,
112.403492770186)) ;
#171369=CARTESIAN_POINT('Ctrl Pts',(-25.8036973649584,-13.9464758835493,
112.464768753956)) ;
#171370=CARTESIAN_POINT('Ctrl Pts',(-25.8775012067237,-13.9464758738248,
112.440537707231)) ;
#171371=CARTESIAN_POINT('Ctrl Pts',(-25.9513050484891,-13.9464758641003,
112.416306660505)) ;
#171372=CARTESIAN_POINT('Ctrl Pts',(-25.9311871136321,-13.9864989157259,
112.355030676735)) ;
#171373=CARTESIAN_POINT('Ctrl Pts',(-25.9110691787752,-14.0265219673515,
112.293754692964)) ;
#171374=CARTESIAN_POINT('Ctrl Pts',(-25.8372653370098,-14.0265219770759,
112.31798573969)) ;
#171375=CARTESIAN_POINT('Ctrl Pts',(-25.7634614952445,-14.0265219868004,
112.342216786415)) ;
#171376=CARTESIAN_POINT('Ctrl Pts',(-25.7835794301014,-13.9864989351748,
112.403492770186)) ;
#171377=CARTESIAN_POINT('Ctrl Pts',(-25.7575024369132,-13.7220237261921,
112.288851169171)) ;
#171378=CARTESIAN_POINT('Ctrl Pts',(-25.780200037052,-13.7004075787871,
112.357984397076)) ;
#171379=CARTESIAN_POINT('Ctrl Pts',(-25.8540038800281,-13.7004075723778,
112.333753354038)) ;
#171380=CARTESIAN_POINT('Ctrl Pts',(-25.9278077230041,-13.7004075659685,
112.309522311)) ;
#171381=CARTESIAN_POINT('Ctrl Pts',(-25.9051101228652,-13.7220237133736,
112.240389083094)) ;
#171382=CARTESIAN_POINT('Ctrl Pts',(-25.8824125227264,-13.7436398607786,
112.171255855189)) ;
#171383=CARTESIAN_POINT('Ctrl Pts',(-25.8086086797504,-13.7436398671878,
112.195486898227)) ;
#171384=CARTESIAN_POINT('Ctrl Pts',(-25.7348048367744,-13.7436398735971,
112.219717941265)) ;
#171385=CARTESIAN_POINT('Ctrl Pts',(-25.7575024369132,-13.7220237261921,
112.288851169171)) ;
#171386=CARTESIAN_POINT('Ctrl Pts',(-25.7546020971339,-13.4322464163541,
112.244321998672)) ;
#171387=CARTESIAN_POINT('Ctrl Pts',(-25.7782752222252,-13.4308324436495,
112.316426518066)) ;
#171388=CARTESIAN_POINT('Ctrl Pts',(-25.8520790657583,-13.4308324430486,
112.292195476725)) ;
#171389=CARTESIAN_POINT('Ctrl Pts',(-25.9258829092914,-13.4308324424476,
112.267964435384)) ;
#171390=CARTESIAN_POINT('Ctrl Pts',(-25.9022097842002,-13.4322464151522,
112.195859915989)) ;
#171391=CARTESIAN_POINT('Ctrl Pts',(-25.878536659109,-13.4336603878567,
112.123755396595)) ;
#171392=CARTESIAN_POINT('Ctrl Pts',(-25.8047328155758,-13.4336603884577,
112.147986437936)) ;
#171393=CARTESIAN_POINT('Ctrl Pts',(-25.7309289720427,-13.4336603890586,
112.172217479278)) ;
#171394=CARTESIAN_POINT('Ctrl Pts',(-25.7546020971339,-13.4322464163541,
112.244321998672)) ;
#171395=CARTESIAN_POINT('Ctrl Pts',(-25.7758240368022,-13.1452897052538,
112.273770028607)) ;
#171396=CARTESIAN_POINT('Ctrl Pts',(-25.7987787120654,-13.1639105046461,
112.343686265702)) ;
#171397=CARTESIAN_POINT('Ctrl Pts',(-25.8725825553839,-13.1639105064164,
112.319455223707)) ;
#171398=CARTESIAN_POINT('Ctrl Pts',(-25.9463863987024,-13.1639105081867,
112.295224181712)) ;
#171399=CARTESIAN_POINT('Ctrl Pts',(-25.9234317234392,-13.1452897087944,
112.225307944617)) ;
#171400=CARTESIAN_POINT('Ctrl Pts',(-25.900477048176,-13.1266689094021,
112.155391707523)) ;
#171401=CARTESIAN_POINT('Ctrl Pts',(-25.8266732048575,-13.1266689076317,
112.179622749518)) ;
#171402=CARTESIAN_POINT('Ctrl Pts',(-25.752869361539,-13.1266689058614,
112.203853791513)) ;
#171403=CARTESIAN_POINT('Ctrl Pts',(-25.7758240368022,-13.1452897052538,
112.273770028607)) ;
#171404=CARTESIAN_POINT('Ctrl Pts',(-25.821130261938,-12.8735307541799,
112.375991971865)) ;
#171405=CARTESIAN_POINT('Ctrl Pts',(-25.8416958911711,-12.9111570713961,
112.438631560189)) ;
#171406=CARTESIAN_POINT('Ctrl Pts',(-25.9154997340476,-12.9111570744422,
112.414400516848)) ;
#171407=CARTESIAN_POINT('Ctrl Pts',(-25.989303576924,-12.9111570774884,
112.390169473506)) ;
#171408=CARTESIAN_POINT('Ctrl Pts',(-25.9687379476908,-12.8735307602723,
112.327529885182)) ;
#171409=CARTESIAN_POINT('Ctrl Pts',(-25.9481723184577,-12.8359044430562,
112.264890296858)) ;
#171410=CARTESIAN_POINT('Ctrl Pts',(-25.8743684755813,-12.83590444001,112.289121340199)) ;
#171411=CARTESIAN_POINT('Ctrl Pts',(-25.8005646327049,-12.8359044369638,
112.31335238354)) ;
#171412=CARTESIAN_POINT('Ctrl Pts',(-25.821130261938,-12.8735307541799,
112.375991971865)) ;
#171413=CARTESIAN_POINT('Ctrl Pts',(-25.8866884207212,-12.6449175335016,
112.54048346263)) ;
#171414=CARTESIAN_POINT('Ctrl Pts',(-25.9034346718771,-12.6985622170396,
112.591489841605)) ;
#171415=CARTESIAN_POINT('Ctrl Pts',(-25.9772385146951,-12.698562218704,
112.567258798085)) ;
#171416=CARTESIAN_POINT('Ctrl Pts',(-26.0510423575131,-12.6985622203683,
112.543027754566)) ;
#171417=CARTESIAN_POINT('Ctrl Pts',(-26.0342961063572,-12.6449175368303,
112.492021375591)) ;
#171418=CARTESIAN_POINT('Ctrl Pts',(-26.0175498552012,-12.5912728532923,
112.441014996616)) ;
#171419=CARTESIAN_POINT('Ctrl Pts',(-25.9437460123832,-12.5912728516279,
112.465246040135)) ;
#171420=CARTESIAN_POINT('Ctrl Pts',(-25.8699421695653,-12.5912728499636,
112.489477083655)) ;
#171421=CARTESIAN_POINT('Ctrl Pts',(-25.8866884207212,-12.6449175335016,
112.54048346263)) ;
#171422=CARTESIAN_POINT('Ctrl Pts',(-25.9697390448969,-12.4692026417619,
112.757943207403)) ;
#171423=CARTESIAN_POINT('Ctrl Pts',(-25.9814453819459,-12.5351960145383,
112.793598821244)) ;
#171424=CARTESIAN_POINT('Ctrl Pts',(-26.0552492253081,-12.5351960141678,
112.769367779382)) ;
#171425=CARTESIAN_POINT('Ctrl Pts',(-26.1290530686703,-12.5351960137972,
112.74513673752)) ;
#171426=CARTESIAN_POINT('Ctrl Pts',(-26.1173467316213,-12.4692026410208,
112.709481123679)) ;
#171427=CARTESIAN_POINT('Ctrl Pts',(-26.1056403945723,-12.4032092682444,
112.673825509837)) ;
#171428=CARTESIAN_POINT('Ctrl Pts',(-26.0318365512101,-12.4032092686149,
112.698056551699)) ;
#171429=CARTESIAN_POINT('Ctrl Pts',(-25.9580327078479,-12.4032092689855,
112.722287593561)) ;
#171430=CARTESIAN_POINT('Ctrl Pts',(-25.9697390448969,-12.4692026417619,
112.757943207403)) ;
#171431=CARTESIAN_POINT('Ctrl Pts',(-26.0651797901007,-12.3617390442732,
113.013009958698)) ;
#171432=CARTESIAN_POINT('Ctrl Pts',(-26.0709763080344,-12.4353332114667,
113.030665217169)) ;
#171433=CARTESIAN_POINT('Ctrl Pts',(-26.1447801531298,-12.4353332096564,
113.006434180586)) ;
#171434=CARTESIAN_POINT('Ctrl Pts',(-26.2185839982252,-12.4353332078462,
112.982203144004)) ;
#171435=CARTESIAN_POINT('Ctrl Pts',(-26.2127874802915,-12.3617390406526,
112.964547885532)) ;
#171436=CARTESIAN_POINT('Ctrl Pts',(-26.2069909623578,-12.2881448734591,
112.946892627061)) ;
#171437=CARTESIAN_POINT('Ctrl Pts',(-26.1331871172624,-12.2881448752694,
112.971123663643)) ;
#171438=CARTESIAN_POINT('Ctrl Pts',(-26.059383272167,-12.2881448770796,
112.995354700226)) ;
#171439=CARTESIAN_POINT('Ctrl Pts',(-26.0651797901007,-12.3617390442732,
113.013009958698)) ;
#171440=CARTESIAN_POINT('Ctrl Pts',(-26.1654275204562,-12.3304471936261,
113.283082395496)) ;
#171441=CARTESIAN_POINT('Ctrl Pts',(-26.1649626053493,-12.4063328156575,
113.281666339294)) ;
#171442=CARTESIAN_POINT('Ctrl Pts',(-26.2387664519881,-12.4063328154178,
113.257435307412)) ;
#171443=CARTESIAN_POINT('Ctrl Pts',(-26.3125702986269,-12.4063328151781,
113.23320427553)) ;
#171444=CARTESIAN_POINT('Ctrl Pts',(-26.3130352137339,-12.3304471931467,
113.234620331733)) ;
#171445=CARTESIAN_POINT('Ctrl Pts',(-26.3135001288408,-12.2545615711153,
113.236036387935)) ;
#171446=CARTESIAN_POINT('Ctrl Pts',(-26.239696282202,-12.254561571355,113.260267419817)) ;
#171447=CARTESIAN_POINT('Ctrl Pts',(-26.1658924355632,-12.2545615715947,
113.284498451699)) ;
#171448=CARTESIAN_POINT('Ctrl Pts',(-26.1654275204562,-12.3304471936261,
113.283082395496)) ;
#171449=CARTESIAN_POINT('Ctrl Pts',(-26.2657660829558,-12.376595059269,
113.553179153048)) ;
#171450=CARTESIAN_POINT('Ctrl Pts',(-26.2590295101417,-12.4493688880087,
113.532660639538)) ;
#171451=CARTESIAN_POINT('Ctrl Pts',(-26.3328333588651,-12.4493688924278,
113.508429614006)) ;
#171452=CARTESIAN_POINT('Ctrl Pts',(-26.4066372075886,-12.4493688968469,
113.484198588473)) ;
#171453=CARTESIAN_POINT('Ctrl Pts',(-26.4133737804027,-12.3765950681072,
113.504717101983)) ;
#171454=CARTESIAN_POINT('Ctrl Pts',(-26.4201103532167,-12.3038212393674,
113.525235615492)) ;
#171455=CARTESIAN_POINT('Ctrl Pts',(-26.3463065044933,-12.3038212349483,
113.549466641025)) ;
#171456=CARTESIAN_POINT('Ctrl Pts',(-26.2725026557699,-12.3038212305292,
113.573697666557)) ;
#171457=CARTESIAN_POINT('Ctrl Pts',(-26.2657660829558,-12.376595059269,
113.553179153048)) ;
#171458=CARTESIAN_POINT('Ctrl Pts',(-26.359065116246,-12.4977240769561,
113.801833331804)) ;
#171459=CARTESIAN_POINT('Ctrl Pts',(-26.3465394344376,-12.5621460088863,
113.763682126528)) ;
#171460=CARTESIAN_POINT('Ctrl Pts',(-26.4203432848208,-12.5621460220276,
113.73945110605)) ;
#171461=CARTESIAN_POINT('Ctrl Pts',(-26.4941471352039,-12.5621460351689,
113.715220085573)) ;
#171462=CARTESIAN_POINT('Ctrl Pts',(-26.5066728170123,-12.4977241032387,
113.753371290849)) ;
#171463=CARTESIAN_POINT('Ctrl Pts',(-26.5191984988206,-12.4333021713085,
113.791522496126)) ;
#171464=CARTESIAN_POINT('Ctrl Pts',(-26.4453946484375,-12.4333021581672,
113.815753516603)) ;
#171465=CARTESIAN_POINT('Ctrl Pts',(-26.3715907980544,-12.4333021450259,
113.83998453708)) ;
#171466=CARTESIAN_POINT('Ctrl Pts',(-26.359065116246,-12.4977240769561,
113.801833331804)) ;
#171467=CARTESIAN_POINT('Ctrl Pts',(-26.4393585568978,-12.6852356935121,
114.010845608305)) ;
#171468=CARTESIAN_POINT('Ctrl Pts',(-26.4219441286147,-12.736658719336,
113.95780407024)) ;
#171469=CARTESIAN_POINT('Ctrl Pts',(-26.4957479795408,-12.7366587448055,
113.933573051417)) ;
#171470=CARTESIAN_POINT('Ctrl Pts',(-26.569551830467,-12.7366587702751,
113.909342032593)) ;
#171471=CARTESIAN_POINT('Ctrl Pts',(-26.58696625875,-12.6852357444512,113.962383570658)) ;
#171472=CARTESIAN_POINT('Ctrl Pts',(-26.6043806870331,-12.6338127186274,
114.015425108723)) ;
#171473=CARTESIAN_POINT('Ctrl Pts',(-26.530576836107,-12.6338126931579,
114.039656127546)) ;
#171474=CARTESIAN_POINT('Ctrl Pts',(-26.4567729851808,-12.6338126676883,
114.063887146369)) ;
#171475=CARTESIAN_POINT('Ctrl Pts',(-26.4393585568978,-12.6852356935121,
114.010845608305)) ;
#171476=CARTESIAN_POINT('Ctrl Pts',(-26.5012600267756,-12.9233901911912,
114.164108379881)) ;
#171477=CARTESIAN_POINT('Ctrl Pts',(-26.4802286428052,-12.9582592987456,
114.100050178518)) ;
#171478=CARTESIAN_POINT('Ctrl Pts',(-26.5540324923643,-12.958259335733,
114.075819155531)) ;
#171479=CARTESIAN_POINT('Ctrl Pts',(-26.6278363419234,-12.9582593727203,
114.051588132544)) ;
#171480=CARTESIAN_POINT('Ctrl Pts',(-26.6488677258939,-12.9233902651659,
114.115646333907)) ;
#171481=CARTESIAN_POINT('Ctrl Pts',(-26.6698991098643,-12.8885211576114,
114.17970453527)) ;
#171482=CARTESIAN_POINT('Ctrl Pts',(-26.5960952603051,-12.8885211206241,
114.203935558257)) ;
#171483=CARTESIAN_POINT('Ctrl Pts',(-26.522291410746,-12.8885210836367,
114.228166581244)) ;
#171484=CARTESIAN_POINT('Ctrl Pts',(-26.5012600267756,-12.9233901911912,
114.164108379881)) ;
#171485=CARTESIAN_POINT('Ctrl Pts',(-26.5420541011494,-13.1995574427629,
114.252712502089)) ;
#171486=CARTESIAN_POINT('Ctrl Pts',(-26.5188815950457,-13.2151953803477,
114.18213278838)) ;
#171487=CARTESIAN_POINT('Ctrl Pts',(-26.5926854420113,-13.2151954315295,
114.157901757494)) ;
#171488=CARTESIAN_POINT('Ctrl Pts',(-26.6664892889769,-13.2151954827113,
114.133670726607)) ;
#171489=CARTESIAN_POINT('Ctrl Pts',(-26.6896617950807,-13.1995575451265,
114.204250440316)) ;
#171490=CARTESIAN_POINT('Ctrl Pts',(-26.7128343011844,-13.1839196075417,
114.274830154024)) ;
#171491=CARTESIAN_POINT('Ctrl Pts',(-26.6390304542188,-13.1839195563599,
114.299061184911)) ;
#171492=CARTESIAN_POINT('Ctrl Pts',(-26.5652266072531,-13.1839195051781,
114.323292215797)) ;
#171493=CARTESIAN_POINT('Ctrl Pts',(-26.5420541011494,-13.1995574427629,
114.252712502089)) ;
#171494=CARTESIAN_POINT('Ctrl Pts',(-26.5586624454798,-13.4900175633602,
114.267844947108)) ;
#171495=CARTESIAN_POINT('Ctrl Pts',(-26.5350304987127,-13.4853985697917,
114.195865851433)) ;
#171496=CARTESIAN_POINT('Ctrl Pts',(-26.6088343410563,-13.4853986306042,
114.171634806468)) ;
#171497=CARTESIAN_POINT('Ctrl Pts',(-26.6826381833999,-13.4853986914167,
114.147403761504)) ;
#171498=CARTESIAN_POINT('Ctrl Pts',(-26.706270130167,-13.4900176849852,
114.219382857179)) ;
#171499=CARTESIAN_POINT('Ctrl Pts',(-26.7299020769341,-13.4946366785538,
114.291361952854)) ;
#171500=CARTESIAN_POINT('Ctrl Pts',(-26.6560982345905,-13.4946366177413,
114.315592997819)) ;
#171501=CARTESIAN_POINT('Ctrl Pts',(-26.5822943922469,-13.4946365569288,
114.339824042783)) ;
#171502=CARTESIAN_POINT('Ctrl Pts',(-26.5586624454798,-13.4900175633602,
114.267844947108)) ;
#171503=CARTESIAN_POINT('Ctrl Pts',(-26.5511685763042,-13.7743854626431,
114.209679423832)) ;
#171504=CARTESIAN_POINT('Ctrl Pts',(-26.5287570348701,-13.7499058485971,
114.141417486027)) ;
#171505=CARTESIAN_POINT('Ctrl Pts',(-26.6025608715152,-13.7499059130724,
114.117186423706)) ;
#171506=CARTESIAN_POINT('Ctrl Pts',(-26.6763647081602,-13.7499059775478,
114.092955361385)) ;
#171507=CARTESIAN_POINT('Ctrl Pts',(-26.6987762495943,-13.7743855915938,
114.161217299189)) ;
#171508=CARTESIAN_POINT('Ctrl Pts',(-26.7211877910284,-13.7988652056398,
114.229479236994)) ;
#171509=CARTESIAN_POINT('Ctrl Pts',(-26.6473839543834,-13.7988651411644,
114.253710299315)) ;
#171510=CARTESIAN_POINT('Ctrl Pts',(-26.5735801177383,-13.7988650766891,
114.277941361636)) ;
#171511=CARTESIAN_POINT('Ctrl Pts',(-26.5511685763042,-13.7743854626431,
114.209679423832)) ;
#171512=CARTESIAN_POINT('Ctrl Pts',(-26.5207255627321,-14.034295085312,
114.081488551575)) ;
#171513=CARTESIAN_POINT('Ctrl Pts',(-26.5011408734775,-13.9916338194208,
114.021836749551)) ;
#171514=CARTESIAN_POINT('Ctrl Pts',(-26.5749447036413,-13.9916338823601,
113.997605667489)) ;
#171515=CARTESIAN_POINT('Ctrl Pts',(-26.648748533805,-13.9916339452994,
113.973374585426)) ;
#171516=CARTESIAN_POINT('Ctrl Pts',(-26.6683332230596,-14.0342952111906,
114.033026387451)) ;
#171517=CARTESIAN_POINT('Ctrl Pts',(-26.6879179123141,-14.0769564770818,
114.092678189475)) ;
#171518=CARTESIAN_POINT('Ctrl Pts',(-26.6141140821504,-14.0769564141425,
114.116909271537)) ;
#171519=CARTESIAN_POINT('Ctrl Pts',(-26.5403102519867,-14.0769563512032,
114.141140353599)) ;
#171520=CARTESIAN_POINT('Ctrl Pts',(-26.5207255627321,-14.034295085312,
114.081488551575)) ;
#171521=CARTESIAN_POINT('Ctrl Pts',(-26.4702129616919,-14.2500983716934,
113.892161270726)) ;
#171522=CARTESIAN_POINT('Ctrl Pts',(-26.4548605002029,-14.1923084690493,
113.84540015175)) ;
#171523=CARTESIAN_POINT('Ctrl Pts',(-26.5286643238617,-14.1923085231576,
113.821169049876)) ;
#171524=CARTESIAN_POINT('Ctrl Pts',(-26.6024681475206,-14.192308577266,
113.796937948001)) ;
#171525=CARTESIAN_POINT('Ctrl Pts',(-26.6178206090096,-14.2500984799102,
113.843699066976)) ;
#171526=CARTESIAN_POINT('Ctrl Pts',(-26.6331730704987,-14.3078883825543,
113.890460185952)) ;
#171527=CARTESIAN_POINT('Ctrl Pts',(-26.5593692468399,-14.307888328446,
113.914691287827)) ;
#171528=CARTESIAN_POINT('Ctrl Pts',(-26.485565423181,-14.3078882743376,
113.938922389702)) ;
#171529=CARTESIAN_POINT('Ctrl Pts',(-26.4702129616919,-14.2500983716934,
113.892161270726)) ;
#171530=CARTESIAN_POINT('Ctrl Pts',(-26.4040228817349,-14.4061684747286,
113.655081180054)) ;
#171531=CARTESIAN_POINT('Ctrl Pts',(-26.3940033136551,-14.3373982174877,
113.62456319407)) ;
#171532=CARTESIAN_POINT('Ctrl Pts',(-26.467807131676,-14.3373982554781,
113.600332075023)) ;
#171533=CARTESIAN_POINT('Ctrl Pts',(-26.5416109496969,-14.3373982934686,
113.576100955976)) ;
#171534=CARTESIAN_POINT('Ctrl Pts',(-26.5516305177767,-14.4061685507095,
113.606618941959)) ;
#171535=CARTESIAN_POINT('Ctrl Pts',(-26.5616500858565,-14.4749388079505,
113.637136927943)) ;
#171536=CARTESIAN_POINT('Ctrl Pts',(-26.4878462678356,-14.47493876996,113.66136804699)) ;
#171537=CARTESIAN_POINT('Ctrl Pts',(-26.4140424498147,-14.4749387319696,
113.685599166037)) ;
#171538=CARTESIAN_POINT('Ctrl Pts',(-26.4040228817349,-14.4061684747286,
113.655081180054)) ;
#171539=CARTESIAN_POINT('Ctrl Pts',(-26.3278700224272,-14.4915146282391,
113.3877465935)) ;
#171540=CARTESIAN_POINT('Ctrl Pts',(-26.323884778629,-14.4166858315879,
113.375608185746)) ;
#171541=CARTESIAN_POINT('Ctrl Pts',(-26.3976885927888,-14.4166858475525,
113.351377054938)) ;
#171542=CARTESIAN_POINT('Ctrl Pts',(-26.4714924069487,-14.4166858635172,
113.327145924131)) ;
#171543=CARTESIAN_POINT('Ctrl Pts',(-26.4754776507469,-14.4915146601683,
113.339284331886)) ;
#171544=CARTESIAN_POINT('Ctrl Pts',(-26.4794628945451,-14.5663434568195,
113.351422739641)) ;
#171545=CARTESIAN_POINT('Ctrl Pts',(-26.4056590803852,-14.5663434408549,
113.375653870448)) ;
#171546=CARTESIAN_POINT('Ctrl Pts',(-26.3318552662254,-14.5663434248902,
113.399885001255)) ;
#171547=CARTESIAN_POINT('Ctrl Pts',(-26.3278700224272,-14.4915146282391,
113.3877465935)) ;
#171548=CARTESIAN_POINT('Ctrl Pts',(-26.2471359022358,-14.4998611303634,
113.106175912195)) ;
#171549=CARTESIAN_POINT('Ctrl Pts',(-26.249519313875,-14.4243396117057,
113.113435401435)) ;
#171550=CARTESIAN_POINT('Ctrl Pts',(-26.3233231259959,-14.4243396013487,
113.089204264417)) ;
#171551=CARTESIAN_POINT('Ctrl Pts',(-26.3971269381168,-14.4243395909917,
113.0649731274)) ;
#171552=CARTESIAN_POINT('Ctrl Pts',(-26.3947435264776,-14.4998611096494,
113.05771363816)) ;
#171553=CARTESIAN_POINT('Ctrl Pts',(-26.3923601148385,-14.5753826283071,
113.05045414892)) ;
#171554=CARTESIAN_POINT('Ctrl Pts',(-26.3185563027175,-14.5753826386642,
113.074685285938)) ;
#171555=CARTESIAN_POINT('Ctrl Pts',(-26.2447524905966,-14.5753826490212,
113.098916422955)) ;
#171556=CARTESIAN_POINT('Ctrl Pts',(-26.2471359022358,-14.4998611303634,
113.106175912195)) ;
#171557=CARTESIAN_POINT('Ctrl Pts',(-26.1698468947087,-14.4309678249663,
112.835496447081)) ;
#171558=CARTESIAN_POINT('Ctrl Pts',(-26.1783596457039,-14.3601461164253,
112.861424915088)) ;
#171559=CARTESIAN_POINT('Ctrl Pts',(-26.2521634589948,-14.3601460788116,
112.837193781634)) ;
#171560=CARTESIAN_POINT('Ctrl Pts',(-26.3259672722857,-14.3601460411978,
112.81296264818)) ;
#171561=CARTESIAN_POINT('Ctrl Pts',(-26.3174545212904,-14.4309677497388,
112.787034180173)) ;
#171562=CARTESIAN_POINT('Ctrl Pts',(-26.3089417702951,-14.5017894582798,
112.761105712166)) ;
#171563=CARTESIAN_POINT('Ctrl Pts',(-26.2351379570042,-14.5017894958936,
112.78533684562)) ;
#171564=CARTESIAN_POINT('Ctrl Pts',(-26.1613341437133,-14.5017895335074,
112.809567979074)) ;
#171565=CARTESIAN_POINT('Ctrl Pts',(-26.1698468947087,-14.4309678249663,
112.835496447081)) ;
#171566=CARTESIAN_POINT('Ctrl Pts',(-26.1008946624863,-14.2895356443573,
112.589987356344)) ;
#171567=CARTESIAN_POINT('Ctrl Pts',(-26.114968245912,-14.2284839799428,
112.632853222754)) ;
#171568=CARTESIAN_POINT('Ctrl Pts',(-26.1887720626717,-14.228483916303,
112.608622099865)) ;
#171569=CARTESIAN_POINT('Ctrl Pts',(-26.2625758794314,-14.2284838526632,
112.584390976976)) ;
#171570=CARTESIAN_POINT('Ctrl Pts',(-26.2485022960057,-14.2895355170776,
112.541525110567)) ;
#171571=CARTESIAN_POINT('Ctrl Pts',(-26.2344287125799,-14.3505871814921,
112.498659244158)) ;
#171572=CARTESIAN_POINT('Ctrl Pts',(-26.1606248958203,-14.3505872451319,
112.522890367047)) ;
#171573=CARTESIAN_POINT('Ctrl Pts',(-26.0868210790606,-14.3505873087717,
112.547121489935)) ;
#171574=CARTESIAN_POINT('Ctrl Pts',(-26.1008946624863,-14.2895356443573,
112.589987356344)) ;
#171575=CARTESIAN_POINT('Ctrl Pts',(-26.0464820576728,-14.0847982621001,
112.388687807396)) ;
#171576=CARTESIAN_POINT('Ctrl Pts',(-26.065111268296,-14.0379502045981,
112.445429379231)) ;
#171577=CARTESIAN_POINT('Ctrl Pts',(-26.1389150910251,-14.0379501191932,
112.421198274525)) ;
#171578=CARTESIAN_POINT('Ctrl Pts',(-26.2127189137541,-14.0379500337882,
112.396967169818)) ;
#171579=CARTESIAN_POINT('Ctrl Pts',(-26.1940897031309,-14.0847980912902,
112.340225597982)) ;
#171580=CARTESIAN_POINT('Ctrl Pts',(-26.1754604925076,-14.1316461487922,
112.283484026146)) ;
#171581=CARTESIAN_POINT('Ctrl Pts',(-26.1016566697786,-14.1316462341972,
112.307715130853)) ;
#171582=CARTESIAN_POINT('Ctrl Pts',(-26.0278528470495,-14.1316463196022,
112.33194623556)) ;
#171583=CARTESIAN_POINT('Ctrl Pts',(-26.0464820576728,-14.0847982621001,
112.388687807396)) ;
#171584=CARTESIAN_POINT('Ctrl Pts',(-26.0114557448713,-13.8335759567493,
112.246624845677)) ;
#171585=CARTESIAN_POINT('Ctrl Pts',(-26.0332898940312,-13.8041981863265,
112.313128143188)) ;
#171586=CARTESIAN_POINT('Ctrl Pts',(-26.1070937245407,-13.8041980860306,
112.288897062179)) ;
#171587=CARTESIAN_POINT('Ctrl Pts',(-26.1808975550502,-13.8041979857347,
112.26466598117)) ;
#171588=CARTESIAN_POINT('Ctrl Pts',(-26.1590634058903,-13.8335757561575,
112.198162683659)) ;
#171589=CARTESIAN_POINT('Ctrl Pts',(-26.1372292567303,-13.8629535265802,
112.131659386148)) ;
#171590=CARTESIAN_POINT('Ctrl Pts',(-26.0634254262208,-13.8629536268761,
112.155890467157)) ;
#171591=CARTESIAN_POINT('Ctrl Pts',(-25.9896215957114,-13.8629537271721,
112.180121548166)) ;
#171592=CARTESIAN_POINT('Ctrl Pts',(-26.0114557448713,-13.8335759567493,
112.246624845677)) ;
#171593=CARTESIAN_POINT('Ctrl Pts',(-25.9988451272596,-13.5504534645936,
112.172558837349)) ;
#171594=CARTESIAN_POINT('Ctrl Pts',(-26.0223300636128,-13.5407982837148,
112.244090166275)) ;
#171595=CARTESIAN_POINT('Ctrl Pts',(-26.0961339029924,-13.540798177125,
112.219859112283)) ;
#171596=CARTESIAN_POINT('Ctrl Pts',(-26.1699377423721,-13.5407980705352,
112.195628058292)) ;
#171597=CARTESIAN_POINT('Ctrl Pts',(-26.1464528060189,-13.5504532514139,
112.124096729365)) ;
#171598=CARTESIAN_POINT('Ctrl Pts',(-26.1229678696658,-13.5601084322927,
112.052565400439)) ;
#171599=CARTESIAN_POINT('Ctrl Pts',(-26.0491640302861,-13.5601085388825,
112.076796454431)) ;
#171600=CARTESIAN_POINT('Ctrl Pts',(-25.9753601909065,-13.5601086454724,
112.101027508423)) ;
#171601=CARTESIAN_POINT('Ctrl Pts',(-25.9988451272596,-13.5504534645936,
112.172558837349)) ;
#171602=CARTESIAN_POINT('Ctrl Pts',(-26.0103230578241,-13.261274370137,
112.172300104021)) ;
#171603=CARTESIAN_POINT('Ctrl Pts',(-26.0337701125521,-13.2717947138784,
112.2437160516)) ;
#171604=CARTESIAN_POINT('Ctrl Pts',(-26.107573960794,-13.2717946091373,
112.219485024601)) ;
#171605=CARTESIAN_POINT('Ctrl Pts',(-26.1813778090358,-13.2717945043963,
112.195253997602)) ;
#171606=CARTESIAN_POINT('Ctrl Pts',(-26.1579307543078,-13.2612741606549,
112.123838050023)) ;
#171607=CARTESIAN_POINT('Ctrl Pts',(-26.1344836995798,-13.2507538169135,
112.052422102443)) ;
#171608=CARTESIAN_POINT('Ctrl Pts',(-26.060679851338,-13.2507539216545,
112.076653129442)) ;
#171609=CARTESIAN_POINT('Ctrl Pts',(-25.9868760030961,-13.2507540263956,
112.100884156441)) ;
#171610=CARTESIAN_POINT('Ctrl Pts',(-26.0103230578241,-13.261274370137,
112.172300104021)) ;
#171611=CARTESIAN_POINT('Ctrl Pts',(-26.045879708841,-12.9807689853667,
112.245060234104)) ;
#171612=CARTESIAN_POINT('Ctrl Pts',(-26.0676147705679,-13.0108889686765,
112.31126172717)) ;
#171613=CARTESIAN_POINT('Ctrl Pts',(-26.1414186269613,-13.0108888747282,
112.287030724999)) ;
#171614=CARTESIAN_POINT('Ctrl Pts',(-26.2152224833546,-13.0108887807799,
112.262799722828)) ;
#171615=CARTESIAN_POINT('Ctrl Pts',(-26.1934874216277,-12.9807687974702,
112.196598229762)) ;
#171616=CARTESIAN_POINT('Ctrl Pts',(-26.1717523599008,-12.9506488141604,
112.130396736695)) ;
#171617=CARTESIAN_POINT('Ctrl Pts',(-26.0979485035075,-12.9506489081087,
112.154627738866)) ;
#171618=CARTESIAN_POINT('Ctrl Pts',(-26.0241446471141,-12.950649002057,
112.178858741037)) ;
#171619=CARTESIAN_POINT('Ctrl Pts',(-26.045879708841,-12.9807689853667,
112.245060234104)) ;
#171620=CARTESIAN_POINT('Ctrl Pts',(-26.1036567739015,-12.7323944980461,
112.385605838434)) ;
#171621=CARTESIAN_POINT('Ctrl Pts',(-26.1221237155167,-12.7799004526929,
112.441853164873)) ;
#171622=CARTESIAN_POINT('Ctrl Pts',(-26.195927578452,-12.7799003762679,
112.417622182628)) ;
#171623=CARTESIAN_POINT('Ctrl Pts',(-26.2697314413873,-12.7799002998429,
112.393391200382)) ;
#171624=CARTESIAN_POINT('Ctrl Pts',(-26.2512644997721,-12.7323943451961,
112.337143873943)) ;
#171625=CARTESIAN_POINT('Ctrl Pts',(-26.2327975581568,-12.6848883905494,
112.280896547504)) ;
#171626=CARTESIAN_POINT('Ctrl Pts',(-26.1589936952215,-12.6848884669744,
112.305127529749)) ;
#171627=CARTESIAN_POINT('Ctrl Pts',(-26.0851898322863,-12.6848885433994,
112.329358511994)) ;
#171628=CARTESIAN_POINT('Ctrl Pts',(-26.1036567739015,-12.7323944980461,
112.385605838434)) ;
#171629=CARTESIAN_POINT('Ctrl Pts',(-26.1804617683959,-12.5325218808407,
112.58401318597)) ;
#171630=CARTESIAN_POINT('Ctrl Pts',(-26.1943293123753,-12.594053905958,
112.626251489216)) ;
#171631=CARTESIAN_POINT('Ctrl Pts',(-26.2681331796008,-12.5940538521665,
112.602020520038)) ;
#171632=CARTESIAN_POINT('Ctrl Pts',(-26.3419370468262,-12.594053798375,
112.57778955086)) ;
#171633=CARTESIAN_POINT('Ctrl Pts',(-26.3280695028469,-12.5325217732577,
112.535551247613)) ;
#171634=CARTESIAN_POINT('Ctrl Pts',(-26.3142019588674,-12.4709897481403,
112.493312944367)) ;
#171635=CARTESIAN_POINT('Ctrl Pts',(-26.240398091642,-12.4709898019318,
112.517543913545)) ;
#171636=CARTESIAN_POINT('Ctrl Pts',(-26.1665942244165,-12.4709898557234,
112.541774882723)) ;
#171637=CARTESIAN_POINT('Ctrl Pts',(-26.1804617683959,-12.5325218808407,
112.58401318597)) ;
#171638=CARTESIAN_POINT('Ctrl Pts',(-26.2714753234597,-12.3964669498525,
112.825699877311)) ;
#171639=CARTESIAN_POINT('Ctrl Pts',(-26.2797444860816,-12.4675909509527,
112.850886414112)) ;
#171640=CARTESIAN_POINT('Ctrl Pts',(-26.3535483549948,-12.4675909216126,
112.826655450075)) ;
#171641=CARTESIAN_POINT('Ctrl Pts',(-26.427352223908,-12.4675908922725,
112.802424486037)) ;
#171642=CARTESIAN_POINT('Ctrl Pts',(-26.4190830612861,-12.3964668911723,
112.777237949236)) ;
#171643=CARTESIAN_POINT('Ctrl Pts',(-26.4108138986641,-12.3253428900721,
112.752051412436)) ;
#171644=CARTESIAN_POINT('Ctrl Pts',(-26.3370100297509,-12.3253429194122,
112.776282376473)) ;
#171645=CARTESIAN_POINT('Ctrl Pts',(-26.2632061608377,-12.3253429487523,
112.800513340511)) ;
#171646=CARTESIAN_POINT('Ctrl Pts',(-26.2714753234597,-12.3964669498525,
112.825699877311)) ;
#171647=CARTESIAN_POINT('Ctrl Pts',(-26.3703204549318,-12.3339203423186,
113.09142883813)) ;
#171648=CARTESIAN_POINT('Ctrl Pts',(-26.3724319867978,-12.4095182646376,
113.097860225065)) ;
#171649=CARTESIAN_POINT('Ctrl Pts',(-26.4462358554049,-12.4095182584409,
113.073629260095)) ;
#171650=CARTESIAN_POINT('Ctrl Pts',(-26.5200397240119,-12.4095182522441,
113.049398295125)) ;
#171651=CARTESIAN_POINT('Ctrl Pts',(-26.5179281921459,-12.3339203299251,
113.04296690819)) ;
#171652=CARTESIAN_POINT('Ctrl Pts',(-26.5158166602798,-12.2583224076062,
113.036535521254)) ;
#171653=CARTESIAN_POINT('Ctrl Pts',(-26.4420127916727,-12.2583224138029,
113.060766486224)) ;
#171654=CARTESIAN_POINT('Ctrl Pts',(-26.3682089230657,-12.2583224199996,
113.084997451194)) ;
#171655=CARTESIAN_POINT('Ctrl Pts',(-26.3703204549318,-12.3339203423186,
113.09142883813)) ;
#171656=CARTESIAN_POINT('Ctrl Pts',(-26.4715172701898,-12.3484596551531,
113.36420418221)) ;
#171657=CARTESIAN_POINT('Ctrl Pts',(-26.467300144392,-12.4231567143316,
113.351359498885)) ;
#171658=CARTESIAN_POINT('Ctrl Pts',(-26.5411040103548,-12.423156728635,
113.327128525861)) ;
#171659=CARTESIAN_POINT('Ctrl Pts',(-26.6149078763176,-12.4231567429385,
113.302897552837)) ;
#171660=CARTESIAN_POINT('Ctrl Pts',(-26.6191250021153,-12.34845968376,113.315742236161)) ;
#171661=CARTESIAN_POINT('Ctrl Pts',(-26.6233421279131,-12.2737626245815,
113.328586919486)) ;
#171662=CARTESIAN_POINT('Ctrl Pts',(-26.5495382619503,-12.2737626102781,
113.35281789251)) ;
#171663=CARTESIAN_POINT('Ctrl Pts',(-26.4757343959875,-12.2737625959746,
113.377048865534)) ;
#171664=CARTESIAN_POINT('Ctrl Pts',(-26.4715172701898,-12.3484596551531,
113.36420418221)) ;
#171665=CARTESIAN_POINT('Ctrl Pts',(-26.5685528855363,-12.44015832593,113.624188802472)) ;
#171666=CARTESIAN_POINT('Ctrl Pts',(-26.5582903689325,-12.5085664478243,
113.592930833998)) ;
#171667=CARTESIAN_POINT('Ctrl Pts',(-26.6320942303672,-12.508566476899,
113.568699847182)) ;
#171668=CARTESIAN_POINT('Ctrl Pts',(-26.705898091802,-12.5085665059736,
113.544468860367)) ;
#171669=CARTESIAN_POINT('Ctrl Pts',(-26.7161606084058,-12.4401583840793,
113.575726828841)) ;
#171670=CARTESIAN_POINT('Ctrl Pts',(-26.7264231250096,-12.371750262185,
113.606984797315)) ;
#171671=CARTESIAN_POINT('Ctrl Pts',(-26.6526192635749,-12.3717502331104,
113.631215784131)) ;
#171672=CARTESIAN_POINT('Ctrl Pts',(-26.5788154021401,-12.3717502040357,
113.655446770947)) ;
#171673=CARTESIAN_POINT('Ctrl Pts',(-26.5685528855363,-12.44015832593,113.624188802472)) ;
#171674=CARTESIAN_POINT('Ctrl Pts',(-26.6546342110012,-12.6016814204418,
113.8509185553)) ;
#171675=CARTESIAN_POINT('Ctrl Pts',(-26.6390796449447,-12.6589156114348,
113.803541857899)) ;
#171676=CARTESIAN_POINT('Ctrl Pts',(-26.7128835013392,-12.6589156492429,
113.779310855731)) ;
#171677=CARTESIAN_POINT('Ctrl Pts',(-26.7866873577338,-12.6589156870509,
113.755079853564)) ;
#171678=CARTESIAN_POINT('Ctrl Pts',(-26.8022419237903,-12.6016814960579,
113.802456550965)) ;
#171679=CARTESIAN_POINT('Ctrl Pts',(-26.8177964898467,-12.5444473050649,
113.849833248366)) ;
#171680=CARTESIAN_POINT('Ctrl Pts',(-26.7439926334522,-12.5444472672568,
113.874064250533)) ;
#171681=CARTESIAN_POINT('Ctrl Pts',(-26.6701887770576,-12.5444472294488,
113.898295252701)) ;
#171682=CARTESIAN_POINT('Ctrl Pts',(-26.6546342110012,-12.6016814204418,
113.8509185553)) ;
#171683=CARTESIAN_POINT('Ctrl Pts',(-26.7247862104349,-12.8223735055108,
114.029031451425)) ;
#171684=CARTESIAN_POINT('Ctrl Pts',(-26.7050456747767,-12.8642856579198,
113.968904965835)) ;
#171685=CARTESIAN_POINT('Ctrl Pts',(-26.7788495259499,-12.8642856973606,
113.944673947764)) ;
#171686=CARTESIAN_POINT('Ctrl Pts',(-26.8526533771231,-12.8642857368014,
113.920442929693)) ;
#171687=CARTESIAN_POINT('Ctrl Pts',(-26.8723939127814,-12.8223735843924,
113.980569415283)) ;
#171688=CARTESIAN_POINT('Ctrl Pts',(-26.8921344484396,-12.7804614319833,
114.040695900874)) ;
#171689=CARTESIAN_POINT('Ctrl Pts',(-26.8183305972664,-12.7804613925425,
114.064926918944)) ;
#171690=CARTESIAN_POINT('Ctrl Pts',(-26.7445267460932,-12.7804613531017,
114.089157937015)) ;
#171691=CARTESIAN_POINT('Ctrl Pts',(-26.7247862104349,-12.8223735055108,
114.029031451425)) ;
#171692=CARTESIAN_POINT('Ctrl Pts',(-26.7742244447704,-13.0840251447648,
114.144298922302)) ;
#171693=CARTESIAN_POINT('Ctrl Pts',(-26.7517329509008,-13.1077315684995,
114.075793461726)) ;
#171694=CARTESIAN_POINT('Ctrl Pts',(-26.8255367978803,-13.1077316062093,
114.051562430882)) ;
#171695=CARTESIAN_POINT('Ctrl Pts',(-26.8993406448597,-13.1077316439191,
114.027331400038)) ;
#171696=CARTESIAN_POINT('Ctrl Pts',(-26.9218321387293,-13.0840252201844,
114.095836860614)) ;
#171697=CARTESIAN_POINT('Ctrl Pts',(-26.9443236325989,-13.0603187964498,
114.16434232119)) ;
#171698=CARTESIAN_POINT('Ctrl Pts',(-26.8705197856195,-13.06031875874,114.188573352034)) ;
#171699=CARTESIAN_POINT('Ctrl Pts',(-26.79671593864,-13.0603187210301,114.212804382878)) ;
#171700=CARTESIAN_POINT('Ctrl Pts',(-26.7742244447704,-13.0840251447648,
114.144298922302)) ;
#171701=CARTESIAN_POINT('Ctrl Pts',(-26.8008417401105,-13.370624374638,
114.189901457534)) ;
#171702=CARTESIAN_POINT('Ctrl Pts',(-26.777191620752,-13.3743556073404,
114.117867010496)) ;
#171703=CARTESIAN_POINT('Ctrl Pts',(-26.8509954643287,-13.3743556381557,
114.093635969288)) ;
#171704=CARTESIAN_POINT('Ctrl Pts',(-26.9247993079053,-13.3743556689709,
114.069404928079)) ;
#171705=CARTESIAN_POINT('Ctrl Pts',(-26.9484494272638,-13.3706244362685,
114.141439375117)) ;
#171706=CARTESIAN_POINT('Ctrl Pts',(-26.9720995466223,-13.3668932035661,
114.213473822155)) ;
#171707=CARTESIAN_POINT('Ctrl Pts',(-26.8982957030456,-13.3668931727509,
114.237704863364)) ;
#171708=CARTESIAN_POINT('Ctrl Pts',(-26.8244918594689,-13.3668931419356,
114.261935904572)) ;
#171709=CARTESIAN_POINT('Ctrl Pts',(-26.8008417401105,-13.370624374638,
114.189901457534)) ;
#171710=CARTESIAN_POINT('Ctrl Pts',(-26.8030999803076,-13.6607958553262,
114.161291000141)) ;
#171711=CARTESIAN_POINT('Ctrl Pts',(-26.7799907261469,-13.6442717980086,
114.090903941066)) ;
#171712=CARTESIAN_POINT('Ctrl Pts',(-26.8537945677839,-13.6442718197528,
114.066672893949)) ;
#171713=CARTESIAN_POINT('Ctrl Pts',(-26.927598409421,-13.6442718414971,
114.042441846833)) ;
#171714=CARTESIAN_POINT('Ctrl Pts',(-26.9507076635816,-13.6607958988147,
114.112828905908)) ;
#171715=CARTESIAN_POINT('Ctrl Pts',(-26.9738169177423,-13.6773199561323,
114.183215964983)) ;
#171716=CARTESIAN_POINT('Ctrl Pts',(-26.9000130761053,-13.6773199343881,
114.207447012099)) ;
#171717=CARTESIAN_POINT('Ctrl Pts',(-26.8262092344683,-13.6773199126438,
114.231678059216)) ;
#171718=CARTESIAN_POINT('Ctrl Pts',(-26.8030999803076,-13.6607958553262,
114.161291000141)) ;
#171719=CARTESIAN_POINT('Ctrl Pts',(-26.7817312465355,-13.9332273193549,
114.060772562073)) ;
#171720=CARTESIAN_POINT('Ctrl Pts',(-26.7608123616796,-13.8976559253995,
113.997057014344)) ;
#171721=CARTESIAN_POINT('Ctrl Pts',(-26.8346162026608,-13.8976559384048,
113.97282596523)) ;
#171722=CARTESIAN_POINT('Ctrl Pts',(-26.908420043642,-13.8976559514102,
113.948594916116)) ;
#171723=CARTESIAN_POINT('Ctrl Pts',(-26.9293389284979,-13.9332273453655,
114.012310463845)) ;
#171724=CARTESIAN_POINT('Ctrl Pts',(-26.9502578133537,-13.9687987393209,
114.076026011573)) ;
#171725=CARTESIAN_POINT('Ctrl Pts',(-26.8764539723725,-13.9687987263155,
114.100257060687)) ;
#171726=CARTESIAN_POINT('Ctrl Pts',(-26.8026501313913,-13.9687987133102,
114.124488109801)) ;
#171727=CARTESIAN_POINT('Ctrl Pts',(-26.7817312465355,-13.9332273193549,
114.060772562073)) ;
#171728=CARTESIAN_POINT('Ctrl Pts',(-26.7386891506316,-14.1696161307288,
113.894076690003)) ;
#171729=CARTESIAN_POINT('Ctrl Pts',(-26.7214807529589,-14.117484643747,
113.841662687406)) ;
#171730=CARTESIAN_POINT('Ctrl Pts',(-26.7952845945881,-14.1174846489895,
113.817431640266)) ;
#171731=CARTESIAN_POINT('Ctrl Pts',(-26.8690884362173,-14.117484654232,
113.793200593126)) ;
#171732=CARTESIAN_POINT('Ctrl Pts',(-26.88629683389,-14.1696161412137,113.845614595723)) ;
#171733=CARTESIAN_POINT('Ctrl Pts',(-26.9035052315627,-14.2217476281955,
113.89802859832)) ;
#171734=CARTESIAN_POINT('Ctrl Pts',(-26.8297013899335,-14.221747622953,
113.92225964546)) ;
#171735=CARTESIAN_POINT('Ctrl Pts',(-26.7558975483042,-14.2217476177105,
113.9464906926)) ;
#171736=CARTESIAN_POINT('Ctrl Pts',(-26.7386891506316,-14.1696161307288,
113.894076690003)) ;
#171737=CARTESIAN_POINT('Ctrl Pts',(-26.6786437912351,-14.3504842744957,
113.675940625879)) ;
#171738=CARTESIAN_POINT('Ctrl Pts',(-26.6663317358567,-14.285645743084,
113.638440091808)) ;
#171739=CARTESIAN_POINT('Ctrl Pts',(-26.7401355782558,-14.2856457445399,
113.614209047013)) ;
#171740=CARTESIAN_POINT('Ctrl Pts',(-26.8139394206549,-14.2856457459958,
113.589978002218)) ;
#171741=CARTESIAN_POINT('Ctrl Pts',(-26.8262514760333,-14.3504842774075,
113.627478536289)) ;
#171742=CARTESIAN_POINT('Ctrl Pts',(-26.8385635314116,-14.4153228088192,
113.66497907036)) ;
#171743=CARTESIAN_POINT('Ctrl Pts',(-26.7647596890125,-14.4153228073633,
113.689210115155)) ;
#171744=CARTESIAN_POINT('Ctrl Pts',(-26.6909558466134,-14.4153228059074,
113.71344115995)) ;
#171745=CARTESIAN_POINT('Ctrl Pts',(-26.6786437912351,-14.3504842744957,
113.675940625879)) ;
#171746=CARTESIAN_POINT('Ctrl Pts',(-26.6051960375763,-14.4664314373378,
113.416506558969)) ;
#171747=CARTESIAN_POINT('Ctrl Pts',(-26.5987335697604,-14.393398523113,
113.396822924687)) ;
#171748=CARTESIAN_POINT('Ctrl Pts',(-26.6725374136152,-14.3933985223856,
113.372591884325)) ;
#171749=CARTESIAN_POINT('Ctrl Pts',(-26.7463412574701,-14.3933985216583,
113.348360843964)) ;
#171750=CARTESIAN_POINT('Ctrl Pts',(-26.752803725286,-14.4664314358832,
113.368044478246)) ;
#171751=CARTESIAN_POINT('Ctrl Pts',(-26.7592661931018,-14.539464350108,
113.387728112529)) ;
#171752=CARTESIAN_POINT('Ctrl Pts',(-26.685462349247,-14.5394643508353,
113.41195915289)) ;
#171753=CARTESIAN_POINT('Ctrl Pts',(-26.6116585053922,-14.5394643515627,
113.436190193252)) ;
#171754=CARTESIAN_POINT('Ctrl Pts',(-26.6051960375763,-14.4664314373378,
113.416506558969)) ;
#171755=CARTESIAN_POINT('Ctrl Pts',(-26.5259715366712,-14.505814940549,
113.139853747979)) ;
#171756=CARTESIAN_POINT('Ctrl Pts',(-26.5257630868686,-14.4299235771365,
113.139218843456)) ;
#171757=CARTESIAN_POINT('Ctrl Pts',(-26.5995669312173,-14.4299235770663,
113.114987804598)) ;
#171758=CARTESIAN_POINT('Ctrl Pts',(-26.673370775566,-14.429923576996,113.090756765741)) ;
#171759=CARTESIAN_POINT('Ctrl Pts',(-26.6735792253686,-14.5058149404085,
113.091391670264)) ;
#171760=CARTESIAN_POINT('Ctrl Pts',(-26.6737876751712,-14.5817063038209,
113.092026574788)) ;
#171761=CARTESIAN_POINT('Ctrl Pts',(-26.5999838308225,-14.5817063038912,
113.116257613645)) ;
#171762=CARTESIAN_POINT('Ctrl Pts',(-26.5261799864738,-14.5817063039614,
113.140488652502)) ;
#171763=CARTESIAN_POINT('Ctrl Pts',(-26.5259715366712,-14.505814940549,
113.139853747979)) ;
#171764=CARTESIAN_POINT('Ctrl Pts',(-26.4466835012553,-14.46830400306,112.863009454041)) ;
#171765=CARTESIAN_POINT('Ctrl Pts',(-26.4527427661064,-14.3949198444241,
112.881464997054)) ;
#171766=CARTESIAN_POINT('Ctrl Pts',(-26.5265466105033,-14.3949198453838,
112.857233958344)) ;
#171767=CARTESIAN_POINT('Ctrl Pts',(-26.6003504549002,-14.3949198463436,
112.833002919634)) ;
#171768=CARTESIAN_POINT('Ctrl Pts',(-26.5942911900492,-14.4683040049795,
112.81454737662)) ;
#171769=CARTESIAN_POINT('Ctrl Pts',(-26.5882319251982,-14.5416881636154,
112.796091833607)) ;
#171770=CARTESIAN_POINT('Ctrl Pts',(-26.5144280808013,-14.5416881626556,
112.820322872317)) ;
#171771=CARTESIAN_POINT('Ctrl Pts',(-26.4406242364043,-14.5416881616959,
112.844553911027)) ;
#171772=CARTESIAN_POINT('Ctrl Pts',(-26.4466835012553,-14.46830400306,112.863009454041)) ;
#171773=CARTESIAN_POINT('Ctrl Pts',(-26.3730710354797,-14.3544455833434,
112.603124137994)) ;
#171774=CARTESIAN_POINT('Ctrl Pts',(-26.3850179196596,-14.28890351008,112.639512419572)) ;
#171775=CARTESIAN_POINT('Ctrl Pts',(-26.458821763171,-14.2889035106551,
112.615281378165)) ;
#171776=CARTESIAN_POINT('Ctrl Pts',(-26.5326256066825,-14.2889035112301,
112.591050336758)) ;
#171777=CARTESIAN_POINT('Ctrl Pts',(-26.5206787225026,-14.3544455844935,
112.554662055179)) ;
#171778=CARTESIAN_POINT('Ctrl Pts',(-26.5087318383227,-14.4199876577569,
112.518273773601)) ;
#171779=CARTESIAN_POINT('Ctrl Pts',(-26.4349279948113,-14.4199876571819,
112.542504815008)) ;
#171780=CARTESIAN_POINT('Ctrl Pts',(-26.3611241512998,-14.4199876566068,
112.566735856416)) ;
#171781=CARTESIAN_POINT('Ctrl Pts',(-26.3730710354797,-14.3544455833434,
112.603124137994)) ;
#171782=CARTESIAN_POINT('Ctrl Pts',(-26.3124728977524,-14.1743504235921,
112.383177448969)) ;
#171783=CARTESIAN_POINT('Ctrl Pts',(-26.3294005699097,-14.1212879349947,
112.434736407154)) ;
#171784=CARTESIAN_POINT('Ctrl Pts',(-26.4032044125281,-14.121287932882,
112.410505363027)) ;
#171785=CARTESIAN_POINT('Ctrl Pts',(-26.4770082551464,-14.1212879307693,
112.386274318899)) ;
#171786=CARTESIAN_POINT('Ctrl Pts',(-26.4600805829891,-14.1743504193667,
112.334715360714)) ;
#171787=CARTESIAN_POINT('Ctrl Pts',(-26.4431529108318,-14.2274129079642,
112.283156402529)) ;
#171788=CARTESIAN_POINT('Ctrl Pts',(-26.3693490682134,-14.2274129100769,
112.307387446657)) ;
#171789=CARTESIAN_POINT('Ctrl Pts',(-26.295545225595,-14.2274129121895,
112.331618490784)) ;
#171790=CARTESIAN_POINT('Ctrl Pts',(-26.3124728977524,-14.1743504235921,
112.383177448969)) ;
#171791=CARTESIAN_POINT('Ctrl Pts',(-26.2691441762916,-13.9404023706078,
112.215800956528)) ;
#171792=CARTESIAN_POINT('Ctrl Pts',(-26.2898545563157,-13.9035978670998,
112.278881432632)) ;
#171793=CARTESIAN_POINT('Ctrl Pts',(-26.3636583983287,-13.903597860184,
112.254650386661)) ;
#171794=CARTESIAN_POINT('Ctrl Pts',(-26.4374622403416,-13.9035978532681,
112.23041934069)) ;
#171795=CARTESIAN_POINT('Ctrl Pts',(-26.4167518603175,-13.940402356776,
112.167338864585)) ;
#171796=CARTESIAN_POINT('Ctrl Pts',(-26.3960414802934,-13.977206860284,
112.10425838848)) ;
#171797=CARTESIAN_POINT('Ctrl Pts',(-26.3222376382805,-13.9772068671999,
112.128489434452)) ;
#171798=CARTESIAN_POINT('Ctrl Pts',(-26.2484337962675,-13.9772068741157,
112.152720480423)) ;
#171799=CARTESIAN_POINT('Ctrl Pts',(-26.2691441762916,-13.9404023706078,
112.215800956528)) ;
#171800=CARTESIAN_POINT('Ctrl Pts',(-26.2470669365409,-13.6671888266285,
112.112924558201)) ;
#171801=CARTESIAN_POINT('Ctrl Pts',(-26.27008647726,-13.6494076085659,112.183038365355)) ;
#171802=CARTESIAN_POINT('Ctrl Pts',(-26.3438903193133,-13.6494075929638,
112.158807319507)) ;
#171803=CARTESIAN_POINT('Ctrl Pts',(-26.4176941613665,-13.6494075773616,
112.134576273658)) ;
#171804=CARTESIAN_POINT('Ctrl Pts',(-26.3946746206473,-13.6671887954242,
112.064462466504)) ;
#171805=CARTESIAN_POINT('Ctrl Pts',(-26.3716550799282,-13.6849700134867,
111.994348659349)) ;
#171806=CARTESIAN_POINT('Ctrl Pts',(-26.297851237875,-13.6849700290889,
112.018579705198)) ;
#171807=CARTESIAN_POINT('Ctrl Pts',(-26.2240473958217,-13.684970044691,
112.042810751047)) ;
#171808=CARTESIAN_POINT('Ctrl Pts',(-26.2470669365409,-13.6671888266285,
112.112924558201)) ;
#171809=CARTESIAN_POINT('Ctrl Pts',(-26.248777373754,-13.3783758394987,
112.082794816685)) ;
#171810=CARTESIAN_POINT('Ctrl Pts',(-26.2724420195243,-13.3807343880949,
112.154873509865)) ;
#171811=CARTESIAN_POINT('Ctrl Pts',(-26.3462458630014,-13.3807343653365,
112.130642468353)) ;
#171812=CARTESIAN_POINT('Ctrl Pts',(-26.4200497064785,-13.3807343425781,
112.106411426841)) ;
#171813=CARTESIAN_POINT('Ctrl Pts',(-26.3963850607081,-13.3783757939819,
112.034332733661)) ;
#171814=CARTESIAN_POINT('Ctrl Pts',(-26.3727204149377,-13.3760172453858,
111.962254040481)) ;
#171815=CARTESIAN_POINT('Ctrl Pts',(-26.2989165714607,-13.3760172681442,
111.986485081993)) ;
#171816=CARTESIAN_POINT('Ctrl Pts',(-26.2251127279836,-13.3760172909026,
112.010716123505)) ;
#171817=CARTESIAN_POINT('Ctrl Pts',(-26.248777373754,-13.3783758394987,
112.082794816685)) ;
#171818=CARTESIAN_POINT('Ctrl Pts',(-26.2746776385701,-13.0914976589315,
112.126226095536)) ;
#171819=CARTESIAN_POINT('Ctrl Pts',(-26.297301844828,-13.1138898142191,
112.19513577799)) ;
#171820=CARTESIAN_POINT('Ctrl Pts',(-26.3711056909002,-13.113889784642,
112.170904744382)) ;
#171821=CARTESIAN_POINT('Ctrl Pts',(-26.4449095369724,-13.1138897550648,
112.146673710775)) ;
#171822=CARTESIAN_POINT('Ctrl Pts',(-26.4222853307145,-13.0914975997771,
112.07776402832)) ;
#171823=CARTESIAN_POINT('Ctrl Pts',(-26.3996611244566,-13.0691054444894,
112.008854345866)) ;
#171824=CARTESIAN_POINT('Ctrl Pts',(-26.3258572783844,-13.0691054740666,
112.033085379473)) ;
#171825=CARTESIAN_POINT('Ctrl Pts',(-26.2520534323122,-13.0691055036438,
112.057316413081)) ;
#171826=CARTESIAN_POINT('Ctrl Pts',(-26.2746776385701,-13.0914976589315,
112.126226095536)) ;
#171827=CARTESIAN_POINT('Ctrl Pts',(-26.3237843579519,-12.827936357185,
112.24033766308)) ;
#171828=CARTESIAN_POINT('Ctrl Pts',(-26.3437463716241,-12.8687628272745,
112.301138736626)) ;
#171829=CARTESIAN_POINT('Ctrl Pts',(-26.4175502214732,-12.8687627938338,
112.276907714522)) ;
#171830=CARTESIAN_POINT('Ctrl Pts',(-26.4913540713223,-12.868762760393,
112.252676692418)) ;
#171831=CARTESIAN_POINT('Ctrl Pts',(-26.4713920576501,-12.8279362903035,
112.191875618872)) ;
#171832=CARTESIAN_POINT('Ctrl Pts',(-26.4514300439778,-12.7871098202139,
112.131074545326)) ;
#171833=CARTESIAN_POINT('Ctrl Pts',(-26.3776261941287,-12.7871098536547,
112.15530556743)) ;
#171834=CARTESIAN_POINT('Ctrl Pts',(-26.3038223442796,-12.7871098870954,
112.179536589534)) ;
#171835=CARTESIAN_POINT('Ctrl Pts',(-26.3237843579519,-12.827936357185,
112.24033766308)) ;
#171836=CARTESIAN_POINT('Ctrl Pts',(-26.3935111615706,-12.6061166858968,
112.417162681011)) ;
#171837=CARTESIAN_POINT('Ctrl Pts',(-26.4093694433139,-12.662489659223,
112.465464449421)) ;
#171838=CARTESIAN_POINT('Ctrl Pts',(-26.4831732979266,-12.6624896260607,
112.441233441827)) ;
#171839=CARTESIAN_POINT('Ctrl Pts',(-26.5569771525393,-12.6624895928983,
112.417002434232)) ;
#171840=CARTESIAN_POINT('Ctrl Pts',(-26.541118870796,-12.6061166195721,
112.368700665822)) ;
#171841=CARTESIAN_POINT('Ctrl Pts',(-26.5252605890526,-12.5497436462459,
112.320398897411)) ;
#171842=CARTESIAN_POINT('Ctrl Pts',(-26.4514567344399,-12.5497436794083,
112.344629905006)) ;
#171843=CARTESIAN_POINT('Ctrl Pts',(-26.3776528798272,-12.5497437125706,
112.3688609126)) ;
#171844=CARTESIAN_POINT('Ctrl Pts',(-26.3935111615706,-12.6061166858968,
112.417162681011)) ;
#171845=CARTESIAN_POINT('Ctrl Pts',(-26.4793526115935,-12.4431271546039,
112.643138615007)) ;
#171846=CARTESIAN_POINT('Ctrl Pts',(-26.4899747011907,-12.5109613838961,
112.675491787168)) ;
#171847=CARTESIAN_POINT('Ctrl Pts',(-26.5637785606393,-12.510961357698,
112.651260794302)) ;
#171848=CARTESIAN_POINT('Ctrl Pts',(-26.6375824200879,-12.5109613315,112.627029801437)) ;
#171849=CARTESIAN_POINT('Ctrl Pts',(-26.6269603304907,-12.4431271022078,
112.594676629277)) ;
#171850=CARTESIAN_POINT('Ctrl Pts',(-26.6163382408936,-12.3752928729157,
112.562323457116)) ;
#171851=CARTESIAN_POINT('Ctrl Pts',(-26.542534381445,-12.3752928991138,
112.586554449982)) ;
#171852=CARTESIAN_POINT('Ctrl Pts',(-26.4687305219963,-12.3752929253118,
112.610785442847)) ;
#171853=CARTESIAN_POINT('Ctrl Pts',(-26.4793526115935,-12.4431271546039,
112.643138615007)) ;
#171854=CARTESIAN_POINT('Ctrl Pts',(-26.575504511702,-12.3502094912987,
112.900682431856)) ;
#171855=CARTESIAN_POINT('Ctrl Pts',(-26.5801595812379,-12.4246287371788,
112.914861023821)) ;
#171856=CARTESIAN_POINT('Ctrl Pts',(-26.6539634444303,-12.4246287241844,
112.890630042359)) ;
#171857=CARTESIAN_POINT('Ctrl Pts',(-26.7277673076227,-12.42462871119,112.866399060897)) ;
#171858=CARTESIAN_POINT('Ctrl Pts',(-26.7231122380868,-12.35020946531,112.852220468932)) ;
#171859=CARTESIAN_POINT('Ctrl Pts',(-26.7184571685509,-12.2757902194299,
112.838041876967)) ;
#171860=CARTESIAN_POINT('Ctrl Pts',(-26.6446533053586,-12.2757902324242,
112.862272858429)) ;
#171861=CARTESIAN_POINT('Ctrl Pts',(-26.5708494421661,-12.2757902454186,
112.886503839892)) ;
#171862=CARTESIAN_POINT('Ctrl Pts',(-26.575504511702,-12.3502094912987,
112.900682431856)) ;
#171863=CARTESIAN_POINT('Ctrl Pts',(-26.6766988977771,-12.3330949628537,
113.1734359646)) ;
#171864=CARTESIAN_POINT('Ctrl Pts',(-26.6750294757674,-12.4088168292008,
113.168351175927)) ;
#171865=CARTESIAN_POINT('Ctrl Pts',(-26.7488333418635,-12.4088168339974,
113.144120203309)) ;
#171866=CARTESIAN_POINT('Ctrl Pts',(-26.8226372079595,-12.408816838794,
113.119889230691)) ;
#171867=CARTESIAN_POINT('Ctrl Pts',(-26.8243066299692,-12.3330949724469,
113.124974019364)) ;
#171868=CARTESIAN_POINT('Ctrl Pts',(-26.8259760519788,-12.2573731060998,
113.130058808036)) ;
#171869=CARTESIAN_POINT('Ctrl Pts',(-26.7521721858828,-12.2573731013032,
113.154289780654)) ;
#171870=CARTESIAN_POINT('Ctrl Pts',(-26.6783683197867,-12.2573730965066,
113.178520753273)) ;
#171871=CARTESIAN_POINT('Ctrl Pts',(-26.6766988977771,-12.3330949628537,
113.1734359646)) ;
#171872=CARTESIAN_POINT('Ctrl Pts',(-26.7762581210695,-12.3941323979468,
113.441132115041)) ;
#171873=CARTESIAN_POINT('Ctrl Pts',(-26.7683708300388,-12.4657028650143,
113.417108700738)) ;
#171874=CARTESIAN_POINT('Ctrl Pts',(-26.8421746972999,-12.4657028918637,
113.392877731668)) ;
#171875=CARTESIAN_POINT('Ctrl Pts',(-26.915978564561,-12.4657029187131,
113.368646762599)) ;
#171876=CARTESIAN_POINT('Ctrl Pts',(-26.9238658555916,-12.3941324516456,
113.392670176902)) ;
#171877=CARTESIAN_POINT('Ctrl Pts',(-26.9317531466222,-12.3225619845781,
113.416693591205)) ;
#171878=CARTESIAN_POINT('Ctrl Pts',(-26.8579492793612,-12.3225619577287,
113.440924560275)) ;
#171879=CARTESIAN_POINT('Ctrl Pts',(-26.7841454121001,-12.3225619308793,
113.465155529345)) ;
#171880=CARTESIAN_POINT('Ctrl Pts',(-26.7762581210695,-12.3941323979468,
113.441132115041)) ;
#171881=CARTESIAN_POINT('Ctrl Pts',(-26.8671458754654,-12.5280047279255,
113.682585935319)) ;
#171882=CARTESIAN_POINT('Ctrl Pts',(-26.8536336294448,-12.5903323506603,
113.641429815818)) ;
#171883=CARTESIAN_POINT('Ctrl Pts',(-26.9274374951756,-12.5903324003766,
113.617198842087)) ;
#171884=CARTESIAN_POINT('Ctrl Pts',(-27.0012413609064,-12.5903324500929,
113.592967868356)) ;
#171885=CARTESIAN_POINT('Ctrl Pts',(-27.014753606927,-12.5280048273581,
113.634123987858)) ;
#171886=CARTESIAN_POINT('Ctrl Pts',(-27.0282658529477,-12.4656772046233,
113.67528010736)) ;
#171887=CARTESIAN_POINT('Ctrl Pts',(-26.9544619872168,-12.465677154907,
113.699511081091)) ;
#171888=CARTESIAN_POINT('Ctrl Pts',(-26.880658121486,-12.4656771051907,
113.723742054821)) ;
#171889=CARTESIAN_POINT('Ctrl Pts',(-26.8671458754654,-12.5280047279255,
113.682585935319)) ;
#171890=CARTESIAN_POINT('Ctrl Pts',(-26.9443518098183,-12.725823043926,
113.882266526049)) ;
#171891=CARTESIAN_POINT('Ctrl Pts',(-26.9261637118994,-12.7744304923816,
113.82686851623)) ;
#171892=CARTESIAN_POINT('Ctrl Pts',(-26.9999675739472,-12.7744305640523,
113.802637531282)) ;
#171893=CARTESIAN_POINT('Ctrl Pts',(-27.073771435995,-12.7744306357229,
113.778406546333)) ;
#171894=CARTESIAN_POINT('Ctrl Pts',(-27.091959533914,-12.7258231872673,
113.833804556152)) ;
#171895=CARTESIAN_POINT('Ctrl Pts',(-27.1101476318329,-12.6772157388117,
113.889202565971)) ;
#171896=CARTESIAN_POINT('Ctrl Pts',(-27.036343769785,-12.677215667141,113.91343355092)) ;
#171897=CARTESIAN_POINT('Ctrl Pts',(-26.9625399077372,-12.6772155954704,
113.937664535868)) ;
#171898=CARTESIAN_POINT('Ctrl Pts',(-26.9443518098183,-12.725823043926,
113.882266526049)) ;
#171899=CARTESIAN_POINT('Ctrl Pts',(-27.0028790263338,-12.9740366931117,
114.024965068217)) ;
#171900=CARTESIAN_POINT('Ctrl Pts',(-26.9813140704319,-13.0053860395,113.959281693945)) ;
#171901=CARTESIAN_POINT('Ctrl Pts',(-27.0551179265467,-13.0053861296798,
113.935050690925)) ;
#171902=CARTESIAN_POINT('Ctrl Pts',(-27.1289217826615,-13.0053862198596,
113.910819687906)) ;
#171903=CARTESIAN_POINT('Ctrl Pts',(-27.1504867385634,-12.9740368734713,
113.976503062178)) ;
#171904=CARTESIAN_POINT('Ctrl Pts',(-27.1720516944653,-12.942687527083,
114.04218643645)) ;
#171905=CARTESIAN_POINT('Ctrl Pts',(-27.0982478383505,-12.9426874369032,
114.06641743947)) ;
#171906=CARTESIAN_POINT('Ctrl Pts',(-27.0244439822357,-12.9426873467234,
114.090648442489)) ;
#171907=CARTESIAN_POINT('Ctrl Pts',(-27.0028790263338,-12.9740366931117,
114.024965068217)) ;
#171908=CARTESIAN_POINT('Ctrl Pts',(-27.0390249126838,-13.2534633118697,
114.099588598299)) ;
#171909=CARTESIAN_POINT('Ctrl Pts',(-27.015638751867,-13.2653501074278,
114.028358127784)) ;
#171910=CARTESIAN_POINT('Ctrl Pts',(-27.0894426002158,-13.2653502091921,
114.004127101111)) ;
#171911=CARTESIAN_POINT('Ctrl Pts',(-27.1632464485645,-13.2653503109564,
113.979896074437)) ;
#171912=CARTESIAN_POINT('Ctrl Pts',(-27.1866326093813,-13.2534635153983,
114.051126544952)) ;
#171913=CARTESIAN_POINT('Ctrl Pts',(-27.210018770198,-13.2415767198401,
114.122357015466)) ;
#171914=CARTESIAN_POINT('Ctrl Pts',(-27.1362149218493,-13.2415766180759,
114.14658804214)) ;
#171915=CARTESIAN_POINT('Ctrl Pts',(-27.0624110735005,-13.2415765163116,
114.170819068813)) ;
#171916=CARTESIAN_POINT('Ctrl Pts',(-27.0390249126838,-13.2534633118697,
114.099588598299)) ;
#171917=CARTESIAN_POINT('Ctrl Pts',(-27.0511093886364,-13.5448240416985,
114.100900424596)) ;
#171918=CARTESIAN_POINT('Ctrl Pts',(-27.02757960726,-13.5363866538712,114.029232509088)) ;
#171919=CARTESIAN_POINT('Ctrl Pts',(-27.1013834468662,-13.5363867591239,
114.005001455786)) ;
#171920=CARTESIAN_POINT('Ctrl Pts',(-27.1751872864724,-13.5363868643766,
113.980770402484)) ;
#171921=CARTESIAN_POINT('Ctrl Pts',(-27.1987170678488,-13.544824252204,
114.052438317993)) ;
#171922=CARTESIAN_POINT('Ctrl Pts',(-27.2222468492252,-13.5532616400314,
114.124106233501)) ;
#171923=CARTESIAN_POINT('Ctrl Pts',(-27.148443009619,-13.5532615347787,
114.148337286803)) ;
#171924=CARTESIAN_POINT('Ctrl Pts',(-27.0746391700128,-13.553261429526,
114.172568340105)) ;
#171925=CARTESIAN_POINT('Ctrl Pts',(-27.0511093886364,-13.5448240416985,
114.100900424596)) ;
#171926=CARTESIAN_POINT('Ctrl Pts',(-27.0391527832181,-13.8260554927979,
114.029131671761)) ;
#171927=CARTESIAN_POINT('Ctrl Pts',(-27.017154679759,-13.7979711605236,
113.962129000086)) ;
#171928=CARTESIAN_POINT('Ctrl Pts',(-27.0909585105926,-13.7979712603347,
113.937897920064)) ;
#171929=CARTESIAN_POINT('Ctrl Pts',(-27.1647623414261,-13.7979713601458,
113.913666840042)) ;
#171930=CARTESIAN_POINT('Ctrl Pts',(-27.1867604448851,-13.8260556924201,
113.980669511717)) ;
#171931=CARTESIAN_POINT('Ctrl Pts',(-27.2087585483442,-13.8541400246944,
114.047672183392)) ;
#171932=CARTESIAN_POINT('Ctrl Pts',(-27.1349547175107,-13.8541399248833,
114.071903263414)) ;
#171933=CARTESIAN_POINT('Ctrl Pts',(-27.0611508866771,-13.8541398250722,
114.096134343436)) ;
#171934=CARTESIAN_POINT('Ctrl Pts',(-27.0391527832181,-13.8260554927979,
114.029131671761)) ;
#171935=CARTESIAN_POINT('Ctrl Pts',(-27.0044729766098,-14.0796928172426,
113.887914543523)) ;
#171936=CARTESIAN_POINT('Ctrl Pts',(-26.9855998097285,-14.0338589352342,
113.830429924472)) ;
#171937=CARTESIAN_POINT('Ctrl Pts',(-27.0594036325612,-14.033859021297,
113.806198820081)) ;
#171938=CARTESIAN_POINT('Ctrl Pts',(-27.133207455394,-14.0338591073598,
113.78196771569)) ;
#171939=CARTESIAN_POINT('Ctrl Pts',(-27.1520806222753,-14.0796929893683,
113.839452334741)) ;
#171940=CARTESIAN_POINT('Ctrl Pts',(-27.1709537891566,-14.1255268713768,
113.896936953791)) ;
#171941=CARTESIAN_POINT('Ctrl Pts',(-27.0971499663238,-14.1255267853139,
113.921168058182)) ;
#171942=CARTESIAN_POINT('Ctrl Pts',(-27.023346143491,-14.1255266992511,
113.945399162573)) ;
#171943=CARTESIAN_POINT('Ctrl Pts',(-27.0044729766098,-14.0796928172426,
113.887914543523)) ;
#171944=CARTESIAN_POINT('Ctrl Pts',(-26.9509127407255,-14.2840883967328,
113.689505698665)) ;
#171945=CARTESIAN_POINT('Ctrl Pts',(-26.9364810188695,-14.223916620712,
113.64554900453)) ;
#171946=CARTESIAN_POINT('Ctrl Pts',(-27.0102848354058,-14.2239166860408,
113.621317880961)) ;
#171947=CARTESIAN_POINT('Ctrl Pts',(-27.0840886519422,-14.2239167513696,
113.597086757393)) ;
#171948=CARTESIAN_POINT('Ctrl Pts',(-27.0985203737982,-14.2840885273904,
113.641043451527)) ;
#171949=CARTESIAN_POINT('Ctrl Pts',(-27.1129520956543,-14.3442603034112,
113.685000145661)) ;
#171950=CARTESIAN_POINT('Ctrl Pts',(-27.0391482791179,-14.3442602380824,
113.70923126923)) ;
#171951=CARTESIAN_POINT('Ctrl Pts',(-26.9653444625816,-14.3442601727535,
113.733462392799)) ;
#171952=CARTESIAN_POINT('Ctrl Pts',(-26.9509127407255,-14.2840883967328,
113.689505698665)) ;
#171953=CARTESIAN_POINT('Ctrl Pts',(-26.8822296015483,-14.4281001590278,
113.444744206038)) ;
#171954=CARTESIAN_POINT('Ctrl Pts',(-26.8733074115915,-14.3577843512303,
113.41756865708)) ;
#171955=CARTESIAN_POINT('Ctrl Pts',(-26.9471112241109,-14.3577843906291,
113.393337521276)) ;
#171956=CARTESIAN_POINT('Ctrl Pts',(-27.0209150366302,-14.357784430028,
113.369106385472)) ;
#171957=CARTESIAN_POINT('Ctrl Pts',(-27.0298372265869,-14.4281002378256,
113.39628193443)) ;
#171958=CARTESIAN_POINT('Ctrl Pts',(-27.0387594165436,-14.4984160456232,
113.423457483389)) ;
#171959=CARTESIAN_POINT('Ctrl Pts',(-26.9649556040243,-14.4984160062243,
113.447688619193)) ;
#171960=CARTESIAN_POINT('Ctrl Pts',(-26.891151791505,-14.4984159668254,
113.471919754997)) ;
#171961=CARTESIAN_POINT('Ctrl Pts',(-26.8822296015483,-14.4281001590278,
113.444744206038)) ;
#171962=CARTESIAN_POINT('Ctrl Pts',(-26.8046693446462,-14.4990916302809,
113.173055466615)) ;
#171963=CARTESIAN_POINT('Ctrl Pts',(-26.8018824452395,-14.4237145145617,
113.164567022696)) ;
#171964=CARTESIAN_POINT('Ctrl Pts',(-26.8756862564281,-14.4237145258999,
113.140335882838)) ;
#171965=CARTESIAN_POINT('Ctrl Pts',(-26.9494900676167,-14.4237145372381,
113.116104742981)) ;
#171966=CARTESIAN_POINT('Ctrl Pts',(-26.9522769670233,-14.4990916529572,
113.124593186901)) ;
#171967=CARTESIAN_POINT('Ctrl Pts',(-26.95506386643,-14.5744687686764,113.13308163082)) ;
#171968=CARTESIAN_POINT('Ctrl Pts',(-26.8812600552414,-14.5744687573382,
113.157312770678)) ;
#171969=CARTESIAN_POINT('Ctrl Pts',(-26.8074562440528,-14.574468746,113.181543910535)) ;
#171970=CARTESIAN_POINT('Ctrl Pts',(-26.8046693446462,-14.4990916302809,
113.173055466615)) ;
#171971=CARTESIAN_POINT('Ctrl Pts',(-26.7243601583869,-14.4927693074735,
112.892974720862)) ;
#171972=CARTESIAN_POINT('Ctrl Pts',(-26.7279100215133,-14.4177207882231,
112.903787033113)) ;
#171973=CARTESIAN_POINT('Ctrl Pts',(-26.8017138340692,-14.4177207722467,
112.879555897421)) ;
#171974=CARTESIAN_POINT('Ctrl Pts',(-26.8755176466252,-14.4177207562703,
112.855324761728)) ;
#171975=CARTESIAN_POINT('Ctrl Pts',(-26.8719677834988,-14.4927692755206,
112.844512449478)) ;
#171976=CARTESIAN_POINT('Ctrl Pts',(-26.8684179203725,-14.567817794771,
112.833700137227)) ;
#171977=CARTESIAN_POINT('Ctrl Pts',(-26.7946141078165,-14.5678178107474,
112.857931272919)) ;
#171978=CARTESIAN_POINT('Ctrl Pts',(-26.7208102952605,-14.5678178267238,
112.882162408612)) ;
#171979=CARTESIAN_POINT('Ctrl Pts',(-26.7243601583869,-14.4927693074735,
112.892974720862)) ;
#171980=CARTESIAN_POINT('Ctrl Pts',(-26.6478394647209,-14.4094376546516,
112.624441415415)) ;
#171981=CARTESIAN_POINT('Ctrl Pts',(-26.6574709542339,-14.3400945271198,
112.653777380281)) ;
#171982=CARTESIAN_POINT('Ctrl Pts',(-26.7312747705731,-14.3400944873417,
112.629546256112)) ;
#171983=CARTESIAN_POINT('Ctrl Pts',(-26.8050785869124,-14.3400944475637,
112.605315131943)) ;
#171984=CARTESIAN_POINT('Ctrl Pts',(-26.7954470973993,-14.4094375750955,
112.575979167076)) ;
#171985=CARTESIAN_POINT('Ctrl Pts',(-26.7858156078862,-14.4787807026274,
112.54664320221)) ;
#171986=CARTESIAN_POINT('Ctrl Pts',(-26.712011791547,-14.4787807424054,
112.570874326379)) ;
#171987=CARTESIAN_POINT('Ctrl Pts',(-26.6382079752078,-14.4787807821835,
112.595105450548)) ;
#171988=CARTESIAN_POINT('Ctrl Pts',(-26.6478394647209,-14.4094376546516,
112.624441415415)) ;
#171989=CARTESIAN_POINT('Ctrl Pts',(-26.5812947221216,-14.2549673486149,
112.386270724262)) ;
#171990=CARTESIAN_POINT('Ctrl Pts',(-26.5963210143004,-14.1963046294673,
112.432038387488)) ;
#171991=CARTESIAN_POINT('Ctrl Pts',(-26.6701248363186,-14.1963045717546,
112.407807280615)) ;
#171992=CARTESIAN_POINT('Ctrl Pts',(-26.7439286583366,-14.1963045140418,
112.383576173743)) ;
#171993=CARTESIAN_POINT('Ctrl Pts',(-26.7289023661578,-14.2549672331893,
112.337808510517)) ;
#171994=CARTESIAN_POINT('Ctrl Pts',(-26.713876073979,-14.3136299523368,
112.292040847291)) ;
#171995=CARTESIAN_POINT('Ctrl Pts',(-26.6400722519609,-14.3136300100496,
112.316271954164)) ;
#171996=CARTESIAN_POINT('Ctrl Pts',(-26.5662684299428,-14.3136300677624,
112.340503061036)) ;
#171997=CARTESIAN_POINT('Ctrl Pts',(-26.5812947221216,-14.2549673486149,
112.386270724262)) ;
#171998=CARTESIAN_POINT('Ctrl Pts',(-26.5303911941234,-14.0408502140836,
112.195800520988)) ;
#171999=CARTESIAN_POINT('Ctrl Pts',(-26.549727194973,-13.9970485144641,
112.254694861334)) ;
#172000=CARTESIAN_POINT('Ctrl Pts',(-26.6235310236397,-13.9970484457834,
112.230463774713)) ;
#172001=CARTESIAN_POINT('Ctrl Pts',(-26.6973348523065,-13.9970483771027,
112.206232688091)) ;
#172002=CARTESIAN_POINT('Ctrl Pts',(-26.6779988514569,-14.0408500767222,
112.147338347744)) ;
#172003=CARTESIAN_POINT('Ctrl Pts',(-26.6586628506072,-14.0846517763417,
112.088444007397)) ;
#172004=CARTESIAN_POINT('Ctrl Pts',(-26.5848590219405,-14.0846518450224,
112.112675094019)) ;
#172005=CARTESIAN_POINT('Ctrl Pts',(-26.5110551932737,-14.0846519137031,
112.136906180641)) ;
#172006=CARTESIAN_POINT('Ctrl Pts',(-26.5303911941234,-14.0408502140836,
112.195800520988)) ;
#172007=CARTESIAN_POINT('Ctrl Pts',(-26.4993318655355,-13.7824650273217,
112.065794986604)) ;
#172008=CARTESIAN_POINT('Ctrl Pts',(-26.5215981506244,-13.7566374523408,
112.133614499815)) ;
#172009=CARTESIAN_POINT('Ctrl Pts',(-26.5954019862457,-13.7566373798381,
112.109383434376)) ;
#172010=CARTESIAN_POINT('Ctrl Pts',(-26.669205821867,-13.7566373073354,
112.085152368936)) ;
#172011=CARTESIAN_POINT('Ctrl Pts',(-26.6469395367781,-13.7824648823164,
112.017332855726)) ;
#172012=CARTESIAN_POINT('Ctrl Pts',(-26.6246732516892,-13.8082924572973,
111.949513342515)) ;
#172013=CARTESIAN_POINT('Ctrl Pts',(-26.5508694160679,-13.8082925298,111.973744407954)) ;
#172014=CARTESIAN_POINT('Ctrl Pts',(-26.4770655804466,-13.8082926023027,
111.997975473393)) ;
#172015=CARTESIAN_POINT('Ctrl Pts',(-26.4993318655355,-13.7824650273217,
112.065794986604)) ;
#172016=CARTESIAN_POINT('Ctrl Pts',(-26.4911724058639,-13.4963851494492,
112.005340368792)) ;
#172017=CARTESIAN_POINT('Ctrl Pts',(-26.5147789143434,-13.4904923432814,
112.077241986031)) ;
#172018=CARTESIAN_POINT('Ctrl Pts',(-26.5885827564685,-13.4904922758106,
112.053010940401)) ;
#172019=CARTESIAN_POINT('Ctrl Pts',(-26.6623865985935,-13.4904922083398,
112.028779894771)) ;
#172020=CARTESIAN_POINT('Ctrl Pts',(-26.6387800901139,-13.4963850145077,
111.956878277532)) ;
#172021=CARTESIAN_POINT('Ctrl Pts',(-26.6151735816344,-13.5022778206756,
111.884976660293)) ;
#172022=CARTESIAN_POINT('Ctrl Pts',(-26.5413697395093,-13.5022778881464,
111.909207705923)) ;
#172023=CARTESIAN_POINT('Ctrl Pts',(-26.4675658973843,-13.5022779556171,
111.933438751553)) ;
#172024=CARTESIAN_POINT('Ctrl Pts',(-26.4911724058639,-13.4963851494492,
112.005340368792)) ;
#172025=CARTESIAN_POINT('Ctrl Pts',(-26.5072441166408,-13.2068554623175,
112.018962167354)) ;
#172026=CARTESIAN_POINT('Ctrl Pts',(-26.5304952118972,-13.2211688965324,
112.089781253125)) ;
#172027=CARTESIAN_POINT('Ctrl Pts',(-26.6042990591768,-13.2211688373046,
112.065550223195)) ;
#172028=CARTESIAN_POINT('Ctrl Pts',(-26.6781029064563,-13.2211687780768,
112.041319193264)) ;
#172029=CARTESIAN_POINT('Ctrl Pts',(-26.6548518111999,-13.2068553438618,
111.970500107494)) ;
#172030=CARTESIAN_POINT('Ctrl Pts',(-26.6316007159434,-13.1925419096468,
111.899681021723)) ;
#172031=CARTESIAN_POINT('Ctrl Pts',(-26.5577968686638,-13.1925419688746,
111.923912051654)) ;
#172032=CARTESIAN_POINT('Ctrl Pts',(-26.4839930213843,-13.1925420281025,
111.948143081584)) ;
#172033=CARTESIAN_POINT('Ctrl Pts',(-26.5072441166408,-13.2068554623175,
112.018962167354)) ;
#172034=CARTESIAN_POINT('Ctrl Pts',(-26.5471201594015,-12.9311896303103,
112.104939986775)) ;
#172035=CARTESIAN_POINT('Ctrl Pts',(-26.568356499574,-12.9647719930566,
112.169622453471)) ;
#172036=CARTESIAN_POINT('Ctrl Pts',(-26.6421603504602,-12.9647719471212,
112.145391434527)) ;
#172037=CARTESIAN_POINT('Ctrl Pts',(-26.7159642013465,-12.9647719011858,
112.121160415582)) ;
#172038=CARTESIAN_POINT('Ctrl Pts',(-26.694727861174,-12.9311895384395,
112.056477948886)) ;
#172039=CARTESIAN_POINT('Ctrl Pts',(-26.6734915210015,-12.8976071756931,
111.99179548219)) ;
#172040=CARTESIAN_POINT('Ctrl Pts',(-26.5996876701152,-12.8976072216285,
112.016026501135)) ;
#172041=CARTESIAN_POINT('Ctrl Pts',(-26.525883819229,-12.8976072675639,
112.04025752008)) ;
#172042=CARTESIAN_POINT('Ctrl Pts',(-26.5471201594015,-12.9311896303103,
112.104939986775)) ;
#172043=CARTESIAN_POINT('Ctrl Pts',(-26.6089561868409,-12.6901579122719,
112.257741738305)) ;
#172044=CARTESIAN_POINT('Ctrl Pts',(-26.6266427444742,-12.7406206917642,
112.311612139959)) ;
#172045=CARTESIAN_POINT('Ctrl Pts',(-26.7004465968938,-12.7406206607923,
112.287381125685)) ;
#172046=CARTESIAN_POINT('Ctrl Pts',(-26.7742504493134,-12.7406206298204,
112.26315011141)) ;
#172047=CARTESIAN_POINT('Ctrl Pts',(-26.75656389168,-12.6901578503282,112.209279709756)) ;
#172048=CARTESIAN_POINT('Ctrl Pts',(-26.7388773340467,-12.639695070836,
112.155409308102)) ;
#172049=CARTESIAN_POINT('Ctrl Pts',(-26.6650734816271,-12.6396951018078,
112.179640322377)) ;
#172050=CARTESIAN_POINT('Ctrl Pts',(-26.5912696292076,-12.6396951327797,
112.203871336652)) ;
#172051=CARTESIAN_POINT('Ctrl Pts',(-26.6089561868409,-12.6901579122719,
112.257741738305)) ;
#172052=CARTESIAN_POINT('Ctrl Pts',(-26.6885029037196,-12.5020099307821,
112.464646899328)) ;
#172053=CARTESIAN_POINT('Ctrl Pts',(-26.7013942584965,-12.5656860202673,
112.503911886632)) ;
#172054=CARTESIAN_POINT('Ctrl Pts',(-26.775198111099,-12.565686002392,112.479680872915)) ;
#172055=CARTESIAN_POINT('Ctrl Pts',(-26.8490019637015,-12.5656859845167,
112.455449859197)) ;
#172056=CARTESIAN_POINT('Ctrl Pts',(-26.8361106089246,-12.5020098950315,
112.416184871893)) ;
#172057=CARTESIAN_POINT('Ctrl Pts',(-26.8232192541478,-12.4383338055463,
112.376919884588)) ;
#172058=CARTESIAN_POINT('Ctrl Pts',(-26.7494154015452,-12.4383338234216,
112.401150898306)) ;
#172059=CARTESIAN_POINT('Ctrl Pts',(-26.6756115489428,-12.4383338412968,
112.425381912023)) ;
#172060=CARTESIAN_POINT('Ctrl Pts',(-26.6885029037196,-12.5020099307821,
112.464646899328)) ;
#172061=CARTESIAN_POINT('Ctrl Pts',(-26.7819225494163,-12.3786471033838,
112.713516599138)) ;
#172062=CARTESIAN_POINT('Ctrl Pts',(-26.789048763939,-12.451033969766,112.735221899233)) ;
#172063=CARTESIAN_POINT('Ctrl Pts',(-26.8628526146505,-12.4510339632927,
112.710990879756)) ;
#172064=CARTESIAN_POINT('Ctrl Pts',(-26.9366564653619,-12.4510339568193,
112.686759860279)) ;
#172065=CARTESIAN_POINT('Ctrl Pts',(-26.9295302508393,-12.378647090437,
112.665054560184)) ;
#172066=CARTESIAN_POINT('Ctrl Pts',(-26.9224040363165,-12.3062602240548,
112.64334926009)) ;
#172067=CARTESIAN_POINT('Ctrl Pts',(-26.848600185605,-12.3062602305281,
112.667580279567)) ;
#172068=CARTESIAN_POINT('Ctrl Pts',(-26.7747963348935,-12.3062602370015,
112.691811299044)) ;
#172069=CARTESIAN_POINT('Ctrl Pts',(-26.7819225494163,-12.3786471033838,
112.713516599138)) ;
#172070=CARTESIAN_POINT('Ctrl Pts',(-26.8814570402713,-12.3306796608346,
112.981418521478)) ;
#172071=CARTESIAN_POINT('Ctrl Pts',(-26.8823738632145,-12.4065247391554,
112.984211016587)) ;
#172072=CARTESIAN_POINT('Ctrl Pts',(-26.9561777123211,-12.4065247391449,
112.959979992222)) ;
#172073=CARTESIAN_POINT('Ctrl Pts',(-27.0299815614278,-12.4065247391344,
112.935748967856)) ;
#172074=CARTESIAN_POINT('Ctrl Pts',(-27.0290647384846,-12.3306796608136,
112.932956472747)) ;
#172075=CARTESIAN_POINT('Ctrl Pts',(-27.0281479155415,-12.2548345824928,
112.930163977638)) ;
#172076=CARTESIAN_POINT('Ctrl Pts',(-26.9543440664348,-12.2548345825033,
112.954395002003)) ;
#172077=CARTESIAN_POINT('Ctrl Pts',(-26.8805402173282,-12.2548345825139,
112.978626026368)) ;
#172078=CARTESIAN_POINT('Ctrl Pts',(-26.8814570402713,-12.3306796608346,
112.981418521478)) ;
#172079=CARTESIAN_POINT('Ctrl Pts',(-26.9826355598295,-12.360155377245,
113.254016856092)) ;
#172080=CARTESIAN_POINT('Ctrl Pts',(-26.977225112592,-12.4340571826112,
113.23753750698)) ;
#172081=CARTESIAN_POINT('Ctrl Pts',(-27.051028959111,-12.4340571856698,
113.213306474733)) ;
#172082=CARTESIAN_POINT('Ctrl Pts',(-27.1248328056299,-12.4340571887285,
113.189075442486)) ;
#172083=CARTESIAN_POINT('Ctrl Pts',(-27.1302432528673,-12.3601553833623,
113.205554791598)) ;
#172084=CARTESIAN_POINT('Ctrl Pts',(-27.1356537001047,-12.2862535779961,
113.22203414071)) ;
#172085=CARTESIAN_POINT('Ctrl Pts',(-27.0618498535858,-12.2862535749374,
113.246265172957)) ;
#172086=CARTESIAN_POINT('Ctrl Pts',(-26.9880460070669,-12.2862535718788,
113.270496205204)) ;
#172087=CARTESIAN_POINT('Ctrl Pts',(-26.9826355598295,-12.360155377245,
113.254016856092)) ;
#172088=CARTESIAN_POINT('Ctrl Pts',(-27.077657915506,-12.4653999327267,
113.508037936239)) ;
#172089=CARTESIAN_POINT('Ctrl Pts',(-27.0663369176674,-12.5320640126139,
113.473556003555)) ;
#172090=CARTESIAN_POINT('Ctrl Pts',(-27.1401407623689,-12.5320640153815,
113.449324965773)) ;
#172091=CARTESIAN_POINT('Ctrl Pts',(-27.2139446070704,-12.5320640181491,
113.42509392799)) ;
#172092=CARTESIAN_POINT('Ctrl Pts',(-27.225265604909,-12.4653999382619,
113.459575860674)) ;
#172093=CARTESIAN_POINT('Ctrl Pts',(-27.2365866027476,-12.3987358583746,
113.494057793358)) ;
#172094=CARTESIAN_POINT('Ctrl Pts',(-27.1627827580461,-12.398735855607,
113.51828883114)) ;
#172095=CARTESIAN_POINT('Ctrl Pts',(-27.0889789133446,-12.3987358528394,
113.542519868923)) ;
#172096=CARTESIAN_POINT('Ctrl Pts',(-27.077657915506,-12.4653999327267,
113.508037936239)) ;
#172097=CARTESIAN_POINT('Ctrl Pts',(-27.1610926480351,-12.6388027493961,
113.726711458191)) ;
#172098=CARTESIAN_POINT('Ctrl Pts',(-27.1446624041515,-12.6934585985942,
113.67666758634)) ;
#172099=CARTESIAN_POINT('Ctrl Pts',(-27.2184662475862,-12.6934585991624,
113.652436544699)) ;
#172100=CARTESIAN_POINT('Ctrl Pts',(-27.2922700910208,-12.6934585997305,
113.628205503058)) ;
#172101=CARTESIAN_POINT('Ctrl Pts',(-27.3087003349045,-12.6388027505324,
113.678249374909)) ;
#172102=CARTESIAN_POINT('Ctrl Pts',(-27.3251305787881,-12.5841469013344,
113.728293246759)) ;
#172103=CARTESIAN_POINT('Ctrl Pts',(-27.2513267353534,-12.5841469007662,
113.7525242884)) ;
#172104=CARTESIAN_POINT('Ctrl Pts',(-27.1775228919187,-12.584146900198,
113.776755330041)) ;
#172105=CARTESIAN_POINT('Ctrl Pts',(-27.1610926480351,-12.6388027493961,
113.726711458191)) ;
#172106=CARTESIAN_POINT('Ctrl Pts',(-27.2275682495383,-12.8679196576227,
113.893744616973)) ;
#172107=CARTESIAN_POINT('Ctrl Pts',(-27.2072050678216,-12.9066583901742,
113.831721651003)) ;
#172108=CARTESIAN_POINT('Ctrl Pts',(-27.281008910791,-12.9066583881138,
113.807490607945)) ;
#172109=CARTESIAN_POINT('Ctrl Pts',(-27.3548127537603,-12.9066583860534,
113.783259564886)) ;
#172110=CARTESIAN_POINT('Ctrl Pts',(-27.3751759354771,-12.8679196535019,
113.845282530856)) ;
#172111=CARTESIAN_POINT('Ctrl Pts',(-27.3955391171939,-12.8291809209503,
113.907305496826)) ;
#172112=CARTESIAN_POINT('Ctrl Pts',(-27.3217352742245,-12.8291809230107,
113.931536539885)) ;
#172113=CARTESIAN_POINT('Ctrl Pts',(-27.2479314312551,-12.8291809250711,
113.955767582943)) ;
#172114=CARTESIAN_POINT('Ctrl Pts',(-27.2275682495383,-12.8679196576227,
113.893744616973)) ;
#172115=CARTESIAN_POINT('Ctrl Pts',(-27.2731763594975,-13.1373001966588,
113.997106443516)) ;
#172116=CARTESIAN_POINT('Ctrl Pts',(-27.2503338197893,-13.1572855705815,
113.927531753129)) ;
#172117=CARTESIAN_POINT('Ctrl Pts',(-27.3241376629308,-13.1572855672865,
113.903300710595)) ;
#172118=CARTESIAN_POINT('Ctrl Pts',(-27.3979415060724,-13.1572855639915,
113.879069668061)) ;
#172119=CARTESIAN_POINT('Ctrl Pts',(-27.4207840457806,-13.1373001900688,
113.948644358448)) ;
#172120=CARTESIAN_POINT('Ctrl Pts',(-27.4436265854888,-13.1173148161461,
114.018219048835)) ;
#172121=CARTESIAN_POINT('Ctrl Pts',(-27.3698227423472,-13.1173148194411,
114.042450091369)) ;
#172122=CARTESIAN_POINT('Ctrl Pts',(-27.2960188992057,-13.1173148227361,
114.066681133903)) ;
#172123=CARTESIAN_POINT('Ctrl Pts',(-27.2731763594975,-13.1373001966588,
113.997106443516)) ;
#172124=CARTESIAN_POINT('Ctrl Pts',(-27.2951340941749,-13.4255234275119,
114.028599916302)) ;
#172125=CARTESIAN_POINT('Ctrl Pts',(-27.2714569883122,-13.425412168657,
113.956483272091)) ;
#172126=CARTESIAN_POINT('Ctrl Pts',(-27.3452608317934,-13.4254121666008,
113.932252230592)) ;
#172127=CARTESIAN_POINT('Ctrl Pts',(-27.4190646752745,-13.4254121645446,
113.908021189092)) ;
#172128=CARTESIAN_POINT('Ctrl Pts',(-27.4427417811371,-13.4255234233994,
113.980137833302)) ;
#172129=CARTESIAN_POINT('Ctrl Pts',(-27.4664188869999,-13.4256346822543,
114.052254477513)) ;
#172130=CARTESIAN_POINT('Ctrl Pts',(-27.3926150435187,-13.4256346843105,
114.076485519012)) ;
#172131=CARTESIAN_POINT('Ctrl Pts',(-27.3188112000376,-13.4256346863667,
114.100716560512)) ;
#172132=CARTESIAN_POINT('Ctrl Pts',(-27.2951340941749,-13.4255234275119,
114.028599916302)) ;
#172133=CARTESIAN_POINT('Ctrl Pts',(-27.2928744217611,-13.7140381962048,
113.986224206085)) ;
#172134=CARTESIAN_POINT('Ctrl Pts',(-27.2700548445963,-13.6937806023833,
113.916719455991)) ;
#172135=CARTESIAN_POINT('Ctrl Pts',(-27.3438586880103,-13.6937806037046,
113.892488414287)) ;
#172136=CARTESIAN_POINT('Ctrl Pts',(-27.4176625314244,-13.6937806050258,
113.868257372583)) ;
#172137=CARTESIAN_POINT('Ctrl Pts',(-27.4404821085892,-13.7140381988474,
113.937762122677)) ;
#172138=CARTESIAN_POINT('Ctrl Pts',(-27.4633016857539,-13.7342957926689,
114.007266872771)) ;
#172139=CARTESIAN_POINT('Ctrl Pts',(-27.3894978423399,-13.7342957913476,
114.031497914475)) ;
#172140=CARTESIAN_POINT('Ctrl Pts',(-27.3156939989258,-13.7342957900263,
114.055728956179)) ;
#172141=CARTESIAN_POINT('Ctrl Pts',(-27.2928744217611,-13.7140381962048,
113.986224206085)) ;
#172142=CARTESIAN_POINT('Ctrl Pts',(-27.2671958080113,-13.981013641758,
113.872559420686)) ;
#172143=CARTESIAN_POINT('Ctrl Pts',(-27.2468695790329,-13.9420847851826,
113.810649006962)) ;
#172144=CARTESIAN_POINT('Ctrl Pts',(-27.3206734215819,-13.9420847906692,
113.786417962623)) ;
#172145=CARTESIAN_POINT('Ctrl Pts',(-27.3944772641309,-13.9420847961559,
113.762186918284)) ;
#172146=CARTESIAN_POINT('Ctrl Pts',(-27.4148034931093,-13.9810136527313,
113.824097332009)) ;
#172147=CARTESIAN_POINT('Ctrl Pts',(-27.4351297220877,-14.0199425093067,
113.886007745734)) ;
#172148=CARTESIAN_POINT('Ctrl Pts',(-27.3613258795387,-14.01994250382,113.910238790073)) ;
#172149=CARTESIAN_POINT('Ctrl Pts',(-27.2875220369897,-14.0199424983334,
113.934469834411)) ;
#172150=CARTESIAN_POINT('Ctrl Pts',(-27.2671958080113,-13.981013641758,
113.872559420686)) ;
#172151=CARTESIAN_POINT('Ctrl Pts',(-27.220752401802,-14.2077526521797,
113.695645507844)) ;
#172152=CARTESIAN_POINT('Ctrl Pts',(-27.2043731538913,-14.1529353062713,
113.645756961726)) ;
#172153=CARTESIAN_POINT('Ctrl Pts',(-27.2781769946741,-14.1529353151086,
113.621525912007)) ;
#172154=CARTESIAN_POINT('Ctrl Pts',(-27.3519808354569,-14.1529353239459,
113.597294862289)) ;
#172155=CARTESIAN_POINT('Ctrl Pts',(-27.3683600833676,-14.2077526698542,
113.647183408407)) ;
#172156=CARTESIAN_POINT('Ctrl Pts',(-27.3847393312783,-14.2625700157626,
113.697071954526)) ;
#172157=CARTESIAN_POINT('Ctrl Pts',(-27.3109354904955,-14.2625700069253,
113.721303004244)) ;
#172158=CARTESIAN_POINT('Ctrl Pts',(-27.2371316497127,-14.2625699980881,
113.745534053962)) ;
#172159=CARTESIAN_POINT('Ctrl Pts',(-27.220752401802,-14.2077526521797,
113.695645507844)) ;
#172160=CARTESIAN_POINT('Ctrl Pts',(-27.1574305770192,-14.3782190485839,
113.46724600276)) ;
#172161=CARTESIAN_POINT('Ctrl Pts',(-27.1461841198955,-14.3114194784183,
113.432991109356)) ;
#172162=CARTESIAN_POINT('Ctrl Pts',(-27.2199879579173,-14.3114194884178,
113.408760051228)) ;
#172163=CARTESIAN_POINT('Ctrl Pts',(-27.2937917959392,-14.3114194984174,
113.384528993101)) ;
#172164=CARTESIAN_POINT('Ctrl Pts',(-27.3050382530629,-14.378219068583,
113.418783886505)) ;
#172165=CARTESIAN_POINT('Ctrl Pts',(-27.3162847101867,-14.4450186387486,
113.453038779909)) ;
#172166=CARTESIAN_POINT('Ctrl Pts',(-27.2424808721648,-14.445018628749,
113.477269838037)) ;
#172167=CARTESIAN_POINT('Ctrl Pts',(-27.168677034143,-14.4450186187495,
113.501500896165)) ;
#172168=CARTESIAN_POINT('Ctrl Pts',(-27.1574305770192,-14.3782190485839,
113.46724600276)) ;
#172169=CARTESIAN_POINT('Ctrl Pts',(-27.082808992056,-14.4794481619843,
113.204510282952)) ;
#172170=CARTESIAN_POINT('Ctrl Pts',(-27.0774900416989,-14.4054839121495,
113.188309618911)) ;
#172171=CARTESIAN_POINT('Ctrl Pts',(-27.1512938766968,-14.4054839189219,
113.164078551572)) ;
#172172=CARTESIAN_POINT('Ctrl Pts',(-27.2250977116947,-14.4054839256943,
113.139847484234)) ;
#172173=CARTESIAN_POINT('Ctrl Pts',(-27.2304166620517,-14.4794481755291,
113.156048148275)) ;
#172174=CARTESIAN_POINT('Ctrl Pts',(-27.2357356124087,-14.5534124253639,
113.172248812316)) ;
#172175=CARTESIAN_POINT('Ctrl Pts',(-27.1619317774109,-14.5534124185915,
113.196479879654)) ;
#172176=CARTESIAN_POINT('Ctrl Pts',(-27.088127942413,-14.5534124118191,
113.220710946992)) ;
#172177=CARTESIAN_POINT('Ctrl Pts',(-27.082808992056,-14.4794481619843,
113.204510282952)) ;
#172178=CARTESIAN_POINT('Ctrl Pts',(-27.0028815148515,-14.5047934992133,
112.925619875355)) ;
#172179=CARTESIAN_POINT('Ctrl Pts',(-27.0038689041954,-14.4289527181918,
112.928627304678)) ;
#172180=CARTESIAN_POINT('Ctrl Pts',(-27.0776727363725,-14.4289527172552,
112.904396228748)) ;
#172181=CARTESIAN_POINT('Ctrl Pts',(-27.1514765685496,-14.4289527163185,
112.880165152818)) ;
#172182=CARTESIAN_POINT('Ctrl Pts',(-27.1504891792057,-14.5047934973399,
112.877157723495)) ;
#172183=CARTESIAN_POINT('Ctrl Pts',(-27.1495017898618,-14.5806342783613,
112.874150294172)) ;
#172184=CARTESIAN_POINT('Ctrl Pts',(-27.0756979576847,-14.580634279298,
112.898381370102)) ;
#172185=CARTESIAN_POINT('Ctrl Pts',(-27.0018941255076,-14.5806342802347,
112.922612446032)) ;
#172186=CARTESIAN_POINT('Ctrl Pts',(-27.0028815148515,-14.5047934992133,
112.925619875355)) ;
#172187=CARTESIAN_POINT('Ctrl Pts',(-26.9239578130133,-14.4522183736054,
112.649725923238)) ;
#172188=CARTESIAN_POINT('Ctrl Pts',(-26.9311917662438,-14.3799386549208,
112.671759378456)) ;
#172189=CARTESIAN_POINT('Ctrl Pts',(-27.0049955962026,-14.3799386416776,
112.647528295769)) ;
#172190=CARTESIAN_POINT('Ctrl Pts',(-27.0787994261614,-14.3799386284344,
112.623297213083)) ;
#172191=CARTESIAN_POINT('Ctrl Pts',(-27.0715654729308,-14.452218347119,
112.601263757865)) ;
#172192=CARTESIAN_POINT('Ctrl Pts',(-27.0643315197003,-14.5244980658035,
112.579230302647)) ;
#172193=CARTESIAN_POINT('Ctrl Pts',(-26.9905276897416,-14.5244980790467,
112.603461385334)) ;
#172194=CARTESIAN_POINT('Ctrl Pts',(-26.9167238597828,-14.5244980922899,
112.62769246802)) ;
#172195=CARTESIAN_POINT('Ctrl Pts',(-26.9239578130133,-14.4522183736054,
112.649725923238)) ;
#172196=CARTESIAN_POINT('Ctrl Pts',(-26.8526625334306,-14.3254100791536,
112.39709109002)) ;
#172197=CARTESIAN_POINT('Ctrl Pts',(-26.8656188998339,-14.2618795112896,
112.436554092626)) ;
#172198=CARTESIAN_POINT('Ctrl Pts',(-26.9394227290838,-14.2618794820993,
112.41232300778)) ;
#172199=CARTESIAN_POINT('Ctrl Pts',(-27.0132265583337,-14.261879452909,
112.388091922934)) ;
#172200=CARTESIAN_POINT('Ctrl Pts',(-27.0002701919304,-14.325410020773,
112.348628920329)) ;
#172201=CARTESIAN_POINT('Ctrl Pts',(-26.9873138255271,-14.3889405886369,
112.309165917724)) ;
#172202=CARTESIAN_POINT('Ctrl Pts',(-26.9135099962773,-14.3889406178272,
112.333397002569)) ;
#172203=CARTESIAN_POINT('Ctrl Pts',(-26.8397061670274,-14.3889406470175,
112.357628087415)) ;
#172204=CARTESIAN_POINT('Ctrl Pts',(-26.8526625334306,-14.3254100791536,
112.39709109002)) ;
#172205=CARTESIAN_POINT('Ctrl Pts',(-26.7949314683662,-14.1342773327245,
112.185876310005)) ;
#172206=CARTESIAN_POINT('Ctrl Pts',(-26.8126691907285,-14.0839997344191,
112.239902551541)) ;
#172207=CARTESIAN_POINT('Ctrl Pts',(-26.8864730213214,-14.0839996884698,
112.215671470786)) ;
#172208=CARTESIAN_POINT('Ctrl Pts',(-26.9602768519143,-14.0839996425206,
112.191440390031)) ;
#172209=CARTESIAN_POINT('Ctrl Pts',(-26.942539129552,-14.134277240826,112.137414148495)) ;
#172210=CARTESIAN_POINT('Ctrl Pts',(-26.9248014071897,-14.1845548391315,
112.083387906959)) ;
#172211=CARTESIAN_POINT('Ctrl Pts',(-26.8509975765968,-14.1845548850807,
112.107618987714)) ;
#172212=CARTESIAN_POINT('Ctrl Pts',(-26.7771937460039,-14.18455493103,112.131850068469)) ;
#172213=CARTESIAN_POINT('Ctrl Pts',(-26.7949314683662,-14.1342773327245,
112.185876310005)) ;
#172214=CARTESIAN_POINT('Ctrl Pts',(-26.7552541991608,-13.8911855385649,
112.029520728032)) ;
#172215=CARTESIAN_POINT('Ctrl Pts',(-26.7765224521165,-13.8578071985554,
112.094300396273)) ;
#172216=CARTESIAN_POINT('Ctrl Pts',(-26.8503262857672,-13.8578071355948,
112.070069324832)) ;
#172217=CARTESIAN_POINT('Ctrl Pts',(-26.9241301194179,-13.8578070726341,
112.04583825339)) ;
#172218=CARTESIAN_POINT('Ctrl Pts',(-26.9028618664622,-13.8911854126436,
111.981058585149)) ;
#172219=CARTESIAN_POINT('Ctrl Pts',(-26.8815936135065,-13.9245637526531,
111.916278916907)) ;
#172220=CARTESIAN_POINT('Ctrl Pts',(-26.8077897798558,-13.9245638156137,
111.940509988349)) ;
#172221=CARTESIAN_POINT('Ctrl Pts',(-26.7339859462051,-13.9245638785744,
111.96474105979)) ;
#172222=CARTESIAN_POINT('Ctrl Pts',(-26.7552541991608,-13.8911855385649,
112.029520728032)) ;
#172223=CARTESIAN_POINT('Ctrl Pts',(-26.7375900351982,-13.6134122049751,
111.940137889731)) ;
#172224=CARTESIAN_POINT('Ctrl Pts',(-26.7608587062214,-13.5993787020081,
112.011010508807)) ;
#172225=CARTESIAN_POINT('Ctrl Pts',(-26.8346625450312,-13.5993786244693,
111.98677945308)) ;
#172226=CARTESIAN_POINT('Ctrl Pts',(-26.9084663838411,-13.5993785469305,
111.962548397352)) ;
#172227=CARTESIAN_POINT('Ctrl Pts',(-26.8851977128179,-13.6134120498975,
111.891675778276)) ;
#172228=CARTESIAN_POINT('Ctrl Pts',(-26.8619290417947,-13.6274455528644,
111.8208031592)) ;
#172229=CARTESIAN_POINT('Ctrl Pts',(-26.7881252029848,-13.6274456304033,
111.845034214927)) ;
#172230=CARTESIAN_POINT('Ctrl Pts',(-26.7143213641749,-13.6274457079421,
111.869265270655)) ;
#172231=CARTESIAN_POINT('Ctrl Pts',(-26.7375900351982,-13.6134122049751,
111.940137889731)) ;
#172232=CARTESIAN_POINT('Ctrl Pts',(-26.7438066268346,-13.3239481087795,
111.923780754692)) ;
#172233=CARTESIAN_POINT('Ctrl Pts',(-26.7674051375456,-13.3301038926875,
111.995658012347)) ;
#172234=CARTESIAN_POINT('Ctrl Pts',(-26.8412089830833,-13.3301038083537,
111.971426977112)) ;
#172235=CARTESIAN_POINT('Ctrl Pts',(-26.915012828621,-13.3301037240199,
111.947195941876)) ;
#172236=CARTESIAN_POINT('Ctrl Pts',(-26.89141431791,-13.3239479401119,111.875318684221)) ;
#172237=CARTESIAN_POINT('Ctrl Pts',(-26.867815807199,-13.3177921562039,
111.803441426566)) ;
#172238=CARTESIAN_POINT('Ctrl Pts',(-26.7940119616613,-13.3177922405377,
111.827672461802)) ;
#172239=CARTESIAN_POINT('Ctrl Pts',(-26.7202081161236,-13.3177923248715,
111.851903497037)) ;
#172240=CARTESIAN_POINT('Ctrl Pts',(-26.7438066268346,-13.3239481087795,
111.923780754692)) ;
#172241=CARTESIAN_POINT('Ctrl Pts',(-26.7742483994232,-13.0394391601657,
111.980982516589)) ;
#172242=CARTESIAN_POINT('Ctrl Pts',(-26.7964908947302,-13.0654672913968,
112.048729570246)) ;
#172243=CARTESIAN_POINT('Ctrl Pts',(-26.8702947479032,-13.0654672055952,
112.024498558267)) ;
#172244=CARTESIAN_POINT('Ctrl Pts',(-26.9440986010763,-13.0654671197937,
112.000267546287)) ;
#172245=CARTESIAN_POINT('Ctrl Pts',(-26.9218561057693,-13.0394389885626,
111.93252049263)) ;
#172246=CARTESIAN_POINT('Ctrl Pts',(-26.8996136104623,-13.0134108573315,
111.864773438973)) ;
#172247=CARTESIAN_POINT('Ctrl Pts',(-26.8258097572892,-13.0134109431331,
111.889004450952)) ;
#172248=CARTESIAN_POINT('Ctrl Pts',(-26.7520059041162,-13.0134110289346,
111.913235462932)) ;
#172249=CARTESIAN_POINT('Ctrl Pts',(-26.7742483994232,-13.0394391601657,
111.980982516589)) ;
#172250=CARTESIAN_POINT('Ctrl Pts',(-26.8274212650553,-12.7825526473998,
112.107498381163)) ;
#172251=CARTESIAN_POINT('Ctrl Pts',(-26.8467171534129,-12.8265535642734,
112.166270545589)) ;
#172252=CARTESIAN_POINT('Ctrl Pts',(-26.9205210143309,-12.8265534855134,
112.1420395572)) ;
#172253=CARTESIAN_POINT('Ctrl Pts',(-26.994324875249,-12.8265534067534,
112.11780856881)) ;
#172254=CARTESIAN_POINT('Ctrl Pts',(-26.9750289868914,-12.7825524898798,
112.059036404385)) ;
#172255=CARTESIAN_POINT('Ctrl Pts',(-26.9557330985337,-12.7385515730062,
112.000264239959)) ;
#172256=CARTESIAN_POINT('Ctrl Pts',(-26.8819292376157,-12.7385516517662,
112.024495228348)) ;
#172257=CARTESIAN_POINT('Ctrl Pts',(-26.8081253766976,-12.7385517305262,
112.048726216737)) ;
#172258=CARTESIAN_POINT('Ctrl Pts',(-26.8274212650553,-12.7825526473998,
112.107498381163)) ;
#172259=CARTESIAN_POINT('Ctrl Pts',(-26.9007740305024,-12.5702685769134,
112.295283657163)) ;
#172260=CARTESIAN_POINT('Ctrl Pts',(-26.9157144494704,-12.6291549421708,
112.340789764681)) ;
#172261=CARTESIAN_POINT('Ctrl Pts',(-26.9895183175866,-12.629154878069,
112.316558798216)) ;
#172262=CARTESIAN_POINT('Ctrl Pts',(-27.0633221857027,-12.6291548139673,
112.292327831751)) ;
#172263=CARTESIAN_POINT('Ctrl Pts',(-27.0483817667347,-12.57026844871,112.246821724232)) ;
#172264=CARTESIAN_POINT('Ctrl Pts',(-27.0334413477666,-12.5113820834526,
112.201315616714)) ;
#172265=CARTESIAN_POINT('Ctrl Pts',(-26.9596374796504,-12.5113821475544,
112.225546583179)) ;
#172266=CARTESIAN_POINT('Ctrl Pts',(-26.8858336115343,-12.5113822116561,
112.249777549644)) ;
#172267=CARTESIAN_POINT('Ctrl Pts',(-26.9007740305024,-12.5702685769134,
112.295283657163)) ;
#172268=CARTESIAN_POINT('Ctrl Pts',(-26.9885711727641,-12.4204037087553,
112.52741789663)) ;
#172269=CARTESIAN_POINT('Ctrl Pts',(-26.9981337239508,-12.4898390976006,
112.556543886653)) ;
#172270=CARTESIAN_POINT('Ctrl Pts',(-27.0719375972436,-12.4898390557385,
112.532312935955)) ;
#172271=CARTESIAN_POINT('Ctrl Pts',(-27.1457414705363,-12.4898390138765,
112.508081985257)) ;
#172272=CARTESIAN_POINT('Ctrl Pts',(-27.1361789193497,-12.4204036250312,
112.478955995234)) ;
#172273=CARTESIAN_POINT('Ctrl Pts',(-27.1266163681631,-12.3509682361859,
112.449830005211)) ;
#172274=CARTESIAN_POINT('Ctrl Pts',(-27.0528124948703,-12.3509682780479,
112.474060955909)) ;
#172275=CARTESIAN_POINT('Ctrl Pts',(-26.9790086215775,-12.35096831991,112.498291906607)) ;
#172276=CARTESIAN_POINT('Ctrl Pts',(-26.9885711727641,-12.4204037087553,
112.52741789663)) ;
#172277=CARTESIAN_POINT('Ctrl Pts',(-27.0866504642312,-12.3408608148814,
112.790617772586)) ;
#172278=CARTESIAN_POINT('Ctrl Pts',(-27.0901148756422,-12.4159518832881,
112.801169812833)) ;
#172279=CARTESIAN_POINT('Ctrl Pts',(-27.163918752128,-12.4159518680668,
112.776938871861)) ;
#172280=CARTESIAN_POINT('Ctrl Pts',(-27.2377226286139,-12.4159518528455,
112.752707930889)) ;
#172281=CARTESIAN_POINT('Ctrl Pts',(-27.2342582172029,-12.3408607844389,
112.742155890641)) ;
#172282=CARTESIAN_POINT('Ctrl Pts',(-27.230793805792,-12.2657697160322,
112.731603850393)) ;
#172283=CARTESIAN_POINT('Ctrl Pts',(-27.1569899293061,-12.2657697312535,
112.755834791366)) ;
#172284=CARTESIAN_POINT('Ctrl Pts',(-27.0831860528202,-12.2657697464747,
112.780065732338)) ;
#172285=CARTESIAN_POINT('Ctrl Pts',(-27.0866504642312,-12.3408608148814,
112.790617772586)) ;
#172286=CARTESIAN_POINT('Ctrl Pts',(-27.1877685515325,-12.3387915853932,
113.063220104296)) ;
#172287=CARTESIAN_POINT('Ctrl Pts',(-27.184910564043,-12.414137720195,113.054515137628)) ;
#172288=CARTESIAN_POINT('Ctrl Pts',(-27.2587144409321,-12.4141377338266,
113.030284197884)) ;
#172289=CARTESIAN_POINT('Ctrl Pts',(-27.3325183178212,-12.4141377474583,
113.00605325814)) ;
#172290=CARTESIAN_POINT('Ctrl Pts',(-27.3353763053107,-12.3387916126566,
113.014758224807)) ;
#172291=CARTESIAN_POINT('Ctrl Pts',(-27.3382342928002,-12.2634454778548,
113.023463191475)) ;
#172292=CARTESIAN_POINT('Ctrl Pts',(-27.2644304159111,-12.2634454642232,
113.047694131219)) ;
#172293=CARTESIAN_POINT('Ctrl Pts',(-27.190626539022,-12.2634454505915,
113.071925070963)) ;
#172294=CARTESIAN_POINT('Ctrl Pts',(-27.1877685515325,-12.3387915853932,
113.063220104296)) ;
#172295=CARTESIAN_POINT('Ctrl Pts',(-27.2861151852823,-12.4137122483728,
113.327284210003)) ;
#172296=CARTESIAN_POINT('Ctrl Pts',(-27.2771210197373,-12.4839393117036,
113.299889435052)) ;
#172297=CARTESIAN_POINT('Ctrl Pts',(-27.3509248943576,-12.4839393535464,
113.275658488397)) ;
#172298=CARTESIAN_POINT('Ctrl Pts',(-27.4247287689778,-12.4839393953892,
113.251427541742)) ;
#172299=CARTESIAN_POINT('Ctrl Pts',(-27.4337229345229,-12.4137123320584,
113.278822316694)) ;
#172300=CARTESIAN_POINT('Ctrl Pts',(-27.442717100068,-12.3434852687276,
113.306217091645)) ;
#172301=CARTESIAN_POINT('Ctrl Pts',(-27.3689132254477,-12.3434852268848,
113.330448038299)) ;
#172302=CARTESIAN_POINT('Ctrl Pts',(-27.2951093508274,-12.343485185042,
113.354678984954)) ;
#172303=CARTESIAN_POINT('Ctrl Pts',(-27.2861151852823,-12.4137122483728,
113.327284210003)) ;
#172304=CARTESIAN_POINT('Ctrl Pts',(-27.3754145778794,-12.5618189977429,
113.56362900409)) ;
#172305=CARTESIAN_POINT('Ctrl Pts',(-27.3609100234517,-12.6218107314417,
113.519450473671)) ;
#172306=CARTESIAN_POINT('Ctrl Pts',(-27.4347138930807,-12.6218107975561,
113.495219511814)) ;
#172307=CARTESIAN_POINT('Ctrl Pts',(-27.5085177627096,-12.6218108636706,
113.470988549956)) ;
#172308=CARTESIAN_POINT('Ctrl Pts',(-27.5230223171373,-12.5618191299718,
113.515167080375)) ;
#172309=CARTESIAN_POINT('Ctrl Pts',(-27.5375268715649,-12.501827396273,
113.559345610793)) ;
#172310=CARTESIAN_POINT('Ctrl Pts',(-27.4637230019359,-12.5018273301586,
113.583576572651)) ;
#172311=CARTESIAN_POINT('Ctrl Pts',(-27.389919132307,-12.5018272640442,
113.607807534508)) ;
#172312=CARTESIAN_POINT('Ctrl Pts',(-27.3754145778794,-12.5618189977429,
113.56362900409)) ;
#172313=CARTESIAN_POINT('Ctrl Pts',(-27.4488280555374,-12.7689119270669,
113.752013523521)) ;
#172314=CARTESIAN_POINT('Ctrl Pts',(-27.429905270597,-12.814533735282,113.694377775808)) ;
#172315=CARTESIAN_POINT('Ctrl Pts',(-27.5037091335364,-12.8145338199658,
113.670146793575)) ;
#172316=CARTESIAN_POINT('Ctrl Pts',(-27.5775129964758,-12.8145339046497,
113.645915811343)) ;
#172317=CARTESIAN_POINT('Ctrl Pts',(-27.5964357814161,-12.7689120964346,
113.703551559055)) ;
#172318=CARTESIAN_POINT('Ctrl Pts',(-27.6153585663564,-12.7232902882195,
113.761187306768)) ;
#172319=CARTESIAN_POINT('Ctrl Pts',(-27.541554703417,-12.7232902035356,
113.785418289001)) ;
#172320=CARTESIAN_POINT('Ctrl Pts',(-27.4677508404777,-12.7232901188518,
113.809649271233)) ;
#172321=CARTESIAN_POINT('Ctrl Pts',(-27.4488280555374,-12.7689119270669,
113.752013523521)) ;
#172322=CARTESIAN_POINT('Ctrl Pts',(-27.5035776459415,-13.0251682484426,
113.883107535979)) ;
#172323=CARTESIAN_POINT('Ctrl Pts',(-27.4815419694659,-13.052967781727,
113.815990422836)) ;
#172324=CARTESIAN_POINT('Ctrl Pts',(-27.5553458241622,-13.0529678764172,
113.791759415496)) ;
#172325=CARTESIAN_POINT('Ctrl Pts',(-27.6291496788585,-13.0529679711075,
113.767528408156)) ;
#172326=CARTESIAN_POINT('Ctrl Pts',(-27.6511853553341,-13.025168437823,
113.834645521299)) ;
#172327=CARTESIAN_POINT('Ctrl Pts',(-27.6732210318097,-12.9973689045386,
113.901762634441)) ;
#172328=CARTESIAN_POINT('Ctrl Pts',(-27.5994171771134,-12.9973688098484,
113.925993641781)) ;
#172329=CARTESIAN_POINT('Ctrl Pts',(-27.5256133224171,-12.9973687151582,
113.950224649121)) ;
#172330=CARTESIAN_POINT('Ctrl Pts',(-27.5035776459415,-13.0251682484426,
113.883107535979)) ;
#172331=CARTESIAN_POINT('Ctrl Pts',(-27.5351792728666,-13.3082750938872,
113.943914512976)) ;
#172332=CARTESIAN_POINT('Ctrl Pts',(-27.5116376544627,-13.3163504016851,
113.872210543615)) ;
#172333=CARTESIAN_POINT('Ctrl Pts',(-27.5854415007842,-13.3163504980826,
113.847979510767)) ;
#172334=CARTESIAN_POINT('Ctrl Pts',(-27.6592453471057,-13.31635059448,113.823748477919)) ;
#172335=CARTESIAN_POINT('Ctrl Pts',(-27.6827869655096,-13.3082752866821,
113.895452447279)) ;
#172336=CARTESIAN_POINT('Ctrl Pts',(-27.7063285839134,-13.3001999788842,
113.967156416639)) ;
#172337=CARTESIAN_POINT('Ctrl Pts',(-27.6325247375919,-13.3001998824867,
113.991387449487)) ;
#172338=CARTESIAN_POINT('Ctrl Pts',(-27.5587208912704,-13.3001997860893,
114.015618482336)) ;
#172339=CARTESIAN_POINT('Ctrl Pts',(-27.5351792728666,-13.3082750938872,
113.943914512976)) ;
#172340=CARTESIAN_POINT('Ctrl Pts',(-27.5426920454856,-13.5983478962611,
113.931443511884)) ;
#172341=CARTESIAN_POINT('Ctrl Pts',(-27.5193221646225,-13.5861829357955,
113.860262627273)) ;
#172342=CARTESIAN_POINT('Ctrl Pts',(-27.5931260031213,-13.5861830266329,
113.836031570598)) ;
#172343=CARTESIAN_POINT('Ctrl Pts',(-27.6669298416201,-13.5861831174704,
113.811800513923)) ;
#172344=CARTESIAN_POINT('Ctrl Pts',(-27.6902997224832,-13.5983480779361,
113.882981398534)) ;
#172345=CARTESIAN_POINT('Ctrl Pts',(-27.7136696033462,-13.6105130384017,
113.954162283145)) ;
#172346=CARTESIAN_POINT('Ctrl Pts',(-27.6398657648474,-13.6105129475642,
113.97839333982)) ;
#172347=CARTESIAN_POINT('Ctrl Pts',(-27.5660619263486,-13.6105128567267,
114.002624396495)) ;
#172348=CARTESIAN_POINT('Ctrl Pts',(-27.5426920454856,-13.5983478962611,
113.931443511884)) ;
#172349=CARTESIAN_POINT('Ctrl Pts',(-27.5263734044367,-13.8761876349326,
113.846318938576)) ;
#172350=CARTESIAN_POINT('Ctrl Pts',(-27.5048406247926,-13.8446061027284,
113.780733567751)) ;
#172351=CARTESIAN_POINT('Ctrl Pts',(-27.5786444566591,-13.8446061808087,
113.756502490876)) ;
#172352=CARTESIAN_POINT('Ctrl Pts',(-27.6524482885256,-13.8446062588889,
113.732271414)) ;
#172353=CARTESIAN_POINT('Ctrl Pts',(-27.6739810681696,-13.8761877910931,
113.797856784825)) ;
#172354=CARTESIAN_POINT('Ctrl Pts',(-27.6955138478137,-13.9077693232973,
113.863442155649)) ;
#172355=CARTESIAN_POINT('Ctrl Pts',(-27.6217100159472,-13.907769245217,
113.887673232525)) ;
#172356=CARTESIAN_POINT('Ctrl Pts',(-27.5479061840807,-13.9077691671368,
113.911904309401)) ;
#172357=CARTESIAN_POINT('Ctrl Pts',(-27.5263734044367,-13.8761876349326,
113.846318938576)) ;
#172358=CARTESIAN_POINT('Ctrl Pts',(-27.4877132850847,-14.1226645874526,
113.692922737031)) ;
#172359=CARTESIAN_POINT('Ctrl Pts',(-27.4695845649599,-14.0738264529784,
113.637705582096)) ;
#172360=CARTESIAN_POINT('Ctrl Pts',(-27.5433883924307,-14.0738265118824,
113.613474491831)) ;
#172361=CARTESIAN_POINT('Ctrl Pts',(-27.6171922199014,-14.0738265707863,
113.589243401567)) ;
#172362=CARTESIAN_POINT('Ctrl Pts',(-27.6353209400262,-14.1226647052604,
113.644460556502)) ;
#172363=CARTESIAN_POINT('Ctrl Pts',(-27.653449660151,-14.1715028397345,
113.699677711437)) ;
#172364=CARTESIAN_POINT('Ctrl Pts',(-27.5796458326802,-14.1715027808306,
113.723908801702)) ;
#172365=CARTESIAN_POINT('Ctrl Pts',(-27.5058420052094,-14.1715027219267,
113.748139891966)) ;
#172366=CARTESIAN_POINT('Ctrl Pts',(-27.4877132850847,-14.1226645874526,
113.692922737031)) ;
#172367=CARTESIAN_POINT('Ctrl Pts',(-27.4306473190199,-14.3171342011777,
113.483654238532)) ;
#172368=CARTESIAN_POINT('Ctrl Pts',(-27.417209160534,-14.2546443269057,
113.442723777381)) ;
#172369=CARTESIAN_POINT('Ctrl Pts',(-27.491012985715,-14.2546443659289,
113.418492680142)) ;
#172370=CARTESIAN_POINT('Ctrl Pts',(-27.5648168108959,-14.2546444049521,
113.394261582903)) ;
#172371=CARTESIAN_POINT('Ctrl Pts',(-27.5782549693818,-14.3171342792242,
113.435192044054)) ;
#172372=CARTESIAN_POINT('Ctrl Pts',(-27.5916931278677,-14.3796241534962,
113.476122505205)) ;
#172373=CARTESIAN_POINT('Ctrl Pts',(-27.5178893026867,-14.379624114473,
113.500353602444)) ;
#172374=CARTESIAN_POINT('Ctrl Pts',(-27.4440854775058,-14.3796240754498,
113.524584699683)) ;
#172375=CARTESIAN_POINT('Ctrl Pts',(-27.4306473190199,-14.3171342011777,
113.483654238532)) ;
#172376=CARTESIAN_POINT('Ctrl Pts',(-27.3601955150723,-14.4470643657725,
113.233728201309)) ;
#172377=CARTESIAN_POINT('Ctrl Pts',(-27.3523873320976,-14.375408398759,
113.209945737037)) ;
#172378=CARTESIAN_POINT('Ctrl Pts',(-27.4261911567725,-14.3754084186234,
113.185714638256)) ;
#172379=CARTESIAN_POINT('Ctrl Pts',(-27.4999949814474,-14.3754084384878,
113.161483539476)) ;
#172380=CARTESIAN_POINT('Ctrl Pts',(-27.5078031644221,-14.4470644055013,
113.185266003749)) ;
#172381=CARTESIAN_POINT('Ctrl Pts',(-27.5156113473968,-14.5187203725148,
113.209048468021)) ;
#172382=CARTESIAN_POINT('Ctrl Pts',(-27.4418075227219,-14.5187203526504,
113.233279566802)) ;
#172383=CARTESIAN_POINT('Ctrl Pts',(-27.368003698047,-14.5187203327861,
113.257510665582)) ;
#172384=CARTESIAN_POINT('Ctrl Pts',(-27.3601955150723,-14.4470643657725,
113.233728201309)) ;
#172385=CARTESIAN_POINT('Ctrl Pts',(-27.2816288073246,-14.503923953364,
112.958964415876)) ;
#172386=CARTESIAN_POINT('Ctrl Pts',(-27.280028179883,-14.4281893560193,
112.954089164008)) ;
#172387=CARTESIAN_POINT('Ctrl Pts',(-27.3538320062244,-14.4281893585944,
112.929858070304)) ;
#172388=CARTESIAN_POINT('Ctrl Pts',(-27.4276358325657,-14.4281893611695,
112.905626976599)) ;
#172389=CARTESIAN_POINT('Ctrl Pts',(-27.4292364600073,-14.5039239585142,
112.910502228467)) ;
#172390=CARTESIAN_POINT('Ctrl Pts',(-27.4308370874489,-14.5796585558589,
112.915377480335)) ;
#172391=CARTESIAN_POINT('Ctrl Pts',(-27.3570332611075,-14.5796585532838,
112.93960857404)) ;
#172392=CARTESIAN_POINT('Ctrl Pts',(-27.2832294347662,-14.5796585507087,
112.963839667744)) ;
#172393=CARTESIAN_POINT('Ctrl Pts',(-27.2816288073246,-14.503923953364,
112.958964415876)) ;
#172394=CARTESIAN_POINT('Ctrl Pts',(-27.2014946791726,-14.4828378904359,
112.679399169153)) ;
#172395=CARTESIAN_POINT('Ctrl Pts',(-27.2062211107245,-14.4084605775559,
112.693795117939)) ;
#172396=CARTESIAN_POINT('Ctrl Pts',(-27.2800249401893,-14.4084605673929,
112.669564033748)) ;
#172397=CARTESIAN_POINT('Ctrl Pts',(-27.3538287696541,-14.40846055723,112.645332949557)) ;
#172398=CARTESIAN_POINT('Ctrl Pts',(-27.3491023381022,-14.48283787011,112.630937000771)) ;
#172399=CARTESIAN_POINT('Ctrl Pts',(-27.3443759065502,-14.5572151829901,
112.616541051985)) ;
#172400=CARTESIAN_POINT('Ctrl Pts',(-27.2705720770854,-14.557215193153,
112.640772136176)) ;
#172401=CARTESIAN_POINT('Ctrl Pts',(-27.1967682476206,-14.557215203316,
112.665003220367)) ;
#172402=CARTESIAN_POINT('Ctrl Pts',(-27.2014946791726,-14.4828378904359,
112.679399169153)) ;
#172403=CARTESIAN_POINT('Ctrl Pts',(-27.1263680307239,-14.385601171439,
112.415108437441)) ;
#172404=CARTESIAN_POINT('Ctrl Pts',(-27.1370810693772,-14.3179002562645,
112.447738625353)) ;
#172405=CARTESIAN_POINT('Ctrl Pts',(-27.2108849026355,-14.3179002385077,
112.423507552716)) ;
#172406=CARTESIAN_POINT('Ctrl Pts',(-27.2846887358938,-14.3179002207509,
112.39927648008)) ;
#172407=CARTESIAN_POINT('Ctrl Pts',(-27.2739756972405,-14.3856011359254,
112.366646292167)) ;
#172408=CARTESIAN_POINT('Ctrl Pts',(-27.2632626585871,-14.4533020510999,
112.334016104255)) ;
#172409=CARTESIAN_POINT('Ctrl Pts',(-27.1894588253288,-14.4533020688567,
112.358247176892)) ;
#172410=CARTESIAN_POINT('Ctrl Pts',(-27.1156549920705,-14.4533020866135,
112.382478249528)) ;
#172411=CARTESIAN_POINT('Ctrl Pts',(-27.1263680307239,-14.385601171439,
112.415108437441)) ;
#172412=CARTESIAN_POINT('Ctrl Pts',(-27.0621909151168,-14.2179717447503,
112.184017247317)) ;
#172413=CARTESIAN_POINT('Ctrl Pts',(-27.0781384399911,-14.1618723407489,
112.232590835486)) ;
#172414=CARTESIAN_POINT('Ctrl Pts',(-27.1519422772901,-14.161872321804,
112.208359775157)) ;
#172415=CARTESIAN_POINT('Ctrl Pts',(-27.2257461145892,-14.1618723028591,
112.184128714828)) ;
#172416=CARTESIAN_POINT('Ctrl Pts',(-27.2097985897148,-14.2179717068605,
112.135555126658)) ;
#172417=CARTESIAN_POINT('Ctrl Pts',(-27.1938510648405,-14.2740711108619,
112.086981538488)) ;
#172418=CARTESIAN_POINT('Ctrl Pts',(-27.1200472275414,-14.2740711298068,
112.111212598818)) ;
#172419=CARTESIAN_POINT('Ctrl Pts',(-27.0462433902424,-14.2740711487517,
112.135443659147)) ;
#172420=CARTESIAN_POINT('Ctrl Pts',(-27.0621909151168,-14.2179717447503,
112.184017247317)) ;
#172421=CARTESIAN_POINT('Ctrl Pts',(-27.0150398235501,-13.9957363810985,
112.005222445318)) ;
#172422=CARTESIAN_POINT('Ctrl Pts',(-27.0350315354715,-13.9550697800569,
112.066113974601)) ;
#172423=CARTESIAN_POINT('Ctrl Pts',(-27.1088353754445,-13.95506976129,112.041882922416)) ;
#172424=CARTESIAN_POINT('Ctrl Pts',(-27.1826392154175,-13.9550697425231,
112.017651870231)) ;
#172425=CARTESIAN_POINT('Ctrl Pts',(-27.162647503496,-13.9957363435648,
111.956760340948)) ;
#172426=CARTESIAN_POINT('Ctrl Pts',(-27.1426557915745,-14.0364029446064,
111.895868811665)) ;
#172427=CARTESIAN_POINT('Ctrl Pts',(-27.0688519516015,-14.0364029633733,
111.92009986385)) ;
#172428=CARTESIAN_POINT('Ctrl Pts',(-26.9950481116286,-14.0364029821402,
111.944330916035)) ;
#172429=CARTESIAN_POINT('Ctrl Pts',(-27.0150398235501,-13.9957363810985,
112.005222445318)) ;
#172430=CARTESIAN_POINT('Ctrl Pts',(-26.9879423735838,-13.7291995183929,
111.88704329511)) ;
#172431=CARTESIAN_POINT('Ctrl Pts',(-27.0105941912921,-13.707082237132,
111.956037077241)) ;
#172432=CARTESIAN_POINT('Ctrl Pts',(-27.0843980337561,-13.7070822245354,
111.931806032644)) ;
#172433=CARTESIAN_POINT('Ctrl Pts',(-27.1582018762201,-13.7070822119389,
111.907574988046)) ;
#172434=CARTESIAN_POINT('Ctrl Pts',(-27.1355500585118,-13.7291994931998,
111.838581205914)) ;
#172435=CARTESIAN_POINT('Ctrl Pts',(-27.1128982408035,-13.7513167744608,
111.769587423783)) ;
#172436=CARTESIAN_POINT('Ctrl Pts',(-27.0390943983395,-13.7513167870574,
111.79381846838)) ;
#172437=CARTESIAN_POINT('Ctrl Pts',(-26.9652905558756,-13.7513167996539,
111.818049512978)) ;
#172438=CARTESIAN_POINT('Ctrl Pts',(-26.9879423735838,-13.7291995183929,
111.88704329511)) ;
#172439=CARTESIAN_POINT('Ctrl Pts',(-26.9843581372536,-13.4423294051305,
111.840765762246)) ;
#172440=CARTESIAN_POINT('Ctrl Pts',(-27.0080260400951,-13.440209694869,
111.912854375641)) ;
#172441=CARTESIAN_POINT('Ctrl Pts',(-27.081829883601,-13.4402096875426,
111.888623334217)) ;
#172442=CARTESIAN_POINT('Ctrl Pts',(-27.1556337271069,-13.4402096802161,
111.864392292792)) ;
#172443=CARTESIAN_POINT('Ctrl Pts',(-27.1319658242654,-13.4423293904776,
111.792303679397)) ;
#172444=CARTESIAN_POINT('Ctrl Pts',(-27.1082979214239,-13.444449100739,
111.720215066002)) ;
#172445=CARTESIAN_POINT('Ctrl Pts',(-27.034494077918,-13.4444491080655,
111.744446107426)) ;
#172446=CARTESIAN_POINT('Ctrl Pts',(-26.9606902344121,-13.444449115392,
111.76867714885)) ;
#172447=CARTESIAN_POINT('Ctrl Pts',(-26.9843581372536,-13.4423294051305,
111.840765762246)) ;
#172448=CARTESIAN_POINT('Ctrl Pts',(-27.0050610704701,-13.1524216120436,
111.868286429054)) ;
#172449=CARTESIAN_POINT('Ctrl Pts',(-27.0280544057654,-13.1705421865172,
111.938320418437)) ;
#172450=CARTESIAN_POINT('Ctrl Pts',(-27.1018582494374,-13.1705421848694,
111.914089377519)) ;
#172451=CARTESIAN_POINT('Ctrl Pts',(-27.1756620931093,-13.1705421832215,
111.889858336601)) ;
#172452=CARTESIAN_POINT('Ctrl Pts',(-27.152668757814,-13.1524216087479,
111.819824347217)) ;
#172453=CARTESIAN_POINT('Ctrl Pts',(-27.1296754225186,-13.1343010342744,
111.749790357834)) ;
#172454=CARTESIAN_POINT('Ctrl Pts',(-27.0558715788467,-13.1343010359222,
111.774021398752)) ;
#172455=CARTESIAN_POINT('Ctrl Pts',(-26.9820677351747,-13.1343010375701,
111.798252439671)) ;
#172456=CARTESIAN_POINT('Ctrl Pts',(-27.0050610704701,-13.1524216120436,
111.868286429054)) ;
#172457=CARTESIAN_POINT('Ctrl Pts',(-27.0492012117308,-12.8827428706973,
111.967358039858)) ;
#172458=CARTESIAN_POINT('Ctrl Pts',(-27.0698787059065,-12.9197213640829,
112.030338350789)) ;
#172459=CARTESIAN_POINT('Ctrl Pts',(-27.143682549157,-12.9197213654279,
112.006107308587)) ;
#172460=CARTESIAN_POINT('Ctrl Pts',(-27.2174863924074,-12.919721366773,
111.981876266384)) ;
#172461=CARTESIAN_POINT('Ctrl Pts',(-27.1968088982317,-12.8827428733873,
111.918895955454)) ;
#172462=CARTESIAN_POINT('Ctrl Pts',(-27.176131404056,-12.8457643800017,
111.855915644523)) ;
#172463=CARTESIAN_POINT('Ctrl Pts',(-27.1023275608056,-12.8457643786566,
111.880146686725)) ;
#172464=CARTESIAN_POINT('Ctrl Pts',(-27.0285237175551,-12.8457643773116,
111.904377728927)) ;
#172465=CARTESIAN_POINT('Ctrl Pts',(-27.0492012117308,-12.8827428706973,
111.967358039858)) ;
#172466=CARTESIAN_POINT('Ctrl Pts',(-27.1146617710616,-12.6504179680888,
112.131229509415)) ;
#172467=CARTESIAN_POINT('Ctrl Pts',(-27.1315339429113,-12.7036746706006,
112.18261942249)) ;
#172468=CARTESIAN_POINT('Ctrl Pts',(-27.2053377856061,-12.7036746730312,
112.158388378596)) ;
#172469=CARTESIAN_POINT('Ctrl Pts',(-27.2791416283009,-12.7036746754618,
112.134157334701)) ;
#172470=CARTESIAN_POINT('Ctrl Pts',(-27.2622694564512,-12.65041797295,112.082767421626)) ;
#172471=CARTESIAN_POINT('Ctrl Pts',(-27.2453972846015,-12.5971612704382,
112.031377508551)) ;
#172472=CARTESIAN_POINT('Ctrl Pts',(-27.1715934419067,-12.5971612680076,
112.055608552446)) ;
#172473=CARTESIAN_POINT('Ctrl Pts',(-27.0977895992119,-12.597161265577,
112.07983959634)) ;
#172474=CARTESIAN_POINT('Ctrl Pts',(-27.1146617710616,-12.6504179680888,
112.131229509415)) ;
#172475=CARTESIAN_POINT('Ctrl Pts',(-27.1972630412984,-12.4733695384466,
112.347366409406)) ;
#172476=CARTESIAN_POINT('Ctrl Pts',(-27.2091258740215,-12.5390682481556,
112.383498683763)) ;
#172477=CARTESIAN_POINT('Ctrl Pts',(-27.2829297166078,-12.5390682494468,
112.359267639538)) ;
#172478=CARTESIAN_POINT('Ctrl Pts',(-27.3567335591942,-12.5390682507379,
112.335036595313)) ;
#172479=CARTESIAN_POINT('Ctrl Pts',(-27.3448707264711,-12.4733695410289,
112.298904320956)) ;
#172480=CARTESIAN_POINT('Ctrl Pts',(-27.3330078937479,-12.4076708313198,
112.262772046599)) ;
#172481=CARTESIAN_POINT('Ctrl Pts',(-27.2592040511616,-12.4076708300287,
112.287003090824)) ;
#172482=CARTESIAN_POINT('Ctrl Pts',(-27.1854002085753,-12.4076708287375,
112.311234135049)) ;
#172483=CARTESIAN_POINT('Ctrl Pts',(-27.1972630412984,-12.4733695384466,
112.347366409406)) ;
#172484=CARTESIAN_POINT('Ctrl Pts',(-27.2924020500798,-12.3637277646619,
112.601520160583)) ;
#172485=CARTESIAN_POINT('Ctrl Pts',(-27.2983761879379,-12.4371796156444,
112.619716420582)) ;
#172486=CARTESIAN_POINT('Ctrl Pts',(-27.3721800314205,-12.4371796152465,
112.595485379087)) ;
#172487=CARTESIAN_POINT('Ctrl Pts',(-27.4459838749031,-12.4371796148486,
112.571254337592)) ;
#172488=CARTESIAN_POINT('Ctrl Pts',(-27.4400097370451,-12.3637277638662,
112.553058077593)) ;
#172489=CARTESIAN_POINT('Ctrl Pts',(-27.434035599187,-12.2902759128838,
112.534861817595)) ;
#172490=CARTESIAN_POINT('Ctrl Pts',(-27.3602317557044,-12.2902759132816,
112.55909285909)) ;
#172491=CARTESIAN_POINT('Ctrl Pts',(-27.2864279122218,-12.2902759136795,
112.583323900585)) ;
#172492=CARTESIAN_POINT('Ctrl Pts',(-27.2924020500798,-12.3637277646619,
112.601520160583)) ;
#172493=CARTESIAN_POINT('Ctrl Pts',(-27.3927913486772,-12.3302633026411,
112.871950604607)) ;
#172494=CARTESIAN_POINT('Ctrl Pts',(-27.3924958222733,-12.4061588446246,
112.871050478946)) ;
#172495=CARTESIAN_POINT('Ctrl Pts',(-27.4662996670084,-12.406158844275,
112.846819441266)) ;
#172496=CARTESIAN_POINT('Ctrl Pts',(-27.5401035117436,-12.4061588439253,
112.822588403586)) ;
#172497=CARTESIAN_POINT('Ctrl Pts',(-27.5403990381475,-12.3302633019418,
112.823488529247)) ;
#172498=CARTESIAN_POINT('Ctrl Pts',(-27.5406945645514,-12.2543677599582,
112.824388654909)) ;
#172499=CARTESIAN_POINT('Ctrl Pts',(-27.4668907198163,-12.2543677603079,
112.848619692589)) ;
#172500=CARTESIAN_POINT('Ctrl Pts',(-27.3930868750811,-12.2543677606575,
112.872850730269)) ;
#172501=CARTESIAN_POINT('Ctrl Pts',(-27.3927913486772,-12.3302633026411,
112.871950604607)) ;
#172502=CARTESIAN_POINT('Ctrl Pts',(-27.4930345233602,-12.3743151570883,
113.14182288393)) ;
#172503=CARTESIAN_POINT('Ctrl Pts',(-27.486472782332,-12.4472453738058,
113.121836879682)) ;
#172504=CARTESIAN_POINT('Ctrl Pts',(-27.5602766287209,-12.4472453760978,
113.097605847039)) ;
#172505=CARTESIAN_POINT('Ctrl Pts',(-27.6340804751099,-12.4472453783898,
113.073374814396)) ;
#172506=CARTESIAN_POINT('Ctrl Pts',(-27.640642216138,-12.3743151616723,
113.093360818644)) ;
#172507=CARTESIAN_POINT('Ctrl Pts',(-27.6472039571662,-12.3013849449547,
113.113346822893)) ;
#172508=CARTESIAN_POINT('Ctrl Pts',(-27.5734001107772,-12.3013849426627,
113.137577855536)) ;
#172509=CARTESIAN_POINT('Ctrl Pts',(-27.4995962643883,-12.3013849403707,
113.161808888179)) ;
#172510=CARTESIAN_POINT('Ctrl Pts',(-27.4930345233602,-12.3743151570883,
113.14182288393)) ;
#172511=CARTESIAN_POINT('Ctrl Pts',(-27.5863812625094,-12.4928395526405,
113.390726218169)) ;
#172512=CARTESIAN_POINT('Ctrl Pts',(-27.5740251224026,-12.5575998714036,
113.353091409372)) ;
#172513=CARTESIAN_POINT('Ctrl Pts',(-27.6478289702466,-12.5575998792926,
113.328860381161)) ;
#172514=CARTESIAN_POINT('Ctrl Pts',(-27.7216328180906,-12.5575998871817,
113.30462935295)) ;
#172515=CARTESIAN_POINT('Ctrl Pts',(-27.7339889581974,-12.4928395684187,
113.342264161746)) ;
#172516=CARTESIAN_POINT('Ctrl Pts',(-27.7463450983042,-12.4280792496557,
113.379898970542)) ;
#172517=CARTESIAN_POINT('Ctrl Pts',(-27.6725412504602,-12.4280792417666,
113.404129998754)) ;
#172518=CARTESIAN_POINT('Ctrl Pts',(-27.5987374026162,-12.4280792338775,
113.428361026965)) ;
#172519=CARTESIAN_POINT('Ctrl Pts',(-27.5863812625094,-12.4928395526405,
113.390726218169)) ;
#172520=CARTESIAN_POINT('Ctrl Pts',(-27.6674288059213,-12.6792484033362,
113.601904231307)) ;
#172521=CARTESIAN_POINT('Ctrl Pts',(-27.6501339912232,-12.7310874670911,
113.549227016744)) ;
#172522=CARTESIAN_POINT('Ctrl Pts',(-27.7239378402491,-12.7310874856029,
113.524995992133)) ;
#172523=CARTESIAN_POINT('Ctrl Pts',(-27.7977416892751,-12.7310875041147,
113.500764967522)) ;
#172524=CARTESIAN_POINT('Ctrl Pts',(-27.8150365039733,-12.6792484403597,
113.553442182085)) ;
#172525=CARTESIAN_POINT('Ctrl Pts',(-27.8323313186715,-12.6274093766048,
113.606119396648)) ;
#172526=CARTESIAN_POINT('Ctrl Pts',(-27.7585274696455,-12.627409358093,
113.630350421259)) ;
#172527=CARTESIAN_POINT('Ctrl Pts',(-27.6847236206195,-12.6274093395813,
113.65458144587)) ;
#172528=CARTESIAN_POINT('Ctrl Pts',(-27.6674288059213,-12.6792484033362,
113.601904231307)) ;
#172529=CARTESIAN_POINT('Ctrl Pts',(-27.7297752283218,-12.9157037711306,
113.756592636286)) ;
#172530=CARTESIAN_POINT('Ctrl Pts',(-27.7088310990503,-12.9511079256509,
113.69280019846)) ;
#172531=CARTESIAN_POINT('Ctrl Pts',(-27.7826349472372,-12.9511079534963,
113.668569171294)) ;
#172532=CARTESIAN_POINT('Ctrl Pts',(-27.8564387954241,-12.9511079813417,
113.644338144128)) ;
#172533=CARTESIAN_POINT('Ctrl Pts',(-27.8773829246957,-12.9157038268213,
113.708130581953)) ;
#172534=CARTESIAN_POINT('Ctrl Pts',(-27.8983270539673,-12.880299672301,
113.771923019778)) ;
#172535=CARTESIAN_POINT('Ctrl Pts',(-27.8245232057804,-12.8802996444556,
113.796154046944)) ;
#172536=CARTESIAN_POINT('Ctrl Pts',(-27.7507193575934,-12.8802996166102,
113.820385074111)) ;
#172537=CARTESIAN_POINT('Ctrl Pts',(-27.7297752283218,-12.9157037711306,
113.756592636286)) ;
#172538=CARTESIAN_POINT('Ctrl Pts',(-27.7712714115266,-13.1914441677562,
113.847288780652)) ;
#172539=CARTESIAN_POINT('Ctrl Pts',(-27.748138134954,-13.2076474543041,
113.776828553575)) ;
#172540=CARTESIAN_POINT('Ctrl Pts',(-27.8219419813756,-13.2076474957357,
113.752597521032)) ;
#172541=CARTESIAN_POINT('Ctrl Pts',(-27.8957458277972,-13.2076475371673,
113.728366488488)) ;
#172542=CARTESIAN_POINT('Ctrl Pts',(-27.9188791043698,-13.1914442506193,
113.798826715565)) ;
#172543=CARTESIAN_POINT('Ctrl Pts',(-27.9420123809424,-13.1752409640713,
113.869286942643)) ;
#172544=CARTESIAN_POINT('Ctrl Pts',(-27.8682085345208,-13.1752409226398,
113.893517975186)) ;
#172545=CARTESIAN_POINT('Ctrl Pts',(-27.7944046880992,-13.1752408812082,
113.917749007729)) ;
#172546=CARTESIAN_POINT('Ctrl Pts',(-27.7712714115266,-13.1914441677562,
113.847288780652)) ;
#172547=CARTESIAN_POINT('Ctrl Pts',(-27.7885541463279,-13.4802992555045,
113.864652632934)) ;
#172548=CARTESIAN_POINT('Ctrl Pts',(-27.7649109140841,-13.4763581958197,
113.792639163296)) ;
#172549=CARTESIAN_POINT('Ctrl Pts',(-27.8387147567996,-13.4763582452253,
113.768408119464)) ;
#172550=CARTESIAN_POINT('Ctrl Pts',(-27.9125185995151,-13.4763582946309,
113.744177075633)) ;
#172551=CARTESIAN_POINT('Ctrl Pts',(-27.9361618317589,-13.4802993543157,
113.816190545271)) ;
#172552=CARTESIAN_POINT('Ctrl Pts',(-27.9598050640028,-13.4842404140005,
113.888204014908)) ;
#172553=CARTESIAN_POINT('Ctrl Pts',(-27.8860012212873,-13.4842403645949,
113.91243505874)) ;
#172554=CARTESIAN_POINT('Ctrl Pts',(-27.8121973785718,-13.4842403151893,
113.936666102571)) ;
#172555=CARTESIAN_POINT('Ctrl Pts',(-27.7885541463279,-13.4802992555045,
113.864652632934)) ;
#172556=CARTESIAN_POINT('Ctrl Pts',(-27.7818265483523,-13.7664087624137,
113.808666272862)) ;
#172557=CARTESIAN_POINT('Ctrl Pts',(-27.7593533008919,-13.7424862734231,
113.740216388272)) ;
#172558=CARTESIAN_POINT('Ctrl Pts',(-27.8331571387186,-13.7424863290053,
113.715985329549)) ;
#172559=CARTESIAN_POINT('Ctrl Pts',(-27.9069609765453,-13.7424863845875,
113.691754270827)) ;
#172560=CARTESIAN_POINT('Ctrl Pts',(-27.9294342240057,-13.766408873578,
113.760204155418)) ;
#172561=CARTESIAN_POINT('Ctrl Pts',(-27.9519074714661,-13.7903313625685,
113.828654040009)) ;
#172562=CARTESIAN_POINT('Ctrl Pts',(-27.8781036336394,-13.7903313069864,
113.852885098731)) ;
#172563=CARTESIAN_POINT('Ctrl Pts',(-27.8042997958127,-13.7903312514042,
113.877116157453)) ;
#172564=CARTESIAN_POINT('Ctrl Pts',(-27.7818265483523,-13.7664087624137,
113.808666272862)) ;
#172565=CARTESIAN_POINT('Ctrl Pts',(-27.7518733154646,-14.0278445854345,
113.681886834829)) ;
#172566=CARTESIAN_POINT('Ctrl Pts',(-27.732194294108,-13.98563446645,113.621947712281)) ;
#172567=CARTESIAN_POINT('Ctrl Pts',(-27.805998125884,-13.9856345227655,
113.597716635129)) ;
#172568=CARTESIAN_POINT('Ctrl Pts',(-27.8798019576601,-13.985634579081,
113.573485557978)) ;
#172569=CARTESIAN_POINT('Ctrl Pts',(-27.8994809790166,-14.0278446980655,
113.633424680526)) ;
#172570=CARTESIAN_POINT('Ctrl Pts',(-27.9191600003732,-14.07005481705,113.693363803075)) ;
#172571=CARTESIAN_POINT('Ctrl Pts',(-27.8453561685971,-14.0700547607345,
113.717594880226)) ;
#172572=CARTESIAN_POINT('Ctrl Pts',(-27.7715523368211,-14.070054704419,
113.741825957378)) ;
#172573=CARTESIAN_POINT('Ctrl Pts',(-27.7518733154646,-14.0278445854345,
113.681886834829)) ;
#172574=CARTESIAN_POINT('Ctrl Pts',(-27.7020071019376,-14.2444016591037,
113.494631735179)) ;
#172575=CARTESIAN_POINT('Ctrl Pts',(-27.6865130848051,-14.1870110797581,
113.447439460386)) ;
#172576=CARTESIAN_POINT('Ctrl Pts',(-27.7603169106574,-14.1870111286872,
113.423208365192)) ;
#172577=CARTESIAN_POINT('Ctrl Pts',(-27.8341207365098,-14.1870111776162,
113.398977269998)) ;
#172578=CARTESIAN_POINT('Ctrl Pts',(-27.8496147536422,-14.2444017569618,
113.446169544791)) ;
#172579=CARTESIAN_POINT('Ctrl Pts',(-27.8651087707747,-14.3017923363074,
113.493361819585)) ;
#172580=CARTESIAN_POINT('Ctrl Pts',(-27.7913049449223,-14.3017922873783,
113.517592914779)) ;
#172581=CARTESIAN_POINT('Ctrl Pts',(-27.71750111907,-14.3017922384493,113.541824009973)) ;
#172582=CARTESIAN_POINT('Ctrl Pts',(-27.7020071019376,-14.2444016591037,
113.494631735179)) ;
#172583=CARTESIAN_POINT('Ctrl Pts',(-27.6362880745386,-14.4026063876543,
113.259009109115)) ;
#172584=CARTESIAN_POINT('Ctrl Pts',(-27.6260934718267,-14.3340872602138,
113.227957995732)) ;
#172585=CARTESIAN_POINT('Ctrl Pts',(-27.699897292193,-14.3340872957345,
113.203726883828)) ;
#172586=CARTESIAN_POINT('Ctrl Pts',(-27.7737011125594,-14.3340873312552,
113.179495771925)) ;
#172587=CARTESIAN_POINT('Ctrl Pts',(-27.7838957152713,-14.4026064586957,
113.210546885308)) ;
#172588=CARTESIAN_POINT('Ctrl Pts',(-27.7940903179833,-14.4711255861363,
113.241597998692)) ;
#172589=CARTESIAN_POINT('Ctrl Pts',(-27.7202864976169,-14.4711255506156,
113.265829110596)) ;
#172590=CARTESIAN_POINT('Ctrl Pts',(-27.6464826772506,-14.4711255150949,
113.290060222499)) ;
#172591=CARTESIAN_POINT('Ctrl Pts',(-27.6362880745386,-14.4026063876543,
113.259009109115)) ;
#172592=CARTESIAN_POINT('Ctrl Pts',(-27.5597118203589,-14.4903817315252,
112.990103568615)) ;
#172593=CARTESIAN_POINT('Ctrl Pts',(-27.5555865779174,-14.4156342594261,
112.977538747483)) ;
#172594=CARTESIAN_POINT('Ctrl Pts',(-27.6293903936794,-14.4156342751567,
112.953307621556)) ;
#172595=CARTESIAN_POINT('Ctrl Pts',(-27.7031942094413,-14.4156342908872,
112.929076495628)) ;
#172596=CARTESIAN_POINT('Ctrl Pts',(-27.7073194518829,-14.4903817629863,
112.94164131676)) ;
#172597=CARTESIAN_POINT('Ctrl Pts',(-27.7114446943244,-14.5651292350854,
112.954206137892)) ;
#172598=CARTESIAN_POINT('Ctrl Pts',(-27.6376408785625,-14.5651292193548,
112.97843726382)) ;
#172599=CARTESIAN_POINT('Ctrl Pts',(-27.5638370628005,-14.5651292036242,
113.002668389747)) ;
#172600=CARTESIAN_POINT('Ctrl Pts',(-27.5597118203589,-14.4903817315252,
112.990103568615)) ;
#172601=CARTESIAN_POINT('Ctrl Pts',(-27.4797523581831,-14.5006966747965,
112.711230829165)) ;
#172602=CARTESIAN_POINT('Ctrl Pts',(-27.4819346624663,-14.4251205193326,
112.71787777773)) ;
#172603=CARTESIAN_POINT('Ctrl Pts',(-27.5557384764387,-14.425120510433,
112.693646646351)) ;
#172604=CARTESIAN_POINT('Ctrl Pts',(-27.6295422904111,-14.4251205015334,
112.669415514973)) ;
#172605=CARTESIAN_POINT('Ctrl Pts',(-27.6273599861279,-14.5006966569974,
112.662768566408)) ;
#172606=CARTESIAN_POINT('Ctrl Pts',(-27.6251776818447,-14.5762728124613,
112.656121617843)) ;
#172607=CARTESIAN_POINT('Ctrl Pts',(-27.5513738678723,-14.5762728213609,
112.680352749221)) ;
#172608=CARTESIAN_POINT('Ctrl Pts',(-27.4775700538999,-14.5762728302605,
112.7045838806)) ;
#172609=CARTESIAN_POINT('Ctrl Pts',(-27.4797523581831,-14.5006966747965,
112.711230829165)) ;
#172610=CARTESIAN_POINT('Ctrl Pts',(-27.4018724922626,-14.4339382681578,
112.438561635708)) ;
#172611=CARTESIAN_POINT('Ctrl Pts',(-27.410228957115,-14.3629125582236,
112.464014081264)) ;
#172612=CARTESIAN_POINT('Ctrl Pts',(-27.4840327714468,-14.3629125229021,
112.43978295098)) ;
#172613=CARTESIAN_POINT('Ctrl Pts',(-27.5578365857786,-14.3629124875806,
112.415551820697)) ;
#172614=CARTESIAN_POINT('Ctrl Pts',(-27.5494801209262,-14.4339381975148,
112.39009937514)) ;
#172615=CARTESIAN_POINT('Ctrl Pts',(-27.5411236560738,-14.504963907449,
112.364646929584)) ;
#172616=CARTESIAN_POINT('Ctrl Pts',(-27.467319841742,-14.5049639427705,
112.388878059868)) ;
#172617=CARTESIAN_POINT('Ctrl Pts',(-27.3935160274102,-14.504963978092,
112.413109190151)) ;
#172618=CARTESIAN_POINT('Ctrl Pts',(-27.4018724922626,-14.4339382681578,
112.438561635708)) ;
#172619=CARTESIAN_POINT('Ctrl Pts',(-27.3324980422359,-14.293783753758,
112.191696223905)) ;
#172620=CARTESIAN_POINT('Ctrl Pts',(-27.3464460369964,-14.2324386627931,
112.234179567453)) ;
#172621=CARTESIAN_POINT('Ctrl Pts',(-27.4202498542642,-14.2324386013355,
112.209948446112)) ;
#172622=CARTESIAN_POINT('Ctrl Pts',(-27.494053671532,-14.2324385398779,
112.185717324771)) ;
#172623=CARTESIAN_POINT('Ctrl Pts',(-27.4801056767715,-14.2937836308428,
112.143233981223)) ;
#172624=CARTESIAN_POINT('Ctrl Pts',(-27.466157682011,-14.3551287218076,
112.100750637675)) ;
#172625=CARTESIAN_POINT('Ctrl Pts',(-27.3923538647432,-14.3551287832652,
112.124981759016)) ;
#172626=CARTESIAN_POINT('Ctrl Pts',(-27.3185500474754,-14.3551288447229,
112.149212880357)) ;
#172627=CARTESIAN_POINT('Ctrl Pts',(-27.3324980422359,-14.293783753758,
112.191696223905)) ;
#172628=CARTESIAN_POINT('Ctrl Pts',(-27.2777747513304,-14.0908689343358,
111.989522154825)) ;
#172629=CARTESIAN_POINT('Ctrl Pts',(-27.2962983047962,-14.0436003014087,
112.045941911977)) ;
#172630=CARTESIAN_POINT('Ctrl Pts',(-27.3701021276253,-14.0436002177779,
112.021710807575)) ;
#172631=CARTESIAN_POINT('Ctrl Pts',(-27.4439059504545,-14.0436001341472,
111.997479703173)) ;
#172632=CARTESIAN_POINT('Ctrl Pts',(-27.4253823969886,-14.0908687670742,
111.941059946021)) ;
#172633=CARTESIAN_POINT('Ctrl Pts',(-27.4068588435228,-14.1381374000013,
111.88464018887)) ;
#172634=CARTESIAN_POINT('Ctrl Pts',(-27.3330550206936,-14.1381374836321,
111.908871293272)) ;
#172635=CARTESIAN_POINT('Ctrl Pts',(-27.2592511978645,-14.1381375672628,
111.933102397674)) ;
#172636=CARTESIAN_POINT('Ctrl Pts',(-27.2777747513304,-14.0908689343358,
111.989522154825)) ;
#172637=CARTESIAN_POINT('Ctrl Pts',(-27.2422913767248,-13.8416080598376,
111.846186549763)) ;
#172638=CARTESIAN_POINT('Ctrl Pts',(-27.2640489773755,-13.8116727384737,
111.912456692852)) ;
#172639=CARTESIAN_POINT('Ctrl Pts',(-27.3378528076801,-13.8116726391883,
111.888225611219)) ;
#172640=CARTESIAN_POINT('Ctrl Pts',(-27.4116566379846,-13.8116725399028,
111.863994529586)) ;
#172641=CARTESIAN_POINT('Ctrl Pts',(-27.3898990373339,-13.8416078612666,
111.797724386496)) ;
#172642=CARTESIAN_POINT('Ctrl Pts',(-27.3681414366833,-13.8715431826305,
111.731454243407)) ;
#172643=CARTESIAN_POINT('Ctrl Pts',(-27.2943376063787,-13.871543281916,
111.75568532504)) ;
#172644=CARTESIAN_POINT('Ctrl Pts',(-27.2205337760742,-13.8715433812015,
111.779916406673)) ;
#172645=CARTESIAN_POINT('Ctrl Pts',(-27.2422913767248,-13.8416080598376,
111.846186549763)) ;
#172646=CARTESIAN_POINT('Ctrl Pts',(-27.2289317162675,-13.5600342116363,
111.76994926141)) ;
#172647=CARTESIAN_POINT('Ctrl Pts',(-27.2523897657781,-13.5497128461305,
111.841398697373)) ;
#172648=CARTESIAN_POINT('Ctrl Pts',(-27.3261936047793,-13.5497127385965,
111.817167642229)) ;
#172649=CARTESIAN_POINT('Ctrl Pts',(-27.3999974437804,-13.5497126310626,
111.792936587084)) ;
#172650=CARTESIAN_POINT('Ctrl Pts',(-27.3765393942697,-13.5600339965684,
111.721487151121)) ;
#172651=CARTESIAN_POINT('Ctrl Pts',(-27.3530813447591,-13.5703553620741,
111.650037715158)) ;
#172652=CARTESIAN_POINT('Ctrl Pts',(-27.279277505758,-13.5703554696081,
111.674268770302)) ;
#172653=CARTESIAN_POINT('Ctrl Pts',(-27.2054736667568,-13.570355577142,
111.698499825447)) ;
#172654=CARTESIAN_POINT('Ctrl Pts',(-27.2289317162675,-13.5600342116363,
111.76994926141)) ;
#172655=CARTESIAN_POINT('Ctrl Pts',(-27.2396919341479,-13.2694053226454,
111.767331334353)) ;
#172656=CARTESIAN_POINT('Ctrl Pts',(-27.2631657848898,-13.2793593921655,
111.838828898307)) ;
#172657=CARTESIAN_POINT('Ctrl Pts',(-27.3369696329492,-13.2793592852709,
111.814597870752)) ;
#172658=CARTESIAN_POINT('Ctrl Pts',(-27.4107734810085,-13.2793591783763,
111.790366843197)) ;
#172659=CARTESIAN_POINT('Ctrl Pts',(-27.3872996302666,-13.2694051088563,
111.718869279243)) ;
#172660=CARTESIAN_POINT('Ctrl Pts',(-27.3638257795247,-13.2594510393362,
111.647371715289)) ;
#172661=CARTESIAN_POINT('Ctrl Pts',(-27.2900219314654,-13.2594511462308,
111.671602742844)) ;
#172662=CARTESIAN_POINT('Ctrl Pts',(-27.216218083406,-13.2594512531254,
111.695833770399)) ;
#172663=CARTESIAN_POINT('Ctrl Pts',(-27.2396919341479,-13.2694053226454,
111.767331334353)) ;
#172664=CARTESIAN_POINT('Ctrl Pts',(-27.2747065150055,-12.9879324368107,
111.838387958707)) ;
#172665=CARTESIAN_POINT('Ctrl Pts',(-27.2965072947084,-13.0175527392448,
111.904789618186)) ;
#172666=CARTESIAN_POINT('Ctrl Pts',(-27.3703111512458,-13.0175526420622,
111.880558616454)) ;
#172667=CARTESIAN_POINT('Ctrl Pts',(-27.4441150077832,-13.0175525448795,
111.856327614721)) ;
#172668=CARTESIAN_POINT('Ctrl Pts',(-27.4223142280803,-12.9879322424453,
111.789925955243)) ;
#172669=CARTESIAN_POINT('Ctrl Pts',(-27.4005134483774,-12.9583119400111,
111.723524295764)) ;
#172670=CARTESIAN_POINT('Ctrl Pts',(-27.32670959184,-12.9583120371938,111.747755297496)) ;
#172671=CARTESIAN_POINT('Ctrl Pts',(-27.2529057353027,-12.9583121343765,
111.771986299228)) ;
#172672=CARTESIAN_POINT('Ctrl Pts',(-27.2747065150055,-12.9879324368107,
111.838387958707)) ;
#172673=CARTESIAN_POINT('Ctrl Pts',(-27.3317369332919,-12.7391527795793,
111.976760771784)) ;
#172674=CARTESIAN_POINT('Ctrl Pts',(-27.3503195226965,-12.786186317019,
112.033360342819)) ;
#172675=CARTESIAN_POINT('Ctrl Pts',(-27.4241233863091,-12.7861862364123,
112.009129362637)) ;
#172676=CARTESIAN_POINT('Ctrl Pts',(-27.4979272499217,-12.7861861558057,
111.984898382455)) ;
#172677=CARTESIAN_POINT('Ctrl Pts',(-27.4793446605171,-12.739152618366,
111.92829881142)) ;
#172678=CARTESIAN_POINT('Ctrl Pts',(-27.4607620711125,-12.6921190809264,
111.871699240384)) ;
#172679=CARTESIAN_POINT('Ctrl Pts',(-27.3869582074999,-12.692119161533,
111.895930220567)) ;
#172680=CARTESIAN_POINT('Ctrl Pts',(-27.3131543438873,-12.6921192421396,
111.920161200749)) ;
#172681=CARTESIAN_POINT('Ctrl Pts',(-27.3317369332919,-12.7391527795793,
111.976760771784)) ;
#172682=CARTESIAN_POINT('Ctrl Pts',(-27.4079460102453,-12.5377712145214,
112.173389855419)) ;
#172683=CARTESIAN_POINT('Ctrl Pts',(-27.4219701244179,-12.5989350569668,
112.216105046329)) ;
#172684=CARTESIAN_POINT('Ctrl Pts',(-27.495773993018,-12.5989349988532,
112.191874081337)) ;
#172685=CARTESIAN_POINT('Ctrl Pts',(-27.569577861618,-12.5989349407397,
112.167643116346)) ;
#172686=CARTESIAN_POINT('Ctrl Pts',(-27.5555537474453,-12.5377710982944,
112.124927925436)) ;
#172687=CARTESIAN_POINT('Ctrl Pts',(-27.5415296332727,-12.476607255849,
112.082212734526)) ;
#172688=CARTESIAN_POINT('Ctrl Pts',(-27.4677257646726,-12.4766073139625,
112.106443699517)) ;
#172689=CARTESIAN_POINT('Ctrl Pts',(-27.3939218960726,-12.476607372076,
112.130674664508)) ;
#172690=CARTESIAN_POINT('Ctrl Pts',(-27.4079460102453,-12.5377712145214,
112.173389855419)) ;
#172691=CARTESIAN_POINT('Ctrl Pts',(-27.4985458011396,-12.3995925801182,
112.413836694041)) ;
#172692=CARTESIAN_POINT('Ctrl Pts',(-27.5070002124818,-12.4704956782947,
112.439587468698)) ;
#172693=CARTESIAN_POINT('Ctrl Pts',(-27.5808040834856,-12.4704956456056,
112.415356511028)) ;
#172694=CARTESIAN_POINT('Ctrl Pts',(-27.6546079544894,-12.4704956129164,
112.391125553358)) ;
#172695=CARTESIAN_POINT('Ctrl Pts',(-27.6461535431472,-12.39959251474,112.365374778702)) ;
#172696=CARTESIAN_POINT('Ctrl Pts',(-27.6376991318051,-12.3286894165636,
112.339624004045)) ;
#172697=CARTESIAN_POINT('Ctrl Pts',(-27.5638952608012,-12.3286894492527,
112.363854961715)) ;
#172698=CARTESIAN_POINT('Ctrl Pts',(-27.4900913897974,-12.3286894819418,
112.388085919384)) ;
#172699=CARTESIAN_POINT('Ctrl Pts',(-27.4985458011396,-12.3995925801182,
112.413836694041)) ;
#172700=CARTESIAN_POINT('Ctrl Pts',(-27.5975500958584,-12.33457880474,112.679937373876)) ;
#172701=CARTESIAN_POINT('Ctrl Pts',(-27.5998384646325,-12.4101277476762,
112.686907377645)) ;
#172702=CARTESIAN_POINT('Ctrl Pts',(-27.6736423355571,-12.4101277401761,
112.662676419734)) ;
#172703=CARTESIAN_POINT('Ctrl Pts',(-27.7474462064816,-12.410127732676,
112.638445461823)) ;
#172704=CARTESIAN_POINT('Ctrl Pts',(-27.7451578377076,-12.3345787897397,
112.631475458053)) ;
#172705=CARTESIAN_POINT('Ctrl Pts',(-27.7428694689335,-12.2590298468035,
112.624505454283)) ;
#172706=CARTESIAN_POINT('Ctrl Pts',(-27.6690655980089,-12.2590298543036,
112.648736412195)) ;
#172707=CARTESIAN_POINT('Ctrl Pts',(-27.5952617270843,-12.2590298618037,
112.672967370106)) ;
#172708=CARTESIAN_POINT('Ctrl Pts',(-27.5975500958584,-12.33457880474,112.679937373876)) ;
#172709=CARTESIAN_POINT('Ctrl Pts',(-27.6987081284443,-12.3470312097476,
112.952618142842)) ;
#172710=CARTESIAN_POINT('Ctrl Pts',(-27.6946703520646,-12.4218246112721,
112.940319729069)) ;
#172711=CARTESIAN_POINT('Ctrl Pts',(-27.7684742206581,-12.4218246263605,
112.916088764058)) ;
#172712=CARTESIAN_POINT('Ctrl Pts',(-27.8422780892516,-12.4218246414487,
112.891857799047)) ;
#172713=CARTESIAN_POINT('Ctrl Pts',(-27.8463158656312,-12.3470312399242,
112.904156212819)) ;
#172714=CARTESIAN_POINT('Ctrl Pts',(-27.8503536420109,-12.2722378383997,
112.916454626591)) ;
#172715=CARTESIAN_POINT('Ctrl Pts',(-27.7765497734175,-12.2722378233114,
112.940685591603)) ;
#172716=CARTESIAN_POINT('Ctrl Pts',(-27.7027459048239,-12.2722378082231,
112.964916556614)) ;
#172717=CARTESIAN_POINT('Ctrl Pts',(-27.6987081284443,-12.3470312097476,
112.952618142842)) ;
#172718=CARTESIAN_POINT('Ctrl Pts',(-27.7957338413212,-12.4361986060041,
113.212662497894)) ;
#172719=CARTESIAN_POINT('Ctrl Pts',(-27.7856498769021,-12.5048795255924,
113.181948370757)) ;
#172720=CARTESIAN_POINT('Ctrl Pts',(-27.8594537412216,-12.5048795584336,
113.157717392728)) ;
#172721=CARTESIAN_POINT('Ctrl Pts',(-27.9332576055411,-12.5048795912748,
113.133486414699)) ;
#172722=CARTESIAN_POINT('Ctrl Pts',(-27.9433415699602,-12.4361986716865,
113.164200541836)) ;
#172723=CARTESIAN_POINT('Ctrl Pts',(-27.9534255343793,-12.3675177520983,
113.194914668972)) ;
#172724=CARTESIAN_POINT('Ctrl Pts',(-27.8796216700598,-12.367517719257,
113.219145647001)) ;
#172725=CARTESIAN_POINT('Ctrl Pts',(-27.8058178057402,-12.3675176864158,
113.24337662503)) ;
#172726=CARTESIAN_POINT('Ctrl Pts',(-27.7957338413212,-12.4361986060041,
113.212662497894)) ;
#172727=CARTESIAN_POINT('Ctrl Pts',(-27.8823349907965,-12.5959885808789,
113.440924329999)) ;
#172728=CARTESIAN_POINT('Ctrl Pts',(-27.8669240730479,-12.6536171134987,
113.39398516236)) ;
#172729=CARTESIAN_POINT('Ctrl Pts',(-27.9407279319121,-12.6536171574683,
113.369754167714)) ;
#172730=CARTESIAN_POINT('Ctrl Pts',(-28.0145317907762,-12.653617201438,
113.345523173069)) ;
#172731=CARTESIAN_POINT('Ctrl Pts',(-28.0299427085247,-12.5959886688182,
113.392462340708)) ;
#172732=CARTESIAN_POINT('Ctrl Pts',(-28.0453536262733,-12.5383601361984,
113.439401508348)) ;
#172733=CARTESIAN_POINT('Ctrl Pts',(-27.9715497674092,-12.5383600922288,
113.463632502993)) ;
#172734=CARTESIAN_POINT('Ctrl Pts',(-27.897745908545,-12.5383600482591,
113.487863497639)) ;
#172735=CARTESIAN_POINT('Ctrl Pts',(-27.8823349907965,-12.5959885808789,
113.440924329999)) ;
#172736=CARTESIAN_POINT('Ctrl Pts',(-27.9528390482715,-12.8143066918053,
113.620229888243)) ;
#172737=CARTESIAN_POINT('Ctrl Pts',(-27.9332154668164,-12.8567794160869,
113.560459626507)) ;
#172738=CARTESIAN_POINT('Ctrl Pts',(-28.0070193200838,-12.8567794648258,
113.536228614815)) ;
#172739=CARTESIAN_POINT('Ctrl Pts',(-28.0808231733512,-12.8567795135646,
113.511997603122)) ;
#172740=CARTESIAN_POINT('Ctrl Pts',(-28.1004467548063,-12.814306789283,
113.571767864859)) ;
#172741=CARTESIAN_POINT('Ctrl Pts',(-28.1200703362614,-12.7718340650015,
113.631538126595)) ;
#172742=CARTESIAN_POINT('Ctrl Pts',(-28.046266482994,-12.7718340162626,
113.655769138288)) ;
#172743=CARTESIAN_POINT('Ctrl Pts',(-27.9724626297266,-12.7718339675238,
113.68000014998)) ;
#172744=CARTESIAN_POINT('Ctrl Pts',(-27.9528390482715,-12.8143066918053,
113.620229888243)) ;
#172745=CARTESIAN_POINT('Ctrl Pts',(-28.0032144890018,-13.0760276863323,
113.738192855668)) ;
#172746=CARTESIAN_POINT('Ctrl Pts',(-27.9807778893923,-13.1002911910354,
113.669854594344)) ;
#172747=CARTESIAN_POINT('Ctrl Pts',(-28.0545817373889,-13.1002912381593,
113.645623566597)) ;
#172748=CARTESIAN_POINT('Ctrl Pts',(-28.1283855853854,-13.1002912852831,
113.621392538851)) ;
#172749=CARTESIAN_POINT('Ctrl Pts',(-28.150822184995,-13.07602778058,113.689730800176)) ;
#172750=CARTESIAN_POINT('Ctrl Pts',(-28.1732587846045,-13.0517642758768,
113.758069061501)) ;
#172751=CARTESIAN_POINT('Ctrl Pts',(-28.0994549366079,-13.051764228753,
113.782300089247)) ;
#172752=CARTESIAN_POINT('Ctrl Pts',(-28.0256510886113,-13.0517641816292,
113.806531116993)) ;
#172753=CARTESIAN_POINT('Ctrl Pts',(-28.0032144890018,-13.0760276863323,
113.738192855668)) ;
#172754=CARTESIAN_POINT('Ctrl Pts',(-28.0304977945719,-13.3628060373472,
113.785759354195)) ;
#172755=CARTESIAN_POINT('Ctrl Pts',(-28.0068574169751,-13.3670829170375,
113.713754579168)) ;
#172756=CARTESIAN_POINT('Ctrl Pts',(-28.0806612607687,-13.3670829569658,
113.68952353862)) ;
#172757=CARTESIAN_POINT('Ctrl Pts',(-28.1544651045623,-13.3670829968941,
113.665292498073)) ;
#172758=CARTESIAN_POINT('Ctrl Pts',(-28.1781054821591,-13.3628061172038,
113.7372972731)) ;
#172759=CARTESIAN_POINT('Ctrl Pts',(-28.2017458597559,-13.3585292375136,
113.809302048127)) ;
#172760=CARTESIAN_POINT('Ctrl Pts',(-28.1279420159623,-13.3585291975852,
113.833533088674)) ;
#172761=CARTESIAN_POINT('Ctrl Pts',(-28.0541381721687,-13.3585291576569,
113.857764129222)) ;
#172762=CARTESIAN_POINT('Ctrl Pts',(-28.0304977945719,-13.3628060373472,
113.785759354195)) ;
#172763=CARTESIAN_POINT('Ctrl Pts',(-28.0334235158312,-13.6523296523906,
113.759282572633)) ;
#172764=CARTESIAN_POINT('Ctrl Pts',(-28.0102753813997,-13.6363976370677,
113.688777090714)) ;
#172765=CARTESIAN_POINT('Ctrl Pts',(-28.0840792224513,-13.636397668316,
113.664546041814)) ;
#172766=CARTESIAN_POINT('Ctrl Pts',(-28.157883063503,-13.6363976995644,
113.640314992915)) ;
#172767=CARTESIAN_POINT('Ctrl Pts',(-28.1810311979345,-13.6523297148873,
113.710820474834)) ;
#172768=CARTESIAN_POINT('Ctrl Pts',(-28.2041793323661,-13.6682617302103,
113.781325956754)) ;
#172769=CARTESIAN_POINT('Ctrl Pts',(-28.1303754913144,-13.6682616989619,
113.805557005653)) ;
#172770=CARTESIAN_POINT('Ctrl Pts',(-28.0565716502628,-13.6682616677135,
113.829788054553)) ;
#172771=CARTESIAN_POINT('Ctrl Pts',(-28.0334235158312,-13.6523296523906,
113.759282572633)) ;
#172772=CARTESIAN_POINT('Ctrl Pts',(-28.012789007875,-13.9253061411165,
113.661037033332)) ;
#172773=CARTESIAN_POINT('Ctrl Pts',(-27.9917790894458,-13.8902899618178,
113.597044212208)) ;
#172774=CARTESIAN_POINT('Ctrl Pts',(-28.0655829290732,-13.8902899830873,
113.57281315897)) ;
#172775=CARTESIAN_POINT('Ctrl Pts',(-28.1393867687006,-13.8902900043567,
113.548582105733)) ;
#172776=CARTESIAN_POINT('Ctrl Pts',(-28.1603966871298,-13.9253061836553,
113.612574926857)) ;
#172777=CARTESIAN_POINT('Ctrl Pts',(-28.1814066055589,-13.960322362954,
113.676567747981)) ;
#172778=CARTESIAN_POINT('Ctrl Pts',(-28.1076027659315,-13.9603223416845,
113.700798801219)) ;
#172779=CARTESIAN_POINT('Ctrl Pts',(-28.0337989263041,-13.9603223204151,
113.725029854456)) ;
#172780=CARTESIAN_POINT('Ctrl Pts',(-28.012789007875,-13.9253061411165,
113.661037033332)) ;
#172781=CARTESIAN_POINT('Ctrl Pts',(-27.9702967268525,-14.1634851116196,
113.495964568205)) ;
#172782=CARTESIAN_POINT('Ctrl Pts',(-27.9529596170839,-14.1117847123966,
113.443158529478)) ;
#172783=CARTESIAN_POINT('Ctrl Pts',(-28.0267634570671,-14.1117847230889,
113.418927477324)) ;
#172784=CARTESIAN_POINT('Ctrl Pts',(-28.1005672970504,-14.1117847337813,
113.39469642517)) ;
#172785=CARTESIAN_POINT('Ctrl Pts',(-28.1179044068189,-14.1634851330044,
113.447502463897)) ;
#172786=CARTESIAN_POINT('Ctrl Pts',(-28.1352415165875,-14.2151855322274,
113.500308502624)) ;
#172787=CARTESIAN_POINT('Ctrl Pts',(-28.0614376766043,-14.215185521535,
113.524539554778)) ;
#172788=CARTESIAN_POINT('Ctrl Pts',(-27.987633836621,-14.2151855108427,
113.548770606932)) ;
#172789=CARTESIAN_POINT('Ctrl Pts',(-27.9702967268525,-14.1634851116196,
113.495964568205)) ;
#172790=CARTESIAN_POINT('Ctrl Pts',(-27.9105275341347,-14.3462889334782,
113.278595975283)) ;
#172791=CARTESIAN_POINT('Ctrl Pts',(-27.8980686802056,-14.2817465742021,
113.240648316631)) ;
#172792=CARTESIAN_POINT('Ctrl Pts',(-27.9718725209529,-14.2817465788419,
113.216417266805)) ;
#172793=CARTESIAN_POINT('Ctrl Pts',(-28.0456763617003,-14.2817465834817,
113.192186216979)) ;
#172794=CARTESIAN_POINT('Ctrl Pts',(-28.0581352156294,-14.3462889427578,
113.23013387563)) ;
#172795=CARTESIAN_POINT('Ctrl Pts',(-28.0705940695586,-14.4108313020339,
113.268081534282)) ;
#172796=CARTESIAN_POINT('Ctrl Pts',(-27.9967902288112,-14.4108312973941,
113.292312584108)) ;
#172797=CARTESIAN_POINT('Ctrl Pts',(-27.9229863880639,-14.4108312927542,
113.316543633935)) ;
#172798=CARTESIAN_POINT('Ctrl Pts',(-27.9105275341347,-14.3462889334782,
113.278595975283)) ;
#172799=CARTESIAN_POINT('Ctrl Pts',(-27.8378250216826,-14.463737953108,
113.021649522263)) ;
#172800=CARTESIAN_POINT('Ctrl Pts',(-27.8311587392697,-14.3908972873577,
113.001345101705)) ;
#172801=CARTESIAN_POINT('Ctrl Pts',(-27.9049625815246,-14.3908972879061,
112.977114056471)) ;
#172802=CARTESIAN_POINT('Ctrl Pts',(-27.9787664237794,-14.3908972884545,
112.952883011236)) ;
#172803=CARTESIAN_POINT('Ctrl Pts',(-27.9854327061922,-14.4637379542048,
112.973187431793)) ;
#172804=CARTESIAN_POINT('Ctrl Pts',(-27.9920989886051,-14.5365786199551,
112.993491852351)) ;
#172805=CARTESIAN_POINT('Ctrl Pts',(-27.9182951463503,-14.5365786194067,
113.017722897585)) ;
#172806=CARTESIAN_POINT('Ctrl Pts',(-27.8444913040955,-14.5365786188583,
113.04195394282)) ;
#172807=CARTESIAN_POINT('Ctrl Pts',(-27.8378250216826,-14.463737953108,
113.021649522263)) ;
#172808=CARTESIAN_POINT('Ctrl Pts',(-27.7583865450976,-14.5058926586063,
112.744197147275)) ;
#172809=CARTESIAN_POINT('Ctrl Pts',(-27.7579918688641,-14.4299991748241,
112.742995027138)) ;
#172810=CARTESIAN_POINT('Ctrl Pts',(-27.8317957124424,-14.4299991745337,
112.718763985934)) ;
#172811=CARTESIAN_POINT('Ctrl Pts',(-27.9055995560207,-14.4299991742434,
112.69453294473)) ;
#172812=CARTESIAN_POINT('Ctrl Pts',(-27.9059942322542,-14.5058926580256,
112.695735064867)) ;
#172813=CARTESIAN_POINT('Ctrl Pts',(-27.9063889084876,-14.5817861418077,
112.696937185004)) ;
#172814=CARTESIAN_POINT('Ctrl Pts',(-27.8325850649093,-14.5817861420981,
112.721168226207)) ;
#172815=CARTESIAN_POINT('Ctrl Pts',(-27.758781221331,-14.5817861423884,
112.745399267411)) ;
#172816=CARTESIAN_POINT('Ctrl Pts',(-27.7583865450976,-14.5058926586063,
112.744197147275)) ;
#172817=CARTESIAN_POINT('Ctrl Pts',(-27.6788939974933,-14.4703114180475,
112.466675473693)) ;
#172818=CARTESIAN_POINT('Ctrl Pts',(-27.6847821157798,-14.3967894542526,
112.484609731894)) ;
#172819=CARTESIAN_POINT('Ctrl Pts',(-27.7585859600674,-14.3967894548516,
112.460378692851)) ;
#172820=CARTESIAN_POINT('Ctrl Pts',(-27.832389804355,-14.3967894554506,
112.436147653808)) ;
#172821=CARTESIAN_POINT('Ctrl Pts',(-27.8265016860686,-14.4703114192455,
112.418213395607)) ;
#172822=CARTESIAN_POINT('Ctrl Pts',(-27.8206135677821,-14.5438333830403,
112.400279137406)) ;
#172823=CARTESIAN_POINT('Ctrl Pts',(-27.7468097234945,-14.5438333824413,
112.424510176449)) ;
#172824=CARTESIAN_POINT('Ctrl Pts',(-27.6730058792069,-14.5438333818423,
112.448741215493)) ;
#172825=CARTESIAN_POINT('Ctrl Pts',(-27.6788939974933,-14.4703114180475,
112.466675473693)) ;
#172826=CARTESIAN_POINT('Ctrl Pts',(-27.6052569535695,-14.359046732277,
112.206841206659)) ;
#172827=CARTESIAN_POINT('Ctrl Pts',(-27.6170316417398,-14.2931851690986,
112.242705006923)) ;
#172828=CARTESIAN_POINT('Ctrl Pts',(-27.6908354860316,-14.2931851708445,
112.218473967892)) ;
#172829=CARTESIAN_POINT('Ctrl Pts',(-27.7646393303234,-14.2931851725905,
112.194242928862)) ;
#172830=CARTESIAN_POINT('Ctrl Pts',(-27.7528646421531,-14.3590467357689,
112.158379128598)) ;
#172831=CARTESIAN_POINT('Ctrl Pts',(-27.7410899539827,-14.4249082989473,
112.122515328334)) ;
#172832=CARTESIAN_POINT('Ctrl Pts',(-27.667286109691,-14.4249082972013,
112.146746367365)) ;
#172833=CARTESIAN_POINT('Ctrl Pts',(-27.5934822653991,-14.4249082954554,
112.170977406395)) ;
#172834=CARTESIAN_POINT('Ctrl Pts',(-27.6052569535695,-14.359046732277,
112.206841206659)) ;
#172835=CARTESIAN_POINT('Ctrl Pts',(-27.5439718545756,-14.1801475215603,
111.984669178458)) ;
#172836=CARTESIAN_POINT('Ctrl Pts',(-27.5607781855889,-14.1266811735188,
112.035858551013)) ;
#172837=CARTESIAN_POINT('Ctrl Pts',(-27.6345820291766,-14.1266811744766,
112.011627509838)) ;
#172838=CARTESIAN_POINT('Ctrl Pts',(-27.7083858727642,-14.1266811754344,
111.987396468662)) ;
#172839=CARTESIAN_POINT('Ctrl Pts',(-27.6915795417509,-14.1801475234759,
111.936207096108)) ;
#172840=CARTESIAN_POINT('Ctrl Pts',(-27.6747732107375,-14.2336138715174,
111.885017723554)) ;
#172841=CARTESIAN_POINT('Ctrl Pts',(-27.6009693671499,-14.2336138705596,
111.909248764729)) ;
#172842=CARTESIAN_POINT('Ctrl Pts',(-27.5271655235622,-14.2336138696018,
111.933479805904)) ;
#172843=CARTESIAN_POINT('Ctrl Pts',(-27.5439718545756,-14.1801475215603,
111.984669178458)) ;
#172844=CARTESIAN_POINT('Ctrl Pts',(-27.5001849340851,-13.9475293921824,
111.815922351132)) ;
#172845=CARTESIAN_POINT('Ctrl Pts',(-27.5208054293407,-13.9102276293421,
111.878729052622)) ;
#172846=CARTESIAN_POINT('Ctrl Pts',(-27.5946092722882,-13.9102276274691,
111.854498009497)) ;
#172847=CARTESIAN_POINT('Ctrl Pts',(-27.6684131152357,-13.910227625596,
111.830266966372)) ;
#172848=CARTESIAN_POINT('Ctrl Pts',(-27.64779261998,-13.9475293884362,111.767460264882)) ;
#172849=CARTESIAN_POINT('Ctrl Pts',(-27.6271721247244,-13.9848311512765,
111.704653563392)) ;
#172850=CARTESIAN_POINT('Ctrl Pts',(-27.5533682817769,-13.9848311531496,
111.728884606518)) ;
#172851=CARTESIAN_POINT('Ctrl Pts',(-27.4795644388295,-13.9848311550226,
111.753115649643)) ;
#172852=CARTESIAN_POINT('Ctrl Pts',(-27.5001849340851,-13.9475293921824,
111.815922351132)) ;
#172853=CARTESIAN_POINT('Ctrl Pts',(-27.4775139177375,-13.6767289638667,
111.711432637832)) ;
#172854=CARTESIAN_POINT('Ctrl Pts',(-27.5004808337837,-13.6582814319255,
111.781386158554)) ;
#172855=CARTESIAN_POINT('Ctrl Pts',(-27.5742846765045,-13.6582814248753,
111.757155114738)) ;
#172856=CARTESIAN_POINT('Ctrl Pts',(-27.6480885192253,-13.658281417825,
111.732924070923)) ;
#172857=CARTESIAN_POINT('Ctrl Pts',(-27.6251216031791,-13.6767289497662,
111.662970550201)) ;
#172858=CARTESIAN_POINT('Ctrl Pts',(-27.6021546871329,-13.6951764817073,
111.59301702948)) ;
#172859=CARTESIAN_POINT('Ctrl Pts',(-27.5283508444121,-13.6951764887576,
111.617248073295)) ;
#172860=CARTESIAN_POINT('Ctrl Pts',(-27.4545470016913,-13.6951764958078,
111.641479117111)) ;
#172861=CARTESIAN_POINT('Ctrl Pts',(-27.4775139177375,-13.6767289638667,
111.711432637832)) ;
#172862=CARTESIAN_POINT('Ctrl Pts',(-27.4783712957127,-13.3875048973073,
111.67862173555)) ;
#172863=CARTESIAN_POINT('Ctrl Pts',(-27.5020447372821,-13.3892252145517,
111.750727219135)) ;
#172864=CARTESIAN_POINT('Ctrl Pts',(-27.5758485805916,-13.3892252011116,
111.726496177112)) ;
#172865=CARTESIAN_POINT('Ctrl Pts',(-27.6496524239011,-13.3892251876716,
111.70226513509)) ;
#172866=CARTESIAN_POINT('Ctrl Pts',(-27.6259789823316,-13.3875048704272,
111.630159651505)) ;
#172867=CARTESIAN_POINT('Ctrl Pts',(-27.6023055407622,-13.3857845531828,
111.558054167921)) ;
#172868=CARTESIAN_POINT('Ctrl Pts',(-27.5285016974527,-13.3857845666228,
111.582285209944)) ;
#172869=CARTESIAN_POINT('Ctrl Pts',(-27.4546978541432,-13.3857845800629,
111.606516251966)) ;
#172870=CARTESIAN_POINT('Ctrl Pts',(-27.4783712957127,-13.3875048973073,
111.67862173555)) ;
#172871=CARTESIAN_POINT('Ctrl Pts',(-27.5037549225319,-13.0987597443669,
111.720294424521)) ;
#172872=CARTESIAN_POINT('Ctrl Pts',(-27.5264280564151,-13.1206437742592,
111.789353132464)) ;
#172873=CARTESIAN_POINT('Ctrl Pts',(-27.6002319016533,-13.1206437527101,
111.765122096317)) ;
#172874=CARTESIAN_POINT('Ctrl Pts',(-27.6740357468916,-13.120643731161,
111.740891060169)) ;
#172875=CARTESIAN_POINT('Ctrl Pts',(-27.6513626130085,-13.0987597012687,
111.671832352226)) ;
#172876=CARTESIAN_POINT('Ctrl Pts',(-27.6286894791254,-13.0768756713763,
111.602773644283)) ;
#172877=CARTESIAN_POINT('Ctrl Pts',(-27.5548856338871,-13.0768756929254,
111.627004680431)) ;
#172878=CARTESIAN_POINT('Ctrl Pts',(-27.4810817886488,-13.0768757144745,
111.651235716578)) ;
#172879=CARTESIAN_POINT('Ctrl Pts',(-27.5037549225319,-13.0987597443669,
111.720294424521)) ;
#172880=CARTESIAN_POINT('Ctrl Pts',(-27.5521194249204,-12.8352678817982,
111.832269007795)) ;
#172881=CARTESIAN_POINT('Ctrl Pts',(-27.5721795947561,-12.8755807524781,
111.893369048984)) ;
#172882=CARTESIAN_POINT('Ctrl Pts',(-27.6459834428958,-12.8755807274115,
111.869138021673)) ;
#172883=CARTESIAN_POINT('Ctrl Pts',(-27.7197872910354,-12.8755807023449,
111.844906994363)) ;
#172884=CARTESIAN_POINT('Ctrl Pts',(-27.6997271211997,-12.8352678316651,
111.783806953174)) ;
#172885=CARTESIAN_POINT('Ctrl Pts',(-27.6796669513639,-12.7949549609852,
111.722706911984)) ;
#172886=CARTESIAN_POINT('Ctrl Pts',(-27.6058631032243,-12.7949549860518,
111.746937939295)) ;
#172887=CARTESIAN_POINT('Ctrl Pts',(-27.5320592550846,-12.7949550111184,
111.771168966605)) ;
#172888=CARTESIAN_POINT('Ctrl Pts',(-27.5521194249204,-12.8352678817982,
111.832269007795)) ;
#172889=CARTESIAN_POINT('Ctrl Pts',(-27.6210545802362,-12.6124277096966,
112.006776869347)) ;
#172890=CARTESIAN_POINT('Ctrl Pts',(-27.6370643810052,-12.6683576543549,
112.055540140046)) ;
#172891=CARTESIAN_POINT('Ctrl Pts',(-27.710868232941,-12.6683576284383,
112.031309124298)) ;
#172892=CARTESIAN_POINT('Ctrl Pts',(-27.784672084877,-12.6683576025217,
112.00707810855)) ;
#172893=CARTESIAN_POINT('Ctrl Pts',(-27.768662284108,-12.6124276578634,
111.958314837852)) ;
#172894=CARTESIAN_POINT('Ctrl Pts',(-27.7526524833391,-12.5564977132051,
111.909551567153)) ;
#172895=CARTESIAN_POINT('Ctrl Pts',(-27.6788486314032,-12.5564977391217,
111.933782582901)) ;
#172896=CARTESIAN_POINT('Ctrl Pts',(-27.6050447794673,-12.5564977650383,
111.958013598649)) ;
#172897=CARTESIAN_POINT('Ctrl Pts',(-27.6210545802362,-12.6124277096966,
112.006776869347)) ;
#172898=CARTESIAN_POINT('Ctrl Pts',(-27.7066454648907,-12.4469021309738,
112.231908874782)) ;
#172899=CARTESIAN_POINT('Ctrl Pts',(-27.7174384370252,-12.5144700927407,
112.264782527379)) ;
#172900=CARTESIAN_POINT('Ctrl Pts',(-27.7912422935081,-12.5144700706049,
112.240551525481)) ;
#172901=CARTESIAN_POINT('Ctrl Pts',(-27.865046149991,-12.514470048469,112.216320523583)) ;
#172902=CARTESIAN_POINT('Ctrl Pts',(-27.8542531778566,-12.4469020867021,
112.183446870986)) ;
#172903=CARTESIAN_POINT('Ctrl Pts',(-27.8434602057222,-12.3793341249352,
112.150573218388)) ;
#172904=CARTESIAN_POINT('Ctrl Pts',(-27.7696563492392,-12.3793341470711,
112.174804220286)) ;
#172905=CARTESIAN_POINT('Ctrl Pts',(-27.6958524927563,-12.3793341692069,
112.199035222185)) ;
#172906=CARTESIAN_POINT('Ctrl Pts',(-27.7066454648907,-12.4469021309738,
112.231908874782)) ;
#172907=CARTESIAN_POINT('Ctrl Pts',(-27.803058956122,-12.3516623128813,
112.490078822438)) ;
#172908=CARTESIAN_POINT('Ctrl Pts',(-27.8078704096533,-12.425977537866,
112.504733734657)) ;
#172909=CARTESIAN_POINT('Ctrl Pts',(-27.8816742702308,-12.4259775261186,
112.48050274523)) ;
#172910=CARTESIAN_POINT('Ctrl Pts',(-27.9554781308084,-12.4259775143711,
112.456271755804)) ;
#172911=CARTESIAN_POINT('Ctrl Pts',(-27.9506666772771,-12.3516622893864,
112.441616843585)) ;
#172912=CARTESIAN_POINT('Ctrl Pts',(-27.9458552237458,-12.2773470644017,
112.426961931365)) ;
#172913=CARTESIAN_POINT('Ctrl Pts',(-27.8720513631682,-12.2773470761492,
112.451192920792)) ;
#172914=CARTESIAN_POINT('Ctrl Pts',(-27.7982475025907,-12.2773470878966,
112.475423910219)) ;
#172915=CARTESIAN_POINT('Ctrl Pts',(-27.803058956122,-12.3516623128813,
112.490078822438)) ;
#172916=CARTESIAN_POINT('Ctrl Pts',(-27.903680048157,-12.3325403630455,
112.761274392716)) ;
#172917=CARTESIAN_POINT('Ctrl Pts',(-27.9022032625788,-12.4082975181779,
112.756776343341)) ;
#172918=CARTESIAN_POINT('Ctrl Pts',(-27.9760071256183,-12.4082975217576,
112.732545361413)) ;
#172919=CARTESIAN_POINT('Ctrl Pts',(-28.0498109886578,-12.4082975253373,
112.708314379486)) ;
#172920=CARTESIAN_POINT('Ctrl Pts',(-28.051287774236,-12.3325403702048,
112.71281242886)) ;
#172921=CARTESIAN_POINT('Ctrl Pts',(-28.0527645598142,-12.2567832150723,
112.717310478235)) ;
#172922=CARTESIAN_POINT('Ctrl Pts',(-27.9789606967747,-12.2567832114927,
112.741541460163)) ;
#172923=CARTESIAN_POINT('Ctrl Pts',(-27.9051568337352,-12.256783207913,
112.765772442091)) ;
#172924=CARTESIAN_POINT('Ctrl Pts',(-27.903680048157,-12.3325403630455,
112.761274392716)) ;
#172925=CARTESIAN_POINT('Ctrl Pts',(-28.0035102323783,-12.3912337324793,
113.029751907953)) ;
#172926=CARTESIAN_POINT('Ctrl Pts',(-27.9957978082671,-12.4630030921761,
113.006261109903)) ;
#172927=CARTESIAN_POINT('Ctrl Pts',(-28.069601673032,-12.4630031154162,
112.982030133231)) ;
#172928=CARTESIAN_POINT('Ctrl Pts',(-28.1434055377969,-12.4630031386562,
112.957799156558)) ;
#172929=CARTESIAN_POINT('Ctrl Pts',(-28.1511179619081,-12.3912337789595,
112.981289954608)) ;
#172930=CARTESIAN_POINT('Ctrl Pts',(-28.1588303860193,-12.3194644192627,
113.004780752658)) ;
#172931=CARTESIAN_POINT('Ctrl Pts',(-28.0850265212543,-12.3194643960226,
113.029011729331)) ;
#172932=CARTESIAN_POINT('Ctrl Pts',(-28.0112226564894,-12.3194643727826,
113.053242706003)) ;
#172933=CARTESIAN_POINT('Ctrl Pts',(-28.0035102323783,-12.3912337324793,
113.029751907953)) ;
#172934=CARTESIAN_POINT('Ctrl Pts',(-28.0947250172942,-12.5231371749147,
113.272201796469)) ;
#172935=CARTESIAN_POINT('Ctrl Pts',(-28.0813650498466,-12.5858011581757,
113.231509492776)) ;
#172936=CARTESIAN_POINT('Ctrl Pts',(-28.155168913654,-12.5858012027222,
113.207278513187)) ;
#172937=CARTESIAN_POINT('Ctrl Pts',(-28.2289727774614,-12.5858012472688,
113.183047533598)) ;
#172938=CARTESIAN_POINT('Ctrl Pts',(-28.242332744909,-12.5231372640078,
113.223739837291)) ;
#172939=CARTESIAN_POINT('Ctrl Pts',(-28.2556927123566,-12.4604732807469,
113.264432140985)) ;
#172940=CARTESIAN_POINT('Ctrl Pts',(-28.1818888485492,-12.4604732362004,
113.288663120574)) ;
#172941=CARTESIAN_POINT('Ctrl Pts',(-28.1080849847418,-12.4604731916538,
113.312894100163)) ;
#172942=CARTESIAN_POINT('Ctrl Pts',(-28.0947250172942,-12.5231371749147,
113.272201796469)) ;
#172943=CARTESIAN_POINT('Ctrl Pts',(-28.1723924962388,-12.7192715563506,
113.473290319783)) ;
#172944=CARTESIAN_POINT('Ctrl Pts',(-28.1543246541495,-12.7683330936011,
113.41825858968)) ;
#172945=CARTESIAN_POINT('Ctrl Pts',(-28.2281285149571,-12.7683331592754,
113.394027600954)) ;
#172946=CARTESIAN_POINT('Ctrl Pts',(-28.3019323757647,-12.7683332249497,
113.369796612228)) ;
#172947=CARTESIAN_POINT('Ctrl Pts',(-28.320000217854,-12.7192716876992,
113.424828342331)) ;
#172948=CARTESIAN_POINT('Ctrl Pts',(-28.3380680599432,-12.6702101504487,
113.479860072434)) ;
#172949=CARTESIAN_POINT('Ctrl Pts',(-28.2642641991356,-12.6702100847745,
113.50409106116)) ;
#172950=CARTESIAN_POINT('Ctrl Pts',(-28.190460338328,-12.6702100191002,
113.528322049886)) ;
#172951=CARTESIAN_POINT('Ctrl Pts',(-28.1723924962388,-12.7192715563506,
113.473290319783)) ;
#172952=CARTESIAN_POINT('Ctrl Pts',(-28.2314642131708,-12.9657766439547,
113.617711015076)) ;
#172953=CARTESIAN_POINT('Ctrl Pts',(-28.2099804696281,-12.9976995891968,
113.552275000424)) ;
#172954=CARTESIAN_POINT('Ctrl Pts',(-28.2837843251922,-12.9976996732378,
113.528043995727)) ;
#172955=CARTESIAN_POINT('Ctrl Pts',(-28.3575881807563,-12.9976997572788,
113.503812991031)) ;
#172956=CARTESIAN_POINT('Ctrl Pts',(-28.379071924299,-12.9657768120367,
113.569249005683)) ;
#172957=CARTESIAN_POINT('Ctrl Pts',(-28.4005556678416,-12.9338538667946,
113.634685020334)) ;
#172958=CARTESIAN_POINT('Ctrl Pts',(-28.3267518122775,-12.9338537827536,
113.658916025031)) ;
#172959=CARTESIAN_POINT('Ctrl Pts',(-28.2529479567134,-12.9338536987126,
113.683147029728)) ;
#172960=CARTESIAN_POINT('Ctrl Pts',(-28.2314642131708,-12.9657766439547,
113.617711015076)) ;
#172961=CARTESIAN_POINT('Ctrl Pts',(-28.2683502437793,-13.2450968718509,
113.694515096532)) ;
#172962=CARTESIAN_POINT('Ctrl Pts',(-28.2449953018678,-13.2575654456473,
113.623379713674)) ;
#172963=CARTESIAN_POINT('Ctrl Pts',(-28.3187991502527,-13.2575655425572,
113.599148687111)) ;
#172964=CARTESIAN_POINT('Ctrl Pts',(-28.3926029986376,-13.2575656394672,
113.574917660547)) ;
#172965=CARTESIAN_POINT('Ctrl Pts',(-28.4159579405491,-13.2450970656709,
113.646053043406)) ;
#172966=CARTESIAN_POINT('Ctrl Pts',(-28.4393128824606,-13.2326284918745,
113.717188426264)) ;
#172967=CARTESIAN_POINT('Ctrl Pts',(-28.3655090340758,-13.2326283949646,
113.741419452827)) ;
#172968=CARTESIAN_POINT('Ctrl Pts',(-28.2917051856909,-13.2326282980546,
113.765650479391)) ;
#172969=CARTESIAN_POINT('Ctrl Pts',(-28.2683502437793,-13.2450968718509,
113.694515096532)) ;
#172970=CARTESIAN_POINT('Ctrl Pts',(-28.2811758969267,-13.5349426349563,
113.698268361909)) ;
#172971=CARTESIAN_POINT('Ctrl Pts',(-28.2576221389113,-13.527193346992,
113.626527417346)) ;
#172972=CARTESIAN_POINT('Ctrl Pts',(-28.331425978995,-13.5271934482019,
113.602296365499)) ;
#172973=CARTESIAN_POINT('Ctrl Pts',(-28.4052298190787,-13.5271935494119,
113.578065313651)) ;
#172974=CARTESIAN_POINT('Ctrl Pts',(-28.428783577094,-13.5349428373762,
113.649806258214)) ;
#172975=CARTESIAN_POINT('Ctrl Pts',(-28.4523373351094,-13.5426921253405,
113.721547202778)) ;
#172976=CARTESIAN_POINT('Ctrl Pts',(-28.3785334950258,-13.5426920241306,
113.745778254625)) ;
#172977=CARTESIAN_POINT('Ctrl Pts',(-28.3047296549421,-13.5426919229206,
113.770009306473)) ;
#172978=CARTESIAN_POINT('Ctrl Pts',(-28.2811758969267,-13.5349426349563,
113.698268361909)) ;
#172979=CARTESIAN_POINT('Ctrl Pts',(-28.2698660181599,-13.8188180807124,
113.628205800714)) ;
#172980=CARTESIAN_POINT('Ctrl Pts',(-28.2478040607929,-13.791238496166,
113.561008640298)) ;
#172981=CARTESIAN_POINT('Ctrl Pts',(-28.3216078921359,-13.7912385944122,
113.536777561828)) ;
#172982=CARTESIAN_POINT('Ctrl Pts',(-28.395411723479,-13.7912386926585,
113.512546483358)) ;
#172983=CARTESIAN_POINT('Ctrl Pts',(-28.417473680846,-13.8188182772049,
113.579743643773)) ;
#172984=CARTESIAN_POINT('Ctrl Pts',(-28.439535638213,-13.8463978617513,
113.646940804189)) ;
#172985=CARTESIAN_POINT('Ctrl Pts',(-28.36573180687,-13.846397763505,113.671171882659)) ;
#172986=CARTESIAN_POINT('Ctrl Pts',(-28.2919279755269,-13.8463976652588,
113.695402961129)) ;
#172987=CARTESIAN_POINT('Ctrl Pts',(-28.2698660181599,-13.8188180807124,
113.628205800714)) ;
#172988=CARTESIAN_POINT('Ctrl Pts',(-28.2358683922085,-14.0726519250138,
113.48919153583)) ;
#172989=CARTESIAN_POINT('Ctrl Pts',(-28.2168813064894,-14.027309972795,
113.431359938362)) ;
#172990=CARTESIAN_POINT('Ctrl Pts',(-28.2906851297376,-14.027310058674,
113.407128835236)) ;
#172991=CARTESIAN_POINT('Ctrl Pts',(-28.3644889529858,-14.027310144553,
113.382897732111)) ;
#172992=CARTESIAN_POINT('Ctrl Pts',(-28.383476038705,-14.0726520967719,
113.440729329579)) ;
#172993=CARTESIAN_POINT('Ctrl Pts',(-28.402463124424,-14.1179940489907,
113.498560927047)) ;
#172994=CARTESIAN_POINT('Ctrl Pts',(-28.3286593011758,-14.1179939631117,
113.522792030172)) ;
#172995=CARTESIAN_POINT('Ctrl Pts',(-28.2548554779276,-14.1179938772327,
113.547023133298)) ;
#172996=CARTESIAN_POINT('Ctrl Pts',(-28.2358683922085,-14.0726519250138,
113.48919153583)) ;
#172997=CARTESIAN_POINT('Ctrl Pts',(-28.1827369648301,-14.2790221021537,
113.292024183099)) ;
#172998=CARTESIAN_POINT('Ctrl Pts',(-28.1681625859469,-14.2192053591173,
113.247632978682)) ;
#172999=CARTESIAN_POINT('Ctrl Pts',(-28.2419664026165,-14.2192054253214,
113.223401855519)) ;
#173000=CARTESIAN_POINT('Ctrl Pts',(-28.3157702192861,-14.2192054915256,
113.199170732356)) ;
#173001=CARTESIAN_POINT('Ctrl Pts',(-28.3303445981694,-14.279022234562,
113.243561936774)) ;
#173002=CARTESIAN_POINT('Ctrl Pts',(-28.3449189770527,-14.3388389775984,
113.287953141191)) ;
#173003=CARTESIAN_POINT('Ctrl Pts',(-28.2711151603831,-14.3388389113943,
113.312184264354)) ;
#173004=CARTESIAN_POINT('Ctrl Pts',(-28.1973113437134,-14.3388388451902,
113.336415387517)) ;
#173005=CARTESIAN_POINT('Ctrl Pts',(-28.1827369648301,-14.2790221021537,
113.292024183099)) ;
#173006=CARTESIAN_POINT('Ctrl Pts',(-28.1145891487937,-14.4246999098251,
113.048988420366)) ;
#173007=CARTESIAN_POINT('Ctrl Pts',(-28.1054848872704,-14.3546239086375,
113.021258310826)) ;
#173008=CARTESIAN_POINT('Ctrl Pts',(-28.1792886994093,-14.3546239496232,
112.997027173864)) ;
#173009=CARTESIAN_POINT('Ctrl Pts',(-28.2530925115482,-14.3546239906089,
112.972796036901)) ;
#173010=CARTESIAN_POINT('Ctrl Pts',(-28.2621967730714,-14.4246999917965,
113.000526146441)) ;
#173011=CARTESIAN_POINT('Ctrl Pts',(-28.2713010345947,-14.4947759929842,
113.02825625598)) ;
#173012=CARTESIAN_POINT('Ctrl Pts',(-28.1974972224558,-14.4947759519985,
113.052487392943)) ;
#173013=CARTESIAN_POINT('Ctrl Pts',(-28.1236934103169,-14.4947759110128,
113.076718529906)) ;
#173014=CARTESIAN_POINT('Ctrl Pts',(-28.1145891487937,-14.4246999098251,
113.048988420366)) ;
#173015=CARTESIAN_POINT('Ctrl Pts',(-28.0369433110204,-14.4982101688668,
112.776913098185)) ;
#173016=CARTESIAN_POINT('Ctrl Pts',(-28.033982577611,-14.4228974545996,
112.767895183996)) ;
#173017=CARTESIAN_POINT('Ctrl Pts',(-28.107786387942,-14.4228974671485,
112.743664041527)) ;
#173018=CARTESIAN_POINT('Ctrl Pts',(-28.181590198273,-14.4228974796974,
112.719432899057)) ;
#173019=CARTESIAN_POINT('Ctrl Pts',(-28.1845509316824,-14.4982101939646,
112.728450813246)) ;
#173020=CARTESIAN_POINT('Ctrl Pts',(-28.1875116650917,-14.5735229082318,
112.737468727435)) ;
#173021=CARTESIAN_POINT('Ctrl Pts',(-28.1137078547607,-14.5735228956829,
112.761699869904)) ;
#173022=CARTESIAN_POINT('Ctrl Pts',(-28.0399040444297,-14.573522883134,
112.785931012374)) ;
#173023=CARTESIAN_POINT('Ctrl Pts',(-28.0369433110204,-14.4982101688668,
112.776913098185)) ;
#173024=CARTESIAN_POINT('Ctrl Pts',(-27.9566667707584,-14.4940193671701,
112.496956548577)) ;
#173025=CARTESIAN_POINT('Ctrl Pts',(-27.9600397432089,-14.4188869609571,
112.50723008045)) ;
#173026=CARTESIAN_POINT('Ctrl Pts',(-28.0338435544589,-14.4188869452096,
112.48299894078)) ;
#173027=CARTESIAN_POINT('Ctrl Pts',(-28.107647365709,-14.4188869294622,
112.45876780111)) ;
#173028=CARTESIAN_POINT('Ctrl Pts',(-28.1042743932586,-14.4940193356751,
112.448494269237)) ;
#173029=CARTESIAN_POINT('Ctrl Pts',(-28.1009014208082,-14.5691517418881,
112.438220737365)) ;
#173030=CARTESIAN_POINT('Ctrl Pts',(-28.0270976095581,-14.5691517576355,
112.462451877035)) ;
#173031=CARTESIAN_POINT('Ctrl Pts',(-27.953293798308,-14.569151773383,112.486683016705)) ;
#173032=CARTESIAN_POINT('Ctrl Pts',(-27.9566667707584,-14.4940193671701,
112.496956548577)) ;
#173033=CARTESIAN_POINT('Ctrl Pts',(-27.8798943064057,-14.4126640845972,
112.227622938821)) ;
#173034=CARTESIAN_POINT('Ctrl Pts',(-27.8893668566243,-14.3430991702555,
112.256474800339)) ;
#173035=CARTESIAN_POINT('Ctrl Pts',(-27.9631706714083,-14.3430991291711,
112.232243671433)) ;
#173036=CARTESIAN_POINT('Ctrl Pts',(-28.0369744861922,-14.3430990880866,
112.208012542526)) ;
#173037=CARTESIAN_POINT('Ctrl Pts',(-28.0275019359736,-14.4126640024283,
112.179160681008)) ;
#173038=CARTESIAN_POINT('Ctrl Pts',(-28.018029385755,-14.48222891677,112.150308819489)) ;
#173039=CARTESIAN_POINT('Ctrl Pts',(-27.9442255709711,-14.4822289578544,
112.174539948395)) ;
#173040=CARTESIAN_POINT('Ctrl Pts',(-27.8704217561871,-14.4822289989389,
112.198771077302)) ;
#173041=CARTESIAN_POINT('Ctrl Pts',(-27.8798943064057,-14.4126640845972,
112.227622938821)) ;
#173042=CARTESIAN_POINT('Ctrl Pts',(-27.8131986851945,-14.2606219622614,
111.989110261264)) ;
#173043=CARTESIAN_POINT('Ctrl Pts',(-27.828073796266,-14.2015682240357,
112.034417451361)) ;
#173044=CARTESIAN_POINT('Ctrl Pts',(-27.9018776164657,-14.2015681626728,
112.01018633895)) ;
#173045=CARTESIAN_POINT('Ctrl Pts',(-27.9756814366654,-14.2015681013099,
111.985955226539)) ;
#173046=CARTESIAN_POINT('Ctrl Pts',(-27.9608063255939,-14.2606218395355,
111.940648036442)) ;
#173047=CARTESIAN_POINT('Ctrl Pts',(-27.9459312145223,-14.3196755777612,
111.895340846344)) ;
#173048=CARTESIAN_POINT('Ctrl Pts',(-27.8721273943226,-14.3196756391241,
111.919571958755)) ;
#173049=CARTESIAN_POINT('Ctrl Pts',(-27.798323574123,-14.319675700487,111.943803071166)) ;
#173050=CARTESIAN_POINT('Ctrl Pts',(-27.8131986851945,-14.2606219622614,
111.989110261264)) ;
#173051=CARTESIAN_POINT('Ctrl Pts',(-27.7615962317299,-14.047641669402,
111.796421873509)) ;
#173052=CARTESIAN_POINT('Ctrl Pts',(-27.7808313920181,-14.003368790847,
111.855009069918)) ;
#173053=CARTESIAN_POINT('Ctrl Pts',(-27.8546352192211,-14.0033687165429,
111.830777978838)) ;
#173054=CARTESIAN_POINT('Ctrl Pts',(-27.928439046424,-14.0033686422388,
111.806546887757)) ;
#173055=CARTESIAN_POINT('Ctrl Pts',(-27.9092038861358,-14.0476415207938,
111.747959691349)) ;
#173056=CARTESIAN_POINT('Ctrl Pts',(-27.8899687258476,-14.0919143993488,
111.689372494941)) ;
#173057=CARTESIAN_POINT('Ctrl Pts',(-27.8161648986446,-14.0919144736529,
111.713603586021)) ;
#173058=CARTESIAN_POINT('Ctrl Pts',(-27.7423610714416,-14.0919145479569,
111.737834677101)) ;
#173059=CARTESIAN_POINT('Ctrl Pts',(-27.7615962317299,-14.047641669402,
111.796421873509)) ;
#173060=CARTESIAN_POINT('Ctrl Pts',(-27.7298973111856,-13.7890886844739,
111.664327213788)) ;
#173061=CARTESIAN_POINT('Ctrl Pts',(-27.7521102111039,-13.7628006589206,
111.731984124516)) ;
#173062=CARTESIAN_POINT('Ctrl Pts',(-27.8259140458139,-13.7628005801191,
111.707753056301)) ;
#173063=CARTESIAN_POINT('Ctrl Pts',(-27.8997178805239,-13.7628005013175,
111.683521988087)) ;
#173064=CARTESIAN_POINT('Ctrl Pts',(-27.8775049806057,-13.7890885268708,
111.615865077358)) ;
#173065=CARTESIAN_POINT('Ctrl Pts',(-27.8552920806875,-13.8153765524241,
111.54820816663)) ;
#173066=CARTESIAN_POINT('Ctrl Pts',(-27.7814882459774,-13.8153766312257,
111.572439234845)) ;
#173067=CARTESIAN_POINT('Ctrl Pts',(-27.7076844112674,-13.8153767100272,
111.59667030306)) ;
#173068=CARTESIAN_POINT('Ctrl Pts',(-27.7298973111856,-13.7890886844739,
111.664327213788)) ;
#173069=CARTESIAN_POINT('Ctrl Pts',(-27.7211529443622,-13.5048564724281,
111.602268903286)) ;
#173070=CARTESIAN_POINT('Ctrl Pts',(-27.7447429129393,-13.4983736613525,
111.674120142827)) ;
#173071=CARTESIAN_POINT('Ctrl Pts',(-27.818546754637,-13.4983735848724,
111.649889095895)) ;
#173072=CARTESIAN_POINT('Ctrl Pts',(-27.8923505963348,-13.4983735083923,
111.625658048964)) ;
#173073=CARTESIAN_POINT('Ctrl Pts',(-27.8687606277577,-13.5048563194679,
111.553806809424)) ;
#173074=CARTESIAN_POINT('Ctrl Pts',(-27.8451706591806,-13.5113391305435,
111.481955569883)) ;
#173075=CARTESIAN_POINT('Ctrl Pts',(-27.7713668174828,-13.5113392070236,
111.506186616814)) ;
#173076=CARTESIAN_POINT('Ctrl Pts',(-27.697562975785,-13.5113392835037,
111.530417663746)) ;
#173077=CARTESIAN_POINT('Ctrl Pts',(-27.7211529443622,-13.5048564724281,
111.602268903286)) ;
#173078=CARTESIAN_POINT('Ctrl Pts',(-27.7365275470258,-13.2147190164361,
111.613706256659)) ;
#173079=CARTESIAN_POINT('Ctrl Pts',(-27.7598120222788,-13.2284837281292,
111.684627012687)) ;
#173080=CARTESIAN_POINT('Ctrl Pts',(-27.8336158699542,-13.2284836599234,
111.660395983963)) ;
#173081=CARTESIAN_POINT('Ctrl Pts',(-27.9074197176295,-13.2284835917175,
111.636164955238)) ;
#173082=CARTESIAN_POINT('Ctrl Pts',(-27.8841352423765,-13.2147188800244,
111.56524419921)) ;
#173083=CARTESIAN_POINT('Ctrl Pts',(-27.8608507671235,-13.2009541683313,
111.494323443181)) ;
#173084=CARTESIAN_POINT('Ctrl Pts',(-27.7870469194481,-13.2009542365372,
111.518554471906)) ;
#173085=CARTESIAN_POINT('Ctrl Pts',(-27.7132430717728,-13.200954304743,
111.54278550063)) ;
#173086=CARTESIAN_POINT('Ctrl Pts',(-27.7365275470258,-13.2147190164361,
111.613706256659)) ;
#173087=CARTESIAN_POINT('Ctrl Pts',(-27.7758074412185,-12.9381997507725,
111.697848661622)) ;
#173088=CARTESIAN_POINT('Ctrl Pts',(-27.7971192532817,-12.9712919342548,
111.762761003699)) ;
#173089=CARTESIAN_POINT('Ctrl Pts',(-27.8709231053441,-12.9712918799021,
111.738529988336)) ;
#173090=CARTESIAN_POINT('Ctrl Pts',(-27.9447269574064,-12.9712918255494,
111.714298972973)) ;
#173091=CARTESIAN_POINT('Ctrl Pts',(-27.9234151453431,-12.9381996420671,
111.649386630897)) ;
#173092=CARTESIAN_POINT('Ctrl Pts',(-27.9021033332798,-12.9051074585849,
111.584474288821)) ;
#173093=CARTESIAN_POINT('Ctrl Pts',(-27.8282994812175,-12.9051075129375,
111.608705304183)) ;
#173094=CARTESIAN_POINT('Ctrl Pts',(-27.7544956291552,-12.9051075672902,
111.632936319546)) ;
#173095=CARTESIAN_POINT('Ctrl Pts',(-27.7758074412185,-12.9381997507725,
111.697848661622)) ;
#173096=CARTESIAN_POINT('Ctrl Pts',(-27.8372160580513,-12.695688487741,
111.849295864408)) ;
#173097=CARTESIAN_POINT('Ctrl Pts',(-27.8550092108468,-12.745763523541,
111.903490937894)) ;
#173098=CARTESIAN_POINT('Ctrl Pts',(-27.9288130649844,-12.7457634857973,
111.879259928853)) ;
#173099=CARTESIAN_POINT('Ctrl Pts',(-28.002616919122,-12.7457634480537,
111.855028919811)) ;
#173100=CARTESIAN_POINT('Ctrl Pts',(-27.9848237663266,-12.6956884122536,
111.800833846325)) ;
#173101=CARTESIAN_POINT('Ctrl Pts',(-27.9670306135311,-12.6456133764535,
111.746638772839)) ;
#173102=CARTESIAN_POINT('Ctrl Pts',(-27.8932267593934,-12.6456134141972,
111.77086978188)) ;
#173103=CARTESIAN_POINT('Ctrl Pts',(-27.8194229052558,-12.6456134519409,
111.795100790922)) ;
#173104=CARTESIAN_POINT('Ctrl Pts',(-27.8372160580513,-12.695688487741,
111.849295864408)) ;
#173105=CARTESIAN_POINT('Ctrl Pts',(-27.9160580941386,-12.5067830863174,
112.054188473819)) ;
#173106=CARTESIAN_POINT('Ctrl Pts',(-27.9291025894933,-12.5701233290617,
112.093919902817)) ;
#173107=CARTESIAN_POINT('Ctrl Pts',(-28.0029064447615,-12.5701233053132,
112.069688897219)) ;
#173108=CARTESIAN_POINT('Ctrl Pts',(-28.0767103000296,-12.5701232815646,
112.04545789162)) ;
#173109=CARTESIAN_POINT('Ctrl Pts',(-28.0636658046749,-12.5067830388203,
112.005726462623)) ;
#173110=CARTESIAN_POINT('Ctrl Pts',(-28.0506213093203,-12.443442796076,
111.965995033625)) ;
#173111=CARTESIAN_POINT('Ctrl Pts',(-27.9768174540521,-12.4434428198246,
111.990226039223)) ;
#173112=CARTESIAN_POINT('Ctrl Pts',(-27.903013598784,-12.4434428435731,
112.014457044821)) ;
#173113=CARTESIAN_POINT('Ctrl Pts',(-27.9160580941386,-12.5067830863174,
112.054188473819)) ;
#173114=CARTESIAN_POINT('Ctrl Pts',(-28.008667920428,-12.3815987000844,
112.300764968466)) ;
#173115=CARTESIAN_POINT('Ctrl Pts',(-28.0160005465217,-12.4537757553205,
112.323098965097)) ;
#173116=CARTESIAN_POINT('Ctrl Pts',(-28.0898044002542,-12.4537757450517,
112.298867954821)) ;
#173117=CARTESIAN_POINT('Ctrl Pts',(-28.1636082539867,-12.453775734783,
112.274636944545)) ;
#173118=CARTESIAN_POINT('Ctrl Pts',(-28.1562756278929,-12.3815986795469,
112.252302947915)) ;
#173119=CARTESIAN_POINT('Ctrl Pts',(-28.1489430017991,-12.3094216243108,
112.229968951285)) ;
#173120=CARTESIAN_POINT('Ctrl Pts',(-28.0751391480667,-12.3094216345796,
112.25419996156)) ;
#173121=CARTESIAN_POINT('Ctrl Pts',(-28.0013352943342,-12.3094216448483,
112.278430971836)) ;
#173122=CARTESIAN_POINT('Ctrl Pts',(-28.008667920428,-12.3815987000844,
112.300764968466)) ;
#173123=CARTESIAN_POINT('Ctrl Pts',(-28.1086587938519,-12.3308693682488,
112.569848181414)) ;
#173124=CARTESIAN_POINT('Ctrl Pts',(-28.1097549437029,-12.4066980840519,
112.573186877588)) ;
#173125=CARTESIAN_POINT('Ctrl Pts',(-28.1835587964667,-12.4066980849149,
112.548955864362)) ;
#173126=CARTESIAN_POINT('Ctrl Pts',(-28.2573626492306,-12.4066980857778,
112.524724851136)) ;
#173127=CARTESIAN_POINT('Ctrl Pts',(-28.2562664993797,-12.3308693699746,
112.521386154962)) ;
#173128=CARTESIAN_POINT('Ctrl Pts',(-28.2551703495287,-12.2550406541715,
112.518047458789)) ;
#173129=CARTESIAN_POINT('Ctrl Pts',(-28.1813664967649,-12.2550406533085,
112.542278472015)) ;
#173130=CARTESIAN_POINT('Ctrl Pts',(-28.107562644001,-12.2550406524456,
112.566509485241)) ;
#173131=CARTESIAN_POINT('Ctrl Pts',(-28.1086587938519,-12.3308693682488,
112.569848181414)) ;
#173132=CARTESIAN_POINT('Ctrl Pts',(-28.2098713901146,-12.3583046491224,
112.842561582163)) ;
#173133=CARTESIAN_POINT('Ctrl Pts',(-28.2046378959205,-12.4323324318187,
112.826621203442)) ;
#173134=CARTESIAN_POINT('Ctrl Pts',(-28.2784417425771,-12.4323324320423,
112.802390171614)) ;
#173135=CARTESIAN_POINT('Ctrl Pts',(-28.3522455892337,-12.4323324322659,
112.778159139786)) ;
#173136=CARTESIAN_POINT('Ctrl Pts',(-28.3574790834278,-12.3583046495696,
112.794099518507)) ;
#173137=CARTESIAN_POINT('Ctrl Pts',(-28.362712577622,-12.2842768668734,
112.810039897228)) ;
#173138=CARTESIAN_POINT('Ctrl Pts',(-28.2889087309654,-12.2842768666498,
112.834270929056)) ;
#173139=CARTESIAN_POINT('Ctrl Pts',(-28.2151048843088,-12.2842768664262,
112.858501960883)) ;
#173140=CARTESIAN_POINT('Ctrl Pts',(-28.2098713901146,-12.3583046491224,
112.842561582163)) ;
#173141=CARTESIAN_POINT('Ctrl Pts',(-28.3051249657282,-12.4612718878677,
113.097301430193)) ;
#173142=CARTESIAN_POINT('Ctrl Pts',(-28.2939651434437,-12.5282228863583,
113.063310412817)) ;
#173143=CARTESIAN_POINT('Ctrl Pts',(-28.3677689949065,-12.5282229072686,
113.039079395629)) ;
#173144=CARTESIAN_POINT('Ctrl Pts',(-28.4415728463693,-12.5282229281789,
113.01484837844)) ;
#173145=CARTESIAN_POINT('Ctrl Pts',(-28.4527326686539,-12.4612719296883,
113.048839395816)) ;
#173146=CARTESIAN_POINT('Ctrl Pts',(-28.4638924909383,-12.3943209311977,
113.082830413191)) ;
#173147=CARTESIAN_POINT('Ctrl Pts',(-28.3900886394755,-12.3943209102874,
113.10706143038)) ;
#173148=CARTESIAN_POINT('Ctrl Pts',(-28.3162847880127,-12.3943208893771,
113.131292447568)) ;
#173149=CARTESIAN_POINT('Ctrl Pts',(-28.3051249657282,-12.4612718878677,
113.097301430193)) ;
#173150=CARTESIAN_POINT('Ctrl Pts',(-28.3893018558163,-12.6338543702633,
113.318075545151)) ;
#173151=CARTESIAN_POINT('Ctrl Pts',(-28.3729836452501,-12.6888516916321,
113.268372907815)) ;
#173152=CARTESIAN_POINT('Ctrl Pts',(-28.4467874809231,-12.6888516559685,
113.244141842533)) ;
#173153=CARTESIAN_POINT('Ctrl Pts',(-28.520591316596,-12.6888516203049,
113.219910777251)) ;
#173154=CARTESIAN_POINT('Ctrl Pts',(-28.5369095271621,-12.6338542989361,
113.269613414587)) ;
#173155=CARTESIAN_POINT('Ctrl Pts',(-28.5532277377282,-12.5788569775673,
113.319316051923)) ;
#173156=CARTESIAN_POINT('Ctrl Pts',(-28.4794239020553,-12.5788570132309,
113.343547117205)) ;
#173157=CARTESIAN_POINT('Ctrl Pts',(-28.4056200663824,-12.5788570488945,
113.367778182487)) ;
#173158=CARTESIAN_POINT('Ctrl Pts',(-28.3893018558163,-12.6338543702633,
113.318075545151)) ;
#173159=CARTESIAN_POINT('Ctrl Pts',(-28.4559528062998,-12.8606317098419,
113.485811899978)) ;
#173160=CARTESIAN_POINT('Ctrl Pts',(-28.4356875294123,-12.8998873118664,
113.424087138298)) ;
#173161=CARTESIAN_POINT('Ctrl Pts',(-28.5094913849229,-12.8998874003437,
113.399856133438)) ;
#173162=CARTESIAN_POINT('Ctrl Pts',(-28.5832952404334,-12.8998874888211,
113.375625128578)) ;
#173163=CARTESIAN_POINT('Ctrl Pts',(-28.6035605173208,-12.8606318867965,
113.437349890258)) ;
#173164=CARTESIAN_POINT('Ctrl Pts',(-28.6238257942082,-12.821376284772,
113.499074651938)) ;
#173165=CARTESIAN_POINT('Ctrl Pts',(-28.5500219386977,-12.8213761962946,
113.523305656798)) ;
#173166=CARTESIAN_POINT('Ctrl Pts',(-28.4762180831872,-12.8213761078173,
113.547536661658)) ;
#173167=CARTESIAN_POINT('Ctrl Pts',(-28.4559528062998,-12.8606317098419,
113.485811899978)) ;
#173168=CARTESIAN_POINT('Ctrl Pts',(-28.5023209234415,-13.129518595729,
113.591432315876)) ;
#173169=CARTESIAN_POINT('Ctrl Pts',(-28.4795225725677,-13.1500300138352,
113.521992214164)) ;
#173170=CARTESIAN_POINT('Ctrl Pts',(-28.5533264028797,-13.1500298440004,
113.497761132554)) ;
#173171=CARTESIAN_POINT('Ctrl Pts',(-28.6271302331918,-13.1500296741656,
113.473530050943)) ;
#173172=CARTESIAN_POINT('Ctrl Pts',(-28.6499285840656,-13.1295182560594,
113.542970152655)) ;
#173173=CARTESIAN_POINT('Ctrl Pts',(-28.6727269349394,-13.1090068379532,
113.612410254366)) ;
#173174=CARTESIAN_POINT('Ctrl Pts',(-28.5989231046273,-13.109007007788,
113.636641335977)) ;
#173175=CARTESIAN_POINT('Ctrl Pts',(-28.5251192743152,-13.1090071776228,
113.660872417588)) ;
#173176=CARTESIAN_POINT('Ctrl Pts',(-28.5023209234415,-13.129518595729,
113.591432315876)) ;
#173177=CARTESIAN_POINT('Ctrl Pts',(-28.5173598286699,-13.3215354698077,
113.613640637198)) ;
#173178=CARTESIAN_POINT('Ctrl Pts',(-28.4939782962573,-13.3286998701254,
113.542424265285)) ;
#173179=CARTESIAN_POINT('Ctrl Pts',(-28.5677821471769,-13.3287000326328,
113.518193246442)) ;
#173180=CARTESIAN_POINT('Ctrl Pts',(-28.6415859980966,-13.3287001951402,
113.493962227599)) ;
#173181=CARTESIAN_POINT('Ctrl Pts',(-28.6649675305092,-13.3215357948224,
113.565178599512)) ;
#173182=CARTESIAN_POINT('Ctrl Pts',(-28.6883490629218,-13.3143713945047,
113.636394971425)) ;
#173183=CARTESIAN_POINT('Ctrl Pts',(-28.6145452120022,-13.3143712319973,
113.660625990268)) ;
#173184=CARTESIAN_POINT('Ctrl Pts',(-28.5407413610825,-13.31437106949,113.684857009111)) ;
#173185=CARTESIAN_POINT('Ctrl Pts',(-28.5173598286699,-13.3215354698077,
113.613640637198)) ;
#173186=CARTESIAN_POINT('Ctrl Pts',(-28.520878677028,-13.4175644257172,
113.612558746724)) ;
#173187=CARTESIAN_POINT('Ctrl Pts',(-28.4974839627901,-13.4180062659798,
113.541302223353)) ;
#173188=CARTESIAN_POINT('Ctrl Pts',(-28.5712878061994,-13.4180063413679,
113.517071181635)) ;
#173189=CARTESIAN_POINT('Ctrl Pts',(-28.6450916496088,-13.4180064167561,
113.492840139917)) ;
#173190=CARTESIAN_POINT('Ctrl Pts',(-28.6684863638467,-13.4175645764935,
113.564096663288)) ;
#173191=CARTESIAN_POINT('Ctrl Pts',(-28.6918810780846,-13.4171227362309,
113.635353186659)) ;
#173192=CARTESIAN_POINT('Ctrl Pts',(-28.6180772346753,-13.4171226608428,
113.659584228377)) ;
#173193=CARTESIAN_POINT('Ctrl Pts',(-28.5442733912659,-13.4171225854547,
113.683815270095)) ;
#173194=CARTESIAN_POINT('Ctrl Pts',(-28.520878677028,-13.4175644257172,
113.612558746724)) ;
#173195=CARTESIAN_POINT('',(-17.4415366461909,-12.9727494438644,115.08882743648)) ;
#173196=CARTESIAN_POINT('',(-17.7467422306782,-14.4181080989129,116.018434402089)) ;
#173197=CARTESIAN_POINT('Ctrl Pts',(-17.4415366461909,-12.9727494438642,
115.08882743648)) ;
#173198=CARTESIAN_POINT('Ctrl Pts',(-17.4416493049237,-12.9729113566649,
115.089170576803)) ;
#173199=CARTESIAN_POINT('Ctrl Pts',(-17.4417445866774,-12.9731380019779,
115.089460789651)) ;
#173200=CARTESIAN_POINT('Ctrl Pts',(-17.4419266128785,-12.9737505696882,
115.09001521209)) ;
#173201=CARTESIAN_POINT('Ctrl Pts',(-17.4420039390573,-12.9741371839328,
115.090250735154)) ;
#173202=CARTESIAN_POINT('Ctrl Pts',(-17.4422222411396,-12.9755496760444,
115.090915648074)) ;
#173203=CARTESIAN_POINT('Ctrl Pts',(-17.4423092903792,-12.9768233272532,
115.091180786012)) ;
#173204=CARTESIAN_POINT('Ctrl Pts',(-17.4424780367696,-12.9812525255357,
115.09169476029)) ;
#173205=CARTESIAN_POINT('Ctrl Pts',(-17.4424107635199,-12.9855810222862,
115.091489856826)) ;
#173206=CARTESIAN_POINT('Ctrl Pts',(-17.4417642698842,-13.0025035797018,
115.089520741523)) ;
#173207=CARTESIAN_POINT('Ctrl Pts',(-17.4406256616663,-13.0192459488914,
115.086052724601)) ;
#173208=CARTESIAN_POINT('Ctrl Pts',(-17.4357398541899,-13.0885454351124,
115.07117134335)) ;
#173209=CARTESIAN_POINT('Ctrl Pts',(-17.4306638807193,-13.1573238043937,
115.055710747168)) ;
#173210=CARTESIAN_POINT('Ctrl Pts',(-17.4232190844825,-13.3846429728215,
115.033035099044)) ;
#173211=CARTESIAN_POINT('Ctrl Pts',(-17.4270784747103,-13.5028371896587,
115.044790178968)) ;
#173212=CARTESIAN_POINT('Ctrl Pts',(-17.4422801026987,-13.7248060299084,
115.091091885046)) ;
#173213=CARTESIAN_POINT('Ctrl Pts',(-17.4575003868623,-13.842674137476,
115.137450414823)) ;
#173214=CARTESIAN_POINT('Ctrl Pts',(-17.5022901009571,-14.0637456275397,
115.273872657162)) ;
#173215=CARTESIAN_POINT('Ctrl Pts',(-17.5324113344876,-14.1629071646496,
115.365617074455)) ;
#173216=CARTESIAN_POINT('Ctrl Pts',(-17.5943601419139,-14.2984535233359,
115.554303146472)) ;
#173217=CARTESIAN_POINT('Ctrl Pts',(-17.6236281361654,-14.3434390384379,
115.643448734658)) ;
#173218=CARTESIAN_POINT('Ctrl Pts',(-17.6844950745686,-14.4029494275453,
115.82883960819)) ;
#173219=CARTESIAN_POINT('Ctrl Pts',(-17.7154604463368,-14.4178650105577,
115.923155134283)) ;
#173220=CARTESIAN_POINT('Ctrl Pts',(-17.7467422306786,-14.4181080983633,
116.018434402091)) ;
#173221=CARTESIAN_POINT('',(-17.7467422306782,-14.5678329207423,116.018434402089)) ;
#173222=CARTESIAN_POINT('Ctrl Pts',(-17.7467422306795,-14.5678329226988,
116.018434402093)) ;
#173223=CARTESIAN_POINT('Ctrl Pts',(-17.7837999493661,-14.5675899683414,
116.131306233972)) ;
#173224=CARTESIAN_POINT('Ctrl Pts',(-17.820553393073,-14.5486809816127,
116.243251293388)) ;
#173225=CARTESIAN_POINT('Ctrl Pts',(-17.8912458202562,-14.474265964022,
116.458569020407)) ;
#173226=CARTESIAN_POINT('Ctrl Pts',(-17.9245709673636,-14.4189847550274,
116.560072041471)) ;
#173227=CARTESIAN_POINT('Ctrl Pts',(-17.9911651174408,-14.261499390111,
116.76290707768)) ;
#173228=CARTESIAN_POINT('Ctrl Pts',(-18.0222422523085,-14.1522077768049,
116.857563016237)) ;
#173229=CARTESIAN_POINT('Ctrl Pts',(-18.0682059255952,-13.906320914405,
116.997560948857)) ;
#173230=CARTESIAN_POINT('Ctrl Pts',(-18.0833283498345,-13.7731365150372,
117.04362141307)) ;
#173231=CARTESIAN_POINT('Ctrl Pts',(-18.0968448267067,-13.4847220177906,
117.084790420747)) ;
#173232=CARTESIAN_POINT('Ctrl Pts',(-18.0920710740004,-13.3621596026309,
117.070250340363)) ;
#173233=CARTESIAN_POINT('Ctrl Pts',(-18.0838242795246,-13.2522859045863,
117.045131935005)) ;
#173234=CARTESIAN_POINT('Ctrl Pts',(-18.0807506711114,-13.2255158773084,
117.035770219586)) ;
#173235=CARTESIAN_POINT('Ctrl Pts',(-18.0778088901523,-13.2094171488094,
117.026810029439)) ;
#173236=CARTESIAN_POINT('Ctrl Pts',(-18.0771326193299,-13.20622369284,117.024750217551)) ;
#173237=CARTESIAN_POINT('Ctrl Pts',(-18.0762733506409,-13.2039870459225,
117.022133023767)) ;
#173238=CARTESIAN_POINT('Ctrl Pts',(-18.0760666869366,-13.2035491479374,
117.021503559547)) ;
#173239=CARTESIAN_POINT('Ctrl Pts',(-18.075717002172,-13.2031450748714,
117.020438476176)) ;
#173240=CARTESIAN_POINT('Ctrl Pts',(-18.0755794005162,-13.2030585898593,
117.020019363734)) ;
#173241=CARTESIAN_POINT('Ctrl Pts',(-18.0753222220269,-13.2030933380485,
117.019236039552)) ;
#173242=CARTESIAN_POINT('Ctrl Pts',(-18.0752104635191,-13.2031822301836,
117.018895641169)) ;
#173243=CARTESIAN_POINT('Ctrl Pts',(-18.0749846821218,-13.2035184810667,
117.018207947462)) ;
#173244=CARTESIAN_POINT('Ctrl Pts',(-18.0748787895421,-13.2037736716702,
117.01788541575)) ;
#173245=CARTESIAN_POINT('Ctrl Pts',(-18.0746299615403,-13.2045590817022,
117.017127525805)) ;
#173246=CARTESIAN_POINT('Ctrl Pts',(-18.0745028132178,-13.2051773697714,
117.01674025253)) ;
#173247=CARTESIAN_POINT('Ctrl Pts',(-18.0741650784759,-13.2071977532132,
117.015711567)) ;
#173248=CARTESIAN_POINT('Ctrl Pts',(-18.0739890260903,-13.2089958124963,
117.015175339839)) ;
#173249=CARTESIAN_POINT('Ctrl Pts',(-18.073432868927,-13.2164449755183,
117.013481374855)) ;
#173250=CARTESIAN_POINT('Ctrl Pts',(-18.0732286091857,-13.2246311944403,
117.012859232641)) ;
#173251=CARTESIAN_POINT('Ctrl Pts',(-18.0723882663157,-13.2885837862774,
117.010299683847)) ;
#173252=CARTESIAN_POINT('Ctrl Pts',(-18.0747562393785,-13.4061630903225,
117.017512147145)) ;
#173253=CARTESIAN_POINT('Ctrl Pts',(-18.0579338010805,-13.6895955424722,
116.96627371438)) ;
#173254=CARTESIAN_POINT('Ctrl Pts',(-18.0424550542148,-13.8180971458136,
116.919127949494)) ;
#173255=CARTESIAN_POINT('Ctrl Pts',(-17.9964872591334,-14.0512183347413,
116.779117462552)) ;
#173256=CARTESIAN_POINT('Ctrl Pts',(-17.9667139535318,-14.1518807047038,
116.688432777588)) ;
#173257=CARTESIAN_POINT('Ctrl Pts',(-17.9047052645825,-14.2916003512213,
116.499564316113)) ;
#173258=CARTESIAN_POINT('Ctrl Pts',(-17.8747540318166,-14.3392564455703,
116.408337693765)) ;
#173259=CARTESIAN_POINT('Ctrl Pts',(-17.8119658998287,-14.4025181298819,
116.217095174557)) ;
#173260=CARTESIAN_POINT('Ctrl Pts',(-17.7794837034873,-14.4183625292707,
116.118159645449)) ;
#173261=CARTESIAN_POINT('Ctrl Pts',(-17.7467422306786,-14.4181080983633,
116.018434402091)) ;
#173262=CARTESIAN_POINT('Ctrl Pts',(-17.7467422940615,-14.5678329187858,
116.018434377539)) ;
#173263=CARTESIAN_POINT('Ctrl Pts',(-17.7332949369721,-14.567921082103,
115.977475887229)) ;
#173264=CARTESIAN_POINT('Ctrl Pts',(-17.7198338964835,-14.5655508478998,
115.936475957776)) ;
#173265=CARTESIAN_POINT('Ctrl Pts',(-17.7064533679514,-14.5607116311535,
115.895721026807)) ;
#173266=CARTESIAN_POINT('Ctrl Pts',(-17.7008963178764,-14.5587018622779,
115.878795148906)) ;
#173267=CARTESIAN_POINT('Ctrl Pts',(-17.6953526550133,-14.556266107077,
115.861910046291)) ;
#173268=CARTESIAN_POINT('Ctrl Pts',(-17.6898291283943,-14.5534035696439,
115.845086275428)) ;
#173269=CARTESIAN_POINT('Ctrl Pts',(-17.6639931539809,-14.540014217337,
115.766394065983)) ;
#173270=CARTESIAN_POINT('Ctrl Pts',(-17.6386072513392,-14.5172883204702,
115.689072933564)) ;
#173271=CARTESIAN_POINT('Ctrl Pts',(-17.6143647373925,-14.4859963413085,
115.615233985268)) ;
#173272=CARTESIAN_POINT('Ctrl Pts',(-17.6088324961802,-14.4788553831919,
115.598383634115)) ;
#173273=CARTESIAN_POINT('Ctrl Pts',(-17.603359769088,-14.4712685294603,
115.58171455876)) ;
#173274=CARTESIAN_POINT('Ctrl Pts',(-17.5979547370195,-14.463245285136,
115.565251703178)) ;
#173275=CARTESIAN_POINT('Ctrl Pts',(-17.5737703925387,-14.4273459783174,
115.491590092019)) ;
#173276=CARTESIAN_POINT('Ctrl Pts',(-17.5509423402976,-14.382706735496,
115.422059045954)) ;
#173277=CARTESIAN_POINT('Ctrl Pts',(-17.5299755060472,-14.3303836683843,
115.358197794957)) ;
#173278=CARTESIAN_POINT('Ctrl Pts',(-17.5257169917526,-14.3197564784817,
115.34522711722)) ;
#173279=CARTESIAN_POINT('Ctrl Pts',(-17.5215352397186,-14.3088124559326,
115.33249024464)) ;
#173280=CARTESIAN_POINT('Ctrl Pts',(-17.5174344587667,-14.2975606758145,
115.319999927519)) ;
#173281=CARTESIAN_POINT('Ctrl Pts',(-17.4986027738424,-14.2458900353905,
115.262641653721)) ;
#173282=CARTESIAN_POINT('Ctrl Pts',(-17.4814806589956,-14.1877300152538,
115.210488620322)) ;
#173283=CARTESIAN_POINT('Ctrl Pts',(-17.4664920220727,-14.1246319652759,
115.164836776727)) ;
#173284=CARTESIAN_POINT('Ctrl Pts',(-17.4621338516685,-14.1062852633449,
115.151562820284)) ;
#173285=CARTESIAN_POINT('Ctrl Pts',(-17.4579560289739,-14.0875212502652,
115.138838227179)) ;
#173286=CARTESIAN_POINT('Ctrl Pts',(-17.4539689063096,-14.0683784694332,
115.126694094864)) ;
#173287=CARTESIAN_POINT('Ctrl Pts',(-17.4412184801284,-14.0071617388599,
115.08785835399)) ;
#173288=CARTESIAN_POINT('Ctrl Pts',(-17.4304212800358,-13.9420796939717,
115.054965888367)) ;
#173289=CARTESIAN_POINT('Ctrl Pts',(-17.421751954825,-13.8743660366251,
115.02856349937)) ;
#173290=CARTESIAN_POINT('Ctrl Pts',(-17.4183697530646,-13.8479486113346,
115.018263019878)) ;
#173291=CARTESIAN_POINT('Ctrl Pts',(-17.4153115283899,-13.8211309228484,
115.008949959065)) ;
#173292=CARTESIAN_POINT('Ctrl Pts',(-17.4125881147126,-13.7939873904681,
115.000654880426)) ;
#173293=CARTESIAN_POINT('Ctrl Pts',(-17.4101304422485,-13.7694924293578,
114.993169206644)) ;
#173294=CARTESIAN_POINT('Ctrl Pts',(-17.4079126625351,-13.7443945944633,
114.986414068217)) ;
#173295=CARTESIAN_POINT('Ctrl Pts',(-17.4059708022617,-13.7189305603966,
114.980499460854)) ;
#173296=CARTESIAN_POINT('Ctrl Pts',(-17.4040278340081,-13.6934519971441,
114.974581478754)) ;
#173297=CARTESIAN_POINT('Ctrl Pts',(-17.4023611764262,-13.6676074929265,
114.969505197951)) ;
#173298=CARTESIAN_POINT('Ctrl Pts',(-17.4009916769738,-13.6416518046287,
114.965334020056)) ;
#173299=CARTESIAN_POINT('Ctrl Pts',(-17.3996215525311,-13.6156842710883,
114.961160938584)) ;
#173300=CARTESIAN_POINT('Ctrl Pts',(-17.3985488961501,-13.5896061785694,
114.957893876415)) ;
#173301=CARTESIAN_POINT('Ctrl Pts',(-17.3977784667299,-13.5636797249837,
114.955547240168)) ;
#173302=CARTESIAN_POINT('Ctrl Pts',(-17.397095896066,-13.5407098900154,
114.953468211227)) ;
#173303=CARTESIAN_POINT('Ctrl Pts',(-17.3966503194363,-13.5178594986711,
114.952110927568)) ;
#173304=CARTESIAN_POINT('Ctrl Pts',(-17.3964343054011,-13.4953086850252,
114.95145298367)) ;
#173305=CARTESIAN_POINT('Ctrl Pts',(-17.3962500641307,-13.4760747933397,
114.950891814488)) ;
#173306=CARTESIAN_POINT('Ctrl Pts',(-17.3962259892308,-13.4562541583979,
114.950817703317)) ;
#173307=CARTESIAN_POINT('Ctrl Pts',(-17.3963872225811,-13.4361251533928,
114.951308483242)) ;
#173308=CARTESIAN_POINT('Ctrl Pts',(-17.3965481904285,-13.4160292948047,
114.951798454999)) ;
#173309=CARTESIAN_POINT('Ctrl Pts',(-17.396893950264,-13.3956265064346,
114.952851695746)) ;
#173310=CARTESIAN_POINT('Ctrl Pts',(-17.39743331335,-13.3751969407048,114.954494975785)) ;
#173311=CARTESIAN_POINT('Ctrl Pts',(-17.3979644398562,-13.3550793535936,
114.956113161397)) ;
#173312=CARTESIAN_POINT('Ctrl Pts',(-17.398683284971,-13.3349362383174,
114.958303394013)) ;
#173313=CARTESIAN_POINT('Ctrl Pts',(-17.399582038043,-13.3150316956181,
114.961041335508)) ;
#173314=CARTESIAN_POINT('Ctrl Pts',(-17.4005016975791,-13.2946641407519,
114.963842965993)) ;
#173315=CARTESIAN_POINT('Ctrl Pts',(-17.4016097540901,-13.274546874533,
114.967218079118)) ;
#173316=CARTESIAN_POINT('Ctrl Pts',(-17.402880521455,-13.2549521381172,
114.971088309475)) ;
#173317=CARTESIAN_POINT('Ctrl Pts',(-17.40415128882,-13.2353574017014,114.974958539832)) ;
#173318=CARTESIAN_POINT('Ctrl Pts',(-17.4055846503689,-13.2162855561395,
114.979323458039)) ;
#173319=CARTESIAN_POINT('Ctrl Pts',(-17.4071386136518,-13.1979917937502,
114.984056579468)) ;
#173320=CARTESIAN_POINT('Ctrl Pts',(-17.4082540624649,-13.1848603666647,
114.987454056576)) ;
#173321=CARTESIAN_POINT('Ctrl Pts',(-17.4094975291958,-13.1713626479554,
114.991241248254)) ;
#173322=CARTESIAN_POINT('Ctrl Pts',(-17.4108532972022,-13.1578519278584,
114.995370749509)) ;
#173323=CARTESIAN_POINT('Ctrl Pts',(-17.4122190841212,-13.1442413656632,
114.99953076713)) ;
#173324=CARTESIAN_POINT('Ctrl Pts',(-17.413698885255,-13.1306181206681,
115.004038216471)) ;
#173325=CARTESIAN_POINT('Ctrl Pts',(-17.4152606318803,-13.1173287413436,
115.0087950996)) ;
#173326=CARTESIAN_POINT('Ctrl Pts',(-17.4168223785057,-13.1040393620192,
115.01355198273)) ;
#173327=CARTESIAN_POINT('Ctrl Pts',(-17.4184659685917,-13.0910842149795,
115.018557874953)) ;
#173328=CARTESIAN_POINT('Ctrl Pts',(-17.4201438439888,-13.078788559479,
115.023668412688)) ;
#173329=CARTESIAN_POINT('Ctrl Pts',(-17.4213745941723,-13.0697694867344,
115.027417079166)) ;
#173330=CARTESIAN_POINT('Ctrl Pts',(-17.4227127612408,-13.0604578336814,
115.03149283626)) ;
#173331=CARTESIAN_POINT('Ctrl Pts',(-17.4241123561879,-13.0513039505984,
115.035755849477)) ;
#173332=CARTESIAN_POINT('Ctrl Pts',(-17.4255204089638,-13.0420947500989,
115.040044624317)) ;
#173333=CARTESIAN_POINT('Ctrl Pts',(-17.4269906419727,-13.0330456384297,
115.044522707934)) ;
#173334=CARTESIAN_POINT('Ctrl Pts',(-17.4284614092985,-13.0245905007224,
115.049002382908)) ;
#173335=CARTESIAN_POINT('Ctrl Pts',(-17.4286223070298,-13.0236655328831,
115.049492446515)) ;
#173336=CARTESIAN_POINT('Ctrl Pts',(-17.4287831970196,-13.0227476464621,
115.049982488066)) ;
#173337=CARTESIAN_POINT('Ctrl Pts',(-17.4289439883956,-13.0218373893616,
115.050472232653)) ;
#173338=CARTESIAN_POINT('Ctrl Pts',(-17.4300528502253,-13.0155600044732,
115.053849646872)) ;
#173339=CARTESIAN_POINT('Ctrl Pts',(-17.4312557380411,-13.0090948676773,
115.057513461095)) ;
#173340=CARTESIAN_POINT('Ctrl Pts',(-17.4324741489107,-13.0030224151988,
115.061224556432)) ;
#173341=CARTESIAN_POINT('Ctrl Pts',(-17.4330581911971,-13.0001115998757,
115.063003460954)) ;
#173342=CARTESIAN_POINT('Ctrl Pts',(-17.4336455972628,-12.9972905938871,
115.064792574661)) ;
#173343=CARTESIAN_POINT('Ctrl Pts',(-17.4342266207035,-12.9946208870877,
115.066562278314)) ;
#173344=CARTESIAN_POINT('Ctrl Pts',(-17.4352177538382,-12.9900667939414,
115.069581109923)) ;
#173345=CARTESIAN_POINT('Ctrl Pts',(-17.4362883606204,-12.9855090222264,
115.07284200544)) ;
#173346=CARTESIAN_POINT('Ctrl Pts',(-17.4373159276886,-12.9817420257543,
115.075971808932)) ;
#173347=CARTESIAN_POINT('Ctrl Pts',(-17.4379198548086,-12.9795280667821,
115.077811273497)) ;
#173348=CARTESIAN_POINT('Ctrl Pts',(-17.4385432102028,-12.977460262646,
115.07970991335)) ;
#173349=CARTESIAN_POINT('Ctrl Pts',(-17.4391363740831,-12.9758473023832,
115.081516594823)) ;
#173350=CARTESIAN_POINT('Ctrl Pts',(-17.4400557041536,-12.9733474150479,
115.084316725884)) ;
#173351=CARTESIAN_POINT('Ctrl Pts',(-17.4409267509016,-12.9718729041419,
115.086969793835)) ;
#173352=CARTESIAN_POINT('Ctrl Pts',(-17.4415366461909,-12.9727494438644,
115.08882743648)) ;
#173353=CARTESIAN_POINT('',(-6.34456572554058,-13.1500241806476,118.666226584225)) ;
#173354=CARTESIAN_POINT('Ctrl Pts',(-6.34456572554058,-13.1500241806476,
118.666226584225)) ;
#173355=CARTESIAN_POINT('Ctrl Pts',(-6.34529362630125,-13.1438552129684,
118.667661018198)) ;
#173356=CARTESIAN_POINT('Ctrl Pts',(-6.35716264371204,-13.045472096163,
118.691303794064)) ;
#173357=CARTESIAN_POINT('Ctrl Pts',(-6.38921314251039,-12.8597742993635,
118.764325222303)) ;
#173358=CARTESIAN_POINT('Ctrl Pts',(-6.45615197626408,-12.6327839415056,
118.932852707777)) ;
#173359=CARTESIAN_POINT('Ctrl Pts',(-6.53996330725217,-12.4610780963096,
119.152681494851)) ;
#173360=CARTESIAN_POINT('Ctrl Pts',(-6.63588982776904,-12.3578311300529,
119.409231710552)) ;
#173361=CARTESIAN_POINT('Ctrl Pts',(-6.736259431342,-12.3309709098726,119.679683383479)) ;
#173362=CARTESIAN_POINT('Ctrl Pts',(-6.83652100223137,-12.3817310335918,
119.949488204916)) ;
#173363=CARTESIAN_POINT('Ctrl Pts',(-6.92897537929249,-12.5067458714326,
120.195657155914)) ;
#173364=CARTESIAN_POINT('Ctrl Pts',(-7.00828982195215,-12.6971218835384,
120.401748881771)) ;
#173365=CARTESIAN_POINT('Ctrl Pts',(-7.06933695913004,-12.9391053860727,
120.552223222998)) ;
#173366=CARTESIAN_POINT('Ctrl Pts',(-7.10853205803656,-13.2152764852227,
120.63614997259)) ;
#173367=CARTESIAN_POINT('Ctrl Pts',(-7.12391162690117,-13.505784356226,
120.64756404441)) ;
#173368=CARTESIAN_POINT('Ctrl Pts',(-7.11491785946518,-13.7916119971123,
120.584527953854)) ;
#173369=CARTESIAN_POINT('Ctrl Pts',(-7.08327931847018,-14.0480477215918,
120.452871020505)) ;
#173370=CARTESIAN_POINT('Ctrl Pts',(-7.03177476396055,-14.2608003622883,
120.260526319525)) ;
#173371=CARTESIAN_POINT('Ctrl Pts',(-6.96488777055259,-14.4130997833176,
120.021344897526)) ;
#173372=CARTESIAN_POINT('Ctrl Pts',(-6.88794749547868,-14.494276858583,
119.751438472986)) ;
#173373=CARTESIAN_POINT('Ctrl Pts',(-6.80764424999997,-14.4979516536895,
119.471388070987)) ;
#173374=CARTESIAN_POINT('Ctrl Pts',(-6.73039780792071,-14.4245500702158,
119.200701305624)) ;
#173375=CARTESIAN_POINT('Ctrl Pts',(-6.66228119436863,-14.27912481409,118.957786696)) ;
#173376=CARTESIAN_POINT('Ctrl Pts',(-6.60891474419106,-14.0717728276009,
118.75974735927)) ;
#173377=CARTESIAN_POINT('Ctrl Pts',(-6.57501586876472,-13.8168218187551,
118.62092447149)) ;
#173378=CARTESIAN_POINT('Ctrl Pts',(-6.56385556381707,-13.535324035321,
118.551622243501)) ;
#173379=CARTESIAN_POINT('Ctrl Pts',(-6.57670200274292,-13.2440746292406,
118.55526577413)) ;
#173380=CARTESIAN_POINT('Ctrl Pts',(-6.61375984173444,-12.9648031401168,
118.632582291307)) ;
#173381=CARTESIAN_POINT('Ctrl Pts',(-6.67258342631208,-12.7194345507308,
118.776404079392)) ;
#173382=CARTESIAN_POINT('Ctrl Pts',(-6.75039015970557,-12.5228537207888,
118.97784552327)) ;
#173383=CARTESIAN_POINT('Ctrl Pts',(-6.84171874623714,-12.3910219564108,
119.220611387595)) ;
#173384=CARTESIAN_POINT('Ctrl Pts',(-6.94152390518599,-12.3324946198483,
119.489024176868)) ;
#173385=CARTESIAN_POINT('Ctrl Pts',(-7.04230587420137,-12.3517941049946,
119.760653819778)) ;
#173386=CARTESIAN_POINT('Ctrl Pts',(-7.13886766534031,-12.4476532719571,
120.019204540318)) ;
#173387=CARTESIAN_POINT('Ctrl Pts',(-7.22405843886179,-12.6128436094032,
120.24325293471)) ;
#173388=CARTESIAN_POINT('Ctrl Pts',(-7.29301191518833,-12.8354722898284,
120.417835047233)) ;
#173389=CARTESIAN_POINT('Ctrl Pts',(-7.34159724157024,-13.101408894203,
120.530187095211)) ;
#173390=CARTESIAN_POINT('Ctrl Pts',(-7.36657138807077,-13.3874022195482,
120.570964865022)) ;
#173391=CARTESIAN_POINT('Ctrl Pts',(-7.36752626591963,-13.6768759171903,
120.538418289664)) ;
#173392=CARTESIAN_POINT('Ctrl Pts',(-7.34470605061851,-13.948608493865,
120.433347699827)) ;
#173393=CARTESIAN_POINT('Ctrl Pts',(-7.30074221590675,-14.181257681225,
120.264014178484)) ;
#173394=CARTESIAN_POINT('Ctrl Pts',(-7.23958451504645,-14.3592650506284,
120.042343425265)) ;
#173395=CARTESIAN_POINT('Ctrl Pts',(-7.16614529781219,-14.4703402370834,
119.783202402502)) ;
#173396=CARTESIAN_POINT('Ctrl Pts',(-7.08630537122041,-14.5059089260168,
119.504470384707)) ;
#173397=CARTESIAN_POINT('Ctrl Pts',(-7.00714711584661,-14.4635906108697,
119.22798980315)) ;
#173398=CARTESIAN_POINT('Ctrl Pts',(-6.9343979792678,-14.3462861335646,
118.970893409468)) ;
#173399=CARTESIAN_POINT('Ctrl Pts',(-6.87439561306881,-14.1620807273187,
118.752616009014)) ;
#173400=CARTESIAN_POINT('Ctrl Pts',(-6.83231279792918,-13.9257450561724,
118.589088105333)) ;
#173401=CARTESIAN_POINT('Ctrl Pts',(-6.81152149947454,-13.6518932520307,
118.490235528419)) ;
#173402=CARTESIAN_POINT('Ctrl Pts',(-6.81458866379034,-13.361350209501,
118.464074361768)) ;
#173403=CARTESIAN_POINT('Ctrl Pts',(-6.84190912425954,-13.0754523993138,
118.511850887542)) ;
#173404=CARTESIAN_POINT('Ctrl Pts',(-6.89221998106671,-12.8139381990977,
118.629651920743)) ;
#173405=CARTESIAN_POINT('Ctrl Pts',(-6.96317166541847,-12.5948180944483,
118.810143346469)) ;
#173406=CARTESIAN_POINT('Ctrl Pts',(-7.04930238281719,-12.4362800048722,
119.037190426179)) ;
#173407=CARTESIAN_POINT('Ctrl Pts',(-7.14639896583729,-12.346922078608,
119.29741677471)) ;
#173408=CARTESIAN_POINT('Ctrl Pts',(-7.24765406779605,-12.3346186385411,
119.570362985162)) ;
#173409=CARTESIAN_POINT('Ctrl Pts',(-7.34665382402801,-12.3998225687949,
119.836445852581)) ;
#173410=CARTESIAN_POINT('Ctrl Pts',(-7.4370740592955,-12.5378477500096,
120.076408147661)) ;
#173411=CARTESIAN_POINT('Ctrl Pts',(-7.5133452204639,-12.7392396507352,
120.273212489585)) ;
#173412=CARTESIAN_POINT('Ctrl Pts',(-7.57051158312834,-12.989236405783,
120.411850909373)) ;
#173413=CARTESIAN_POINT('Ctrl Pts',(-7.60526793750275,-13.269049028932,
120.482338834054)) ;
#173414=CARTESIAN_POINT('Ctrl Pts',(-7.61610217928452,-13.560604521515,
120.479829556645)) ;
#173415=CARTESIAN_POINT('Ctrl Pts',(-7.60265701261583,-13.8423158077137,
120.4033105886)) ;
#173416=CARTESIAN_POINT('Ctrl Pts',(-7.56703031046435,-14.0920492190499,
120.259455200578)) ;
#173417=CARTESIAN_POINT('Ctrl Pts',(-7.51204303377268,-14.2950965364046,
120.056387264096)) ;
#173418=CARTESIAN_POINT('Ctrl Pts',(-7.44273831121475,-14.434335219557,
119.809815786678)) ;
#173419=CARTESIAN_POINT('Ctrl Pts',(-7.36521040000063,-14.5007530721094,
119.538381721836)) ;
#173420=CARTESIAN_POINT('Ctrl Pts',(-7.28479809434297,-14.4901437351793,
119.257926243117)) ;
#173421=CARTESIAN_POINT('Ctrl Pts',(-7.20843821052364,-14.402041943339,
118.989761053497)) ;
#173422=CARTESIAN_POINT('Ctrl Pts',(-7.1427835920666,-14.243691286176,118.754343222241)) ;
#173423=CARTESIAN_POINT('Ctrl Pts',(-7.09305076334606,-14.0272168477211,
118.567541759605)) ;
#173424=CARTESIAN_POINT('Ctrl Pts',(-7.06320365437595,-13.7664028194368,
118.441170630651)) ;
#173425=CARTESIAN_POINT('Ctrl Pts',(-7.05638533636368,-13.4798811075686,
118.384860283325)) ;
#173426=CARTESIAN_POINT('Ctrl Pts',(-7.07408092560861,-13.1885796838075,
118.403166688914)) ;
#173427=CARTESIAN_POINT('Ctrl Pts',(-7.11507198338345,-12.9166253502417,
118.492814113544)) ;
#173428=CARTESIAN_POINT('Ctrl Pts',(-7.1780574208389,-12.6775835687805,
118.649064501798)) ;
#173429=CARTESIAN_POINT('Ctrl Pts',(-7.25891893918462,-12.4925681740676,
118.859833268336)) ;
#173430=CARTESIAN_POINT('Ctrl Pts',(-7.35188793041178,-12.3743553948694,
119.107715107246)) ;
#173431=CARTESIAN_POINT('Ctrl Pts',(-7.45265031525607,-12.3300586716913,
119.37899047094)) ;
#173432=CARTESIAN_POINT('Ctrl Pts',(-7.55337524562207,-12.3643855283945,
119.650314676817)) ;
#173433=CARTESIAN_POINT('Ctrl Pts',(-7.64773366833853,-12.4735026256636,
119.902366613272)) ;
#173434=CARTESIAN_POINT('Ctrl Pts',(-7.73041986817396,-12.6505044221707,
120.118738891923)) ;
#173435=CARTESIAN_POINT('Ctrl Pts',(-7.79595012127722,-12.883421947767,
120.282755379935)) ;
#173436=CARTESIAN_POINT('Ctrl Pts',(-7.83999077408972,-13.1527514798463,
120.381574983125)) ;
#173437=CARTESIAN_POINT('Ctrl Pts',(-7.86072974007722,-13.4437023579035,
120.40908356129)) ;
#173438=CARTESIAN_POINT('Ctrl Pts',(-7.85692244140455,-13.7306193771303,
120.362100112163)) ;
#173439=CARTESIAN_POINT('Ctrl Pts',(-7.83012410737516,-13.9949086675026,
120.245151518457)) ;
#173440=CARTESIAN_POINT('Ctrl Pts',(-7.78237083717385,-14.2196906214034,
120.06409456817)) ;
#173441=CARTESIAN_POINT('Ctrl Pts',(-7.71854875724072,-14.3856064052365,
119.834353268658)) ;
#173442=CARTESIAN_POINT('Ctrl Pts',(-7.64334502750247,-14.4829720573525,
119.569777363778)) ;
#173443=CARTESIAN_POINT('Ctrl Pts',(-7.56338289868114,-14.5039687036518,
119.290821303275)) ;
#173444=CARTESIAN_POINT('Ctrl Pts',(-7.48437547453331,-14.4466173797893,
119.014508165448)) ;
#173445=CARTESIAN_POINT('Ctrl Pts',(-7.41403834460529,-14.3162716014842,
118.764955621569)) ;
#173446=CARTESIAN_POINT('Ctrl Pts',(-7.35704039989976,-14.1214968775469,
118.555885778132)) ;
#173447=CARTESIAN_POINT('Ctrl Pts',(-7.31852311276589,-13.8749956323593,
118.402954989973)) ;
#173448=CARTESIAN_POINT('Ctrl Pts',(-7.30231103568058,-13.5974682752699,
118.318202627209)) ;
#173449=CARTESIAN_POINT('Ctrl Pts',(-7.30987663537963,-13.3070931499256,
118.305860700972)) ;
#173450=CARTESIAN_POINT('Ctrl Pts',(-7.34175942853511,-13.0233508116479,
118.36742076646)) ;
#173451=CARTESIAN_POINT('Ctrl Pts',(-7.39618528009665,-12.7688607554056,
118.497769967232)) ;
#173452=CARTESIAN_POINT('Ctrl Pts',(-7.47020228300154,-12.5604071436069,
118.687726339368)) ;
#173453=CARTESIAN_POINT('Ctrl Pts',(-7.55906350518853,-12.4137261008746,
118.922952330464)) ;
#173454=CARTESIAN_POINT('Ctrl Pts',(-7.65717245038672,-12.3387040702925,
119.186368813652)) ;
#173455=CARTESIAN_POINT('Ctrl Pts',(-7.75884035692309,-12.3410592400664,
119.460451576393)) ;
#173456=CARTESIAN_POINT('Ctrl Pts',(-7.85654736634483,-12.4205041979803,
119.722651987663)) ;
#173457=CARTESIAN_POINT('Ctrl Pts',(-7.94481318053513,-12.5715202421064,
119.956000118428)) ;
#173458=CARTESIAN_POINT('Ctrl Pts',(-8.01771408381364,-12.7831706996134,
120.142578445181)) ;
#173459=CARTESIAN_POINT('Ctrl Pts',(-8.07085503105618,-13.0400861903177,
120.268992723008)) ;
#173460=CARTESIAN_POINT('Ctrl Pts',(-8.1012449479731,-13.3242719779506,
120.326083671067)) ;
#173461=CARTESIAN_POINT('Ctrl Pts',(-8.10739844779683,-13.6152878377403,
120.309341878199)) ;
#173462=CARTESIAN_POINT('Ctrl Pts',(-8.08962004095609,-13.8920338673762,
120.219720905231)) ;
#173463=CARTESIAN_POINT('Ctrl Pts',(-8.05001723486067,-14.1346381572922,
120.063660745971)) ;
#173464=CARTESIAN_POINT('Ctrl Pts',(-7.992024762362,-14.3262307223465,119.85152566265)) ;
#173465=CARTESIAN_POINT('Ctrl Pts',(-7.92087420413947,-14.4523301137118,
119.599430244914)) ;
#173466=CARTESIAN_POINT('Ctrl Pts',(-7.84204196997817,-14.5048566464616,
119.323854472488)) ;
#173467=CARTESIAN_POINT('Ctrl Pts',(-7.76186601911956,-14.4792282215674,
119.044096181178)) ;
#173468=CARTESIAN_POINT('Ctrl Pts',(-7.68732567425835,-14.3776591931245,
118.781625479166)) ;
#173469=CARTESIAN_POINT('Ctrl Pts',(-7.62415597339361,-14.2073582471136,
118.553754081591)) ;
#173470=CARTESIAN_POINT('Ctrl Pts',(-7.57772822356053,-13.980463190757,
118.376876023582)) ;
#173471=CARTESIAN_POINT('Ctrl Pts',(-7.55211423680401,-13.7134648384933,
118.263415580786)) ;
#173472=CARTESIAN_POINT('Ctrl Pts',(-7.54988396928805,-13.4252028157263,
118.221162235282)) ;
#173473=CARTESIAN_POINT('Ctrl Pts',(-7.57190400588021,-13.136660084581,
118.252804065339)) ;
#173474=CARTESIAN_POINT('Ctrl Pts',(-7.61755830701388,-12.8674128564449,
118.356315160482)) ;
#173475=CARTESIAN_POINT('Ctrl Pts',(-7.68406859821228,-12.6383938778605,
118.523453892796)) ;
#173476=CARTESIAN_POINT('Ctrl Pts',(-7.76755837693475,-12.465038874388,
118.74228416299)) ;
#173477=CARTESIAN_POINT('Ctrl Pts',(-7.86272316977547,-12.3599344396702,
118.99669592537)) ;
#173478=CARTESIAN_POINT('Ctrl Pts',(-7.96381251944024,-12.3306429195518,
119.269059347859)) ;
#173479=CARTESIAN_POINT('Ctrl Pts',(-8.06368380821921,-12.3792038030185,
119.537856629935)) ;
#173480=CARTESIAN_POINT('Ctrl Pts',(-8.15659748944132,-12.502250920438,
119.785364900155)) ;
#173481=CARTESIAN_POINT('Ctrl Pts',(-8.23623754753109,-12.690704289041,
119.992502391065)) ;
#173482=CARTESIAN_POINT('Ctrl Pts',(-8.29787978612712,-12.9312491813812,
120.144802031741)) ;
#173483=CARTESIAN_POINT('Ctrl Pts',(-8.33778763616187,-13.2069304836541,
120.230868966777)) ;
#173484=CARTESIAN_POINT('Ctrl Pts',(-8.35386611104003,-13.4971323588194,
120.244433805866)) ;
#173485=CARTESIAN_POINT('Ctrl Pts',(-8.34559176606117,-13.7832858649534,
120.183607286869)) ;
#173486=CARTESIAN_POINT('Ctrl Pts',(-8.31464185127322,-14.0408293277911,
120.054056184709)) ;
#173487=CARTESIAN_POINT('Ctrl Pts',(-8.26340664177902,-14.255952322556,
119.862377902584)) ;
#173488=CARTESIAN_POINT('Ctrl Pts',(-8.1971249772834,-14.4094466686143,
119.625180693076)) ;
#173489=CARTESIAN_POINT('Ctrl Pts',(-8.12040152389499,-14.4929694646286,
119.35593056019)) ;
#173490=CARTESIAN_POINT('Ctrl Pts',(-8.04009022848257,-14.4990155260453,
119.075851461994)) ;
#173491=CARTESIAN_POINT('Ctrl Pts',(-7.9625098388441,-14.4275804860338,
118.804068220134)) ;
#173492=CARTESIAN_POINT('Ctrl Pts',(-7.8941100124004,-14.284309082368,118.560336785865)) ;
#173493=CARTESIAN_POINT('Ctrl Pts',(-7.84012347499757,-14.0775350374868,
118.360268383229)) ;
#173494=CARTESIAN_POINT('Ctrl Pts',(-7.80588583848825,-13.8261134335288,
118.220747745965)) ;
#173495=CARTESIAN_POINT('Ctrl Pts',(-7.79385768957157,-13.5428648342343,
118.148500404782)) ;
#173496=CARTESIAN_POINT('Ctrl Pts',(-7.80612682657335,-13.252182353688,
118.150461687266)) ;
#173497=CARTESIAN_POINT('Ctrl Pts',(-7.84228893480843,-12.9730234465435,
118.225161565708)) ;
#173498=CARTESIAN_POINT('Ctrl Pts',(-7.90103421558884,-12.724731390434,
118.368470996422)) ;
#173499=CARTESIAN_POINT('Ctrl Pts',(-7.97782116130876,-12.5280561031159,
118.567077843843)) ;
#173500=CARTESIAN_POINT('Ctrl Pts',(-8.0692686377754,-12.3935893009494,
118.810023631757)) ;
#173501=CARTESIAN_POINT('Ctrl Pts',(-8.16837016553241,-12.333081965445,
119.076502994386)) ;
#173502=CARTESIAN_POINT('Ctrl Pts',(-8.27009279108481,-12.3505128306963,
119.350670896121)) ;
#173503=CARTESIAN_POINT('Ctrl Pts',(-8.3658449010965,-12.4433828921911,
119.60714075347)) ;
#173504=CARTESIAN_POINT('Ctrl Pts',(-8.45197505795687,-12.607349424796,
119.833841108759)) ;
#173505=CARTESIAN_POINT('Ctrl Pts',(-8.52120977492203,-12.8279036385121,
120.00940010572)) ;
#173506=CARTESIAN_POINT('Ctrl Pts',(-8.57055325895007,-13.0930059035689,
120.124025527535)) ;
#173507=CARTESIAN_POINT('Ctrl Pts',(-8.59625204583721,-13.3789266137586,
120.166977376249)) ;
#173508=CARTESIAN_POINT('Ctrl Pts',(-8.59788852250651,-13.6686885717782,
120.136495690536)) ;
#173509=CARTESIAN_POINT('Ctrl Pts',(-8.57580906244584,-13.9407698971193,
120.033752331659)) ;
#173510=CARTESIAN_POINT('Ctrl Pts',(-8.53228870836988,-14.1754452261927,
119.865663575393)) ;
#173511=CARTESIAN_POINT('Ctrl Pts',(-8.47162858688881,-14.3550939223612,
119.645549235714)) ;
#173512=CARTESIAN_POINT('Ctrl Pts',(-8.39799248590873,-14.468598908444,
119.385596001449)) ;
#173513=CARTESIAN_POINT('Ctrl Pts',(-8.31877491440371,-14.5058659881171,
119.109007145666)) ;
#173514=CARTESIAN_POINT('Ctrl Pts',(-8.23941378855136,-14.465907705861,
118.831859781048)) ;
#173515=CARTESIAN_POINT('Ctrl Pts',(-8.16647270185438,-14.3507454275659,
118.574221540228)) ;
#173516=CARTESIAN_POINT('Ctrl Pts',(-8.10601871451368,-14.1684902162708,
118.354580107972)) ;
#173517=CARTESIAN_POINT('Ctrl Pts',(-8.06327379464778,-13.9330107336615,
118.188967146787)) ;
#173518=CARTESIAN_POINT('Ctrl Pts',(-8.04188464728271,-13.6600763512271,
118.088315145107)) ;
#173519=CARTESIAN_POINT('Ctrl Pts',(-8.04415984284868,-13.3704757504778,
118.059833665652)) ;
#173520=CARTESIAN_POINT('Ctrl Pts',(-8.07098859328993,-13.0823700026988,
118.105885959188)) ;
#173521=CARTESIAN_POINT('Ctrl Pts',(-8.120503467602,-12.8213180178566,118.221441446184)) ;
#173522=CARTESIAN_POINT('Ctrl Pts',(-8.19068066224925,-12.6009816910039,
118.399651162582)) ;
#173523=CARTESIAN_POINT('Ctrl Pts',(-8.27663038654765,-12.4399155910324,
118.626049746092)) ;
#173524=CARTESIAN_POINT('Ctrl Pts',(-8.37377653671491,-12.3483508718252,
118.886335164228)) ;
#173525=CARTESIAN_POINT('Ctrl Pts',(-8.47470424960895,-12.3338872424077,
119.158388022071)) ;
#173526=CARTESIAN_POINT('Ctrl Pts',(-8.5740859453798,-12.396923495094,119.425556245681)) ;
#173527=CARTESIAN_POINT('Ctrl Pts',(-8.6649277864638,-12.5334553693914,
119.666748762957)) ;
#173528=CARTESIAN_POINT('Ctrl Pts',(-8.74128429943828,-12.7322215761211,
119.863992617795)) ;
#173529=CARTESIAN_POINT('Ctrl Pts',(-8.79916573819104,-12.9810049412899,
120.004790749052)) ;
#173530=CARTESIAN_POINT('Ctrl Pts',(-8.83469320205863,-13.2609753303157,
120.077533333241)) ;
#173531=CARTESIAN_POINT('Ctrl Pts',(-8.84616539838749,-13.5522070361543,
120.07700191012)) ;
#173532=CARTESIAN_POINT('Ctrl Pts',(-8.83352879857719,-13.8335794690488,
120.003072712917)) ;
#173533=CARTESIAN_POINT('Ctrl Pts',(-8.79840525558534,-14.0854850074698,
119.86061077159)) ;
#173534=CARTESIAN_POINT('Ctrl Pts',(-8.74411665331808,-14.2893882283517,
119.659805611785)) ;
#173535=CARTESIAN_POINT('Ctrl Pts',(-8.67521497823715,-14.4310416708449,
119.414456500244)) ;
#173536=CARTESIAN_POINT('Ctrl Pts',(-8.59746348536126,-14.4999960091202,
119.142167399687)) ;
#173537=CARTESIAN_POINT('Ctrl Pts',(-8.51725220866625,-14.4914668725251,
118.862420893709)) ;
#173538=CARTESIAN_POINT('Ctrl Pts',(-8.44094453814601,-14.4062237339893,
118.594550823069)) ;
#173539=CARTESIAN_POINT('Ctrl Pts',(-8.37461958404781,-14.2495321967945,
118.356968882225)) ;
#173540=CARTESIAN_POINT('Ctrl Pts',(-8.32425634296907,-14.0340281298451,
118.168167653125)) ;
#173541=CARTESIAN_POINT('Ctrl Pts',(-8.29382206288613,-13.7742259092907,
118.040014681808)) ;
#173542=CARTESIAN_POINT('Ctrl Pts',(-8.28631480334285,-13.488993839479,
117.981708548653)) ;
#173543=CARTESIAN_POINT('Ctrl Pts',(-8.30320195637338,-13.1975717487405,
117.997560479062)) ;
#173544=CARTESIAN_POINT('Ctrl Pts',(-8.3436703131233,-12.9237175982201,
118.085475777875)) ;
#173545=CARTESIAN_POINT('Ctrl Pts',(-8.4062239104521,-12.6833926232874,
118.240377888327)) ;
#173546=CARTESIAN_POINT('Ctrl Pts',(-8.48615190099208,-12.4975233316372,
118.448503252107)) ;
#173547=CARTESIAN_POINT('Ctrl Pts',(-8.57934667074232,-12.3765652756753,
118.696871045336)) ;
#173548=CARTESIAN_POINT('Ctrl Pts',(-8.67942447659642,-12.3303669115662,
118.966269185261)) ;
#173549=CARTESIAN_POINT('Ctrl Pts',(-8.78046560292115,-12.3620831181533,
119.23847587387)) ;
#173550=CARTESIAN_POINT('Ctrl Pts',(-8.87549407917763,-12.4697592102098,
119.49241363428)) ;
#173551=CARTESIAN_POINT('Ctrl Pts',(-8.95832054343873,-12.6447797711106,
119.709301795168)) ;
#173552=CARTESIAN_POINT('Ctrl Pts',(-9.02420754409074,-12.8750273852739,
119.874571217192)) ;
#173553=CARTESIAN_POINT('Ctrl Pts',(-9.06917668282671,-13.1453257818208,
119.975977828757)) ;
#173554=CARTESIAN_POINT('Ctrl Pts',(-9.09047067571145,-13.4336234546741,
120.005474883971)) ;
#173555=CARTESIAN_POINT('Ctrl Pts',(-9.08746787607695,-13.7229316022969,
119.960694301127)) ;
#173556=CARTESIAN_POINT('Ctrl Pts',(-9.06117191970581,-13.9881204584926,
119.845257989114)) ;
#173557=CARTESIAN_POINT('Ctrl Pts',(-9.01419630762022,-14.2135626266573,
119.66671241156)) ;
#173558=CARTESIAN_POINT('Ctrl Pts',(-8.95045579816424,-14.3820856851378,
119.437041610208)) ;
#173559=CARTESIAN_POINT('Ctrl Pts',(-8.87581727914137,-14.4811007735871,
119.174352555604)) ;
#173560=CARTESIAN_POINT('Ctrl Pts',(-8.79562316232527,-14.5043853087956,
118.894554465702)) ;
#173561=CARTESIAN_POINT('Ctrl Pts',(-8.71698219857194,-14.4497319209782,
118.619592459032)) ;
#173562=CARTESIAN_POINT('Ctrl Pts',(-8.64580441276013,-14.3208489038209,
118.36724001526)) ;
#173563=CARTESIAN_POINT('Ctrl Pts',(-8.5883553866719,-14.1269083086763,
118.156726837458)) ;
#173564=CARTESIAN_POINT('Ctrl Pts',(-8.54955936673305,-13.8839530008224,
118.003271664693)) ;
#173565=CARTESIAN_POINT('Ctrl Pts',(-8.53248329253628,-13.6058131007772,
117.915704634662)) ;
#173566=CARTESIAN_POINT('Ctrl Pts',(-8.53937026013509,-13.3154623494247,
117.901296893058)) ;
#173567=CARTESIAN_POINT('Ctrl Pts',(-8.57069168239456,-13.0305252756843,
117.961054033285)) ;
#173568=CARTESIAN_POINT('Ctrl Pts',(-8.62430702145784,-12.7760411077928,
118.089081673625)) ;
#173569=CARTESIAN_POINT('Ctrl Pts',(-8.69778013803695,-12.5658693797106,
118.277375059853)) ;
#173570=CARTESIAN_POINT('Ctrl Pts',(-8.78628545767639,-12.4170609140262,
118.511509776539)) ;
#173571=CARTESIAN_POINT('Ctrl Pts',(-8.88463232709871,-12.3396249333132,
118.775501151269)) ;
#173572=CARTESIAN_POINT('Ctrl Pts',(-8.9861492359783,-12.340046412335,119.04917803503)) ;
#173573=CARTESIAN_POINT('Ctrl Pts',(-9.08378193823022,-12.4170460254182,
119.311248494083)) ;
#173574=CARTESIAN_POINT('Ctrl Pts',(-9.17250255530307,-12.5662136094611,
119.545947051563)) ;
#173575=CARTESIAN_POINT('Ctrl Pts',(-9.24585112857785,-12.7760199991739,
119.733930887948)) ;
#173576=CARTESIAN_POINT('Ctrl Pts',(-9.29969159508292,-13.0322696653641,
119.862416821601)) ;
#173577=CARTESIAN_POINT('Ctrl Pts',(-9.33072971583805,-13.3151090323585,
119.921587753964)) ;
#173578=CARTESIAN_POINT('Ctrl Pts',(-9.33762134165996,-13.6075492018493,
119.906927850832)) ;
#173579=CARTESIAN_POINT('Ctrl Pts',(-9.32055446084888,-13.8839937911961,
119.819605029903)) ;
#173580=CARTESIAN_POINT('Ctrl Pts',(-9.28147726722591,-14.1283418739825,
119.665069210431)) ;
#173581=CARTESIAN_POINT('Ctrl Pts',(-9.22417716238159,-14.321085337762,
119.455168775729)) ;
#173582=CARTESIAN_POINT('Ctrl Pts',(-9.1528918141783,-14.4501544762085,
119.202433516862)) ;
#173583=CARTESIAN_POINT('Ctrl Pts',(-9.07410157725992,-14.504350239421,
118.926962323926)) ;
#173584=CARTESIAN_POINT('Ctrl Pts',(-8.99439714763998,-14.4811635345991,
118.648874617531)) ;
#173585=CARTESIAN_POINT('Ctrl Pts',(-8.91938092952298,-14.3816036851556,
118.384850057937)) ;
#173586=CARTESIAN_POINT('Ctrl Pts',(-8.8558492241993,-14.2132115910195,
118.155902462999)) ;
#173587=CARTESIAN_POINT('Ctrl Pts',(-8.80875359263179,-13.9871283531687,
117.97689596451)) ;
#173588=CARTESIAN_POINT('Ctrl Pts',(-8.78260162901795,-13.7209751384546,
117.86180531742)) ;
#173589=CARTESIAN_POINT('Ctrl Pts',(-8.7796418761099,-13.4341833204507,
117.817471206849)) ;
#173590=CARTESIAN_POINT('Ctrl Pts',(-8.80108831291345,-13.1440226446982,
117.847195297999)) ;
#173591=CARTESIAN_POINT('Ctrl Pts',(-8.84592426043001,-12.8750223963181,
117.948364040509)) ;
#173592=CARTESIAN_POINT('Ctrl Pts',(-8.91216833972909,-12.6437154561283,
118.114539740324)) ;
#173593=CARTESIAN_POINT('Ctrl Pts',(-8.99483011325719,-12.4695015573388,
118.331032618802)) ;
#173594=CARTESIAN_POINT('Ctrl Pts',(-9.08998111303647,-12.3618253102505,
118.585299380963)) ;
#173595=CARTESIAN_POINT('Ctrl Pts',(-9.1909709333649,-12.3304086987919,
118.857374561843)) ;
#173596=CARTESIAN_POINT('Ctrl Pts',(-9.29090632432286,-12.3767667157857,
119.126380154863)) ;
#173597=CARTESIAN_POINT('Ctrl Pts',(-9.38394796937826,-12.4973266925111,
119.374354583408)) ;
#173598=CARTESIAN_POINT('Ctrl Pts',(-9.4644362377349,-12.6849702880242,
119.583900943341)) ;
#173599=CARTESIAN_POINT('Ctrl Pts',(-9.5264642676195,-12.9239536141708,
119.737443599299)) ;
#173600=CARTESIAN_POINT('Ctrl Pts',(-9.56699499377198,-13.198264514804,
119.825482569648)) ;
#173601=CARTESIAN_POINT('Ctrl Pts',(-9.58379794756891,-13.4887696764051,
119.841196258796)) ;
#173602=CARTESIAN_POINT('Ctrl Pts',(-9.57628694483019,-13.7747050880232,
119.782787604556)) ;
#173603=CARTESIAN_POINT('Ctrl Pts',(-9.54578275574017,-14.0346989777519,
119.65439454944)) ;
#173604=CARTESIAN_POINT('Ctrl Pts',(-9.49516719411495,-14.2504823475427,
119.464718649369)) ;
#173605=CARTESIAN_POINT('Ctrl Pts',(-9.42925750378619,-14.4061007577842,
119.228637274552)) ;
#173606=CARTESIAN_POINT('Ctrl Pts',(-9.35244000585146,-14.4917978275685,
118.958975475398)) ;
#173607=CARTESIAN_POINT('Ctrl Pts',(-9.27254720983972,-14.4998539330622,
118.680348428381)) ;
#173608=CARTESIAN_POINT('Ctrl Pts',(-9.19483422021103,-14.4309092256038,
118.408185227294)) ;
#173609=CARTESIAN_POINT('Ctrl Pts',(-9.12600873086239,-14.2894596882656,
118.163115988674)) ;
#173610=CARTESIAN_POINT('Ctrl Pts',(-9.07154849099475,-14.0846391379262,
117.961648450783)) ;
#173611=CARTESIAN_POINT('Ctrl Pts',(-9.036633988908,-13.833584389583,117.819961399887)) ;
#173612=CARTESIAN_POINT('Ctrl Pts',(-9.02391466502751,-13.5522887119168,
117.745782719323)) ;
#173613=CARTESIAN_POINT('Ctrl Pts',(-9.03557274648368,-13.2592972529684,
117.745601612871)) ;
#173614=CARTESIAN_POINT('Ctrl Pts',(-9.07098090557538,-12.9811038250668,
117.818197097558)) ;
#173615=CARTESIAN_POINT('Ctrl Pts',(-9.1288816653457,-12.7319954339599,
117.959013661815)) ;
#173616=CARTESIAN_POINT('Ctrl Pts',(-9.20542108821079,-12.5329045763516,
118.156747660811)) ;
#173617=CARTESIAN_POINT('Ctrl Pts',(-9.2965722776736,-12.3964115152595,
118.398783809131)) ;
#173618=CARTESIAN_POINT('Ctrl Pts',(-9.39560158322444,-12.3338312624075,
118.665015098447)) ;
#173619=CARTESIAN_POINT('Ctrl Pts',(-9.4968318946719,-12.3486707517994,
118.937874104534)) ;
#173620=CARTESIAN_POINT('Ctrl Pts',(-9.59343723857601,-12.4397941697449,
119.196716726627)) ;
#173621=CARTESIAN_POINT('Ctrl Pts',(-9.67989153670841,-12.6021170084136,
119.424415022172)) ;
#173622=CARTESIAN_POINT('Ctrl Pts',(-9.74951237514481,-12.8208593941247,
119.601209318802)) ;
#173623=CARTESIAN_POINT('Ctrl Pts',(-9.79944954754396,-13.084370773037,
119.717716848365)) ;
#173624=CARTESIAN_POINT('Ctrl Pts',(-9.82597149657916,-13.3711928765175,
119.763016540292)) ;
#173625=CARTESIAN_POINT('Ctrl Pts',(-9.82819214417096,-13.6609866789311,
119.734331572361)) ;
#173626=CARTESIAN_POINT('Ctrl Pts',(-9.8068991329201,-13.9327616913683,
119.63413267067)) ;
#173627=CARTESIAN_POINT('Ctrl Pts',(-9.76382464831486,-14.1696775509721,
119.467276311035)) ;
#173628=CARTESIAN_POINT('Ctrl Pts',(-9.7036673139555,-14.3505522399701,
119.248758719857)) ;
#173629=CARTESIAN_POINT('Ctrl Pts',(-9.63071094051081,-14.4659895814683,
118.991045032151)) ;
#173630=CARTESIAN_POINT('Ctrl Pts',(-9.55101925277455,-14.5060552317741,
118.712756531787)) ;
#173631=CARTESIAN_POINT('Ctrl Pts',(-9.4714813916173,-14.4677867862301,
118.435025022222)) ;
#173632=CARTESIAN_POINT('Ctrl Pts',(-9.39862983053746,-14.3553856703914,
118.177844077314)) ;
#173633=CARTESIAN_POINT('Ctrl Pts',(-9.33739442485482,-14.1738642018268,
117.955618487218)) ;
#173634=CARTESIAN_POINT('Ctrl Pts',(-9.29429158603599,-13.9401973275635,
117.789022041494)) ;
#173635=CARTESIAN_POINT('Ctrl Pts',(-9.27225194137694,-13.6684975496401,
117.686437026218)) ;
#173636=CARTESIAN_POINT('Ctrl Pts',(-9.27379869131216,-13.3792258998284,
117.65575130022)) ;
#173637=CARTESIAN_POINT('Ctrl Pts',(-9.29992444127897,-13.0905267308239,
117.699639537515)) ;
#173638=CARTESIAN_POINT('Ctrl Pts',(-9.34881358143102,-12.8284630006125,
117.813282587224)) ;
#173639=CARTESIAN_POINT('Ctrl Pts',(-9.41846234787993,-12.6065365051644,
117.989873611575)) ;
#173640=CARTESIAN_POINT('Ctrl Pts',(-9.50417588053103,-12.4434900571409,
118.215497616744)) ;
#173641=CARTESIAN_POINT('Ctrl Pts',(-9.60073723451511,-12.3500508502058,
118.474134121631)) ;
#173642=CARTESIAN_POINT('Ctrl Pts',(-9.70194573753584,-12.3331953888952,
118.746927131276)) ;
#173643=CARTESIAN_POINT('Ctrl Pts',(-9.80131762641198,-12.3940161187778,
119.014124252987)) ;
#173644=CARTESIAN_POINT('Ctrl Pts',(-9.89248329484562,-12.5284976067023,
119.256301286483)) ;
#173645=CARTESIAN_POINT('Ctrl Pts',(-9.9693440763676,-12.7253590046235,
119.455101779986)) ;
#173646=CARTESIAN_POINT('Ctrl Pts',(-10.0281574646971,-12.9750336085797,
119.598466100957)) ;
#173647=CARTESIAN_POINT('Ctrl Pts',(-10.0639625581,-13.2518773391213,119.672384712737)) ;
#173648=CARTESIAN_POINT('Ctrl Pts',(-10.0762711870781,-13.5442043587849,
119.674255680769)) ;
#173649=CARTESIAN_POINT('Ctrl Pts',(-10.0642632265541,-13.8259451748865,
119.602266518667)) ;
#173650=CARTESIAN_POINT('Ctrl Pts',(-10.0296964583947,-14.0792480619856,
119.461456237366)) ;
#173651=CARTESIAN_POINT('Ctrl Pts',(-9.97588775903519,-14.2845087011992,
119.262132122512)) ;
#173652=CARTESIAN_POINT('Ctrl Pts',(-9.90744210014645,-14.4278905637469,
119.018229253178)) ;
#173653=CARTESIAN_POINT('Ctrl Pts',(-9.82982242385163,-14.49909499359,118.746322529544)) ;
#173654=CARTESIAN_POINT('Ctrl Pts',(-9.74956192660519,-14.492829252027,
118.466414353285)) ;
#173655=CARTESIAN_POINT('Ctrl Pts',(-9.67283879350772,-14.4093444300335,
118.197174970448)) ;
#173656=CARTESIAN_POINT('Ctrl Pts',(-9.60626579738372,-14.2544052422715,
117.958871810111)) ;
#173657=CARTESIAN_POINT('Ctrl Pts',(-9.55553746479956,-14.0410991720381,
117.769068814144)) ;
#173658=CARTESIAN_POINT('Ctrl Pts',(-9.52441285793816,-13.7816895970119,
117.638727760598)) ;
#173659=CARTESIAN_POINT('Ctrl Pts',(-9.51628185017245,-13.4976199910735,
117.578613119079)) ;
#173660=CARTESIAN_POINT('Ctrl Pts',(-9.53237212691088,-13.2063007087737,
117.592070626438)) ;
#173661=CARTESIAN_POINT('Ctrl Pts',(-9.57232919510587,-12.9308185504047,
117.678310643569)) ;
#173662=CARTESIAN_POINT('Ctrl Pts',(-9.634113078639,-12.690040453889,117.830986128613)) ;
#173663=CARTESIAN_POINT('Ctrl Pts',(-9.713580692807,-12.5021903792694,118.037691814633)) ;
#173664=CARTESIAN_POINT('Ctrl Pts',(-9.80659684966496,-12.3790435207342,
118.285471103814)) ;
#173665=CARTESIAN_POINT('Ctrl Pts',(-9.90658661047469,-12.3305042760163,
118.554594905817)) ;
#173666=CARTESIAN_POINT('Ctrl Pts',(-10.008066495342,-12.3604684800267,
118.827998813982)) ;
#173667=CARTESIAN_POINT('Ctrl Pts',(-10.1026122259296,-12.4650891112354,
119.080754567184)) ;
#173668=CARTESIAN_POINT('Ctrl Pts',(-10.1865625678926,-12.6397680496829,
119.300758559966)) ;
#173669=CARTESIAN_POINT('Ctrl Pts',(-10.2525551850904,-12.8673926753431,
119.466570849935)) ;
#173670=CARTESIAN_POINT('Ctrl Pts',(-10.2984413344148,-13.138383085188,
119.5705591487)) ;
#173671=CARTESIAN_POINT('Ctrl Pts',(-10.3201874020919,-13.4250580301084,
119.601606079011)) ;
#173672=CARTESIAN_POINT('Ctrl Pts',(-10.3180530372285,-13.713663843469,
119.559606091718)) ;
#173673=CARTESIAN_POINT('Ctrl Pts',(-10.2921786001434,-13.9818996954329,
119.445166371893)) ;
#173674=CARTESIAN_POINT('Ctrl Pts',(-10.245938215231,-14.2073240866329,
119.269059645356)) ;
#173675=CARTESIAN_POINT('Ctrl Pts',(-10.1827043131007,-14.3779496982449,
119.040941067964)) ;
#173676=CARTESIAN_POINT('Ctrl Pts',(-10.1079403524329,-14.4795452062324,
118.777702483988)) ;
#173677=CARTESIAN_POINT('Ctrl Pts',(-10.0277788315133,-14.504675613756,
118.497994836855)) ;
#173678=CARTESIAN_POINT('Ctrl Pts',(-9.94934961424335,-14.4524935600785,
118.223832977652)) ;
#173679=CARTESIAN_POINT('Ctrl Pts',(-9.8776805943081,-14.3253673837965,
117.969892660447)) ;
#173680=CARTESIAN_POINT('Ctrl Pts',(-9.81989105535084,-14.1335026343525,
117.758421157027)) ;
#173681=CARTESIAN_POINT('Ctrl Pts',(-9.78045273451247,-13.8914689377216,
117.602957988204)) ;
#173682=CARTESIAN_POINT('Ctrl Pts',(-9.76271568007487,-13.6147208150664,
117.513467417372)) ;
#173683=CARTESIAN_POINT('Ctrl Pts',(-9.76890870119331,-13.3237687258409,
117.4968563122)) ;
#173684=CARTESIAN_POINT('Ctrl Pts',(-9.79936071736111,-13.0396242352637,
117.554132453179)) ;
#173685=CARTESIAN_POINT('Ctrl Pts',(-9.85239927743223,-12.7830678889279,
117.680294085095)) ;
#173686=CARTESIAN_POINT('Ctrl Pts',(-9.9257847579806,-12.5704752635878,
117.868146840537)) ;
#173687=CARTESIAN_POINT('Ctrl Pts',(-10.0135422022618,-12.4206416986158,
118.100172237485)) ;
#173688=CARTESIAN_POINT('Ctrl Pts',(-10.1114862816905,-12.3408954926335,
118.363002383417)) ;
#173689=CARTESIAN_POINT('Ctrl Pts',(-10.2131168846024,-12.3388375024718,
118.636985267721)) ;
#173690=CARTESIAN_POINT('Ctrl Pts',(-10.3111631418804,-12.413706142133,
118.900239883285)) ;
#173691=CARTESIAN_POINT('Ctrl Pts',(-10.4005037459975,-12.5617183582742,
119.136700846574)) ;
#173692=CARTESIAN_POINT('Ctrl Pts',(-10.4738998219897,-12.7688407831079,
119.325034793762)) ;
#173693=CARTESIAN_POINT('Ctrl Pts',(-10.528497781938,-13.0241117816514,
119.455791678547)) ;
#173694=CARTESIAN_POINT('Ctrl Pts',(-10.5602307777131,-13.3070010234793,
119.517011250028)) ;
#173695=CARTESIAN_POINT('Ctrl Pts',(-10.5678547390295,-13.5985554109386,
119.504704332823)) ;
#173696=CARTESIAN_POINT('Ctrl Pts',(-10.5513598758863,-13.8770852609277,
119.418937728725)) ;
#173697=CARTESIAN_POINT('Ctrl Pts',(-10.5130330103292,-14.1214182763711,
119.266862919213)) ;
#173698=CARTESIAN_POINT('Ctrl Pts',(-10.4561208615973,-14.3164119676812,
119.058063869766)) ;
#173699=CARTESIAN_POINT('Ctrl Pts',(-10.3852189870946,-14.4472714989735,
118.806537992562)) ;
#173700=CARTESIAN_POINT('Ctrl Pts',(-10.3066385089528,-14.5039655219921,
118.531734459687)) ;
#173701=CARTESIAN_POINT('Ctrl Pts',(-10.2263549450695,-14.4826373105238,
118.251644902637)) ;
#173702=CARTESIAN_POINT('Ctrl Pts',(-10.1515928117172,-14.3855815012644,
117.988618093193)) ;
#173703=CARTESIAN_POINT('Ctrl Pts',(-10.0875742094217,-14.2190969785884,
117.758158308275)) ;
#173704=CARTESIAN_POINT('Ctrl Pts',(-10.0400271797391,-13.9949296481822,
117.577849034879)) ;
#173705=CARTESIAN_POINT('Ctrl Pts',(-10.013089520595,-13.7298783707897,
117.46036854867)) ;
#173706=CARTESIAN_POINT('Ctrl Pts',(-10.0095205229371,-13.4411780607526,
117.413901364897)) ;
#173707=CARTESIAN_POINT('Ctrl Pts',(-10.0300438994439,-13.1535366585443,
117.441164670617)) ;
#173708=CARTESIAN_POINT('Ctrl Pts',(-10.0745982760158,-12.8812078446008,
117.541146052817)) ;
#173709=CARTESIAN_POINT('Ctrl Pts',(-10.1399166575301,-12.6502697095916,
117.704747539768)) ;
#173710=CARTESIAN_POINT('Ctrl Pts',(-10.2222158366404,-12.4736381112203,
117.920071829275)) ;
#173711=CARTESIAN_POINT('Ctrl Pts',(-10.3174784950143,-12.3636957343507,
118.174552893488)) ;
#173712=CARTESIAN_POINT('Ctrl Pts',(-10.4179636590566,-12.3303161657527,
118.445239950958)) ;
#173713=CARTESIAN_POINT('Ctrl Pts',(-10.5180970410555,-12.3741418831008,
118.71482587813)) ;
#173714=CARTESIAN_POINT('Ctrl Pts',(-10.611946558723,-12.4937241519796,
118.965043678186)) ;
#173715=CARTESIAN_POINT('Ctrl Pts',(-10.6922395149728,-12.6783961032596,
119.174263610413)) ;
#173716=CARTESIAN_POINT('Ctrl Pts',(-10.7550368562695,-12.9163766433386,
119.330077430903)) ;
#173717=CARTESIAN_POINT('Ctrl Pts',(-10.7962673301715,-13.1903758945546,
119.420199225543)) ;
#173718=CARTESIAN_POINT('Ctrl Pts',(-10.8137492360295,-13.481432819081,
119.437894714578)) ;
#173719=CARTESIAN_POINT('Ctrl Pts',(-10.8068277964098,-13.7673558416161,
119.38132985396)) ;
#173720=CARTESIAN_POINT('Ctrl Pts',(-10.7770884508321,-14.0271101613543,
119.255429248926)) ;
#173721=CARTESIAN_POINT('Ctrl Pts',(-10.7271574214564,-14.2445027860115,
119.067879150203)) ;
#173722=CARTESIAN_POINT('Ctrl Pts',(-10.6612093802085,-14.4028029107363,
118.831466877353)) ;
#173723=CARTESIAN_POINT('Ctrl Pts',(-10.5852730928227,-14.4900131921161,
118.564801583323)) ;
#173724=CARTESIAN_POINT('Ctrl Pts',(-10.5049910429359,-14.5009049303826,
118.284799184651)) ;
#173725=CARTESIAN_POINT('Ctrl Pts',(-10.4268806844919,-14.4337694493022,
118.011321719883)) ;
#173726=CARTESIAN_POINT('Ctrl Pts',(-10.3576955154029,-14.2939322119372,
117.765123850201)) ;
#173727=CARTESIAN_POINT('Ctrl Pts',(-10.3029320432203,-14.0911613446941,
117.562827612356)) ;
#173728=CARTESIAN_POINT('Ctrl Pts',(-10.2673499177128,-13.8412394795533,
117.419099337292)) ;
#173729=CARTESIAN_POINT('Ctrl Pts',(-10.254056072628,-13.5592605313859,
117.343020397243)) ;
#173730=CARTESIAN_POINT('Ctrl Pts',(-10.2648180246204,-13.2696223387077,
117.34052655831)) ;
#173731=CARTESIAN_POINT('Ctrl Pts',(-10.2997358790123,-12.9883139496615,
117.411316976137)) ;
#173732=CARTESIAN_POINT('Ctrl Pts',(-10.3569669367904,-12.7386910562247,
117.550180832731)) ;
#173733=CARTESIAN_POINT('Ctrl Pts',(-10.4331834431151,-12.5375785963018,
117.746852091262)) ;
#173734=CARTESIAN_POINT('Ctrl Pts',(-10.5236752561247,-12.3995778757378,
117.98701193378)) ;
#173735=CARTESIAN_POINT('Ctrl Pts',(-10.6227835579732,-12.3345174279643,
118.253393687995)) ;
#173736=CARTESIAN_POINT('Ctrl Pts',(-10.7239238622889,-12.3471393395654,
118.526024465767)) ;
#173737=CARTESIAN_POINT('Ctrl Pts',(-10.8207516399519,-12.4360428670471,
118.785542422515)) ;
#173738=CARTESIAN_POINT('Ctrl Pts',(-10.9075644967453,-12.5962612233629,
119.014358156929)) ;
#173739=CARTESIAN_POINT('Ctrl Pts',(-10.9778413211601,-12.8139558923281,
119.19307998567)) ;
#173740=CARTESIAN_POINT('Ctrl Pts',(-11.0282836106079,-13.0756188660845,
119.311240887642)) ;
#173741=CARTESIAN_POINT('Ctrl Pts',(-11.0555791922085,-13.3624251132735,
119.358838014228)) ;
#173742=CARTESIAN_POINT('Ctrl Pts',(-11.0586048593759,-13.651982180129,
119.332672404455)) ;
#173743=CARTESIAN_POINT('Ctrl Pts',(-11.0376843527776,-13.9268736432231,
119.23328044909)) ;
#173744=CARTESIAN_POINT('Ctrl Pts',(-10.9956210330096,-14.1624927779437,
119.069898286994)) ;
#173745=CARTESIAN_POINT('Ctrl Pts',(-10.9354933314548,-14.3467872124729,
118.851183898762)) ;
#173746=CARTESIAN_POINT('Ctrl Pts',(-10.8629481065443,-14.4636106389172,
118.594821165369)) ;
#173747=CARTESIAN_POINT('Ctrl Pts',(-10.7836225816458,-14.505904926533,
118.317753204467)) ;
#173748=CARTESIAN_POINT('Ctrl Pts',(-10.7040268941245,-14.4703681622542,
118.039876785396)) ;
#173749=CARTESIAN_POINT('Ctrl Pts',(-10.6303958446743,-14.359008640194,
117.780055371545)) ;
#173750=CARTESIAN_POINT('Ctrl Pts',(-10.5692768535784,-14.1808823670753,
117.558510542006)) ;
#173751=CARTESIAN_POINT('Ctrl Pts',(-10.525296106505,-13.9476582149858,
117.389059170047)) ;
#173752=CARTESIAN_POINT('Ctrl Pts',(-10.5026217165176,-13.6767014389998,
117.284544765499)) ;
#173753=CARTESIAN_POINT('Ctrl Pts',(-10.503514877856,-13.3872299120028,
117.251810399679)) ;
#173754=CARTESIAN_POINT('Ctrl Pts',(-10.5287931159004,-13.0993467868879,
117.2932723904)) ;
#173755=CARTESIAN_POINT('Ctrl Pts',(-10.5772819647789,-12.8349662721153,
117.405511188278)) ;
#173756=CARTESIAN_POINT('Ctrl Pts',(-10.6462390061054,-12.6123125745559,
117.580099001699)) ;
#173757=CARTESIAN_POINT('Ctrl Pts',(-10.7316789245276,-12.447065748415,
117.804830116923)) ;
#173758=CARTESIAN_POINT('Ctrl Pts',(-10.8280555786512,-12.3516677675638,
118.062896940008)) ;
#173759=CARTESIAN_POINT('Ctrl Pts',(-10.9289420861559,-12.3325934792249,
118.334805693187)) ;
#173760=CARTESIAN_POINT('Ctrl Pts',(-11.0285549216706,-12.3910918553195,
118.602705295816)) ;
#173761=CARTESIAN_POINT('Ctrl Pts',(-11.1202575355664,-12.5239274893633,
118.846436016608)) ;
#173762=CARTESIAN_POINT('Ctrl Pts',(-11.1974790053523,-12.7192927751428,
119.046348283817)) ;
#173763=CARTESIAN_POINT('Ctrl Pts',(-11.256570149613,-12.9658343070978,
119.190811409268)) ;
#173764=CARTESIAN_POINT('Ctrl Pts',(-11.2934413311918,-13.2443245338218,
119.267674974483)) ;
#173765=CARTESIAN_POINT('Ctrl Pts',(-11.3062978123674,-13.5367809605308,
119.271198329631)) ;
#173766=CARTESIAN_POINT('Ctrl Pts',(-11.2949986489025,-13.8179726435299,
119.201501210985)) ;
#173767=CARTESIAN_POINT('Ctrl Pts',(-11.2610571461274,-14.0724753431544,
119.062587049155)) ;
#173768=CARTESIAN_POINT('Ctrl Pts',(-11.2078251507878,-14.279096140685,
118.865063933435)) ;
#173769=CARTESIAN_POINT('Ctrl Pts',(-11.1396467770328,-14.4248617955916,
118.621919734993)) ;
#173770=CARTESIAN_POINT('Ctrl Pts',(-11.0618371790876,-14.4982152843021,
118.349277506824)) ;
#173771=CARTESIAN_POINT('Ctrl Pts',(-10.9820685755435,-14.4941260357652,
118.071094122751)) ;
#173772=CARTESIAN_POINT('Ctrl Pts',(-10.9049115286395,-14.4126782343137,
117.800421801026)) ;
#173773=CARTESIAN_POINT('Ctrl Pts',(-10.8381211251888,-14.2599648668114,
117.561542528994)) ;
#173774=CARTESIAN_POINT('Ctrl Pts',(-10.7868067530969,-14.0478524029628,
117.369893536837)) ;
#173775=CARTESIAN_POINT('Ctrl Pts',(-10.7550957653846,-13.7904112840523,
117.237886359139)) ;
#173776=CARTESIAN_POINT('Ctrl Pts',(-10.7462257200646,-13.5044552055669,
117.175225916484)) ;
#173777=CARTESIAN_POINT('Ctrl Pts',(-10.7617483985087,-13.2137879040768,
117.187050717025)) ;
#173778=CARTESIAN_POINT('Ctrl Pts',(-10.8009076226651,-12.9385963486889,
117.270982185733)) ;
#173779=CARTESIAN_POINT('Ctrl Pts',(-10.8619688891867,-12.6966955833364,
117.421502681034)) ;
#173780=CARTESIAN_POINT('Ctrl Pts',(-10.9413222714456,-12.5064217313258,
117.627710657807)) ;
#173781=CARTESIAN_POINT('Ctrl Pts',(-11.0338914556794,-12.3814205030376,
117.874194374824)) ;
#173782=CARTESIAN_POINT('Ctrl Pts',(-11.1342884555144,-12.3309490204366,
118.144369386401)) ;
#173783=CARTESIAN_POINT('Ctrl Pts',(-11.2344352101216,-12.3579787522632,
118.414220057428)) ;
#173784=CARTESIAN_POINT('Ctrl Pts',(-11.3303750050126,-12.461461206882,
118.670792503069)) ;
#173785=CARTESIAN_POINT('Ctrl Pts',(-11.4139998494669,-12.6327579824641,
118.890139759141)) ;
#173786=CARTESIAN_POINT('Ctrl Pts',(-11.4811854191605,-12.8610649262646,
119.059239036713)) ;
#173787=CARTESIAN_POINT('Ctrl Pts',(-11.5272358980316,-13.1282120035714,
119.164129227647)) ;
#173788=CARTESIAN_POINT('Ctrl Pts',(-11.550031999704,-13.4170777357306,
119.198051643061)) ;
#173789=CARTESIAN_POINT('Ctrl Pts',(-11.5484863559817,-13.7056413839055,
119.157890620187)) ;
#173790=CARTESIAN_POINT('Ctrl Pts',(-11.5233022878553,-13.9747406301587,
119.04555969316)) ;
#173791=CARTESIAN_POINT('Ctrl Pts',(-11.4774772491034,-14.201974810105,
118.870644857214)) ;
#173792=CARTESIAN_POINT('Ctrl Pts',(-11.4147391200156,-14.3739130003505,
118.644102382187)) ;
#173793=CARTESIAN_POINT('Ctrl Pts',(-11.3404625025784,-14.4775305035498,
118.382452018192)) ;
#173794=CARTESIAN_POINT('Ctrl Pts',(-11.2600762837107,-14.5050608269986,
118.101928838668)) ;
#173795=CARTESIAN_POINT('Ctrl Pts',(-11.1816706187826,-14.4551363613954,
117.827909095909)) ;
#173796=CARTESIAN_POINT('Ctrl Pts',(-11.1096219883487,-14.3298705824412,
117.57276605832)) ;
#173797=CARTESIAN_POINT('Ctrl Pts',(-11.0516186729526,-14.1407879039854,
117.36082074906)) ;
#173798=CARTESIAN_POINT('Ctrl Pts',(-11.01133249899,-13.8991517087972,117.202620381188)) ;
#173799=CARTESIAN_POINT('Ctrl Pts',(-10.9929531483878,-13.622377664187,
117.111093121158)) ;
#173800=CARTESIAN_POINT('Ctrl Pts',(-10.9984700935864,-13.3324243748073,
117.092526186947)) ;
#173801=CARTESIAN_POINT('Ctrl Pts',(-11.0281068838988,-13.0478498918573,
117.147341996027)) ;
#173802=CARTESIAN_POINT('Ctrl Pts',(-11.081052628238,-12.7884262570381,
117.272939564718)) ;
#173803=CARTESIAN_POINT('Ctrl Pts',(-11.1532846644103,-12.5764203972658,
117.457617573228)) ;
#173804=CARTESIAN_POINT('Ctrl Pts',(-11.2410864798589,-12.4236100991773,
117.689588048581)) ;
#173805=CARTESIAN_POINT('Ctrl Pts',(-11.3390837070061,-12.3419562515338,
117.95250976013)) ;
#173806=CARTESIAN_POINT('Ctrl Pts',(-11.440496530574,-12.3379525743983,
118.225901103267)) ;
#173807=CARTESIAN_POINT('Ctrl Pts',(-11.5383739159563,-12.4104778611719,
118.488760855449)) ;
#173808=CARTESIAN_POINT('Ctrl Pts',(-11.6278480336845,-12.5557718304403,
118.725738663281)) ;
#173809=CARTESIAN_POINT('Ctrl Pts',(-11.7021593126348,-12.7621800376528,
118.916687014316)) ;
#173810=CARTESIAN_POINT('Ctrl Pts',(-11.7573807659036,-13.0168738808962,
119.049290511668)) ;
#173811=CARTESIAN_POINT('Ctrl Pts',(-11.7896803869344,-13.2984278863564,
119.112337306604)) ;
#173812=CARTESIAN_POINT('Ctrl Pts',(-11.7980400482597,-13.5897265030932,
119.102308017698)) ;
#173813=CARTESIAN_POINT('Ctrl Pts',(-11.7822956103083,-13.8688372211758,
119.018847493834)) ;
#173814=CARTESIAN_POINT('Ctrl Pts',(-11.7444566994981,-14.1152016754008,
118.868145849198)) ;
#173815=CARTESIAN_POINT('Ctrl Pts',(-11.6880197549201,-14.3116011164225,
118.660817745576)) ;
#173816=CARTESIAN_POINT('Ctrl Pts',(-11.6176369249549,-14.4442909382302,
118.410962690409)) ;
#173817=CARTESIAN_POINT('Ctrl Pts',(-11.5390960272606,-14.5033545209173,
118.136228492371)) ;
#173818=CARTESIAN_POINT('Ctrl Pts',(-11.4590251392824,-14.4845849990311,
117.856907062077)) ;
#173819=CARTESIAN_POINT('Ctrl Pts',(-11.383664627329,-14.3894948595566,
117.591898604544)) ;
#173820=CARTESIAN_POINT('Ctrl Pts',(-11.3191676650949,-14.2243477865837,
117.359917217915)) ;
#173821=CARTESIAN_POINT('Ctrl Pts',(-11.2712397649004,-14.0022176408066,
117.178548503574)) ;
#173822=CARTESIAN_POINT('Ctrl Pts',(-11.2436435716615,-13.738467096939,
117.059098820409)) ;
#173823=CARTESIAN_POINT('Ctrl Pts',(-11.2393171495216,-13.4497089979361,
117.010273305457)) ;
#173824=CARTESIAN_POINT('Ctrl Pts',(-11.2592549423813,-13.1612741016994,
117.035679695456)) ;
#173825=CARTESIAN_POINT('Ctrl Pts',(-11.3028442445725,-12.8897094409154,
117.132937982061)) ;
#173826=CARTESIAN_POINT('Ctrl Pts',(-11.3677649574765,-12.6562456914582,
117.295185497117)) ;
#173827=CARTESIAN_POINT('Ctrl Pts',(-11.4498623668221,-12.4776727385034,
117.509821759606)) ;
#173828=CARTESIAN_POINT('Ctrl Pts',(-11.5443175113425,-12.3662041520314,
117.762040087288)) ;
#173829=CARTESIAN_POINT('Ctrl Pts',(-11.6448025118947,-12.3300379060018,
118.032692201155)) ;
#173830=CARTESIAN_POINT('Ctrl Pts',(-11.7455128333517,-12.3719948524369,
118.303864829156)) ;
#173831=CARTESIAN_POINT('Ctrl Pts',(-11.8390028851572,-12.4886302946211,
118.553235459183)) ;
#173832=CARTESIAN_POINT('Ctrl Pts',(-11.9200724717719,-12.6716133926028,
118.764723942327)) ;
#173833=CARTESIAN_POINT('Ctrl Pts',(-11.983729776495,-12.9096205473869,
118.922975846097)) ;
#173834=CARTESIAN_POINT('Ctrl Pts',(-12.0254107822208,-13.1819739695916,
119.014592567458)) ;
#173835=CARTESIAN_POINT('Ctrl Pts',(-12.0436296355972,-13.4720244815185,
119.034627026831)) ;
#173836=CARTESIAN_POINT('Ctrl Pts',(-12.0374852966316,-13.7591219512168,
118.980348270067)) ;
#173837=CARTESIAN_POINT('Ctrl Pts',(-12.0081585226799,-14.0209982570872,
118.855533677512)) ;
#173838=CARTESIAN_POINT('Ctrl Pts',(-11.9589803424424,-14.2386408615737,
118.670464829268)) ;
#173839=CARTESIAN_POINT('Ctrl Pts',(-11.8933789786321,-14.3991847031552,
118.435064542878)) ;
#173840=CARTESIAN_POINT('Ctrl Pts',(-11.8176447978217,-14.4885294284138,
118.169014818533)) ;
#173841=CARTESIAN_POINT('Ctrl Pts',(-11.7374057481524,-14.5016597743674,
117.889145533914)) ;
#173842=CARTESIAN_POINT('Ctrl Pts',(-11.6592539148603,-14.437009415365,
117.615605436135)) ;
#173843=CARTESIAN_POINT('Ctrl Pts',(-11.5896054471436,-14.2988734246617,
117.367922624978)) ;
#173844=CARTESIAN_POINT('Ctrl Pts',(-11.5345577224684,-14.0989764690058,
117.164944532834)) ;
#173845=CARTESIAN_POINT('Ctrl Pts',(-11.4980687401448,-13.8484694868484,
117.018190484838)) ;
#173846=CARTESIAN_POINT('Ctrl Pts',(-11.484185252244,-13.5679794956402,
116.940440639052)) ;
#173847=CARTESIAN_POINT('Ctrl Pts',(-11.4942413352023,-13.2778704302602,
116.935732247541)) ;
#173848=CARTESIAN_POINT('Ctrl Pts',(-11.5283649580948,-12.9966579805532,
117.004198786349)) ;
#173849=CARTESIAN_POINT('Ctrl Pts',(-11.5851655684408,-12.7449733317735,
117.141625652285)) ;
#173850=CARTESIAN_POINT('Ctrl Pts',(-11.6608769322514,-12.5424420519023,
117.336783089927)) ;
#173851=CARTESIAN_POINT('Ctrl Pts',(-11.751128641274,-12.4024494998622,
117.576178163021)) ;
#173852=CARTESIAN_POINT('Ctrl Pts',(-11.849749431196,-12.33540698977,117.841192600071)) ;
#173853=CARTESIAN_POINT('Ctrl Pts',(-11.9511794851965,-12.3455818235887,
118.114616538353)) ;
#173854=CARTESIAN_POINT('Ctrl Pts',(-12.048568512048,-12.433061741337,118.375702938129)) ;
#173855=CARTESIAN_POINT('Ctrl Pts',(-12.1352985452608,-12.5907670484714,
118.604444245422)) ;
#173856=CARTESIAN_POINT('Ctrl Pts',(-12.2062338243243,-12.8072730343164,
118.785110454359)) ;
#173857=CARTESIAN_POINT('Ctrl Pts',(-12.2572961681927,-13.0681776762317,
118.90514030015)) ;
#173858=CARTESIAN_POINT('Ctrl Pts',(-12.2852469770119,-13.3550287065478,
118.954680417514)) ;
#173859=CARTESIAN_POINT('Ctrl Pts',(-12.288870726614,-13.6436167217993,
118.930470264435)) ;
#173860=CARTESIAN_POINT('Ctrl Pts',(-12.2688371151345,-13.9180811572707,
118.833953017997)) ;
#173861=CARTESIAN_POINT('Ctrl Pts',(-12.2271646134758,-14.156549136634,
118.671552459278)) ;
#173862=CARTESIAN_POINT('Ctrl Pts',(-12.1674566622439,-14.3423727651068,
118.454127809899)) ;
#173863=CARTESIAN_POINT('Ctrl Pts',(-12.0952414310603,-14.4613427108393,
118.198784751216)) ;
#173864=CARTESIAN_POINT('Ctrl Pts',(-12.0156536366213,-14.5057889124528,
117.920757945584)) ;
#173865=CARTESIAN_POINT('Ctrl Pts',(-11.9363592364177,-14.4724226584541,
117.643968542152)) ;
#173866=CARTESIAN_POINT('Ctrl Pts',(-11.8623371282566,-14.3630839653471,
117.382899183667)) ;
#173867=CARTESIAN_POINT('Ctrl Pts',(-11.8008173863079,-14.1865023299291,
117.160124591948)) ;
#173868=CARTESIAN_POINT('Ctrl Pts',(-11.7563748042704,-13.9552367476643,
116.989354134913)) ;
#173869=CARTESIAN_POINT('Ctrl Pts',(-11.7329833978953,-13.6844063432408,
116.882563304078)) ;
#173870=CARTESIAN_POINT('Ctrl Pts',(-11.7332475390205,-13.395616216205,
116.847967590773)) ;
#173871=CARTESIAN_POINT('Ctrl Pts',(-11.7576801957441,-13.1080920804484,
116.886949996486)) ;
#173872=CARTESIAN_POINT('Ctrl Pts',(-11.8057887216514,-12.8414911099526,
116.997851240026)) ;
#173873=CARTESIAN_POINT('Ctrl Pts',(-11.8738646701692,-12.6185827250958,
117.169942474425)) ;
#173874=CARTESIAN_POINT('Ctrl Pts',(-11.959020038101,-12.4509854490646,
117.393736018184)) ;
#173875=CARTESIAN_POINT('Ctrl Pts',(-12.0550313167262,-12.3534810644787,
117.650738776618)) ;
#173876=CARTESIAN_POINT('Ctrl Pts',(-12.1561839108002,-12.3320089256095,
117.923345972253)) ;
#173877=CARTESIAN_POINT('Ctrl Pts',(-12.2558122040571,-12.3884256006082,
118.1913322941)) ;
#173878=CARTESIAN_POINT('Ctrl Pts',(-12.3475394657345,-12.5185566369419,
118.43526353432)) ;
#173879=CARTESIAN_POINT('Ctrl Pts',(-12.4255960408986,-12.7128146761132,
118.637581654736)) ;
#173880=CARTESIAN_POINT('Ctrl Pts',(-12.4854118400066,-12.9591843124397,
118.784128401409)) ;
#173881=CARTESIAN_POINT('Ctrl Pts',(-12.5227062774273,-13.2359003760254,
118.862430198041)) ;
#173882=CARTESIAN_POINT('Ctrl Pts',(-12.5363357220994,-13.5269168879405,
118.86847314923)) ;
#173883=CARTESIAN_POINT('Ctrl Pts',(-12.5257513802662,-13.8100818853549,
118.80078051953)) ;
#173884=CARTESIAN_POINT('Ctrl Pts',(-12.4923757936398,-14.0658493622321,
118.663565106864)) ;
#173885=CARTESIAN_POINT('Ctrl Pts',(-12.4395119409733,-14.2744004374724,
118.467090668042)) ;
#173886=CARTESIAN_POINT('Ctrl Pts',(-12.371795140951,-14.4215076088756,
118.225429654782)) ;
#173887=CARTESIAN_POINT('Ctrl Pts',(-12.2946403903294,-14.4970287487176,
117.954986337942)) ;
#173888=CARTESIAN_POINT('Ctrl Pts',(-12.2142494904348,-14.495364180026,
117.674634887753)) ;
#173889=CARTESIAN_POINT('Ctrl Pts',(-12.1371207254048,-14.4159600881982,
117.404140731358)) ;
#173890=CARTESIAN_POINT('Ctrl Pts',(-12.0701819932153,-14.2660479877099,
117.164946413806)) ;
#173891=CARTESIAN_POINT('Ctrl Pts',(-12.0180738968896,-14.0549162780305,
116.970748910434)) ;
#173892=CARTESIAN_POINT('Ctrl Pts',(-11.9857272141969,-13.7973888984154,
116.836670452939)) ;
#173893=CARTESIAN_POINT('Ctrl Pts',(-11.9762272551923,-13.5143192821472,
116.772389751235)) ;
#173894=CARTESIAN_POINT('Ctrl Pts',(-11.9909277151902,-13.2228141005811,
116.78161966851)) ;
#173895=CARTESIAN_POINT('Ctrl Pts',(-12.0294614824962,-12.9463122499942,
116.863581031885)) ;
#173896=CARTESIAN_POINT('Ctrl Pts',(-12.0901776028958,-12.7025112775513,
117.012934916738)) ;
#173897=CARTESIAN_POINT('Ctrl Pts',(-12.1687375174296,-12.5113386435153,
117.216879767183)) ;
#173898=CARTESIAN_POINT('Ctrl Pts',(-12.2612290461381,-12.3839986409936,
117.463033125205)) ;
#173899=CARTESIAN_POINT('Ctrl Pts',(-12.3609719875208,-12.3313598679509,
117.731405074504)) ;
#173900=CARTESIAN_POINT('Ctrl Pts',(-12.4619148744611,-12.3561484752169,
118.003421771831)) ;
#173901=CARTESIAN_POINT('Ctrl Pts',(-12.558035703025,-12.4578681360596,
118.260559283857)) ;
#173902=CARTESIAN_POINT('Ctrl Pts',(-12.6418650591551,-12.6270814220524,
118.480600547495)) ;
#173903=CARTESIAN_POINT('Ctrl Pts',(-12.709500616301,-12.8533401319523,
118.65115248197)) ;
#173904=CARTESIAN_POINT('Ctrl Pts',(-12.7564269379405,-13.1210491167834,
118.758518890216)) ;
#173905=CARTESIAN_POINT('Ctrl Pts',(-12.7797729830741,-13.40900770729,118.794199282391)) ;
#173906=CARTESIAN_POINT('Ctrl Pts',(-12.7789054138412,-13.6972694862933,
118.756166722536)) ;
#173907=CARTESIAN_POINT('Ctrl Pts',(-12.7545947470765,-13.9663054532962,
118.646647736907)) ;
#173908=CARTESIAN_POINT('Ctrl Pts',(-12.708953623995,-14.1969043333081,
118.471990317947)) ;
#173909=CARTESIAN_POINT('Ctrl Pts',(-12.6467531532713,-14.3698914257013,
118.24719675644)) ;
#173910=CARTESIAN_POINT('Ctrl Pts',(-12.5727418641631,-14.4755193866787,
117.986353001203)) ;
#173911=CARTESIAN_POINT('Ctrl Pts',(-12.4928027634597,-14.5054697818126,
117.707363787146)) ;
#173912=CARTESIAN_POINT('Ctrl Pts',(-12.4137352350169,-14.4574393177702,
117.431077181479)) ;
#173913=CARTESIAN_POINT('Ctrl Pts',(-12.3418324266654,-14.3349211938034,
117.176601530105)) ;
#173914=CARTESIAN_POINT('Ctrl Pts',(-12.2830970975097,-14.1470800055845,
116.962290261975)) ;
#173915=CARTESIAN_POINT('Ctrl Pts',(-12.2422554856577,-13.9065331674936,
116.80239048803)) ;
#173916=CARTESIAN_POINT('Ctrl Pts',(-12.2232261811748,-13.630738678715,
116.708912567899)) ;
#173917=CARTESIAN_POINT('Ctrl Pts',(-12.2280126456687,-13.3408270196336,
116.688112612688)) ;
#173918=CARTESIAN_POINT('Ctrl Pts',(-12.2570791816381,-13.0553492265632,
116.741127681574)) ;
#173919=CARTESIAN_POINT('Ctrl Pts',(-12.3090343418545,-12.7963986353394,
116.863927628217)) ;
#173920=CARTESIAN_POINT('Ctrl Pts',(-12.3809755753915,-12.581755675213,
117.047570548939)) ;
#173921=CARTESIAN_POINT('Ctrl Pts',(-12.4684134110327,-12.4271874700909,
117.278442488482)) ;
#173922=CARTESIAN_POINT('Ctrl Pts',(-12.5658597005341,-12.3434882644401,
117.539803720469)) ;
#173923=CARTESIAN_POINT('Ctrl Pts',(-12.6672936908425,-12.3367187774922,
117.813250325772)) ;
#173924=CARTESIAN_POINT('Ctrl Pts',(-12.765948884936,-12.4076100218016,
118.078256939231)) ;
#173925=CARTESIAN_POINT('Ctrl Pts',(-12.8553355026567,-12.5503272886106,
118.315139856333)) ;
#173926=CARTESIAN_POINT('Ctrl Pts',(-12.9304176070875,-12.7556871760659,
118.508319195545)) ;
#173927=CARTESIAN_POINT('Ctrl Pts',(-12.9861723417227,-13.0091921750313,
118.642571963292)) ;
#173928=CARTESIAN_POINT('Ctrl Pts',(-13.0191734609878,-13.2902503547293,
118.707745845769)) ;
#173929=CARTESIAN_POINT('Ctrl Pts',(-13.028209715569,-13.5823834440121,
118.699683255514)) ;
#173930=CARTESIAN_POINT('Ctrl Pts',(-13.0130366717192,-13.8618181146796,
118.617988137292)) ;
#173931=CARTESIAN_POINT('Ctrl Pts',(-12.9759659852745,-14.1083106024044,
118.469780251358)) ;
#173932=CARTESIAN_POINT('Ctrl Pts',(-12.9198792403032,-14.3070623418306,
118.263416505571)) ;
#173933=CARTESIAN_POINT('Ctrl Pts',(-12.849560606782,-14.4418892785907,
118.013651989613)) ;
#173934=CARTESIAN_POINT('Ctrl Pts',(-12.7712938037721,-14.502692884587,
117.739819479159)) ;
#173935=CARTESIAN_POINT('Ctrl Pts',(-12.691443150556,-14.4862255258319,
117.461283982672)) ;
#173936=CARTESIAN_POINT('Ctrl Pts',(-12.6158746315244,-14.3934141564473,
117.195652815533)) ;
#173937=CARTESIAN_POINT('Ctrl Pts',(-12.5509163096876,-14.2302607448999,
116.962257398382)) ;
#173938=CARTESIAN_POINT('Ctrl Pts',(-12.5022332898898,-14.0081666908763,
116.778385267356)) ;
#173939=CARTESIAN_POINT('Ctrl Pts',(-12.4742506823548,-13.7466548362381,
116.657950049822)) ;
#173940=CARTESIAN_POINT('Ctrl Pts',(-12.4691100549571,-13.4587847124533,
116.606699386214)) ;
#173941=CARTESIAN_POINT('Ctrl Pts',(-12.4885192361608,-13.1685102080527,
116.630294437279)) ;
#173942=CARTESIAN_POINT('Ctrl Pts',(-12.5312093541707,-12.8978336872395,
116.725034238603)) ;
#173943=CARTESIAN_POINT('Ctrl Pts',(-12.5957395733222,-12.6619537350285,
116.885954892402)) ;
#173944=CARTESIAN_POINT('Ctrl Pts',(-12.6776143419512,-12.4816257056073,
117.099854766256)) ;
#173945=CARTESIAN_POINT('Ctrl Pts',(-12.7713529617644,-12.3684889471066,
117.350055385643)) ;
#173946=CARTESIAN_POINT('Ctrl Pts',(-12.8723202400041,-12.3299903879882,
117.621972650026)) ;
#173947=CARTESIAN_POINT('Ctrl Pts',(-12.9724385289638,-12.3696139932957,
117.891584408557)) ;
#173948=CARTESIAN_POINT('Ctrl Pts',(-13.0664515487238,-12.4839372794238,
118.142479880966)) ;
#173949=CARTESIAN_POINT('Ctrl Pts',(-13.1484405032608,-12.6667316342934,
118.356525775525)) ;
#173950=CARTESIAN_POINT('Ctrl Pts',(-13.2121850011556,-12.9020313562946,
118.515277498017)) ;
#173951=CARTESIAN_POINT('Ctrl Pts',(-13.2546371352095,-13.1740426154344,
118.609174623203)) ;
#173952=CARTESIAN_POINT('Ctrl Pts',(-13.2734900958146,-13.4634545824485,
118.631199247328)) ;
#173953=CARTESIAN_POINT('Ctrl Pts',(-13.2680796257058,-13.7505708131454,
118.579201045788)) ;
#173954=CARTESIAN_POINT('Ctrl Pts',(-13.2394962360415,-14.0133363300327,
118.456684613439)) ;
#173955=CARTESIAN_POINT('Ctrl Pts',(-13.1905999974754,-14.2335678065818,
118.272293478368)) ;
#173956=CARTESIAN_POINT('Ctrl Pts',(-13.1253712311633,-14.3958087768564,
118.038043104771)) ;
#173957=CARTESIAN_POINT('Ctrl Pts',(-13.0496091296525,-14.4872051600084,
117.771802663667)) ;
#173958=CARTESIAN_POINT('Ctrl Pts',(-12.9697977471393,-14.5023836342265,
117.493417412762)) ;
#173959=CARTESIAN_POINT('Ctrl Pts',(-12.8911729784752,-14.4395233841403,
117.218279983479)) ;
#173960=CARTESIAN_POINT('Ctrl Pts',(-12.8215722521092,-14.3038981389521,
116.970926660863)) ;
#173961=CARTESIAN_POINT('Ctrl Pts',(-12.765908924504,-14.1052991872385,
116.765996341192)) ;
#173962=CARTESIAN_POINT('Ctrl Pts',(-12.7289194558588,-13.8563431079666,
116.617783489361)) ;
#173963=CARTESIAN_POINT('Ctrl Pts',(-12.7143046569284,-13.5768529523028,
116.537845772707)) ;
#173964=CARTESIAN_POINT('Ctrl Pts',(-12.7237017190187,-13.2855121533732,
116.530980294664)) ;
#173965=CARTESIAN_POINT('Ctrl Pts',(-12.7572168622974,-13.0041275578471,
116.597631042541)) ;
#173966=CARTESIAN_POINT('Ctrl Pts',(-12.8130794083186,-12.7524010633512,
116.732371814801)) ;
#173967=CARTESIAN_POINT('Ctrl Pts',(-12.88854761512,-12.5474082659178,116.92665451824)) ;
#173968=CARTESIAN_POINT('Ctrl Pts',(-12.9782123177536,-12.4057612857423,
117.164359360981)) ;
#173969=CARTESIAN_POINT('Ctrl Pts',(-13.0770064791105,-12.3361751661113,
117.429775138385)) ;
#173970=CARTESIAN_POINT('Ctrl Pts',(-13.1783190413846,-12.3442704255669,
117.702890794258)) ;
#173971=CARTESIAN_POINT('Ctrl Pts',(-13.2756527267231,-12.4291570429794,
117.963909021848)) ;
#173972=CARTESIAN_POINT('Ctrl Pts',(-13.36292678935,-12.5849331529663,118.194259899517)) ;
#173973=CARTESIAN_POINT('Ctrl Pts',(-13.4345794652228,-12.8005108515807,
118.377018028647)) ;
#173974=CARTESIAN_POINT('Ctrl Pts',(-13.4861674949149,-13.060269126664,
118.498676029101)) ;
#173975=CARTESIAN_POINT('Ctrl Pts',(-13.5147933718825,-13.3453693583979,
118.550429429881)) ;
#173976=CARTESIAN_POINT('Ctrl Pts',(-13.5191703640909,-13.6361640667827,
118.528261672456)) ;
#173977=CARTESIAN_POINT('Ctrl Pts',(-13.4997846887976,-13.9104324089111,
118.433833737107)) ;
#173978=CARTESIAN_POINT('Ctrl Pts',(-13.4587413574297,-14.1501784561149,
118.27335686083)) ;
#173979=CARTESIAN_POINT('Ctrl Pts',(-13.39950930923,-14.3377944456025,118.057390334685)) ;
#173980=CARTESIAN_POINT('Ctrl Pts',(-13.32749153125,-14.4588735568458,117.802602901111)) ;
#173981=CARTESIAN_POINT('Ctrl Pts',(-13.2483458924945,-14.5056122473976,
117.526071610546)) ;
#173982=CARTESIAN_POINT('Ctrl Pts',(-13.1685437749415,-14.4743736272664,
117.247539732196)) ;
#173983=CARTESIAN_POINT('Ctrl Pts',(-13.0946020226361,-14.3676054099568,
116.986884001878)) ;
#173984=CARTESIAN_POINT('Ctrl Pts',(-13.0324910029511,-14.1926642104704,
116.762231273457)) ;
#173985=CARTESIAN_POINT('Ctrl Pts',(-12.9874746142067,-13.9629645552833,
116.589736773677)) ;
#173986=CARTESIAN_POINT('Ctrl Pts',(-12.9633562559811,-13.6916669453695,
116.48056065792)) ;
#173987=CARTESIAN_POINT('Ctrl Pts',(-12.9629691653421,-13.4042886281479,
116.444129256868)) ;
#173988=CARTESIAN_POINT('Ctrl Pts',(-12.9867239596031,-13.1160881842174,
116.481000353099)) ;
#173989=CARTESIAN_POINT('Ctrl Pts',(-13.0339690435015,-12.8495738757798,
116.589413701142)) ;
#173990=CARTESIAN_POINT('Ctrl Pts',(-13.1016362988514,-12.6242652876755,
116.76014561289)) ;
#173991=CARTESIAN_POINT('Ctrl Pts',(-13.1868381515301,-12.4543477917217,
116.98391806025)) ;
#173992=CARTESIAN_POINT('Ctrl Pts',(-13.282130994495,-12.3553371823295,
117.238917231087)) ;
#173993=CARTESIAN_POINT('Ctrl Pts',(-13.3835527278556,-12.3315537600446,
117.512226746283)) ;
#173994=CARTESIAN_POINT('Ctrl Pts',(-13.4828912406925,-12.3856473127391,
117.779479511165)) ;
#173995=CARTESIAN_POINT('Ctrl Pts',(-13.5751280064643,-12.513656004823,
118.024906933845)) ;
#173996=CARTESIAN_POINT('Ctrl Pts',(-13.6539134068514,-12.707439556573,
118.229281918463)) ;
#173997=CARTESIAN_POINT('Ctrl Pts',(-13.7137234776106,-12.9500051005904,
118.376179984501)) ;
#173998=CARTESIAN_POINT('Ctrl Pts',(-13.7520689708624,-13.2274462581565,
118.457479335507)) ;
#173999=CARTESIAN_POINT('Ctrl Pts',(-13.7663393260749,-13.5192262317475,
118.465377287378)) ;
#174000=CARTESIAN_POINT('Ctrl Pts',(-13.7564573176797,-13.8018769048648,
118.399949096535)) ;
#174001=CARTESIAN_POINT('Ctrl Pts',(-13.7237468055255,-14.058784271986,
118.264759363062)) ;
#174002=CARTESIAN_POINT('Ctrl Pts',(-13.6714025576082,-14.2690401451517,
118.069862285334)) ;
#174003=CARTESIAN_POINT('Ctrl Pts',(-13.6038901489006,-14.418345814643,
117.828744781992)) ;
#174004=CARTESIAN_POINT('Ctrl Pts',(-13.5270066699605,-14.4960013207205,
117.559173432525)) ;
#174005=CARTESIAN_POINT('Ctrl Pts',(-13.4463172125483,-14.4962457299704,
117.277772265082)) ;
#174006=CARTESIAN_POINT('Ctrl Pts',(-13.3696988473351,-14.4198799151553,
117.009166760654)) ;
#174007=CARTESIAN_POINT('Ctrl Pts',(-13.3017866089322,-14.2709014086462,
116.76670550127)) ;
#174008=CARTESIAN_POINT('Ctrl Pts',(-13.2493889815294,-14.0614284920593,
116.571702252918)) ;
#174009=CARTESIAN_POINT('Ctrl Pts',(-13.2164243628667,-13.8059370930909,
116.435853274894)) ;
#174010=CARTESIAN_POINT('Ctrl Pts',(-13.2062477246467,-13.5211628984478,
116.369237660814)) ;
#174011=CARTESIAN_POINT('Ctrl Pts',(-13.2201829843462,-13.2317212421624,
116.376408413708)) ;
#174012=CARTESIAN_POINT('Ctrl Pts',(-13.2582351273943,-12.953209842425,
116.456720631326)) ;
#174013=CARTESIAN_POINT('Ctrl Pts',(-13.3179987777289,-12.7094642616823,
116.60338316649)) ;
#174014=CARTESIAN_POINT('Ctrl Pts',(-13.3968395702768,-12.5150572905195,
116.807856696789)) ;
#174015=CARTESIAN_POINT('Ctrl Pts',(-13.4880657336334,-12.3871819681861,
117.050541251165)) ;
#174016=CARTESIAN_POINT('Ctrl Pts',(-13.5882207279045,-12.3316884564228,
117.319958997263)) ;
#174017=CARTESIAN_POINT('Ctrl Pts',(-13.6888941607603,-12.3542922095437,
117.591275254107)) ;
#174018=CARTESIAN_POINT('Ctrl Pts',(-13.7853698113562,-12.4537268763868,
117.849457635997)) ;
#174019=CARTESIAN_POINT('Ctrl Pts',(-13.8696982601704,-12.6212675456056,
118.070986029358)) ;
#174020=CARTESIAN_POINT('Ctrl Pts',(-13.9378798134609,-12.846192059173,
118.243189707452)) ;
#174021=CARTESIAN_POINT('Ctrl Pts',(-13.9854016724836,-13.1124184461725,
118.352441492381)) ;
#174022=CARTESIAN_POINT('Ctrl Pts',(-14.0095130072085,-13.400879749144,
118.390345126407)) ;
#174023=CARTESIAN_POINT('Ctrl Pts',(-14.0093724892591,-13.6891262166377,
118.354574264124)) ;
#174024=CARTESIAN_POINT('Ctrl Pts',(-13.985414910218,-13.9605413879786,
118.245894494186)) ;
#174025=CARTESIAN_POINT('Ctrl Pts',(-13.9409451108123,-14.1894540736428,
118.075288407443)) ;
#174026=CARTESIAN_POINT('Ctrl Pts',(-13.8788030525502,-14.3660067048925,
117.850395877402)) ;
#174027=CARTESIAN_POINT('Ctrl Pts',(-13.805049295041,-14.4734792612079,
117.590360278057)) ;
#174028=CARTESIAN_POINT('Ctrl Pts',(-13.7251059804211,-14.5056975632985,
117.311316857951)) ;
#174029=CARTESIAN_POINT('Ctrl Pts',(-13.6460687434891,-14.4599236721213,
117.035189019244)) ;
#174030=CARTESIAN_POINT('Ctrl Pts',(-13.5738853047407,-14.3395761921465,
116.779866121718)) ;
#174031=CARTESIAN_POINT('Ctrl Pts',(-13.5146382184193,-14.1535350418836,
116.563988746602)) ;
#174032=CARTESIAN_POINT('Ctrl Pts',(-13.4731069605417,-13.9130985111844,
116.401832242531)) ;
#174033=CARTESIAN_POINT('Ctrl Pts',(-13.4535360973529,-13.6395736822347,
116.306908957539)) ;
#174034=CARTESIAN_POINT('Ctrl Pts',(-13.4576157743933,-13.3487006076146,
116.283814176628)) ;
#174035=CARTESIAN_POINT('Ctrl Pts',(-13.4859406302875,-13.0636371844073,
116.334679965118)) ;
#174036=CARTESIAN_POINT('Ctrl Pts',(-13.537302484578,-12.803286823163,116.455624512449)) ;
#174037=CARTESIAN_POINT('Ctrl Pts',(-13.6086911430819,-12.5872505028287,
116.637604570861)) ;
#174038=CARTESIAN_POINT('Ctrl Pts',(-13.6958832608641,-12.4304809457012,
116.867672531912)) ;
#174039=CARTESIAN_POINT('Ctrl Pts',(-13.7933144950255,-12.3447676693836,
117.128927982332)) ;
#174040=CARTESIAN_POINT('Ctrl Pts',(-13.8942106173158,-12.3358385329225,
117.400917482378)) ;
#174041=CARTESIAN_POINT('Ctrl Pts',(-13.9931058830893,-12.4042599768703,
117.666636589428)) ;
#174042=CARTESIAN_POINT('Ctrl Pts',(-14.0830802598219,-12.5454038835963,
117.905215825566)) ;
#174043=CARTESIAN_POINT('Ctrl Pts',(-14.1585388443987,-12.7490645526663,
118.099576579279)) ;
#174044=CARTESIAN_POINT('Ctrl Pts',(-14.2147792241185,-13.0004109945635,
118.235435558541)) ;
#174045=CARTESIAN_POINT('Ctrl Pts',(-14.2486273894212,-13.281956740539,
118.303050309436)) ;
#174046=CARTESIAN_POINT('Ctrl Pts',(-14.2583346166308,-13.573019683806,
118.297166121252)) ;
#174047=CARTESIAN_POINT('Ctrl Pts',(-14.2439797697,-13.8532505028034,118.217957846964)) ;
#174048=CARTESIAN_POINT('Ctrl Pts',(-14.2073259241701,-14.1021597581384,
118.070845549194)) ;
#174049=CARTESIAN_POINT('Ctrl Pts',(-14.1518319080389,-14.3018608409922,
117.866383830764)) ;
#174050=CARTESIAN_POINT('Ctrl Pts',(-14.0821691837154,-14.4384983198451,
117.618753194085)) ;
#174051=CARTESIAN_POINT('Ctrl Pts',(-14.0038053646086,-14.5020770602936,
117.344502812886)) ;
#174052=CARTESIAN_POINT('Ctrl Pts',(-13.9237302084394,-14.48777877411,117.065203884427)) ;
#174053=CARTESIAN_POINT('Ctrl Pts',(-13.8479693987333,-14.3970097456745,
116.798993617263)) ;
#174054=CARTESIAN_POINT('Ctrl Pts',(-13.782799826033,-14.2362612997962,
116.5650573821)) ;
#174055=CARTESIAN_POINT('Ctrl Pts',(-13.733518100292,-14.0159101115065,
116.379369583749)) ;
#174056=CARTESIAN_POINT('Ctrl Pts',(-13.7047590259111,-13.7543350935969,
116.256429298379)) ;
#174057=CARTESIAN_POINT('Ctrl Pts',(-13.699032750653,-13.4665595551094,
116.203361929234)) ;
#174058=CARTESIAN_POINT('Ctrl Pts',(-13.7175768117472,-13.1776643244991,
116.224521765399)) ;
#174059=CARTESIAN_POINT('Ctrl Pts',(-13.7598364090687,-12.90467088677,116.317749177515)) ;
#174060=CARTESIAN_POINT('Ctrl Pts',(-13.8234518415385,-12.6688603640825,
116.476089051097)) ;
#174061=CARTESIAN_POINT('Ctrl Pts',(-13.9049557333608,-12.48602188738,116.688787580776)) ;
#174062=CARTESIAN_POINT('Ctrl Pts',(-13.9989576689692,-12.3704601308902,
116.939602004027)) ;
#174063=CARTESIAN_POINT('Ctrl Pts',(-14.0992273955684,-12.3301504850153,
117.209607062401)) ;
#174064=CARTESIAN_POINT('Ctrl Pts',(-14.1995620772837,-12.3670848663884,
117.479845083354)) ;
#174065=CARTESIAN_POINT('Ctrl Pts',(-14.2945308343906,-12.4806961242678,
117.733368848111)) ;
#174066=CARTESIAN_POINT('Ctrl Pts',(-14.3760228392886,-12.659847054779,
117.946296624332)) ;
#174067=CARTESIAN_POINT('Ctrl Pts',(-14.4406901314542,-12.8944266812495,
118.107719161995)) ;
#174068=CARTESIAN_POINT('Ctrl Pts',(-14.4837690484985,-13.1656332510844,
118.203535687924)) ;
#174069=CARTESIAN_POINT('Ctrl Pts',(-14.5033674776862,-13.455130793988,
118.227791066086)) ;
#174070=CARTESIAN_POINT('Ctrl Pts',(-14.4986092754277,-13.7427936624919,
118.177758141915)) ;
#174071=CARTESIAN_POINT('Ctrl Pts',(-14.4707221810934,-14.0059776158613,
118.057435006683)) ;
#174072=CARTESIAN_POINT('Ctrl Pts',(-14.422360755841,-14.2279037819529,
117.874652010575)) ;
#174073=CARTESIAN_POINT('Ctrl Pts',(-14.3575106947756,-14.3919406672911,
117.641551257708)) ;
#174074=CARTESIAN_POINT('Ctrl Pts',(-14.2822303298045,-14.4855253459423,
117.376890300863)) ;
#174075=CARTESIAN_POINT('Ctrl Pts',(-14.2019505143216,-14.5029122651219,
117.09684616291)) ;
#174076=CARTESIAN_POINT('Ctrl Pts',(-14.1238906002577,-14.4429567945224,
116.823764513881)) ;
#174077=CARTESIAN_POINT('Ctrl Pts',(-14.0534400115056,-14.3088313127917,
116.573580387455)) ;
#174078=CARTESIAN_POINT('Ctrl Pts',(-13.9973344587926,-14.1118280044828,
116.36732016952)) ;
#174079=CARTESIAN_POINT('Ctrl Pts',(-13.9596840563562,-13.8633524569287,
116.216996890361)) ;
#174080=CARTESIAN_POINT('Ctrl Pts',(-13.9444872281656,-13.5856086171591,
116.135434675017)) ;
#174081=CARTESIAN_POINT('Ctrl Pts',(-13.9531206776375,-13.29429050433,116.126236655127)) ;
#174082=CARTESIAN_POINT('Ctrl Pts',(-13.9859156053883,-13.0122145331766,
116.19068657179)) ;
#174083=CARTESIAN_POINT('Ctrl Pts',(-14.0414265852797,-12.7583429519339,
116.324206721183)) ;
#174084=CARTESIAN_POINT('Ctrl Pts',(-14.1163566701285,-12.5522896132778,
116.516904433369)) ;
#174085=CARTESIAN_POINT('Ctrl Pts',(-14.2054208500919,-12.4090180636989,
116.75287655481)) ;
#174086=CARTESIAN_POINT('Ctrl Pts',(-14.3041315741692,-12.3371174607651,
117.018003366661)) ;
#174087=CARTESIAN_POINT('Ctrl Pts',(-14.4053499510961,-12.3428658905722,
117.290874128105)) ;
#174088=CARTESIAN_POINT('Ctrl Pts',(-14.5030362331871,-12.4257351119528,
117.55290734156)) ;
#174089=CARTESIAN_POINT('Ctrl Pts',(-14.5904621270827,-12.5790185234623,
117.783826332769)) ;
#174090=CARTESIAN_POINT('Ctrl Pts',(-14.6629652552051,-12.7940406828703,
117.969008479269)) ;
#174091=CARTESIAN_POINT('Ctrl Pts',(-14.7149782729242,-13.0518842131347,
118.092091883262)) ;
#174092=CARTESIAN_POINT('Ctrl Pts',(-14.7443671066665,-13.3370763555055,
118.146092536195)) ;
#174093=CARTESIAN_POINT('Ctrl Pts',(-14.7494764883566,-13.6270297095458,
118.126281327732)) ;
#174094=CARTESIAN_POINT('Ctrl Pts',(-14.7306708206297,-13.9038567932623,
118.033390708072)) ;
#174095=CARTESIAN_POINT('Ctrl Pts',(-14.690027558541,-14.1447030861545,
117.874109045323)) ;
#174096=CARTESIAN_POINT('Ctrl Pts',(-14.6316472186503,-14.332817774621,
117.660971076182)) ;
#174097=CARTESIAN_POINT('Ctrl Pts',(-14.5597455784243,-14.45646682902,117.406433016193)) ;
#174098=CARTESIAN_POINT('Ctrl Pts',(-14.4807629365922,-14.5053560860543,
117.130424369544)) ;
#174099=CARTESIAN_POINT('Ctrl Pts',(-14.4006764355962,-14.4762759602464,
116.850932976369)) ;
#174100=CARTESIAN_POINT('Ctrl Pts',(-14.3265390078925,-14.3712943997113,
116.589686458049)) ;
#174101=CARTESIAN_POINT('Ctrl Pts',(-14.2642291252365,-14.1990455522355,
116.364581017991)) ;
#174102=CARTESIAN_POINT('Ctrl Pts',(-14.2184481514674,-13.969268231171,
116.189542795207)) ;
#174103=CARTESIAN_POINT('Ctrl Pts',(-14.1938561787033,-13.7012052922517,
116.079239578809)) ;
#174104=CARTESIAN_POINT('Ctrl Pts',(-14.1927076708075,-13.4115854195081,
116.040169663763)) ;
#174105=CARTESIAN_POINT('Ctrl Pts',(-14.2158186831131,-13.1240520278943,
116.075200920001)) ;
#174106=CARTESIAN_POINT('Ctrl Pts',(-14.2623847117566,-12.8565945311091,
116.181543563239)) ;
#174107=CARTESIAN_POINT('Ctrl Pts',(-14.3295805648497,-12.6299321000607,
116.350826699486)) ;
#174108=CARTESIAN_POINT('Ctrl Pts',(-14.4139535876279,-12.458754218581,
116.572235100756)) ;
#174109=CARTESIAN_POINT('Ctrl Pts',(-14.5094836498744,-12.3569969390507,
116.827772100287)) ;
#174110=CARTESIAN_POINT('Ctrl Pts',(-14.6106904064239,-12.3311725454961,
117.10048536176)) ;
#174111=CARTESIAN_POINT('Ctrl Pts',(-14.7103650458112,-12.3830921654557,
117.368691273652)) ;
#174112=CARTESIAN_POINT('Ctrl Pts',(-14.8029787361383,-12.5097082549453,
117.615209351864)) ;
#174113=CARTESIAN_POINT('Ctrl Pts',(-14.8815949767115,-12.6999655173835,
117.819379893254)) ;
#174114=CARTESIAN_POINT('Ctrl Pts',(-14.9425172204992,-12.9431519741363,
117.969375033027)) ;
#174115=CARTESIAN_POINT('Ctrl Pts',(-14.9812992054159,-13.2187420743147,
118.052168315938)) ;
#174116=CARTESIAN_POINT('Ctrl Pts',(-14.9963500333539,-13.5111774969548,
118.062342681364)) ;
#174117=CARTESIAN_POINT('Ctrl Pts',(-14.9871457345053,-13.7940494918521,
117.999019373326)) ;
#174118=CARTESIAN_POINT('Ctrl Pts',(-14.9548742901699,-14.0529110285333,
117.865026253004)) ;
#174119=CARTESIAN_POINT('Ctrl Pts',(-14.9032500009219,-14.2634870650102,
117.672503574574)) ;
#174120=CARTESIAN_POINT('Ctrl Pts',(-14.8361924144871,-14.4148461022599,
117.432794192959)) ;
#174121=CARTESIAN_POINT('Ctrl Pts',(-14.7594134311292,-14.494780073978,
117.16350011444)) ;
#174122=CARTESIAN_POINT('Ctrl Pts',(-14.6788165394104,-14.4974507314962,
116.882424493313)) ;
#174123=CARTESIAN_POINT('Ctrl Pts',(-14.6018098242213,-14.4229495346006,
116.612531368624)) ;
#174124=CARTESIAN_POINT('Ctrl Pts',(-14.5338249366433,-14.2768020033666,
116.370022693878)) ;
#174125=CARTESIAN_POINT('Ctrl Pts',(-14.4805103340185,-14.0672719747909,
116.171945276152)) ;
#174126=CARTESIAN_POINT('Ctrl Pts',(-14.4472092133991,-13.8140437794069,
116.035263380737)) ;
#174127=CARTESIAN_POINT('Ctrl Pts',(-14.4362486432515,-13.5305545368903,
115.96633944488)) ;
#174128=CARTESIAN_POINT('Ctrl Pts',(-14.449486240473,-13.2400469135056,
115.971266296655)) ;
#174129=CARTESIAN_POINT('Ctrl Pts',(-14.4868824566312,-12.9607801917685,
116.04957346963)) ;
#174130=CARTESIAN_POINT('Ctrl Pts',(-14.5461400633249,-12.7157522020321,
116.194666581357)) ;
#174131=CARTESIAN_POINT('Ctrl Pts',(-14.6240444846692,-12.5205021117526,
116.396478689841)) ;
#174132=CARTESIAN_POINT('Ctrl Pts',(-14.7155078962198,-12.3896091910669,
116.639659815513)) ;
#174133=CARTESIAN_POINT('Ctrl Pts',(-14.8155283401331,-12.3322116649338,
116.908678402663)) ;
#174134=CARTESIAN_POINT('Ctrl Pts',(-14.9160696924354,-12.3526193896652,
117.179651593861)) ;
#174135=CARTESIAN_POINT('Ctrl Pts',(-15.0126074976825,-12.4495335034968,
117.438097138294)) ;
#174136=CARTESIAN_POINT('Ctrl Pts',(-15.0977303726993,-12.6159519111974,
117.661885772396)) ;
#174137=CARTESIAN_POINT('Ctrl Pts',(-15.1663307990368,-12.8395609374739,
117.835382986547)) ;
#174138=CARTESIAN_POINT('Ctrl Pts',(-15.2143261495517,-13.1036924153161,
117.946224932861)) ;
#174139=CARTESIAN_POINT('Ctrl Pts',(-15.2392646854199,-13.3927905140901,
117.986526462558)) ;
#174140=CARTESIAN_POINT('Ctrl Pts',(-15.2397192982517,-13.6807940128297,
117.9526185938)) ;
#174141=CARTESIAN_POINT('Ctrl Pts',(-15.2167475033035,-13.9516407801447,
117.847166620473)) ;
#174142=CARTESIAN_POINT('Ctrl Pts',(-15.1722328786369,-14.1848191645832,
117.675959254401)) ;
#174143=CARTESIAN_POINT('Ctrl Pts',(-15.1111116959615,-14.3611535147467,
117.45455531879)) ;
#174144=CARTESIAN_POINT('Ctrl Pts',(-15.03716340119,-14.4717132500286,117.193678534081)) ;
#174145=CARTESIAN_POINT('Ctrl Pts',(-14.9574931202988,-14.5058049610956,
116.91556782578)) ;
#174146=CARTESIAN_POINT('Ctrl Pts',(-14.8782558620267,-14.4622432474708,
116.638782637704)) ;
#174147=CARTESIAN_POINT('Ctrl Pts',(-14.8058079691528,-14.343914063795,
116.382668771781)) ;
#174148=CARTESIAN_POINT('Ctrl Pts',(-14.7461096383968,-14.1592285094383,
116.165376277947)) ;
#174149=CARTESIAN_POINT('Ctrl Pts',(-14.7042341925757,-13.9218383285055,
116.002418128098)) ;
#174150=CARTESIAN_POINT('Ctrl Pts',(-14.6838147453501,-13.6477929587425,
115.904727451076)) ;
#174151=CARTESIAN_POINT('Ctrl Pts',(-14.6872087463539,-13.3573882946602,
115.879587299227)) ;
#174152=CARTESIAN_POINT('Ctrl Pts',(-14.7148769500706,-13.0713760146383,
115.928387341854)) ;
#174153=CARTESIAN_POINT('Ctrl Pts',(-14.7656221631295,-12.8101300373193,
116.047465559082)) ;
#174154=CARTESIAN_POINT('Ctrl Pts',(-14.836499389826,-12.5926203368979,
116.227885615043)) ;
#174155=CARTESIAN_POINT('Ctrl Pts',(-14.9232190242914,-12.4341144288436,
116.456553356206)) ;
#174156=CARTESIAN_POINT('Ctrl Pts',(-15.0204191933641,-12.346259851331,
116.717108536912)) ;
#174157=CARTESIAN_POINT('Ctrl Pts',(-15.1212516203235,-12.3348158852733,
116.98892332195)) ;
#174158=CARTESIAN_POINT('Ctrl Pts',(-15.2210253617375,-12.4019396871859,
117.257046128186)) ;
#174159=CARTESIAN_POINT('Ctrl Pts',(-15.3104774186011,-12.5400212389952,
117.494364772624)) ;
#174160=CARTESIAN_POINT('Ctrl Pts',(-15.386781464252,-12.7426569389483,
117.691155444074)) ;
#174161=CARTESIAN_POINT('Ctrl Pts',(-15.4435452552671,-12.9928209893326,
117.828633943598)) ;
#174162=CARTESIAN_POINT('Ctrl Pts',(-15.4780991318046,-13.274121349933,
117.89835399274)) ;
#174163=CARTESIAN_POINT('Ctrl Pts',(-15.4884434105682,-13.5650423075934,
117.894429498399)) ;
#174164=CARTESIAN_POINT('Ctrl Pts',(-15.4747873042015,-13.8454220244642,
117.817406765733)) ;
#174165=CARTESIAN_POINT('Ctrl Pts',(-15.4387248228193,-14.095635489283,
117.672076552588)) ;
#174166=CARTESIAN_POINT('Ctrl Pts',(-15.3836965141025,-14.2970558104585,
117.469021551389)) ;
#174167=CARTESIAN_POINT('Ctrl Pts',(-15.3141371945857,-14.4359480747077,
117.221601988843)) ;
#174168=CARTESIAN_POINT('Ctrl Pts',(-15.2359817859273,-14.501304829004,
116.948020668741)) ;
#174169=CARTESIAN_POINT('Ctrl Pts',(-15.1561240539043,-14.4893139259723,
116.669494222094)) ;
#174170=CARTESIAN_POINT('Ctrl Pts',(-15.0799694117837,-14.4004454436412,
116.401998946719)) ;
#174171=CARTESIAN_POINT('Ctrl Pts',(-15.0146075791838,-14.2418718140722,
116.167568446909)) ;
#174172=CARTESIAN_POINT('Ctrl Pts',(-14.9647824826636,-14.0233785235775,
115.98025836275)) ;
#174173=CARTESIAN_POINT('Ctrl Pts',(-14.9353130383132,-13.7618917263419,
115.855036424513)) ;
#174174=CARTESIAN_POINT('Ctrl Pts',(-14.9289325059808,-13.4754623735639,
115.800094097423)) ;
#174175=CARTESIAN_POINT('Ctrl Pts',(-14.9467156400316,-13.1862230579374,
115.818918808621)) ;
#174176=CARTESIAN_POINT('Ctrl Pts',(-14.9883696704994,-12.9121173454345,
115.910257352319)) ;
#174177=CARTESIAN_POINT('Ctrl Pts',(-15.0514075082548,-12.6748571224349,
116.066831542999)) ;
#174178=CARTESIAN_POINT('Ctrl Pts',(-15.1328444729729,-12.4898752939566,
116.279188009529)) ;
#174179=CARTESIAN_POINT('Ctrl Pts',(-15.2258152326025,-12.3730682967797,
116.527146434279)) ;
#174180=CARTESIAN_POINT('Ctrl Pts',(-15.3267957548085,-12.330125354393,
116.799022433184)) ;
#174181=CARTESIAN_POINT('Ctrl Pts',(-15.4267371080215,-12.3650026478225,
117.068234016832)) ;
#174182=CARTESIAN_POINT('Ctrl Pts',(-15.5220396277674,-12.4764750890778,
117.322748096145)) ;
#174183=CARTESIAN_POINT('Ctrl Pts',(-15.6038717305927,-12.6535586984017,
117.536764515105)) ;
#174184=CARTESIAN_POINT('Ctrl Pts',(-15.6692705920402,-12.8875907025722,
117.700299247988)) ;
#174185=CARTESIAN_POINT('Ctrl Pts',(-15.7128057696858,-13.1564738506933,
117.797702690961)) ;
#174186=CARTESIAN_POINT('Ctrl Pts',(-15.7332548587096,-13.4476180482474,
117.824312090504)) ;
#174187=CARTESIAN_POINT('Ctrl Pts',(-15.7291353924876,-13.7346448783816,
117.776350799521)) ;
#174188=CARTESIAN_POINT('Ctrl Pts',(-15.7018297830167,-13.9993799399049,
117.657715317448)) ;
#174189=CARTESIAN_POINT('Ctrl Pts',(-15.6540905337258,-14.2219559568416,
117.476929036007)) ;
#174190=CARTESIAN_POINT('Ctrl Pts',(-15.5899295337492,-14.3877271051732,
117.246044868715)) ;
#174191=CARTESIAN_POINT('Ctrl Pts',(-15.5142887883934,-14.4840522417127,
116.980008252819)) ;
#174192=CARTESIAN_POINT('Ctrl Pts',(-15.4346677192972,-14.5035551456864,
116.702251625481)) ;
#174193=CARTESIAN_POINT('Ctrl Pts',(-15.3559292275796,-14.4455933724693,
116.426856756554)) ;
#174194=CARTESIAN_POINT('Ctrl Pts',(-15.285414304366,-14.3137077173971,
116.176599635695)) ;
#174195=CARTESIAN_POINT('Ctrl Pts',(-15.2287932761951,-14.118290994482,
115.968741900664)) ;
#174196=CARTESIAN_POINT('Ctrl Pts',(-15.190662017011,-13.8721339097932,
115.817104400349)) ;
#174197=CARTESIAN_POINT('Ctrl Pts',(-15.1746169230128,-13.5943341067766,
115.732853741077)) ;
#174198=CARTESIAN_POINT('Ctrl Pts',(-15.1826673766295,-13.3016132059809,
115.721705106696)) ;
#174199=CARTESIAN_POINT('Ctrl Pts',(-15.2146933752457,-13.0203974601351,
115.783981898111)) ;
#174200=CARTESIAN_POINT('Ctrl Pts',(-15.269404025713,-12.7657619407627,
115.915129891759)) ;
#174201=CARTESIAN_POINT('Ctrl Pts',(-15.3438708491905,-12.5577255499837,
116.10637631446)) ;
#174202=CARTESIAN_POINT('Ctrl Pts',(-15.4327636159981,-12.4120606642955,
116.34175086754)) ;
#174203=CARTESIAN_POINT('Ctrl Pts',(-15.5316685213714,-12.3380220880362,
116.60734315125)) ;
#174204=CARTESIAN_POINT('Ctrl Pts',(-15.6323103361434,-12.3416277493325,
116.878663222145)) ;
#174205=CARTESIAN_POINT('Ctrl Pts',(-15.7303191792415,-12.4221117178776,
117.141642652826)) ;
#174206=CARTESIAN_POINT('Ctrl Pts',(-15.818253094992,-12.5739000669618,
117.37404115853)) ;
#174207=CARTESIAN_POINT('Ctrl Pts',(-15.8910677122169,-12.7865530350162,
117.560294460758)) ;
#174208=CARTESIAN_POINT('Ctrl Pts',(-15.943961350988,-13.044698151263,117.685874037695)) ;
#174209=CARTESIAN_POINT('Ctrl Pts',(-15.973861910085,-13.328059924083,117.741608955228)) ;
#174210=CARTESIAN_POINT('Ctrl Pts',(-15.9797490331987,-13.6187777866059,
117.724086355187)) ;
#174211=CARTESIAN_POINT('Ctrl Pts',(-15.9616058932464,-13.8959727795492,
117.633255070877)) ;
#174212=CARTESIAN_POINT('Ctrl Pts',(-15.92165968614,-14.1380897314584,117.476125293794)) ;
#174213=CARTESIAN_POINT('Ctrl Pts',(-15.8633008249773,-14.3289912800735,
117.262814844311)) ;
#174214=CARTESIAN_POINT('Ctrl Pts',(-15.7921118917969,-14.4536834307714,
117.01067142375)) ;
#174215=CARTESIAN_POINT('Ctrl Pts',(-15.7132086075603,-14.5050447602448,
116.734875307883)) ;
#174216=CARTESIAN_POINT('Ctrl Pts',(-15.6332196110999,-14.4782940097224,
116.455753006044)) ;
#174217=CARTESIAN_POINT('Ctrl Pts',(-15.5587696998728,-14.3758709565101,
116.193557985972)) ;
#174218=CARTESIAN_POINT('Ctrl Pts',(-15.4956323923376,-14.2038414128419,
115.965654894124)) ;
#174219=CARTESIAN_POINT('Ctrl Pts',(-15.4497236558171,-13.9777022974474,
115.790578372436)) ;
#174220=CARTESIAN_POINT('Ctrl Pts',(-15.4242298945828,-13.7081471730545,
115.677198196239)) ;
#174221=CARTESIAN_POINT('Ctrl Pts',(-15.4224756486748,-13.4207218926891,
115.636530543552)) ;
#174222=CARTESIAN_POINT('Ctrl Pts',(-15.4448455283626,-13.1323473586493,
115.669233043994)) ;
#174223=CARTESIAN_POINT('Ctrl Pts',(-15.4907259221535,-12.8640039527127,
115.773502605509)) ;
#174224=CARTESIAN_POINT('Ctrl Pts',(-15.5576964345495,-12.6351955964259,
115.941952413121)) ;
#174225=CARTESIAN_POINT('Ctrl Pts',(-15.6410494594336,-12.4633049543151,
116.160508256525)) ;
#174226=CARTESIAN_POINT('Ctrl Pts',(-15.73692924491,-12.3586842738095,116.416876897232)) ;
#174227=CARTESIAN_POINT('Ctrl Pts',(-15.837547597677,-12.3308701665295,
116.687989713795)) ;
#174228=CARTESIAN_POINT('Ctrl Pts',(-15.9375214249544,-12.3804185210795,
116.95704231323)) ;
#174229=CARTESIAN_POINT('Ctrl Pts',(-16.0302559090412,-12.5045865657479,
117.204009987315)) ;
#174230=CARTESIAN_POINT('Ctrl Pts',(-16.1096439036277,-12.6936012415773,
117.410410771102)) ;
#174231=CARTESIAN_POINT('Ctrl Pts',(-16.1712738995267,-12.9362801376937,
117.56247016244)) ;
#174232=CARTESIAN_POINT('Ctrl Pts',(-16.2106239956556,-13.2112926431605,
117.646987028832)) ;
#174233=CARTESIAN_POINT('Ctrl Pts',(-16.2263302334408,-13.5026318637497,
117.659280382526)) ;
#174234=CARTESIAN_POINT('Ctrl Pts',(-16.2177424879971,-13.7865927515763,
117.59774844092)) ;
#174235=CARTESIAN_POINT('Ctrl Pts',(-16.1863917194238,-14.0445932154009,
117.466837858413)) ;
#174236=CARTESIAN_POINT('Ctrl Pts',(-16.1351369456625,-14.2581092551482,
117.275260073732)) ;
#174237=CARTESIAN_POINT('Ctrl Pts',(-16.0682061521682,-14.4117380229187,
117.035830487134)) ;
#174238=CARTESIAN_POINT('Ctrl Pts',(-15.9915317982417,-14.4936441507055,
116.76682264577)) ;
#174239=CARTESIAN_POINT('Ctrl Pts',(-15.9111646098176,-14.4983888239063,
116.486541384417)) ;
#174240=CARTESIAN_POINT('Ctrl Pts',(-15.8339367194652,-14.426207251784,
116.215966892118)) ;
#174241=CARTESIAN_POINT('Ctrl Pts',(-15.7654080575456,-14.2809809264381,
115.971651595224)) ;
#174242=CARTESIAN_POINT('Ctrl Pts',(-15.7121638592197,-14.0755731076895,
115.774205354296)) ;
#174243=CARTESIAN_POINT('Ctrl Pts',(-15.6778558958867,-13.8214647968314,
115.634145099666)) ;
#174244=CARTESIAN_POINT('Ctrl Pts',(-15.6663008904224,-13.5390721929965,
115.563497706539)) ;
#174245=CARTESIAN_POINT('Ctrl Pts',(-15.6788710235298,-13.2479213210197,
115.566312381468)) ;
#174246=CARTESIAN_POINT('Ctrl Pts',(-15.7154570310451,-12.9689956696526,
115.642283838143)) ;
#174247=CARTESIAN_POINT('Ctrl Pts',(-15.7742309880506,-12.7220961737177,
115.785813685881)) ;
#174248=CARTESIAN_POINT('Ctrl Pts',(-15.8515784407682,-12.5254520180373,
115.985975276655)) ;
#174249=CARTESIAN_POINT('Ctrl Pts',(-15.94270937751,-12.3924871288094,116.22814157512)) ;
#174250=CARTESIAN_POINT('Ctrl Pts',(-16.0425166341127,-12.3327720085306,
116.496536154784)) ;
#174251=CARTESIAN_POINT('Ctrl Pts',(-16.1432965454572,-12.3509988977752,
116.768165464397)) ;
#174252=CARTESIAN_POINT('Ctrl Pts',(-16.2397734663179,-12.4453838611795,
117.026540426964)) ;
#174253=CARTESIAN_POINT('Ctrl Pts',(-16.3254447848863,-12.6100760699984,
117.251940625839)) ;
#174254=CARTESIAN_POINT('Ctrl Pts',(-16.3945559404646,-12.8316470477012,
117.427060764436)) ;
#174255=CARTESIAN_POINT('Ctrl Pts',(-16.4435312853677,-13.0973555362981,
117.540560244616)) ;
#174256=CARTESIAN_POINT('Ctrl Pts',(-16.4688621130792,-13.3829827267331,
117.582449970111)) ;
#174257=CARTESIAN_POINT('Ctrl Pts',(-16.470124542703,-13.6735145155205,
117.550719313167)) ;
#174258=CARTESIAN_POINT('Ctrl Pts',(-16.4477134830108,-13.9443960540442,
117.447059781621)) ;
#174259=CARTESIAN_POINT('Ctrl Pts',(-16.4040416496053,-14.1780473237906,
117.278577420489)) ;
#174260=CARTESIAN_POINT('Ctrl Pts',(-16.3431014881368,-14.3571729772058,
117.057559267268)) ;
#174261=CARTESIAN_POINT('Ctrl Pts',(-16.2692843220695,-14.4697035049953,
116.797034589842)) ;
#174262=CARTESIAN_POINT('Ctrl Pts',(-16.189974204939,-14.5058316151569,
116.520142021784)) ;
#174263=CARTESIAN_POINT('Ctrl Pts',(-16.1107202304642,-14.4647781183691,
116.243348321315)) ;
#174264=CARTESIAN_POINT('Ctrl Pts',(-16.03788617739,-14.3484987257117,115.986015587949)) ;
#174265=CARTESIAN_POINT('Ctrl Pts',(-15.9776687836141,-14.1655053892491,
115.767116814539)) ;
#174266=CARTESIAN_POINT('Ctrl Pts',(-15.9351536436701,-13.9286208259661,
115.602105173613)) ;
#174267=CARTESIAN_POINT('Ctrl Pts',(-15.9141622270948,-13.6565946963034,
115.502836000379)) ;
#174268=CARTESIAN_POINT('Ctrl Pts',(-15.9168400704658,-13.3650274692435,
115.475347116262)) ;
#174269=CARTESIAN_POINT('Ctrl Pts',(-15.943917468856,-13.0788343995772,
115.522370330454)) ;
#174270=CARTESIAN_POINT('Ctrl Pts',(-15.9938421820601,-12.8175211583994,
115.639074782229)) ;
#174271=CARTESIAN_POINT('Ctrl Pts',(-16.0641439891467,-12.5984995679009,
115.817749196681)) ;
#174272=CARTESIAN_POINT('Ctrl Pts',(-16.1502868270294,-12.4381081950322,
116.044719588303)) ;
#174273=CARTESIAN_POINT('Ctrl Pts',(-16.2478432903342,-12.3474840033873,
116.306149605933)) ;
#174274=CARTESIAN_POINT('Ctrl Pts',(-16.3485101468529,-12.3342746176406,
116.577507728098)) ;
#174275=CARTESIAN_POINT('Ctrl Pts',(-16.4477907403322,-12.3983523506611,
116.844372055818)) ;
#174276=CARTESIAN_POINT('Ctrl Pts',(-16.5383794781962,-12.5353914606374,
117.084853142342)) ;
#174277=CARTESIAN_POINT('Ctrl Pts',(-16.6151024200091,-12.7368848040207,
117.282902758644)) ;
#174278=CARTESIAN_POINT('Ctrl Pts',(-16.6722339594684,-12.9849643669818,
117.421634700217)) ;
#174279=CARTESIAN_POINT('Ctrl Pts',(-16.7074953741335,-13.2657001242146,
117.493501410732)) ;
#174280=CARTESIAN_POINT('Ctrl Pts',(-16.7185435095042,-13.5562446654925,
117.491765214544)) ;
#174281=CARTESIAN_POINT('Ctrl Pts',(-16.7056071827156,-13.837740260252,
117.416879374421)) ;
#174282=CARTESIAN_POINT('Ctrl Pts',(-16.6698983566585,-14.0900089023239,
117.272469305418)) ;
#174283=CARTESIAN_POINT('Ctrl Pts',(-16.615678314691,-14.2916996646196,
117.072102717414)) ;
#174284=CARTESIAN_POINT('Ctrl Pts',(-16.5462715072985,-14.4330905333239,
116.82503637481)) ;
#174285=CARTESIAN_POINT('Ctrl Pts',(-16.4684461424741,-14.5004556458798,
116.552546390901)) ;
#174286=CARTESIAN_POINT('Ctrl Pts',(-16.3884429132822,-14.4906784452632,
116.273515768952)) ;
#174287=CARTESIAN_POINT('Ctrl Pts',(-16.3122978006783,-14.4044504861589,
116.006169416252)) ;
#174288=CARTESIAN_POINT('Ctrl Pts',(-16.2460229579914,-14.2464177648016,
115.768663223049)) ;
#174289=CARTESIAN_POINT('Ctrl Pts',(-16.1959322208732,-14.0296079395376,
115.58064014647)) ;
#174290=CARTESIAN_POINT('Ctrl Pts',(-16.1659524449804,-13.7700542634679,
115.453985376571)) ;
#174291=CARTESIAN_POINT('Ctrl Pts',(-16.1588094450499,-13.4844393542531,
115.396766680954)) ;
#174292=CARTESIAN_POINT('Ctrl Pts',(-16.1759899887603,-13.1938467066394,
115.413606223146)) ;
#174293=CARTESIAN_POINT('Ctrl Pts',(-16.2169131908586,-12.9193998282655,
115.502784611301)) ;
#174294=CARTESIAN_POINT('Ctrl Pts',(-16.2798288449759,-12.679977460876,
115.658797492625)) ;
#174295=CARTESIAN_POINT('Ctrl Pts',(-16.3596321413727,-12.4956043021029,
115.866685267832)) ;
#174296=CARTESIAN_POINT('Ctrl Pts',(-16.4533735886139,-12.3751190535725,
116.11656191809)) ;
#174297=CARTESIAN_POINT('Ctrl Pts',(-16.5533514223054,-12.3303020351126,
116.385717677923)) ;
#174298=CARTESIAN_POINT('Ctrl Pts',(-16.6543061351395,-12.3631774170788,
116.657672551658)) ;
#174299=CARTESIAN_POINT('Ctrl Pts',(-16.7488808914051,-12.4713342743348,
116.91035898593)) ;
#174300=CARTESIAN_POINT('Ctrl Pts',(-16.8318207118205,-12.6476404276989,
117.12747273466)) ;
#174301=CARTESIAN_POINT('Ctrl Pts',(-16.8975001296176,-12.8790215196565,
117.292056197982)) ;
#174302=CARTESIAN_POINT('Ctrl Pts',(-16.942134561038,-13.1499133657009,
117.392426703096)) ;
#174303=CARTESIAN_POINT('Ctrl Pts',(-16.9630233535542,-13.4386144880716,
117.420658950536)) ;
#174304=CARTESIAN_POINT('Ctrl Pts',(-16.9596443378371,-13.7268235527867,
117.37484372471)) ;
#174305=CARTESIAN_POINT('Ctrl Pts',(-16.9330916364897,-13.9914324144424,
117.258649259076)) ;
#174306=CARTESIAN_POINT('Ctrl Pts',(-16.8858015410838,-14.2164140691066,
117.079108171634)) ;
#174307=CARTESIAN_POINT('Ctrl Pts',(-16.8218713013157,-14.384032579335,
116.848865519025)) ;
#174308=CARTESIAN_POINT('Ctrl Pts',(-16.7469781937031,-14.4820529544929,
116.585338242812)) ;
#174309=CARTESIAN_POINT('Ctrl Pts',(-16.6668754248099,-14.5042250600488,
116.305877110692)) ;
#174310=CARTESIAN_POINT('Ctrl Pts',(-16.5879598850496,-14.4479097103847,
116.029910236852)) ;
#174311=CARTESIAN_POINT('Ctrl Pts',(-16.5174994343308,-14.3189148106109,
115.780020371028)) ;
#174312=CARTESIAN_POINT('Ctrl Pts',(-16.4601033314479,-14.1239822238445,
115.569589941592)) ;
#174313=CARTESIAN_POINT('Ctrl Pts',(-16.4215747130303,-13.8804446676162,
115.416952493218)) ;
#174314=CARTESIAN_POINT('Ctrl Pts',(-16.4047818629355,-13.6007259227713,
115.330092652858)) ;
#174315=CARTESIAN_POINT('Ctrl Pts',(-16.4121369550956,-13.310886389785,
115.317177989403)) ;
#174316=CARTESIAN_POINT('Ctrl Pts',(-16.4435486385353,-13.0275729196668,
115.377389997303)) ;
#174317=CARTESIAN_POINT('Ctrl Pts',(-16.4978834158618,-12.7715214711428,
115.507323795441)) ;
#174318=CARTESIAN_POINT('Ctrl Pts',(-16.5717603357923,-12.5625540682405,
115.696844987537)) ;
#174319=CARTESIAN_POINT('Ctrl Pts',(-16.6600063471763,-12.4155360311479,
115.930369190556)) ;
#174320=CARTESIAN_POINT('Ctrl Pts',(-16.7583961657612,-12.339199302571,
116.194502768036)) ;
#174321=CARTESIAN_POINT('Ctrl Pts',(-16.8595422687567,-12.3403409953756,
116.467185667784)) ;
#174322=CARTESIAN_POINT('Ctrl Pts',(-16.9578689738167,-12.4190382667156,
116.731080805892)) ;
#174323=CARTESIAN_POINT('Ctrl Pts',(-17.0458999041783,-12.5685297170459,
116.963876177155)) ;
#174324=CARTESIAN_POINT('Ctrl Pts',(-17.1191748552296,-12.7793086778933,
117.151568386626)) ;
#174325=CARTESIAN_POINT('Ctrl Pts',(-17.1727252854914,-13.0361487300971,
117.279168850677)) ;
#174326=CARTESIAN_POINT('Ctrl Pts',(-17.2034288318534,-13.3199156358865,
117.337236471295)) ;
#174327=CARTESIAN_POINT('Ctrl Pts',(-17.2099599842142,-13.61053350134,117.321699031089)) ;
#174328=CARTESIAN_POINT('Ctrl Pts',(-17.1925797786754,-13.8877845324202,
117.233281417969)) ;
#174329=CARTESIAN_POINT('Ctrl Pts',(-17.1531888988296,-14.1315208949384,
117.077791857519)) ;
#174330=CARTESIAN_POINT('Ctrl Pts',(-17.0955345319982,-14.3236676354294,
116.866747533545)) ;
#174331=CARTESIAN_POINT('Ctrl Pts',(-17.0243702739968,-14.451213086268,
116.614520189238)) ;
#174332=CARTESIAN_POINT('Ctrl Pts',(-16.9454296666756,-14.5046478984509,
116.338545787343)) ;
#174333=CARTESIAN_POINT('Ctrl Pts',(-16.8656122340257,-14.4801334339684,
116.060046712965)) ;
#174334=CARTESIAN_POINT('Ctrl Pts',(-16.790980956793,-14.3800974324411,
115.797335713982)) ;
#174335=CARTESIAN_POINT('Ctrl Pts',(-16.7272992435064,-14.2097836883392,
115.567723704897)) ;
#174336=CARTESIAN_POINT('Ctrl Pts',(-16.6808108315259,-13.9844447661634,
115.3908060488)) ;
#174337=CARTESIAN_POINT('Ctrl Pts',(-16.6547738612727,-13.7175338810347,
115.275995973862)) ;
#174338=CARTESIAN_POINT('Ctrl Pts',(-16.6522344647069,-13.4290941380284,
115.232763303442)) ;
#174339=CARTESIAN_POINT('Ctrl Pts',(-16.6738872742428,-13.1407025280343,
115.263323344163)) ;
#174340=CARTESIAN_POINT('Ctrl Pts',(-16.7192914965339,-12.8707969653127,
115.366034947544)) ;
#174341=CARTESIAN_POINT('Ctrl Pts',(-16.7852951087572,-12.6417711077458,
115.53174600974)) ;
#174342=CARTESIAN_POINT('Ctrl Pts',(-16.8687385029215,-12.4670674817275,
115.750354845925)) ;
#174343=CARTESIAN_POINT('Ctrl Pts',(-16.9635606886986,-12.3610581795072,
116.003803286491)) ;
#174344=CARTESIAN_POINT('Ctrl Pts',(-17.0649420670116,-12.3304705905987,
116.27693713892)) ;
#174345=CARTESIAN_POINT('Ctrl Pts',(-17.1648109896159,-12.3780041179342,
116.545751053977)) ;
#174346=CARTESIAN_POINT('Ctrl Pts',(-17.2579372276331,-12.5002675543906,
116.79387021803)) ;
#174347=CARTESIAN_POINT('Ctrl Pts',(-17.3375779201861,-12.6872113223539,
117.001122929289)) ;
#174348=CARTESIAN_POINT('Ctrl Pts',(-17.3998316457169,-12.928470822573,
117.155087519117)) ;
#174349=CARTESIAN_POINT('Ctrl Pts',(-17.4399174994754,-13.2034657060163,
117.241757837914)) ;
#174350=CARTESIAN_POINT('Ctrl Pts',(-17.4562690855038,-13.4939400108665,
117.256107218264)) ;
#174351=CARTESIAN_POINT('Ctrl Pts',(-17.4483972852435,-13.7785749983251,
117.196730556268)) ;
#174352=CARTESIAN_POINT('Ctrl Pts',(-17.4176717828043,-14.0376123935157,
117.067726587636)) ;
#174353=CARTESIAN_POINT('Ctrl Pts',(-17.3669381628985,-14.2526152270872,
116.877737714805)) ;
#174354=CARTESIAN_POINT('Ctrl Pts',(-17.300521743148,-14.4080507138092,
116.639938676009)) ;
#174355=CARTESIAN_POINT('Ctrl Pts',(-17.2239015581171,-14.4922598223547,
116.371021974036)) ;
#174356=CARTESIAN_POINT('Ctrl Pts',(-17.1439517410193,-14.4995566650645,
116.092195902509)) ;
#174357=CARTESIAN_POINT('Ctrl Pts',(-17.0659766810491,-14.4291954268347,
115.819082015723)) ;
#174358=CARTESIAN_POINT('Ctrl Pts',(-16.9973489861747,-14.2862746553945,
115.574590132372)) ;
#174359=CARTESIAN_POINT('Ctrl Pts',(-16.943507599311,-14.0821782924177,
115.375260361907)) ;
#174360=CARTESIAN_POINT('Ctrl Pts',(-16.9086511894243,-13.8298750263426,
115.233624849604)) ;
#174361=CARTESIAN_POINT('Ctrl Pts',(-16.8963479197035,-13.5470860719876,
115.160572447035)) ;
#174362=CARTESIAN_POINT('Ctrl Pts',(-16.90824578111,-13.2560613841224,115.161364252542)) ;
#174363=CARTESIAN_POINT('Ctrl Pts',(-16.9442254493305,-12.9762949722028,
115.235455446136)) ;
#174364=CARTESIAN_POINT('Ctrl Pts',(-17.0022072372073,-12.729021213087,
115.376690040029)) ;
#174365=CARTESIAN_POINT('Ctrl Pts',(-17.0792272362676,-12.5300504685621,
115.575764889513)) ;
#174366=CARTESIAN_POINT('Ctrl Pts',(-17.1704529515286,-12.3949013412461,
115.818078836631)) ;
#174367=CARTESIAN_POINT('Ctrl Pts',(-17.2696316491355,-12.3334783627152,
116.084736767084)) ;
#174368=CARTESIAN_POINT('Ctrl Pts',(-17.3706199437548,-12.3494129205617,
116.356939612366)) ;
#174369=CARTESIAN_POINT('Ctrl Pts',(-17.4673694639669,-12.4418688951199,
116.61612522571)) ;
#174370=CARTESIAN_POINT('Ctrl Pts',(-17.5535183531139,-12.6051421932678,
116.842927305494)) ;
#174371=CARTESIAN_POINT('Ctrl Pts',(-17.6228267175663,-12.824581983231,
117.018781891196)) ;
#174372=CARTESIAN_POINT('Ctrl Pts',(-17.6723197045104,-13.0878606072953,
117.134031445032)) ;
#174373=CARTESIAN_POINT('Ctrl Pts',(-17.6985731634041,-13.3747557627756,
117.178522404017)) ;
#174374=CARTESIAN_POINT('Ctrl Pts',(-17.7004702306017,-13.6654070056361,
117.148736694593)) ;
#174375=CARTESIAN_POINT('Ctrl Pts',(-17.6787592525954,-13.9370542943595,
117.047221465574)) ;
#174376=CARTESIAN_POINT('Ctrl Pts',(-17.6354116057115,-14.1729033532404,
116.879576215049)) ;
#174377=CARTESIAN_POINT('Ctrl Pts',(-17.5750711191891,-14.3528610645483,
116.660517699246)) ;
#174378=CARTESIAN_POINT('Ctrl Pts',(-17.5017177853474,-14.4673900074207,
116.401484107417)) ;
#174379=CARTESIAN_POINT('Ctrl Pts',(-17.4223560273365,-14.5059091307987,
116.124370136875)) ;
#174380=CARTESIAN_POINT('Ctrl Pts',(-17.3429501969861,-14.467003448986,
115.847090385579)) ;
#174381=CARTESIAN_POINT('Ctrl Pts',(-17.2698268935793,-14.3526296857438,
115.58886231961)) ;
#174382=CARTESIAN_POINT('Ctrl Pts',(-17.209359096455,-14.1719531187117,
115.369308707155)) ;
#174383=CARTESIAN_POINT('Ctrl Pts',(-17.1661919090706,-13.936583984801,
115.202313468294)) ;
#174384=CARTESIAN_POINT('Ctrl Pts',(-17.1445055243567,-13.6642946874373,
115.100795313256)) ;
#174385=CARTESIAN_POINT('Ctrl Pts',(-17.1464540999734,-13.3747428455626,
115.07130654278)) ;
#174386=CARTESIAN_POINT('Ctrl Pts',(-17.1727178775642,-13.0876482903165,
115.115799669676)) ;
#174387=CARTESIAN_POINT('Ctrl Pts',(-17.2222028953257,-12.8243385253649,
115.231028671208)) ;
#174388=CARTESIAN_POINT('Ctrl Pts',(-17.2919810291401,-12.6038922563675,
115.408113946603)) ;
#174389=CARTESIAN_POINT('Ctrl Pts',(-17.3779184788419,-12.4415502102937,
115.634396370926)) ;
#174390=CARTESIAN_POINT('Ctrl Pts',(-17.4746658472938,-12.3493107874977,
115.89357675197)) ;
#174391=CARTESIAN_POINT('Ctrl Pts',(-17.5755185168944,-12.3333698024851,
116.165420915511)) ;
#174392=CARTESIAN_POINT('Ctrl Pts',(-17.6754893328123,-12.3958418590805,
116.434192181454)) ;
#174393=CARTESIAN_POINT('Ctrl Pts',(-17.7659177540856,-12.5305465195612,
116.674353272671)) ;
#174394=CARTESIAN_POINT('Ctrl Pts',(-17.8428696280429,-12.7291635452138,
116.873260297753)) ;
#174395=CARTESIAN_POINT('Ctrl Pts',(-17.900952909542,-12.9771312925897,
117.014719731031)) ;
#174396=CARTESIAN_POINT('Ctrl Pts',(-17.9368966294271,-13.2574946761857,
117.088639322891)) ;
#174397=CARTESIAN_POINT('Ctrl Pts',(-17.9486369502931,-13.5486172877669,
117.088938884935)) ;
#174398=CARTESIAN_POINT('Ctrl Pts',(-17.9363162489277,-13.8299622964239,
117.016005420011)) ;
#174399=CARTESIAN_POINT('Ctrl Pts',(-17.9015308192628,-14.082140489746,
116.874612226591)) ;
#174400=CARTESIAN_POINT('Ctrl Pts',(-17.8474297188587,-14.2871395255682,
116.67433526165)) ;
#174401=CARTESIAN_POINT('Ctrl Pts',(-17.7784858967829,-14.4298488440199,
116.428771121435)) ;
#174402=CARTESIAN_POINT('Ctrl Pts',(-17.7011619828439,-14.4994383097765,
116.157945215762)) ;
#174403=CARTESIAN_POINT('Ctrl Pts',(-17.6208255769599,-14.4922423916848,
115.877768836137)) ;
#174404=CARTESIAN_POINT('Ctrl Pts',(-17.5442238721124,-14.4074859363464,
115.60889672167)) ;
#174405=CARTESIAN_POINT('Ctrl Pts',(-17.4781148630412,-14.2527213410347,
115.372193987303)) ;
#174406=CARTESIAN_POINT('Ctrl Pts',(-17.4272659714627,-14.0372448891262,
115.181771156024)) ;
#174407=CARTESIAN_POINT('Ctrl Pts',(-17.3965606435217,-13.7782273369584,
115.052841406963)) ;
#174408=CARTESIAN_POINT('Ctrl Pts',(-17.3887643996198,-13.4921296981973,
114.993517684583)) ;
#174409=CARTESIAN_POINT('Ctrl Pts',(-17.4043330444271,-13.217409939261,
115.007409012445)) ;
#174410=CARTESIAN_POINT('Ctrl Pts',(-17.4280438693922,-13.0469696088692,
115.057750935805)) ;
#174411=CARTESIAN_POINT('Ctrl Pts',(-17.4415366461909,-12.9727494438644,
115.08882743648)) ;
#174412=CARTESIAN_POINT('',(-6.39568111142174,-13.1317299129408,118.572890161645)) ;
#174413=CARTESIAN_POINT('Origin',(-6.41836956894997,-13.1500241806476,118.641995542507)) ;
#174414=CARTESIAN_POINT('',(-6.44105802647819,-13.1683184483544,118.711100923369)) ;
#174415=CARTESIAN_POINT('Origin',(-6.41836956894997,-13.1500241806476,118.641995542507)) ;
#174416=CARTESIAN_POINT('Origin',(-6.41836956894997,-13.1500241806476,118.641995542507)) ;
#174417=CARTESIAN_POINT('Ctrl Pts',(-6.34456572554058,-13.1500241806476,
118.666226584225)) ;
#174418=CARTESIAN_POINT('Ctrl Pts',(-6.34331320628583,-13.1861488576831,
118.656365702645)) ;
#174419=CARTESIAN_POINT('Ctrl Pts',(-6.34019257639539,-13.2629207728781,
118.653629878536)) ;
#174420=CARTESIAN_POINT('Ctrl Pts',(-6.33463380664346,-13.3681754735787,
118.700728440715)) ;
#174421=CARTESIAN_POINT('Ctrl Pts',(-6.32932953020779,-13.4419954208924,
118.789585923991)) ;
#174422=CARTESIAN_POINT('Ctrl Pts',(-6.3266820427946,-13.4603090867706,
118.864513089041)) ;
#174423=CARTESIAN_POINT('Ctrl Pts',(-6.32571868123136,-13.4607127643287,
118.902106572586)) ;
#174424=CARTESIAN_POINT('Ctrl Pts',(-6.36725418306881,-13.1683184483544,
118.735331965087)) ;
#174425=CARTESIAN_POINT('Ctrl Pts',(-6.36636841296643,-13.1940059114669,
118.728126747212)) ;
#174426=CARTESIAN_POINT('Ctrl Pts',(-6.36415538975798,-13.2486867737934,
118.725794983451)) ;
#174427=CARTESIAN_POINT('Ctrl Pts',(-6.36019871534406,-13.3239058135206,
118.758824526017)) ;
#174428=CARTESIAN_POINT('Ctrl Pts',(-6.35641083129055,-13.3769362528745,
118.821760884763)) ;
#174429=CARTESIAN_POINT('Ctrl Pts',(-6.35451160798637,-13.3903536795156,
118.87504961753)) ;
#174430=CARTESIAN_POINT('Ctrl Pts',(-6.35381761696714,-13.3908270508895,
118.901830161472)) ;
#174431=CARTESIAN_POINT('Ctrl Pts',(-6.44105802647819,-13.1683184483544,
118.711100923369)) ;
#174432=CARTESIAN_POINT('Ctrl Pts',(-6.44002943016128,-13.1977103078297,
118.703455895044)) ;
#174433=CARTESIAN_POINT('Ctrl Pts',(-6.43747870841564,-13.2599976587319,
118.701985311717)) ;
#174434=CARTESIAN_POINT('Ctrl Pts',(-6.43296369962062,-13.3449026924378,
118.741207405795)) ;
#174435=CARTESIAN_POINT('Ctrl Pts',(-6.4286795521859,-13.4039111623081,
118.813989174412)) ;
#174436=CARTESIAN_POINT('Ctrl Pts',(-6.42655805213203,-13.4180394153483,
118.874932709186)) ;
#174437=CARTESIAN_POINT('Ctrl Pts',(-6.42579176677498,-13.4180036036418,
118.905424525735)) ;
#174438=CARTESIAN_POINT('Ctrl Pts',(-6.51486186988758,-13.1683184483544,
118.686869881651)) ;
#174439=CARTESIAN_POINT('Ctrl Pts',(-6.51369044735612,-13.2014147041926,
118.678785042876)) ;
#174440=CARTESIAN_POINT('Ctrl Pts',(-6.5108020270733,-13.2713085436704,
118.678175639983)) ;
#174441=CARTESIAN_POINT('Ctrl Pts',(-6.50572868389717,-13.365899571355,
118.723590285574)) ;
#174442=CARTESIAN_POINT('Ctrl Pts',(-6.50094827308125,-13.4308860717416,
118.806217464061)) ;
#174443=CARTESIAN_POINT('Ctrl Pts',(-6.49860449627767,-13.4457251511809,
118.874815800842)) ;
#174444=CARTESIAN_POINT('Ctrl Pts',(-6.49776591658281,-13.445180156394,
118.909018889999)) ;
#174445=CARTESIAN_POINT('Ctrl Pts',(-6.49217341235936,-13.1500241806476,
118.617764500789)) ;
#174446=CARTESIAN_POINT('Ctrl Pts',(-6.49063524067551,-13.1935576504088,
118.607023998309)) ;
#174447=CARTESIAN_POINT('Ctrl Pts',(-6.48683921371072,-13.2855425427551,
118.606010535068)) ;
#174448=CARTESIAN_POINT('Ctrl Pts',(-6.48016377519658,-13.4101692314131,
118.665494200272)) ;
#174449=CARTESIAN_POINT('Ctrl Pts',(-6.47386697199849,-13.4959452397595,
118.774042503289)) ;
#174450=CARTESIAN_POINT('Ctrl Pts',(-6.4707749310859,-13.515680558436,118.864279272352)) ;
#174451=CARTESIAN_POINT('Ctrl Pts',(-6.46966698084703,-13.5150658698332,
118.909295301113)) ;
#174452=CARTESIAN_POINT('Ctrl Pts',(-6.46948495483114,-13.1317299129408,
118.548659119927)) ;
#174453=CARTESIAN_POINT('Ctrl Pts',(-6.4675800339949,-13.185700596625,118.535262953743)) ;
#174454=CARTESIAN_POINT('Ctrl Pts',(-6.46287640034814,-13.2997765418398,
118.533845430152)) ;
#174455=CARTESIAN_POINT('Ctrl Pts',(-6.45459886649599,-13.4544388914713,
118.60739811497)) ;
#174456=CARTESIAN_POINT('Ctrl Pts',(-6.44678567091572,-13.5610044077774,
118.741867542516)) ;
#174457=CARTESIAN_POINT('Ctrl Pts',(-6.44294536589413,-13.585635965691,
118.853742743863)) ;
#174458=CARTESIAN_POINT('Ctrl Pts',(-6.44156804511125,-13.5849515832724,
118.909571712227)) ;
#174459=CARTESIAN_POINT('Ctrl Pts',(-6.39568111142176,-13.1317299129408,
118.572890161645)) ;
#174460=CARTESIAN_POINT('Ctrl Pts',(-6.39391901680005,-13.1819962002622,
118.559933805911)) ;
#174461=CARTESIAN_POINT('Ctrl Pts',(-6.38955308169047,-13.2884656569013,
118.557655101886)) ;
#174462=CARTESIAN_POINT('Ctrl Pts',(-6.38183388221942,-13.433442012554,
118.625015235192)) ;
#174463=CARTESIAN_POINT('Ctrl Pts',(-6.37451695002037,-13.5340294983438,
118.749639252867)) ;
#174464=CARTESIAN_POINT('Ctrl Pts',(-6.37089892174848,-13.5579502298583,
118.853859652207)) ;
#174465=CARTESIAN_POINT('Ctrl Pts',(-6.36959389530342,-13.5577750305201,
118.905977347964)) ;
#174466=CARTESIAN_POINT('Ctrl Pts',(-6.32187726801236,-13.1317299129408,
118.597121203363)) ;
#174467=CARTESIAN_POINT('Ctrl Pts',(-6.32025799960521,-13.1782918038993,
118.584604658079)) ;
#174468=CARTESIAN_POINT('Ctrl Pts',(-6.31622976303281,-13.2771547719628,
118.58146477362)) ;
#174469=CARTESIAN_POINT('Ctrl Pts',(-6.30906889794287,-13.4124451336368,
118.642632355413)) ;
#174470=CARTESIAN_POINT('Ctrl Pts',(-6.30224822912501,-13.5070545889103,
118.757410963219)) ;
#174471=CARTESIAN_POINT('Ctrl Pts',(-6.29885247760283,-13.5302644940257,
118.853976560551)) ;
#174472=CARTESIAN_POINT('Ctrl Pts',(-6.29761974549558,-13.5305984777679,
118.9023829837)) ;
#174473=CARTESIAN_POINT('Ctrl Pts',(-6.34456572554058,-13.1500241806476,
118.666226584225)) ;
#174474=CARTESIAN_POINT('Ctrl Pts',(-6.34331320628583,-13.1861488576831,
118.656365702645)) ;
#174475=CARTESIAN_POINT('Ctrl Pts',(-6.34019257639539,-13.2629207728781,
118.653629878536)) ;
#174476=CARTESIAN_POINT('Ctrl Pts',(-6.33463380664346,-13.3681754735787,
118.700728440715)) ;
#174477=CARTESIAN_POINT('Ctrl Pts',(-6.32932953020779,-13.4419954208924,
118.789585923991)) ;
#174478=CARTESIAN_POINT('Ctrl Pts',(-6.3266820427946,-13.4603090867706,
118.864513089041)) ;
#174479=CARTESIAN_POINT('Ctrl Pts',(-6.32571868123136,-13.4607127643287,
118.902106572586)) ;
#174480=CARTESIAN_POINT('',(-6.32571868123136,-13.4607127643287,118.902106572586)) ;
#174481=CARTESIAN_POINT('Ctrl Pts',(-6.34456572554058,-13.1500241806476,
118.666226584225)) ;
#174482=CARTESIAN_POINT('Ctrl Pts',(-6.34331320628583,-13.1861488576831,
118.656365702645)) ;
#174483=CARTESIAN_POINT('Ctrl Pts',(-6.34019257639539,-13.2629207728781,
118.653629878536)) ;
#174484=CARTESIAN_POINT('Ctrl Pts',(-6.33463380664346,-13.3681754735787,
118.700728440715)) ;
#174485=CARTESIAN_POINT('Ctrl Pts',(-6.32932953020779,-13.4419954208924,
118.789585923991)) ;
#174486=CARTESIAN_POINT('Ctrl Pts',(-6.3266820427946,-13.4603090867706,
118.864513089041)) ;
#174487=CARTESIAN_POINT('Ctrl Pts',(-6.32571868123136,-13.4607127643287,
118.902106572586)) ;
#174488=CARTESIAN_POINT('Origin',(-6.39769283103919,-13.4878893170809,118.905700936849)) ;
#174489=CARTESIAN_POINT('Ctrl Pts',(-6.32571868123136,-13.4607127643287,
118.902106572586)) ;
#174490=CARTESIAN_POINT('Ctrl Pts',(-6.31605107706768,-13.4607136600768,
119.285257587653)) ;
#174491=CARTESIAN_POINT('Ctrl Pts',(-6.30638347290399,-13.460714555825,
119.668408602719)) ;
#174492=CARTESIAN_POINT('Ctrl Pts',(-6.29671586874031,-13.4607154515732,
120.051559617786)) ;
#174493=CARTESIAN_POINT('Ctrl Pts',(-6.35381761696714,-13.3908270508895,
118.901830161472)) ;
#174494=CARTESIAN_POINT('Ctrl Pts',(-6.34415001280346,-13.3908279466377,
119.284981176539)) ;
#174495=CARTESIAN_POINT('Ctrl Pts',(-6.33448240863977,-13.3908288423858,
119.668132191605)) ;
#174496=CARTESIAN_POINT('Ctrl Pts',(-6.32481480447609,-13.390829738134,
120.051283206672)) ;
#174497=CARTESIAN_POINT('Ctrl Pts',(-6.42579176677498,-13.4180036036418,
118.905424525735)) ;
#174498=CARTESIAN_POINT('Ctrl Pts',(-6.41612416261129,-13.4180044993899,
119.288575540802)) ;
#174499=CARTESIAN_POINT('Ctrl Pts',(-6.4064565584476,-13.4180053951381,
119.671726555869)) ;
#174500=CARTESIAN_POINT('Ctrl Pts',(-6.39678895428392,-13.4180062908863,
120.054877570935)) ;
#174501=CARTESIAN_POINT('Ctrl Pts',(-6.49776591658281,-13.445180156394,
118.909018889999)) ;
#174502=CARTESIAN_POINT('Ctrl Pts',(-6.48809831241913,-13.4451810521422,
119.292169905065)) ;
#174503=CARTESIAN_POINT('Ctrl Pts',(-6.47843070825543,-13.4451819478904,
119.675320920132)) ;
#174504=CARTESIAN_POINT('Ctrl Pts',(-6.46876310409176,-13.4451828436386,
120.058471935199)) ;
#174505=CARTESIAN_POINT('Ctrl Pts',(-6.46966698084703,-13.5150658698332,
118.909295301113)) ;
#174506=CARTESIAN_POINT('Ctrl Pts',(-6.45999937668335,-13.5150667655814,
119.29244631618)) ;
#174507=CARTESIAN_POINT('Ctrl Pts',(-6.45033177251965,-13.5150676613296,
119.675597331246)) ;
#174508=CARTESIAN_POINT('Ctrl Pts',(-6.44066416835598,-13.5150685570778,
120.058748346313)) ;
#174509=CARTESIAN_POINT('Ctrl Pts',(-6.44156804511125,-13.5849515832724,
118.909571712227)) ;
#174510=CARTESIAN_POINT('Ctrl Pts',(-6.43190044094756,-13.5849524790206,
119.292722727294)) ;
#174511=CARTESIAN_POINT('Ctrl Pts',(-6.42223283678388,-13.5849533747688,
119.67587374236)) ;
#174512=CARTESIAN_POINT('Ctrl Pts',(-6.4125652326202,-13.5849542705169,
120.059024757427)) ;
#174513=CARTESIAN_POINT('Ctrl Pts',(-6.36959389530342,-13.5577750305201,
118.905977347964)) ;
#174514=CARTESIAN_POINT('Ctrl Pts',(-6.35992629113973,-13.5577759262683,
119.28912836303)) ;
#174515=CARTESIAN_POINT('Ctrl Pts',(-6.35025868697604,-13.5577768220165,
119.672279378097)) ;
#174516=CARTESIAN_POINT('Ctrl Pts',(-6.34059108281237,-13.5577777177647,
120.055430393163)) ;
#174517=CARTESIAN_POINT('Ctrl Pts',(-6.29761974549558,-13.5305984777679,
118.9023829837)) ;
#174518=CARTESIAN_POINT('Ctrl Pts',(-6.2879521413319,-13.530599373516,119.285533998767)) ;
#174519=CARTESIAN_POINT('Ctrl Pts',(-6.2782845371682,-13.5306002692642,
119.668685013833)) ;
#174520=CARTESIAN_POINT('Ctrl Pts',(-6.26861693300453,-13.5306011650124,
120.0518360289)) ;
#174521=CARTESIAN_POINT('Ctrl Pts',(-6.32571868123136,-13.4607127643287,
118.902106572586)) ;
#174522=CARTESIAN_POINT('Ctrl Pts',(-6.31605107706768,-13.4607136600768,
119.285257587653)) ;
#174523=CARTESIAN_POINT('Ctrl Pts',(-6.30638347290399,-13.460714555825,
119.668408602719)) ;
#174524=CARTESIAN_POINT('Ctrl Pts',(-6.29671586874031,-13.4607154515732,
120.051559617786)) ;
#174525=CARTESIAN_POINT('',(-6.29671586874031,-13.4607154515732,120.051559617786)) ;
#174526=CARTESIAN_POINT('',(-6.32571868123136,-13.4607127643287,118.902106572586)) ;
#174527=CARTESIAN_POINT('',(-6.36858491589695,-13.562875855635,120.056714214132)) ;
#174528=CARTESIAN_POINT('Origin',(-6.36869001854814,-13.4878920043255,120.055153982049)) ;
#174529=CARTESIAN_POINT('',(-6.36879525992063,-13.4129081530202,120.053593755801)) ;
#174530=CARTESIAN_POINT('Origin',(-6.36869001854814,-13.4878920043255,120.055153982049)) ;
#174531=CARTESIAN_POINT('Origin',(-6.36869001854814,-13.4878920043255,120.055153982049)) ;
#174532=CARTESIAN_POINT('Ctrl Pts',(-6.29671586874031,-13.4607154515732,
120.051559617786)) ;
#174533=CARTESIAN_POINT('Ctrl Pts',(-6.28976012863649,-13.4607154515732,
120.117372634366)) ;
#174534=CARTESIAN_POINT('Ctrl Pts',(-6.25432280440511,-13.4607154515732,
120.250618929773)) ;
#174535=CARTESIAN_POINT('Ctrl Pts',(-6.140310678484,-13.4607154515732,120.428143665408)) ;
#174536=CARTESIAN_POINT('Ctrl Pts',(-5.97568444568715,-13.4607154515732,
120.563316664804)) ;
#174537=CARTESIAN_POINT('Ctrl Pts',(-5.78097860437995,-13.4607154515732,
120.642680062699)) ;
#174538=CARTESIAN_POINT('Ctrl Pts',(-5.57200742713837,-13.4607154515732,
120.662582212011)) ;
#174539=CARTESIAN_POINT('Ctrl Pts',(-5.36445339342349,-13.4607154515732,
120.618928922871)) ;
#174540=CARTESIAN_POINT('Ctrl Pts',(-5.18265709814504,-13.4607154515732,
120.514149932282)) ;
#174541=CARTESIAN_POINT('Ctrl Pts',(-5.04597897894181,-13.4607154515732,
120.362468390451)) ;
#174542=CARTESIAN_POINT('Ctrl Pts',(-4.96280251429834,-13.4607154515732,
120.177172641054)) ;
#174543=CARTESIAN_POINT('Ctrl Pts',(-4.94189991062264,-13.4607154515732,
119.97127049429)) ;
#174544=CARTESIAN_POINT('Ctrl Pts',(-4.98833964154144,-13.4607154515732,
119.767982106043)) ;
#174545=CARTESIAN_POINT('Ctrl Pts',(-5.09419415993757,-13.4607154515732,
119.590012717272)) ;
#174546=CARTESIAN_POINT('Ctrl Pts',(-5.24909308706152,-13.4607154515732,
119.449653557218)) ;
#174547=CARTESIAN_POINT('Ctrl Pts',(-5.44305976208226,-13.4607154515732,
119.359449641273)) ;
#174548=CARTESIAN_POINT('Ctrl Pts',(-5.65504200079475,-13.4607154515732,
119.332086511174)) ;
#174549=CARTESIAN_POINT('Ctrl Pts',(-5.7931791132922,-13.4607154515732,
119.35624483207)) ;
#174550=CARTESIAN_POINT('Ctrl Pts',(-5.85699395434883,-13.4607154515732,
119.377580402306)) ;
#174551=CARTESIAN_POINT('Ctrl Pts',(-6.32481480447609,-13.390829738134,
120.051283206672)) ;
#174552=CARTESIAN_POINT('Ctrl Pts',(-6.31782971791387,-13.390829738134,
120.119848720537)) ;
#174553=CARTESIAN_POINT('Ctrl Pts',(-6.28144487665748,-13.390829738134,
120.258747479054)) ;
#174554=CARTESIAN_POINT('Ctrl Pts',(-6.16339232015985,-13.390829738134,
120.444052341949)) ;
#174555=CARTESIAN_POINT('Ctrl Pts',(-5.99245343202574,-13.390829738134,
120.585439812146)) ;
#174556=CARTESIAN_POINT('Ctrl Pts',(-5.78996355328214,-13.390829738134,
120.668817841647)) ;
#174557=CARTESIAN_POINT('Ctrl Pts',(-5.57238022299922,-13.390829738134,
120.690324475555)) ;
#174558=CARTESIAN_POINT('Ctrl Pts',(-5.35602195824038,-13.390829738134,
120.6456373742)) ;
#174559=CARTESIAN_POINT('Ctrl Pts',(-5.16625123437035,-13.390829738134,
120.53719608567)) ;
#174560=CARTESIAN_POINT('Ctrl Pts',(-5.02328983170725,-13.390829738134,
120.379740742889)) ;
#174561=CARTESIAN_POINT('Ctrl Pts',(-4.93592236622143,-13.390829738134,
120.187078915218)) ;
#174562=CARTESIAN_POINT('Ctrl Pts',(-4.91333724036518,-13.390829738134,
119.972724565564)) ;
#174563=CARTESIAN_POINT('Ctrl Pts',(-4.9609054258806,-13.390829738134,119.760840908715)) ;
#174564=CARTESIAN_POINT('Ctrl Pts',(-5.07045935759837,-13.390829738134,
119.575103418979)) ;
#174565=CARTESIAN_POINT('Ctrl Pts',(-5.23124591495442,-13.390829738134,
119.428351239574)) ;
#174566=CARTESIAN_POINT('Ctrl Pts',(-5.43292307170264,-13.390829738134,
119.333686344338)) ;
#174567=CARTESIAN_POINT('Ctrl Pts',(-5.65361322097818,-13.390829738134,
119.304398393744)) ;
#174568=CARTESIAN_POINT('Ctrl Pts',(-5.79759063622383,-13.390829738134,
119.329041972343)) ;
#174569=CARTESIAN_POINT('Ctrl Pts',(-5.86414369407748,-13.390829738134,
119.351023259812)) ;
#174570=CARTESIAN_POINT('Ctrl Pts',(-6.39678895428392,-13.4180062908863,
120.054877570935)) ;
#174571=CARTESIAN_POINT('Ctrl Pts',(-6.38928263696362,-13.4180062908863,
120.130502647309)) ;
#174572=CARTESIAN_POINT('Ctrl Pts',(-6.34955616782122,-13.4180062908863,
120.28376286067)) ;
#174573=CARTESIAN_POINT('Ctrl Pts',(-6.21989971795512,-13.4180062908863,
120.488415929437)) ;
#174574=CARTESIAN_POINT('Ctrl Pts',(-6.03179411045853,-13.4180062908863,
120.644785453841)) ;
#174575=CARTESIAN_POINT('Ctrl Pts',(-5.80872751617359,-13.4180062908863,
120.737274468594)) ;
#174576=CARTESIAN_POINT('Ctrl Pts',(-5.56883823195218,-13.4180062908863,
120.76157980652)) ;
#174577=CARTESIAN_POINT('Ctrl Pts',(-5.33010991940545,-13.4180062908863,
120.712891018481)) ;
#174578=CARTESIAN_POINT('Ctrl Pts',(-5.12051933501212,-13.4180062908863,
120.593829347392)) ;
#174579=CARTESIAN_POINT('Ctrl Pts',(-4.96240938664547,-13.4180062908863,
120.42059364654)) ;
#174580=CARTESIAN_POINT('Ctrl Pts',(-4.8655073932878,-13.4180062908863,
120.208385475096)) ;
#174581=CARTESIAN_POINT('Ctrl Pts',(-4.8399851269984,-13.4180062908863,
119.972081541481)) ;
#174582=CARTESIAN_POINT('Ctrl Pts',(-4.89183506722446,-13.4180062908863,
119.738311675287)) ;
#174583=CARTESIAN_POINT('Ctrl Pts',(-5.0121179866212,-13.4180062908863,
119.533204612542)) ;
#174584=CARTESIAN_POINT('Ctrl Pts',(-5.18901219649234,-13.4180062908863,
119.370947050179)) ;
#174585=CARTESIAN_POINT('Ctrl Pts',(-5.41115011774361,-13.4180062908863,
119.266014389055)) ;
#174586=CARTESIAN_POINT('Ctrl Pts',(-5.65444326492148,-13.4180062908863,
119.233120285394)) ;
#174587=CARTESIAN_POINT('Ctrl Pts',(-5.81329239186224,-13.4180062908863,
119.259903763088)) ;
#174588=CARTESIAN_POINT('Ctrl Pts',(-5.88675024835855,-13.4180062908863,
119.283961627338)) ;
#174589=CARTESIAN_POINT('Ctrl Pts',(-6.46876310409176,-13.4451828436386,
120.058471935199)) ;
#174590=CARTESIAN_POINT('Ctrl Pts',(-6.46073555601338,-13.4451828436386,
120.141156574081)) ;
#174591=CARTESIAN_POINT('Ctrl Pts',(-6.41766745898496,-13.4451828436386,
120.308778242286)) ;
#174592=CARTESIAN_POINT('Ctrl Pts',(-6.27640711575039,-13.4451828436386,
120.532779516925)) ;
#174593=CARTESIAN_POINT('Ctrl Pts',(-6.07113478889131,-13.4451828436386,
120.704131095535)) ;
#174594=CARTESIAN_POINT('Ctrl Pts',(-5.82749147906504,-13.4451828436386,
120.805731095541)) ;
#174595=CARTESIAN_POINT('Ctrl Pts',(-5.56529624090513,-13.4451828436386,
120.832835137485)) ;
#174596=CARTESIAN_POINT('Ctrl Pts',(-5.30419788057051,-13.4451828436386,
120.780144662762)) ;
#174597=CARTESIAN_POINT('Ctrl Pts',(-5.07478743565387,-13.4451828436386,
120.650462609113)) ;
#174598=CARTESIAN_POINT('Ctrl Pts',(-4.90152894158368,-13.4451828436386,
120.461446550191)) ;
#174599=CARTESIAN_POINT('Ctrl Pts',(-4.79509242035417,-13.4451828436386,
120.229692034974)) ;
#174600=CARTESIAN_POINT('Ctrl Pts',(-4.76663301363163,-13.4451828436386,
119.971438517398)) ;
#174601=CARTESIAN_POINT('Ctrl Pts',(-4.82276470856832,-13.4451828436386,
119.71578244186)) ;
#174602=CARTESIAN_POINT('Ctrl Pts',(-4.95377661564404,-13.4451828436386,
119.491305806106)) ;
#174603=CARTESIAN_POINT('Ctrl Pts',(-5.14677847803024,-13.4451828436386,
119.313542860783)) ;
#174604=CARTESIAN_POINT('Ctrl Pts',(-5.38937716378458,-13.4451828436386,
119.198342433773)) ;
#174605=CARTESIAN_POINT('Ctrl Pts',(-5.6552733088648,-13.4451828436386,
119.161842177043)) ;
#174606=CARTESIAN_POINT('Ctrl Pts',(-5.82899414750066,-13.4451828436386,
119.190765553834)) ;
#174607=CARTESIAN_POINT('Ctrl Pts',(-5.90935680263961,-13.4451828436386,
119.216899994865)) ;
#174608=CARTESIAN_POINT('Ctrl Pts',(-6.44066416835598,-13.5150685570778,
120.058748346313)) ;
#174609=CARTESIAN_POINT('Ctrl Pts',(-6.43266596673601,-13.5150685570778,
120.13868048791)) ;
#174610=CARTESIAN_POINT('Ctrl Pts',(-6.39054538673258,-13.5150685570778,
120.300649693005)) ;
#174611=CARTESIAN_POINT('Ctrl Pts',(-6.25332547407455,-13.5150685570778,
120.516870840384)) ;
#174612=CARTESIAN_POINT('Ctrl Pts',(-6.05436580255273,-13.5150685570778,
120.682007948193)) ;
#174613=CARTESIAN_POINT('Ctrl Pts',(-5.81850653016284,-13.5150685570778,
120.779593316593)) ;
#174614=CARTESIAN_POINT('Ctrl Pts',(-5.56492344504428,-13.5150685570778,
120.805092873941)) ;
#174615=CARTESIAN_POINT('Ctrl Pts',(-5.31262931575362,-13.5150685570778,
120.753436211433)) ;
#174616=CARTESIAN_POINT('Ctrl Pts',(-5.09119329942855,-13.5150685570778,
120.627416455725)) ;
#174617=CARTESIAN_POINT('Ctrl Pts',(-4.92421808881825,-13.5150685570778,
120.444174197752)) ;
#174618=CARTESIAN_POINT('Ctrl Pts',(-4.82197256843109,-13.5150685570778,
120.219785760809)) ;
#174619=CARTESIAN_POINT('Ctrl Pts',(-4.79519568388909,-13.5150685570778,
119.969984446124)) ;
#174620=CARTESIAN_POINT('Ctrl Pts',(-4.85019892422917,-13.5150685570778,
119.722923639187)) ;
#174621=CARTESIAN_POINT('Ctrl Pts',(-4.97751141798325,-13.5150685570778,
119.5062151044)) ;
#174622=CARTESIAN_POINT('Ctrl Pts',(-5.16462565013734,-13.5150685570778,
119.334845178426)) ;
#174623=CARTESIAN_POINT('Ctrl Pts',(-5.39951385416421,-13.5150685570778,
119.224105730708)) ;
#174624=CARTESIAN_POINT('Ctrl Pts',(-5.65670208868136,-13.5150685570778,
119.189530294473)) ;
#174625=CARTESIAN_POINT('Ctrl Pts',(-5.82458262456902,-13.5150685570778,
119.21796841356)) ;
#174626=CARTESIAN_POINT('Ctrl Pts',(-5.90220706291095,-13.5150685570778,
119.243457137359)) ;
#174627=CARTESIAN_POINT('Ctrl Pts',(-6.4125652326202,-13.5849542705169,
120.059024757427)) ;
#174628=CARTESIAN_POINT('Ctrl Pts',(-6.40459637745865,-13.5849542705169,
120.136204401739)) ;
#174629=CARTESIAN_POINT('Ctrl Pts',(-6.3634233144802,-13.5849542705169,
120.292521143724)) ;
#174630=CARTESIAN_POINT('Ctrl Pts',(-6.23024383239871,-13.5849542705169,
120.500962163843)) ;
#174631=CARTESIAN_POINT('Ctrl Pts',(-6.03759681621414,-13.5849542705169,
120.659884800851)) ;
#174632=CARTESIAN_POINT('Ctrl Pts',(-5.80952158126064,-13.5849542705169,
120.753455537645)) ;
#174633=CARTESIAN_POINT('Ctrl Pts',(-5.56455064918341,-13.5849542705169,
120.777350610398)) ;
#174634=CARTESIAN_POINT('Ctrl Pts',(-5.32106075093673,-13.5849542705169,
120.726727760105)) ;
#174635=CARTESIAN_POINT('Ctrl Pts',(-5.10759916320323,-13.5849542705169,
120.604370302337)) ;
#174636=CARTESIAN_POINT('Ctrl Pts',(-4.94690723605281,-13.5849542705169,
120.426901845314)) ;
#174637=CARTESIAN_POINT('Ctrl Pts',(-4.848852716508,-13.5849542705169,120.209879486644)) ;
#174638=CARTESIAN_POINT('Ctrl Pts',(-4.82375835414656,-13.5849542705169,
119.96853037485)) ;
#174639=CARTESIAN_POINT('Ctrl Pts',(-4.87763313989,-13.5849542705169,119.730064836515)) ;
#174640=CARTESIAN_POINT('Ctrl Pts',(-5.00124622032246,-13.5849542705169,
119.521124402693)) ;
#174641=CARTESIAN_POINT('Ctrl Pts',(-5.18247282224443,-13.5849542705169,
119.356147496069)) ;
#174642=CARTESIAN_POINT('Ctrl Pts',(-5.40965054454383,-13.5849542705169,
119.249869027643)) ;
#174643=CARTESIAN_POINT('Ctrl Pts',(-5.65813086849792,-13.5849542705169,
119.217218411902)) ;
#174644=CARTESIAN_POINT('Ctrl Pts',(-5.82017110163739,-13.5849542705169,
119.245171273287)) ;
#174645=CARTESIAN_POINT('Ctrl Pts',(-5.89505732318229,-13.5849542705169,
119.270014279853)) ;
#174646=CARTESIAN_POINT('Ctrl Pts',(-6.34059108281237,-13.5577777177647,
120.055430393163)) ;
#174647=CARTESIAN_POINT('Ctrl Pts',(-6.33314345840889,-13.5577777177647,
120.125550474967)) ;
#174648=CARTESIAN_POINT('Ctrl Pts',(-6.29531202331647,-13.5577777177647,
120.267505762107)) ;
#174649=CARTESIAN_POINT('Ctrl Pts',(-6.17373643460343,-13.5577777177647,
120.456598576355)) ;
#174650=CARTESIAN_POINT('Ctrl Pts',(-5.99825613778136,-13.5577777177647,
120.600539159156)) ;
#174651=CARTESIAN_POINT('Ctrl Pts',(-5.7907576183692,-13.5577777177647,
120.684998910698)) ;
#174652=CARTESIAN_POINT('Ctrl Pts',(-5.56809264023046,-13.5577777177647,
120.706095279433)) ;
#174653=CARTESIAN_POINT('Ctrl Pts',(-5.34697278977167,-13.5577777177647,
120.659474115823)) ;
#174654=CARTESIAN_POINT('Ctrl Pts',(-5.15333106256147,-13.5577777177647,
120.547737040615)) ;
#174655=CARTESIAN_POINT('Ctrl Pts',(-5.0077876811146,-13.5577777177647,
120.386048941664)) ;
#174656=CARTESIAN_POINT('Ctrl Pts',(-4.91926768944164,-13.5577777177647,
120.188572926766)) ;
#174657=CARTESIAN_POINT('Ctrl Pts',(-4.89711046751333,-13.5577777177647,
119.969173398933)) ;
#174658=CARTESIAN_POINT('Ctrl Pts',(-4.94670349854615,-13.5577777177647,
119.752594069943)) ;
#174659=CARTESIAN_POINT('Ctrl Pts',(-5.05958759129963,-13.5577777177647,
119.563023209129)) ;
#174660=CARTESIAN_POINT('Ctrl Pts',(-5.22470654070653,-13.5577777177647,
119.413551685465)) ;
#174661=CARTESIAN_POINT('Ctrl Pts',(-5.43142349850286,-13.5577777177647,
119.317540982926)) ;
#174662=CARTESIAN_POINT('Ctrl Pts',(-5.65730082455462,-13.5577777177647,
119.288496520253)) ;
#174663=CARTESIAN_POINT('Ctrl Pts',(-5.80446934599897,-13.5577777177647,
119.314309482542)) ;
#174664=CARTESIAN_POINT('Ctrl Pts',(-5.87245076890124,-13.5577777177647,
119.337075912327)) ;
#174665=CARTESIAN_POINT('Ctrl Pts',(-6.26861693300453,-13.5306011650124,
120.0518360289)) ;
#174666=CARTESIAN_POINT('Ctrl Pts',(-6.26169053935913,-13.5306011650124,
120.114896548195)) ;
#174667=CARTESIAN_POINT('Ctrl Pts',(-6.22720073215273,-13.5306011650124,
120.242490380491)) ;
#174668=CARTESIAN_POINT('Ctrl Pts',(-6.11722903680817,-13.5306011650124,
120.412234988866)) ;
#174669=CARTESIAN_POINT('Ctrl Pts',(-5.95891545934857,-13.5306011650124,
120.541193517462)) ;
#174670=CARTESIAN_POINT('Ctrl Pts',(-5.77199365547776,-13.5306011650124,
120.616542283751)) ;
#174671=CARTESIAN_POINT('Ctrl Pts',(-5.57163463127751,-13.5306011650124,
120.634839948468)) ;
#174672=CARTESIAN_POINT('Ctrl Pts',(-5.37288482860661,-13.5306011650124,
120.592220471542)) ;
#174673=CARTESIAN_POINT('Ctrl Pts',(-5.19906296191971,-13.5306011650124,
120.491103778893)) ;
#174674=CARTESIAN_POINT('Ctrl Pts',(-5.06866812617638,-13.5306011650124,
120.345196038013)) ;
#174675=CARTESIAN_POINT('Ctrl Pts',(-4.98968266237526,-13.5306011650124,
120.167266366889)) ;
#174676=CARTESIAN_POINT('Ctrl Pts',(-4.9704625808801,-13.5306011650124,
119.969816423016)) ;
#174677=CARTESIAN_POINT('Ctrl Pts',(-5.01577385720228,-13.5306011650124,
119.77512330337)) ;
#174678=CARTESIAN_POINT('Ctrl Pts',(-5.11792896227678,-13.5306011650124,
119.604922015565)) ;
#174679=CARTESIAN_POINT('Ctrl Pts',(-5.26694025916861,-13.5306011650124,
119.470955874861)) ;
#174680=CARTESIAN_POINT('Ctrl Pts',(-5.45319645246189,-13.5306011650124,
119.385212938208)) ;
#174681=CARTESIAN_POINT('Ctrl Pts',(-5.6564707806113,-13.5306011650124,
119.359774628604)) ;
#174682=CARTESIAN_POINT('Ctrl Pts',(-5.78876759036056,-13.5306011650124,
119.383447691797)) ;
#174683=CARTESIAN_POINT('Ctrl Pts',(-5.84984421462017,-13.5306011650124,
119.4041375448)) ;
#174684=CARTESIAN_POINT('Ctrl Pts',(-6.29671586874031,-13.4607154515732,
120.051559617786)) ;
#174685=CARTESIAN_POINT('Ctrl Pts',(-6.28976012863649,-13.4607154515732,
120.117372634366)) ;
#174686=CARTESIAN_POINT('Ctrl Pts',(-6.25432280440511,-13.4607154515732,
120.250618929773)) ;
#174687=CARTESIAN_POINT('Ctrl Pts',(-6.140310678484,-13.4607154515732,120.428143665408)) ;
#174688=CARTESIAN_POINT('Ctrl Pts',(-5.97568444568715,-13.4607154515732,
120.563316664804)) ;
#174689=CARTESIAN_POINT('Ctrl Pts',(-5.78097860437995,-13.4607154515732,
120.642680062699)) ;
#174690=CARTESIAN_POINT('Ctrl Pts',(-5.57200742713837,-13.4607154515732,
120.662582212011)) ;
#174691=CARTESIAN_POINT('Ctrl Pts',(-5.36445339342349,-13.4607154515732,
120.618928922871)) ;
#174692=CARTESIAN_POINT('Ctrl Pts',(-5.18265709814504,-13.4607154515732,
120.514149932282)) ;
#174693=CARTESIAN_POINT('Ctrl Pts',(-5.04597897894181,-13.4607154515732,
120.362468390451)) ;
#174694=CARTESIAN_POINT('Ctrl Pts',(-4.96280251429834,-13.4607154515732,
120.177172641054)) ;
#174695=CARTESIAN_POINT('Ctrl Pts',(-4.94189991062264,-13.4607154515732,
119.97127049429)) ;
#174696=CARTESIAN_POINT('Ctrl Pts',(-4.98833964154144,-13.4607154515732,
119.767982106043)) ;
#174697=CARTESIAN_POINT('Ctrl Pts',(-5.09419415993757,-13.4607154515732,
119.590012717272)) ;
#174698=CARTESIAN_POINT('Ctrl Pts',(-5.24909308706152,-13.4607154515732,
119.449653557218)) ;
#174699=CARTESIAN_POINT('Ctrl Pts',(-5.44305976208226,-13.4607154515732,
119.359449641273)) ;
#174700=CARTESIAN_POINT('Ctrl Pts',(-5.65504200079475,-13.4607154515732,
119.332086511174)) ;
#174701=CARTESIAN_POINT('Ctrl Pts',(-5.7931791132922,-13.4607154515732,
119.35624483207)) ;
#174702=CARTESIAN_POINT('Ctrl Pts',(-5.85699395434883,-13.4607154515732,
119.377580402306)) ;
#174703=CARTESIAN_POINT('Ctrl Pts',(-6.29671586874031,-13.4607154515732,
120.051559617786)) ;
#174704=CARTESIAN_POINT('Ctrl Pts',(-6.28976012863649,-13.4607154515732,
120.117372634366)) ;
#174705=CARTESIAN_POINT('Ctrl Pts',(-6.25432280440511,-13.4607154515732,
120.250618929773)) ;
#174706=CARTESIAN_POINT('Ctrl Pts',(-6.140310678484,-13.4607154515732,120.428143665408)) ;
#174707=CARTESIAN_POINT('Ctrl Pts',(-5.97568444568715,-13.4607154515732,
120.563316664804)) ;
#174708=CARTESIAN_POINT('Ctrl Pts',(-5.78097860437995,-13.4607154515732,
120.642680062699)) ;
#174709=CARTESIAN_POINT('Ctrl Pts',(-5.57200742713837,-13.4607154515732,
120.662582212011)) ;
#174710=CARTESIAN_POINT('Ctrl Pts',(-5.36445339342349,-13.4607154515732,
120.618928922871)) ;
#174711=CARTESIAN_POINT('Ctrl Pts',(-5.18265709814504,-13.4607154515732,
120.514149932282)) ;
#174712=CARTESIAN_POINT('Ctrl Pts',(-5.04597897894181,-13.4607154515732,
120.362468390451)) ;
#174713=CARTESIAN_POINT('Ctrl Pts',(-4.96280251429834,-13.4607154515732,
120.177172641054)) ;
#174714=CARTESIAN_POINT('Ctrl Pts',(-4.94189991062264,-13.4607154515732,
119.97127049429)) ;
#174715=CARTESIAN_POINT('Ctrl Pts',(-4.98833964154144,-13.4607154515732,
119.767982106043)) ;
#174716=CARTESIAN_POINT('Ctrl Pts',(-5.09419415993757,-13.4607154515732,
119.590012717272)) ;
#174717=CARTESIAN_POINT('Ctrl Pts',(-5.24909308706152,-13.4607154515732,
119.449653557218)) ;
#174718=CARTESIAN_POINT('Ctrl Pts',(-5.44305976208226,-13.4607154515732,
119.359449641273)) ;
#174719=CARTESIAN_POINT('Ctrl Pts',(-5.65504200079475,-13.4607154515732,
119.332086511174)) ;
#174720=CARTESIAN_POINT('Ctrl Pts',(-5.7931791132922,-13.4607154515732,
119.35624483207)) ;
#174721=CARTESIAN_POINT('Ctrl Pts',(-5.85699395434883,-13.4607154515732,
119.377580402306)) ;
#174722=CARTESIAN_POINT('Origin',(-29.5801015914784,-13.4878920043255,112.829331611621)) ;
#174723=CARTESIAN_POINT('',(-29.6364905070076,-13.4607154515732,112.659288401873)) ;
#174724=CARTESIAN_POINT('Origin',(-29.6138839527266,-13.4878920043255,112.726350034346)) ;
#174725=CARTESIAN_POINT('Ctrl Pts',(-29.1489187358159,-13.1500241806476,
113.370642219953)) ;
#174726=CARTESIAN_POINT('Ctrl Pts',(-29.1262302782877,-13.1683184483544,
113.301536839092)) ;
#174727=CARTESIAN_POINT('Ctrl Pts',(-29.0524264348783,-13.1683184483544,
113.32576788081)) ;
#174728=CARTESIAN_POINT('Ctrl Pts',(-28.9786225914689,-13.1683184483544,
113.349998922528)) ;
#174729=CARTESIAN_POINT('Ctrl Pts',(-29.0013110489971,-13.1500241806476,
113.41910430339)) ;
#174730=CARTESIAN_POINT('Ctrl Pts',(-29.0239995065253,-13.1317299129408,
113.488209684252)) ;
#174731=CARTESIAN_POINT('Ctrl Pts',(-29.0978033499347,-13.1317299129408,
113.463978642533)) ;
#174732=CARTESIAN_POINT('Ctrl Pts',(-29.1716071933441,-13.1317299129408,
113.439747600815)) ;
#174733=CARTESIAN_POINT('Ctrl Pts',(-29.1489187358159,-13.1500241806476,
113.370642219953)) ;
#174734=CARTESIAN_POINT('Ctrl Pts',(-29.1481908350552,-13.1438552129684,
113.369207785981)) ;
#174735=CARTESIAN_POINT('Ctrl Pts',(-29.1255364269104,-13.1625827638083,
113.300206114203)) ;
#174736=CARTESIAN_POINT('Ctrl Pts',(-29.0517325842656,-13.1625827713816,
113.32443715825)) ;
#174737=CARTESIAN_POINT('Ctrl Pts',(-28.9779287416207,-13.1625827789549,
113.348668202297)) ;
#174738=CARTESIAN_POINT('Ctrl Pts',(-29.0005831497655,-13.143855228115,
113.417669874074)) ;
#174739=CARTESIAN_POINT('Ctrl Pts',(-29.0232375579103,-13.1251276772751,
113.486671545852)) ;
#174740=CARTESIAN_POINT('Ctrl Pts',(-29.0970414005551,-13.1251276697018,
113.462440501806)) ;
#174741=CARTESIAN_POINT('Ctrl Pts',(-29.1708452432,-13.1251276621286,113.438209457759)) ;
#174742=CARTESIAN_POINT('Ctrl Pts',(-29.1481908350552,-13.1438552129684,
113.369207785981)) ;
#174743=CARTESIAN_POINT('Ctrl Pts',(-29.1363218176444,-13.045472096163,
113.345565010115)) ;
#174744=CARTESIAN_POINT('Ctrl Pts',(-29.1142262333781,-13.0710887780094,
113.27826542217)) ;
#174745=CARTESIAN_POINT('Ctrl Pts',(-29.0404223713575,-13.0710886158947,
113.302496407201)) ;
#174746=CARTESIAN_POINT('Ctrl Pts',(-28.9666185093369,-13.07108845378,113.326727392232)) ;
#174747=CARTESIAN_POINT('Ctrl Pts',(-28.9887140936032,-13.0454717719336,
113.394026980177)) ;
#174748=CARTESIAN_POINT('Ctrl Pts',(-29.0108096778695,-13.0198550900872,
113.461326568122)) ;
#174749=CARTESIAN_POINT('Ctrl Pts',(-29.0846135398901,-13.0198552522019,
113.437095583091)) ;
#174750=CARTESIAN_POINT('Ctrl Pts',(-29.1584174019107,-13.0198554143166,
113.41286459806)) ;
#174751=CARTESIAN_POINT('Ctrl Pts',(-29.1363218176444,-13.045472096163,
113.345565010115)) ;
#174752=CARTESIAN_POINT('Ctrl Pts',(-29.1042713188461,-12.8597742993635,
113.272543581875)) ;
#174753=CARTESIAN_POINT('Ctrl Pts',(-29.0838803914435,-12.8983625293638,
113.210436108561)) ;
#174754=CARTESIAN_POINT('Ctrl Pts',(-29.0100765562992,-12.8983626007157,
113.234667175454)) ;
#174755=CARTESIAN_POINT('Ctrl Pts',(-28.9362727211549,-12.8983626720675,
113.258898242346)) ;
#174756=CARTESIAN_POINT('Ctrl Pts',(-28.9566636485575,-12.8597744420672,
113.32100571566)) ;
#174757=CARTESIAN_POINT('Ctrl Pts',(-28.97705457596,-12.821186212067,113.383113188974)) ;
#174758=CARTESIAN_POINT('Ctrl Pts',(-29.0508584111043,-12.8211861407151,
113.358882122082)) ;
#174759=CARTESIAN_POINT('Ctrl Pts',(-29.1246622462486,-12.8211860693632,
113.334651055189)) ;
#174760=CARTESIAN_POINT('Ctrl Pts',(-29.1042713188461,-12.8597742993635,
113.272543581875)) ;
#174761=CARTESIAN_POINT('Ctrl Pts',(-29.0373324850924,-12.6327839415056,
113.104016096402)) ;
#174762=CARTESIAN_POINT('Ctrl Pts',(-29.020854571842,-12.6872840912264,
113.053827030836)) ;
#174763=CARTESIAN_POINT('Ctrl Pts',(-28.9470507251008,-12.6872840678826,
113.078058062406)) ;
#174764=CARTESIAN_POINT('Ctrl Pts',(-28.8732468783596,-12.6872840445389,
113.102289093976)) ;
#174765=CARTESIAN_POINT('Ctrl Pts',(-28.88972479161,-12.6327838948181,113.152478159542)) ;
#174766=CARTESIAN_POINT('Ctrl Pts',(-28.9062027048603,-12.5782837450973,
113.202667225107)) ;
#174767=CARTESIAN_POINT('Ctrl Pts',(-28.9800065516015,-12.578283768441,
113.178436193537)) ;
#174768=CARTESIAN_POINT('Ctrl Pts',(-29.0538103983427,-12.5782837917848,
113.154205161967)) ;
#174769=CARTESIAN_POINT('Ctrl Pts',(-29.0373324850924,-12.6327839415056,
113.104016096402)) ;
#174770=CARTESIAN_POINT('Ctrl Pts',(-28.9535211541043,-12.4610780963096,
112.884187309328)) ;
#174771=CARTESIAN_POINT('Ctrl Pts',(-28.9421376564659,-12.5276451730564,
112.849515012138)) ;
#174772=CARTESIAN_POINT('Ctrl Pts',(-28.8683338107351,-12.52764517241,112.873746046785)) ;
#174773=CARTESIAN_POINT('Ctrl Pts',(-28.7945299650043,-12.5276451717636,
112.897977081433)) ;
#174774=CARTESIAN_POINT('Ctrl Pts',(-28.8059134626427,-12.4610780950169,
112.932649378623)) ;
#174775=CARTESIAN_POINT('Ctrl Pts',(-28.817296960281,-12.3945110182701,
112.967321675813)) ;
#174776=CARTESIAN_POINT('Ctrl Pts',(-28.8911008060119,-12.3945110189165,
112.943090641166)) ;
#174777=CARTESIAN_POINT('Ctrl Pts',(-28.9649046517427,-12.3945110195628,
112.918859606518)) ;
#174778=CARTESIAN_POINT('Ctrl Pts',(-28.9535211541043,-12.4610780963096,
112.884187309328)) ;
#174779=CARTESIAN_POINT('Ctrl Pts',(-28.8575946335874,-12.3578311300529,
112.627637093626)) ;
#174780=CARTESIAN_POINT('Ctrl Pts',(-28.8521552951405,-12.431704833434,
112.611069745946)) ;
#174781=CARTESIAN_POINT('Ctrl Pts',(-28.7783514457022,-12.4317048270663,
112.635300769301)) ;
#174782=CARTESIAN_POINT('Ctrl Pts',(-28.7045475962638,-12.4317048206985,
112.659531792655)) ;
#174783=CARTESIAN_POINT('Ctrl Pts',(-28.7099869347107,-12.3578311173174,
112.676099140336)) ;
#174784=CARTESIAN_POINT('Ctrl Pts',(-28.7154262731576,-12.2839574139363,
112.692666488017)) ;
#174785=CARTESIAN_POINT('Ctrl Pts',(-28.7892301225959,-12.283957420304,
112.668435464662)) ;
#174786=CARTESIAN_POINT('Ctrl Pts',(-28.8630339720343,-12.2839574266718,
112.644204441307)) ;
#174787=CARTESIAN_POINT('Ctrl Pts',(-28.8575946335874,-12.3578311300529,
112.627637093626)) ;
#174788=CARTESIAN_POINT('Ctrl Pts',(-28.7572250300145,-12.3309709098726,
112.357185420699)) ;
#174789=CARTESIAN_POINT('Ctrl Pts',(-28.7580561715402,-12.4068262743209,
112.359716943198)) ;
#174790=CARTESIAN_POINT('Ctrl Pts',(-28.684252320216,-12.4068262750749,
112.383947960808)) ;
#174791=CARTESIAN_POINT('Ctrl Pts',(-28.6104484688917,-12.4068262758288,
112.408178978419)) ;
#174792=CARTESIAN_POINT('Ctrl Pts',(-28.609617327366,-12.3309709113806,
112.405647455921)) ;
#174793=CARTESIAN_POINT('Ctrl Pts',(-28.6087861858402,-12.2551155469323,
112.403115933422)) ;
#174794=CARTESIAN_POINT('Ctrl Pts',(-28.6825900371645,-12.2551155461783,
112.378884915812)) ;
#174795=CARTESIAN_POINT('Ctrl Pts',(-28.7563938884887,-12.2551155454244,
112.354653898201)) ;
#174796=CARTESIAN_POINT('Ctrl Pts',(-28.7572250300145,-12.3309709098726,
112.357185420699)) ;
#174797=CARTESIAN_POINT('Ctrl Pts',(-28.6569634591251,-12.3817310335918,
112.087380599263)) ;
#174798=CARTESIAN_POINT('Ctrl Pts',(-28.6640600261264,-12.4541523823842,
112.108995596646)) ;
#174799=CARTESIAN_POINT('Ctrl Pts',(-28.5902561722792,-12.4541523921254,
112.133226606572)) ;
#174800=CARTESIAN_POINT('Ctrl Pts',(-28.5164523184319,-12.4541524018665,
112.157457616498)) ;
#174801=CARTESIAN_POINT('Ctrl Pts',(-28.5093557514307,-12.3817310530741,
112.135842619115)) ;
#174802=CARTESIAN_POINT('Ctrl Pts',(-28.5022591844293,-12.3093097042818,
112.114227621731)) ;
#174803=CARTESIAN_POINT('Ctrl Pts',(-28.5760630382766,-12.3093096945406,
112.089996611805)) ;
#174804=CARTESIAN_POINT('Ctrl Pts',(-28.6498668921238,-12.3093096847995,
112.065765601879)) ;
#174805=CARTESIAN_POINT('Ctrl Pts',(-28.6569634591251,-12.3817310335918,
112.087380599263)) ;
#174806=CARTESIAN_POINT('Ctrl Pts',(-28.564509082064,-12.5067458714326,
111.841211648264)) ;
#174807=CARTESIAN_POINT('Ctrl Pts',(-28.5773378755298,-12.5705432422448,
111.880286082408)) ;
#174808=CARTESIAN_POINT('Ctrl Pts',(-28.5035340207076,-12.57054326527,111.904517089365)) ;
#174809=CARTESIAN_POINT('Ctrl Pts',(-28.4297301658854,-12.5705432882951,
111.928748096321)) ;
#174810=CARTESIAN_POINT('Ctrl Pts',(-28.4169013724195,-12.5067459174828,
111.889673662177)) ;
#174811=CARTESIAN_POINT('Ctrl Pts',(-28.4040725789537,-12.4429485466705,
111.850599228033)) ;
#174812=CARTESIAN_POINT('Ctrl Pts',(-28.4778764337759,-12.4429485236454,
111.826368221076)) ;
#174813=CARTESIAN_POINT('Ctrl Pts',(-28.5516802885981,-12.4429485006203,
111.80213721412)) ;
#174814=CARTESIAN_POINT('Ctrl Pts',(-28.564509082064,-12.5067458714326,
111.841211648264)) ;
#174815=CARTESIAN_POINT('Ctrl Pts',(-28.4851946394043,-12.6971218835384,
111.635119922408)) ;
#174816=CARTESIAN_POINT('Ctrl Pts',(-28.5028453351627,-12.7477196021645,
111.688881092751)) ;
#174817=CARTESIAN_POINT('Ctrl Pts',(-28.4290414807966,-12.7477196406968,
111.713112101097)) ;
#174818=CARTESIAN_POINT('Ctrl Pts',(-28.3552376264306,-12.7477196792291,
111.737343109443)) ;
#174819=CARTESIAN_POINT('Ctrl Pts',(-28.3375869306722,-12.697121960603,
111.6835819391)) ;
#174820=CARTESIAN_POINT('Ctrl Pts',(-28.3199362349139,-12.646524241977,
111.629820768757)) ;
#174821=CARTESIAN_POINT('Ctrl Pts',(-28.3937400892799,-12.6465242034447,
111.605589760411)) ;
#174822=CARTESIAN_POINT('Ctrl Pts',(-28.4675439436459,-12.6465241649123,
111.581358752065)) ;
#174823=CARTESIAN_POINT('Ctrl Pts',(-28.4851946394043,-12.6971218835384,
111.635119922408)) ;
#174824=CARTESIAN_POINT('Ctrl Pts',(-28.4241475022264,-12.9391053860727,
111.48464558118)) ;
#174825=CARTESIAN_POINT('Ctrl Pts',(-28.4453520755906,-12.9728813246928,
111.549231289129)) ;
#174826=CARTESIAN_POINT('Ctrl Pts',(-28.3715482236367,-12.9728813789312,
111.573462304821)) ;
#174827=CARTESIAN_POINT('Ctrl Pts',(-28.2977443716827,-12.9728814331696,
111.597693320514)) ;
#174828=CARTESIAN_POINT('Ctrl Pts',(-28.2765397983185,-12.9391054945495,
111.533107612566)) ;
#174829=CARTESIAN_POINT('Ctrl Pts',(-28.2553352249542,-12.9053295559293,
111.468521904618)) ;
#174830=CARTESIAN_POINT('Ctrl Pts',(-28.3291390769082,-12.9053295016909,
111.444290888925)) ;
#174831=CARTESIAN_POINT('Ctrl Pts',(-28.4029429288622,-12.9053294474525,
111.420059873232)) ;
#174832=CARTESIAN_POINT('Ctrl Pts',(-28.4241475022264,-12.9391053860727,
111.48464558118)) ;
#174833=CARTESIAN_POINT('Ctrl Pts',(-28.3849524033199,-13.2152764852227,
111.400718831589)) ;
#174834=CARTESIAN_POINT('Ctrl Pts',(-28.4081905270802,-13.2298195844166,
111.471498405773)) ;
#174835=CARTESIAN_POINT('Ctrl Pts',(-28.3343866794691,-13.2298196519975,
111.495729434694)) ;
#174836=CARTESIAN_POINT('Ctrl Pts',(-28.260582831858,-13.2298197195784,
111.519960463614)) ;
#174837=CARTESIAN_POINT('Ctrl Pts',(-28.2373447080977,-13.2152766203844,
111.44918088943)) ;
#174838=CARTESIAN_POINT('Ctrl Pts',(-28.2141065843374,-13.2007335211905,
111.378401315245)) ;
#174839=CARTESIAN_POINT('Ctrl Pts',(-28.2879104319485,-13.2007334536096,
111.354170286325)) ;
#174840=CARTESIAN_POINT('Ctrl Pts',(-28.3617142795596,-13.2007333860287,
111.329939257405)) ;
#174841=CARTESIAN_POINT('Ctrl Pts',(-28.3849524033199,-13.2152764852227,
111.400718831589)) ;
#174842=CARTESIAN_POINT('Ctrl Pts',(-28.3695728344553,-13.505784356226,
111.389304759768)) ;
#174843=CARTESIAN_POINT('Ctrl Pts',(-28.3931852419853,-13.5000660445819,
111.461224341778)) ;
#174844=CARTESIAN_POINT('Ctrl Pts',(-28.3193814002774,-13.5000661208921,
111.485455388679)) ;
#174845=CARTESIAN_POINT('Ctrl Pts',(-28.2455775585696,-13.5000661972022,
111.50968643558)) ;
#174846=CARTESIAN_POINT('Ctrl Pts',(-28.2219651510396,-13.5057845088464,
111.437766853569)) ;
#174847=CARTESIAN_POINT('Ctrl Pts',(-28.1983527435096,-13.5115028204905,
111.365847271559)) ;
#174848=CARTESIAN_POINT('Ctrl Pts',(-28.2721565852175,-13.5115027441803,
111.341616224659)) ;
#174849=CARTESIAN_POINT('Ctrl Pts',(-28.3459604269253,-13.5115026678702,
111.317385177758)) ;
#174850=CARTESIAN_POINT('Ctrl Pts',(-28.3695728344553,-13.505784356226,
111.389304759768)) ;
#174851=CARTESIAN_POINT('Ctrl Pts',(-28.3785666018913,-13.7916119971123,
111.452340850324)) ;
#174852=CARTESIAN_POINT('Ctrl Pts',(-28.4008480409797,-13.7659297998844,
111.520206517047)) ;
#174853=CARTESIAN_POINT('Ctrl Pts',(-28.3270442065118,-13.7659298799449,
111.544437585999)) ;
#174854=CARTESIAN_POINT('Ctrl Pts',(-28.2532403720439,-13.7659299600053,
111.568668654952)) ;
#174855=CARTESIAN_POINT('Ctrl Pts',(-28.2309589329554,-13.7916121572332,
111.500802988229)) ;
#174856=CARTESIAN_POINT('Ctrl Pts',(-28.2086774938669,-13.817294354461,
111.432937321506)) ;
#174857=CARTESIAN_POINT('Ctrl Pts',(-28.2824813283349,-13.8172942744006,
111.408706252554)) ;
#174858=CARTESIAN_POINT('Ctrl Pts',(-28.3562851628028,-13.8172941943401,
111.384475183601)) ;
#174859=CARTESIAN_POINT('Ctrl Pts',(-28.3785666018913,-13.7916119971123,
111.452340850324)) ;
#174860=CARTESIAN_POINT('Ctrl Pts',(-28.4102051428863,-14.0480477215918,
111.583997783673)) ;
#174861=CARTESIAN_POINT('Ctrl Pts',(-28.4295796916699,-14.00442476396,111.643009531454)) ;
#174862=CARTESIAN_POINT('Ctrl Pts',(-28.3557758644425,-14.0044248376781,
111.66724062246)) ;
#174863=CARTESIAN_POINT('Ctrl Pts',(-28.2819720372152,-14.0044249113963,
111.691471713466)) ;
#174864=CARTESIAN_POINT('Ctrl Pts',(-28.2625974884316,-14.0480478690281,
111.632459965685)) ;
#174865=CARTESIAN_POINT('Ctrl Pts',(-28.2432229396479,-14.0916708266599,
111.573448217904)) ;
#174866=CARTESIAN_POINT('Ctrl Pts',(-28.3170267668753,-14.0916707529417,
111.549217126898)) ;
#174867=CARTESIAN_POINT('Ctrl Pts',(-28.3908305941027,-14.0916706792236,
111.524986035892)) ;
#174868=CARTESIAN_POINT('Ctrl Pts',(-28.4102051428863,-14.0480477215918,
111.583997783673)) ;
#174869=CARTESIAN_POINT('Ctrl Pts',(-28.4617096973959,-14.2608003622883,
111.776342484654)) ;
#174870=CARTESIAN_POINT('Ctrl Pts',(-28.4767827056386,-14.2022602348381,
111.822252433888)) ;
#174871=CARTESIAN_POINT('Ctrl Pts',(-28.4029788852957,-14.2022602957698,
111.846483545863)) ;
#174872=CARTESIAN_POINT('Ctrl Pts',(-28.3291750649528,-14.2022603567015,
111.870714657838)) ;
#174873=CARTESIAN_POINT('Ctrl Pts',(-28.3141020567101,-14.2608004841518,
111.824804708603)) ;
#174874=CARTESIAN_POINT('Ctrl Pts',(-28.2990290484674,-14.319340611602,
111.778894759369)) ;
#174875=CARTESIAN_POINT('Ctrl Pts',(-28.3728328688103,-14.3193405506703,
111.754663647394)) ;
#174876=CARTESIAN_POINT('Ctrl Pts',(-28.4466366891532,-14.3193404897386,
111.730432535419)) ;
#174877=CARTESIAN_POINT('Ctrl Pts',(-28.4617096973959,-14.2608003622883,
111.776342484654)) ;
#174878=CARTESIAN_POINT('Ctrl Pts',(-28.5285966908039,-14.4130997833176,
112.015523906653)) ;
#174879=CARTESIAN_POINT('Ctrl Pts',(-28.5382883279063,-14.3438411557226,
112.045043067585)) ;
#174880=CARTESIAN_POINT('Ctrl Pts',(-28.464484513117,-14.3438411966561,
112.069274196476)) ;
#174881=CARTESIAN_POINT('Ctrl Pts',(-28.3906806983278,-14.3438412375897,
112.093505325366)) ;
#174882=CARTESIAN_POINT('Ctrl Pts',(-28.3809890612254,-14.4130998651847,
112.063986164433)) ;
#174883=CARTESIAN_POINT('Ctrl Pts',(-28.371297424123,-14.4823584927798,
112.034467003501)) ;
#174884=CARTESIAN_POINT('Ctrl Pts',(-28.4451012389122,-14.4823584518462,
112.010235874611)) ;
#174885=CARTESIAN_POINT('Ctrl Pts',(-28.5189050537015,-14.4823584109127,
111.98600474572)) ;
#174886=CARTESIAN_POINT('Ctrl Pts',(-28.5285966908039,-14.4130997833176,
112.015523906653)) ;
#174887=CARTESIAN_POINT('Ctrl Pts',(-28.6055369658778,-14.494276858583,
112.285430331193)) ;
#174888=CARTESIAN_POINT('Ctrl Pts',(-28.6091354502607,-14.419248986888,
112.296390731991)) ;
#174889=CARTESIAN_POINT('Ctrl Pts',(-28.5353316390701,-14.4192490024428,
112.320621871842)) ;
#174890=CARTESIAN_POINT('Ctrl Pts',(-28.4615278278796,-14.4192490179976,
112.344853011694)) ;
#174891=CARTESIAN_POINT('Ctrl Pts',(-28.4579293434966,-14.4942768896926,
112.333892610895)) ;
#174892=CARTESIAN_POINT('Ctrl Pts',(-28.4543308591137,-14.5693047613875,
112.322932210097)) ;
#174893=CARTESIAN_POINT('Ctrl Pts',(-28.5281346703043,-14.5693047458327,
112.298701070246)) ;
#174894=CARTESIAN_POINT('Ctrl Pts',(-28.6019384814949,-14.569304730278,
112.274469930394)) ;
#174895=CARTESIAN_POINT('Ctrl Pts',(-28.6055369658778,-14.494276858583,
112.285430331193)) ;
#174896=CARTESIAN_POINT('Ctrl Pts',(-28.6858402113565,-14.4979516536895,
112.565480733191)) ;
#174897=CARTESIAN_POINT('Ctrl Pts',(-28.6831038105203,-14.4225568687656,
112.557146095696)) ;
#174898=CARTESIAN_POINT('Ctrl Pts',(-28.6093000001973,-14.4225568559479,
112.58137723819)) ;
#174899=CARTESIAN_POINT('Ctrl Pts',(-28.5354961898742,-14.4225568431301,
112.605608380683)) ;
#174900=CARTESIAN_POINT('Ctrl Pts',(-28.5382325907104,-14.497951628054,
112.613943018178)) ;
#174901=CARTESIAN_POINT('Ctrl Pts',(-28.5409689915465,-14.5733464129779,
112.622277655674)) ;
#174902=CARTESIAN_POINT('Ctrl Pts',(-28.6147728018696,-14.5733464257956,
112.59804651318)) ;
#174903=CARTESIAN_POINT('Ctrl Pts',(-28.6885766121926,-14.5733464386134,
112.573815370686)) ;
#174904=CARTESIAN_POINT('Ctrl Pts',(-28.6858402113565,-14.4979516536895,
112.565480733191)) ;
#174905=CARTESIAN_POINT('Ctrl Pts',(-28.7630866534358,-14.4245500702158,
112.836167498554)) ;
#174906=CARTESIAN_POINT('Ctrl Pts',(-28.754220545165,-14.3541688694618,
112.809162761213)) ;
#174907=CARTESIAN_POINT('Ctrl Pts',(-28.6804167329619,-14.3541688284501,
112.83339389798)) ;
#174908=CARTESIAN_POINT('Ctrl Pts',(-28.6066129207587,-14.3541687874384,
112.857625034748)) ;
#174909=CARTESIAN_POINT('Ctrl Pts',(-28.6154790290295,-14.4245499881925,
112.884629772089)) ;
#174910=CARTESIAN_POINT('Ctrl Pts',(-28.6243451373003,-14.4949311889465,
112.91163450943)) ;
#174911=CARTESIAN_POINT('Ctrl Pts',(-28.6981489495034,-14.4949312299582,
112.887403372663)) ;
#174912=CARTESIAN_POINT('Ctrl Pts',(-28.7719527617065,-14.4949312709699,
112.863172235896)) ;
#174913=CARTESIAN_POINT('Ctrl Pts',(-28.7630866534358,-14.4245500702158,
112.836167498554)) ;
#174914=CARTESIAN_POINT('Ctrl Pts',(-28.8312032669878,-14.27912481409,113.079082108179)) ;
#174915=CARTESIAN_POINT('Ctrl Pts',(-28.8168350433287,-14.2187925848184,
113.035318815122)) ;
#174916=CARTESIAN_POINT('Ctrl Pts',(-28.7430312266753,-14.2187925185092,
113.059549938334)) ;
#174917=CARTESIAN_POINT('Ctrl Pts',(-28.6692274100218,-14.2187924522,113.083781061547)) ;
#174918=CARTESIAN_POINT('Ctrl Pts',(-28.6835956336809,-14.2791246814716,
113.127544354603)) ;
#174919=CARTESIAN_POINT('Ctrl Pts',(-28.69796385734,-14.3394569107431,113.17130764766)) ;
#174920=CARTESIAN_POINT('Ctrl Pts',(-28.7717676739935,-14.3394569770523,
113.147076524447)) ;
#174921=CARTESIAN_POINT('Ctrl Pts',(-28.8455714906469,-14.3394570433615,
113.122845401235)) ;
#174922=CARTESIAN_POINT('Ctrl Pts',(-28.8312032669878,-14.27912481409,113.079082108179)) ;
#174923=CARTESIAN_POINT('Ctrl Pts',(-28.8845697171654,-14.0717728276009,
113.277121444909)) ;
#174924=CARTESIAN_POINT('Ctrl Pts',(-28.8657198886564,-14.0258274816855,
113.2197079066)) ;
#174925=CARTESIAN_POINT('Ctrl Pts',(-28.79191606536,-14.0258273955752,113.243939009579)) ;
#174926=CARTESIAN_POINT('Ctrl Pts',(-28.7181122420636,-14.025827309465,
113.268170112557)) ;
#174927=CARTESIAN_POINT('Ctrl Pts',(-28.7369620705726,-14.0717726553804,
113.325583650866)) ;
#174928=CARTESIAN_POINT('Ctrl Pts',(-28.7558118990816,-14.1177180012958,
113.382997189175)) ;
#174929=CARTESIAN_POINT('Ctrl Pts',(-28.829615722378,-14.1177180874061,
113.358766086196)) ;
#174930=CARTESIAN_POINT('Ctrl Pts',(-28.9034195456744,-14.1177181735163,
113.334534983217)) ;
#174931=CARTESIAN_POINT('Ctrl Pts',(-28.8845697171654,-14.0717728276009,
113.277121444909)) ;
#174932=CARTESIAN_POINT('Ctrl Pts',(-28.9184685925918,-13.8168218187551,
113.415944332688)) ;
#174933=CARTESIAN_POINT('Ctrl Pts',(-28.8964878467621,-13.7886075890761,
113.348994525439)) ;
#174934=CARTESIAN_POINT('Ctrl Pts',(-28.8226840152995,-13.7886074911404,
113.373225603545)) ;
#174935=CARTESIAN_POINT('Ctrl Pts',(-28.748880183837,-13.7886073932047,
113.397456681651)) ;
#174936=CARTESIAN_POINT('Ctrl Pts',(-28.7708609296667,-13.8168216228837,
113.464406488901)) ;
#174937=CARTESIAN_POINT('Ctrl Pts',(-28.7928416754963,-13.8450358525627,
113.53135629615)) ;
#174938=CARTESIAN_POINT('Ctrl Pts',(-28.8666455069589,-13.8450359504984,
113.507125218044)) ;
#174939=CARTESIAN_POINT('Ctrl Pts',(-28.9404493384214,-13.8450360484341,
113.482894139938)) ;
#174940=CARTESIAN_POINT('Ctrl Pts',(-28.9184685925918,-13.8168218187551,
113.415944332688)) ;
#174941=CARTESIAN_POINT('Ctrl Pts',(-28.9296288975394,-13.535324035321,
113.485246560678)) ;
#174942=CARTESIAN_POINT('Ctrl Pts',(-28.9061056378455,-13.5267213387171,
113.413598505133)) ;
#174943=CARTESIAN_POINT('Ctrl Pts',(-28.8323017977866,-13.5267212367711,
113.437829557056)) ;
#174944=CARTESIAN_POINT('Ctrl Pts',(-28.7584979577277,-13.526721134825,
113.462060608979)) ;
#174945=CARTESIAN_POINT('Ctrl Pts',(-28.7820212174216,-13.5353238314288,
113.533708664524)) ;
#174946=CARTESIAN_POINT('Ctrl Pts',(-28.8055444771154,-13.5439265280327,
113.605356720069)) ;
#174947=CARTESIAN_POINT('Ctrl Pts',(-28.8793483171744,-13.5439266299788,
113.581125668146)) ;
#174948=CARTESIAN_POINT('Ctrl Pts',(-28.9531521572333,-13.5439267319248,
113.556894616223)) ;
#174949=CARTESIAN_POINT('Ctrl Pts',(-28.9296288975394,-13.535324035321,
113.485246560678)) ;
#174950=CARTESIAN_POINT('Ctrl Pts',(-28.9167824586136,-13.2440746292406,
113.481603030049)) ;
#174951=CARTESIAN_POINT('Ctrl Pts',(-28.893386607582,-13.2557932048074,
113.410343040812)) ;
#174952=CARTESIAN_POINT('Ctrl Pts',(-28.8195827591104,-13.2557931077727,
113.434574067111)) ;
#174953=CARTESIAN_POINT('Ctrl Pts',(-28.7457789106387,-13.2557930107381,
113.45880509341)) ;
#174954=CARTESIAN_POINT('Ctrl Pts',(-28.7691747616702,-13.2440744351713,
113.530065082647)) ;
#174955=CARTESIAN_POINT('Ctrl Pts',(-28.7925706127017,-13.2323558596045,
113.601325071884)) ;
#174956=CARTESIAN_POINT('Ctrl Pts',(-28.8663744611734,-13.2323559566392,
113.577094045585)) ;
#174957=CARTESIAN_POINT('Ctrl Pts',(-28.940178309645,-13.2323560536738,
113.552863019286)) ;
#174958=CARTESIAN_POINT('Ctrl Pts',(-28.9167824586136,-13.2440746292406,
113.481603030049)) ;
#174959=CARTESIAN_POINT('Ctrl Pts',(-28.879724619622,-12.9648031401168,
113.404286512872)) ;
#174960=CARTESIAN_POINT('Ctrl Pts',(-28.8581450995204,-12.9960374765742,
113.338558774695)) ;
#174961=CARTESIAN_POINT('Ctrl Pts',(-28.784341243934,-12.9960373926029,
113.362789779324)) ;
#174962=CARTESIAN_POINT('Ctrl Pts',(-28.7105373883475,-12.9960373086315,
113.387020783953)) ;
#174963=CARTESIAN_POINT('Ctrl Pts',(-28.7321169084492,-12.964802972174,
113.452748522129)) ;
#174964=CARTESIAN_POINT('Ctrl Pts',(-28.7536964285508,-12.9335686357166,
113.518476260305)) ;
#174965=CARTESIAN_POINT('Ctrl Pts',(-28.8275002841372,-12.933568719688,
113.494245255677)) ;
#174966=CARTESIAN_POINT('Ctrl Pts',(-28.9013041397237,-12.9335688036593,
113.470014251048)) ;
#174967=CARTESIAN_POINT('Ctrl Pts',(-28.879724619622,-12.9648031401168,
113.404286512872)) ;
#174968=CARTESIAN_POINT('Ctrl Pts',(-28.8209010350444,-12.7194345507308,
113.260464724787)) ;
#174969=CARTESIAN_POINT('Ctrl Pts',(-28.8026647225913,-12.7678470581872,
113.204919857785)) ;
#174970=CARTESIAN_POINT('Ctrl Pts',(-28.7288608615466,-12.7678469916176,
113.229150845788)) ;
#174971=CARTESIAN_POINT('Ctrl Pts',(-28.6550570005018,-12.767846925048,
113.253381833792)) ;
#174972=CARTESIAN_POINT('Ctrl Pts',(-28.6732933129549,-12.7194344175916,
113.308926700794)) ;
#174973=CARTESIAN_POINT('Ctrl Pts',(-28.691529625408,-12.6710219101352,
113.364471567796)) ;
#174974=CARTESIAN_POINT('Ctrl Pts',(-28.7653334864528,-12.6710219767048,
113.340240579793)) ;
#174975=CARTESIAN_POINT('Ctrl Pts',(-28.8391373474975,-12.6710220432744,
113.316009591789)) ;
#174976=CARTESIAN_POINT('Ctrl Pts',(-28.8209010350444,-12.7194345507308,
113.260464724787)) ;
#174977=CARTESIAN_POINT('Ctrl Pts',(-28.7430943016509,-12.5228537207888,
113.059023280909)) ;
#174978=CARTESIAN_POINT('Ctrl Pts',(-28.7295272533621,-12.5850644655665,
113.017700239312)) ;
#174979=CARTESIAN_POINT('Ctrl Pts',(-28.6557233893278,-12.5850644207041,
113.04193121821)) ;
#174980=CARTESIAN_POINT('Ctrl Pts',(-28.5819195252936,-12.5850643758416,
113.066162197108)) ;
#174981=CARTESIAN_POINT('Ctrl Pts',(-28.5954865735824,-12.522853631064,
113.107485238705)) ;
#174982=CARTESIAN_POINT('Ctrl Pts',(-28.6090536218712,-12.4606428862864,
113.148808280301)) ;
#174983=CARTESIAN_POINT('Ctrl Pts',(-28.6828574859055,-12.4606429311488,
113.124577301403)) ;
#174984=CARTESIAN_POINT('Ctrl Pts',(-28.7566613499397,-12.4606429760112,
113.100346322505)) ;
#174985=CARTESIAN_POINT('Ctrl Pts',(-28.7430943016509,-12.5228537207888,
113.059023280909)) ;
#174986=CARTESIAN_POINT('Ctrl Pts',(-28.6517657151193,-12.3910219564108,
112.816257416584)) ;
#174987=CARTESIAN_POINT('Ctrl Pts',(-28.6438220478864,-12.4625310700348,
112.792062286491)) ;
#174988=CARTESIAN_POINT('Ctrl Pts',(-28.5700181829588,-12.4625310467126,
112.816293262668)) ;
#174989=CARTESIAN_POINT('Ctrl Pts',(-28.4962143180312,-12.4625310233905,
112.840524238845)) ;
#174990=CARTESIAN_POINT('Ctrl Pts',(-28.5041579852641,-12.3910219097665,
112.864719368938)) ;
#174991=CARTESIAN_POINT('Ctrl Pts',(-28.5121016524971,-12.3195127961425,
112.888914499031)) ;
#174992=CARTESIAN_POINT('Ctrl Pts',(-28.5859055174246,-12.3195128194647,
112.864683522854)) ;
#174993=CARTESIAN_POINT('Ctrl Pts',(-28.6597093823522,-12.3195128427868,
112.840452546677)) ;
#174994=CARTESIAN_POINT('Ctrl Pts',(-28.6517657151193,-12.3910219564108,
112.816257416584)) ;
#174995=CARTESIAN_POINT('Ctrl Pts',(-28.5519605561705,-12.3324946198483,
112.547844627311)) ;
#174996=CARTESIAN_POINT('Ctrl Pts',(-28.5502370298838,-12.408198760168,
112.542595043101)) ;
#174997=CARTESIAN_POINT('Ctrl Pts',(-28.4764331666314,-12.4081987566325,
112.56682602438)) ;
#174998=CARTESIAN_POINT('Ctrl Pts',(-28.402629303379,-12.4081987530971,
112.59105700566)) ;
#174999=CARTESIAN_POINT('Ctrl Pts',(-28.4043528296657,-12.3324946127775,
112.59630658987)) ;
#175000=CARTESIAN_POINT('Ctrl Pts',(-28.4060763559524,-12.2567904724578,
112.60155617408)) ;
#175001=CARTESIAN_POINT('Ctrl Pts',(-28.4798802192048,-12.2567904759932,
112.577325192801)) ;
#175002=CARTESIAN_POINT('Ctrl Pts',(-28.5536840824571,-12.2567904795287,
112.553094211521)) ;
#175003=CARTESIAN_POINT('Ctrl Pts',(-28.5519605561705,-12.3324946198483,
112.547844627311)) ;
#175004=CARTESIAN_POINT('Ctrl Pts',(-28.4511785871551,-12.3517941049946,
112.2762149844)) ;
#175005=CARTESIAN_POINT('Ctrl Pts',(-28.4557579295196,-12.426265134033,
112.290162921278)) ;
#175006=CARTESIAN_POINT('Ctrl Pts',(-28.3819540689083,-12.426265145997,
112.314393910602)) ;
#175007=CARTESIAN_POINT('Ctrl Pts',(-28.308150208297,-12.4262651579609,
112.338624899925)) ;
#175008=CARTESIAN_POINT('Ctrl Pts',(-28.3035708659325,-12.3517941289225,
112.324676963048)) ;
#175009=CARTESIAN_POINT('Ctrl Pts',(-28.298991523568,-12.2773230998841,
112.310729026171)) ;
#175010=CARTESIAN_POINT('Ctrl Pts',(-28.3727953841793,-12.2773230879201,
112.286498036847)) ;
#175011=CARTESIAN_POINT('Ctrl Pts',(-28.4465992447906,-12.2773230759562,
112.262267047523)) ;
#175012=CARTESIAN_POINT('Ctrl Pts',(-28.4511785871551,-12.3517941049946,
112.2762149844)) ;
#175013=CARTESIAN_POINT('Ctrl Pts',(-28.3546167960162,-12.4476532719571,
112.01766426386)) ;
#175014=CARTESIAN_POINT('Ctrl Pts',(-28.365209322812,-12.5155445566341,
112.049927390478)) ;
#175015=CARTESIAN_POINT('Ctrl Pts',(-28.2914054664986,-12.5155445785794,
112.074158392892)) ;
#175016=CARTESIAN_POINT('Ctrl Pts',(-28.2176016101851,-12.5155446005247,
112.098389395307)) ;
#175017=CARTESIAN_POINT('Ctrl Pts',(-28.2070090833893,-12.4476533158478,
112.066126268689)) ;
#175018=CARTESIAN_POINT('Ctrl Pts',(-28.1964165565935,-12.3797620311708,
112.033863142072)) ;
#175019=CARTESIAN_POINT('Ctrl Pts',(-28.2702204129069,-12.3797620092255,
112.009632139657)) ;
#175020=CARTESIAN_POINT('Ctrl Pts',(-28.3440242692203,-12.3797619872802,
111.985401137243)) ;
#175021=CARTESIAN_POINT('Ctrl Pts',(-28.3546167960162,-12.4476532719571,
112.01766426386)) ;
#175022=CARTESIAN_POINT('Ctrl Pts',(-28.2694260224947,-12.6128436094032,
111.793615869469)) ;
#175023=CARTESIAN_POINT('Ctrl Pts',(-28.2852496876729,-12.6693038141033,
111.841812199719)) ;
#175024=CARTESIAN_POINT('Ctrl Pts',(-28.211445835532,-12.669303840492,111.866043214843)) ;
#175025=CARTESIAN_POINT('Ctrl Pts',(-28.1376419833911,-12.6693038668807,
111.890274229966)) ;
#175026=CARTESIAN_POINT('Ctrl Pts',(-28.1218183182129,-12.6128436621805,
111.842077899716)) ;
#175027=CARTESIAN_POINT('Ctrl Pts',(-28.1059946530346,-12.5563834574804,
111.793881569465)) ;
#175028=CARTESIAN_POINT('Ctrl Pts',(-28.1797985051756,-12.5563834310917,
111.769650554342)) ;
#175029=CARTESIAN_POINT('Ctrl Pts',(-28.2536023573165,-12.556383404703,
111.745419539218)) ;
#175030=CARTESIAN_POINT('Ctrl Pts',(-28.2694260224947,-12.6128436094032,
111.793615869469)) ;
#175031=CARTESIAN_POINT('Ctrl Pts',(-28.2004725461681,-12.8354722898284,
111.619033756946)) ;
#175032=CARTESIAN_POINT('Ctrl Pts',(-28.2204013581391,-12.8764735343339,
111.679733702125)) ;
#175033=CARTESIAN_POINT('Ctrl Pts',(-28.1465975099213,-12.8764735602594,
111.703964729197)) ;
#175034=CARTESIAN_POINT('Ctrl Pts',(-28.0727936617034,-12.8764735861849,
111.728195756269)) ;
#175035=CARTESIAN_POINT('Ctrl Pts',(-28.0528648497324,-12.8354723416794,
111.667495811091)) ;
#175036=CARTESIAN_POINT('Ctrl Pts',(-28.0329360377614,-12.794471097174,
111.606795865912)) ;
#175037=CARTESIAN_POINT('Ctrl Pts',(-28.1067398859793,-12.7944710712485,
111.582564838839)) ;
#175038=CARTESIAN_POINT('Ctrl Pts',(-28.1805437341971,-12.794471045323,
111.558333811767)) ;
#175039=CARTESIAN_POINT('Ctrl Pts',(-28.2004725461681,-12.8354722898284,
111.619033756946)) ;
#175040=CARTESIAN_POINT('Ctrl Pts',(-28.1518872197862,-13.101408894203,
111.506681708968)) ;
#175041=CARTESIAN_POINT('Ctrl Pts',(-28.1745014661494,-13.1239035578376,
111.575561054197)) ;
#175042=CARTESIAN_POINT('Ctrl Pts',(-28.1006976210795,-13.1239035777503,
111.599792090857)) ;
#175043=CARTESIAN_POINT('Ctrl Pts',(-28.0268937760095,-13.1239035976629,
111.624023127518)) ;
#175044=CARTESIAN_POINT('Ctrl Pts',(-28.0042795296463,-13.1014089340283,
111.555143782289)) ;
#175045=CARTESIAN_POINT('Ctrl Pts',(-27.9816652832831,-13.0789142703937,
111.48626443706)) ;
#175046=CARTESIAN_POINT('Ctrl Pts',(-28.0554691283531,-13.078914250481,
111.462033400399)) ;
#175047=CARTESIAN_POINT('Ctrl Pts',(-28.129272973423,-13.0789142305684,
111.437802363739)) ;
#175048=CARTESIAN_POINT('Ctrl Pts',(-28.1518872197862,-13.101408894203,
111.506681708968)) ;
#175049=CARTESIAN_POINT('Ctrl Pts',(-28.1269130732857,-13.3874022195482,
111.465903939157)) ;
#175050=CARTESIAN_POINT('Ctrl Pts',(-28.150574864272,-13.3899614744304,
111.537973936401)) ;
#175051=CARTESIAN_POINT('Ctrl Pts',(-28.0767710208941,-13.389961489155,
111.562204978215)) ;
#175052=CARTESIAN_POINT('Ctrl Pts',(-28.0029671775161,-13.3899615038795,
111.586436020028)) ;
#175053=CARTESIAN_POINT('Ctrl Pts',(-27.9793053865298,-13.3874022489973,
111.514366022785)) ;
#175054=CARTESIAN_POINT('Ctrl Pts',(-27.9556435955435,-13.384842994115,
111.442296025541)) ;
#175055=CARTESIAN_POINT('Ctrl Pts',(-28.0294474389214,-13.3848429793905,
111.418064983727)) ;
#175056=CARTESIAN_POINT('Ctrl Pts',(-28.1032512822994,-13.3848429646659,
111.393833941913)) ;
#175057=CARTESIAN_POINT('Ctrl Pts',(-28.1269130732857,-13.3874022195482,
111.465903939157)) ;
#175058=CARTESIAN_POINT('Ctrl Pts',(-28.1259581954368,-13.6768759171903,
111.498450514514)) ;
#175059=CARTESIAN_POINT('Ctrl Pts',(-28.1489886412209,-13.6592264507691,
111.568597536266)) ;
#175060=CARTESIAN_POINT('Ctrl Pts',(-28.0751847985998,-13.6592264585441,
111.592828580385)) ;
#175061=CARTESIAN_POINT('Ctrl Pts',(-28.0013809559787,-13.6592264663191,
111.617059624505)) ;
#175062=CARTESIAN_POINT('Ctrl Pts',(-27.9783505101947,-13.6768759327404,
111.546912602753)) ;
#175063=CARTESIAN_POINT('Ctrl Pts',(-27.9553200644106,-13.6945253991617,
111.476765581001)) ;
#175064=CARTESIAN_POINT('Ctrl Pts',(-28.0291239070317,-13.6945253913867,
111.452534536881)) ;
#175065=CARTESIAN_POINT('Ctrl Pts',(-28.1029277496528,-13.6945253836116,
111.428303492762)) ;
#175066=CARTESIAN_POINT('Ctrl Pts',(-28.1259581954368,-13.6768759171903,
111.498450514514)) ;
#175067=CARTESIAN_POINT('Ctrl Pts',(-28.1487784107379,-13.948608493865,
111.603521104352)) ;
#175068=CARTESIAN_POINT('Ctrl Pts',(-28.1695141104945,-13.9119580024122,
111.666678700074)) ;
#175069=CARTESIAN_POINT('Ctrl Pts',(-28.095710267544,-13.9119580041773,
111.69090974319)) ;
#175070=CARTESIAN_POINT('Ctrl Pts',(-28.0219064245936,-13.9119580059424,
111.715140786306)) ;
#175071=CARTESIAN_POINT('Ctrl Pts',(-28.001170724837,-13.9486084973951,
111.651983190584)) ;
#175072=CARTESIAN_POINT('Ctrl Pts',(-27.9804350250805,-13.9852589888479,
111.588825594862)) ;
#175073=CARTESIAN_POINT('Ctrl Pts',(-28.0542388680309,-13.9852589870828,
111.564594551746)) ;
#175074=CARTESIAN_POINT('Ctrl Pts',(-28.1280427109814,-13.9852589853178,
111.54036350863)) ;
#175075=CARTESIAN_POINT('Ctrl Pts',(-28.1487784107379,-13.948608493865,
111.603521104352)) ;
#175076=CARTESIAN_POINT('Ctrl Pts',(-28.1927422454497,-14.181257681225,
111.772854625694)) ;
#175077=CARTESIAN_POINT('Ctrl Pts',(-28.209705905835,-14.12830707033,111.824523198175)) ;
#175078=CARTESIAN_POINT('Ctrl Pts',(-28.135902062206,-14.1283070692883,
111.848754239225)) ;
#175079=CARTESIAN_POINT('Ctrl Pts',(-28.0620982185771,-14.1283070682466,
111.872985280274)) ;
#175080=CARTESIAN_POINT('Ctrl Pts',(-28.0451345581918,-14.1812576791416,
111.821316707793)) ;
#175081=CARTESIAN_POINT('Ctrl Pts',(-28.0281708978066,-14.2342082900366,
111.769648135312)) ;
#175082=CARTESIAN_POINT('Ctrl Pts',(-28.1019747414355,-14.2342082910783,
111.745417094263)) ;
#175083=CARTESIAN_POINT('Ctrl Pts',(-28.1757785850644,-14.23420829212,111.721186053214)) ;
#175084=CARTESIAN_POINT('Ctrl Pts',(-28.1927422454497,-14.181257681225,
111.772854625694)) ;
#175085=CARTESIAN_POINT('Ctrl Pts',(-28.25389994631,-14.3592650506284,111.994525378914)) ;
#175086=CARTESIAN_POINT('Ctrl Pts',(-28.2658858395401,-14.2938058183535,
112.031032475836)) ;
#175087=CARTESIAN_POINT('Ctrl Pts',(-28.1920819953039,-14.2938058167003,
112.055263515036)) ;
#175088=CARTESIAN_POINT('Ctrl Pts',(-28.1182781510676,-14.293805815047,
112.079494554236)) ;
#175089=CARTESIAN_POINT('Ctrl Pts',(-28.1062922578376,-14.359265047322,
112.042987457314)) ;
#175090=CARTESIAN_POINT('Ctrl Pts',(-28.0943063646075,-14.4247242795969,
112.006480360391)) ;
#175091=CARTESIAN_POINT('Ctrl Pts',(-28.1681102088437,-14.4247242812501,
111.982249321192)) ;
#175092=CARTESIAN_POINT('Ctrl Pts',(-28.24191405308,-14.4247242829034,111.958018281992)) ;
#175093=CARTESIAN_POINT('Ctrl Pts',(-28.25389994631,-14.3592650506284,111.994525378914)) ;
#175094=CARTESIAN_POINT('Ctrl Pts',(-28.3273391635443,-14.4703402370834,
112.253666401676)) ;
#175095=CARTESIAN_POINT('Ctrl Pts',(-28.3334807725046,-14.3970277006435,
112.272372751686)) ;
#175096=CARTESIAN_POINT('Ctrl Pts',(-28.2596769281304,-14.3970276999611,
112.296603790465)) ;
#175097=CARTESIAN_POINT('Ctrl Pts',(-28.1858730837562,-14.3970276992787,
112.320834829245)) ;
#175098=CARTESIAN_POINT('Ctrl Pts',(-28.1797314747959,-14.4703402357187,
112.302128479236)) ;
#175099=CARTESIAN_POINT('Ctrl Pts',(-28.1735898658356,-14.5436527721586,
112.283422129226)) ;
#175100=CARTESIAN_POINT('Ctrl Pts',(-28.2473937102098,-14.543652772841,
112.259191090447)) ;
#175101=CARTESIAN_POINT('Ctrl Pts',(-28.321197554584,-14.5436527735234,
112.234960051667)) ;
#175102=CARTESIAN_POINT('Ctrl Pts',(-28.3273391635443,-14.4703402370834,
112.253666401676)) ;
#175103=CARTESIAN_POINT('Ctrl Pts',(-28.4071790901361,-14.5059089260168,
112.532398419472)) ;
#175104=CARTESIAN_POINT('Ctrl Pts',(-28.4070188716446,-14.4300045540626,
112.531910419809)) ;
#175105=CARTESIAN_POINT('Ctrl Pts',(-28.3332150280579,-14.4300045543585,
112.556141460987)) ;
#175106=CARTESIAN_POINT('Ctrl Pts',(-28.2594111844711,-14.4300045546544,
112.580372502165)) ;
#175107=CARTESIAN_POINT('Ctrl Pts',(-28.2595714029626,-14.5059089266086,
112.580860501828)) ;
#175108=CARTESIAN_POINT('Ctrl Pts',(-28.259731621454,-14.5818132985628,
112.581348501491)) ;
#175109=CARTESIAN_POINT('Ctrl Pts',(-28.3335354650407,-14.5818132982669,
112.557117460313)) ;
#175110=CARTESIAN_POINT('Ctrl Pts',(-28.4073393086275,-14.581813297971,
112.532886419135)) ;
#175111=CARTESIAN_POINT('Ctrl Pts',(-28.4071790901361,-14.5059089260168,
112.532398419472)) ;
#175112=CARTESIAN_POINT('Ctrl Pts',(-28.4863373455099,-14.4635906108697,
112.808879001028)) ;
#175113=CARTESIAN_POINT('Ctrl Pts',(-28.4799175167862,-14.3905302812958,
112.789325238511)) ;
#175114=CARTESIAN_POINT('Ctrl Pts',(-28.4061136743483,-14.3905302808225,
112.813556283188)) ;
#175115=CARTESIAN_POINT('Ctrl Pts',(-28.3323098319104,-14.3905302803492,
112.837787327865)) ;
#175116=CARTESIAN_POINT('Ctrl Pts',(-28.3387296606341,-14.4635906099231,
112.857341090383)) ;
#175117=CARTESIAN_POINT('Ctrl Pts',(-28.3451494893579,-14.536650939497,
112.8768948529)) ;
#175118=CARTESIAN_POINT('Ctrl Pts',(-28.4189533317957,-14.5366509399703,
112.852663808223)) ;
#175119=CARTESIAN_POINT('Ctrl Pts',(-28.4927571742336,-14.5366509404436,
112.828432763546)) ;
#175120=CARTESIAN_POINT('Ctrl Pts',(-28.4863373455099,-14.4635906108697,
112.808879001028)) ;
#175121=CARTESIAN_POINT('Ctrl Pts',(-28.5590864820887,-14.3462861335646,
113.06597539471)) ;
#175122=CARTESIAN_POINT('Ctrl Pts',(-28.5468426175345,-14.2813098903358,
113.028682558647)) ;
#175123=CARTESIAN_POINT('Ctrl Pts',(-28.4730387765814,-14.2813098862363,
113.052913607847)) ;
#175124=CARTESIAN_POINT('Ctrl Pts',(-28.3992349356284,-14.2813098821367,
113.077144657047)) ;
#175125=CARTESIAN_POINT('Ctrl Pts',(-28.4114788001826,-14.3462861253655,
113.11443749311)) ;
#175126=CARTESIAN_POINT('Ctrl Pts',(-28.4237226647368,-14.4112623685942,
113.151730329173)) ;
#175127=CARTESIAN_POINT('Ctrl Pts',(-28.4975265056898,-14.4112623726938,
113.127499279973)) ;
#175128=CARTESIAN_POINT('Ctrl Pts',(-28.5713303466429,-14.4112623767934,
113.103268230773)) ;
#175129=CARTESIAN_POINT('Ctrl Pts',(-28.5590864820887,-14.3462861335646,
113.06597539471)) ;
#175130=CARTESIAN_POINT('Ctrl Pts',(-28.6190888482877,-14.1620807273187,
113.284252795165)) ;
#175131=CARTESIAN_POINT('Ctrl Pts',(-28.6019025244461,-14.1098718676652,
113.231906025436)) ;
#175132=CARTESIAN_POINT('Ctrl Pts',(-28.5280986845969,-14.1098718563613,
113.256137077998)) ;
#175133=CARTESIAN_POINT('Ctrl Pts',(-28.4542948447477,-14.1098718450575,
113.28036813056)) ;
#175134=CARTESIAN_POINT('Ctrl Pts',(-28.4714811685893,-14.162080704711,
113.332714900289)) ;
#175135=CARTESIAN_POINT('Ctrl Pts',(-28.4886674924309,-14.2142895643646,
113.385061670018)) ;
#175136=CARTESIAN_POINT('Ctrl Pts',(-28.5624713322801,-14.2142895756684,
113.360830617456)) ;
#175137=CARTESIAN_POINT('Ctrl Pts',(-28.6362751721293,-14.2142895869723,
113.336599564894)) ;
#175138=CARTESIAN_POINT('Ctrl Pts',(-28.6190888482877,-14.1620807273187,
113.284252795165)) ;
#175139=CARTESIAN_POINT('Ctrl Pts',(-28.6611716634273,-13.9257450561724,
113.447780698845)) ;
#175140=CARTESIAN_POINT('Ctrl Pts',(-28.6402906964383,-13.8899621379748,
113.384180642091)) ;
#175141=CARTESIAN_POINT('Ctrl Pts',(-28.5664868565058,-13.8899621182589,
113.408411694399)) ;
#175142=CARTESIAN_POINT('Ctrl Pts',(-28.4926830165733,-13.889962098543,
113.432642746707)) ;
#175143=CARTESIAN_POINT('Ctrl Pts',(-28.5135639835622,-13.9257450167406,
113.496242803462)) ;
#175144=CARTESIAN_POINT('Ctrl Pts',(-28.5344449505512,-13.9615279349381,
113.559842860216)) ;
#175145=CARTESIAN_POINT('Ctrl Pts',(-28.6082487904837,-13.961527954654,
113.535611807908)) ;
#175146=CARTESIAN_POINT('Ctrl Pts',(-28.6820526304163,-13.9615279743699,
113.5113807556)) ;
#175147=CARTESIAN_POINT('Ctrl Pts',(-28.6611716634273,-13.9257450561724,
113.447780698845)) ;
#175148=CARTESIAN_POINT('Ctrl Pts',(-28.6819629618819,-13.6518932520307,
113.54663327576)) ;
#175149=CARTESIAN_POINT('Ctrl Pts',(-28.6588649077152,-13.6351791904555,
113.476280329019)) ;
#175150=CARTESIAN_POINT('Ctrl Pts',(-28.5850610666532,-13.6351791600229,
113.500511377887)) ;
#175151=CARTESIAN_POINT('Ctrl Pts',(-28.5112572255911,-13.6351791295903,
113.524742426755)) ;
#175152=CARTESIAN_POINT('Ctrl Pts',(-28.5343552797579,-13.6518931911655,
113.595095373495)) ;
#175153=CARTESIAN_POINT('Ctrl Pts',(-28.5574533339246,-13.6686072527407,
113.665448320236)) ;
#175154=CARTESIAN_POINT('Ctrl Pts',(-28.6312571749866,-13.6686072831733,
113.641217271368)) ;
#175155=CARTESIAN_POINT('Ctrl Pts',(-28.7050610160487,-13.6686073136059,
113.6169862225)) ;
#175156=CARTESIAN_POINT('Ctrl Pts',(-28.6819629618819,-13.6518932520307,
113.54663327576)) ;
#175157=CARTESIAN_POINT('Ctrl Pts',(-28.6788957975661,-13.361350209501,
113.572794442411)) ;
#175158=CARTESIAN_POINT('Ctrl Pts',(-28.6552438087377,-13.3648978107094,
113.500754299894)) ;
#175159=CARTESIAN_POINT('Ctrl Pts',(-28.58143996491,-13.3648977704052,113.524985340338)) ;
#175160=CARTESIAN_POINT('Ctrl Pts',(-28.5076361210823,-13.364897730101,
113.549216380782)) ;
#175161=CARTESIAN_POINT('Ctrl Pts',(-28.5312881099107,-13.3613501288926,
113.621256523299)) ;
#175162=CARTESIAN_POINT('Ctrl Pts',(-28.5549400987392,-13.3578025276842,
113.693296665815)) ;
#175163=CARTESIAN_POINT('Ctrl Pts',(-28.6287439425669,-13.3578025679884,
113.669065625371)) ;
#175164=CARTESIAN_POINT('Ctrl Pts',(-28.7025477863946,-13.3578026082926,
113.644834584927)) ;
#175165=CARTESIAN_POINT('Ctrl Pts',(-28.6788957975661,-13.361350209501,
113.572794442411)) ;
#175166=CARTESIAN_POINT('Ctrl Pts',(-28.6515753370969,-13.0754523993138,
113.525017916636)) ;
#175167=CARTESIAN_POINT('Ctrl Pts',(-28.629063419331,-13.0989663539562,
113.456450246463)) ;
#175168=CARTESIAN_POINT('Ctrl Pts',(-28.5552595713404,-13.0989663074807,
113.480681274228)) ;
#175169=CARTESIAN_POINT('Ctrl Pts',(-28.4814557233498,-13.0989662610053,
113.504912301992)) ;
#175170=CARTESIAN_POINT('Ctrl Pts',(-28.5039676411157,-13.0754523063629,
113.573479972165)) ;
#175171=CARTESIAN_POINT('Ctrl Pts',(-28.5264795588817,-13.0519383517206,
113.642047642338)) ;
#175172=CARTESIAN_POINT('Ctrl Pts',(-28.6002834068723,-13.051938398196,
113.617816614573)) ;
#175173=CARTESIAN_POINT('Ctrl Pts',(-28.6740872548629,-13.0519384446715,
113.593585586809)) ;
#175174=CARTESIAN_POINT('Ctrl Pts',(-28.6515753370969,-13.0754523993138,
113.525017916636)) ;
#175175=CARTESIAN_POINT('Ctrl Pts',(-28.6012644802897,-12.8139381990977,
113.407216883436)) ;
#175176=CARTESIAN_POINT('Ctrl Pts',(-28.5814994051075,-12.8557446579336,
113.347015652409)) ;
#175177=CARTESIAN_POINT('Ctrl Pts',(-28.5076955520102,-12.8557446099044,
113.371246664619)) ;
#175178=CARTESIAN_POINT('Ctrl Pts',(-28.4338916989129,-12.8557445618753,
113.395477676829)) ;
#175179=CARTESIAN_POINT('Ctrl Pts',(-28.4536567740952,-12.8139381030394,
113.455678907856)) ;
#175180=CARTESIAN_POINT('Ctrl Pts',(-28.4734218492774,-12.7721316442036,
113.515880138883)) ;
#175181=CARTESIAN_POINT('Ctrl Pts',(-28.5472257023747,-12.7721316922327,
113.491649126673)) ;
#175182=CARTESIAN_POINT('Ctrl Pts',(-28.621029555472,-12.7721317402619,
113.467418114463)) ;
#175183=CARTESIAN_POINT('Ctrl Pts',(-28.6012644802897,-12.8139381990977,
113.407216883436)) ;
#175184=CARTESIAN_POINT('Ctrl Pts',(-28.530312795938,-12.5948180944483,
113.22672545771)) ;
#175185=CARTESIAN_POINT('Ctrl Pts',(-28.5147357585645,-12.6519838381849,
113.17928031392)) ;
#175186=CARTESIAN_POINT('Ctrl Pts',(-28.4409318994849,-12.6519837938663,
113.20351130791)) ;
#175187=CARTESIAN_POINT('Ctrl Pts',(-28.3671280404052,-12.6519837495477,
113.227742301899)) ;
#175188=CARTESIAN_POINT('Ctrl Pts',(-28.3827050777788,-12.5948180058111,
113.275187445688)) ;
#175189=CARTESIAN_POINT('Ctrl Pts',(-28.3982821151524,-12.5376522620745,
113.322632589477)) ;
#175190=CARTESIAN_POINT('Ctrl Pts',(-28.472085974232,-12.537652306393,113.298401595488)) ;
#175191=CARTESIAN_POINT('Ctrl Pts',(-28.5458898333115,-12.5376523507116,
113.274170601499)) ;
#175192=CARTESIAN_POINT('Ctrl Pts',(-28.530312795938,-12.5948180944483,
113.22672545771)) ;
#175193=CARTESIAN_POINT('Ctrl Pts',(-28.4441820785393,-12.4362800048722,
112.999678378)) ;
#175194=CARTESIAN_POINT('Ctrl Pts',(-28.4338657622434,-12.5045968794166,
112.968256541675)) ;
#175195=CARTESIAN_POINT('Ctrl Pts',(-28.3600618982417,-12.5045968472639,
112.992487520672)) ;
#175196=CARTESIAN_POINT('Ctrl Pts',(-28.28625803424,-12.5045968151111,113.016718499669)) ;
#175197=CARTESIAN_POINT('Ctrl Pts',(-28.2965743505358,-12.4362799405667,
113.048140335994)) ;
#175198=CARTESIAN_POINT('Ctrl Pts',(-28.3068906668317,-12.3679630660223,
113.079562172319)) ;
#175199=CARTESIAN_POINT('Ctrl Pts',(-28.3806945308334,-12.367963098175,
113.055331193322)) ;
#175200=CARTESIAN_POINT('Ctrl Pts',(-28.4544983948351,-12.3679631303278,
113.031100214324)) ;
#175201=CARTESIAN_POINT('Ctrl Pts',(-28.4441820785393,-12.4362800048722,
112.999678378)) ;
#175202=CARTESIAN_POINT('Ctrl Pts',(-28.3470854955192,-12.346922078608,
112.739452029468)) ;
#175203=CARTESIAN_POINT('Ctrl Pts',(-28.3427983341584,-12.4215768384595,
112.726394026123)) ;
#175204=CARTESIAN_POINT('Ctrl Pts',(-28.2689944658137,-12.4215768235296,
112.750624991892)) ;
#175205=CARTESIAN_POINT('Ctrl Pts',(-28.195190597469,-12.4215768085998,
112.774855957661)) ;
#175206=CARTESIAN_POINT('Ctrl Pts',(-28.1994777588298,-12.3469220487482,
112.787913961007)) ;
#175207=CARTESIAN_POINT('Ctrl Pts',(-28.2037649201905,-12.2722672888967,
112.800971964352)) ;
#175208=CARTESIAN_POINT('Ctrl Pts',(-28.2775687885352,-12.2722673038266,
112.776740998583)) ;
#175209=CARTESIAN_POINT('Ctrl Pts',(-28.3513726568799,-12.2722673187564,
112.752510032814)) ;
#175210=CARTESIAN_POINT('Ctrl Pts',(-28.3470854955192,-12.346922078608,
112.739452029468)) ;
#175211=CARTESIAN_POINT('Ctrl Pts',(-28.2458303935604,-12.3346186385411,
112.466505819017)) ;
#175212=CARTESIAN_POINT('Ctrl Pts',(-28.2478725713665,-12.4102408597983,
112.472725961409)) ;
#175213=CARTESIAN_POINT('Ctrl Pts',(-28.1740687006002,-12.4102408673589,
112.496956919802)) ;
#175214=CARTESIAN_POINT('Ctrl Pts',(-28.1002648298339,-12.4102408749196,
112.521187878196)) ;
#175215=CARTESIAN_POINT('Ctrl Pts',(-28.0982226520278,-12.3346186536624,
112.514967735804)) ;
#175216=CARTESIAN_POINT('Ctrl Pts',(-28.0961804742218,-12.2589964324052,
112.508747593412)) ;
#175217=CARTESIAN_POINT('Ctrl Pts',(-28.1699843449881,-12.2589964248446,
112.484516635018)) ;
#175218=CARTESIAN_POINT('Ctrl Pts',(-28.2437882157544,-12.2589964172839,
112.460285676625)) ;
#175219=CARTESIAN_POINT('Ctrl Pts',(-28.2458303935604,-12.3346186385411,
112.466505819017)) ;
#175220=CARTESIAN_POINT('Ctrl Pts',(-28.1468306373285,-12.3998225687949,
112.200422951598)) ;
#175221=CARTESIAN_POINT('Ctrl Pts',(-28.1550539935489,-12.4710025852177,
112.225469965997)) ;
#175222=CARTESIAN_POINT('Ctrl Pts',(-28.0812501226881,-12.4710026178869,
112.249700924103)) ;
#175223=CARTESIAN_POINT('Ctrl Pts',(-28.0074462518273,-12.4710026505561,
112.273931882208)) ;
#175224=CARTESIAN_POINT('Ctrl Pts',(-27.9992228956068,-12.3998226341332,
112.248884867808)) ;
#175225=CARTESIAN_POINT('Ctrl Pts',(-27.9909995393864,-12.3286426177104,
112.223837853409)) ;
#175226=CARTESIAN_POINT('Ctrl Pts',(-28.0648034102472,-12.3286425850412,
112.199606895303)) ;
#175227=CARTESIAN_POINT('Ctrl Pts',(-28.138607281108,-12.328642552372,112.175375937198)) ;
#175228=CARTESIAN_POINT('Ctrl Pts',(-28.1468306373285,-12.3998225687949,
112.200422951598)) ;
#175229=CARTESIAN_POINT('Ctrl Pts',(-28.056410402061,-12.5378477500096,
111.960460656517)) ;
#175230=CARTESIAN_POINT('Ctrl Pts',(-28.0702251886927,-12.599495230749,
112.002538265681)) ;
#175231=CARTESIAN_POINT('Ctrl Pts',(-27.9964213202855,-12.5994952885301,
112.026769231259)) ;
#175232=CARTESIAN_POINT('Ctrl Pts',(-27.9226174518782,-12.5994953463112,
112.051000196837)) ;
#175233=CARTESIAN_POINT('Ctrl Pts',(-27.9088026652464,-12.5378478655717,
112.008922587674)) ;
#175234=CARTESIAN_POINT('Ctrl Pts',(-27.8949878786146,-12.4762003848323,
111.966844978511)) ;
#175235=CARTESIAN_POINT('Ctrl Pts',(-27.9687917470219,-12.4762003270512,
111.942614012932)) ;
#175236=CARTESIAN_POINT('Ctrl Pts',(-28.0425956154292,-12.4762002692701,
111.918383047354)) ;
#175237=CARTESIAN_POINT('Ctrl Pts',(-28.056410402061,-12.5378477500096,
111.960460656517)) ;
#175238=CARTESIAN_POINT('Ctrl Pts',(-27.9801392408926,-12.7392396507352,
111.763656314593)) ;
#175239=CARTESIAN_POINT('Ctrl Pts',(-27.9985645664945,-12.7869171442881,
111.81977688147)) ;
#175240=CARTESIAN_POINT('Ctrl Pts',(-27.9247607029675,-12.7869172246325,
111.844007861913)) ;
#175241=CARTESIAN_POINT('Ctrl Pts',(-27.8509568394405,-12.786917304977,
111.868238842356)) ;
#175242=CARTESIAN_POINT('Ctrl Pts',(-27.8325315138385,-12.7392398114241,
111.812118275479)) ;
#175243=CARTESIAN_POINT('Ctrl Pts',(-27.8141061882366,-12.6915623178712,
111.755997708602)) ;
#175244=CARTESIAN_POINT('Ctrl Pts',(-27.8879100517636,-12.6915622375267,
111.731766728159)) ;
#175245=CARTESIAN_POINT('Ctrl Pts',(-27.9617139152906,-12.6915621571823,
111.707535747716)) ;
#175246=CARTESIAN_POINT('Ctrl Pts',(-27.9801392408926,-12.7392396507352,
111.763656314593)) ;
#175247=CARTESIAN_POINT('Ctrl Pts',(-27.9229728782281,-12.989236405783,
111.625017894805)) ;
#175248=CARTESIAN_POINT('Ctrl Pts',(-27.9446822619997,-13.019530175167,
111.69114117293)) ;
#175249=CARTESIAN_POINT('Ctrl Pts',(-27.8708784055218,-13.019530272485,
111.715372174843)) ;
#175250=CARTESIAN_POINT('Ctrl Pts',(-27.7970745490438,-13.0195303698031,
111.739603176756)) ;
#175251=CARTESIAN_POINT('Ctrl Pts',(-27.7753651652723,-12.9892366004191,
111.673479898632)) ;
#175252=CARTESIAN_POINT('Ctrl Pts',(-27.7536557815007,-12.9589428310352,
111.607356620507)) ;
#175253=CARTESIAN_POINT('Ctrl Pts',(-27.8274596379786,-12.9589427337171,
111.583125618594)) ;
#175254=CARTESIAN_POINT('Ctrl Pts',(-27.9012634944566,-12.9589426363991,
111.558894616681)) ;
#175255=CARTESIAN_POINT('Ctrl Pts',(-27.9229728782281,-12.989236405783,
111.625017894805)) ;
#175256=CARTESIAN_POINT('Ctrl Pts',(-27.8882165238537,-13.269049028932,
111.554529970124)) ;
#175257=CARTESIAN_POINT('Ctrl Pts',(-27.9116524234391,-13.279851801729,
111.625911936813)) ;
#175258=CARTESIAN_POINT('Ctrl Pts',(-27.8378485754109,-13.2798519083315,
111.650142964463)) ;
#175259=CARTESIAN_POINT('Ctrl Pts',(-27.7640447273828,-13.279852014934,
111.674373992113)) ;
#175260=CARTESIAN_POINT('Ctrl Pts',(-27.7406088277974,-13.269049242137,
111.602992025424)) ;
#175261=CARTESIAN_POINT('Ctrl Pts',(-27.717172928212,-13.2582464693401,
111.531610058736)) ;
#175262=CARTESIAN_POINT('Ctrl Pts',(-27.7909767762402,-13.2582463627375,
111.507379031086)) ;
#175263=CARTESIAN_POINT('Ctrl Pts',(-27.8647806242683,-13.258246256135,
111.483148003436)) ;
#175264=CARTESIAN_POINT('Ctrl Pts',(-27.8882165238537,-13.269049028932,
111.554529970124)) ;
#175265=CARTESIAN_POINT('Ctrl Pts',(-27.8773822820719,-13.560604521515,
111.557039247534)) ;
#175266=CARTESIAN_POINT('Ctrl Pts',(-27.9008745338674,-13.5510680943663,
111.628592853945)) ;
#175267=CARTESIAN_POINT('Ctrl Pts',(-27.827070694905,-13.5510682019353,
111.652823909208)) ;
#175268=CARTESIAN_POINT('Ctrl Pts',(-27.7532668559424,-13.5510683095042,
111.67705496447)) ;
#175269=CARTESIAN_POINT('Ctrl Pts',(-27.7297746041469,-13.5606047366529,
111.605501358059)) ;
#175270=CARTESIAN_POINT('Ctrl Pts',(-27.7062823523514,-13.5701411638016,
111.533947751647)) ;
#175271=CARTESIAN_POINT('Ctrl Pts',(-27.7800861913139,-13.5701410562327,
111.509716696385)) ;
#175272=CARTESIAN_POINT('Ctrl Pts',(-27.8538900302764,-13.5701409486637,
111.485485641123)) ;
#175273=CARTESIAN_POINT('Ctrl Pts',(-27.8773822820719,-13.560604521515,
111.557039247534)) ;
#175274=CARTESIAN_POINT('Ctrl Pts',(-27.8908274487406,-13.8423158077137,
111.633558215579)) ;
#175275=CARTESIAN_POINT('Ctrl Pts',(-27.912680022347,-13.8130971975032,
111.700117626799)) ;
#175276=CARTESIAN_POINT('Ctrl Pts',(-27.8388761921,-13.8130972967894,111.724348708607)) ;
#175277=CARTESIAN_POINT('Ctrl Pts',(-27.765072361853,-13.8130973960757,
111.748579790416)) ;
#175278=CARTESIAN_POINT('Ctrl Pts',(-27.7432197882467,-13.8423160062862,
111.682020379196)) ;
#175279=CARTESIAN_POINT('Ctrl Pts',(-27.7213672146404,-13.8715346164967,
111.615460967976)) ;
#175280=CARTESIAN_POINT('Ctrl Pts',(-27.7951710448874,-13.8715345172104,
111.591229886167)) ;
#175281=CARTESIAN_POINT('Ctrl Pts',(-27.8689748751343,-13.8715344179242,
111.566998804359)) ;
#175282=CARTESIAN_POINT('Ctrl Pts',(-27.8908274487406,-13.8423158077137,
111.633558215579)) ;
#175283=CARTESIAN_POINT('Ctrl Pts',(-27.9264541508921,-14.0920492190499,
111.777413603601)) ;
#175284=CARTESIAN_POINT('Ctrl Pts',(-27.9451204832836,-14.0453516515009,
111.834268238205)) ;
#175285=CARTESIAN_POINT('Ctrl Pts',(-27.8713166605116,-14.0453517349523,
111.858499342782)) ;
#175286=CARTESIAN_POINT('Ctrl Pts',(-27.7975128377397,-14.0453518184037,
111.882730447358)) ;
#175287=CARTESIAN_POINT('Ctrl Pts',(-27.7788465053482,-14.0920493859528,
111.825875812753)) ;
#175288=CARTESIAN_POINT('Ctrl Pts',(-27.7601801729567,-14.1387469535018,
111.769021178149)) ;
#175289=CARTESIAN_POINT('Ctrl Pts',(-27.8339839957287,-14.1387468700504,
111.744790073572)) ;
#175290=CARTESIAN_POINT('Ctrl Pts',(-27.9077878185007,-14.138746786599,
111.720558968996)) ;
#175291=CARTESIAN_POINT('Ctrl Pts',(-27.9264541508921,-14.0920492190499,
111.777413603601)) ;
#175292=CARTESIAN_POINT('Ctrl Pts',(-27.9814414275838,-14.2950965364046,
111.980481540082)) ;
#175293=CARTESIAN_POINT('Ctrl Pts',(-27.9955603817965,-14.2341530477557,
112.02348559453)) ;
#175294=CARTESIAN_POINT('Ctrl Pts',(-27.9217565644726,-14.2341531086755,
112.0477167157)) ;
#175295=CARTESIAN_POINT('Ctrl Pts',(-27.8479527471487,-14.2341531695953,
112.07194783687)) ;
#175296=CARTESIAN_POINT('Ctrl Pts',(-27.833833792936,-14.2950966582441,
112.028943782423)) ;
#175297=CARTESIAN_POINT('Ctrl Pts',(-27.8197148387233,-14.3560401468929,
111.985939727975)) ;
#175298=CARTESIAN_POINT('Ctrl Pts',(-27.8935186560472,-14.3560400859732,
111.961708606805)) ;
#175299=CARTESIAN_POINT('Ctrl Pts',(-27.9673224733711,-14.3560400250534,
111.937477485635)) ;
#175300=CARTESIAN_POINT('Ctrl Pts',(-27.9814414275838,-14.2950965364046,
111.980481540082)) ;
#175301=CARTESIAN_POINT('Ctrl Pts',(-28.0507461501417,-14.434335219557,
112.227053017501)) ;
#175302=CARTESIAN_POINT('Ctrl Pts',(-28.0593134198574,-14.3635791231233,
112.25314753681)) ;
#175303=CARTESIAN_POINT('Ctrl Pts',(-27.9855096054518,-14.3635791582218,
112.277378666869)) ;
#175304=CARTESIAN_POINT('Ctrl Pts',(-27.9117057910462,-14.3635791933204,
112.301609796927)) ;
#175305=CARTESIAN_POINT('Ctrl Pts',(-27.9031385213306,-14.4343352897541,
112.275515277618)) ;
#175306=CARTESIAN_POINT('Ctrl Pts',(-27.8945712516149,-14.5050913861879,
112.249420758309)) ;
#175307=CARTESIAN_POINT('Ctrl Pts',(-27.9683750660205,-14.5050913510893,
112.22518962825)) ;
#175308=CARTESIAN_POINT('Ctrl Pts',(-28.0421788804261,-14.5050913159907,
112.200958498192)) ;
#175309=CARTESIAN_POINT('Ctrl Pts',(-28.0507461501417,-14.434335219557,
112.227053017501)) ;
#175310=CARTESIAN_POINT('Ctrl Pts',(-28.1282740613558,-14.5007530721094,
112.498487082343)) ;
#175311=CARTESIAN_POINT('Ctrl Pts',(-28.1307109212733,-14.4252541131167,
112.505909362619)) ;
#175312=CARTESIAN_POINT('Ctrl Pts',(-28.0569071075311,-14.4252541219683,
112.530140494699)) ;
#175313=CARTESIAN_POINT('Ctrl Pts',(-27.9831032937888,-14.4252541308198,
112.554371626778)) ;
#175314=CARTESIAN_POINT('Ctrl Pts',(-27.9806664338714,-14.5007530898126,
112.546949346501)) ;
#175315=CARTESIAN_POINT('Ctrl Pts',(-27.9782295739539,-14.5762520488053,
112.539527066225)) ;
#175316=CARTESIAN_POINT('Ctrl Pts',(-28.0520333876961,-14.5762520399537,
112.515295934145)) ;
#175317=CARTESIAN_POINT('Ctrl Pts',(-28.1258372014383,-14.5762520311022,
112.491064802066)) ;
#175318=CARTESIAN_POINT('Ctrl Pts',(-28.1282740613558,-14.5007530721094,
112.498487082343)) ;
#175319=CARTESIAN_POINT('Ctrl Pts',(-28.2086863670135,-14.4901437351793,
112.778942561062)) ;
#175320=CARTESIAN_POINT('Ctrl Pts',(-28.204777466643,-14.415271701562,112.767036679503)) ;
#175321=CARTESIAN_POINT('Ctrl Pts',(-28.1309736506996,-14.4152716856427,
112.791267804878)) ;
#175322=CARTESIAN_POINT('Ctrl Pts',(-28.0571698347562,-14.4152716697234,
112.815498930253)) ;
#175323=CARTESIAN_POINT('Ctrl Pts',(-28.0610787351267,-14.4901437033406,
112.827404811812)) ;
#175324=CARTESIAN_POINT('Ctrl Pts',(-28.0649876354972,-14.5650157369579,
112.83931069337)) ;
#175325=CARTESIAN_POINT('Ctrl Pts',(-28.1387914514406,-14.5650157528772,
112.815079567995)) ;
#175326=CARTESIAN_POINT('Ctrl Pts',(-28.2125952673839,-14.5650157687965,
112.79084844262)) ;
#175327=CARTESIAN_POINT('Ctrl Pts',(-28.2086863670135,-14.4901437351793,
112.778942561062)) ;
#175328=CARTESIAN_POINT('Ctrl Pts',(-28.2850462508329,-14.402041943339,
113.047107750682)) ;
#175329=CARTESIAN_POINT('Ctrl Pts',(-28.2750637657936,-14.3332076954044,
113.016702710337)) ;
#175330=CARTESIAN_POINT('Ctrl Pts',(-28.2012599453933,-14.3332076598222,
113.040933822138)) ;
#175331=CARTESIAN_POINT('Ctrl Pts',(-28.127456124993,-14.33320762424,113.065164933938)) ;
#175332=CARTESIAN_POINT('Ctrl Pts',(-28.1374386100323,-14.4020418721746,
113.095569974282)) ;
#175333=CARTESIAN_POINT('Ctrl Pts',(-28.1474210950715,-14.4708761201093,
113.125975014626)) ;
#175334=CARTESIAN_POINT('Ctrl Pts',(-28.2212249154718,-14.4708761556915,
113.101743902826)) ;
#175335=CARTESIAN_POINT('Ctrl Pts',(-28.2950287358721,-14.4708761912736,
113.077512791026)) ;
#175336=CARTESIAN_POINT('Ctrl Pts',(-28.2850462508329,-14.402041943339,
113.047107750682)) ;
#175337=CARTESIAN_POINT('Ctrl Pts',(-28.3507008692899,-14.243691286176,
113.282525581938)) ;
#175338=CARTESIAN_POINT('Ctrl Pts',(-28.3353858951182,-14.18580899599,113.23587864023)) ;
#175339=CARTESIAN_POINT('Ctrl Pts',(-28.2615820692535,-14.1858089469242,
113.260109735386)) ;
#175340=CARTESIAN_POINT('Ctrl Pts',(-28.1877782433888,-14.1858088978584,
113.284340830543)) ;
#175341=CARTESIAN_POINT('Ctrl Pts',(-28.2030932175605,-14.2436911880444,
113.33098777225)) ;
#175342=CARTESIAN_POINT('Ctrl Pts',(-28.2184081917321,-14.3015734782304,
113.377634713958)) ;
#175343=CARTESIAN_POINT('Ctrl Pts',(-28.2922120175968,-14.3015735272962,
113.353403618801)) ;
#175344=CARTESIAN_POINT('Ctrl Pts',(-28.3660158434615,-14.301573576362,
113.329172523645)) ;
#175345=CARTESIAN_POINT('Ctrl Pts',(-28.3507008692899,-14.243691286176,
113.282525581938)) ;
#175346=CARTESIAN_POINT('Ctrl Pts',(-28.4004336980104,-14.0272168477211,
113.469327044574)) ;
#175347=CARTESIAN_POINT('Ctrl Pts',(-28.3808923587898,-13.9843615039812,
113.409807276976)) ;
#175348=CARTESIAN_POINT('Ctrl Pts',(-28.3070885270855,-13.9843614472663,
113.434038354347)) ;
#175349=CARTESIAN_POINT('Ctrl Pts',(-28.2332846953813,-13.9843613905514,
113.458269431717)) ;
#175350=CARTESIAN_POINT('Ctrl Pts',(-28.252826034602,-14.0272167342913,
113.517789199314)) ;
#175351=CARTESIAN_POINT('Ctrl Pts',(-28.2723673738227,-14.0700720780313,
113.577308966911)) ;
#175352=CARTESIAN_POINT('Ctrl Pts',(-28.3461712055269,-14.0700721347462,
113.553077889541)) ;
#175353=CARTESIAN_POINT('Ctrl Pts',(-28.4199750372311,-14.0700721914611,
113.528846812171)) ;
#175354=CARTESIAN_POINT('Ctrl Pts',(-28.4004336980104,-14.0272168477211,
113.469327044574)) ;
#175355=CARTESIAN_POINT('Ctrl Pts',(-28.4302808069805,-13.7664028194368,
113.595698173527)) ;
#175356=CARTESIAN_POINT('Ctrl Pts',(-28.4078921270372,-13.7416926429616,
113.527505865666)) ;
#175357=CARTESIAN_POINT('Ctrl Pts',(-28.3340882893571,-13.7416925860971,
113.551736924834)) ;
#175358=CARTESIAN_POINT('Ctrl Pts',(-28.260284451677,-13.7416925292327,
113.575967984003)) ;
#175359=CARTESIAN_POINT('Ctrl Pts',(-28.2826731316204,-13.7664027057079,
113.644160291865)) ;
#175360=CARTESIAN_POINT('Ctrl Pts',(-28.3050618115637,-13.791112882183,
113.712352599726)) ;
#175361=CARTESIAN_POINT('Ctrl Pts',(-28.3788656492438,-13.7911129390475,
113.688121540558)) ;
#175362=CARTESIAN_POINT('Ctrl Pts',(-28.4526694869239,-13.7911129959119,
113.663890481389)) ;
#175363=CARTESIAN_POINT('Ctrl Pts',(-28.4302808069805,-13.7664028194368,
113.595698173527)) ;
#175364=CARTESIAN_POINT('Ctrl Pts',(-28.4370991249928,-13.4798811075686,
113.652008520853)) ;
#175365=CARTESIAN_POINT('Ctrl Pts',(-28.4134648567007,-13.4751386073872,
113.580022352038)) ;
#175366=CARTESIAN_POINT('Ctrl Pts',(-28.3396610138886,-13.4751385570953,
113.604253395576)) ;
#175367=CARTESIAN_POINT('Ctrl Pts',(-28.2658571710766,-13.4751385068035,
113.628484439113)) ;
#175368=CARTESIAN_POINT('Ctrl Pts',(-28.2894914393687,-13.4798810069848,
113.700470607928)) ;
#175369=CARTESIAN_POINT('Ctrl Pts',(-28.3131257076607,-13.4846235071661,
113.772456776744)) ;
#175370=CARTESIAN_POINT('Ctrl Pts',(-28.3869295504728,-13.484623557458,
113.748225733206)) ;
#175371=CARTESIAN_POINT('Ctrl Pts',(-28.4607333932849,-13.4846236077499,
113.723994689669)) ;
#175372=CARTESIAN_POINT('Ctrl Pts',(-28.4370991249928,-13.4798811075686,
113.652008520853)) ;
#175373=CARTESIAN_POINT('Ctrl Pts',(-28.4194035357479,-13.1885796838075,
113.633702115265)) ;
#175374=CARTESIAN_POINT('Ctrl Pts',(-28.3962323278668,-13.2041693777773,
113.563126353939)) ;
#175375=CARTESIAN_POINT('Ctrl Pts',(-28.3224284815918,-13.2041693384602,
113.587357386929)) ;
#175376=CARTESIAN_POINT('Ctrl Pts',(-28.2486246353168,-13.2041692991432,
113.611588419919)) ;
#175377=CARTESIAN_POINT('Ctrl Pts',(-28.2717958431979,-13.1885796051734,
113.682164181245)) ;
#175378=CARTESIAN_POINT('Ctrl Pts',(-28.294967051079,-13.1729899112036,
113.75273994257)) ;
#175379=CARTESIAN_POINT('Ctrl Pts',(-28.368770897354,-13.1729899505207,
113.72850890958)) ;
#175380=CARTESIAN_POINT('Ctrl Pts',(-28.442574743629,-13.1729899898377,
113.70427787659)) ;
#175381=CARTESIAN_POINT('Ctrl Pts',(-28.4194035357479,-13.1885796838075,
113.633702115265)) ;
#175382=CARTESIAN_POINT('Ctrl Pts',(-28.378412477973,-12.9166253502417,
113.544054690634)) ;
#175383=CARTESIAN_POINT('Ctrl Pts',(-28.3573399589958,-12.9512269476541,
113.479871197205)) ;
#175384=CARTESIAN_POINT('Ctrl Pts',(-28.2835361104725,-12.951226917539,
113.504102223347)) ;
#175385=CARTESIAN_POINT('Ctrl Pts',(-28.2097322619491,-12.951226887424,
113.528333249489)) ;
#175386=CARTESIAN_POINT('Ctrl Pts',(-28.2308047809263,-12.9166252900117,
113.592516742918)) ;
#175387=CARTESIAN_POINT('Ctrl Pts',(-28.2518772999035,-12.8820236925993,
113.656700236347)) ;
#175388=CARTESIAN_POINT('Ctrl Pts',(-28.3256811484268,-12.8820237227144,
113.632469210205)) ;
#175389=CARTESIAN_POINT('Ctrl Pts',(-28.3994849969502,-12.8820237528294,
113.608238184063)) ;
#175390=CARTESIAN_POINT('Ctrl Pts',(-28.378412477973,-12.9166253502417,
113.544054690634)) ;
#175391=CARTESIAN_POINT('Ctrl Pts',(-28.3154270405176,-12.6775835687805,
113.387804302381)) ;
#175392=CARTESIAN_POINT('Ctrl Pts',(-28.2979837813993,-12.7289285556427,
113.334674949088)) ;
#175393=CARTESIAN_POINT('Ctrl Pts',(-28.224179932538,-12.728928538127,113.358905974201)) ;
#175394=CARTESIAN_POINT('Ctrl Pts',(-28.1503760836767,-12.7289285206112,
113.383136999314)) ;
#175395=CARTESIAN_POINT('Ctrl Pts',(-28.167819342795,-12.6775835337489,
113.436266352606)) ;
#175396=CARTESIAN_POINT('Ctrl Pts',(-28.1852626019133,-12.6262385468866,
113.489395705899)) ;
#175397=CARTESIAN_POINT('Ctrl Pts',(-28.2590664507746,-12.6262385644024,
113.465164680786)) ;
#175398=CARTESIAN_POINT('Ctrl Pts',(-28.3328702996358,-12.6262385819182,
113.440933655674)) ;
#175399=CARTESIAN_POINT('Ctrl Pts',(-28.3154270405176,-12.6775835687805,
113.387804302381)) ;
#175400=CARTESIAN_POINT('Ctrl Pts',(-28.2345655221718,-12.4925681740676,
113.177035535843)) ;
#175401=CARTESIAN_POINT('Ctrl Pts',(-28.2220068985588,-12.5569096995895,
113.138783994323)) ;
#175402=CARTESIAN_POINT('Ctrl Pts',(-28.1482030506511,-12.5569096913385,
113.16301502234)) ;
#175403=CARTESIAN_POINT('Ctrl Pts',(-28.0743992027434,-12.5569096830874,
113.187246050357)) ;
#175404=CARTESIAN_POINT('Ctrl Pts',(-28.0869578263564,-12.4925681575655,
113.225497591877)) ;
#175405=CARTESIAN_POINT('Ctrl Pts',(-28.0995164499695,-12.4282266320435,
113.263749133397)) ;
#175406=CARTESIAN_POINT('Ctrl Pts',(-28.1733202978772,-12.4282266402946,
113.23951810538)) ;
#175407=CARTESIAN_POINT('Ctrl Pts',(-28.2471241457849,-12.4282266485456,
113.215287077363)) ;
#175408=CARTESIAN_POINT('Ctrl Pts',(-28.2345655221718,-12.4925681740676,
113.177035535843)) ;
#175409=CARTESIAN_POINT('Ctrl Pts',(-28.1415965309447,-12.3743553948694,
112.929153696932)) ;
#175410=CARTESIAN_POINT('Ctrl Pts',(-28.1347803018979,-12.4470477080891,
112.908392562837)) ;
#175411=CARTESIAN_POINT('Ctrl Pts',(-28.0609764551353,-12.447047705519,
112.932623594341)) ;
#175412=CARTESIAN_POINT('Ctrl Pts',(-27.9871726083727,-12.4470477029489,
112.956854625846)) ;
#175413=CARTESIAN_POINT('Ctrl Pts',(-27.9939888374195,-12.3743553897291,
112.977615759942)) ;
#175414=CARTESIAN_POINT('Ctrl Pts',(-28.0008050664662,-12.3016630765093,
112.998376894037)) ;
#175415=CARTESIAN_POINT('Ctrl Pts',(-28.0746089132289,-12.3016630790795,
112.974145862532)) ;
#175416=CARTESIAN_POINT('Ctrl Pts',(-28.1484127599915,-12.3016630816496,
112.949914831028)) ;
#175417=CARTESIAN_POINT('Ctrl Pts',(-28.1415965309447,-12.3743553948694,
112.929153696932)) ;
#175418=CARTESIAN_POINT('Ctrl Pts',(-28.0408341461004,-12.3300586716913,
112.657878333238)) ;
#175419=CARTESIAN_POINT('Ctrl Pts',(-28.0403061969979,-12.4059540802535,
112.656270285379)) ;
#175420=CARTESIAN_POINT('Ctrl Pts',(-27.9665023523273,-12.4059540807321,
112.680501323255)) ;
#175421=CARTESIAN_POINT('Ctrl Pts',(-27.8926985076568,-12.4059540812107,
112.704732361132)) ;
#175422=CARTESIAN_POINT('Ctrl Pts',(-27.8932264567592,-12.3300586726485,
112.706340408992)) ;
#175423=CARTESIAN_POINT('Ctrl Pts',(-27.8937544058617,-12.2541632640863,
112.707948456852)) ;
#175424=CARTESIAN_POINT('Ctrl Pts',(-27.9675582505323,-12.2541632636077,
112.683717418975)) ;
#175425=CARTESIAN_POINT('Ctrl Pts',(-28.0413620952029,-12.254163263129,
112.659486381098)) ;
#175426=CARTESIAN_POINT('Ctrl Pts',(-28.0408341461004,-12.3300586716913,
112.657878333238)) ;
#175427=CARTESIAN_POINT('Ctrl Pts',(-27.9401092157344,-12.3643855283945,
112.386554127362)) ;
#175428=CARTESIAN_POINT('Ctrl Pts',(-27.9458798751018,-12.4379977305632,
112.404130624705)) ;
#175429=CARTESIAN_POINT('Ctrl Pts',(-27.8720760317625,-12.4379977307755,
112.428361666637)) ;
#175430=CARTESIAN_POINT('Ctrl Pts',(-27.7982721884232,-12.4379977309879,
112.452592708569)) ;
#175431=CARTESIAN_POINT('Ctrl Pts',(-27.7925015290558,-12.3643855288192,
112.435016211225)) ;
#175432=CARTESIAN_POINT('Ctrl Pts',(-27.7867308696884,-12.2907733266505,
112.417439713881)) ;
#175433=CARTESIAN_POINT('Ctrl Pts',(-27.8605347130277,-12.2907733264382,
112.39320867195)) ;
#175434=CARTESIAN_POINT('Ctrl Pts',(-27.934338556367,-12.2907733262258,
112.368977630018)) ;
#175435=CARTESIAN_POINT('Ctrl Pts',(-27.9401092157344,-12.3643855283945,
112.386554127362)) ;
#175436=CARTESIAN_POINT('Ctrl Pts',(-27.8457507930179,-12.4735026256636,
112.134502190906)) ;
#175437=CARTESIAN_POINT('Ctrl Pts',(-27.857387277919,-12.5396050352221,
112.169945046424)) ;
#175438=CARTESIAN_POINT('Ctrl Pts',(-27.7835834352188,-12.5396050341181,
112.194176090302)) ;
#175439=CARTESIAN_POINT('Ctrl Pts',(-27.7097795925186,-12.5396050330141,
112.21840713418)) ;
#175440=CARTESIAN_POINT('Ctrl Pts',(-27.6981431076176,-12.4735026234556,
112.182964278663)) ;
#175441=CARTESIAN_POINT('Ctrl Pts',(-27.6865066227165,-12.4074002138971,
112.147521423146)) ;
#175442=CARTESIAN_POINT('Ctrl Pts',(-27.7603104654167,-12.4074002150011,
112.123290379267)) ;
#175443=CARTESIAN_POINT('Ctrl Pts',(-27.8341143081169,-12.4074002161051,
112.099059335389)) ;
#175444=CARTESIAN_POINT('Ctrl Pts',(-27.8457507930179,-12.4735026256636,
112.134502190906)) ;
#175445=CARTESIAN_POINT('Ctrl Pts',(-27.7630645931825,-12.6505044221707,
111.918129912256)) ;
#175446=CARTESIAN_POINT('Ctrl Pts',(-27.77975811883,-12.7043450691342,111.968975697955)) ;
#175447=CARTESIAN_POINT('Ctrl Pts',(-27.7059542761778,-12.7043450666146,
111.99320674198)) ;
#175448=CARTESIAN_POINT('Ctrl Pts',(-27.6321504335255,-12.7043450640951,
112.017437786004)) ;
#175449=CARTESIAN_POINT('Ctrl Pts',(-27.615456907878,-12.6505044171317,
111.966592000305)) ;
#175450=CARTESIAN_POINT('Ctrl Pts',(-27.5987633822305,-12.5966637701682,
111.915746214605)) ;
#175451=CARTESIAN_POINT('Ctrl Pts',(-27.6725672248828,-12.5966637726878,
111.891515170581)) ;
#175452=CARTESIAN_POINT('Ctrl Pts',(-27.746371067535,-12.5966637752073,
111.867284126556)) ;
#175453=CARTESIAN_POINT('Ctrl Pts',(-27.7630645931825,-12.6505044221707,
111.918129912256)) ;
#175454=CARTESIAN_POINT('Ctrl Pts',(-27.6975343400792,-12.883421947767,
111.754113424243)) ;
#175455=CARTESIAN_POINT('Ctrl Pts',(-27.7180922115168,-12.9210776018657,
111.816729383672)) ;
#175456=CARTESIAN_POINT('Ctrl Pts',(-27.6442883682897,-12.9210776004055,
111.840960425945)) ;
#175457=CARTESIAN_POINT('Ctrl Pts',(-27.5704845250626,-12.9210775989452,
111.865191468218)) ;
#175458=CARTESIAN_POINT('Ctrl Pts',(-27.5499266536251,-12.8834219448465,
111.80257550879)) ;
#175459=CARTESIAN_POINT('Ctrl Pts',(-27.5293687821876,-12.8457662907479,
111.739959549362)) ;
#175460=CARTESIAN_POINT('Ctrl Pts',(-27.6031726254146,-12.8457662922081,
111.715728507089)) ;
#175461=CARTESIAN_POINT('Ctrl Pts',(-27.6769764686417,-12.8457662936684,
111.691497464815)) ;
#175462=CARTESIAN_POINT('Ctrl Pts',(-27.6975343400792,-12.883421947767,
111.754113424243)) ;
#175463=CARTESIAN_POINT('Ctrl Pts',(-27.6534936872668,-13.1527514798463,
111.655293821054)) ;
#175464=CARTESIAN_POINT('Ctrl Pts',(-27.6764258063521,-13.1716560829413,
111.725141355679)) ;
#175465=CARTESIAN_POINT('Ctrl Pts',(-27.6026219627207,-13.1716560841151,
111.749372396721)) ;
#175466=CARTESIAN_POINT('Ctrl Pts',(-27.5288181190892,-13.1716560852888,
111.773603437763)) ;
#175467=CARTESIAN_POINT('Ctrl Pts',(-27.5058860000039,-13.1527514821937,
111.703755903138)) ;
#175468=CARTESIAN_POINT('Ctrl Pts',(-27.4829538809186,-13.1338468790986,
111.633908368513)) ;
#175469=CARTESIAN_POINT('Ctrl Pts',(-27.55675772455,-13.1338468779249,111.609677327471)) ;
#175470=CARTESIAN_POINT('Ctrl Pts',(-27.6305615681814,-13.1338468767512,
111.585446286429)) ;
#175471=CARTESIAN_POINT('Ctrl Pts',(-27.6534936872668,-13.1527514798463,
111.655293821054)) ;
#175472=CARTESIAN_POINT('Ctrl Pts',(-27.6327547212792,-13.4437023579035,
111.627785242889)) ;
#175473=CARTESIAN_POINT('Ctrl Pts',(-27.6564307043907,-13.4423185568972,
111.699898467197)) ;
#175474=CARTESIAN_POINT('Ctrl Pts',(-27.5826268608532,-13.442318564338,
111.724129508525)) ;
#175475=CARTESIAN_POINT('Ctrl Pts',(-27.5088230173157,-13.4423185717788,
111.748360549853)) ;
#175476=CARTESIAN_POINT('Ctrl Pts',(-27.4851470342043,-13.443702372785,
111.676247325545)) ;
#175477=CARTESIAN_POINT('Ctrl Pts',(-27.4614710510928,-13.4450861737913,
111.604134101237)) ;
#175478=CARTESIAN_POINT('Ctrl Pts',(-27.5352748946303,-13.4450861663505,
111.579903059909)) ;
#175479=CARTESIAN_POINT('Ctrl Pts',(-27.6090787381678,-13.4450861589097,
111.555672018581)) ;
#175480=CARTESIAN_POINT('Ctrl Pts',(-27.6327547212792,-13.4437023579035,
111.627785242889)) ;
#175481=CARTESIAN_POINT('Ctrl Pts',(-27.6365620199519,-13.7306193771303,
111.674768692016)) ;
#175482=CARTESIAN_POINT('Ctrl Pts',(-27.6592742254984,-13.7091999974399,
111.74394640525)) ;
#175483=CARTESIAN_POINT('Ctrl Pts',(-27.5854703831493,-13.7092000104109,
111.768177450198)) ;
#175484=CARTESIAN_POINT('Ctrl Pts',(-27.5116665408002,-13.7092000233819,
111.792408495146)) ;
#175485=CARTESIAN_POINT('Ctrl Pts',(-27.4889543352537,-13.7306194030722,
111.723230781911)) ;
#175486=CARTESIAN_POINT('Ctrl Pts',(-27.4662421297072,-13.7520387827626,
111.654053068677)) ;
#175487=CARTESIAN_POINT('Ctrl Pts',(-27.5400459720564,-13.7520387697916,
111.629822023729)) ;
#175488=CARTESIAN_POINT('Ctrl Pts',(-27.6138498144055,-13.7520387568206,
111.605590978781)) ;
#175489=CARTESIAN_POINT('Ctrl Pts',(-27.6365620199519,-13.7306193771303,
111.674768692016)) ;
#175490=CARTESIAN_POINT('Ctrl Pts',(-27.6633603539813,-13.9949086675026,
111.791717285722)) ;
#175491=CARTESIAN_POINT('Ctrl Pts',(-27.6835032907012,-13.9550051326843,
111.853069420544)) ;
#175492=CARTESIAN_POINT('Ctrl Pts',(-27.609699450319,-13.9550051495312,
111.877300471483)) ;
#175493=CARTESIAN_POINT('Ctrl Pts',(-27.5358956099367,-13.9550051663781,
111.901531522421)) ;
#175494=CARTESIAN_POINT('Ctrl Pts',(-27.5157526732168,-13.9949087011963,
111.840179387599)) ;
#175495=CARTESIAN_POINT('Ctrl Pts',(-27.4956097364969,-14.0348122360146,
111.778827252776)) ;
#175496=CARTESIAN_POINT('Ctrl Pts',(-27.5694135768792,-14.0348122191677,
111.754596201838)) ;
#175497=CARTESIAN_POINT('Ctrl Pts',(-27.6432174172614,-14.0348122023208,
111.730365150899)) ;
#175498=CARTESIAN_POINT('Ctrl Pts',(-27.6633603539813,-13.9949086675026,
111.791717285722)) ;
#175499=CARTESIAN_POINT('Ctrl Pts',(-27.7111136241826,-14.2196906214034,
111.972774236008)) ;
#175500=CARTESIAN_POINT('Ctrl Pts',(-27.727214755997,-14.1640342666894,
112.021815685053)) ;
#175501=CARTESIAN_POINT('Ctrl Pts',(-27.653410919021,-14.1640342866179,
112.046046746366)) ;
#175502=CARTESIAN_POINT('Ctrl Pts',(-27.579607082045,-14.1640343065465,
112.070277807679)) ;
#175503=CARTESIAN_POINT('Ctrl Pts',(-27.5635059502306,-14.2196906612605,
112.021236358635)) ;
#175504=CARTESIAN_POINT('Ctrl Pts',(-27.5474048184161,-14.2753470159745,
111.97219490959)) ;
#175505=CARTESIAN_POINT('Ctrl Pts',(-27.6212086553922,-14.275346996046,
111.947963848277)) ;
#175506=CARTESIAN_POINT('Ctrl Pts',(-27.6950124923682,-14.2753469761174,
111.923732786964)) ;
#175507=CARTESIAN_POINT('Ctrl Pts',(-27.7111136241826,-14.2196906214034,
111.972774236008)) ;
#175508=CARTESIAN_POINT('Ctrl Pts',(-27.7749357041157,-14.3856064052365,
112.20251553552)) ;
#175509=CARTESIAN_POINT('Ctrl Pts',(-27.7858724825749,-14.3182855334349,
112.235827197368)) ;
#175510=CARTESIAN_POINT('Ctrl Pts',(-27.7120686490727,-14.3182855505584,
112.260058269261)) ;
#175511=CARTESIAN_POINT('Ctrl Pts',(-27.6382648155704,-14.318285567682,
112.284289341155)) ;
#175512=CARTESIAN_POINT('Ctrl Pts',(-27.6273280371112,-14.3856064394836,
112.250977679308)) ;
#175513=CARTESIAN_POINT('Ctrl Pts',(-27.616391258652,-14.4529273112853,
112.217666017461)) ;
#175514=CARTESIAN_POINT('Ctrl Pts',(-27.6901950921543,-14.4529272941617,
112.193434945567)) ;
#175515=CARTESIAN_POINT('Ctrl Pts',(-27.7639989256566,-14.4529272770382,
112.169203873673)) ;
#175516=CARTESIAN_POINT('Ctrl Pts',(-27.7749357041157,-14.3856064052365,
112.20251553552)) ;
#175517=CARTESIAN_POINT('Ctrl Pts',(-27.850139433854,-14.4829720573525,
112.467091440401)) ;
#175518=CARTESIAN_POINT('Ctrl Pts',(-27.8551063751374,-14.4087556909408,
112.482219941263)) ;
#175519=CARTESIAN_POINT('Ctrl Pts',(-27.7813025454846,-14.4087557009118,
112.506451024881)) ;
#175520=CARTESIAN_POINT('Ctrl Pts',(-27.7074987158318,-14.4087557108828,
112.530682108499)) ;
#175521=CARTESIAN_POINT('Ctrl Pts',(-27.7025317745484,-14.4829720772946,
112.515553607637)) ;
#175522=CARTESIAN_POINT('Ctrl Pts',(-27.6975648332649,-14.5571884437063,
112.500425106775)) ;
#175523=CARTESIAN_POINT('Ctrl Pts',(-27.7713686629178,-14.5571884337353,
112.476194023157)) ;
#175524=CARTESIAN_POINT('Ctrl Pts',(-27.8451724925706,-14.5571884237643,
112.451962939539)) ;
#175525=CARTESIAN_POINT('Ctrl Pts',(-27.850139433854,-14.4829720573525,
112.467091440401)) ;
#175526=CARTESIAN_POINT('Ctrl Pts',(-27.9301015626753,-14.5039687036518,
112.746047500903)) ;
#175527=CARTESIAN_POINT('Ctrl Pts',(-27.9287602067411,-14.4281793222941,
112.741961946123)) ;
#175528=CARTESIAN_POINT('Ctrl Pts',(-27.8549563799724,-14.4281793198172,
112.766193038526)) ;
#175529=CARTESIAN_POINT('Ctrl Pts',(-27.7811525532036,-14.4281793173403,
112.790424130929)) ;
#175530=CARTESIAN_POINT('Ctrl Pts',(-27.7824939091379,-14.503968698698,
112.794509685709)) ;
#175531=CARTESIAN_POINT('Ctrl Pts',(-27.7838352650722,-14.5797580800556,
112.798595240489)) ;
#175532=CARTESIAN_POINT('Ctrl Pts',(-27.8576390918409,-14.5797580825325,
112.774364148086)) ;
#175533=CARTESIAN_POINT('Ctrl Pts',(-27.9314429186096,-14.5797580850095,
112.750133055684)) ;
#175534=CARTESIAN_POINT('Ctrl Pts',(-27.9301015626753,-14.5039687036518,
112.746047500903)) ;
#175535=CARTESIAN_POINT('Ctrl Pts',(-28.0091089868232,-14.4466173797893,
113.02236063873)) ;
#175536=CARTESIAN_POINT('Ctrl Pts',(-28.0015114372109,-14.3747219587681,
112.999219727237)) ;
#175537=CARTESIAN_POINT('Ctrl Pts',(-27.9277076127128,-14.3747219386736,
113.023450826556)) ;
#175538=CARTESIAN_POINT('Ctrl Pts',(-27.8539037882146,-14.3747219185791,
113.047681925874)) ;
#175539=CARTESIAN_POINT('Ctrl Pts',(-27.8615013378269,-14.4466173396002,
113.070822837368)) ;
#175540=CARTESIAN_POINT('Ctrl Pts',(-27.8690988874391,-14.5185127606213,
113.093963748861)) ;
#175541=CARTESIAN_POINT('Ctrl Pts',(-27.9429027119373,-14.5185127807159,
113.069732649542)) ;
#175542=CARTESIAN_POINT('Ctrl Pts',(-28.0167065364354,-14.5185128008104,
113.045501550224)) ;
#175543=CARTESIAN_POINT('Ctrl Pts',(-28.0091089868232,-14.4466173797893,
113.02236063873)) ;
#175544=CARTESIAN_POINT('Ctrl Pts',(-28.0794461167512,-14.3162716014842,
113.27191318261)) ;
#175545=CARTESIAN_POINT('Ctrl Pts',(-28.0661960468092,-14.2533730380978,
113.231555606093)) ;
#175546=CARTESIAN_POINT('Ctrl Pts',(-27.9923922216887,-14.2533729987048,
113.255786703516)) ;
#175547=CARTESIAN_POINT('Ctrl Pts',(-27.9185883965682,-14.2533729593119,
113.280017800938)) ;
#175548=CARTESIAN_POINT('Ctrl Pts',(-27.9318384665101,-14.3162715226984,
113.320375377456)) ;
#175549=CARTESIAN_POINT('Ctrl Pts',(-27.945088536452,-14.3791700860849,
113.360732953973)) ;
#175550=CARTESIAN_POINT('Ctrl Pts',(-28.0188923615726,-14.3791701254778,
113.33650185655)) ;
#175551=CARTESIAN_POINT('Ctrl Pts',(-28.0926961866931,-14.3791701648707,
113.312270759127)) ;
#175552=CARTESIAN_POINT('Ctrl Pts',(-28.0794461167512,-14.3162716014842,
113.27191318261)) ;
#175553=CARTESIAN_POINT('Ctrl Pts',(-28.1364440614567,-14.1214968775469,
113.480983026046)) ;
#175554=CARTESIAN_POINT('Ctrl Pts',(-28.1184615726977,-14.0721057771866,
113.426211265236)) ;
#175555=CARTESIAN_POINT('Ctrl Pts',(-28.044657745267,-14.0721057178665,
113.450442355622)) ;
#175556=CARTESIAN_POINT('Ctrl Pts',(-27.9708539178362,-14.0721056585463,
113.474673446009)) ;
#175557=CARTESIAN_POINT('Ctrl Pts',(-27.9888364065952,-14.1214967589066,
113.529445206819)) ;
#175558=CARTESIAN_POINT('Ctrl Pts',(-28.0068188953542,-14.170887859267,
113.58421696763)) ;
#175559=CARTESIAN_POINT('Ctrl Pts',(-28.080622722785,-14.1708879185871,
113.559985877244)) ;
#175560=CARTESIAN_POINT('Ctrl Pts',(-28.1544265502157,-14.1708879779072,
113.535754786857)) ;
#175561=CARTESIAN_POINT('Ctrl Pts',(-28.1364440614567,-14.1214968775469,
113.480983026046)) ;
#175562=CARTESIAN_POINT('Ctrl Pts',(-28.1749613485906,-13.8749956323593,
113.633913814206)) ;
#175563=CARTESIAN_POINT('Ctrl Pts',(-28.153526591033,-13.8427423803111,
113.568626999499)) ;
#175564=CARTESIAN_POINT('Ctrl Pts',(-28.0797227591213,-13.8427423020325,
113.592858076237)) ;
#175565=CARTESIAN_POINT('Ctrl Pts',(-28.0059189272095,-13.8427422237539,
113.617089152975)) ;
#175566=CARTESIAN_POINT('Ctrl Pts',(-28.0273536847671,-13.8749954758022,
113.682375967682)) ;
#175567=CARTESIAN_POINT('Ctrl Pts',(-28.0487884423247,-13.9072487278505,
113.747662782389)) ;
#175568=CARTESIAN_POINT('Ctrl Pts',(-28.1225922742364,-13.907248806129,
113.723431705651)) ;
#175569=CARTESIAN_POINT('Ctrl Pts',(-28.1963961061482,-13.9072488844076,
113.699200628913)) ;
#175570=CARTESIAN_POINT('Ctrl Pts',(-28.1749613485906,-13.8749956323593,
113.633913814206)) ;
#175571=CARTESIAN_POINT('Ctrl Pts',(-28.1911734256759,-13.5974682752699,
113.718666176969)) ;
#175572=CARTESIAN_POINT('Ctrl Pts',(-28.1678437469537,-13.5845442893725,
113.647607738033)) ;
#175573=CARTESIAN_POINT('Ctrl Pts',(-28.0940399083953,-13.584544198723,
113.671838794527)) ;
#175574=CARTESIAN_POINT('Ctrl Pts',(-28.0202360698369,-13.5845441080735,
113.69606985102)) ;
#175575=CARTESIAN_POINT('Ctrl Pts',(-28.0435657485591,-13.597468093971,
113.767128289956)) ;
#175576=CARTESIAN_POINT('Ctrl Pts',(-28.0668954272813,-13.6103920798684,
113.838186728891)) ;
#175577=CARTESIAN_POINT('Ctrl Pts',(-28.1406992658397,-13.6103921705179,
113.813955672398)) ;
#175578=CARTESIAN_POINT('Ctrl Pts',(-28.2145031043981,-13.6103922611673,
113.789724615905)) ;
#175579=CARTESIAN_POINT('Ctrl Pts',(-28.1911734256759,-13.5974682752699,
113.718666176969)) ;
#175580=CARTESIAN_POINT('Ctrl Pts',(-28.1836078259768,-13.3070931499256,
113.731008103206)) ;
#175581=CARTESIAN_POINT('Ctrl Pts',(-28.160040222229,-13.3144232873773,
113.659224982936)) ;
#175582=CARTESIAN_POINT('Ctrl Pts',(-28.0862363758644,-13.3144231909102,
113.683456015653)) ;
#175583=CARTESIAN_POINT('Ctrl Pts',(-28.0124325294998,-13.314423094443,
113.70768704837)) ;
#175584=CARTESIAN_POINT('Ctrl Pts',(-28.0360001332477,-13.3070929569913,
113.77947016864)) ;
#175585=CARTESIAN_POINT('Ctrl Pts',(-28.0595677369956,-13.2997628195396,
113.851253288911)) ;
#175586=CARTESIAN_POINT('Ctrl Pts',(-28.1333715833601,-13.2997629160068,
113.827022256194)) ;
#175587=CARTESIAN_POINT('Ctrl Pts',(-28.2071754297247,-13.2997630124739,
113.802791223477)) ;
#175588=CARTESIAN_POINT('Ctrl Pts',(-28.1836078259768,-13.3070931499256,
113.731008103206)) ;
#175589=CARTESIAN_POINT('Ctrl Pts',(-28.1517250328214,-13.0233508116479,
113.669448037719)) ;
#175590=CARTESIAN_POINT('Ctrl Pts',(-28.1296132234237,-13.0505014151777,
113.602099032054)) ;
#175591=CARTESIAN_POINT('Ctrl Pts',(-28.0558093685922,-13.0505013202395,
113.626330038982)) ;
#175592=CARTESIAN_POINT('Ctrl Pts',(-27.9820055137606,-13.0505012253013,
113.65056104591)) ;
#175593=CARTESIAN_POINT('Ctrl Pts',(-28.0041173231583,-13.0233506217714,
113.717910051575)) ;
#175594=CARTESIAN_POINT('Ctrl Pts',(-28.0262291325559,-12.9962000182415,
113.785259057239)) ;
#175595=CARTESIAN_POINT('Ctrl Pts',(-28.1000329873874,-12.9962001131797,
113.761028050311)) ;
#175596=CARTESIAN_POINT('Ctrl Pts',(-28.173836842219,-12.996200208118,113.736797043383)) ;
#175597=CARTESIAN_POINT('Ctrl Pts',(-28.1517250328214,-13.0233508116479,
113.669448037719)) ;
#175598=CARTESIAN_POINT('Ctrl Pts',(-28.0972991812598,-12.7688607554056,
113.539098836946)) ;
#175599=CARTESIAN_POINT('Ctrl Pts',(-28.0782218167453,-12.8138186885295,
113.480992260729)) ;
#175600=CARTESIAN_POINT('Ctrl Pts',(-28.0044179538581,-12.8138186042271,
113.505223243121)) ;
#175601=CARTESIAN_POINT('Ctrl Pts',(-27.930614090971,-12.8138185199248,
113.529454225513)) ;
#175602=CARTESIAN_POINT('Ctrl Pts',(-27.9496914554855,-12.7688605868009,
113.58756080173)) ;
#175603=CARTESIAN_POINT('Ctrl Pts',(-27.96876882,-12.723902653677,113.645667377947)) ;
#175604=CARTESIAN_POINT('Ctrl Pts',(-28.0425726828872,-12.7239027379794,
113.621436395555)) ;
#175605=CARTESIAN_POINT('Ctrl Pts',(-28.1163765457744,-12.7239028222818,
113.597205413164)) ;
#175606=CARTESIAN_POINT('Ctrl Pts',(-28.0972991812598,-12.7688607554056,
113.539098836946)) ;
#175607=CARTESIAN_POINT('Ctrl Pts',(-28.0232821783549,-12.5604071436069,
113.349142464811)) ;
#175608=CARTESIAN_POINT('Ctrl Pts',(-28.0086100031326,-12.6199846631104,
113.304453384358)) ;
#175609=CARTESIAN_POINT('Ctrl Pts',(-27.9348061333776,-12.6199845970407,
113.328684345831)) ;
#175610=CARTESIAN_POINT('Ctrl Pts',(-27.8610022636226,-12.6199845309711,
113.352915307305)) ;
#175611=CARTESIAN_POINT('Ctrl Pts',(-27.8756744388449,-12.5604070114677,
113.397604387758)) ;
#175612=CARTESIAN_POINT('Ctrl Pts',(-27.8903466140673,-12.5008294919642,
113.442293468211)) ;
#175613=CARTESIAN_POINT('Ctrl Pts',(-27.9641504838223,-12.5008295580339,
113.418062506738)) ;
#175614=CARTESIAN_POINT('Ctrl Pts',(-28.0379543535773,-12.5008296241035,
113.393831545264)) ;
#175615=CARTESIAN_POINT('Ctrl Pts',(-28.0232821783549,-12.5604071436069,
113.349142464811)) ;
#175616=CARTESIAN_POINT('Ctrl Pts',(-27.9344209561679,-12.4137261008746,
113.113916473714)) ;
#175617=CARTESIAN_POINT('Ctrl Pts',(-27.9251979860237,-12.4836322376362,
113.085824792683)) ;
#175618=CARTESIAN_POINT('Ctrl Pts',(-27.8513941114389,-12.4836321960017,
113.110055739446)) ;
#175619=CARTESIAN_POINT('Ctrl Pts',(-27.7775902368542,-12.4836321543672,
113.134286686209)) ;
#175620=CARTESIAN_POINT('Ctrl Pts',(-27.7868132069984,-12.4137260176056,
113.16237836724)) ;
#175621=CARTESIAN_POINT('Ctrl Pts',(-27.7960361771427,-12.343819880844,
113.190470048271)) ;
#175622=CARTESIAN_POINT('Ctrl Pts',(-27.8698400517275,-12.3438199224785,
113.166239101509)) ;
#175623=CARTESIAN_POINT('Ctrl Pts',(-27.9436439263122,-12.343819964113,
113.142008154746)) ;
#175624=CARTESIAN_POINT('Ctrl Pts',(-27.9344209561679,-12.4137261008746,
113.113916473714)) ;
#175625=CARTESIAN_POINT('Ctrl Pts',(-27.8363120109697,-12.3387040702925,
112.850499990527)) ;
#175626=CARTESIAN_POINT('Ctrl Pts',(-27.8331923780007,-12.4139513070211,
112.840998089759)) ;
#175627=CARTESIAN_POINT('Ctrl Pts',(-27.7593885010528,-12.4139512934304,
112.865229029324)) ;
#175628=CARTESIAN_POINT('Ctrl Pts',(-27.6855846241048,-12.4139512798397,
112.889459968889)) ;
#175629=CARTESIAN_POINT('Ctrl Pts',(-27.6887042570738,-12.3387040431111,
112.898961869656)) ;
#175630=CARTESIAN_POINT('Ctrl Pts',(-27.6918238900428,-12.2634568063825,
112.908463770423)) ;
#175631=CARTESIAN_POINT('Ctrl Pts',(-27.7656277669908,-12.2634568199732,
112.884232830859)) ;
#175632=CARTESIAN_POINT('Ctrl Pts',(-27.8394316439388,-12.2634568335639,
112.860001891294)) ;
#175633=CARTESIAN_POINT('Ctrl Pts',(-27.8363120109697,-12.3387040702925,
112.850499990527)) ;
#175634=CARTESIAN_POINT('Ctrl Pts',(-27.7346441044334,-12.3410592400664,
112.576417227786)) ;
#175635=CARTESIAN_POINT('Ctrl Pts',(-27.7378816475841,-12.4162542159503,
112.586278259778)) ;
#175636=CARTESIAN_POINT('Ctrl Pts',(-27.6640777711242,-12.4162542313705,
112.610509200829)) ;
#175637=CARTESIAN_POINT('Ctrl Pts',(-27.5902738946642,-12.4162542467908,
112.63474014188)) ;
#175638=CARTESIAN_POINT('Ctrl Pts',(-27.5870363515135,-12.3410592709069,
112.624879109888)) ;
#175639=CARTESIAN_POINT('Ctrl Pts',(-27.5837988083628,-12.265864295023,
112.615018077896)) ;
#175640=CARTESIAN_POINT('Ctrl Pts',(-27.6576026848227,-12.2658642796027,
112.590787136845)) ;
#175641=CARTESIAN_POINT('Ctrl Pts',(-27.7314065612827,-12.2658642641825,
112.566556195793)) ;
#175642=CARTESIAN_POINT('Ctrl Pts',(-27.7346441044334,-12.3410592400664,
112.576417227786)) ;
#175643=CARTESIAN_POINT('Ctrl Pts',(-27.6369370950116,-12.4205041979803,
112.314216816515)) ;
#175644=CARTESIAN_POINT('Ctrl Pts',(-27.6462685982017,-12.4902644552577,
112.342639067573)) ;
#175645=CARTESIAN_POINT('Ctrl Pts',(-27.5724647248296,-12.4902644973908,
112.366870018029)) ;
#175646=CARTESIAN_POINT('Ctrl Pts',(-27.4986608514575,-12.4902645395239,
112.391100968485)) ;
#175647=CARTESIAN_POINT('Ctrl Pts',(-27.4893293482674,-12.4205042822464,
112.362678717428)) ;
#175648=CARTESIAN_POINT('Ctrl Pts',(-27.4799978450774,-12.350744024969,
112.334256466371)) ;
#175649=CARTESIAN_POINT('Ctrl Pts',(-27.5538017184495,-12.3507439828359,
112.310025515914)) ;
#175650=CARTESIAN_POINT('Ctrl Pts',(-27.6276055918215,-12.3507439407028,
112.285794565458)) ;
#175651=CARTESIAN_POINT('Ctrl Pts',(-27.6369370950116,-12.4205041979803,
112.314216816515)) ;
#175652=CARTESIAN_POINT('Ctrl Pts',(-27.5486712808213,-12.5715202421064,
112.080868685751)) ;
#175653=CARTESIAN_POINT('Ctrl Pts',(-27.563444732966,-12.6308413998765,
112.125866235335)) ;
#175654=CARTESIAN_POINT('Ctrl Pts',(-27.4896408650169,-12.6308414639116,
112.150097202309)) ;
#175655=CARTESIAN_POINT('Ctrl Pts',(-27.4158369970678,-12.6308415279467,
112.174328169283)) ;
#175656=CARTESIAN_POINT('Ctrl Pts',(-27.4010635449232,-12.5715203701767,
112.129330619699)) ;
#175657=CARTESIAN_POINT('Ctrl Pts',(-27.3862900927785,-12.5121992124066,
112.084333070114)) ;
#175658=CARTESIAN_POINT('Ctrl Pts',(-27.4600939607276,-12.5121991483715,
112.06010210314)) ;
#175659=CARTESIAN_POINT('Ctrl Pts',(-27.5338978286767,-12.5121990843364,
112.035871136166)) ;
#175660=CARTESIAN_POINT('Ctrl Pts',(-27.5486712808213,-12.5715202421064,
112.080868685751)) ;
#175661=CARTESIAN_POINT('Ctrl Pts',(-27.4757703775428,-12.7831706996134,
111.894290358998)) ;
#175662=CARTESIAN_POINT('Ctrl Pts',(-27.4949218870949,-12.827803906149,
111.952622765135)) ;
#175663=CARTESIAN_POINT('Ctrl Pts',(-27.4211180261548,-12.8278039851649,
111.976853753457)) ;
#175664=CARTESIAN_POINT('Ctrl Pts',(-27.3473141652147,-12.8278040641808,
112.00108474178)) ;
#175665=CARTESIAN_POINT('Ctrl Pts',(-27.3281626556626,-12.7831708576452,
111.942752335642)) ;
#175666=CARTESIAN_POINT('Ctrl Pts',(-27.3090111461105,-12.7385376511096,
111.884419929505)) ;
#175667=CARTESIAN_POINT('Ctrl Pts',(-27.3828150070506,-12.7385375720937,
111.860188941183)) ;
#175668=CARTESIAN_POINT('Ctrl Pts',(-27.4566188679907,-12.7385374930778,
111.835957952861)) ;
#175669=CARTESIAN_POINT('Ctrl Pts',(-27.4757703775428,-12.7831706996134,
111.894290358998)) ;
#175670=CARTESIAN_POINT('Ctrl Pts',(-27.4226294303003,-13.0400861903177,
111.76787608117)) ;
#175671=CARTESIAN_POINT('Ctrl Pts',(-27.4447864917915,-13.0668491450616,
111.835362913672)) ;
#175672=CARTESIAN_POINT('Ctrl Pts',(-27.3709826386055,-13.0668492312408,
111.859593925612)) ;
#175673=CARTESIAN_POINT('Ctrl Pts',(-27.2971787854195,-13.06684931742,111.883824937552)) ;
#175674=CARTESIAN_POINT('Ctrl Pts',(-27.2750217239283,-13.0400863626762,
111.81633810505)) ;
#175675=CARTESIAN_POINT('Ctrl Pts',(-27.2528646624371,-13.0133234079323,
111.748851272549)) ;
#175676=CARTESIAN_POINT('Ctrl Pts',(-27.3266685156231,-13.0133233217531,
111.724620260609)) ;
#175677=CARTESIAN_POINT('Ctrl Pts',(-27.4004723688091,-13.0133232355738,
111.700389248669)) ;
#175678=CARTESIAN_POINT('Ctrl Pts',(-27.4226294303003,-13.0400861903177,
111.76787608117)) ;
#175679=CARTESIAN_POINT('Ctrl Pts',(-27.3922395133834,-13.3242719779506,
111.710785133111)) ;
#175680=CARTESIAN_POINT('Ctrl Pts',(-27.4158177602532,-13.3312338876365,
111.78260066709)) ;
#175681=CARTESIAN_POINT('Ctrl Pts',(-27.3420139147462,-13.3312339727679,
111.806831702419)) ;
#175682=CARTESIAN_POINT('Ctrl Pts',(-27.2682100692392,-13.3312340578993,
111.831062737749)) ;
#175683=CARTESIAN_POINT('Ctrl Pts',(-27.2446318223695,-13.3242721482135,
111.75924720377)) ;
#175684=CARTESIAN_POINT('Ctrl Pts',(-27.2210535754997,-13.3173102385276,
111.687431669791)) ;
#175685=CARTESIAN_POINT('Ctrl Pts',(-27.2948574210066,-13.3173101533962,
111.663200634461)) ;
#175686=CARTESIAN_POINT('Ctrl Pts',(-27.3686612665136,-13.3173100682647,
111.638969599132)) ;
#175687=CARTESIAN_POINT('Ctrl Pts',(-27.3922395133834,-13.3242719779506,
111.710785133111)) ;
#175688=CARTESIAN_POINT('Ctrl Pts',(-27.3860860135596,-13.6152878377403,
111.727526925979)) ;
#175689=CARTESIAN_POINT('Ctrl Pts',(-27.4093952705665,-13.601941852712,
111.798523160376)) ;
#175690=CARTESIAN_POINT('Ctrl Pts',(-27.3355914317948,-13.6019419294696,
111.82275421622)) ;
#175691=CARTESIAN_POINT('Ctrl Pts',(-27.2617875930231,-13.6019420062272,
111.846985272064)) ;
#175692=CARTESIAN_POINT('Ctrl Pts',(-27.2384783360162,-13.6152879912555,
111.775989037666)) ;
#175693=CARTESIAN_POINT('Ctrl Pts',(-27.2151690790093,-13.6286339762838,
111.704992803269)) ;
#175694=CARTESIAN_POINT('Ctrl Pts',(-27.288972917781,-13.6286338995262,
111.680761747426)) ;
#175695=CARTESIAN_POINT('Ctrl Pts',(-27.3627767565527,-13.6286338227686,
111.656530691582)) ;
#175696=CARTESIAN_POINT('Ctrl Pts',(-27.3860860135596,-13.6152878377403,
111.727526925979)) ;
#175697=CARTESIAN_POINT('Ctrl Pts',(-27.4038644204004,-13.8920338673762,
111.817147898947)) ;
#175698=CARTESIAN_POINT('Ctrl Pts',(-27.4252336909941,-13.8593453805719,
111.882235247896)) ;
#175699=CARTESIAN_POINT('Ctrl Pts',(-27.3514298573554,-13.8593454436439,
111.906466319374)) ;
#175700=CARTESIAN_POINT('Ctrl Pts',(-27.2776260237166,-13.859345506716,
111.930697390851)) ;
#175701=CARTESIAN_POINT('Ctrl Pts',(-27.2562567531229,-13.8920339935203,
111.865610041903)) ;
#175702=CARTESIAN_POINT('Ctrl Pts',(-27.2348874825291,-13.9247224803246,
111.800522692954)) ;
#175703=CARTESIAN_POINT('Ctrl Pts',(-27.3086913161678,-13.9247224172525,
111.776291621476)) ;
#175704=CARTESIAN_POINT('Ctrl Pts',(-27.3824951498066,-13.9247223541804,
111.752060549998)) ;
#175705=CARTESIAN_POINT('Ctrl Pts',(-27.4038644204004,-13.8920338673762,
111.817147898947)) ;
#175706=CARTESIAN_POINT('Ctrl Pts',(-27.4434672264958,-14.1346381572922,
111.973208058208)) ;
#175707=CARTESIAN_POINT('Ctrl Pts',(-27.4613705016364,-14.0849615058488,
112.027738544396)) ;
#175708=CARTESIAN_POINT('Ctrl Pts',(-27.3875666712477,-14.0849615523416,
112.051969625773)) ;
#175709=CARTESIAN_POINT('Ctrl Pts',(-27.3137628408591,-14.0849615988343,
112.07620070715)) ;
#175710=CARTESIAN_POINT('Ctrl Pts',(-27.2958595657186,-14.1346382502777,
112.021670220963)) ;
#175711=CARTESIAN_POINT('Ctrl Pts',(-27.277956290578,-14.1843149017211,
111.967139734775)) ;
#175712=CARTESIAN_POINT('Ctrl Pts',(-27.3517601209666,-14.1843148552283,
111.942908653398)) ;
#175713=CARTESIAN_POINT('Ctrl Pts',(-27.4255639513552,-14.1843148087356,
111.91867757202)) ;
#175714=CARTESIAN_POINT('Ctrl Pts',(-27.4434672264958,-14.1346381572922,
111.973208058208)) ;
#175715=CARTESIAN_POINT('Ctrl Pts',(-27.5014596989945,-14.3262307223465,
112.185343141529)) ;
#175716=CARTESIAN_POINT('Ctrl Pts',(-27.5146064763552,-14.263101480961,
112.225386103109)) ;
#175717=CARTESIAN_POINT('Ctrl Pts',(-27.4408026470349,-14.2631015098285,
112.24961718774)) ;
#175718=CARTESIAN_POINT('Ctrl Pts',(-27.3669988177146,-14.263101538696,
112.273848272371)) ;
#175719=CARTESIAN_POINT('Ctrl Pts',(-27.3538520403539,-14.3262307800815,
112.233805310791)) ;
#175720=CARTESIAN_POINT('Ctrl Pts',(-27.3407052629932,-14.3893600214671,
112.193762349211)) ;
#175721=CARTESIAN_POINT('Ctrl Pts',(-27.4145090923135,-14.3893599925996,
112.16953126458)) ;
#175722=CARTESIAN_POINT('Ctrl Pts',(-27.4883129216338,-14.3893599637321,
112.145300179949)) ;
#175723=CARTESIAN_POINT('Ctrl Pts',(-27.5014596989945,-14.3262307223465,
112.185343141529)) ;
#175724=CARTESIAN_POINT('Ctrl Pts',(-27.572610257217,-14.4523301137118,
112.437438559264)) ;
#175725=CARTESIAN_POINT('Ctrl Pts',(-27.5800769215645,-14.380300846747,
112.460180813242)) ;
#175726=CARTESIAN_POINT('Ctrl Pts',(-27.5062730917788,-14.3803008602231,
112.484411896455)) ;
#175727=CARTESIAN_POINT('Ctrl Pts',(-27.432469261993,-14.3803008736991,
112.508642979669)) ;
#175728=CARTESIAN_POINT('Ctrl Pts',(-27.4250025976456,-14.4523301406639,
112.485900725692)) ;
#175729=CARTESIAN_POINT('Ctrl Pts',(-27.4175359332981,-14.5243594076287,
112.463158471714)) ;
#175730=CARTESIAN_POINT('Ctrl Pts',(-27.4913397630838,-14.5243593941527,
112.438927388501)) ;
#175731=CARTESIAN_POINT('Ctrl Pts',(-27.5651435928695,-14.5243593806767,
112.414696305287)) ;
#175732=CARTESIAN_POINT('Ctrl Pts',(-27.572610257217,-14.4523301137118,
112.437438559264)) ;
#175733=CARTESIAN_POINT('Ctrl Pts',(-27.6514424913783,-14.5048566464616,
112.713014331691)) ;
#175734=CARTESIAN_POINT('Ctrl Pts',(-27.6526823497262,-14.4290505733795,
112.716790739453)) ;
#175735=CARTESIAN_POINT('Ctrl Pts',(-27.5788785178575,-14.4290505742608,
112.741021816322)) ;
#175736=CARTESIAN_POINT('Ctrl Pts',(-27.5050746859887,-14.429050575142,
112.765252893191)) ;
#175737=CARTESIAN_POINT('Ctrl Pts',(-27.5038348276408,-14.5048566482241,
112.761476485429)) ;
#175738=CARTESIAN_POINT('Ctrl Pts',(-27.5025949692929,-14.5806627213062,
112.757700077666)) ;
#175739=CARTESIAN_POINT('Ctrl Pts',(-27.5763988011616,-14.580662720425,
112.733469000797)) ;
#175740=CARTESIAN_POINT('Ctrl Pts',(-27.6502026330304,-14.5806627195438,
112.709237923928)) ;
#175741=CARTESIAN_POINT('Ctrl Pts',(-27.6514424913783,-14.5048566464616,
112.713014331691)) ;
#175742=CARTESIAN_POINT('Ctrl Pts',(-27.7316184422369,-14.4792282215674,
112.992772623)) ;
#175743=CARTESIAN_POINT('Ctrl Pts',(-27.7265262449823,-14.405096385773,
112.977262611251)) ;
#175744=CARTESIAN_POINT('Ctrl Pts',(-27.6527224099425,-14.4050963789129,
113.001493678461)) ;
#175745=CARTESIAN_POINT('Ctrl Pts',(-27.5789185749027,-14.4050963720528,
113.025724745672)) ;
#175746=CARTESIAN_POINT('Ctrl Pts',(-27.5840107721573,-14.4792282078472,
113.041234757421)) ;
#175747=CARTESIAN_POINT('Ctrl Pts',(-27.5891029694118,-14.5533600436416,
113.056744769171)) ;
#175748=CARTESIAN_POINT('Ctrl Pts',(-27.6629068044517,-14.5533600505017,
113.03251370196)) ;
#175749=CARTESIAN_POINT('Ctrl Pts',(-27.7367106394915,-14.5533600573618,
113.00828263475)) ;
#175750=CARTESIAN_POINT('Ctrl Pts',(-27.7316184422369,-14.4792282215674,
112.992772623)) ;
#175751=CARTESIAN_POINT('Ctrl Pts',(-27.8061587870981,-14.3776591931245,
113.255243325012)) ;
#175752=CARTESIAN_POINT('Ctrl Pts',(-27.7951209341155,-14.3105071713144,
113.221623805391)) ;
#175753=CARTESIAN_POINT('Ctrl Pts',(-27.7213170961176,-14.3105071612984,
113.245854863592)) ;
#175754=CARTESIAN_POINT('Ctrl Pts',(-27.6475132581198,-14.3105071512824,
113.270085921793)) ;
#175755=CARTESIAN_POINT('Ctrl Pts',(-27.6585511111024,-14.3776591730925,
113.303705441414)) ;
#175756=CARTESIAN_POINT('Ctrl Pts',(-27.669588964085,-14.4448111949025,
113.337324961035)) ;
#175757=CARTESIAN_POINT('Ctrl Pts',(-27.7433928020829,-14.4448112049185,
113.313093902834)) ;
#175758=CARTESIAN_POINT('Ctrl Pts',(-27.8171966400807,-14.4448112149345,
113.288862844633)) ;
#175759=CARTESIAN_POINT('Ctrl Pts',(-27.8061587870981,-14.3776591931245,
113.255243325012)) ;
#175760=CARTESIAN_POINT('Ctrl Pts',(-27.8693284879629,-14.2073582471136,
113.483114722588)) ;
#175761=CARTESIAN_POINT('Ctrl Pts',(-27.8531291806685,-14.1519959883529,
113.433774246071)) ;
#175762=CARTESIAN_POINT('Ctrl Pts',(-27.7793253400122,-14.1519959791231,
113.458005296175)) ;
#175763=CARTESIAN_POINT('Ctrl Pts',(-27.705521499356,-14.1519959698933,
113.482236346279)) ;
#175764=CARTESIAN_POINT('Ctrl Pts',(-27.7217208066503,-14.207358228654,
113.531576822795)) ;
#175765=CARTESIAN_POINT('Ctrl Pts',(-27.7379201139447,-14.2627204874147,
113.580917299312)) ;
#175766=CARTESIAN_POINT('Ctrl Pts',(-27.8117239546009,-14.2627204966445,
113.556686249208)) ;
#175767=CARTESIAN_POINT('Ctrl Pts',(-27.8855277952572,-14.2627205058743,
113.532455199104)) ;
#175768=CARTESIAN_POINT('Ctrl Pts',(-27.8693284879629,-14.2073582471136,
113.483114722588)) ;
#175769=CARTESIAN_POINT('Ctrl Pts',(-27.9157562377959,-13.980463190757,
113.659992780597)) ;
#175770=CARTESIAN_POINT('Ctrl Pts',(-27.8955566894573,-13.9408606598198,
113.598468215417)) ;
#175771=CARTESIAN_POINT('Ctrl Pts',(-27.8217528469617,-13.9408606539983,
113.622699259918)) ;
#175772=CARTESIAN_POINT('Ctrl Pts',(-27.7479490044661,-13.9408606481768,
113.64693030442)) ;
#175773=CARTESIAN_POINT('Ctrl Pts',(-27.7681485528048,-13.9804631791139,
113.7084548696)) ;
#175774=CARTESIAN_POINT('Ctrl Pts',(-27.7883481011434,-14.0200657100511,
113.76997943478)) ;
#175775=CARTESIAN_POINT('Ctrl Pts',(-27.862151943639,-14.0200657158726,
113.745748390279)) ;
#175776=CARTESIAN_POINT('Ctrl Pts',(-27.9359557861346,-14.0200657216941,
113.721517345777)) ;
#175777=CARTESIAN_POINT('Ctrl Pts',(-27.9157562377959,-13.980463190757,
113.659992780597)) ;
#175778=CARTESIAN_POINT('Ctrl Pts',(-27.9413702245525,-13.7134648384933,
113.773453223393)) ;
#175779=CARTESIAN_POINT('Ctrl Pts',(-27.9186183026862,-13.6924464842837,
113.704154540366)) ;
#175780=CARTESIAN_POINT('Ctrl Pts',(-27.8448144593015,-13.6924464826294,
113.728385582159)) ;
#175781=CARTESIAN_POINT('Ctrl Pts',(-27.7710106159168,-13.6924464809751,
113.752616623953)) ;
#175782=CARTESIAN_POINT('Ctrl Pts',(-27.7937625377831,-13.7134648351847,
113.82191530698)) ;
#175783=CARTESIAN_POINT('Ctrl Pts',(-27.8165144596494,-13.7344831893942,
113.891213990007)) ;
#175784=CARTESIAN_POINT('Ctrl Pts',(-27.8903183030341,-13.7344831910485,
113.866982948213)) ;
#175785=CARTESIAN_POINT('Ctrl Pts',(-27.9641221464188,-13.7344831927028,
113.84275190642)) ;
#175786=CARTESIAN_POINT('Ctrl Pts',(-27.9413702245525,-13.7134648384933,
113.773453223393)) ;
#175787=CARTESIAN_POINT('Ctrl Pts',(-27.9436004920684,-13.4252028157263,
113.815706568897)) ;
#175788=CARTESIAN_POINT('Ctrl Pts',(-27.9199249631736,-13.4242817506044,
113.74359472795)) ;
#175789=CARTESIAN_POINT('Ctrl Pts',(-27.8461211196883,-13.4242817523867,
113.767825769437)) ;
#175790=CARTESIAN_POINT('Ctrl Pts',(-27.7723172762029,-13.4242817541689,
113.792056810924)) ;
#175791=CARTESIAN_POINT('Ctrl Pts',(-27.7959928050977,-13.4252028192908,
113.864168651871)) ;
#175792=CARTESIAN_POINT('Ctrl Pts',(-27.8196683339925,-13.4261238844127,
113.936280492817)) ;
#175793=CARTESIAN_POINT('Ctrl Pts',(-27.8934721774779,-13.4261238826305,
113.91204945133)) ;
#175794=CARTESIAN_POINT('Ctrl Pts',(-27.9672760209632,-13.4261238808483,
113.887818409844)) ;
#175795=CARTESIAN_POINT('Ctrl Pts',(-27.9436004920684,-13.4252028157263,
113.815706568897)) ;
#175796=CARTESIAN_POINT('Ctrl Pts',(-27.9215804554763,-13.136660084581,
113.78406473884)) ;
#175797=CARTESIAN_POINT('Ctrl Pts',(-27.8986741696855,-13.1558861878268,
113.714295888302)) ;
#175798=CARTESIAN_POINT('Ctrl Pts',(-27.824870326538,-13.1558861911127,
113.738526930818)) ;
#175799=CARTESIAN_POINT('Ctrl Pts',(-27.7510664833906,-13.1558861943986,
113.762757973334)) ;
#175800=CARTESIAN_POINT('Ctrl Pts',(-27.7739727691814,-13.1366600911528,
113.832526823872)) ;
#175801=CARTESIAN_POINT('Ctrl Pts',(-27.7968790549722,-13.117433987907,
113.90229567441)) ;
#175802=CARTESIAN_POINT('Ctrl Pts',(-27.8706828981197,-13.1174339846211,
113.878064631894)) ;
#175803=CARTESIAN_POINT('Ctrl Pts',(-27.9444867412671,-13.1174339813352,
113.853833589377)) ;
#175804=CARTESIAN_POINT('Ctrl Pts',(-27.9215804554763,-13.136660084581,
113.78406473884)) ;
#175805=CARTESIAN_POINT('Ctrl Pts',(-27.8759261543426,-12.8674128564449,
113.680553643697)) ;
#175806=CARTESIAN_POINT('Ctrl Pts',(-27.8554383685418,-12.9054690960976,
113.61815115389)) ;
#175807=CARTESIAN_POINT('Ctrl Pts',(-27.7816345255925,-12.9054690982831,
113.64238219701)) ;
#175808=CARTESIAN_POINT('Ctrl Pts',(-27.7078306826432,-12.9054691004687,
113.666613240129)) ;
#175809=CARTESIAN_POINT('Ctrl Pts',(-27.728318468444,-12.867412860816,113.729015729936)) ;
#175810=CARTESIAN_POINT('Ctrl Pts',(-27.7488062542447,-12.8293566211633,
113.791418219742)) ;
#175811=CARTESIAN_POINT('Ctrl Pts',(-27.8226100971941,-12.8293566189777,
113.767187176623)) ;
#175812=CARTESIAN_POINT('Ctrl Pts',(-27.8964139401434,-12.8293566167922,
113.742956133503)) ;
#175813=CARTESIAN_POINT('Ctrl Pts',(-27.8759261543426,-12.8674128564449,
113.680553643697)) ;
#175814=CARTESIAN_POINT('Ctrl Pts',(-27.8094158631442,-12.6383938778605,
113.513414911382)) ;
#175815=CARTESIAN_POINT('Ctrl Pts',(-27.7928087845804,-12.6924977231703,
113.462832429616)) ;
#175816=CARTESIAN_POINT('Ctrl Pts',(-27.7190049412073,-12.6924977228183,
113.487063471445)) ;
#175817=CARTESIAN_POINT('Ctrl Pts',(-27.6452010978342,-12.6924977224664,
113.511294513273)) ;
#175818=CARTESIAN_POINT('Ctrl Pts',(-27.6618081763979,-12.6383938771567,
113.561876995039)) ;
#175819=CARTESIAN_POINT('Ctrl Pts',(-27.6784152549617,-12.5842900318469,
113.612459476805)) ;
#175820=CARTESIAN_POINT('Ctrl Pts',(-27.7522190983348,-12.5842900321988,
113.588228434977)) ;
#175821=CARTESIAN_POINT('Ctrl Pts',(-27.8260229417079,-12.5842900325507,
113.563997393148)) ;
#175822=CARTESIAN_POINT('Ctrl Pts',(-27.8094158631442,-12.6383938778605,
113.513414911382)) ;
#175823=CARTESIAN_POINT('Ctrl Pts',(-27.7259260844217,-12.465038874388,
113.294584641188)) ;
#175824=CARTESIAN_POINT('Ctrl Pts',(-27.7143905181872,-12.531326536537,
113.259449167606)) ;
#175825=CARTESIAN_POINT('Ctrl Pts',(-27.6405866735841,-12.5313265339241,
113.283680205688)) ;
#175826=CARTESIAN_POINT('Ctrl Pts',(-27.566782828981,-12.5313265313111,
113.30791124377)) ;
#175827=CARTESIAN_POINT('Ctrl Pts',(-27.5783183952155,-12.4650388691621,
113.343046717353)) ;
#175828=CARTESIAN_POINT('Ctrl Pts',(-27.5898539614499,-12.3987512070131,
113.378182190936)) ;
#175829=CARTESIAN_POINT('Ctrl Pts',(-27.6636578060531,-12.3987512096261,
113.353951152854)) ;
#175830=CARTESIAN_POINT('Ctrl Pts',(-27.7374616506562,-12.398751212239,
113.329720114771)) ;
#175831=CARTESIAN_POINT('Ctrl Pts',(-27.7259260844217,-12.465038874388,
113.294584641188)) ;
#175832=CARTESIAN_POINT('Ctrl Pts',(-27.630761291581,-12.3599344396702,
113.040172878809)) ;
#175833=CARTESIAN_POINT('Ctrl Pts',(-27.6251202578705,-12.4336574817887,
113.022991200105)) ;
#175834=CARTESIAN_POINT('Ctrl Pts',(-27.5513164113796,-12.4336574787988,
113.047222232437)) ;
#175835=CARTESIAN_POINT('Ctrl Pts',(-27.4775125648887,-12.4336574758088,
113.07145326477)) ;
#175836=CARTESIAN_POINT('Ctrl Pts',(-27.4831535985992,-12.3599344336902,
113.088634943473)) ;
#175837=CARTESIAN_POINT('Ctrl Pts',(-27.4887946323096,-12.2862113915716,
113.105816622177)) ;
#175838=CARTESIAN_POINT('Ctrl Pts',(-27.5625984788005,-12.2862113945616,
113.081585589845)) ;
#175839=CARTESIAN_POINT('Ctrl Pts',(-27.6364023252914,-12.2862113975516,
113.057354557512)) ;
#175840=CARTESIAN_POINT('Ctrl Pts',(-27.630761291581,-12.3599344396702,
113.040172878809)) ;
#175841=CARTESIAN_POINT('Ctrl Pts',(-27.5296719419162,-12.3306429195518,
112.767809456319)) ;
#175842=CARTESIAN_POINT('Ctrl Pts',(-27.5303457069297,-12.4065184959483,
112.769861635494)) ;
#175843=CARTESIAN_POINT('Ctrl Pts',(-27.4565418579544,-12.4065184959014,
112.794092660259)) ;
#175844=CARTESIAN_POINT('Ctrl Pts',(-27.3827380089791,-12.4065184958546,
112.818323685024)) ;
#175845=CARTESIAN_POINT('Ctrl Pts',(-27.3820642439656,-12.330642919458,
112.81627150585)) ;
#175846=CARTESIAN_POINT('Ctrl Pts',(-27.3813904789522,-12.2547673430615,
112.814219326675)) ;
#175847=CARTESIAN_POINT('Ctrl Pts',(-27.4551943279275,-12.2547673431084,
112.78998830191)) ;
#175848=CARTESIAN_POINT('Ctrl Pts',(-27.5289981769028,-12.2547673431553,
112.765757277145)) ;
#175849=CARTESIAN_POINT('Ctrl Pts',(-27.5296719419162,-12.3306429195518,
112.767809456319)) ;
#175850=CARTESIAN_POINT('Ctrl Pts',(-27.4298006531373,-12.3792038030185,
112.499012174243)) ;
#175851=CARTESIAN_POINT('Ctrl Pts',(-27.4367161594043,-12.4517984874487,
112.520075690037)) ;
#175852=CARTESIAN_POINT('Ctrl Pts',(-27.3629123084857,-12.4517984942269,
112.544306708883)) ;
#175853=CARTESIAN_POINT('Ctrl Pts',(-27.2891084575671,-12.4517985010052,
112.568537727729)) ;
#175854=CARTESIAN_POINT('Ctrl Pts',(-27.2821929513001,-12.379203816575,
112.547474211936)) ;
#175855=CARTESIAN_POINT('Ctrl Pts',(-27.275277445033,-12.3066091321447,
112.526410696142)) ;
#175856=CARTESIAN_POINT('Ctrl Pts',(-27.3490812959516,-12.3066091253665,
112.502179677296)) ;
#175857=CARTESIAN_POINT('Ctrl Pts',(-27.4228851468702,-12.3066091185883,
112.47794865845)) ;
#175858=CARTESIAN_POINT('Ctrl Pts',(-27.4298006531373,-12.3792038030185,
112.499012174243)) ;
#175859=CARTESIAN_POINT('Ctrl Pts',(-27.3368869719151,-12.502250920438,
112.251503904024)) ;
#175860=CARTESIAN_POINT('Ctrl Pts',(-27.3495653984223,-12.5663594268052,
112.29012034486)) ;
#175861=CARTESIAN_POINT('Ctrl Pts',(-27.2757615460824,-12.5663594442773,
112.314351359377)) ;
#175862=CARTESIAN_POINT('Ctrl Pts',(-27.2019576937426,-12.5663594617495,
112.338582373895)) ;
#175863=CARTESIAN_POINT('Ctrl Pts',(-27.1892792672354,-12.5022509553824,
112.299965933058)) ;
#175864=CARTESIAN_POINT('Ctrl Pts',(-27.1766008407283,-12.4381424490152,
112.261349492222)) ;
#175865=CARTESIAN_POINT('Ctrl Pts',(-27.2504046930681,-12.4381424315431,
112.237118477705)) ;
#175866=CARTESIAN_POINT('Ctrl Pts',(-27.324208545408,-12.4381424140709,
112.212887463188)) ;
#175867=CARTESIAN_POINT('Ctrl Pts',(-27.3368869719151,-12.502250920438,
112.251503904024)) ;
#175868=CARTESIAN_POINT('Ctrl Pts',(-27.2572469138254,-12.690704289041,
112.044366413114)) ;
#175869=CARTESIAN_POINT('Ctrl Pts',(-27.2747709167392,-12.7417475393675,
112.097741697693)) ;
#175870=CARTESIAN_POINT('Ctrl Pts',(-27.2009670644347,-12.7417475700136,
112.121972712318)) ;
#175871=CARTESIAN_POINT('Ctrl Pts',(-27.1271632121303,-12.7417476006596,
112.146203726943)) ;
#175872=CARTESIAN_POINT('Ctrl Pts',(-27.1096392092165,-12.6907043503331,
112.092828442364)) ;
#175873=CARTESIAN_POINT('Ctrl Pts',(-27.0921152063027,-12.6396611000066,
112.039453157785)) ;
#175874=CARTESIAN_POINT('Ctrl Pts',(-27.1659190586071,-12.6396610693606,
112.01522214316)) ;
#175875=CARTESIAN_POINT('Ctrl Pts',(-27.2397229109116,-12.6396610387145,
111.990991128535)) ;
#175876=CARTESIAN_POINT('Ctrl Pts',(-27.2572469138254,-12.690704289041,
112.044366413114)) ;
#175877=CARTESIAN_POINT('Ctrl Pts',(-27.1956046752294,-12.9312491813812,
111.892066772438)) ;
#175878=CARTESIAN_POINT('Ctrl Pts',(-27.2167242051917,-12.9655714979513,
111.956393452104)) ;
#175879=CARTESIAN_POINT('Ctrl Pts',(-27.1429203545228,-12.9655715427417,
111.980624471711)) ;
#175880=CARTESIAN_POINT('Ctrl Pts',(-27.0691165038539,-12.9655715875322,
112.004855491318)) ;
#175881=CARTESIAN_POINT('Ctrl Pts',(-27.0479969738915,-12.9312492709622,
111.940528811651)) ;
#175882=CARTESIAN_POINT('Ctrl Pts',(-27.0268774439292,-12.8969269543922,
111.876202131985)) ;
#175883=CARTESIAN_POINT('Ctrl Pts',(-27.1006812945981,-12.8969269096017,
111.851971112378)) ;
#175884=CARTESIAN_POINT('Ctrl Pts',(-27.174485145267,-12.8969268648112,
111.827740092771)) ;
#175885=CARTESIAN_POINT('Ctrl Pts',(-27.1956046752294,-12.9312491813812,
111.892066772438)) ;
#175886=CARTESIAN_POINT('Ctrl Pts',(-27.1556968251946,-13.2069304836541,
111.805999837402)) ;
#175887=CARTESIAN_POINT('Ctrl Pts',(-27.1788989285037,-13.2220547357584,
111.87666969929)) ;
#175888=CARTESIAN_POINT('Ctrl Pts',(-27.1050950812972,-13.2220547937704,
111.900900729442)) ;
#175889=CARTESIAN_POINT('Ctrl Pts',(-27.0312912340907,-13.2220548517825,
111.925131759595)) ;
#175890=CARTESIAN_POINT('Ctrl Pts',(-27.0080891307815,-13.2069305996783,
111.854461897707)) ;
#175891=CARTESIAN_POINT('Ctrl Pts',(-26.9848870274724,-13.191806347574,
111.783792035819)) ;
#175892=CARTESIAN_POINT('Ctrl Pts',(-27.0586908746789,-13.191806289562,
111.759561005666)) ;
#175893=CARTESIAN_POINT('Ctrl Pts',(-27.1324947218855,-13.1918062315499,
111.735329975513)) ;
#175894=CARTESIAN_POINT('Ctrl Pts',(-27.1556968251946,-13.2069304836541,
111.805999837402)) ;
#175895=CARTESIAN_POINT('Ctrl Pts',(-27.1396183503164,-13.4971323588194,
111.792434998313)) ;
#175896=CARTESIAN_POINT('Ctrl Pts',(-27.163243869223,-13.4920171795336,
111.864394515641)) ;
#175897=CARTESIAN_POINT('Ctrl Pts',(-27.0894400270983,-13.4920172465716,
111.888625561272)) ;
#175898=CARTESIAN_POINT('Ctrl Pts',(-27.0156361849736,-13.4920173136096,
111.912856606903)) ;
#175899=CARTESIAN_POINT('Ctrl Pts',(-26.992010666067,-13.4971324928954,
111.840897089575)) ;
#175900=CARTESIAN_POINT('Ctrl Pts',(-26.9683851471604,-13.5022476721812,
111.768937572246)) ;
#175901=CARTESIAN_POINT('Ctrl Pts',(-27.0421889892851,-13.5022476051432,
111.744706526615)) ;
#175902=CARTESIAN_POINT('Ctrl Pts',(-27.1159928314098,-13.5022475381053,
111.720475480984)) ;
#175903=CARTESIAN_POINT('Ctrl Pts',(-27.1396183503164,-13.4971323588194,
111.792434998313)) ;
#175904=CARTESIAN_POINT('Ctrl Pts',(-27.1478926952953,-13.7832858649534,
111.853261517309)) ;
#175905=CARTESIAN_POINT('Ctrl Pts',(-27.1702377683041,-13.7581847544607,
111.921321002853)) ;
#175906=CARTESIAN_POINT('Ctrl Pts',(-27.0964339327126,-13.7581848266256,
111.945552068383)) ;
#175907=CARTESIAN_POINT('Ctrl Pts',(-27.0226300971212,-13.7581848987905,
111.969783133914)) ;
#175908=CARTESIAN_POINT('Ctrl Pts',(-27.0002850241124,-13.7832860092831,
111.90172364837)) ;
#175909=CARTESIAN_POINT('Ctrl Pts',(-26.9779399511036,-13.8083871197758,
111.833664162826)) ;
#175910=CARTESIAN_POINT('Ctrl Pts',(-27.0517437866951,-13.808387047611,
111.809433097296)) ;
#175911=CARTESIAN_POINT('Ctrl Pts',(-27.1255476222865,-13.8083869754461,
111.785202031766)) ;
#175912=CARTESIAN_POINT('Ctrl Pts',(-27.1478926952953,-13.7832858649534,
111.853261517309)) ;
#175913=CARTESIAN_POINT('Ctrl Pts',(-27.1788426100833,-14.0408293277911,
111.98281261947)) ;
#175914=CARTESIAN_POINT('Ctrl Pts',(-27.1983290352884,-13.9977110227071,
112.042165124933)) ;
#175915=CARTESIAN_POINT('Ctrl Pts',(-27.1245252064214,-13.997711090453,
112.066396210945)) ;
#175916=CARTESIAN_POINT('Ctrl Pts',(-27.0507213775545,-13.9977111581989,
112.090627296957)) ;
#175917=CARTESIAN_POINT('Ctrl Pts',(-27.0312349523494,-14.0408294632829,
112.031274791494)) ;
#175918=CARTESIAN_POINT('Ctrl Pts',(-27.0117485271443,-14.0839477683669,
111.971922286031)) ;
#175919=CARTESIAN_POINT('Ctrl Pts',(-27.0855523560112,-14.083947700621,
111.947691200019)) ;
#175920=CARTESIAN_POINT('Ctrl Pts',(-27.1593561848781,-14.0839476328751,
111.923460114007)) ;
#175921=CARTESIAN_POINT('Ctrl Pts',(-27.1788426100833,-14.0408293277911,
111.98281261947)) ;
#175922=CARTESIAN_POINT('Ctrl Pts',(-27.2300778195774,-14.255952322556,
112.174490901595)) ;
#175923=CARTESIAN_POINT('Ctrl Pts',(-27.2452785325984,-14.1977519640159,
112.220789819091)) ;
#175924=CARTESIAN_POINT('Ctrl Pts',(-27.1714747106939,-14.1977520218044,
112.24502092631)) ;
#175925=CARTESIAN_POINT('Ctrl Pts',(-27.0976708887894,-14.1977520795929,
112.269252033528)) ;
#175926=CARTESIAN_POINT('Ctrl Pts',(-27.0824701757685,-14.2559524381331,
112.222953116032)) ;
#175927=CARTESIAN_POINT('Ctrl Pts',(-27.0672694627476,-14.3141527966732,
112.176654198535)) ;
#175928=CARTESIAN_POINT('Ctrl Pts',(-27.141073284652,-14.3141527388846,
112.152423091316)) ;
#175929=CARTESIAN_POINT('Ctrl Pts',(-27.2148771065565,-14.3141526810961,
112.128191984098)) ;
#175930=CARTESIAN_POINT('Ctrl Pts',(-27.2300778195774,-14.255952322556,
112.174490901595)) ;
#175931=CARTESIAN_POINT('Ctrl Pts',(-27.2963594840731,-14.4094466686143,
112.411688111103)) ;
#175932=CARTESIAN_POINT('Ctrl Pts',(-27.3062239782014,-14.3404453655438,
112.441733766757)) ;
#175933=CARTESIAN_POINT('Ctrl Pts',(-27.2324201616656,-14.3404454048825,
112.465964890328)) ;
#175934=CARTESIAN_POINT('Ctrl Pts',(-27.1586163451298,-14.3404454442213,
112.490196013899)) ;
#175935=CARTESIAN_POINT('Ctrl Pts',(-27.1487518510015,-14.4094467472918,
112.460150358244)) ;
#175936=CARTESIAN_POINT('Ctrl Pts',(-27.1388873568732,-14.4784480503623,
112.43010470259)) ;
#175937=CARTESIAN_POINT('Ctrl Pts',(-27.212691173409,-14.4784480110235,
112.405873579019)) ;
#175938=CARTESIAN_POINT('Ctrl Pts',(-27.2864949899448,-14.4784479716848,
112.381642455449)) ;
#175939=CARTESIAN_POINT('Ctrl Pts',(-27.2963594840731,-14.4094466686143,
112.411688111103)) ;
#175940=CARTESIAN_POINT('Ctrl Pts',(-27.3730829374615,-14.4929694646286,
112.680938243989)) ;
#175941=CARTESIAN_POINT('Ctrl Pts',(-27.3768695303142,-14.4180358803258,
112.692471592919)) ;
#175942=CARTESIAN_POINT('Ctrl Pts',(-27.3030657177336,-14.4180358961808,
112.716702728537)) ;
#175943=CARTESIAN_POINT('Ctrl Pts',(-27.2292619051531,-14.4180359120358,
112.740933864154)) ;
#175944=CARTESIAN_POINT('Ctrl Pts',(-27.2254753123004,-14.4929694963386,
112.729400515224)) ;
#175945=CARTESIAN_POINT('Ctrl Pts',(-27.2216887194477,-14.5679030806414,
112.717867166294)) ;
#175946=CARTESIAN_POINT('Ctrl Pts',(-27.2954925320283,-14.5679030647864,
112.693636030676)) ;
#175947=CARTESIAN_POINT('Ctrl Pts',(-27.3692963446088,-14.5679030489314,
112.669404895059)) ;
#175948=CARTESIAN_POINT('Ctrl Pts',(-27.3730829374615,-14.4929694646286,
112.680938243989)) ;
#175949=CARTESIAN_POINT('Ctrl Pts',(-27.4533942328739,-14.4990155260453,
112.961017342185)) ;
#175950=CARTESIAN_POINT('Ctrl Pts',(-27.4508455544286,-14.4235500005798,
112.953254476862)) ;
#175951=CARTESIAN_POINT('Ctrl Pts',(-27.3770417432059,-14.4235499890681,
112.977485616615)) ;
#175952=CARTESIAN_POINT('Ctrl Pts',(-27.3032379319832,-14.4235499775565,
113.001716756368)) ;
#175953=CARTESIAN_POINT('Ctrl Pts',(-27.3057866104284,-14.499015503022,
113.009479621691)) ;
#175954=CARTESIAN_POINT('Ctrl Pts',(-27.3083352888737,-14.5744810284875,
113.017242487014)) ;
#175955=CARTESIAN_POINT('Ctrl Pts',(-27.3821391000964,-14.5744810399991,
112.993011347261)) ;
#175956=CARTESIAN_POINT('Ctrl Pts',(-27.4559429113192,-14.5744810515108,
112.968780207508)) ;
#175957=CARTESIAN_POINT('Ctrl Pts',(-27.4533942328739,-14.4990155260453,
112.961017342185)) ;
#175958=CARTESIAN_POINT('Ctrl Pts',(-27.5309746225123,-14.4275804860338,
113.232800584045)) ;
#175959=CARTESIAN_POINT('Ctrl Pts',(-27.5222715844995,-14.3569912762542,
113.20629253243)) ;
#175960=CARTESIAN_POINT('Ctrl Pts',(-27.4484677719345,-14.3569912367052,
113.230523668094)) ;
#175961=CARTESIAN_POINT('Ctrl Pts',(-27.3746639593695,-14.3569911971563,
113.254754803759)) ;
#175962=CARTESIAN_POINT('Ctrl Pts',(-27.3833669973824,-14.4275804069359,
113.281262855375)) ;
#175963=CARTESIAN_POINT('Ctrl Pts',(-27.3920700353952,-14.4981696167155,
113.30777090699)) ;
#175964=CARTESIAN_POINT('Ctrl Pts',(-27.4658738479602,-14.4981696562644,
113.283539771325)) ;
#175965=CARTESIAN_POINT('Ctrl Pts',(-27.5396776605252,-14.4981696958134,
113.25930863566)) ;
#175966=CARTESIAN_POINT('Ctrl Pts',(-27.5309746225123,-14.4275804860338,
113.232800584045)) ;
#175967=CARTESIAN_POINT('Ctrl Pts',(-27.5993744489561,-14.284309082368,
113.476532018314)) ;
#175968=CARTESIAN_POINT('Ctrl Pts',(-27.5851507849207,-14.223618657059,
113.433209030554)) ;
#175969=CARTESIAN_POINT('Ctrl Pts',(-27.5113469683492,-14.2236185917218,
113.457440154016)) ;
#175970=CARTESIAN_POINT('Ctrl Pts',(-27.4375431517776,-14.2236185263845,
113.481671277477)) ;
#175971=CARTESIAN_POINT('Ctrl Pts',(-27.4517668158129,-14.2843089516935,
113.524994265237)) ;
#175972=CARTESIAN_POINT('Ctrl Pts',(-27.4659904798483,-14.3449993770025,
113.568317252997)) ;
#175973=CARTESIAN_POINT('Ctrl Pts',(-27.5397942964199,-14.3449994423398,
113.544086129535)) ;
#175974=CARTESIAN_POINT('Ctrl Pts',(-27.6135981129914,-14.3449995076771,
113.519855006074)) ;
#175975=CARTESIAN_POINT('Ctrl Pts',(-27.5993744489561,-14.284309082368,
113.476532018314)) ;
#175976=CARTESIAN_POINT('Ctrl Pts',(-27.6533609863589,-14.0775350374868,
113.67660042095)) ;
#175977=CARTESIAN_POINT('Ctrl Pts',(-27.634609746819,-14.0311904705444,
113.619487168718)) ;
#175978=CARTESIAN_POINT('Ctrl Pts',(-27.5608059238945,-14.0311903843125,
113.643718272829)) ;
#175979=CARTESIAN_POINT('Ctrl Pts',(-27.4870021009699,-14.0311902980806,
113.66794937694)) ;
#175980=CARTESIAN_POINT('Ctrl Pts',(-27.5057533405098,-14.0775348650229,
113.725062629172)) ;
#175981=CARTESIAN_POINT('Ctrl Pts',(-27.5245045800497,-14.1238794319653,
113.782175881404)) ;
#175982=CARTESIAN_POINT('Ctrl Pts',(-27.5983084029742,-14.1238795181972,
113.757944777293)) ;
#175983=CARTESIAN_POINT('Ctrl Pts',(-27.6721122258988,-14.1238796044292,
113.733713673182)) ;
#175984=CARTESIAN_POINT('Ctrl Pts',(-27.6533609863589,-14.0775350374868,
113.67660042095)) ;
#175985=CARTESIAN_POINT('Ctrl Pts',(-27.6875986228682,-13.8261134335288,
113.816121058213)) ;
#175986=CARTESIAN_POINT('Ctrl Pts',(-27.665700207824,-13.7972540806325,
113.749422017201)) ;
#175987=CARTESIAN_POINT('Ctrl Pts',(-27.5918963769847,-13.7972539806286,
113.773653097205)) ;
#175988=CARTESIAN_POINT('Ctrl Pts',(-27.5180925461453,-13.7972538806247,
113.797884177209)) ;
#175989=CARTESIAN_POINT('Ctrl Pts',(-27.5399909611896,-13.826113233521,
113.864583218222)) ;
#175990=CARTESIAN_POINT('Ctrl Pts',(-27.5618893762338,-13.8549725864173,
113.931282259234)) ;
#175991=CARTESIAN_POINT('Ctrl Pts',(-27.6356932070732,-13.8549726864212,
113.90705117923)) ;
#175992=CARTESIAN_POINT('Ctrl Pts',(-27.7094970379125,-13.8549727864252,
113.882820099226)) ;
#175993=CARTESIAN_POINT('Ctrl Pts',(-27.6875986228682,-13.8261134335288,
113.816121058213)) ;
#175994=CARTESIAN_POINT('Ctrl Pts',(-27.6996267717849,-13.5428648342343,
113.888368399397)) ;
#175995=CARTESIAN_POINT('Ctrl Pts',(-27.676119024517,-13.5337376171051,
113.816767592136)) ;
#175996=CARTESIAN_POINT('Ctrl Pts',(-27.6023151848084,-13.5337375120109,
113.840998645126)) ;
#175997=CARTESIAN_POINT('Ctrl Pts',(-27.5285113450998,-13.5337374069167,
113.865229698116)) ;
#175998=CARTESIAN_POINT('Ctrl Pts',(-27.5520190923677,-13.5428646240459,
113.936830505377)) ;
#175999=CARTESIAN_POINT('Ctrl Pts',(-27.5755268396356,-13.551991841175,
114.008431312637)) ;
#176000=CARTESIAN_POINT('Ctrl Pts',(-27.6493306793442,-13.5519919462692,
113.984200259648)) ;
#176001=CARTESIAN_POINT('Ctrl Pts',(-27.7231345190528,-13.5519920513634,
113.959969206658)) ;
#176002=CARTESIAN_POINT('Ctrl Pts',(-27.6996267717849,-13.5428648342343,
113.888368399397)) ;
#176003=CARTESIAN_POINT('Ctrl Pts',(-27.6873576347831,-13.252182353688,
113.886407116913)) ;
#176004=CARTESIAN_POINT('Ctrl Pts',(-27.6639387565465,-13.263336213575,
113.815076990438)) ;
#176005=CARTESIAN_POINT('Ctrl Pts',(-27.5901349081512,-13.2633361119795,
113.83930801697)) ;
#176006=CARTESIAN_POINT('Ctrl Pts',(-27.5163310597558,-13.2633360103841,
113.863539043501)) ;
#176007=CARTESIAN_POINT('Ctrl Pts',(-27.5397499379924,-13.2521821504971,
113.934869169976)) ;
#176008=CARTESIAN_POINT('Ctrl Pts',(-27.563168816229,-13.2410282906101,
114.00619929645)) ;
#176009=CARTESIAN_POINT('Ctrl Pts',(-27.6369726646243,-13.2410283922056,
113.981968269918)) ;
#176010=CARTESIAN_POINT('Ctrl Pts',(-27.7107765130197,-13.241028493801,
113.957737243387)) ;
#176011=CARTESIAN_POINT('Ctrl Pts',(-27.6873576347831,-13.252182353688,
113.886407116913)) ;
#176012=CARTESIAN_POINT('Ctrl Pts',(-27.651195526548,-12.9730234465435,
113.811707238471)) ;
#176013=CARTESIAN_POINT('Ctrl Pts',(-27.6295329359788,-13.0036840588297,
113.745726480929)) ;
#176014=CARTESIAN_POINT('Ctrl Pts',(-27.5557290797921,-13.0036839686776,
113.769957483729)) ;
#176015=CARTESIAN_POINT('Ctrl Pts',(-27.4819252236053,-13.0036838785254,
113.794188486529)) ;
#176016=CARTESIAN_POINT('Ctrl Pts',(-27.5035878141745,-12.9730232662392,
113.860169244071)) ;
#176017=CARTESIAN_POINT('Ctrl Pts',(-27.5252504047438,-12.9423626539529,
113.926150001612)) ;
#176018=CARTESIAN_POINT('Ctrl Pts',(-27.5990542609305,-12.942362744105,
113.901918998812)) ;
#176019=CARTESIAN_POINT('Ctrl Pts',(-27.6728581171173,-12.9423628342572,
113.877687996012)) ;
#176020=CARTESIAN_POINT('Ctrl Pts',(-27.651195526548,-12.9730234465435,
113.811707238471)) ;
#176021=CARTESIAN_POINT('Ctrl Pts',(-27.5924502457676,-12.724731390434,
113.668397807756)) ;
#176022=CARTESIAN_POINT('Ctrl Pts',(-27.5741193939568,-12.77277340565,113.612564989016)) ;
#176023=CARTESIAN_POINT('Ctrl Pts',(-27.5003155319448,-12.7727733343003,
113.636795974073)) ;
#176024=CARTESIAN_POINT('Ctrl Pts',(-27.4265116699327,-12.7727732629506,
113.66102695913)) ;
#176025=CARTESIAN_POINT('Ctrl Pts',(-27.4448425217436,-12.7247312477346,
113.716859777871)) ;
#176026=CARTESIAN_POINT('Ctrl Pts',(-27.4631733735544,-12.6766892325185,
113.772692596611)) ;
#176027=CARTESIAN_POINT('Ctrl Pts',(-27.5369772355664,-12.6766893038683,
113.748461611554)) ;
#176028=CARTESIAN_POINT('Ctrl Pts',(-27.6107810975784,-12.676689375218,
113.724230626497)) ;
#176029=CARTESIAN_POINT('Ctrl Pts',(-27.5924502457676,-12.724731390434,
113.668397807756)) ;
#176030=CARTESIAN_POINT('Ctrl Pts',(-27.5156633000477,-12.5280561031159,
113.469790960335)) ;
#176031=CARTESIAN_POINT('Ctrl Pts',(-27.5019362584244,-12.5899016984486,
113.427980604694)) ;
#176032=CARTESIAN_POINT('Ctrl Pts',(-27.4281323923887,-12.5899016481567,
113.452211577496)) ;
#176033=CARTESIAN_POINT('Ctrl Pts',(-27.354328526353,-12.5899015978648,
113.476442550298)) ;
#176034=CARTESIAN_POINT('Ctrl Pts',(-27.3680555679764,-12.5280560025322,
113.518252905939)) ;
#176035=CARTESIAN_POINT('Ctrl Pts',(-27.3817826095997,-12.4662104071995,
113.560063261581)) ;
#176036=CARTESIAN_POINT('Ctrl Pts',(-27.4555864756354,-12.4662104574914,
113.535832288779)) ;
#176037=CARTESIAN_POINT('Ctrl Pts',(-27.5293903416711,-12.4662105077833,
113.511601315976)) ;
#176038=CARTESIAN_POINT('Ctrl Pts',(-27.5156633000477,-12.5280561031159,
113.469790960335)) ;
#176039=CARTESIAN_POINT('Ctrl Pts',(-27.4242158235811,-12.3935893009494,
113.226845172422)) ;
#176040=CARTESIAN_POINT('Ctrl Pts',(-27.4161163215766,-12.4649167907205,
113.202175394608)) ;
#176041=CARTESIAN_POINT('Ctrl Pts',(-27.3423124544162,-12.464916764178,
113.226406363984)) ;
#176042=CARTESIAN_POINT('Ctrl Pts',(-27.2685085872558,-12.4649167376354,
113.250637333361)) ;
#176043=CARTESIAN_POINT('Ctrl Pts',(-27.2766080892603,-12.3935892478642,
113.275307111174)) ;
#176044=CARTESIAN_POINT('Ctrl Pts',(-27.2847075912648,-12.322261758093,
113.299976888988)) ;
#176045=CARTESIAN_POINT('Ctrl Pts',(-27.3585114584252,-12.3222617846356,
113.275745919611)) ;
#176046=CARTESIAN_POINT('Ctrl Pts',(-27.4323153255855,-12.3222618111782,
113.251514950235)) ;
#176047=CARTESIAN_POINT('Ctrl Pts',(-27.4242158235811,-12.3935893009494,
113.226845172422)) ;
#176048=CARTESIAN_POINT('Ctrl Pts',(-27.3251142958241,-12.333081965445,
112.960365809793)) ;
#176049=CARTESIAN_POINT('Ctrl Pts',(-27.3231899346653,-12.4087416290775,
112.954504514769)) ;
#176050=CARTESIAN_POINT('Ctrl Pts',(-27.2493860682454,-12.4087416242859,
112.9787354864)) ;
#176051=CARTESIAN_POINT('Ctrl Pts',(-27.1755822018255,-12.4087416194943,
113.002966458032)) ;
#176052=CARTESIAN_POINT('Ctrl Pts',(-27.1775065629843,-12.3330819558618,
113.008827753056)) ;
#176053=CARTESIAN_POINT('Ctrl Pts',(-27.179430924143,-12.2574222922293,
113.01468904808)) ;
#176054=CARTESIAN_POINT('Ctrl Pts',(-27.2532347905629,-12.2574222970209,
112.990458076449)) ;
#176055=CARTESIAN_POINT('Ctrl Pts',(-27.3270386569828,-12.2574223018125,
112.966227104817)) ;
#176056=CARTESIAN_POINT('Ctrl Pts',(-27.3251142958241,-12.333081965445,
112.960365809793)) ;
#176057=CARTESIAN_POINT('Ctrl Pts',(-27.2233916702717,-12.3505128306963,
112.686197908057)) ;
#176058=CARTESIAN_POINT('Ctrl Pts',(-27.2278287044319,-12.4250706656238,
112.699712396958)) ;
#176059=CARTESIAN_POINT('Ctrl Pts',(-27.1540248414432,-12.4250706786686,
112.723943379041)) ;
#176060=CARTESIAN_POINT('Ctrl Pts',(-27.0802209784545,-12.4250706917134,
112.748174361124)) ;
#176061=CARTESIAN_POINT('Ctrl Pts',(-27.0757839442942,-12.3505128567859,
112.734659872223)) ;
#176062=CARTESIAN_POINT('Ctrl Pts',(-27.0713469101339,-12.2759550218584,
112.721145383321)) ;
#176063=CARTESIAN_POINT('Ctrl Pts',(-27.1451507731226,-12.2759550088136,
112.696914401239)) ;
#176064=CARTESIAN_POINT('Ctrl Pts',(-27.2189546361114,-12.2759549957688,
112.672683419156)) ;
#176065=CARTESIAN_POINT('Ctrl Pts',(-27.2233916702717,-12.3505128306963,
112.686197908057)) ;
#176066=CARTESIAN_POINT('Ctrl Pts',(-27.12763956026,-12.4433828921911,112.429728050708)) ;
#176067=CARTESIAN_POINT('Ctrl Pts',(-27.1380408629042,-12.5115686405398,
112.46140873919)) ;
#176068=CARTESIAN_POINT('Ctrl Pts',(-27.0642370032903,-12.5115686671103,
112.485639731552)) ;
#176069=CARTESIAN_POINT('Ctrl Pts',(-26.9904331436763,-12.5115686936807,
112.509870723913)) ;
#176070=CARTESIAN_POINT('Ctrl Pts',(-26.980031841032,-12.443382945332,112.478190035431)) ;
#176071=CARTESIAN_POINT('Ctrl Pts',(-26.9696305383877,-12.3751971969833,
112.446509346949)) ;
#176072=CARTESIAN_POINT('Ctrl Pts',(-27.0434343980017,-12.3751971704129,
112.422278354588)) ;
#176073=CARTESIAN_POINT('Ctrl Pts',(-27.1172382576157,-12.3751971438424,
112.398047362226)) ;
#176074=CARTESIAN_POINT('Ctrl Pts',(-27.12763956026,-12.4433828921911,112.429728050708)) ;
#176075=CARTESIAN_POINT('Ctrl Pts',(-27.0415094033996,-12.607349424796,
112.20302769542)) ;
#176076=CARTESIAN_POINT('Ctrl Pts',(-27.0572028168899,-12.6641907157574,
112.25082729986)) ;
#176077=CARTESIAN_POINT('Ctrl Pts',(-26.9833989624742,-12.6641907484467,
112.275058308054)) ;
#176078=CARTESIAN_POINT('Ctrl Pts',(-26.9095951080584,-12.664190781136,
112.299289316249)) ;
#176079=CARTESIAN_POINT('Ctrl Pts',(-26.8939016945682,-12.6073494901747,
112.251489711809)) ;
#176080=CARTESIAN_POINT('Ctrl Pts',(-26.8782082810779,-12.5505081992133,
112.203690107369)) ;
#176081=CARTESIAN_POINT('Ctrl Pts',(-26.9520121354936,-12.5505081665239,
112.179459099174)) ;
#176082=CARTESIAN_POINT('Ctrl Pts',(-27.0258159899093,-12.5505081338346,
112.15522809098)) ;
#176083=CARTESIAN_POINT('Ctrl Pts',(-27.0415094033996,-12.607349424796,
112.20302769542)) ;
#176084=CARTESIAN_POINT('Ctrl Pts',(-26.9722746864344,-12.8279036385121,
112.027468698458)) ;
#176085=CARTESIAN_POINT('Ctrl Pts',(-26.9920950650029,-12.8694313461383,
112.087838372784)) ;
#176086=CARTESIAN_POINT('Ctrl Pts',(-26.9182912149163,-12.8694313807778,
112.112069394164)) ;
#176087=CARTESIAN_POINT('Ctrl Pts',(-26.8444873648296,-12.8694314154173,
112.136300415545)) ;
#176088=CARTESIAN_POINT('Ctrl Pts',(-26.8246669862611,-12.8279037077911,
112.075930741219)) ;
#176089=CARTESIAN_POINT('Ctrl Pts',(-26.8048466076927,-12.7863760001649,
112.015561066893)) ;
#176090=CARTESIAN_POINT('Ctrl Pts',(-26.8786504577793,-12.7863759655254,
111.991330045513)) ;
#176091=CARTESIAN_POINT('Ctrl Pts',(-26.9524543078659,-12.7863759308859,
111.967099024132)) ;
#176092=CARTESIAN_POINT('Ctrl Pts',(-26.9722746864344,-12.8279036385121,
112.027468698458)) ;
#176093=CARTESIAN_POINT('Ctrl Pts',(-26.9229312024064,-13.0930059035689,
111.912843276643)) ;
#176094=CARTESIAN_POINT('Ctrl Pts',(-26.9454890591512,-13.1160865947577,
111.981550868007)) ;
#176095=CARTESIAN_POINT('Ctrl Pts',(-26.8716852131677,-13.1160866238806,
112.005781901885)) ;
#176096=CARTESIAN_POINT('Ctrl Pts',(-26.7978813671843,-13.1160866530036,
112.030012935763)) ;
#176097=CARTESIAN_POINT('Ctrl Pts',(-26.7753235104395,-13.0930059618148,
111.961305344399)) ;
#176098=CARTESIAN_POINT('Ctrl Pts',(-26.7527656536947,-13.069925270626,
111.892597753036)) ;
#176099=CARTESIAN_POINT('Ctrl Pts',(-26.8265694996782,-13.069925241503,
111.868366719158)) ;
#176100=CARTESIAN_POINT('Ctrl Pts',(-26.9003733456616,-13.0699252123801,
111.84413568528)) ;
#176101=CARTESIAN_POINT('Ctrl Pts',(-26.9229312024064,-13.0930059035689,
111.912843276643)) ;
#176102=CARTESIAN_POINT('Ctrl Pts',(-26.8972324155193,-13.3789266137586,
111.86989142793)) ;
#176103=CARTESIAN_POINT('Ctrl Pts',(-26.9208877456924,-13.3820781397035,
111.941941746411)) ;
#176104=CARTESIAN_POINT('Ctrl Pts',(-26.8470839022087,-13.3820781631016,
111.966172787903)) ;
#176105=CARTESIAN_POINT('Ctrl Pts',(-26.7732800587249,-13.3820781864996,
111.990403829394)) ;
#176106=CARTESIAN_POINT('Ctrl Pts',(-26.7496247285517,-13.3789266605547,
111.918353510913)) ;
#176107=CARTESIAN_POINT('Ctrl Pts',(-26.7259693983785,-13.3757751346097,
111.846303192431)) ;
#176108=CARTESIAN_POINT('Ctrl Pts',(-26.7997732418623,-13.3757751112117,
111.82207215094)) ;
#176109=CARTESIAN_POINT('Ctrl Pts',(-26.8735770853461,-13.3757750878137,
111.797841109448)) ;
#176110=CARTESIAN_POINT('Ctrl Pts',(-26.8972324155193,-13.3789266137586,
111.86989142793)) ;
#176111=CARTESIAN_POINT('Ctrl Pts',(-26.89559593885,-13.6686885717782,111.900373113643)) ;
#176112=CARTESIAN_POINT('Ctrl Pts',(-26.9186673845928,-13.6516124113894,
111.970645014506)) ;
#176113=CARTESIAN_POINT('Ctrl Pts',(-26.8448635425279,-13.6516124266104,
111.99487606032)) ;
#176114=CARTESIAN_POINT('Ctrl Pts',(-26.771059700463,-13.6516124418314,
112.019107106133)) ;
#176115=CARTESIAN_POINT('Ctrl Pts',(-26.7479882547202,-13.6686886022201,
111.94883520527)) ;
#176116=CARTESIAN_POINT('Ctrl Pts',(-26.7249168089774,-13.6857647626089,
111.878563304406)) ;
#176117=CARTESIAN_POINT('Ctrl Pts',(-26.7987206510423,-13.6857647473879,
111.854332258593)) ;
#176118=CARTESIAN_POINT('Ctrl Pts',(-26.8725244931072,-13.6857647321669,
111.83010121278)) ;
#176119=CARTESIAN_POINT('Ctrl Pts',(-26.89559593885,-13.6686885717782,111.900373113643)) ;
#176120=CARTESIAN_POINT('Ctrl Pts',(-26.9176753989106,-13.9407698971193,
112.00311647252)) ;
#176121=CARTESIAN_POINT('Ctrl Pts',(-26.9385054854947,-13.9046696710089,
112.066561555162)) ;
#176122=CARTESIAN_POINT('Ctrl Pts',(-26.8647016435677,-13.904669678464,
112.090792601395)) ;
#176123=CARTESIAN_POINT('Ctrl Pts',(-26.7908978016408,-13.9046696859191,
112.115023647629)) ;
#176124=CARTESIAN_POINT('Ctrl Pts',(-26.7700677150567,-13.9407699120296,
112.051578564986)) ;
#176125=CARTESIAN_POINT('Ctrl Pts',(-26.7492376284726,-13.97687013814,111.988133482344)) ;
#176126=CARTESIAN_POINT('Ctrl Pts',(-26.8230414703995,-13.9768701306849,
111.963902436111)) ;
#176127=CARTESIAN_POINT('Ctrl Pts',(-26.8968453123265,-13.9768701232298,
111.939671389877)) ;
#176128=CARTESIAN_POINT('Ctrl Pts',(-26.9176753989106,-13.9407698971193,
112.00311647252)) ;
#176129=CARTESIAN_POINT('Ctrl Pts',(-26.9611957529866,-14.1754452261927,
112.171205228785)) ;
#176130=CARTESIAN_POINT('Ctrl Pts',(-26.978282970121,-14.122903887043,112.223250135106)) ;
#176131=CARTESIAN_POINT('Ctrl Pts',(-26.9044791274635,-14.1229038889288,
112.247481179114)) ;
#176132=CARTESIAN_POINT('Ctrl Pts',(-26.8306752848061,-14.1229038908147,
112.271712223123)) ;
#176133=CARTESIAN_POINT('Ctrl Pts',(-26.8135880676717,-14.1754452299645,
112.219667316802)) ;
#176134=CARTESIAN_POINT('Ctrl Pts',(-26.7965008505373,-14.2279865691142,
112.167622410482)) ;
#176135=CARTESIAN_POINT('Ctrl Pts',(-26.8703046931948,-14.2279865672284,
112.143391366473)) ;
#176136=CARTESIAN_POINT('Ctrl Pts',(-26.9441085358522,-14.2279865653425,
112.119160322465)) ;
#176137=CARTESIAN_POINT('Ctrl Pts',(-26.9611957529866,-14.1754452261927,
112.171205228785)) ;
#176138=CARTESIAN_POINT('Ctrl Pts',(-27.0218558744677,-14.3550939223612,
112.391319568465)) ;
#176139=CARTESIAN_POINT('Ctrl Pts',(-27.034001323059,-14.2899298530335,
112.428312645225)) ;
#176140=CARTESIAN_POINT('Ctrl Pts',(-26.9601974795246,-14.2899298524596,
112.452543686563)) ;
#176141=CARTESIAN_POINT('Ctrl Pts',(-26.8863936359901,-14.2899298518858,
112.4767747279)) ;
#176142=CARTESIAN_POINT('Ctrl Pts',(-26.8742481873988,-14.3550939212134,
112.43978165114)) ;
#176143=CARTESIAN_POINT('Ctrl Pts',(-26.8621027388075,-14.4202579905411,
112.402788574379)) ;
#176144=CARTESIAN_POINT('Ctrl Pts',(-26.9359065823419,-14.420257991115,
112.378557533042)) ;
#176145=CARTESIAN_POINT('Ctrl Pts',(-27.0097104258763,-14.4202579916889,
112.354326491705)) ;
#176146=CARTESIAN_POINT('Ctrl Pts',(-27.0218558744677,-14.3550939223612,
112.391319568465)) ;
#176147=CARTESIAN_POINT('Ctrl Pts',(-27.0954919754477,-14.468598908444,
112.65127280273)) ;
#176148=CARTESIAN_POINT('Ctrl Pts',(-27.1017753646167,-14.3954110161889,
112.670410992381)) ;
#176149=CARTESIAN_POINT('Ctrl Pts',(-27.0279715202262,-14.3954110152214,
112.694642031111)) ;
#176150=CARTESIAN_POINT('Ctrl Pts',(-26.9541676758356,-14.395411014254,
112.718873069841)) ;
#176151=CARTESIAN_POINT('Ctrl Pts',(-26.9478842866667,-14.4685989065091,
112.69973488019)) ;
#176152=CARTESIAN_POINT('Ctrl Pts',(-26.9416008974978,-14.5417867987642,
112.680596690539)) ;
#176153=CARTESIAN_POINT('Ctrl Pts',(-27.0154047418883,-14.5417867997317,
112.656365651809)) ;
#176154=CARTESIAN_POINT('Ctrl Pts',(-27.0892085862788,-14.5417868006991,
112.632134613079)) ;
#176155=CARTESIAN_POINT('Ctrl Pts',(-27.0954919754477,-14.468598908444,
112.65127280273)) ;
#176156=CARTESIAN_POINT('Ctrl Pts',(-27.1747095469528,-14.5058659881171,
112.927861658512)) ;
#176157=CARTESIAN_POINT('Ctrl Pts',(-27.1747399305109,-14.4299679241318,
112.927954201987)) ;
#176158=CARTESIAN_POINT('Ctrl Pts',(-27.1009360861394,-14.4299679242476,
112.952185240775)) ;
#176159=CARTESIAN_POINT('Ctrl Pts',(-27.027132241768,-14.4299679243634,
112.976416279563)) ;
#176160=CARTESIAN_POINT('Ctrl Pts',(-27.0271018582099,-14.5058659883488,
112.976323736088)) ;
#176161=CARTESIAN_POINT('Ctrl Pts',(-27.0270714746518,-14.5817640523341,
112.976231192613)) ;
#176162=CARTESIAN_POINT('Ctrl Pts',(-27.1008753190232,-14.5817640522183,
112.952000153825)) ;
#176163=CARTESIAN_POINT('Ctrl Pts',(-27.1746791633947,-14.5817640521025,
112.927769115037)) ;
#176164=CARTESIAN_POINT('Ctrl Pts',(-27.1747095469528,-14.5058659881171,
112.927861658512)) ;
#176165=CARTESIAN_POINT('Ctrl Pts',(-27.2540706728051,-14.465907705861,
113.205009023131)) ;
#176166=CARTESIAN_POINT('Ctrl Pts',(-27.247826374031,-14.3926881487027,
113.185989896604)) ;
#176167=CARTESIAN_POINT('Ctrl Pts',(-27.1740225302469,-14.3926881492861,
113.210220937181)) ;
#176168=CARTESIAN_POINT('Ctrl Pts',(-27.1002186864629,-14.3926881498695,
113.234451977758)) ;
#176169=CARTESIAN_POINT('Ctrl Pts',(-27.106462985237,-14.4659077070278,
113.253471104285)) ;
#176170=CARTESIAN_POINT('Ctrl Pts',(-27.112707284011,-14.5391272641861,
113.272490230812)) ;
#176171=CARTESIAN_POINT('Ctrl Pts',(-27.1865111277951,-14.5391272636027,
113.248259190235)) ;
#176172=CARTESIAN_POINT('Ctrl Pts',(-27.2603149715792,-14.5391272630193,
113.224028149658)) ;
#176173=CARTESIAN_POINT('Ctrl Pts',(-27.2540706728051,-14.465907705861,
113.205009023131)) ;
#176174=CARTESIAN_POINT('Ctrl Pts',(-27.3270117595021,-14.3507454275659,
113.462647263951)) ;
#176175=CARTESIAN_POINT('Ctrl Pts',(-27.3149310079399,-14.2854599330561,
113.425851243866)) ;
#176176=CARTESIAN_POINT('Ctrl Pts',(-27.2411271652632,-14.2854599321569,
113.450082287816)) ;
#176177=CARTESIAN_POINT('Ctrl Pts',(-27.1673233225865,-14.2854599312576,
113.474313331766)) ;
#176178=CARTESIAN_POINT('Ctrl Pts',(-27.1794040741487,-14.3507454257675,
113.51110935185)) ;
#176179=CARTESIAN_POINT('Ctrl Pts',(-27.1914848257109,-14.4160309202774,
113.547905371935)) ;
#176180=CARTESIAN_POINT('Ctrl Pts',(-27.2652886683876,-14.4160309211766,
113.523674327985)) ;
#176181=CARTESIAN_POINT('Ctrl Pts',(-27.3390925110643,-14.4160309220758,
113.499443284035)) ;
#176182=CARTESIAN_POINT('Ctrl Pts',(-27.3270117595021,-14.3507454275659,
113.462647263951)) ;
#176183=CARTESIAN_POINT('Ctrl Pts',(-27.3874657468428,-14.1684902162708,
113.682288696207)) ;
#176184=CARTESIAN_POINT('Ctrl Pts',(-27.3704113071499,-14.1158354027091,
113.63034362447)) ;
#176185=CARTESIAN_POINT('Ctrl Pts',(-27.2966074655942,-14.1158353972228,
113.654574671834)) ;
#176186=CARTESIAN_POINT('Ctrl Pts',(-27.2228036240385,-14.1158353917364,
113.678805719198)) ;
#176187=CARTESIAN_POINT('Ctrl Pts',(-27.2398580637314,-14.1684902052981,
113.730750790935)) ;
#176188=CARTESIAN_POINT('Ctrl Pts',(-27.2569125034242,-14.2211450188598,
113.782695862672)) ;
#176189=CARTESIAN_POINT('Ctrl Pts',(-27.33071634498,-14.2211450243462,113.758464815308)) ;
#176190=CARTESIAN_POINT('Ctrl Pts',(-27.4045201865357,-14.2211450298325,
113.734233767944)) ;
#176191=CARTESIAN_POINT('Ctrl Pts',(-27.3874657468428,-14.1684902162708,
113.682288696207)) ;
#176192=CARTESIAN_POINT('Ctrl Pts',(-27.4302106667087,-13.9330107336615,
113.847901657391)) ;
#176193=CARTESIAN_POINT('Ctrl Pts',(-27.4094139181739,-13.8967214466837,
113.784558116622)) ;
#176194=CARTESIAN_POINT('Ctrl Pts',(-27.3356100770456,-13.8967214344113,
113.808789165288)) ;
#176195=CARTESIAN_POINT('Ctrl Pts',(-27.2618062359173,-13.8967214221389,
113.833020213954)) ;
#176196=CARTESIAN_POINT('Ctrl Pts',(-27.282602984452,-13.9330107091168,
113.896363754723)) ;
#176197=CARTESIAN_POINT('Ctrl Pts',(-27.3033997329868,-13.9692999960946,
113.959707295493)) ;
#176198=CARTESIAN_POINT('Ctrl Pts',(-27.3772035741151,-13.969300008367,
113.935476246827)) ;
#176199=CARTESIAN_POINT('Ctrl Pts',(-27.4510074152434,-13.9693000206394,
113.911245198161)) ;
#176200=CARTESIAN_POINT('Ctrl Pts',(-27.4302106667087,-13.9330107336615,
113.847901657391)) ;
#176201=CARTESIAN_POINT('Ctrl Pts',(-27.4515998140738,-13.6600763512271,
113.948553659072)) ;
#176202=CARTESIAN_POINT('Ctrl Pts',(-27.4285447209372,-13.6427914121404,
113.878331564877)) ;
#176203=CARTESIAN_POINT('Ctrl Pts',(-27.3547408792523,-13.6427913908253,
113.902562611848)) ;
#176204=CARTESIAN_POINT('Ctrl Pts',(-27.2809370375673,-13.6427913695102,
113.926793658818)) ;
#176205=CARTESIAN_POINT('Ctrl Pts',(-27.3039921307039,-13.6600763085969,
113.997015753013)) ;
#176206=CARTESIAN_POINT('Ctrl Pts',(-27.3270472238404,-13.6773612476836,
114.067237847207)) ;
#176207=CARTESIAN_POINT('Ctrl Pts',(-27.4008510655254,-13.6773612689987,
114.043006800237)) ;
#176208=CARTESIAN_POINT('Ctrl Pts',(-27.4746549072103,-13.6773612903137,
114.018775753266)) ;
#176209=CARTESIAN_POINT('Ctrl Pts',(-27.4515998140738,-13.6600763512271,
113.948553659072)) ;
#176210=CARTESIAN_POINT('Ctrl Pts',(-27.4493246185078,-13.3704757504778,
113.977035138527)) ;
#176211=CARTESIAN_POINT('Ctrl Pts',(-27.4256622922529,-13.3733860820227,
113.904963510084)) ;
#176212=CARTESIAN_POINT('Ctrl Pts',(-27.3518584487016,-13.3733860523621,
113.92919455137)) ;
#176213=CARTESIAN_POINT('Ctrl Pts',(-27.2780546051503,-13.3733860227015,
113.953425592656)) ;
#176214=CARTESIAN_POINT('Ctrl Pts',(-27.3017169314052,-13.3704756911566,
114.025497221099)) ;
#176215=CARTESIAN_POINT('Ctrl Pts',(-27.3253792576601,-13.3675653596117,
114.097568849542)) ;
#176216=CARTESIAN_POINT('Ctrl Pts',(-27.3991831012114,-13.3675653892723,
114.073337808256)) ;
#176217=CARTESIAN_POINT('Ctrl Pts',(-27.4729869447627,-13.3675654189329,
114.04910676697)) ;
#176218=CARTESIAN_POINT('Ctrl Pts',(-27.4493246185078,-13.3704757504778,
113.977035138527)) ;
#176219=CARTESIAN_POINT('Ctrl Pts',(-27.4224958680665,-13.0823700026988,
113.93098284499)) ;
#176220=CARTESIAN_POINT('Ctrl Pts',(-27.3999343634008,-13.1054004112685,
113.862264141289)) ;
#176221=CARTESIAN_POINT('Ctrl Pts',(-27.3261305163557,-13.1054003729185,
113.886495171933)) ;
#176222=CARTESIAN_POINT('Ctrl Pts',(-27.2523266693107,-13.1054003345686,
113.910726202578)) ;
#176223=CARTESIAN_POINT('Ctrl Pts',(-27.2748881739764,-13.0823699259989,
113.979444906279)) ;
#176224=CARTESIAN_POINT('Ctrl Pts',(-27.2974496786422,-13.0593395174292,
114.048163609981)) ;
#176225=CARTESIAN_POINT('Ctrl Pts',(-27.3712535256872,-13.0593395557792,
114.023932579336)) ;
#176226=CARTESIAN_POINT('Ctrl Pts',(-27.4450573727323,-13.0593395941291,
113.999701548692)) ;
#176227=CARTESIAN_POINT('Ctrl Pts',(-27.4224958680665,-13.0823700026988,
113.93098284499)) ;
#176228=CARTESIAN_POINT('Ctrl Pts',(-27.3729809937545,-12.8213180178566,
113.815427357995)) ;
#176229=CARTESIAN_POINT('Ctrl Pts',(-27.3531145848407,-12.8626079589609,
113.754917480972)) ;
#176230=CARTESIAN_POINT('Ctrl Pts',(-27.2793107335955,-12.862607919451,
113.779148498824)) ;
#176231=CARTESIAN_POINT('Ctrl Pts',(-27.2055068823504,-12.8626078799411,
113.803379516675)) ;
#176232=CARTESIAN_POINT('Ctrl Pts',(-27.2253732912641,-12.8213179388368,
113.863889393698)) ;
#176233=CARTESIAN_POINT('Ctrl Pts',(-27.2452397001779,-12.7800279977325,
113.92439927072)) ;
#176234=CARTESIAN_POINT('Ctrl Pts',(-27.3190435514231,-12.7800280372424,
113.900168252869)) ;
#176235=CARTESIAN_POINT('Ctrl Pts',(-27.3928474026682,-12.7800280767523,
113.875937235017)) ;
#176236=CARTESIAN_POINT('Ctrl Pts',(-27.3729809937545,-12.8213180178566,
113.815427357995)) ;
#176237=CARTESIAN_POINT('Ctrl Pts',(-27.3028037991072,-12.6009816910039,
113.637217641596)) ;
#176238=CARTESIAN_POINT('Ctrl Pts',(-27.2870729381168,-12.6577150521394,
113.589303976099)) ;
#176239=CARTESIAN_POINT('Ctrl Pts',(-27.2132690817063,-12.6577150144821,
113.613534978217)) ;
#176240=CARTESIAN_POINT('Ctrl Pts',(-27.1394652252959,-12.6577149768248,
113.637765980336)) ;
#176241=CARTESIAN_POINT('Ctrl Pts',(-27.1551960862862,-12.6009816156892,
113.685679645834)) ;
#176242=CARTESIAN_POINT('Ctrl Pts',(-27.1709269472766,-12.5442482545536,
113.733593311332)) ;
#176243=CARTESIAN_POINT('Ctrl Pts',(-27.2447308036871,-12.5442482922109,
113.709362309213)) ;
#176244=CARTESIAN_POINT('Ctrl Pts',(-27.3185346600976,-12.5442483298683,
113.685131307094)) ;
#176245=CARTESIAN_POINT('Ctrl Pts',(-27.3028037991072,-12.6009816910039,
113.637217641596)) ;
#176246=CARTESIAN_POINT('Ctrl Pts',(-27.2168540748088,-12.4399155910324,
113.410819058086)) ;
#176247=CARTESIAN_POINT('Ctrl Pts',(-27.2063690680483,-12.5079761461326,
113.378883418007)) ;
#176248=CARTESIAN_POINT('Ctrl Pts',(-27.132565206792,-12.5079761174331,
113.403114405366)) ;
#176249=CARTESIAN_POINT('Ctrl Pts',(-27.0587613455356,-12.5079760887335,
113.427345392725)) ;
#176250=CARTESIAN_POINT('Ctrl Pts',(-27.0692463522961,-12.4399155336333,
113.459281032804)) ;
#176251=CARTESIAN_POINT('Ctrl Pts',(-27.0797313590565,-12.3718549785331,
113.491216672884)) ;
#176252=CARTESIAN_POINT('Ctrl Pts',(-27.1535352203129,-12.3718550072327,
113.466985685525)) ;
#176253=CARTESIAN_POINT('Ctrl Pts',(-27.2273390815693,-12.3718550359322,
113.442754698166)) ;
#176254=CARTESIAN_POINT('Ctrl Pts',(-27.2168540748088,-12.4399155910324,
113.410819058086)) ;
#176255=CARTESIAN_POINT('Ctrl Pts',(-27.1197079246416,-12.3483508718252,
113.15053363995)) ;
#176256=CARTESIAN_POINT('Ctrl Pts',(-27.1152534269706,-12.4229031690547,
113.136965957357)) ;
#176257=CARTESIAN_POINT('Ctrl Pts',(-27.0414495611112,-12.4229031549688,
113.161196930696)) ;
#176258=CARTESIAN_POINT('Ctrl Pts',(-26.9676456952518,-12.4229031408829,
113.185427904035)) ;
#176259=CARTESIAN_POINT('Ctrl Pts',(-26.9721001929228,-12.3483508436534,
113.198995586628)) ;
#176260=CARTESIAN_POINT('Ctrl Pts',(-26.9765546905938,-12.2737985464239,
113.212563269221)) ;
#176261=CARTESIAN_POINT('Ctrl Pts',(-27.0503585564532,-12.2737985605098,
113.188332295882)) ;
#176262=CARTESIAN_POINT('Ctrl Pts',(-27.1241624223126,-12.2737985745957,
113.164101322543)) ;
#176263=CARTESIAN_POINT('Ctrl Pts',(-27.1197079246416,-12.3483508718252,
113.15053363995)) ;
#176264=CARTESIAN_POINT('Ctrl Pts',(-27.0187802117475,-12.3338872424077,
112.878480782108)) ;
#176265=CARTESIAN_POINT('Ctrl Pts',(-27.0206341859005,-12.4095571114995,
112.884127686696)) ;
#176266=CARTESIAN_POINT('Ctrl Pts',(-26.9468303176289,-12.4095571176329,
112.908358652687)) ;
#176267=CARTESIAN_POINT('Ctrl Pts',(-26.8730264493573,-12.4095571237664,
112.932589618679)) ;
#176268=CARTESIAN_POINT('Ctrl Pts',(-26.8711724752043,-12.3338872546745,
112.926942714091)) ;
#176269=CARTESIAN_POINT('Ctrl Pts',(-26.8693185010513,-12.2582173855827,
112.921295809504)) ;
#176270=CARTESIAN_POINT('Ctrl Pts',(-26.9431223693229,-12.2582173794493,
112.897064843512)) ;
#176271=CARTESIAN_POINT('Ctrl Pts',(-27.0169262375945,-12.2582173733159,
112.87283387752)) ;
#176272=CARTESIAN_POINT('Ctrl Pts',(-27.0187802117475,-12.3338872424077,
112.878480782108)) ;
#176273=CARTESIAN_POINT('Ctrl Pts',(-26.9193985159767,-12.396923495094,
112.611312558498)) ;
#176274=CARTESIAN_POINT('Ctrl Pts',(-26.9274584480283,-12.4683025104667,
112.635861809373)) ;
#176275=CARTESIAN_POINT('Ctrl Pts',(-26.8536545789805,-12.4683025400751,
112.660092773001)) ;
#176276=CARTESIAN_POINT('Ctrl Pts',(-26.7798507099327,-12.4683025696834,
112.684323736628)) ;
#176277=CARTESIAN_POINT('Ctrl Pts',(-26.7717907778811,-12.3969235543106,
112.659774485753)) ;
#176278=CARTESIAN_POINT('Ctrl Pts',(-26.7637308458295,-12.3255445389379,
112.635225234877)) ;
#176279=CARTESIAN_POINT('Ctrl Pts',(-26.8375347148773,-12.3255445093296,
112.61099427125)) ;
#176280=CARTESIAN_POINT('Ctrl Pts',(-26.9113385839251,-12.3255444797213,
112.586763307622)) ;
#176281=CARTESIAN_POINT('Ctrl Pts',(-26.9193985159767,-12.396923495094,
112.611312558498)) ;
#176282=CARTESIAN_POINT('Ctrl Pts',(-26.8285566748927,-12.5334553693914,
112.370120041222)) ;
#176283=CARTESIAN_POINT('Ctrl Pts',(-26.8422361287122,-12.595406254364,
112.411785448577)) ;
#176284=CARTESIAN_POINT('Ctrl Pts',(-26.7684322615119,-12.5954063084814,
112.436016417832)) ;
#176285=CARTESIAN_POINT('Ctrl Pts',(-26.6946283943116,-12.5954063625988,
112.460247387086)) ;
#176286=CARTESIAN_POINT('Ctrl Pts',(-26.6809489404921,-12.5334554776262,
112.418581979731)) ;
#176287=CARTESIAN_POINT('Ctrl Pts',(-26.6672694866725,-12.4715045926535,
112.376916572376)) ;
#176288=CARTESIAN_POINT('Ctrl Pts',(-26.7410733538728,-12.4715045385361,
112.352685603122)) ;
#176289=CARTESIAN_POINT('Ctrl Pts',(-26.8148772210732,-12.4715044844187,
112.328454633867)) ;
#176290=CARTESIAN_POINT('Ctrl Pts',(-26.8285566748927,-12.5334553693914,
112.370120041222)) ;
#176291=CARTESIAN_POINT('Ctrl Pts',(-26.7522001619182,-12.7322215761211,
112.172876186384)) ;
#176292=CARTESIAN_POINT('Ctrl Pts',(-26.7704995100276,-12.7803853400704,
112.228613046245)) ;
#176293=CARTESIAN_POINT('Ctrl Pts',(-26.696695647293,-12.7803854158274,
112.252844029101)) ;
#176294=CARTESIAN_POINT('Ctrl Pts',(-26.6228917845584,-12.7803854915845,
112.277075011958)) ;
#176295=CARTESIAN_POINT('Ctrl Pts',(-26.604592436449,-12.7322217276352,
112.221338152097)) ;
#176296=CARTESIAN_POINT('Ctrl Pts',(-26.5862930883396,-12.6840579636859,
112.165601292236)) ;
#176297=CARTESIAN_POINT('Ctrl Pts',(-26.6600969510742,-12.6840578879289,
112.141370309379)) ;
#176298=CARTESIAN_POINT('Ctrl Pts',(-26.7339008138088,-12.6840578121718,
112.117139326523)) ;
#176299=CARTESIAN_POINT('Ctrl Pts',(-26.7522001619182,-12.7322215761211,
112.172876186384)) ;
#176300=CARTESIAN_POINT('Ctrl Pts',(-26.6943187231654,-12.9810049412899,
112.032078055127)) ;
#176301=CARTESIAN_POINT('Ctrl Pts',(-26.7159513885438,-13.0118702151138,
112.097967661475)) ;
#176302=CARTESIAN_POINT('Ctrl Pts',(-26.6421475322302,-13.0118703086727,
112.122198663889)) ;
#176303=CARTESIAN_POINT('Ctrl Pts',(-26.5683436759166,-13.0118704022315,
112.146429666303)) ;
#176304=CARTESIAN_POINT('Ctrl Pts',(-26.5467110105383,-12.9810051284076,
112.080540059955)) ;
#176305=CARTESIAN_POINT('Ctrl Pts',(-26.52507834516,-12.9501398545836,112.014650453607)) ;
#176306=CARTESIAN_POINT('Ctrl Pts',(-26.5988822014735,-12.9501397610248,
111.990419451193)) ;
#176307=CARTESIAN_POINT('Ctrl Pts',(-26.6726860577871,-12.9501396674659,
111.966188448779)) ;
#176308=CARTESIAN_POINT('Ctrl Pts',(-26.6943187231654,-12.9810049412899,
112.032078055127)) ;
#176309=CARTESIAN_POINT('Ctrl Pts',(-26.6587912592978,-13.2609753303157,
111.959335470938)) ;
#176310=CARTESIAN_POINT('Ctrl Pts',(-26.6822021833276,-13.2723394892272,
112.030641366156)) ;
#176311=CARTESIAN_POINT('Ctrl Pts',(-26.6083983351151,-13.2723395935458,
112.054872393245)) ;
#176312=CARTESIAN_POINT('Ctrl Pts',(-26.5345944869027,-13.2723396978644,
112.079103420333)) ;
#176313=CARTESIAN_POINT('Ctrl Pts',(-26.511183562873,-13.260975538953,112.007797525115)) ;
#176314=CARTESIAN_POINT('Ctrl Pts',(-26.4877726388432,-13.2496113800415,
111.936491629897)) ;
#176315=CARTESIAN_POINT('Ctrl Pts',(-26.5615764870557,-13.2496112757229,
111.912260602808)) ;
#176316=CARTESIAN_POINT('Ctrl Pts',(-26.6353803352681,-13.2496111714043,
111.88802957572)) ;
#176317=CARTESIAN_POINT('Ctrl Pts',(-26.6587912592978,-13.2609753303157,
111.959335470938)) ;
#176318=CARTESIAN_POINT('Ctrl Pts',(-26.647319062969,-13.5522070361543,
111.959866894059)) ;
#176319=CARTESIAN_POINT('Ctrl Pts',(-26.6708314077499,-13.5432552863656,
112.031481700481)) ;
#176320=CARTESIAN_POINT('Ctrl Pts',(-26.59702756845,-13.5432553930549,112.055712754716)) ;
#176321=CARTESIAN_POINT('Ctrl Pts',(-26.52322372915,-13.5432554997441,112.079943808951)) ;
#176322=CARTESIAN_POINT('Ctrl Pts',(-26.4997113843691,-13.5522072495328,
112.008329002528)) ;
#176323=CARTESIAN_POINT('Ctrl Pts',(-26.4761990395882,-13.5611589993214,
111.936714196106)) ;
#176324=CARTESIAN_POINT('Ctrl Pts',(-26.5500028788881,-13.5611588926322,
111.912483141871)) ;
#176325=CARTESIAN_POINT('Ctrl Pts',(-26.623806718188,-13.5611587859429,
111.888252087637)) ;
#176326=CARTESIAN_POINT('Ctrl Pts',(-26.647319062969,-13.5522070361543,
111.959866894059)) ;
#176327=CARTESIAN_POINT('Ctrl Pts',(-26.6599556627793,-13.8335794690488,
112.033796091262)) ;
#176328=CARTESIAN_POINT('Ctrl Pts',(-26.6818871675792,-13.8049701426201,
112.100595914152)) ;
#176329=CARTESIAN_POINT('Ctrl Pts',(-26.6080833370899,-13.8049702427903,
112.124826995223)) ;
#176330=CARTESIAN_POINT('Ctrl Pts',(-26.5342795066006,-13.8049703429605,
112.149058076293)) ;
#176331=CARTESIAN_POINT('Ctrl Pts',(-26.5123480018007,-13.8335796693892,
112.082258253403)) ;
#176332=CARTESIAN_POINT('Ctrl Pts',(-26.4904164970008,-13.862188995818,
112.015458430512)) ;
#176333=CARTESIAN_POINT('Ctrl Pts',(-26.5642203274901,-13.8621888956478,
111.991227349442)) ;
#176334=CARTESIAN_POINT('Ctrl Pts',(-26.6380241579794,-13.8621887954776,
111.966996268371)) ;
#176335=CARTESIAN_POINT('Ctrl Pts',(-26.6599556627793,-13.8335794690488,
112.033796091262)) ;
#176336=CARTESIAN_POINT('Ctrl Pts',(-26.6950792057711,-14.0854850074698,
112.176258032588)) ;
#176337=CARTESIAN_POINT('Ctrl Pts',(-26.7138568726991,-14.0392461681425,
112.233451774195)) ;
#176338=CARTESIAN_POINT('Ctrl Pts',(-26.6400530500181,-14.0392462534928,
112.257682879048)) ;
#176339=CARTESIAN_POINT('Ctrl Pts',(-26.5662492273371,-14.039246338843,
112.281913983902)) ;
#176340=CARTESIAN_POINT('Ctrl Pts',(-26.5474715604091,-14.0854851781703,
112.224720242295)) ;
#176341=CARTESIAN_POINT('Ctrl Pts',(-26.5286938934811,-14.1317240174977,
112.167526500688)) ;
#176342=CARTESIAN_POINT('Ctrl Pts',(-26.6024977161621,-14.1317239321474,
112.143295395835)) ;
#176343=CARTESIAN_POINT('Ctrl Pts',(-26.6763015388431,-14.1317238467972,
112.119064290982)) ;
#176344=CARTESIAN_POINT('Ctrl Pts',(-26.6950792057711,-14.0854850074698,
112.176258032588)) ;
#176345=CARTESIAN_POINT('Ctrl Pts',(-26.7493678080384,-14.2893882283517,
112.377063192394)) ;
#176346=CARTESIAN_POINT('Ctrl Pts',(-26.7636496039739,-14.2288448467623,
112.42056323639)) ;
#176347=CARTESIAN_POINT('Ctrl Pts',(-26.6898457872909,-14.2288449105474,
112.444794359512)) ;
#176348=CARTESIAN_POINT('Ctrl Pts',(-26.6160419706078,-14.2288449743324,
112.469025482634)) ;
#176349=CARTESIAN_POINT('Ctrl Pts',(-26.6017601746723,-14.2893883559219,
112.425525438638)) ;
#176350=CARTESIAN_POINT('Ctrl Pts',(-26.5874783787368,-14.3499317375113,
112.382025394642)) ;
#176351=CARTESIAN_POINT('Ctrl Pts',(-26.6612821954199,-14.3499316737262,
112.35779427152)) ;
#176352=CARTESIAN_POINT('Ctrl Pts',(-26.7350860121029,-14.3499316099411,
112.333563148398)) ;
#176353=CARTESIAN_POINT('Ctrl Pts',(-26.7493678080384,-14.2893882283517,
112.377063192394)) ;
#176354=CARTESIAN_POINT('Ctrl Pts',(-26.8182694831193,-14.4310416708449,
112.622412303935)) ;
#176355=CARTESIAN_POINT('Ctrl Pts',(-26.8270278462195,-14.3605181681089,
112.649088862766)) ;
#176356=CARTESIAN_POINT('Ctrl Pts',(-26.7532240331301,-14.3605182058442,
112.673319996834)) ;
#176357=CARTESIAN_POINT('Ctrl Pts',(-26.6794202200406,-14.3605182435796,
112.697551130901)) ;
#176358=CARTESIAN_POINT('Ctrl Pts',(-26.6706618569405,-14.4310417463156,
112.67087457207)) ;
#176359=CARTESIAN_POINT('Ctrl Pts',(-26.6619034938403,-14.5015652490516,
112.644198013239)) ;
#176360=CARTESIAN_POINT('Ctrl Pts',(-26.7357073069297,-14.5015652113162,
112.619966879171)) ;
#176361=CARTESIAN_POINT('Ctrl Pts',(-26.8095111200191,-14.5015651735809,
112.595735745103)) ;
#176362=CARTESIAN_POINT('Ctrl Pts',(-26.8182694831193,-14.4310416708449,
112.622412303935)) ;
#176363=CARTESIAN_POINT('Ctrl Pts',(-26.8960209759952,-14.4999960091202,
112.894701404491)) ;
#176364=CARTESIAN_POINT('Ctrl Pts',(-26.8986301066341,-14.4245527843061,
112.902648393491)) ;
#176365=CARTESIAN_POINT('Ctrl Pts',(-26.8248262944529,-14.4245527944394,
112.926879530325)) ;
#176366=CARTESIAN_POINT('Ctrl Pts',(-26.7510224822716,-14.4245528045727,
112.951110667159)) ;
#176367=CARTESIAN_POINT('Ctrl Pts',(-26.7484133516328,-14.4999960293868,
112.943163678159)) ;
#176368=CARTESIAN_POINT('Ctrl Pts',(-26.7458042209939,-14.5754392542009,
112.93521668916)) ;
#176369=CARTESIAN_POINT('Ctrl Pts',(-26.8196080331751,-14.5754392440676,
112.910985552326)) ;
#176370=CARTESIAN_POINT('Ctrl Pts',(-26.8934118453563,-14.5754392339344,
112.886754415492)) ;
#176371=CARTESIAN_POINT('Ctrl Pts',(-26.8960209759952,-14.4999960091202,
112.894701404491)) ;
#176372=CARTESIAN_POINT('Ctrl Pts',(-26.9762322526902,-14.4914668725251,
113.174447910469)) ;
#176373=CARTESIAN_POINT('Ctrl Pts',(-26.9725118930449,-14.4165060453907,
113.163116293409)) ;
#176374=CARTESIAN_POINT('Ctrl Pts',(-26.8987080792064,-14.4165060293028,
113.187347425195)) ;
#176375=CARTESIAN_POINT('Ctrl Pts',(-26.8249042653679,-14.416506013215,
113.211578556981)) ;
#176376=CARTESIAN_POINT('Ctrl Pts',(-26.8286246250133,-14.4914668403494,
113.222910174041)) ;
#176377=CARTESIAN_POINT('Ctrl Pts',(-26.8323449846586,-14.5664276674838,
113.234241791102)) ;
#176378=CARTESIAN_POINT('Ctrl Pts',(-26.906148798497,-14.5664276835716,
113.210010659315)) ;
#176379=CARTESIAN_POINT('Ctrl Pts',(-26.9799526123356,-14.5664276996595,
113.185779527529)) ;
#176380=CARTESIAN_POINT('Ctrl Pts',(-26.9762322526902,-14.4914668725251,
113.174447910469)) ;
#176381=CARTESIAN_POINT('Ctrl Pts',(-27.0525399232105,-14.4062237339893,
113.44231798111)) ;
#176382=CARTESIAN_POINT('Ctrl Pts',(-27.0427528161706,-14.3371017134928,
113.412508030457)) ;
#176383=CARTESIAN_POINT('Ctrl Pts',(-26.9689489983906,-14.337101674971,
113.436739150238)) ;
#176384=CARTESIAN_POINT('Ctrl Pts',(-26.8951451806107,-14.3371016364492,
113.460970270019)) ;
#176385=CARTESIAN_POINT('Ctrl Pts',(-26.9049322876505,-14.4062236569457,
113.490780220672)) ;
#176386=CARTESIAN_POINT('Ctrl Pts',(-26.9147193946903,-14.4753456774423,
113.520590171325)) ;
#176387=CARTESIAN_POINT('Ctrl Pts',(-26.9885232124703,-14.4753457159641,
113.496359051544)) ;
#176388=CARTESIAN_POINT('Ctrl Pts',(-27.0623270302503,-14.4753457544858,
113.472127931763)) ;
#176389=CARTESIAN_POINT('Ctrl Pts',(-27.0525399232105,-14.4062237339893,
113.44231798111)) ;
#176390=CARTESIAN_POINT('Ctrl Pts',(-27.1188648773087,-14.2495321967945,
113.679899921954)) ;
#176391=CARTESIAN_POINT('Ctrl Pts',(-27.103696319169,-14.1912456004984,
113.633698939684)) ;
#176392=CARTESIAN_POINT('Ctrl Pts',(-27.0298924955446,-14.1912455461204,
113.657930041664)) ;
#176393=CARTESIAN_POINT('Ctrl Pts',(-26.9560886719202,-14.1912454917425,
113.682161143644)) ;
#176394=CARTESIAN_POINT('Ctrl Pts',(-26.9712572300598,-14.2495320880387,
113.728362125914)) ;
#176395=CARTESIAN_POINT('Ctrl Pts',(-26.9864257881994,-14.3078186843349,
113.774563108183)) ;
#176396=CARTESIAN_POINT('Ctrl Pts',(-27.0602296118238,-14.3078187387128,
113.750332006204)) ;
#176397=CARTESIAN_POINT('Ctrl Pts',(-27.1340334354483,-14.3078187930907,
113.726100904224)) ;
#176398=CARTESIAN_POINT('Ctrl Pts',(-27.1188648773087,-14.2495321967945,
113.679899921954)) ;
#176399=CARTESIAN_POINT('Ctrl Pts',(-27.1692281183874,-14.0340281298451,
113.868701151054)) ;
#176400=CARTESIAN_POINT('Ctrl Pts',(-27.149787780751,-13.990699945468,113.809489017816)) ;
#176401=CARTESIAN_POINT('Ctrl Pts',(-27.075983950736,-13.9906998817967,
113.833720100331)) ;
#176402=CARTESIAN_POINT('Ctrl Pts',(-27.0021801207209,-13.9906998181254,
113.857951182846)) ;
#176403=CARTESIAN_POINT('Ctrl Pts',(-27.0216204583573,-14.0340280025025,
113.917163316084)) ;
#176404=CARTESIAN_POINT('Ctrl Pts',(-27.0410607959936,-14.0773561868796,
113.976375449322)) ;
#176405=CARTESIAN_POINT('Ctrl Pts',(-27.1148646260087,-14.0773562505509,
113.952144366807)) ;
#176406=CARTESIAN_POINT('Ctrl Pts',(-27.1886684560238,-14.0773563142222,
113.927913284292)) ;
#176407=CARTESIAN_POINT('Ctrl Pts',(-27.1692281183874,-14.0340281298451,
113.868701151054)) ;
#176408=CARTESIAN_POINT('Ctrl Pts',(-27.1996623984703,-13.7742259092907,
113.99685412237)) ;
#176409=CARTESIAN_POINT('Ctrl Pts',(-27.1773340852671,-13.7489714833696,
113.928845681678)) ;
#176410=CARTESIAN_POINT('Ctrl Pts',(-27.1035302487081,-13.7489714178304,
113.953076744261)) ;
#176411=CARTESIAN_POINT('Ctrl Pts',(-27.0297264121491,-13.7489713522911,
113.977307806844)) ;
#176412=CARTESIAN_POINT('Ctrl Pts',(-27.0520547253523,-13.7742257782122,
114.045316247537)) ;
#176413=CARTESIAN_POINT('Ctrl Pts',(-27.0743830385556,-13.7994802041333,
114.113324688229)) ;
#176414=CARTESIAN_POINT('Ctrl Pts',(-27.1481868751146,-13.7994802696726,
114.089093625646)) ;
#176415=CARTESIAN_POINT('Ctrl Pts',(-27.2219907116736,-13.7994803352118,
114.064862563063)) ;
#176416=CARTESIAN_POINT('Ctrl Pts',(-27.1996623984703,-13.7742259092907,
113.99685412237)) ;
#176417=CARTESIAN_POINT('Ctrl Pts',(-27.2071696580136,-13.488993839479,
114.055160255525)) ;
#176418=CARTESIAN_POINT('Ctrl Pts',(-27.1835500172681,-13.4836161224244,
113.983218639649)) ;
#176419=CARTESIAN_POINT('Ctrl Pts',(-27.1097461748366,-13.4836160614426,
114.007449684346)) ;
#176420=CARTESIAN_POINT('Ctrl Pts',(-27.0359423324051,-13.4836160004609,
114.031680729042)) ;
#176421=CARTESIAN_POINT('Ctrl Pts',(-27.0595619731506,-13.4889937175154,
114.103622344918)) ;
#176422=CARTESIAN_POINT('Ctrl Pts',(-27.0831816138961,-13.49437143457,114.175563960794)) ;
#176423=CARTESIAN_POINT('Ctrl Pts',(-27.1569854563276,-13.4943714955518,
114.151332916098)) ;
#176424=CARTESIAN_POINT('Ctrl Pts',(-27.2307892987591,-13.4943715565336,
114.127101871401)) ;
#176425=CARTESIAN_POINT('Ctrl Pts',(-27.2071696580136,-13.488993839479,
114.055160255525)) ;
#176426=CARTESIAN_POINT('Ctrl Pts',(-27.1902825049831,-13.1975717487405,
114.039308325117)) ;
#176427=CARTESIAN_POINT('Ctrl Pts',(-27.1670696758155,-13.2125333094721,
113.968605791857)) ;
#176428=CARTESIAN_POINT('Ctrl Pts',(-27.0932658289276,-13.2125332593627,
113.99283682298)) ;
#176429=CARTESIAN_POINT('Ctrl Pts',(-27.0194619820398,-13.2125332092533,
114.017067854103)) ;
#176430=CARTESIAN_POINT('Ctrl Pts',(-27.0426748112073,-13.1975716485217,
114.087770387363)) ;
#176431=CARTESIAN_POINT('Ctrl Pts',(-27.0658876403749,-13.1826100877902,
114.158472920623)) ;
#176432=CARTESIAN_POINT('Ctrl Pts',(-27.1396914872628,-13.1826101378995,
114.1342418895)) ;
#176433=CARTESIAN_POINT('Ctrl Pts',(-27.2134953341506,-13.1826101880089,
114.110010858377)) ;
#176434=CARTESIAN_POINT('Ctrl Pts',(-27.1902825049831,-13.1975717487405,
114.039308325117)) ;
#176435=CARTESIAN_POINT('Ctrl Pts',(-27.1498141482332,-12.9237175982201,
113.951393026303)) ;
#176436=CARTESIAN_POINT('Ctrl Pts',(-27.1286603816229,-12.9578227208983,
113.88696206551)) ;
#176437=CARTESIAN_POINT('Ctrl Pts',(-27.0548565317877,-12.9578226823066,
113.911193087656)) ;
#176438=CARTESIAN_POINT('Ctrl Pts',(-26.9810526819526,-12.9578226437149,
113.935424109803)) ;
#176439=CARTESIAN_POINT('Ctrl Pts',(-27.002206448563,-12.9237175210368,
113.999855070596)) ;
#176440=CARTESIAN_POINT('Ctrl Pts',(-27.0233602151733,-12.8896123983586,
114.064286031389)) ;
#176441=CARTESIAN_POINT('Ctrl Pts',(-27.0971640650084,-12.8896124369503,
114.040055009243)) ;
#176442=CARTESIAN_POINT('Ctrl Pts',(-27.1709679148435,-12.889612475542,
114.015823987097)) ;
#176443=CARTESIAN_POINT('Ctrl Pts',(-27.1498141482332,-12.9237175982201,
113.951393026303)) ;
#176444=CARTESIAN_POINT('Ctrl Pts',(-27.0872605509044,-12.6833926232874,
113.796490915852)) ;
#176445=CARTESIAN_POINT('Ctrl Pts',(-27.069705007748,-12.7343299181759,
113.743019563325)) ;
#176446=CARTESIAN_POINT('Ctrl Pts',(-26.9959011570845,-12.7343298939571,
113.767250582949)) ;
#176447=CARTESIAN_POINT('Ctrl Pts',(-26.9220973064211,-12.7343298697383,
113.791481602572)) ;
#176448=CARTESIAN_POINT('Ctrl Pts',(-26.9396528495775,-12.6833925748499,
113.844952955098)) ;
#176449=CARTESIAN_POINT('Ctrl Pts',(-26.9572083927339,-12.6324552799614,
113.898424307625)) ;
#176450=CARTESIAN_POINT('Ctrl Pts',(-27.0310122433973,-12.6324553041802,
113.874193288001)) ;
#176451=CARTESIAN_POINT('Ctrl Pts',(-27.1048160940608,-12.632455328399,
113.849962268378)) ;
#176452=CARTESIAN_POINT('Ctrl Pts',(-27.0872605509044,-12.6833926232874,
113.796490915852)) ;
#176453=CARTESIAN_POINT('Ctrl Pts',(-27.0073325603644,-12.4975233316372,
113.588365552072)) ;
#176454=CARTESIAN_POINT('Ctrl Pts',(-26.994600389807,-12.5615155230103,
113.549585414369)) ;
#176455=CARTESIAN_POINT('Ctrl Pts',(-26.9207965392856,-12.5615155094136,
113.573816434425)) ;
#176456=CARTESIAN_POINT('Ctrl Pts',(-26.8469926887642,-12.561515495817,
113.598047454481)) ;
#176457=CARTESIAN_POINT('Ctrl Pts',(-26.8597248593216,-12.4975233044439,
113.636827592184)) ;
#176458=CARTESIAN_POINT('Ctrl Pts',(-26.872457029879,-12.4335311130708,
113.675607729887)) ;
#176459=CARTESIAN_POINT('Ctrl Pts',(-26.9462608804004,-12.4335311266674,
113.651376709831)) ;
#176460=CARTESIAN_POINT('Ctrl Pts',(-27.0200647309218,-12.433531140264,
113.627145689775)) ;
#176461=CARTESIAN_POINT('Ctrl Pts',(-27.0073325603644,-12.4975233316372,
113.588365552072)) ;
#176462=CARTESIAN_POINT('Ctrl Pts',(-26.9141377906141,-12.3765652756753,
113.339997758843)) ;
#176463=CARTESIAN_POINT('Ctrl Pts',(-26.907159197438,-12.4491001941253,
113.318742089663)) ;
#176464=CARTESIAN_POINT('Ctrl Pts',(-26.8333553484405,-12.44910018943,113.342973114361)) ;
#176465=CARTESIAN_POINT('Ctrl Pts',(-26.759551499443,-12.4491001847347,
113.367204139058)) ;
#176466=CARTESIAN_POINT('Ctrl Pts',(-26.7665300926192,-12.3765652662847,
113.388459808238)) ;
#176467=CARTESIAN_POINT('Ctrl Pts',(-26.7735086857953,-12.3040303478347,
113.409715477419)) ;
#176468=CARTESIAN_POINT('Ctrl Pts',(-26.8473125347928,-12.30403035253,113.385484452721)) ;
#176469=CARTESIAN_POINT('Ctrl Pts',(-26.9211163837903,-12.3040303572253,
113.361253428023)) ;
#176470=CARTESIAN_POINT('Ctrl Pts',(-26.9141377906141,-12.3765652756753,
113.339997758843)) ;
#176471=CARTESIAN_POINT('Ctrl Pts',(-26.8140599847601,-12.3303669115662,
113.070599618917)) ;
#176472=CARTESIAN_POINT('Ctrl Pts',(-26.8133257493235,-12.4062370893219,
113.068363256019)) ;
#176473=CARTESIAN_POINT('Ctrl Pts',(-26.7395219022542,-12.4062370896233,
113.09259428659)) ;
#176474=CARTESIAN_POINT('Ctrl Pts',(-26.6657180551848,-12.4062370899248,
113.11682531716)) ;
#176475=CARTESIAN_POINT('Ctrl Pts',(-26.6664522906214,-12.3303669121692,
113.119061680059)) ;
#176476=CARTESIAN_POINT('Ctrl Pts',(-26.6671865260579,-12.2544967344135,
113.121298042957)) ;
#176477=CARTESIAN_POINT('Ctrl Pts',(-26.7409903731273,-12.2544967341121,
113.097067012386)) ;
#176478=CARTESIAN_POINT('Ctrl Pts',(-26.8147942201966,-12.2544967338106,
113.072835981815)) ;
#176479=CARTESIAN_POINT('Ctrl Pts',(-26.8140599847601,-12.3303669115662,
113.070599618917)) ;
#176480=CARTESIAN_POINT('Ctrl Pts',(-26.7130188584353,-12.3620831181533,
112.798392930309)) ;
#176481=CARTESIAN_POINT('Ctrl Pts',(-26.7186032170259,-12.4358532268962,
112.815401985444)) ;
#176482=CARTESIAN_POINT('Ctrl Pts',(-26.6447993721143,-12.4358532286459,
112.839633022587)) ;
#176483=CARTESIAN_POINT('Ctrl Pts',(-26.5709955272026,-12.4358532303956,
112.863864059729)) ;
#176484=CARTESIAN_POINT('Ctrl Pts',(-26.565411168612,-12.3620831216526,
112.846855004594)) ;
#176485=CARTESIAN_POINT('Ctrl Pts',(-26.5598268100214,-12.2883130129096,
112.829845949458)) ;
#176486=CARTESIAN_POINT('Ctrl Pts',(-26.6336306549331,-12.28831301116,112.805614912316)) ;
#176487=CARTESIAN_POINT('Ctrl Pts',(-26.7074344998447,-12.2883130094103,
112.781383875173)) ;
#176488=CARTESIAN_POINT('Ctrl Pts',(-26.7130188584353,-12.3620831181533,
112.798392930309)) ;
#176489=CARTESIAN_POINT('Ctrl Pts',(-26.6179903821788,-12.4697592102098,
112.544455169899)) ;
#176490=CARTESIAN_POINT('Ctrl Pts',(-26.6294840061736,-12.536121336536,
112.579462894091)) ;
#176491=CARTESIAN_POINT('Ctrl Pts',(-26.5556801627136,-12.5361213369903,
112.603693935654)) ;
#176492=CARTESIAN_POINT('Ctrl Pts',(-26.4818763192536,-12.5361213374447,
112.627924977218)) ;
#176493=CARTESIAN_POINT('Ctrl Pts',(-26.4703826952588,-12.4697592111185,
112.592917253027)) ;
#176494=CARTESIAN_POINT('Ctrl Pts',(-26.458889071264,-12.4033970847922,
112.557909528835)) ;
#176495=CARTESIAN_POINT('Ctrl Pts',(-26.532692914724,-12.4033970843379,
112.533678487271)) ;
#176496=CARTESIAN_POINT('Ctrl Pts',(-26.6064967581841,-12.4033970838835,
112.509447445707)) ;
#176497=CARTESIAN_POINT('Ctrl Pts',(-26.6179903821788,-12.4697592102098,
112.544455169899)) ;
#176498=CARTESIAN_POINT('Ctrl Pts',(-26.5351639179177,-12.6447797711106,
112.32756700901)) ;
#176499=CARTESIAN_POINT('Ctrl Pts',(-26.5517258863331,-12.6990195583039,
112.378012092584)) ;
#176500=CARTESIAN_POINT('Ctrl Pts',(-26.4779220434683,-12.69901955683,112.40224313596)) ;
#176501=CARTESIAN_POINT('Ctrl Pts',(-26.4041182006034,-12.6990195553562,
112.426474179337)) ;
#176502=CARTESIAN_POINT('Ctrl Pts',(-26.3875562321881,-12.6447797681629,
112.376029095764)) ;
#176503=CARTESIAN_POINT('Ctrl Pts',(-26.3709942637727,-12.5905399809696,
112.325584012191)) ;
#176504=CARTESIAN_POINT('Ctrl Pts',(-26.4447981066375,-12.5905399824434,
112.301352968814)) ;
#176505=CARTESIAN_POINT('Ctrl Pts',(-26.5186019495023,-12.5905399839173,
112.277121925437)) ;
#176506=CARTESIAN_POINT('Ctrl Pts',(-26.5351639179177,-12.6447797711106,
112.32756700901)) ;
#176507=CARTESIAN_POINT('Ctrl Pts',(-26.4692769172657,-12.8750273852739,
112.162297586987)) ;
#176508=CARTESIAN_POINT('Ctrl Pts',(-26.4897314257756,-12.9132697898462,
112.224598719652)) ;
#176509=CARTESIAN_POINT('Ctrl Pts',(-26.4159275829037,-12.9132697868245,
112.248829763007)) ;
#176510=CARTESIAN_POINT('Ctrl Pts',(-26.3421237400317,-12.9132697838028,
112.273060806362)) ;
#176511=CARTESIAN_POINT('Ctrl Pts',(-26.3216692315218,-12.8750273792305,
112.210759673697)) ;
#176512=CARTESIAN_POINT('Ctrl Pts',(-26.3012147230119,-12.8367849746583,
112.148458541031)) ;
#176513=CARTESIAN_POINT('Ctrl Pts',(-26.3750185658839,-12.8367849776799,
112.124227497676)) ;
#176514=CARTESIAN_POINT('Ctrl Pts',(-26.4488224087558,-12.8367849807016,
112.099996454321)) ;
#176515=CARTESIAN_POINT('Ctrl Pts',(-26.4692769172657,-12.8750273852739,
112.162297586987)) ;
#176516=CARTESIAN_POINT('Ctrl Pts',(-26.4243077785298,-13.1453257818208,
112.060890975421)) ;
#176517=CARTESIAN_POINT('Ctrl Pts',(-26.4471967824451,-13.1647498113274,
112.13060718826)) ;
#176518=CARTESIAN_POINT('Ctrl Pts',(-26.3733929391465,-13.1647498092517,
112.154838230316)) ;
#176519=CARTESIAN_POINT('Ctrl Pts',(-26.2995890958478,-13.164749807176,
112.179069272371)) ;
#176520=CARTESIAN_POINT('Ctrl Pts',(-26.2767000919324,-13.1453257776693,
112.109353059532)) ;
#176521=CARTESIAN_POINT('Ctrl Pts',(-26.2538110880171,-13.1259017481627,
112.039636846693)) ;
#176522=CARTESIAN_POINT('Ctrl Pts',(-26.3276149313157,-13.1259017502384,
112.015405804637)) ;
#176523=CARTESIAN_POINT('Ctrl Pts',(-26.4014187746144,-13.1259017523141,
111.991174762582)) ;
#176524=CARTESIAN_POINT('Ctrl Pts',(-26.4243077785298,-13.1453257818208,
112.060890975421)) ;
#176525=CARTESIAN_POINT('Ctrl Pts',(-26.403013785645,-13.4336234546741,
112.031393920208)) ;
#176526=CARTESIAN_POINT('Ctrl Pts',(-26.4266913940733,-13.4329452228824,
112.103512095099)) ;
#176527=CARTESIAN_POINT('Ctrl Pts',(-26.3528875505435,-13.4329452235498,
112.127743136451)) ;
#176528=CARTESIAN_POINT('Ctrl Pts',(-26.2790837070136,-13.4329452242172,
112.151974177802)) ;
#176529=CARTESIAN_POINT('Ctrl Pts',(-26.2554060985854,-13.433623456009,
112.07985600291)) ;
#176530=CARTESIAN_POINT('Ctrl Pts',(-26.2317284901571,-13.4343016878008,
112.007737828018)) ;
#176531=CARTESIAN_POINT('Ctrl Pts',(-26.3055323336869,-13.4343016871333,
111.983506786667)) ;
#176532=CARTESIAN_POINT('Ctrl Pts',(-26.3793361772167,-13.4343016864659,
111.959275745316)) ;
#176533=CARTESIAN_POINT('Ctrl Pts',(-26.403013785645,-13.4336234546741,
112.031393920208)) ;
#176534=CARTESIAN_POINT('Ctrl Pts',(-26.4060165852795,-13.7229316022969,
112.076174503052)) ;
#176535=CARTESIAN_POINT('Ctrl Pts',(-26.4287818404388,-13.7020508739217,
112.145513796983)) ;
#176536=CARTESIAN_POINT('Ctrl Pts',(-26.3549779974329,-13.7020508801849,
112.16974483993)) ;
#176537=CARTESIAN_POINT('Ctrl Pts',(-26.281174154427,-13.7020508864481,
112.193975882877)) ;
#176538=CARTESIAN_POINT('Ctrl Pts',(-26.2584088992677,-13.7229316148234,
112.124636588946)) ;
#176539=CARTESIAN_POINT('Ctrl Pts',(-26.2356436441084,-13.7438123431986,
112.055297295015)) ;
#176540=CARTESIAN_POINT('Ctrl Pts',(-26.3094474871143,-13.7438123369354,
112.031066252067)) ;
#176541=CARTESIAN_POINT('Ctrl Pts',(-26.3832513301202,-13.7438123306722,
112.00683520912)) ;
#176542=CARTESIAN_POINT('Ctrl Pts',(-26.4060165852795,-13.7229316022969,
112.076174503052)) ;
#176543=CARTESIAN_POINT('Ctrl Pts',(-26.4323125416507,-13.9881204584926,
112.191610815065)) ;
#176544=CARTESIAN_POINT('Ctrl Pts',(-26.4525433595489,-13.948693047744,
112.253230621924)) ;
#176545=CARTESIAN_POINT('Ctrl Pts',(-26.3787395179286,-13.9486930580491,
112.277461669092)) ;
#176546=CARTESIAN_POINT('Ctrl Pts',(-26.3049356763083,-13.9486930683542,
112.301692716259)) ;
#176547=CARTESIAN_POINT('Ctrl Pts',(-26.2847048584101,-13.9881204791028,
112.2400729094)) ;
#176548=CARTESIAN_POINT('Ctrl Pts',(-26.2644740405119,-14.0275478898515,
112.17845310254)) ;
#176549=CARTESIAN_POINT('Ctrl Pts',(-26.3382778821322,-14.0275478795464,
112.154222055372)) ;
#176550=CARTESIAN_POINT('Ctrl Pts',(-26.4120817237525,-14.0275478692412,
112.129991008205)) ;
#176551=CARTESIAN_POINT('Ctrl Pts',(-26.4323125416507,-13.9881204584926,
112.191610815065)) ;
#176552=CARTESIAN_POINT('Ctrl Pts',(-26.4792881537362,-14.2135626266573,
112.370156392619)) ;
#176553=CARTESIAN_POINT('Ctrl Pts',(-26.4955344715119,-14.1583369427659,
112.419640054866)) ;
#176554=CARTESIAN_POINT('Ctrl Pts',(-26.4217306322404,-14.1583369561378,
112.443871109188)) ;
#176555=CARTESIAN_POINT('Ctrl Pts',(-26.347926792969,-14.1583369695098,
112.468102163509)) ;
#176556=CARTESIAN_POINT('Ctrl Pts',(-26.3316804751934,-14.2135626534012,
112.418618501262)) ;
#176557=CARTESIAN_POINT('Ctrl Pts',(-26.3154341574177,-14.2687883372926,
112.369134839015)) ;
#176558=CARTESIAN_POINT('Ctrl Pts',(-26.3892379966892,-14.2687883239207,
112.344903784693)) ;
#176559=CARTESIAN_POINT('Ctrl Pts',(-26.4630418359606,-14.2687883105487,
112.320672730372)) ;
#176560=CARTESIAN_POINT('Ctrl Pts',(-26.4792881537362,-14.2135626266573,
112.370156392619)) ;
#176561=CARTESIAN_POINT('Ctrl Pts',(-26.5430286631922,-14.3820856851378,
112.599827193971)) ;
#176562=CARTESIAN_POINT('Ctrl Pts',(-26.5541128714066,-14.3150132250762,
112.633587903234)) ;
#176563=CARTESIAN_POINT('Ctrl Pts',(-26.4803090354461,-14.3150132383268,
112.65781896764)) ;
#176564=CARTESIAN_POINT('Ctrl Pts',(-26.4065051994856,-14.3150132515775,
112.682050032046)) ;
#176565=CARTESIAN_POINT('Ctrl Pts',(-26.3954209912713,-14.3820857116392,
112.648289322784)) ;
#176566=CARTESIAN_POINT('Ctrl Pts',(-26.3843367830569,-14.4491581717009,
112.614528613521)) ;
#176567=CARTESIAN_POINT('Ctrl Pts',(-26.4581406190174,-14.4491581584502,
112.590297549115)) ;
#176568=CARTESIAN_POINT('Ctrl Pts',(-26.5319444549779,-14.4491581451995,
112.566066484708)) ;
#176569=CARTESIAN_POINT('Ctrl Pts',(-26.5430286631922,-14.3820856851378,
112.599827193971)) ;
#176570=CARTESIAN_POINT('Ctrl Pts',(-26.6176671822151,-14.4811007735871,
112.862516248575)) ;
#176571=CARTESIAN_POINT('Ctrl Pts',(-26.6228245412953,-14.4070183383993,
112.878224731527)) ;
#176572=CARTESIAN_POINT('Ctrl Pts',(-26.5490207083938,-14.4070183464706,
112.902455805251)) ;
#176573=CARTESIAN_POINT('Ctrl Pts',(-26.4752168754924,-14.4070183545419,
112.926686878974)) ;
#176574=CARTESIAN_POINT('Ctrl Pts',(-26.4700595164122,-14.4811007897297,
112.910978396022)) ;
#176575=CARTESIAN_POINT('Ctrl Pts',(-26.464902157332,-14.5551832249176,
112.89526991307)) ;
#176576=CARTESIAN_POINT('Ctrl Pts',(-26.5387059902335,-14.5551832168463,
112.871038839346)) ;
#176577=CARTESIAN_POINT('Ctrl Pts',(-26.6125098231349,-14.555183208775,
112.846807765623)) ;
#176578=CARTESIAN_POINT('Ctrl Pts',(-26.6176671822151,-14.4811007735871,
112.862516248575)) ;
#176579=CARTESIAN_POINT('Ctrl Pts',(-26.6978612990312,-14.5043853087956,
113.142314338476)) ;
#176580=CARTESIAN_POINT('Ctrl Pts',(-26.6966915575993,-14.4285698473868,
113.138751493961)) ;
#176581=CARTESIAN_POINT('Ctrl Pts',(-26.622887727907,-14.4285698457663,
113.16298257746)) ;
#176582=CARTESIAN_POINT('Ctrl Pts',(-26.5490838982148,-14.4285698441458,
113.187213660958)) ;
#176583=CARTESIAN_POINT('Ctrl Pts',(-26.5502536396466,-14.5043853055546,
113.190776505473)) ;
#176584=CARTESIAN_POINT('Ctrl Pts',(-26.5514233810785,-14.5802007669634,
113.194339349988)) ;
#176585=CARTESIAN_POINT('Ctrl Pts',(-26.6252272107708,-14.5802007685839,
113.17010826649)) ;
#176586=CARTESIAN_POINT('Ctrl Pts',(-26.6990310404631,-14.5802007702044,
113.145877182991)) ;
#176587=CARTESIAN_POINT('Ctrl Pts',(-26.6978612990312,-14.5043853087956,
113.142314338476)) ;
#176588=CARTESIAN_POINT('Ctrl Pts',(-26.7765022627845,-14.4497319209782,
113.417276345146)) ;
#176589=CARTESIAN_POINT('Ctrl Pts',(-26.769106971723,-14.3776228604659,
113.394751480785)) ;
#176590=CARTESIAN_POINT('Ctrl Pts',(-26.6953031438992,-14.3776228445383,
113.418982569975)) ;
#176591=CARTESIAN_POINT('Ctrl Pts',(-26.6214993160755,-14.3776228286107,
113.443213659164)) ;
#176592=CARTESIAN_POINT('Ctrl Pts',(-26.628894607137,-14.449731889123,113.465738523525)) ;
#176593=CARTESIAN_POINT('Ctrl Pts',(-26.6362898981985,-14.5218409496353,
113.488263387886)) ;
#176594=CARTESIAN_POINT('Ctrl Pts',(-26.7100937260223,-14.5218409655629,
113.464032298697)) ;
#176595=CARTESIAN_POINT('Ctrl Pts',(-26.7838975538461,-14.5218409814906,
113.439801209507)) ;
#176596=CARTESIAN_POINT('Ctrl Pts',(-26.7765022627845,-14.4497319209782,
113.417276345146)) ;
#176597=CARTESIAN_POINT('Ctrl Pts',(-26.8476800485963,-14.3208489038209,
113.669628788919)) ;
#176598=CARTESIAN_POINT('Ctrl Pts',(-26.83456878888,-14.25763373208,113.62969400612)) ;
#176599=CARTESIAN_POINT('Ctrl Pts',(-26.7607649616458,-14.2576336982123,
113.653925097105)) ;
#176600=CARTESIAN_POINT('Ctrl Pts',(-26.6869611344116,-14.2576336643446,
113.67815618809)) ;
#176601=CARTESIAN_POINT('Ctrl Pts',(-26.700072394128,-14.3208488360855,
113.718090970889)) ;
#176602=CARTESIAN_POINT('Ctrl Pts',(-26.7131836538443,-14.3840640078265,
113.758025753688)) ;
#176603=CARTESIAN_POINT('Ctrl Pts',(-26.7869874810785,-14.3840640416942,
113.733794662703)) ;
#176604=CARTESIAN_POINT('Ctrl Pts',(-26.8607913083127,-14.3840640755619,
113.709563571718)) ;
#176605=CARTESIAN_POINT('Ctrl Pts',(-26.8476800485963,-14.3208489038209,
113.669628788919)) ;
#176606=CARTESIAN_POINT('Ctrl Pts',(-26.9051290746846,-14.1269083086763,
113.880141966721)) ;
#176607=CARTESIAN_POINT('Ctrl Pts',(-26.8872525909099,-14.0771420046429,
113.825693080136)) ;
#176608=CARTESIAN_POINT('Ctrl Pts',(-26.8134487620136,-14.0771419513953,
113.849924166059)) ;
#176609=CARTESIAN_POINT('Ctrl Pts',(-26.7396449331174,-14.0771418981477,
113.874155251982)) ;
#176610=CARTESIAN_POINT('Ctrl Pts',(-26.7575214168921,-14.1269082021811,
113.928604138566)) ;
#176611=CARTESIAN_POINT('Ctrl Pts',(-26.7753979006668,-14.1766745062146,
113.983053025151)) ;
#176612=CARTESIAN_POINT('Ctrl Pts',(-26.8492017295631,-14.1766745594622,
113.958821939228)) ;
#176613=CARTESIAN_POINT('Ctrl Pts',(-26.9230055584593,-14.1766746127098,
113.934590853305)) ;
#176614=CARTESIAN_POINT('Ctrl Pts',(-26.9051290746846,-14.1269083086763,
113.880141966721)) ;
#176615=CARTESIAN_POINT('Ctrl Pts',(-26.9439250946234,-13.8839530008224,
114.033597139485)) ;
#176616=CARTESIAN_POINT('Ctrl Pts',(-26.9225840143864,-13.8510774674815,
113.968595650967)) ;
#176617=CARTESIAN_POINT('Ctrl Pts',(-26.8487801814222,-13.8510773982051,
113.992826724499)) ;
#176618=CARTESIAN_POINT('Ctrl Pts',(-26.774976348458,-13.8510773289287,
114.017057798032)) ;
#176619=CARTESIAN_POINT('Ctrl Pts',(-26.7963174286951,-13.8839528622696,
114.08205928655)) ;
#176620=CARTESIAN_POINT('Ctrl Pts',(-26.8176585089322,-13.9168283956105,
114.147060775069)) ;
#176621=CARTESIAN_POINT('Ctrl Pts',(-26.8914623418963,-13.9168284648869,
114.122829701536)) ;
#176622=CARTESIAN_POINT('Ctrl Pts',(-26.9652661748605,-13.9168285341632,
114.098598628004)) ;
#176623=CARTESIAN_POINT('Ctrl Pts',(-26.9439250946234,-13.8839530008224,
114.033597139485)) ;
#176624=CARTESIAN_POINT('Ctrl Pts',(-26.9610011688202,-13.6058131007772,
114.121164169516)) ;
#176625=CARTESIAN_POINT('Ctrl Pts',(-26.9377011273381,-13.592308546656,
114.05019600097)) ;
#176626=CARTESIAN_POINT('Ctrl Pts',(-26.863897288672,-13.5923084632408,
114.074427057136)) ;
#176627=CARTESIAN_POINT('Ctrl Pts',(-26.790093450006,-13.5923083798256,
114.098658113301)) ;
#176628=CARTESIAN_POINT('Ctrl Pts',(-26.8133934914881,-13.6058129339469,
114.169626281847)) ;
#176629=CARTESIAN_POINT('Ctrl Pts',(-26.8366935329702,-13.6193174880682,
114.240594450393)) ;
#176630=CARTESIAN_POINT('Ctrl Pts',(-26.9104973716362,-13.6193175714834,
114.216363394227)) ;
#176631=CARTESIAN_POINT('Ctrl Pts',(-26.9843012103023,-13.6193176548985,
114.192132338062)) ;
#176632=CARTESIAN_POINT('Ctrl Pts',(-26.9610011688202,-13.6058131007772,
114.121164169516)) ;
#176633=CARTESIAN_POINT('Ctrl Pts',(-26.9541142012214,-13.3154623494247,
114.135571911121)) ;
#176634=CARTESIAN_POINT('Ctrl Pts',(-26.9305290130074,-13.3222095128514,
114.063735231526)) ;
#176635=CARTESIAN_POINT('Ctrl Pts',(-26.8567251670928,-13.3222094225439,
114.087966265613)) ;
#176636=CARTESIAN_POINT('Ctrl Pts',(-26.7829213211782,-13.3222093322365,
114.112197299701)) ;
#176637=CARTESIAN_POINT('Ctrl Pts',(-26.8065065093922,-13.3154621688099,
114.184033979296)) ;
#176638=CARTESIAN_POINT('Ctrl Pts',(-26.8300916976061,-13.3087150053832,
114.255870658891)) ;
#176639=CARTESIAN_POINT('Ctrl Pts',(-26.9038955435208,-13.3087150956907,
114.231639624804)) ;
#176640=CARTESIAN_POINT('Ctrl Pts',(-26.9776993894353,-13.3087151859981,
114.207408590716)) ;
#176641=CARTESIAN_POINT('Ctrl Pts',(-26.9541142012214,-13.3154623494247,
114.135571911121)) ;
#176642=CARTESIAN_POINT('Ctrl Pts',(-26.9227927789619,-13.0305252756843,
114.075814770893)) ;
#176643=CARTESIAN_POINT('Ctrl Pts',(-26.9006222531828,-13.057175468413,
114.008286924693)) ;
#176644=CARTESIAN_POINT('Ctrl Pts',(-26.8268183990987,-13.0571753774731,
114.032517933897)) ;
#176645=CARTESIAN_POINT('Ctrl Pts',(-26.7530145450145,-13.0571752865332,
114.056748943102)) ;
#176646=CARTESIAN_POINT('Ctrl Pts',(-26.7751850707936,-13.0305250938045,
114.124276789302)) ;
#176647=CARTESIAN_POINT('Ctrl Pts',(-26.7973555965728,-13.0038749010759,
114.191804635502)) ;
#176648=CARTESIAN_POINT('Ctrl Pts',(-26.8711594506569,-13.0038749920158,
114.167573626298)) ;
#176649=CARTESIAN_POINT('Ctrl Pts',(-26.944963304741,-13.0038750829557,
114.143342617093)) ;
#176650=CARTESIAN_POINT('Ctrl Pts',(-26.9227927789619,-13.0305252756843,
114.075814770893)) ;
#176651=CARTESIAN_POINT('Ctrl Pts',(-26.8691774398986,-12.7760411077928,
113.947787130553)) ;
#176652=CARTESIAN_POINT('Ctrl Pts',(-26.8499879959769,-12.8204973460342,
113.889339178628)) ;
#176653=CARTESIAN_POINT('Ctrl Pts',(-26.7761841340996,-12.8204972646132,
113.913570164095)) ;
#176654=CARTESIAN_POINT('Ctrl Pts',(-26.7023802722222,-12.8204971831922,
113.937801149563)) ;
#176655=CARTESIAN_POINT('Ctrl Pts',(-26.721569716144,-12.7760409449508,
113.996249101488)) ;
#176656=CARTESIAN_POINT('Ctrl Pts',(-26.7407591600657,-12.7315847067095,
114.054697053414)) ;
#176657=CARTESIAN_POINT('Ctrl Pts',(-26.814563021943,-12.7315847881305,
114.030466067947)) ;
#176658=CARTESIAN_POINT('Ctrl Pts',(-26.8883668838204,-12.7315848695515,
114.006235082479)) ;
#176659=CARTESIAN_POINT('Ctrl Pts',(-26.8691774398986,-12.7760411077928,
113.947787130553)) ;
#176660=CARTESIAN_POINT('Ctrl Pts',(-26.7957043233195,-12.5658693797106,
113.759493744326)) ;
#176661=CARTESIAN_POINT('Ctrl Pts',(-26.7808818986988,-12.6250641545161,
113.714347028503)) ;
#176662=CARTESIAN_POINT('Ctrl Pts',(-26.7070780298316,-12.6250640894152,
113.73857799268)) ;
#176663=CARTESIAN_POINT('Ctrl Pts',(-26.6332741609643,-12.6250640243143,
113.762808956858)) ;
#176664=CARTESIAN_POINT('Ctrl Pts',(-26.6480965855851,-12.5658692495088,
113.807955672681)) ;
#176665=CARTESIAN_POINT('Ctrl Pts',(-26.6629190102057,-12.5066744747032,
113.853102388504)) ;
#176666=CARTESIAN_POINT('Ctrl Pts',(-26.736722879073,-12.5066745398042,
113.828871424327)) ;
#176667=CARTESIAN_POINT('Ctrl Pts',(-26.8105267479402,-12.506674604905,
113.804640460149)) ;
#176668=CARTESIAN_POINT('Ctrl Pts',(-26.7957043233195,-12.5658693797106,
113.759493744326)) ;
#176669=CARTESIAN_POINT('Ctrl Pts',(-26.7071990036801,-12.4170609140262,
113.52535902764)) ;
#176670=CARTESIAN_POINT('Ctrl Pts',(-26.6978006274313,-12.4867319202062,
113.496733087944)) ;
#176671=CARTESIAN_POINT('Ctrl Pts',(-26.6239967533843,-12.4867318782286,
113.520964036345)) ;
#176672=CARTESIAN_POINT('Ctrl Pts',(-26.5501928793373,-12.4867318362511,
113.545194984746)) ;
#176673=CARTESIAN_POINT('Ctrl Pts',(-26.5595912555861,-12.4170608300712,
113.573820924441)) ;
#176674=CARTESIAN_POINT('Ctrl Pts',(-26.5689896318348,-12.3473898238912,
113.602446864137)) ;
#176675=CARTESIAN_POINT('Ctrl Pts',(-26.6427935058819,-12.3473898658687,
113.578215915736)) ;
#176676=CARTESIAN_POINT('Ctrl Pts',(-26.7165973799289,-12.3473899078463,
113.553984967335)) ;
#176677=CARTESIAN_POINT('Ctrl Pts',(-26.7071990036801,-12.4170609140262,
113.52535902764)) ;
#176678=CARTESIAN_POINT('Ctrl Pts',(-26.6088521342578,-12.3396249333132,
113.261367652909)) ;
#176679=CARTESIAN_POINT('Ctrl Pts',(-26.6055702780408,-12.4148052434578,
113.251371646305)) ;
#176680=CARTESIAN_POINT('Ctrl Pts',(-26.5317664011453,-12.4148052290128,
113.275602586029)) ;
#176681=CARTESIAN_POINT('Ctrl Pts',(-26.4579625242497,-12.4148052145678,
113.299833525754)) ;
#176682=CARTESIAN_POINT('Ctrl Pts',(-26.4612443804668,-12.3396249044232,
113.309829532358)) ;
#176683=CARTESIAN_POINT('Ctrl Pts',(-26.4645262366838,-12.2644445942785,
113.319825538963)) ;
#176684=CARTESIAN_POINT('Ctrl Pts',(-26.5383301135793,-12.2644446087235,
113.295594599239)) ;
#176685=CARTESIAN_POINT('Ctrl Pts',(-26.6121339904748,-12.2644446231686,
113.271363659514)) ;
#176686=CARTESIAN_POINT('Ctrl Pts',(-26.6088521342578,-12.3396249333132,
113.261367652909)) ;
#176687=CARTESIAN_POINT('Ctrl Pts',(-26.5073352253782,-12.340046412335,
112.987690769148)) ;
#176688=CARTESIAN_POINT('Ctrl Pts',(-26.5104009195119,-12.4153088432885,
112.997028376739)) ;
#176689=CARTESIAN_POINT('Ctrl Pts',(-26.4365970426382,-12.4153088579802,
113.02125931653)) ;
#176690=CARTESIAN_POINT('Ctrl Pts',(-26.3627931657646,-12.4153088726718,
113.045490256321)) ;
#176691=CARTESIAN_POINT('Ctrl Pts',(-26.3597274716308,-12.3400464417183,
113.03615264873)) ;
#176692=CARTESIAN_POINT('Ctrl Pts',(-26.3566617774971,-12.2647840107648,
113.02681504114)) ;
#176693=CARTESIAN_POINT('Ctrl Pts',(-26.4304656543708,-12.2647839960732,
113.002584101349)) ;
#176694=CARTESIAN_POINT('Ctrl Pts',(-26.5042695312444,-12.2647839813815,
112.978353161558)) ;
#176695=CARTESIAN_POINT('Ctrl Pts',(-26.5073352253782,-12.340046412335,
112.987690769148)) ;
#176696=CARTESIAN_POINT('Ctrl Pts',(-26.4097025231263,-12.4170460254182,
112.725620310096)) ;
#176697=CARTESIAN_POINT('Ctrl Pts',(-26.4188586939777,-12.4870438442232,
112.753508527089)) ;
#176698=CARTESIAN_POINT('Ctrl Pts',(-26.3450548197485,-12.487043886487,
112.777739474935)) ;
#176699=CARTESIAN_POINT('Ctrl Pts',(-26.2712509455193,-12.4870439287509,
112.801970422781)) ;
#176700=CARTESIAN_POINT('Ctrl Pts',(-26.2620947746679,-12.4170461099459,
112.774082205787)) ;
#176701=CARTESIAN_POINT('Ctrl Pts',(-26.2529386038164,-12.3470482911409,
112.746193988793)) ;
#176702=CARTESIAN_POINT('Ctrl Pts',(-26.3267424780456,-12.3470482488771,
112.721963040948)) ;
#176703=CARTESIAN_POINT('Ctrl Pts',(-26.4005463522748,-12.3470482066133,
112.697732093102)) ;
#176704=CARTESIAN_POINT('Ctrl Pts',(-26.4097025231263,-12.4170460254182,
112.725620310096)) ;
#176705=CARTESIAN_POINT('Ctrl Pts',(-26.3209819060534,-12.5662136094611,
112.490921752616)) ;
#176706=CARTESIAN_POINT('Ctrl Pts',(-26.3356107191864,-12.625901534808,
112.535478755034)) ;
#176707=CARTESIAN_POINT('Ctrl Pts',(-26.2618068501208,-12.6259016005162,
112.559709718608)) ;
#176708=CARTESIAN_POINT('Ctrl Pts',(-26.1880029810553,-12.6259016662244,
112.583940682181)) ;
#176709=CARTESIAN_POINT('Ctrl Pts',(-26.1733741679223,-12.5662137408776,
112.539383679763)) ;
#176710=CARTESIAN_POINT('Ctrl Pts',(-26.1587453547893,-12.5065258155307,
112.494826677344)) ;
#176711=CARTESIAN_POINT('Ctrl Pts',(-26.2325492238549,-12.5065257498225,
112.470595713771)) ;
#176712=CARTESIAN_POINT('Ctrl Pts',(-26.3063530929204,-12.5065256841143,
112.446364750198)) ;
#176713=CARTESIAN_POINT('Ctrl Pts',(-26.3209819060534,-12.5662136094611,
112.490921752616)) ;
#176714=CARTESIAN_POINT('Ctrl Pts',(-26.2476333327786,-12.7760199991739,
112.30293791623)) ;
#176715=CARTESIAN_POINT('Ctrl Pts',(-26.2666719877246,-12.8211489416697,
112.360926585345)) ;
#176716=CARTESIAN_POINT('Ctrl Pts',(-26.1928681256039,-12.8211490243987,
112.385157570071)) ;
#176717=CARTESIAN_POINT('Ctrl Pts',(-26.1190642634831,-12.8211491071278,
112.409388554798)) ;
#176718=CARTESIAN_POINT('Ctrl Pts',(-26.1000256085371,-12.776020164632,
112.351399885683)) ;
#176719=CARTESIAN_POINT('Ctrl Pts',(-26.0809869535911,-12.7308912221363,
112.293411216568)) ;
#176720=CARTESIAN_POINT('Ctrl Pts',(-26.1547908157119,-12.7308911394072,
112.269180231842)) ;
#176721=CARTESIAN_POINT('Ctrl Pts',(-26.2285946778326,-12.7308910566782,
112.244949247116)) ;
#176722=CARTESIAN_POINT('Ctrl Pts',(-26.2476333327786,-12.7760199991739,
112.30293791623)) ;
#176723=CARTESIAN_POINT('Ctrl Pts',(-26.1937928662736,-13.0322696653641,
112.174451982578)) ;
#176724=CARTESIAN_POINT('Ctrl Pts',(-26.2158844526486,-13.0595756323769,
112.241739388323)) ;
#176725=CARTESIAN_POINT('Ctrl Pts',(-26.1420805985489,-13.059575723918,
112.26597039748)) ;
#176726=CARTESIAN_POINT('Ctrl Pts',(-26.0682767444492,-13.0595758154591,
112.290201406637)) ;
#176727=CARTESIAN_POINT('Ctrl Pts',(-26.0461851580742,-13.0322698484462,
112.222914000892)) ;
#176728=CARTESIAN_POINT('Ctrl Pts',(-26.0240935716991,-13.0049638814334,
112.155626595147)) ;
#176729=CARTESIAN_POINT('Ctrl Pts',(-26.0978974257988,-13.0049637898923,
112.13139558599)) ;
#176730=CARTESIAN_POINT('Ctrl Pts',(-26.1717012798985,-13.0049636983512,
112.107164576833)) ;
#176731=CARTESIAN_POINT('Ctrl Pts',(-26.1937928662736,-13.0322696653641,
112.174451982578)) ;
#176732=CARTESIAN_POINT('Ctrl Pts',(-26.1627547455184,-13.3151090323585,
112.115281050215)) ;
#176733=CARTESIAN_POINT('Ctrl Pts',(-26.186314657556,-13.3227086607463,
112.187040739103)) ;
#176734=CARTESIAN_POINT('Ctrl Pts',(-26.1125108115818,-13.3227087535366,
112.211271773009)) ;
#176735=CARTESIAN_POINT('Ctrl Pts',(-26.0387069656076,-13.3227088463268,
112.235502806915)) ;
#176736=CARTESIAN_POINT('Ctrl Pts',(-26.0151470535699,-13.315109217939,
112.163743118026)) ;
#176737=CARTESIAN_POINT('Ctrl Pts',(-25.9915871415323,-13.3075095895512,
112.091983429138)) ;
#176738=CARTESIAN_POINT('Ctrl Pts',(-26.0653909875065,-13.307509496761,
112.067752395232)) ;
#176739=CARTESIAN_POINT('Ctrl Pts',(-26.1391948334808,-13.3075094039707,
112.043521361326)) ;
#176740=CARTESIAN_POINT('Ctrl Pts',(-26.1627547455184,-13.3151090323585,
112.115281050215)) ;
#176741=CARTESIAN_POINT('Ctrl Pts',(-26.1558631196965,-13.6075492018493,
112.129940953347)) ;
#176742=CARTESIAN_POINT('Ctrl Pts',(-26.1792021826536,-13.5947427678056,
112.201027971714)) ;
#176743=CARTESIAN_POINT('Ctrl Pts',(-26.1053983440989,-13.5947428521219,
112.225259028218)) ;
#176744=CARTESIAN_POINT('Ctrl Pts',(-26.0315945055442,-13.594742936438,
112.249490084723)) ;
#176745=CARTESIAN_POINT('Ctrl Pts',(-26.0082554425871,-13.6075493704817,
112.178403066356)) ;
#176746=CARTESIAN_POINT('Ctrl Pts',(-25.98491637963,-13.6203558045254,112.107316047989)) ;
#176747=CARTESIAN_POINT('Ctrl Pts',(-26.0587202181847,-13.6203557202092,
112.083084991485)) ;
#176748=CARTESIAN_POINT('Ctrl Pts',(-26.1325240567394,-13.620355635893,
112.05885393498)) ;
#176749=CARTESIAN_POINT('Ctrl Pts',(-26.1558631196965,-13.6075492018493,
112.129940953347)) ;
#176750=CARTESIAN_POINT('Ctrl Pts',(-26.1729300005076,-13.8839937911961,
112.217263774275)) ;
#176751=CARTESIAN_POINT('Ctrl Pts',(-26.1943813283139,-13.8518669319433,
112.282601056074)) ;
#176752=CARTESIAN_POINT('Ctrl Pts',(-26.1205774957318,-13.8518670036745,
112.30683213077)) ;
#176753=CARTESIAN_POINT('Ctrl Pts',(-26.0467736631496,-13.8518670754058,
112.331063205466)) ;
#176754=CARTESIAN_POINT('Ctrl Pts',(-26.0253223353433,-13.8839939346586,
112.265725923668)) ;
#176755=CARTESIAN_POINT('Ctrl Pts',(-26.003871007537,-13.9161207939113,
112.200388641869)) ;
#176756=CARTESIAN_POINT('Ctrl Pts',(-26.0776748401191,-13.9161207221801,
112.176157567173)) ;
#176757=CARTESIAN_POINT('Ctrl Pts',(-26.1514786727013,-13.9161206504489,
112.151926492477)) ;
#176758=CARTESIAN_POINT('Ctrl Pts',(-26.1729300005076,-13.8839937911961,
112.217263774275)) ;
#176759=CARTESIAN_POINT('Ctrl Pts',(-26.2120071941306,-14.1283418739825,
112.371799593747)) ;
#176760=CARTESIAN_POINT('Ctrl Pts',(-26.2300278122176,-14.0791061363548,
112.426687487438)) ;
#176761=CARTESIAN_POINT('Ctrl Pts',(-26.1562239835833,-14.079106190233,
112.450918574159)) ;
#176762=CARTESIAN_POINT('Ctrl Pts',(-26.082420154949,-14.0791062441112,
112.475149660879)) ;
#176763=CARTESIAN_POINT('Ctrl Pts',(-26.064399536862,-14.1283419817388,
112.420261767188)) ;
#176764=CARTESIAN_POINT('Ctrl Pts',(-26.046378918775,-14.1775777193664,
112.365373873497)) ;
#176765=CARTESIAN_POINT('Ctrl Pts',(-26.1201827474093,-14.1775776654883,
112.341142786777)) ;
#176766=CARTESIAN_POINT('Ctrl Pts',(-26.1939865760436,-14.1775776116101,
112.316911700056)) ;
#176767=CARTESIAN_POINT('Ctrl Pts',(-26.2120071941306,-14.1283418739825,
112.371799593747)) ;
#176768=CARTESIAN_POINT('Ctrl Pts',(-26.2693072989749,-14.321085337762,
112.58170002845)) ;
#176769=CARTESIAN_POINT('Ctrl Pts',(-26.2826224774496,-14.2583178356259,
112.622255912442)) ;
#176770=CARTESIAN_POINT('Ctrl Pts',(-26.2088186508594,-14.2583178709165,
112.646487005389)) ;
#176771=CARTESIAN_POINT('Ctrl Pts',(-26.1350148242692,-14.2583179062071,
112.670718098336)) ;
#176772=CARTESIAN_POINT('Ctrl Pts',(-26.1216996457945,-14.3210854083432,
112.630162214343)) ;
#176773=CARTESIAN_POINT('Ctrl Pts',(-26.1083844673198,-14.3838529104793,
112.589606330351)) ;
#176774=CARTESIAN_POINT('Ctrl Pts',(-26.18218829391,-14.3838528751887,112.565375237404)) ;
#176775=CARTESIAN_POINT('Ctrl Pts',(-26.2559921205002,-14.3838528398981,
112.541144144458)) ;
#176776=CARTESIAN_POINT('Ctrl Pts',(-26.2693072989749,-14.321085337762,
112.58170002845)) ;
#176777=CARTESIAN_POINT('Ctrl Pts',(-26.3405926471782,-14.4501544762085,
112.834435287317)) ;
#176778=CARTESIAN_POINT('Ctrl Pts',(-26.3482140059273,-14.3782797175252,
112.857648715311)) ;
#176779=CARTESIAN_POINT('Ctrl Pts',(-26.274410178748,-14.378279733915,112.881879806463)) ;
#176780=CARTESIAN_POINT('Ctrl Pts',(-26.2006063515687,-14.3782797503047,
112.906110897615)) ;
#176781=CARTESIAN_POINT('Ctrl Pts',(-26.1929849928196,-14.450154508988,
112.882897469621)) ;
#176782=CARTESIAN_POINT('Ctrl Pts',(-26.1853636340705,-14.5220292676713,
112.859684041627)) ;
#176783=CARTESIAN_POINT('Ctrl Pts',(-26.2591674612498,-14.5220292512815,
112.835452950475)) ;
#176784=CARTESIAN_POINT('Ctrl Pts',(-26.3329712884291,-14.5220292348918,
112.811221859322)) ;
#176785=CARTESIAN_POINT('Ctrl Pts',(-26.3405926471782,-14.4501544762085,
112.834435287317)) ;
#176786=CARTESIAN_POINT('Ctrl Pts',(-26.4193828840965,-14.504350239421,
113.109906480253)) ;
#176787=CARTESIAN_POINT('Ctrl Pts',(-26.4207801489466,-14.4285822954382,
113.114162322657)) ;
#176788=CARTESIAN_POINT('Ctrl Pts',(-26.346976319745,-14.4285822971821,
113.13839340765)) ;
#176789=CARTESIAN_POINT('Ctrl Pts',(-26.2731724905434,-14.4285822989259,
113.162624492643)) ;
#176790=CARTESIAN_POINT('Ctrl Pts',(-26.2717752256934,-14.5043502429086,
113.158368650239)) ;
#176791=CARTESIAN_POINT('Ctrl Pts',(-26.2703779608434,-14.5801181868914,
113.154112807834)) ;
#176792=CARTESIAN_POINT('Ctrl Pts',(-26.3441817900449,-14.5801181851475,
113.129881722841)) ;
#176793=CARTESIAN_POINT('Ctrl Pts',(-26.4179856192465,-14.5801181834037,
113.105650637849)) ;
#176794=CARTESIAN_POINT('Ctrl Pts',(-26.4193828840965,-14.504350239421,
113.109906480253)) ;
#176795=CARTESIAN_POINT('Ctrl Pts',(-26.4990873137165,-14.4811635345991,
113.387994186648)) ;
#176796=CARTESIAN_POINT('Ctrl Pts',(-26.4941906716139,-14.4069000332384,
113.373079804133)) ;
#176797=CARTESIAN_POINT('Ctrl Pts',(-26.4203868398276,-14.4069000243761,
113.397310881253)) ;
#176798=CARTESIAN_POINT('Ctrl Pts',(-26.3465830080412,-14.4069000155138,
113.421541958373)) ;
#176799=CARTESIAN_POINT('Ctrl Pts',(-26.3514796501438,-14.4811635168746,
113.436456340888)) ;
#176800=CARTESIAN_POINT('Ctrl Pts',(-26.3563762922464,-14.5554270182353,
113.451370723402)) ;
#176801=CARTESIAN_POINT('Ctrl Pts',(-26.4301801240328,-14.5554270270976,
113.427139646282)) ;
#176802=CARTESIAN_POINT('Ctrl Pts',(-26.5039839558191,-14.5554270359599,
113.402908569162)) ;
#176803=CARTESIAN_POINT('Ctrl Pts',(-26.4990873137165,-14.4811635345991,
113.387994186648)) ;
#176804=CARTESIAN_POINT('Ctrl Pts',(-26.5741035318335,-14.3816036851556,
113.652018746242)) ;
#176805=CARTESIAN_POINT('Ctrl Pts',(-26.5632261840353,-14.3141789361096,
113.61888809934)) ;
#176806=CARTESIAN_POINT('Ctrl Pts',(-26.4894223485548,-14.3141789218921,
113.643119165208)) ;
#176807=CARTESIAN_POINT('Ctrl Pts',(-26.4156185130744,-14.3141789076745,
113.667350231076)) ;
#176808=CARTESIAN_POINT('Ctrl Pts',(-26.4264958608725,-14.3816036567204,
113.700480877978)) ;
#176809=CARTESIAN_POINT('Ctrl Pts',(-26.4373732086707,-14.4490284057664,
113.73361152488)) ;
#176810=CARTESIAN_POINT('Ctrl Pts',(-26.5111770441512,-14.449028419984,
113.709380459012)) ;
#176811=CARTESIAN_POINT('Ctrl Pts',(-26.5849808796317,-14.4490284342016,
113.685149393144)) ;
#176812=CARTESIAN_POINT('Ctrl Pts',(-26.5741035318335,-14.3816036851556,
113.652018746242)) ;
#176813=CARTESIAN_POINT('Ctrl Pts',(-26.6376352371572,-14.2132115910195,
113.88096634118)) ;
#176814=CARTESIAN_POINT('Ctrl Pts',(-26.6215719998171,-14.1574425718006,
113.832040311625)) ;
#176815=CARTESIAN_POINT('Ctrl Pts',(-26.5477681610995,-14.1574425567691,
113.856271367634)) ;
#176816=CARTESIAN_POINT('Ctrl Pts',(-26.4739643223819,-14.1574425417376,
113.880502423642)) ;
#176817=CARTESIAN_POINT('Ctrl Pts',(-26.490027559722,-14.2132115609565,
113.929428453197)) ;
#176818=CARTESIAN_POINT('Ctrl Pts',(-26.5060907970621,-14.2689805801753,
113.978354482753)) ;
#176819=CARTESIAN_POINT('Ctrl Pts',(-26.5798946357797,-14.2689805952068,
113.954123426744)) ;
#176820=CARTESIAN_POINT('Ctrl Pts',(-26.6536984744973,-14.2689806102383,
113.929892370735)) ;
#176821=CARTESIAN_POINT('Ctrl Pts',(-26.6376352371572,-14.2132115910195,
113.88096634118)) ;
#176822=CARTESIAN_POINT('Ctrl Pts',(-26.6847308687247,-13.9871283531687,
114.059972839669)) ;
#176823=CARTESIAN_POINT('Ctrl Pts',(-26.6646189109287,-13.9470611393289,
113.998715061021)) ;
#176824=CARTESIAN_POINT('Ctrl Pts',(-26.5908150694804,-13.9470611278095,
114.022946108712)) ;
#176825=CARTESIAN_POINT('Ctrl Pts',(-26.5170112280321,-13.9470611162902,
114.047177156404)) ;
#176826=CARTESIAN_POINT('Ctrl Pts',(-26.5371231858281,-13.98712833013,114.108434935051)) ;
#176827=CARTESIAN_POINT('Ctrl Pts',(-26.5572351436241,-14.0271955439699,
114.169692713699)) ;
#176828=CARTESIAN_POINT('Ctrl Pts',(-26.6310389850724,-14.0271955554892,
114.145461666007)) ;
#176829=CARTESIAN_POINT('Ctrl Pts',(-26.7048428265207,-14.0271955670085,
114.121230618316)) ;
#176830=CARTESIAN_POINT('Ctrl Pts',(-26.6847308687247,-13.9871283531687,
114.059972839669)) ;
#176831=CARTESIAN_POINT('Ctrl Pts',(-26.7108828323385,-13.7209751384546,
114.175063486759)) ;
#176832=CARTESIAN_POINT('Ctrl Pts',(-26.6881811765791,-13.6994320003675,
114.105917906077)) ;
#176833=CARTESIAN_POINT('Ctrl Pts',(-26.6143773336532,-13.6994319934453,
114.130148949268)) ;
#176834=CARTESIAN_POINT('Ctrl Pts',(-26.5405734907274,-13.699431986523,
114.154379992459)) ;
#176835=CARTESIAN_POINT('Ctrl Pts',(-26.5632751464868,-13.72097512461,114.223525573141)) ;
#176836=CARTESIAN_POINT('Ctrl Pts',(-26.5859768022463,-13.7425182626971,
114.292671153823)) ;
#176837=CARTESIAN_POINT('Ctrl Pts',(-26.6597806451721,-13.7425182696194,
114.268440110632)) ;
#176838=CARTESIAN_POINT('Ctrl Pts',(-26.733584488098,-13.7425182765416,
114.244209067441)) ;
#176839=CARTESIAN_POINT('Ctrl Pts',(-26.7108828323385,-13.7209751384546,
114.175063486759)) ;
#176840=CARTESIAN_POINT('Ctrl Pts',(-26.7138425852466,-13.4341833204507,
114.21939759733)) ;
#176841=CARTESIAN_POINT('Ctrl Pts',(-26.6901693704343,-13.4326332891495,
114.14729280462)) ;
#176842=CARTESIAN_POINT('Ctrl Pts',(-26.6163655269116,-13.4326332865185,
114.171523845993)) ;
#176843=CARTESIAN_POINT('Ctrl Pts',(-26.5425616833888,-13.4326332838874,
114.195754887366)) ;
#176844=CARTESIAN_POINT('Ctrl Pts',(-26.566234898201,-13.4341833151887,
114.267859680076)) ;
#176845=CARTESIAN_POINT('Ctrl Pts',(-26.5899081130133,-13.4357333464899,
114.339964472785)) ;
#176846=CARTESIAN_POINT('Ctrl Pts',(-26.663711956536,-13.435733349121,114.315733431413)) ;
#176847=CARTESIAN_POINT('Ctrl Pts',(-26.7375158000588,-13.435733351752,
114.29150239004)) ;
#176848=CARTESIAN_POINT('Ctrl Pts',(-26.7138425852466,-13.4341833204507,
114.21939759733)) ;
#176849=CARTESIAN_POINT('Ctrl Pts',(-26.692396148443,-13.1440226446982,
114.18967350618)) ;
#176850=CARTESIAN_POINT('Ctrl Pts',(-26.6694482345518,-13.1627318776024,
114.119777863131)) ;
#176851=CARTESIAN_POINT('Ctrl Pts',(-26.5956443911823,-13.1627318792492,
114.14400890497)) ;
#176852=CARTESIAN_POINT('Ctrl Pts',(-26.5218405478128,-13.1627318808959,
114.16823994681)) ;
#176853=CARTESIAN_POINT('Ctrl Pts',(-26.544788461704,-13.1440226479917,
114.238135589859)) ;
#176854=CARTESIAN_POINT('Ctrl Pts',(-26.5677363755952,-13.1253134150875,
114.308031232908)) ;
#176855=CARTESIAN_POINT('Ctrl Pts',(-26.6415402189648,-13.1253134134407,
114.283800191069)) ;
#176856=CARTESIAN_POINT('Ctrl Pts',(-26.7153440623343,-13.125313411794,
114.259569149229)) ;
#176857=CARTESIAN_POINT('Ctrl Pts',(-26.692396148443,-13.1440226446982,
114.18967350618)) ;
#176858=CARTESIAN_POINT('Ctrl Pts',(-26.6475602009265,-12.8750223963181,
114.08850476367)) ;
#176859=CARTESIAN_POINT('Ctrl Pts',(-26.6269765050809,-12.9125432630704,
114.025810147355)) ;
#176860=CARTESIAN_POINT('Ctrl Pts',(-26.5531726621819,-12.9125432659671,
114.050041190628)) ;
#176861=CARTESIAN_POINT('Ctrl Pts',(-26.4793688192829,-12.9125432688638,
114.074272233901)) ;
#176862=CARTESIAN_POINT('Ctrl Pts',(-26.4999525151284,-12.8750224021116,
114.136966850215)) ;
#176863=CARTESIAN_POINT('Ctrl Pts',(-26.520536210974,-12.8375015353593,
114.19966146653)) ;
#176864=CARTESIAN_POINT('Ctrl Pts',(-26.594340053873,-12.8375015324626,
114.175430423257)) ;
#176865=CARTESIAN_POINT('Ctrl Pts',(-26.668143896772,-12.8375015295659,
114.151199379984)) ;
#176866=CARTESIAN_POINT('Ctrl Pts',(-26.6475602009265,-12.8750223963181,
114.08850476367)) ;
#176867=CARTESIAN_POINT('Ctrl Pts',(-26.5813161216274,-12.6437154561283,
113.922329063855)) ;
#176868=CARTESIAN_POINT('Ctrl Pts',(-26.5645911383237,-12.6974444198838,
113.87138746333)) ;
#176869=CARTESIAN_POINT('Ctrl Pts',(-26.4907872955394,-12.6974444216942,
113.895618506952)) ;
#176870=CARTESIAN_POINT('Ctrl Pts',(-26.4169834527552,-12.6974444235046,
113.919849550574)) ;
#176871=CARTESIAN_POINT('Ctrl Pts',(-26.4337084360588,-12.6437154597491,
113.970791151099)) ;
#176872=CARTESIAN_POINT('Ctrl Pts',(-26.4504334193625,-12.5899864959936,
114.021732751624)) ;
#176873=CARTESIAN_POINT('Ctrl Pts',(-26.5242372621468,-12.5899864941832,
113.997501708002)) ;
#176874=CARTESIAN_POINT('Ctrl Pts',(-26.598041104931,-12.5899864923728,
113.973270664379)) ;
#176875=CARTESIAN_POINT('Ctrl Pts',(-26.5813161216274,-12.6437154561283,
113.922329063855)) ;
#176876=CARTESIAN_POINT('Ctrl Pts',(-26.4986543480993,-12.4695015573388,
113.705836185377)) ;
#176877=CARTESIAN_POINT('Ctrl Pts',(-26.4869467016397,-12.5354737259947,
113.670176583294)) ;
#176878=CARTESIAN_POINT('Ctrl Pts',(-26.413142858443,-12.5354737260558,
113.69440762566)) ;
#176879=CARTESIAN_POINT('Ctrl Pts',(-26.3393390152463,-12.5354737261168,
113.718638668026)) ;
#176880=CARTESIAN_POINT('Ctrl Pts',(-26.3510466617059,-12.4695015574609,
113.754298270108)) ;
#176881=CARTESIAN_POINT('Ctrl Pts',(-26.3627543081655,-12.403529388805,
113.789957872191)) ;
#176882=CARTESIAN_POINT('Ctrl Pts',(-26.4365581513622,-12.403529388744,
113.765726829825)) ;
#176883=CARTESIAN_POINT('Ctrl Pts',(-26.5103619945589,-12.4035293886829,
113.741495787459)) ;
#176884=CARTESIAN_POINT('Ctrl Pts',(-26.4986543480993,-12.4695015573388,
113.705836185377)) ;
#176885=CARTESIAN_POINT('Ctrl Pts',(-26.40350334832,-12.3618253102505,113.451569423215)) ;
#176886=CARTESIAN_POINT('Ctrl Pts',(-26.3976869586198,-12.4354130130407,
113.433853638586)) ;
#176887=CARTESIAN_POINT('Ctrl Pts',(-26.323883114103,-12.4354130116483,
113.458084676931)) ;
#176888=CARTESIAN_POINT('Ctrl Pts',(-26.2500792695861,-12.4354130102558,
113.482315715276)) ;
#176889=CARTESIAN_POINT('Ctrl Pts',(-26.2558956592862,-12.3618253074657,
113.500031499905)) ;
#176890=CARTESIAN_POINT('Ctrl Pts',(-26.2617120489864,-12.2882376046756,
113.517747284534)) ;
#176891=CARTESIAN_POINT('Ctrl Pts',(-26.3355158935033,-12.288237606068,
113.493516246189)) ;
#176892=CARTESIAN_POINT('Ctrl Pts',(-26.4093197380202,-12.2882376074604,
113.469285207844)) ;
#176893=CARTESIAN_POINT('Ctrl Pts',(-26.40350334832,-12.3618253102505,113.451569423215)) ;
#176894=CARTESIAN_POINT('Ctrl Pts',(-26.3025135279916,-12.3304086987919,
113.179494242336)) ;
#176895=CARTESIAN_POINT('Ctrl Pts',(-26.3030051536482,-12.406297480682,
113.18099165457)) ;
#176896=CARTESIAN_POINT('Ctrl Pts',(-26.2292013071264,-12.4062974803833,
113.205222686808)) ;
#176897=CARTESIAN_POINT('Ctrl Pts',(-26.1553974606047,-12.4062974800845,
113.229453719047)) ;
#176898=CARTESIAN_POINT('Ctrl Pts',(-26.1549058349481,-12.3304086981944,
113.227956306813)) ;
#176899=CARTESIAN_POINT('Ctrl Pts',(-26.1544142092914,-12.2545199163043,
113.226458894579)) ;
#176900=CARTESIAN_POINT('Ctrl Pts',(-26.2282180558132,-12.2545199166031,
113.20222786234)) ;
#176901=CARTESIAN_POINT('Ctrl Pts',(-26.3020219023349,-12.2545199169019,
113.177996830102)) ;
#176902=CARTESIAN_POINT('Ctrl Pts',(-26.3025135279916,-12.3304086987919,
113.179494242336)) ;
#176903=CARTESIAN_POINT('Ctrl Pts',(-26.2025781370336,-12.3767667157857,
112.910488649315)) ;
#176904=CARTESIAN_POINT('Ctrl Pts',(-26.2093160933167,-12.4495286298161,
112.931011376676)) ;
#176905=CARTESIAN_POINT('Ctrl Pts',(-26.13551224504,-12.4495286339673,112.95524240357)) ;
#176906=CARTESIAN_POINT('Ctrl Pts',(-26.0617083967634,-12.4495286381184,
112.979473430463)) ;
#176907=CARTESIAN_POINT('Ctrl Pts',(-26.0549704404803,-12.376766724088,
112.958950703102)) ;
#176908=CARTESIAN_POINT('Ctrl Pts',(-26.0482324841972,-12.3040048100576,
112.938427975741)) ;
#176909=CARTESIAN_POINT('Ctrl Pts',(-26.1220363324738,-12.3040048059064,
112.914196948848)) ;
#176910=CARTESIAN_POINT('Ctrl Pts',(-26.1958401807505,-12.3040048017553,
112.889965921954)) ;
#176911=CARTESIAN_POINT('Ctrl Pts',(-26.2025781370336,-12.3767667157857,
112.910488649315)) ;
#176912=CARTESIAN_POINT('Ctrl Pts',(-26.1095364919782,-12.4973266925111,
112.662514220771)) ;
#176913=CARTESIAN_POINT('Ctrl Pts',(-26.1220476976156,-12.5617762145597,
112.700621334017)) ;
#176914=CARTESIAN_POINT('Ctrl Pts',(-26.048243847935,-12.5617762263117,
112.724852356634)) ;
#176915=CARTESIAN_POINT('Ctrl Pts',(-25.9744399982544,-12.5617762380637,
112.749083379251)) ;
#176916=CARTESIAN_POINT('Ctrl Pts',(-25.961928792617,-12.497326716015,112.710976266005)) ;
#176917=CARTESIAN_POINT('Ctrl Pts',(-25.9494175869796,-12.4328771939664,
112.672869152759)) ;
#176918=CARTESIAN_POINT('Ctrl Pts',(-26.0232214366602,-12.4328771822144,
112.648638130142)) ;
#176919=CARTESIAN_POINT('Ctrl Pts',(-26.0970252863408,-12.4328771704624,
112.624407107525)) ;
#176920=CARTESIAN_POINT('Ctrl Pts',(-26.1095364919782,-12.4973266925111,
112.662514220771)) ;
#176921=CARTESIAN_POINT('Ctrl Pts',(-26.0290482236216,-12.6849702880242,
112.452967860837)) ;
#176922=CARTESIAN_POINT('Ctrl Pts',(-26.0464605995771,-12.7364118506539,
112.506003147886)) ;
#176923=CARTESIAN_POINT('Ctrl Pts',(-25.9726567490838,-12.7364118743968,
112.530234168028)) ;
#176924=CARTESIAN_POINT('Ctrl Pts',(-25.8988528985905,-12.7364118981397,
112.55446518817)) ;
#176925=CARTESIAN_POINT('Ctrl Pts',(-25.881440522635,-12.68497033551,112.501429901121)) ;
#176926=CARTESIAN_POINT('Ctrl Pts',(-25.8640281466795,-12.6335287728803,
112.448394614072)) ;
#176927=CARTESIAN_POINT('Ctrl Pts',(-25.9378319971728,-12.6335287491374,
112.42416359393)) ;
#176928=CARTESIAN_POINT('Ctrl Pts',(-26.0116358476661,-12.6335287253945,
112.399932573788)) ;
#176929=CARTESIAN_POINT('Ctrl Pts',(-26.0290482236216,-12.6849702880242,
112.452967860837)) ;
#176930=CARTESIAN_POINT('Ctrl Pts',(-25.967020193737,-12.9239536141708,
112.299425204879)) ;
#176931=CARTESIAN_POINT('Ctrl Pts',(-25.9880562807875,-12.958783516276,
112.363497731089)) ;
#176932=CARTESIAN_POINT('Ctrl Pts',(-25.9142524314298,-12.9587835522301,
112.387728754689)) ;
#176933=CARTESIAN_POINT('Ctrl Pts',(-25.8404485820722,-12.9587835881843,
112.41195977829)) ;
#176934=CARTESIAN_POINT('Ctrl Pts',(-25.8194124950216,-12.9239536860792,
112.347887252081)) ;
#176935=CARTESIAN_POINT('Ctrl Pts',(-25.7983764079711,-12.889123783974,
112.283814725871)) ;
#176936=CARTESIAN_POINT('Ctrl Pts',(-25.8721802573288,-12.8891237480199,
112.25958370227)) ;
#176937=CARTESIAN_POINT('Ctrl Pts',(-25.9459841066864,-12.8891237120657,
112.23535267867)) ;
#176938=CARTESIAN_POINT('Ctrl Pts',(-25.967020193737,-12.9239536141708,
112.299425204879)) ;
#176939=CARTESIAN_POINT('Ctrl Pts',(-25.9264894675845,-13.198264514804,
112.211386234531)) ;
#176940=CARTESIAN_POINT('Ctrl Pts',(-25.949652990304,-13.2139924714054,
112.28193858637)) ;
#176941=CARTESIAN_POINT('Ctrl Pts',(-25.8758491435936,-13.2139925191053,
112.306169618033)) ;
#176942=CARTESIAN_POINT('Ctrl Pts',(-25.8020452968831,-13.2139925668051,
112.330400649697)) ;
#176943=CARTESIAN_POINT('Ctrl Pts',(-25.7788817741636,-13.1982646102037,
112.259848297858)) ;
#176944=CARTESIAN_POINT('Ctrl Pts',(-25.755718251444,-13.1825366536022,
112.189295946019)) ;
#176945=CARTESIAN_POINT('Ctrl Pts',(-25.8295220981545,-13.1825366059024,
112.165064914356)) ;
#176946=CARTESIAN_POINT('Ctrl Pts',(-25.9033259448649,-13.1825365582025,
112.140833882692)) ;
#176947=CARTESIAN_POINT('Ctrl Pts',(-25.9264894675845,-13.198264514804,
112.211386234531)) ;
#176948=CARTESIAN_POINT('Ctrl Pts',(-25.9096865137876,-13.4887696764051,
112.195672545383)) ;
#176949=CARTESIAN_POINT('Ctrl Pts',(-25.9333228151172,-13.4842376804655,
112.267664904418)) ;
#176950=CARTESIAN_POINT('Ctrl Pts',(-25.8595189726337,-13.4842377379434,
112.291895948956)) ;
#176951=CARTESIAN_POINT('Ctrl Pts',(-25.7857151301502,-13.4842377954214,
112.316126993494)) ;
#176952=CARTESIAN_POINT('Ctrl Pts',(-25.7620788288205,-13.488769791361,
112.244134634459)) ;
#176953=CARTESIAN_POINT('Ctrl Pts',(-25.7384425274908,-13.4933017873006,
112.172142275424)) ;
#176954=CARTESIAN_POINT('Ctrl Pts',(-25.8122463699744,-13.4933017298226,
112.147911230886)) ;
#176955=CARTESIAN_POINT('Ctrl Pts',(-25.8860502124579,-13.4933016723446,
112.123680186348)) ;
#176956=CARTESIAN_POINT('Ctrl Pts',(-25.9096865137876,-13.4887696764051,
112.195672545383)) ;
#176957=CARTESIAN_POINT('Ctrl Pts',(-25.9171975165263,-13.7747050880232,
112.254081199622)) ;
#176958=CARTESIAN_POINT('Ctrl Pts',(-25.9396084474025,-13.7502030722453,
112.322341277794)) ;
#176959=CARTESIAN_POINT('Ctrl Pts',(-25.8658046105853,-13.7502031353853,
112.346572339591)) ;
#176960=CARTESIAN_POINT('Ctrl Pts',(-25.7920007737681,-13.7502031985253,
112.370803401388)) ;
#176961=CARTESIAN_POINT('Ctrl Pts',(-25.7695898428919,-13.7747052143032,
112.302543323216)) ;
#176962=CARTESIAN_POINT('Ctrl Pts',(-25.7471789120157,-13.7992072300811,
112.234283245044)) ;
#176963=CARTESIAN_POINT('Ctrl Pts',(-25.8209827488329,-13.7992071669411,
112.210052183247)) ;
#176964=CARTESIAN_POINT('Ctrl Pts',(-25.89478658565,-13.7992071038011,112.18582112145)) ;
#176965=CARTESIAN_POINT('Ctrl Pts',(-25.9171975165263,-13.7747050880232,
112.254081199622)) ;
#176966=CARTESIAN_POINT('Ctrl Pts',(-25.9477017056163,-14.0346989777519,
112.382474254739)) ;
#176967=CARTESIAN_POINT('Ctrl Pts',(-25.9672811895643,-13.9920093582588,
112.442110202262)) ;
#176968=CARTESIAN_POINT('Ctrl Pts',(-25.8934773591914,-13.9920094202152,
112.466341283687)) ;
#176969=CARTESIAN_POINT('Ctrl Pts',(-25.8196735288186,-13.9920094821717,
112.490572365113)) ;
#176970=CARTESIAN_POINT('Ctrl Pts',(-25.8000940448706,-14.0346991016648,
112.430936417589)) ;
#176971=CARTESIAN_POINT('Ctrl Pts',(-25.7805145609227,-14.077388721158,
112.371300470066)) ;
#176972=CARTESIAN_POINT('Ctrl Pts',(-25.8543183912955,-14.0773886592015,
112.34706938864)) ;
#176973=CARTESIAN_POINT('Ctrl Pts',(-25.9281222216683,-14.077388597245,
112.322838307215)) ;
#176974=CARTESIAN_POINT('Ctrl Pts',(-25.9477017056163,-14.0346989777519,
112.382474254739)) ;
#176975=CARTESIAN_POINT('Ctrl Pts',(-25.9983172672415,-14.2504823475427,
112.572150154809)) ;
#176976=CARTESIAN_POINT('Ctrl Pts',(-26.0136566144146,-14.1926653559339,
112.618871329711)) ;
#176977=CARTESIAN_POINT('Ctrl Pts',(-25.9398527905619,-14.192665409366,
112.643102430996)) ;
#176978=CARTESIAN_POINT('Ctrl Pts',(-25.8660489667091,-14.1926654627981,
112.66733353228)) ;
#176979=CARTESIAN_POINT('Ctrl Pts',(-25.8507096195361,-14.2504824544068,
112.620612357378)) ;
#176980=CARTESIAN_POINT('Ctrl Pts',(-25.8353702723631,-14.3082994460156,
112.573891182476)) ;
#176981=CARTESIAN_POINT('Ctrl Pts',(-25.9091740962158,-14.3082993925835,
112.549660081192)) ;
#176982=CARTESIAN_POINT('Ctrl Pts',(-25.9829779200685,-14.3082993391515,
112.525428979907)) ;
#176983=CARTESIAN_POINT('Ctrl Pts',(-25.9983172672415,-14.2504823475427,
112.572150154809)) ;
#176984=CARTESIAN_POINT('Ctrl Pts',(-26.0642269575703,-14.4061007577842,
112.808231529626)) ;
#176985=CARTESIAN_POINT('Ctrl Pts',(-26.0742558502766,-14.3373352952271,
112.838777916951)) ;
#176986=CARTESIAN_POINT('Ctrl Pts',(-26.0004520317635,-14.3373353326338,
112.863009034499)) ;
#176987=CARTESIAN_POINT('Ctrl Pts',(-25.9266482132503,-14.3373353700405,
112.887240152047)) ;
#176988=CARTESIAN_POINT('Ctrl Pts',(-25.916619320544,-14.4061008325976,
112.856693764722)) ;
#176989=CARTESIAN_POINT('Ctrl Pts',(-25.9065904278376,-14.4748662951547,
112.826147377397)) ;
#176990=CARTESIAN_POINT('Ctrl Pts',(-25.9803942463508,-14.474866257748,
112.80191625985)) ;
#176991=CARTESIAN_POINT('Ctrl Pts',(-26.0541980648639,-14.4748662203413,
112.777685142302)) ;
#176992=CARTESIAN_POINT('Ctrl Pts',(-26.0642269575703,-14.4061007577842,
112.808231529626)) ;
#176993=CARTESIAN_POINT('Ctrl Pts',(-26.141044455505,-14.4917978275685,
113.07789332878)) ;
#176994=CARTESIAN_POINT('Ctrl Pts',(-26.144986537673,-14.4169485235802,
113.089900273168)) ;
#176995=CARTESIAN_POINT('Ctrl Pts',(-26.0711827236024,-14.4169485394119,
113.114131404247)) ;
#176996=CARTESIAN_POINT('Ctrl Pts',(-25.9973789095318,-14.4169485552436,
113.138362535326)) ;
#176997=CARTESIAN_POINT('Ctrl Pts',(-25.9934368273637,-14.4917978592319,
113.126355590938)) ;
#176998=CARTESIAN_POINT('Ctrl Pts',(-25.9894947451957,-14.5666471632202,
113.114348646551)) ;
#176999=CARTESIAN_POINT('Ctrl Pts',(-26.0632985592663,-14.5666471473885,
113.090117515472)) ;
#177000=CARTESIAN_POINT('Ctrl Pts',(-26.137102373337,-14.5666471315568,
113.065886384393)) ;
#177001=CARTESIAN_POINT('Ctrl Pts',(-26.141044455505,-14.4917978275685,
113.07789332878)) ;
#177002=CARTESIAN_POINT('Ctrl Pts',(-26.2209372515167,-14.4998539330622,
113.356520375798)) ;
#177003=CARTESIAN_POINT('Ctrl Pts',(-26.2185770638367,-14.4243333592347,
113.349331623022)) ;
#177004=CARTESIAN_POINT('Ctrl Pts',(-26.1447732512048,-14.4243333490761,
113.373562758484)) ;
#177005=CARTESIAN_POINT('Ctrl Pts',(-26.0709694385729,-14.4243333389175,
113.397793893945)) ;
#177006=CARTESIAN_POINT('Ctrl Pts',(-26.0733296262529,-14.4998539127449,
113.40498264672)) ;
#177007=CARTESIAN_POINT('Ctrl Pts',(-26.0756898139329,-14.5753744865724,
113.412171399495)) ;
#177008=CARTESIAN_POINT('Ctrl Pts',(-26.1494936265649,-14.575374496731,
113.387940264034)) ;
#177009=CARTESIAN_POINT('Ctrl Pts',(-26.2232974391968,-14.5753745068897,
113.363709128573)) ;
#177010=CARTESIAN_POINT('Ctrl Pts',(-26.2209372515167,-14.4998539330622,
113.356520375798)) ;
#177011=CARTESIAN_POINT('Ctrl Pts',(-26.2986502411454,-14.4309092256038,
113.628683576885)) ;
#177012=CARTESIAN_POINT('Ctrl Pts',(-26.2901272303962,-14.3600915226302,
113.602723859332)) ;
#177013=CARTESIAN_POINT('Ctrl Pts',(-26.2163234169747,-14.3600914852358,
113.626954992388)) ;
#177014=CARTESIAN_POINT('Ctrl Pts',(-26.1425196035533,-14.3600914478414,
113.651186125444)) ;
#177015=CARTESIAN_POINT('Ctrl Pts',(-26.1510426143025,-14.430909150815,
113.677145842998)) ;
#177016=CARTESIAN_POINT('Ctrl Pts',(-26.1595656250517,-14.5017268537886,
113.703105560551)) ;
#177017=CARTESIAN_POINT('Ctrl Pts',(-26.2333694384732,-14.501726891183,
113.678874427494)) ;
#177018=CARTESIAN_POINT('Ctrl Pts',(-26.3071732518947,-14.5017269285774,
113.654643294438)) ;
#177019=CARTESIAN_POINT('Ctrl Pts',(-26.2986502411454,-14.4309092256038,
113.628683576885)) ;
#177020=CARTESIAN_POINT('Ctrl Pts',(-26.3674757304941,-14.2894596882656,
113.873752815504)) ;
#177021=CARTESIAN_POINT('Ctrl Pts',(-26.3534018257283,-14.2284134835687,
113.830885970355)) ;
#177022=CARTESIAN_POINT('Ctrl Pts',(-26.2795980088395,-14.2284134202247,
113.85511709285)) ;
#177023=CARTESIAN_POINT('Ctrl Pts',(-26.2057941919506,-14.2284133568807,
113.879348215345)) ;
#177024=CARTESIAN_POINT('Ctrl Pts',(-26.2198680967164,-14.2894595615776,
113.922215060495)) ;
#177025=CARTESIAN_POINT('Ctrl Pts',(-26.2339420014822,-14.3505057662746,
113.965081905644)) ;
#177026=CARTESIAN_POINT('Ctrl Pts',(-26.307745818371,-14.3505058296186,
113.940850783149)) ;
#177027=CARTESIAN_POINT('Ctrl Pts',(-26.3815496352599,-14.3505058929625,
113.916619660653)) ;
#177028=CARTESIAN_POINT('Ctrl Pts',(-26.3674757304941,-14.2894596882656,
113.873752815504)) ;
#177029=CARTESIAN_POINT('Ctrl Pts',(-26.4219359703617,-14.0846391379262,
114.075220353395)) ;
#177030=CARTESIAN_POINT('Ctrl Pts',(-26.4033026567669,-14.0378023203219,
114.018466284573)) ;
#177031=CARTESIAN_POINT('Ctrl Pts',(-26.3294988340054,-14.0378022350358,
114.042697389181)) ;
#177032=CARTESIAN_POINT('Ctrl Pts',(-26.2556950112439,-14.0378021497496,
114.066928493789)) ;
#177033=CARTESIAN_POINT('Ctrl Pts',(-26.2743283248387,-14.0846389673539,
114.123682562611)) ;
#177034=CARTESIAN_POINT('Ctrl Pts',(-26.2929616384335,-14.1314757849582,
114.180436631434)) ;
#177035=CARTESIAN_POINT('Ctrl Pts',(-26.366765461195,-14.1314758702443,
114.156205526826)) ;
#177036=CARTESIAN_POINT('Ctrl Pts',(-26.4405692839565,-14.1314759555304,
114.131974422218)) ;
#177037=CARTESIAN_POINT('Ctrl Pts',(-26.4219359703617,-14.0846391379262,
114.075220353395)) ;
#177038=CARTESIAN_POINT('Ctrl Pts',(-26.4568504724485,-13.833584389583,
114.216907404291)) ;
#177039=CARTESIAN_POINT('Ctrl Pts',(-26.4350207703579,-13.8042063937381,
114.150417651839)) ;
#177040=CARTESIAN_POINT('Ctrl Pts',(-26.3612169398539,-13.8042062935713,
114.174648732864)) ;
#177041=CARTESIAN_POINT('Ctrl Pts',(-26.2874131093499,-13.8042061934045,
114.19887981389)) ;
#177042=CARTESIAN_POINT('Ctrl Pts',(-26.3092428114404,-13.8335841892493,
114.265369566343)) ;
#177043=CARTESIAN_POINT('Ctrl Pts',(-26.3310725135309,-13.8629621850941,
114.331859318795)) ;
#177044=CARTESIAN_POINT('Ctrl Pts',(-26.404876344035,-13.862962285261,114.30762823777)) ;
#177045=CARTESIAN_POINT('Ctrl Pts',(-26.478680174539,-13.8629623854278,
114.283397156744)) ;
#177046=CARTESIAN_POINT('Ctrl Pts',(-26.4568504724485,-13.833584389583,
114.216907404291)) ;
#177047=CARTESIAN_POINT('Ctrl Pts',(-26.469569796329,-13.5522887119168,
114.291086084856)) ;
#177048=CARTESIAN_POINT('Ctrl Pts',(-26.4460864891027,-13.5425061564868,
114.219559717974)) ;
#177049=CARTESIAN_POINT('Ctrl Pts',(-26.3722826498022,-13.542506049205,
114.243790772206)) ;
#177050=CARTESIAN_POINT('Ctrl Pts',(-26.2984788105016,-13.5425059419231,
114.268021826439)) ;
#177051=CARTESIAN_POINT('Ctrl Pts',(-26.3219621177278,-13.5522884973531,
114.339548193321)) ;
#177052=CARTESIAN_POINT('Ctrl Pts',(-26.345445424954,-13.5620710527831,
114.411074560204)) ;
#177053=CARTESIAN_POINT('Ctrl Pts',(-26.4192492642546,-13.5620711600649,
114.386843505971)) ;
#177054=CARTESIAN_POINT('Ctrl Pts',(-26.4930531035552,-13.5620712673468,
114.362612451738)) ;
#177055=CARTESIAN_POINT('Ctrl Pts',(-26.469569796329,-13.5522887119168,
114.291086084856)) ;
#177056=CARTESIAN_POINT('Ctrl Pts',(-26.4579117148728,-13.2592972529684,
114.291267191308)) ;
#177057=CARTESIAN_POINT('Ctrl Pts',(-26.4344686810137,-13.2699555383047,
114.219863490648)) ;
#177058=CARTESIAN_POINT('Ctrl Pts',(-26.3606648327152,-13.2699554336479,
114.244094517474)) ;
#177059=CARTESIAN_POINT('Ctrl Pts',(-26.2868609844167,-13.2699553289911,
114.268325544301)) ;
#177060=CARTESIAN_POINT('Ctrl Pts',(-26.3103040182758,-13.2592970436547,
114.339729244961)) ;
#177061=CARTESIAN_POINT('Ctrl Pts',(-26.3337470521349,-13.2486387583184,
114.411132945621)) ;
#177062=CARTESIAN_POINT('Ctrl Pts',(-26.4075509004334,-13.2486388629752,
114.386901918795)) ;
#177063=CARTESIAN_POINT('Ctrl Pts',(-26.4813547487319,-13.248638967632,
114.362670891968)) ;
#177064=CARTESIAN_POINT('Ctrl Pts',(-26.4579117148728,-13.2592972529684,
114.291267191308)) ;
#177065=CARTESIAN_POINT('Ctrl Pts',(-26.4225035557811,-12.9811038250668,
114.218671706621)) ;
#177066=CARTESIAN_POINT('Ctrl Pts',(-26.4007684106376,-13.0112007681919,
114.152469959464)) ;
#177067=CARTESIAN_POINT('Ctrl Pts',(-26.3269645541615,-13.0112006734562,
114.176700961383)) ;
#177068=CARTESIAN_POINT('Ctrl Pts',(-26.2531606976853,-13.0112005787204,
114.200931963302)) ;
#177069=CARTESIAN_POINT('Ctrl Pts',(-26.2748958428288,-12.9811036355953,
114.267133710458)) ;
#177070=CARTESIAN_POINT('Ctrl Pts',(-26.2966309879723,-12.9510066924703,
114.333335457615)) ;
#177071=CARTESIAN_POINT('Ctrl Pts',(-26.3704348444484,-12.951006787206,
114.309104455696)) ;
#177072=CARTESIAN_POINT('Ctrl Pts',(-26.4442387009246,-12.9510068819417,
114.284873453778)) ;
#177073=CARTESIAN_POINT('Ctrl Pts',(-26.4225035557811,-12.9811038250668,
114.218671706621)) ;
#177074=CARTESIAN_POINT('Ctrl Pts',(-26.3646027960108,-12.7319954339599,
114.077855142364)) ;
#177075=CARTESIAN_POINT('Ctrl Pts',(-26.3461421281083,-12.7795294847017,
114.021626924628)) ;
#177076=CARTESIAN_POINT('Ctrl Pts',(-26.2723382650299,-12.7795294077386,
114.045857906437)) ;
#177077=CARTESIAN_POINT('Ctrl Pts',(-26.1985344019515,-12.7795293307755,
114.070088888246)) ;
#177078=CARTESIAN_POINT('Ctrl Pts',(-26.2169950698539,-12.7319952800337,
114.126317105982)) ;
#177079=CARTESIAN_POINT('Ctrl Pts',(-26.2354557377563,-12.6844612292919,
114.182545323718)) ;
#177080=CARTESIAN_POINT('Ctrl Pts',(-26.3092596008348,-12.684461306255,
114.158314341908)) ;
#177081=CARTESIAN_POINT('Ctrl Pts',(-26.3830634639132,-12.6844613832181,
114.134083360099)) ;
#177082=CARTESIAN_POINT('Ctrl Pts',(-26.3646027960108,-12.7319954339599,
114.077855142364)) ;
#177083=CARTESIAN_POINT('Ctrl Pts',(-26.2880633731457,-12.5329045763516,
113.880121143368)) ;
#177084=CARTESIAN_POINT('Ctrl Pts',(-26.2741865157817,-12.5944099452727,
113.837854473023)) ;
#177085=CARTESIAN_POINT('Ctrl Pts',(-26.2003826481654,-12.5944098904592,
113.862085441011)) ;
#177086=CARTESIAN_POINT('Ctrl Pts',(-26.126578780549,-12.5944098356456,
113.886316408998)) ;
#177087=CARTESIAN_POINT('Ctrl Pts',(-26.140455637913,-12.5329044667245,
113.928583079342)) ;
#177088=CARTESIAN_POINT('Ctrl Pts',(-26.1543324952769,-12.4713990978033,
113.970849749687)) ;
#177089=CARTESIAN_POINT('Ctrl Pts',(-26.2281363628933,-12.4713991526168,
113.946618781699)) ;
#177090=CARTESIAN_POINT('Ctrl Pts',(-26.3019402305097,-12.4713992074304,
113.922387813712)) ;
#177091=CARTESIAN_POINT('Ctrl Pts',(-26.2880633731457,-12.5329045763516,
113.880121143368)) ;
#177092=CARTESIAN_POINT('Ctrl Pts',(-26.1969121836829,-12.3964115152595,
113.638084995048)) ;
#177093=CARTESIAN_POINT('Ctrl Pts',(-26.1886417973733,-12.467539433598,
113.612894731063)) ;
#177094=CARTESIAN_POINT('Ctrl Pts',(-26.1148379280184,-12.4675394037743,
113.637125693755)) ;
#177095=CARTESIAN_POINT('Ctrl Pts',(-26.0410340586634,-12.4675393739507,
113.661356656447)) ;
#177096=CARTESIAN_POINT('Ctrl Pts',(-26.049304444973,-12.3964114556122,
113.686546920432)) ;
#177097=CARTESIAN_POINT('Ctrl Pts',(-26.0575748312825,-12.3252835372738,
113.711737184416)) ;
#177098=CARTESIAN_POINT('Ctrl Pts',(-26.1313787006375,-12.3252835670974,
113.687506221724)) ;
#177099=CARTESIAN_POINT('Ctrl Pts',(-26.2051825699924,-12.3252835969211,
113.663275259032)) ;
#177100=CARTESIAN_POINT('Ctrl Pts',(-26.1969121836829,-12.3964115152595,
113.638084995048)) ;
#177101=CARTESIAN_POINT('Ctrl Pts',(-26.097882878132,-12.3338312624075,
113.371853705732)) ;
#177102=CARTESIAN_POINT('Ctrl Pts',(-26.0957817313739,-12.4094356003857,
113.365453950137)) ;
#177103=CARTESIAN_POINT('Ctrl Pts',(-26.0219778624167,-12.409435594184,
113.389684914041)) ;
#177104=CARTESIAN_POINT('Ctrl Pts',(-25.9481739934595,-12.4094355879822,
113.413915877944)) ;
#177105=CARTESIAN_POINT('Ctrl Pts',(-25.9502751402177,-12.333831250004,
113.420315633539)) ;
#177106=CARTESIAN_POINT('Ctrl Pts',(-25.9523762869759,-12.2582269120257,
113.426715389133)) ;
#177107=CARTESIAN_POINT('Ctrl Pts',(-26.026180155933,-12.2582269182275,
113.40248442523)) ;
#177108=CARTESIAN_POINT('Ctrl Pts',(-26.0999840248902,-12.2582269244292,
113.378253461326)) ;
#177109=CARTESIAN_POINT('Ctrl Pts',(-26.097882878132,-12.3338312624075,
113.371853705732)) ;
#177110=CARTESIAN_POINT('Ctrl Pts',(-25.9966525666846,-12.3486707517994,
113.098994699644)) ;
#177111=CARTESIAN_POINT('Ctrl Pts',(-26.0008820645952,-12.4233532981751,
113.111877066409)) ;
#177112=CARTESIAN_POINT('Ctrl Pts',(-25.9270781983048,-12.4233533125853,
113.136108038435)) ;
#177113=CARTESIAN_POINT('Ctrl Pts',(-25.8532743320144,-12.4233533269956,
113.160339010461)) ;
#177114=CARTESIAN_POINT('Ctrl Pts',(-25.8490448341037,-12.3486707806198,
113.147456643697)) ;
#177115=CARTESIAN_POINT('Ctrl Pts',(-25.8448153361931,-12.2739882342441,
113.134574276932)) ;
#177116=CARTESIAN_POINT('Ctrl Pts',(-25.9186192024836,-12.2739882198339,
113.110343304906)) ;
#177117=CARTESIAN_POINT('Ctrl Pts',(-25.992423068774,-12.2739882054237,
113.08611233288)) ;
#177118=CARTESIAN_POINT('Ctrl Pts',(-25.9966525666846,-12.3486707517994,
113.098994699644)) ;
#177119=CARTESIAN_POINT('Ctrl Pts',(-25.9000472227805,-12.4397941697449,
112.840152077552)) ;
#177120=CARTESIAN_POINT('Ctrl Pts',(-25.9102955213586,-12.5082273902753,
112.871366740162)) ;
#177121=CARTESIAN_POINT('Ctrl Pts',(-25.8364916591708,-12.5082274205257,
112.895597724684)) ;
#177122=CARTESIAN_POINT('Ctrl Pts',(-25.762687796983,-12.508227450776,112.919828709206)) ;
#177123=CARTESIAN_POINT('Ctrl Pts',(-25.7524394984049,-12.4397942302456,
112.888614046596)) ;
#177124=CARTESIAN_POINT('Ctrl Pts',(-25.7421911998268,-12.3713610097152,
112.857399383986)) ;
#177125=CARTESIAN_POINT('Ctrl Pts',(-25.8159950620145,-12.3713609794648,
112.833168399464)) ;
#177126=CARTESIAN_POINT('Ctrl Pts',(-25.8897989242023,-12.3713609492144,
112.808937414942)) ;
#177127=CARTESIAN_POINT('Ctrl Pts',(-25.9000472227805,-12.4397941697449,
112.840152077552)) ;
#177128=CARTESIAN_POINT('Ctrl Pts',(-25.8135929246481,-12.6021170084136,
112.612453782006)) ;
#177129=CARTESIAN_POINT('Ctrl Pts',(-25.8291558937232,-12.6593209317561,
112.659856073623)) ;
#177130=CARTESIAN_POINT('Ctrl Pts',(-25.7553520370272,-12.6593209703252,
112.684087074872)) ;
#177131=CARTESIAN_POINT('Ctrl Pts',(-25.6815481803312,-12.6593210088944,
112.708318076122)) ;
#177132=CARTESIAN_POINT('Ctrl Pts',(-25.665985211256,-12.6021170855519,
112.660915784504)) ;
#177133=CARTESIAN_POINT('Ctrl Pts',(-25.6504222421809,-12.5449131622094,
112.613513492887)) ;
#177134=CARTESIAN_POINT('Ctrl Pts',(-25.7242260988769,-12.5449131236403,
112.589282491638)) ;
#177135=CARTESIAN_POINT('Ctrl Pts',(-25.7980299555729,-12.5449130850712,
112.565051490389)) ;
#177136=CARTESIAN_POINT('Ctrl Pts',(-25.8135929246481,-12.6021170084136,
112.612453782006)) ;
#177137=CARTESIAN_POINT('Ctrl Pts',(-25.7439720862117,-12.8208593941247,
112.435659485376)) ;
#177138=CARTESIAN_POINT('Ctrl Pts',(-25.7636899177223,-12.862876765698,
112.495716817716)) ;
#177139=CARTESIAN_POINT('Ctrl Pts',(-25.6898860658087,-12.8628768085356,
112.519947833531)) ;
#177140=CARTESIAN_POINT('Ctrl Pts',(-25.6160822138952,-12.8628768513732,
112.544178849347)) ;
#177141=CARTESIAN_POINT('Ctrl Pts',(-25.5963643823846,-12.8208594798,112.484121517008)) ;
#177142=CARTESIAN_POINT('Ctrl Pts',(-25.576646550874,-12.7788421082267,
112.424064184669)) ;
#177143=CARTESIAN_POINT('Ctrl Pts',(-25.6504504027875,-12.7788420653891,
112.399833168853)) ;
#177144=CARTESIAN_POINT('Ctrl Pts',(-25.7242542547011,-12.7788420225515,
112.375602153037)) ;
#177145=CARTESIAN_POINT('Ctrl Pts',(-25.7439720862117,-12.8208593941247,
112.435659485376)) ;
#177146=CARTESIAN_POINT('Ctrl Pts',(-25.6940349138125,-13.084370773037,
112.319151955814)) ;
#177147=CARTESIAN_POINT('Ctrl Pts',(-25.7165329425454,-13.1080532494665,
112.387677320502)) ;
#177148=CARTESIAN_POINT('Ctrl Pts',(-25.6427290954994,-13.1080532886094,
112.411908351144)) ;
#177149=CARTESIAN_POINT('Ctrl Pts',(-25.5689252484535,-13.1080533277524,
112.436139381786)) ;
#177150=CARTESIAN_POINT('Ctrl Pts',(-25.5464272197206,-13.0843708513228,
112.367614017098)) ;
#177151=CARTESIAN_POINT('Ctrl Pts',(-25.5239291909878,-13.0606883748933,
112.29908865241)) ;
#177152=CARTESIAN_POINT('Ctrl Pts',(-25.5977330380337,-13.0606883357504,
112.274857621768)) ;
#177153=CARTESIAN_POINT('Ctrl Pts',(-25.6715368850796,-13.0606882966075,
112.250626591126)) ;
#177154=CARTESIAN_POINT('Ctrl Pts',(-25.6940349138125,-13.084370773037,
112.319151955814)) ;
#177155=CARTESIAN_POINT('Ctrl Pts',(-25.6675129647773,-13.3711928765175,
112.273852263887)) ;
#177156=CARTESIAN_POINT('Ctrl Pts',(-25.6911627416641,-13.3748845002412,
112.345885667787)) ;
#177157=CARTESIAN_POINT('Ctrl Pts',(-25.6173588980609,-13.3748845322642,
112.370116708915)) ;
#177158=CARTESIAN_POINT('Ctrl Pts',(-25.5435550544577,-13.3748845642871,
112.394347750043)) ;
#177159=CARTESIAN_POINT('Ctrl Pts',(-25.5199052775709,-13.3711929405634,
112.322314346143)) ;
#177160=CARTESIAN_POINT('Ctrl Pts',(-25.4962555006842,-13.3675013168397,
112.250280942242)) ;
#177161=CARTESIAN_POINT('Ctrl Pts',(-25.5700593442874,-13.3675012848167,
112.226049901115)) ;
#177162=CARTESIAN_POINT('Ctrl Pts',(-25.6438631878906,-13.3675012527938,
112.201818859987)) ;
#177163=CARTESIAN_POINT('Ctrl Pts',(-25.6675129647773,-13.3711928765175,
112.273852263887)) ;
#177164=CARTESIAN_POINT('Ctrl Pts',(-25.6652923171855,-13.6609866789311,
112.302537231817)) ;
#177165=CARTESIAN_POINT('Ctrl Pts',(-25.6883993942946,-13.644449399206,
112.372917659915)) ;
#177166=CARTESIAN_POINT('Ctrl Pts',(-25.6145955527509,-13.6444494224757,
112.397148707316)) ;
#177167=CARTESIAN_POINT('Ctrl Pts',(-25.5407917112072,-13.6444494457453,
112.421379754716)) ;
#177168=CARTESIAN_POINT('Ctrl Pts',(-25.5176846340981,-13.6609867254704,
112.350999326619)) ;
#177169=CARTESIAN_POINT('Ctrl Pts',(-25.494577556989,-13.6775240051955,
112.280618898521)) ;
#177170=CARTESIAN_POINT('Ctrl Pts',(-25.5683813985327,-13.6775239819258,
112.256387851121)) ;
#177171=CARTESIAN_POINT('Ctrl Pts',(-25.6421852400764,-13.6775239586562,
112.23215680372)) ;
#177172=CARTESIAN_POINT('Ctrl Pts',(-25.6652923171855,-13.6609866789311,
112.302537231817)) ;
#177173=CARTESIAN_POINT('Ctrl Pts',(-25.6865853284364,-13.9327616913683,
112.402736133509)) ;
#177174=CARTESIAN_POINT('Ctrl Pts',(-25.7075091126915,-13.8972231314794,
112.466466603975)) ;
#177175=CARTESIAN_POINT('Ctrl Pts',(-25.633705272027,-13.8972231463685,
112.490697654054)) ;
#177176=CARTESIAN_POINT('Ctrl Pts',(-25.5599014313626,-13.8972231612576,
112.514928704133)) ;
#177177=CARTESIAN_POINT('Ctrl Pts',(-25.5389776471075,-13.9327617211465,
112.451198233666)) ;
#177178=CARTESIAN_POINT('Ctrl Pts',(-25.5180538628524,-13.9683002810353,
112.3874677632)) ;
#177179=CARTESIAN_POINT('Ctrl Pts',(-25.5918577035168,-13.9683002661462,
112.363236713121)) ;
#177180=CARTESIAN_POINT('Ctrl Pts',(-25.6656615441813,-13.9683002512571,
112.339005663042)) ;
#177181=CARTESIAN_POINT('Ctrl Pts',(-25.6865853284364,-13.9327616913683,
112.402736133509)) ;
#177182=CARTESIAN_POINT('Ctrl Pts',(-25.7296598130416,-14.1696775509721,
112.569592493143)) ;
#177183=CARTESIAN_POINT('Ctrl Pts',(-25.7468696670354,-14.117542024341,
112.622010931435)) ;
#177184=CARTESIAN_POINT('Ctrl Pts',(-25.6730658257034,-14.1175420304562,
112.64624197948)) ;
#177185=CARTESIAN_POINT('Ctrl Pts',(-25.5992619843714,-14.1175420365713,
112.670473027526)) ;
#177186=CARTESIAN_POINT('Ctrl Pts',(-25.5820521303776,-14.1696775632024,
112.618054589234)) ;
#177187=CARTESIAN_POINT('Ctrl Pts',(-25.5648422763838,-14.2218130898334,
112.565636150943)) ;
#177188=CARTESIAN_POINT('Ctrl Pts',(-25.6386461177158,-14.2218130837183,
112.541405102897)) ;
#177189=CARTESIAN_POINT('Ctrl Pts',(-25.7124499590478,-14.2218130776032,
112.517174054852)) ;
#177190=CARTESIAN_POINT('Ctrl Pts',(-25.7296598130416,-14.1696775509721,
112.569592493143)) ;
#177191=CARTESIAN_POINT('Ctrl Pts',(-25.789817147401,-14.3505522399701,
112.788110084322)) ;
#177192=CARTESIAN_POINT('Ctrl Pts',(-25.802122003876,-14.2857090044566,
112.825588691676)) ;
#177193=CARTESIAN_POINT('Ctrl Pts',(-25.7283181617367,-14.2857090064648,
112.849819737262)) ;
#177194=CARTESIAN_POINT('Ctrl Pts',(-25.6545143195973,-14.285709008473,
112.874050782848)) ;
#177195=CARTESIAN_POINT('Ctrl Pts',(-25.6422094631223,-14.3505522439865,
112.836572175495)) ;
#177196=CARTESIAN_POINT('Ctrl Pts',(-25.6299046066472,-14.4153954795,112.799093568141)) ;
#177197=CARTESIAN_POINT('Ctrl Pts',(-25.7037084487866,-14.4153954774918,
112.774862522554)) ;
#177198=CARTESIAN_POINT('Ctrl Pts',(-25.7775122909259,-14.4153954754836,
112.750631476968)) ;
#177199=CARTESIAN_POINT('Ctrl Pts',(-25.789817147401,-14.3505522399701,
112.788110084322)) ;
#177200=CARTESIAN_POINT('Ctrl Pts',(-25.8627735208457,-14.4659895814683,
113.045823772028)) ;
#177201=CARTESIAN_POINT('Ctrl Pts',(-25.8692678377504,-14.39298831287,113.065604413469)) ;
#177202=CARTESIAN_POINT('Ctrl Pts',(-25.7954639943258,-14.392988312459,
113.089835455141)) ;
#177203=CARTESIAN_POINT('Ctrl Pts',(-25.7216601509012,-14.3929883120481,
113.114066496812)) ;
#177204=CARTESIAN_POINT('Ctrl Pts',(-25.7151658339964,-14.4659895806463,
113.094285855372)) ;
#177205=CARTESIAN_POINT('Ctrl Pts',(-25.7086715170917,-14.5389908492445,
113.074505213931)) ;
#177206=CARTESIAN_POINT('Ctrl Pts',(-25.7824753605163,-14.5389908496555,
113.050274172259)) ;
#177207=CARTESIAN_POINT('Ctrl Pts',(-25.8562792039409,-14.5389908500665,
113.026043130587)) ;
#177208=CARTESIAN_POINT('Ctrl Pts',(-25.8627735208457,-14.4659895814683,
113.045823772028)) ;
#177209=CARTESIAN_POINT('Ctrl Pts',(-25.9424652085819,-14.5060552317741,
113.324112272392)) ;
#177210=CARTESIAN_POINT('Ctrl Pts',(-25.9426684827821,-14.4301469447621,
113.324731412865)) ;
#177211=CARTESIAN_POINT('Ctrl Pts',(-25.8688646384337,-14.4301469446393,
113.348962451724)) ;
#177212=CARTESIAN_POINT('Ctrl Pts',(-25.7950607940854,-14.4301469445164,
113.373193490582)) ;
#177213=CARTESIAN_POINT('Ctrl Pts',(-25.7948575198852,-14.5060552315285,
113.372574350108)) ;
#177214=CARTESIAN_POINT('Ctrl Pts',(-25.7946542456851,-14.5819635185405,
113.371955209635)) ;
#177215=CARTESIAN_POINT('Ctrl Pts',(-25.8684580900334,-14.5819635186633,
113.347724170776)) ;
#177216=CARTESIAN_POINT('Ctrl Pts',(-25.9422619343817,-14.5819635187861,
113.323493131918)) ;
#177217=CARTESIAN_POINT('Ctrl Pts',(-25.9424652085819,-14.5060552317741,
113.324112272392)) ;
#177218=CARTESIAN_POINT('Ctrl Pts',(-26.0220030697392,-14.4677867862301,
113.601843781957)) ;
#177219=CARTESIAN_POINT('Ctrl Pts',(-26.0159183962998,-14.3944382757636,
113.58331084848)) ;
#177220=CARTESIAN_POINT('Ctrl Pts',(-25.9421145519418,-14.3944382766233,
113.607541887308)) ;
#177221=CARTESIAN_POINT('Ctrl Pts',(-25.8683107075837,-14.3944382774829,
113.631772926137)) ;
#177222=CARTESIAN_POINT('Ctrl Pts',(-25.874395381023,-14.4677867879495,
113.650305859614)) ;
#177223=CARTESIAN_POINT('Ctrl Pts',(-25.8804800544623,-14.541135298416,
113.668838793091)) ;
#177224=CARTESIAN_POINT('Ctrl Pts',(-25.9542838988204,-14.5411352975563,
113.644607754262)) ;
#177225=CARTESIAN_POINT('Ctrl Pts',(-26.0280877431785,-14.5411352966967,
113.620376715434)) ;
#177226=CARTESIAN_POINT('Ctrl Pts',(-26.0220030697392,-14.4677867862301,
113.601843781957)) ;
#177227=CARTESIAN_POINT('Ctrl Pts',(-26.094854630819,-14.3553856703914,
113.859024726864)) ;
#177228=CARTESIAN_POINT('Ctrl Pts',(-26.0829438233281,-14.2897781146532,
113.822746329087)) ;
#177229=CARTESIAN_POINT('Ctrl Pts',(-26.0091399794359,-14.2897781158864,
113.846977369334)) ;
#177230=CARTESIAN_POINT('Ctrl Pts',(-25.9353361355436,-14.2897781171196,
113.871208409582)) ;
#177231=CARTESIAN_POINT('Ctrl Pts',(-25.9472469430345,-14.3553856728579,
113.907486807359)) ;
#177232=CARTESIAN_POINT('Ctrl Pts',(-25.9591577505255,-14.4209932285961,
113.943765205137)) ;
#177233=CARTESIAN_POINT('Ctrl Pts',(-26.0329615944177,-14.4209932273629,
113.91953416489)) ;
#177234=CARTESIAN_POINT('Ctrl Pts',(-26.1067654383099,-14.4209932261297,
113.895303124642)) ;
#177235=CARTESIAN_POINT('Ctrl Pts',(-26.094854630819,-14.3553856703914,
113.859024726864)) ;
#177236=CARTESIAN_POINT('Ctrl Pts',(-26.1560900365016,-14.1738642018268,
114.081250316961)) ;
#177237=CARTESIAN_POINT('Ctrl Pts',(-26.1391465634837,-14.1208352191847,
114.029643231916)) ;
#177238=CARTESIAN_POINT('Ctrl Pts',(-26.0653427207382,-14.1208352175881,
114.053874275657)) ;
#177239=CARTESIAN_POINT('Ctrl Pts',(-25.9915388779928,-14.1208352159916,
114.078105319397)) ;
#177240=CARTESIAN_POINT('Ctrl Pts',(-26.0084823510107,-14.1738641986337,
114.129712404442)) ;
#177241=CARTESIAN_POINT('Ctrl Pts',(-26.0254258240287,-14.2268931812759,
114.181319489486)) ;
#177242=CARTESIAN_POINT('Ctrl Pts',(-26.0992296667742,-14.2268931828724,
114.157088445746)) ;
#177243=CARTESIAN_POINT('Ctrl Pts',(-26.1730335095196,-14.226893184469,
114.132857402005)) ;
#177244=CARTESIAN_POINT('Ctrl Pts',(-26.1560900365016,-14.1738642018268,
114.081250316961)) ;
#177245=CARTESIAN_POINT('Ctrl Pts',(-26.1991928753205,-13.9401973275635,
114.247846762684)) ;
#177246=CARTESIAN_POINT('Ctrl Pts',(-26.1784844305647,-13.9034069013251,
114.184772181116)) ;
#177247=CARTESIAN_POINT('Ctrl Pts',(-26.1046805883513,-13.9034068952956,
114.209003226477)) ;
#177248=CARTESIAN_POINT('Ctrl Pts',(-26.0308767461379,-13.903406889266,
114.233234271838)) ;
#177249=CARTESIAN_POINT('Ctrl Pts',(-26.0515851908937,-13.9401973155044,
114.296308853406)) ;
#177250=CARTESIAN_POINT('Ctrl Pts',(-26.0722936356495,-13.9769877417428,
114.359383434975)) ;
#177251=CARTESIAN_POINT('Ctrl Pts',(-26.1460974778628,-13.9769877477723,
114.335152389614)) ;
#177252=CARTESIAN_POINT('Ctrl Pts',(-26.2199013200762,-13.9769877538019,
114.310921344253)) ;
#177253=CARTESIAN_POINT('Ctrl Pts',(-26.1991928753205,-13.9401973275635,
114.247846762684)) ;
#177254=CARTESIAN_POINT('Ctrl Pts',(-26.2212325199795,-13.6684975496401,
114.35043177796)) ;
#177255=CARTESIAN_POINT('Ctrl Pts',(-26.1982213483443,-13.650624726406,
114.280343461741)) ;
#177256=CARTESIAN_POINT('Ctrl Pts',(-26.1244175060552,-13.6506247135771,
114.304574506871)) ;
#177257=CARTESIAN_POINT('Ctrl Pts',(-26.0506136637662,-13.6506247007482,
114.328805552001)) ;
#177258=CARTESIAN_POINT('Ctrl Pts',(-26.0736248354014,-13.6684975239824,
114.398893868221)) ;
#177259=CARTESIAN_POINT('Ctrl Pts',(-26.0966360070366,-13.6863703472165,
114.468982184441)) ;
#177260=CARTESIAN_POINT('Ctrl Pts',(-26.1704398493257,-13.6863703600454,
114.444751139311)) ;
#177261=CARTESIAN_POINT('Ctrl Pts',(-26.2442436916147,-13.6863703728742,
114.42052009418)) ;
#177262=CARTESIAN_POINT('Ctrl Pts',(-26.2212325199795,-13.6684975496401,
114.35043177796)) ;
#177263=CARTESIAN_POINT('Ctrl Pts',(-26.2196857700443,-13.3792258998284,
114.381117503958)) ;
#177264=CARTESIAN_POINT('Ctrl Pts',(-26.1960167906977,-13.3815248172849,
114.309025611457)) ;
#177265=CARTESIAN_POINT('Ctrl Pts',(-26.1222129473121,-13.3815247972218,
114.333256653248)) ;
#177266=CARTESIAN_POINT('Ctrl Pts',(-26.0484091039266,-13.3815247771587,
114.357487695039)) ;
#177267=CARTESIAN_POINT('Ctrl Pts',(-26.0720780832732,-13.3792258597022,
114.42957958754)) ;
#177268=CARTESIAN_POINT('Ctrl Pts',(-26.0957470626198,-13.3769269422458,
114.501671480041)) ;
#177269=CARTESIAN_POINT('Ctrl Pts',(-26.1695509060054,-13.3769269623089,
114.47744043825)) ;
#177270=CARTESIAN_POINT('Ctrl Pts',(-26.2433547493909,-13.3769269823719,
114.453209396459)) ;
#177271=CARTESIAN_POINT('Ctrl Pts',(-26.2196857700443,-13.3792258998284,
114.381117503958)) ;
#177272=CARTESIAN_POINT('Ctrl Pts',(-26.1935600200775,-13.0905267308239,
114.337229266664)) ;
#177273=CARTESIAN_POINT('Ctrl Pts',(-26.1709422477314,-13.1129867022683,
114.26833918088)) ;
#177274=CARTESIAN_POINT('Ctrl Pts',(-26.0971384017158,-13.1129866733618,
114.29257021466)) ;
#177275=CARTESIAN_POINT('Ctrl Pts',(-26.0233345557003,-13.1129866444553,
114.31680124844)) ;
#177276=CARTESIAN_POINT('Ctrl Pts',(-26.0459523280465,-13.0905266730108,
114.385691334224)) ;
#177277=CARTESIAN_POINT('Ctrl Pts',(-26.0685701003926,-13.0680667015663,
114.454581420009)) ;
#177278=CARTESIAN_POINT('Ctrl Pts',(-26.1423739464081,-13.0680667304729,
114.430350386228)) ;
#177279=CARTESIAN_POINT('Ctrl Pts',(-26.2161777924237,-13.0680667593794,
114.406119352448)) ;
#177280=CARTESIAN_POINT('Ctrl Pts',(-26.1935600200775,-13.0905267308239,
114.337229266664)) ;
#177281=CARTESIAN_POINT('Ctrl Pts',(-26.1446708799254,-12.8284630006125,
114.223586216955)) ;
#177282=CARTESIAN_POINT('Ctrl Pts',(-26.1247043042031,-12.8692525646979,
114.162771248191)) ;
#177283=CARTESIAN_POINT('Ctrl Pts',(-26.0509004547599,-12.869252533481,
114.187002271531)) ;
#177284=CARTESIAN_POINT('Ctrl Pts',(-25.9770966053167,-12.869252502264,
114.211233294871)) ;
#177285=CARTESIAN_POINT('Ctrl Pts',(-25.9970631810391,-12.8284629381786,
114.272048263635)) ;
#177286=CARTESIAN_POINT('Ctrl Pts',(-26.0170297567614,-12.7876733740933,
114.3328632324)) ;
#177287=CARTESIAN_POINT('Ctrl Pts',(-26.0908336062046,-12.7876734053102,
114.30863220906)) ;
#177288=CARTESIAN_POINT('Ctrl Pts',(-26.1646374556478,-12.7876734365271,
114.28440118572)) ;
#177289=CARTESIAN_POINT('Ctrl Pts',(-26.1446708799254,-12.8284630006125,
114.223586216955)) ;
#177290=CARTESIAN_POINT('Ctrl Pts',(-26.0750221134765,-12.6065365051644,
114.046995192604)) ;
#177291=CARTESIAN_POINT('Ctrl Pts',(-26.0591539020257,-12.6628800161341,
113.998663179958)) ;
#177292=CARTESIAN_POINT('Ctrl Pts',(-25.9853500480458,-12.6628799847594,
114.022894189481)) ;
#177293=CARTESIAN_POINT('Ctrl Pts',(-25.9115461940659,-12.6628799533848,
114.047125199003)) ;
#177294=CARTESIAN_POINT('Ctrl Pts',(-25.9274144055167,-12.6065364424151,
114.095457211648)) ;
#177295=CARTESIAN_POINT('Ctrl Pts',(-25.9432826169676,-12.5501929314454,
114.143789224293)) ;
#177296=CARTESIAN_POINT('Ctrl Pts',(-26.0170864709474,-12.5501929628201,
114.119558214771)) ;
#177297=CARTESIAN_POINT('Ctrl Pts',(-26.0908903249274,-12.5501929941947,
114.095327205249)) ;
#177298=CARTESIAN_POINT('Ctrl Pts',(-26.0750221134765,-12.6065365051644,
114.046995192604)) ;
#177299=CARTESIAN_POINT('Ctrl Pts',(-25.9893085808254,-12.4434900571409,
113.821371187434)) ;
#177300=CARTESIAN_POINT('Ctrl Pts',(-25.9786684347472,-12.5112986804866,
113.788963018204)) ;
#177301=CARTESIAN_POINT('Ctrl Pts',(-25.9048645761478,-12.5112986555149,
113.813194013656)) ;
#177302=CARTESIAN_POINT('Ctrl Pts',(-25.8310607175484,-12.5112986305432,
113.837425009108)) ;
#177303=CARTESIAN_POINT('Ctrl Pts',(-25.8417008636267,-12.4434900071976,
113.869833178338)) ;
#177304=CARTESIAN_POINT('Ctrl Pts',(-25.8523410097049,-12.3756813838519,
113.902241347569)) ;
#177305=CARTESIAN_POINT('Ctrl Pts',(-25.9261448683043,-12.3756814088236,
113.878010352117)) ;
#177306=CARTESIAN_POINT('Ctrl Pts',(-25.9999487269037,-12.3756814337953,
113.853779356665)) ;
#177307=CARTESIAN_POINT('Ctrl Pts',(-25.9893085808254,-12.4434900571409,
113.821371187434)) ;
#177308=CARTESIAN_POINT('Ctrl Pts',(-25.8927472268414,-12.3500508502058,
113.562734682547)) ;
#177309=CARTESIAN_POINT('Ctrl Pts',(-25.888099410984,-12.4244812912888,
113.548578184144)) ;
#177310=CARTESIAN_POINT('Ctrl Pts',(-25.8142955482319,-12.424481278477,
113.572809166948)) ;
#177311=CARTESIAN_POINT('Ctrl Pts',(-25.7404916854798,-12.4244812656651,
113.597040149751)) ;
#177312=CARTESIAN_POINT('Ctrl Pts',(-25.7451395013371,-12.3500508245822,
113.611196648154)) ;
#177313=CARTESIAN_POINT('Ctrl Pts',(-25.7497873171944,-12.2756203834992,
113.625353146556)) ;
#177314=CARTESIAN_POINT('Ctrl Pts',(-25.8235911799465,-12.275620396311,
113.601122163753)) ;
#177315=CARTESIAN_POINT('Ctrl Pts',(-25.8973950426987,-12.2756204091229,
113.57689118095)) ;
#177316=CARTESIAN_POINT('Ctrl Pts',(-25.8927472268414,-12.3500508502058,
113.562734682547)) ;
#177317=CARTESIAN_POINT('Ctrl Pts',(-25.7915387238206,-12.3331953888952,
113.289941672903)) ;
#177318=CARTESIAN_POINT('Ctrl Pts',(-25.7932163469713,-12.4089103805945,
113.295051440953)) ;
#177319=CARTESIAN_POINT('Ctrl Pts',(-25.7194124813001,-12.4089103853774,
113.319282414866)) ;
#177320=CARTESIAN_POINT('Ctrl Pts',(-25.6456086156289,-12.4089103901604,
113.343513388778)) ;
#177321=CARTESIAN_POINT('Ctrl Pts',(-25.6439309924783,-12.3331953984611,
113.338403620727)) ;
#177322=CARTESIAN_POINT('Ctrl Pts',(-25.6422533693277,-12.2574804067618,
113.333293852676)) ;
#177323=CARTESIAN_POINT('Ctrl Pts',(-25.7160572349988,-12.2574804019789,
113.309062878764)) ;
#177324=CARTESIAN_POINT('Ctrl Pts',(-25.78986110067,-12.2574803971959,113.284831904852)) ;
#177325=CARTESIAN_POINT('Ctrl Pts',(-25.7915387238206,-12.3331953888952,
113.289941672903)) ;
#177326=CARTESIAN_POINT('Ctrl Pts',(-25.6921668349445,-12.3940161187778,
113.022744551192)) ;
#177327=CARTESIAN_POINT('Ctrl Pts',(-25.7000507376626,-12.4655945537366,
113.046757645277)) ;
#177328=CARTESIAN_POINT('Ctrl Pts',(-25.626246870914,-12.4655945799172,
113.070988615907)) ;
#177329=CARTESIAN_POINT('Ctrl Pts',(-25.5524430041654,-12.4655946060978,
113.095219586538)) ;
#177330=CARTESIAN_POINT('Ctrl Pts',(-25.5445591014473,-12.3940161711391,
113.071206492453)) ;
#177331=CARTESIAN_POINT('Ctrl Pts',(-25.5366751987291,-12.3224377361804,
113.047193398368)) ;
#177332=CARTESIAN_POINT('Ctrl Pts',(-25.6104790654777,-12.3224377099997,
113.022962427738)) ;
#177333=CARTESIAN_POINT('Ctrl Pts',(-25.6842829322263,-12.3224376838191,
112.998731457107)) ;
#177334=CARTESIAN_POINT('Ctrl Pts',(-25.6921668349445,-12.3940161187778,
113.022744551192)) ;
#177335=CARTESIAN_POINT('Ctrl Pts',(-25.6010011665108,-12.5284976067023,
112.780567517695)) ;
#177336=CARTESIAN_POINT('Ctrl Pts',(-25.614526906004,-12.5907910171459,
112.821764736152)) ;
#177337=CARTESIAN_POINT('Ctrl Pts',(-25.5407230404825,-12.590791066487,
112.84599571052)) ;
#177338=CARTESIAN_POINT('Ctrl Pts',(-25.4669191749609,-12.5907911158281,
112.870226684888)) ;
#177339=CARTESIAN_POINT('Ctrl Pts',(-25.4533934354677,-12.5284977053845,
112.829029466431)) ;
#177340=CARTESIAN_POINT('Ctrl Pts',(-25.4398676959746,-12.466204294941,
112.787832247975)) ;
#177341=CARTESIAN_POINT('Ctrl Pts',(-25.5136715614961,-12.4662042455999,
112.763601273607)) ;
#177342=CARTESIAN_POINT('Ctrl Pts',(-25.5874754270177,-12.4662041962588,
112.739370299239)) ;
#177343=CARTESIAN_POINT('Ctrl Pts',(-25.6010011665108,-12.5284976067023,
112.780567517695)) ;
#177344=CARTESIAN_POINT('Ctrl Pts',(-25.5241403849889,-12.7253590046235,
112.581767024192)) ;
#177345=CARTESIAN_POINT('Ctrl Pts',(-25.5423213548809,-12.7739984449888,
112.637143323225)) ;
#177346=CARTESIAN_POINT('Ctrl Pts',(-25.4685174931494,-12.7739985153053,
112.661374309137)) ;
#177347=CARTESIAN_POINT('Ctrl Pts',(-25.3947136314178,-12.7739985856217,
112.685605295048)) ;
#177348=CARTESIAN_POINT('Ctrl Pts',(-25.3765326615258,-12.7253591452565,
112.630228996016)) ;
#177349=CARTESIAN_POINT('Ctrl Pts',(-25.3583516916337,-12.6767197048912,
112.574852696983)) ;
#177350=CARTESIAN_POINT('Ctrl Pts',(-25.4321555533653,-12.6767196345747,
112.550621711072)) ;
#177351=CARTESIAN_POINT('Ctrl Pts',(-25.5059594150968,-12.6767195642582,
112.52639072516)) ;
#177352=CARTESIAN_POINT('Ctrl Pts',(-25.5241403849889,-12.7253590046235,
112.581767024192)) ;
#177353=CARTESIAN_POINT('Ctrl Pts',(-25.4653269966594,-12.9750336085797,
112.438402703222)) ;
#177354=CARTESIAN_POINT('Ctrl Pts',(-25.4869006596714,-13.0063134744705,
112.504112597953)) ;
#177355=CARTESIAN_POINT('Ctrl Pts',(-25.4130968036294,-13.0063135643594,
112.528343601194)) ;
#177356=CARTESIAN_POINT('Ctrl Pts',(-25.3392929475873,-13.0063136542484,
112.552574604435)) ;
#177357=CARTESIAN_POINT('Ctrl Pts',(-25.3177192845753,-12.9750337883576,
112.486864709703)) ;
#177358=CARTESIAN_POINT('Ctrl Pts',(-25.2961456215632,-12.9437539224668,
112.421154814972)) ;
#177359=CARTESIAN_POINT('Ctrl Pts',(-25.3699494776053,-12.9437538325779,
112.396923811731)) ;
#177360=CARTESIAN_POINT('Ctrl Pts',(-25.4437533336474,-12.943753742689,
112.372692808491)) ;
#177361=CARTESIAN_POINT('Ctrl Pts',(-25.4653269966594,-12.9750336085797,
112.438402703222)) ;
#177362=CARTESIAN_POINT('Ctrl Pts',(-25.4295219032565,-13.2518773391213,
112.364484091442)) ;
#177363=CARTESIAN_POINT('Ctrl Pts',(-25.4528995946163,-13.2638740920304,
112.435688765391)) ;
#177364=CARTESIAN_POINT('Ctrl Pts',(-25.3790957463178,-13.2638741920649,
112.459919792217)) ;
#177365=CARTESIAN_POINT('Ctrl Pts',(-25.3052918980194,-13.2638742920995,
112.484150819044)) ;
#177366=CARTESIAN_POINT('Ctrl Pts',(-25.2819142066595,-13.2518775391904,
112.412946145095)) ;
#177367=CARTESIAN_POINT('Ctrl Pts',(-25.2585365152996,-13.2398807862813,
112.341741471146)) ;
#177368=CARTESIAN_POINT('Ctrl Pts',(-25.3323403635981,-13.2398806862467,
112.31751044432)) ;
#177369=CARTESIAN_POINT('Ctrl Pts',(-25.4061442118966,-13.2398805862122,
112.293279417493)) ;
#177370=CARTESIAN_POINT('Ctrl Pts',(-25.4295219032565,-13.2518773391213,
112.364484091442)) ;
#177371=CARTESIAN_POINT('Ctrl Pts',(-25.4172132742783,-13.5442043587849,
112.36261312341)) ;
#177372=CARTESIAN_POINT('Ctrl Pts',(-25.4407477286695,-13.5358098803519,
112.434295272181)) ;
#177373=CARTESIAN_POINT('Ctrl Pts',(-25.3669438889883,-13.5358099849276,
112.458526325254)) ;
#177374=CARTESIAN_POINT('Ctrl Pts',(-25.2931400493071,-13.5358100895033,
112.482757378328)) ;
#177375=CARTESIAN_POINT('Ctrl Pts',(-25.2696055949159,-13.5442045679364,
112.411075229557)) ;
#177376=CARTESIAN_POINT('Ctrl Pts',(-25.2460711405248,-13.5525990463694,
112.339393080786)) ;
#177377=CARTESIAN_POINT('Ctrl Pts',(-25.319874980206,-13.5525989417936,
112.315162027713)) ;
#177378=CARTESIAN_POINT('Ctrl Pts',(-25.3936788198872,-13.5525988372179,
112.290930974639)) ;
#177379=CARTESIAN_POINT('Ctrl Pts',(-25.4172132742783,-13.5442043587849,
112.36261312341)) ;
#177380=CARTESIAN_POINT('Ctrl Pts',(-25.4292212348024,-13.8259451748865,
112.434602285511)) ;
#177381=CARTESIAN_POINT('Ctrl Pts',(-25.4512191540056,-13.7978682383242,
112.50160439598)) ;
#177382=CARTESIAN_POINT('Ctrl Pts',(-25.37741532312,-13.7978683377893,112.525835475844)) ;
#177383=CARTESIAN_POINT('Ctrl Pts',(-25.3036114922345,-13.7978684372543,
112.550066555707)) ;
#177384=CARTESIAN_POINT('Ctrl Pts',(-25.2816135730313,-13.8259453738167,
112.483064445239)) ;
#177385=CARTESIAN_POINT('Ctrl Pts',(-25.2596156538282,-13.8540223103791,
112.41606233477)) ;
#177386=CARTESIAN_POINT('Ctrl Pts',(-25.3334194847137,-13.854022210914,
112.391831254906)) ;
#177387=CARTESIAN_POINT('Ctrl Pts',(-25.4072233155992,-13.8540221114489,
112.367600175042)) ;
#177388=CARTESIAN_POINT('Ctrl Pts',(-25.4292212348024,-13.8259451748865,
112.434602285511)) ;
#177389=CARTESIAN_POINT('Ctrl Pts',(-25.4637880029618,-14.0792480619856,
112.575412566812)) ;
#177390=CARTESIAN_POINT('Ctrl Pts',(-25.4826700787463,-14.0334450409061,
112.632924320946)) ;
#177391=CARTESIAN_POINT('Ctrl Pts',(-25.4088662558851,-14.0334451269848,
112.65715542525)) ;
#177392=CARTESIAN_POINT('Ctrl Pts',(-25.3350624330239,-14.0334452130635,
112.681386529554)) ;
#177393=CARTESIAN_POINT('Ctrl Pts',(-25.3161803572393,-14.079248234143,
112.623874775421)) ;
#177394=CARTESIAN_POINT('Ctrl Pts',(-25.2972982814547,-14.1250512552225,
112.566363021288)) ;
#177395=CARTESIAN_POINT('Ctrl Pts',(-25.371102104316,-14.1250511691438,
112.542131916984)) ;
#177396=CARTESIAN_POINT('Ctrl Pts',(-25.4449059271772,-14.1250510830651,
112.517900812679)) ;
#177397=CARTESIAN_POINT('Ctrl Pts',(-25.4637880029618,-14.0792480619856,
112.575412566812)) ;
#177398=CARTESIAN_POINT('Ctrl Pts',(-25.5175967023213,-14.2845087011992,
112.774736681666)) ;
#177399=CARTESIAN_POINT('Ctrl Pts',(-25.5320168624218,-14.2243072924303,
112.818658160557)) ;
#177400=CARTESIAN_POINT('Ctrl Pts',(-25.4582130459194,-14.2243073577872,
112.842889284229)) ;
#177401=CARTESIAN_POINT('Ctrl Pts',(-25.3844092294169,-14.2243074231441,
112.867120407901)) ;
#177402=CARTESIAN_POINT('Ctrl Pts',(-25.3699890693164,-14.284508831913,
112.823198929011)) ;
#177403=CARTESIAN_POINT('Ctrl Pts',(-25.3555689092159,-14.3447102406819,
112.77927745012)) ;
#177404=CARTESIAN_POINT('Ctrl Pts',(-25.4293727257183,-14.344710175325,
112.755046326448)) ;
#177405=CARTESIAN_POINT('Ctrl Pts',(-25.5031765422207,-14.3447101099681,
112.730815202776)) ;
#177406=CARTESIAN_POINT('Ctrl Pts',(-25.5175967023213,-14.2845087011992,
112.774736681666)) ;
#177407=CARTESIAN_POINT('Ctrl Pts',(-25.58604236121,-14.4278905637469,113.018639551001)) ;
#177408=CARTESIAN_POINT('Ctrl Pts',(-25.5949722174165,-14.3575893614837,
113.045838450109)) ;
#177409=CARTESIAN_POINT('Ctrl Pts',(-25.5211684050333,-14.3575894011323,
113.070069586328)) ;
#177410=CARTESIAN_POINT('Ctrl Pts',(-25.4473645926501,-14.3575894407809,
113.094300722547)) ;
#177411=CARTESIAN_POINT('Ctrl Pts',(-25.4384347364437,-14.4278906430441,
113.067101823439)) ;
#177412=CARTESIAN_POINT('Ctrl Pts',(-25.4295048802372,-14.4981918453073,
113.03990292433)) ;
#177413=CARTESIAN_POINT('Ctrl Pts',(-25.5033086926204,-14.4981918056587,
113.015671788111)) ;
#177414=CARTESIAN_POINT('Ctrl Pts',(-25.5771125050036,-14.4981917660102,
112.991440651893)) ;
#177415=CARTESIAN_POINT('Ctrl Pts',(-25.58604236121,-14.4278905637469,113.018639551001)) ;
#177416=CARTESIAN_POINT('Ctrl Pts',(-25.6636620375048,-14.49909499359,113.290546274635)) ;
#177417=CARTESIAN_POINT('Ctrl Pts',(-25.6664517281903,-14.4237176570017,
113.299043220325)) ;
#177418=CARTESIAN_POINT('Ctrl Pts',(-25.592647917231,-14.4237176684641,
113.323274360881)) ;
#177419=CARTESIAN_POINT('Ctrl Pts',(-25.5188441062716,-14.4237176799264,
113.347505501436)) ;
#177420=CARTESIAN_POINT('Ctrl Pts',(-25.5160544155862,-14.4990950165147,
113.339008555746)) ;
#177421=CARTESIAN_POINT('Ctrl Pts',(-25.5132647249008,-14.5744723531029,
113.330511610056)) ;
#177422=CARTESIAN_POINT('Ctrl Pts',(-25.5870685358601,-14.5744723416406,
113.3062804695)) ;
#177423=CARTESIAN_POINT('Ctrl Pts',(-25.6608723468194,-14.5744723301783,
113.282049328944)) ;
#177424=CARTESIAN_POINT('Ctrl Pts',(-25.6636620375048,-14.49909499359,113.290546274635)) ;
#177425=CARTESIAN_POINT('Ctrl Pts',(-25.7439225347513,-14.492829252027,
113.570454450893)) ;
#177426=CARTESIAN_POINT('Ctrl Pts',(-25.7403793642402,-14.4177767154629,
113.559662523248)) ;
#177427=CARTESIAN_POINT('Ctrl Pts',(-25.6665755520265,-14.4177766993577,
113.583893659982)) ;
#177428=CARTESIAN_POINT('Ctrl Pts',(-25.5927717398128,-14.4177766832525,
113.608124796717)) ;
#177429=CARTESIAN_POINT('Ctrl Pts',(-25.5963149103238,-14.4928292198167,
113.618916724363)) ;
#177430=CARTESIAN_POINT('Ctrl Pts',(-25.5998580808348,-14.5678817563809,
113.629708652009)) ;
#177431=CARTESIAN_POINT('Ctrl Pts',(-25.6736618930486,-14.567881772486,
113.605477515274)) ;
#177432=CARTESIAN_POINT('Ctrl Pts',(-25.7474657052623,-14.5678817885912,
113.581246378539)) ;
#177433=CARTESIAN_POINT('Ctrl Pts',(-25.7439225347513,-14.492829252027,
113.570454450893)) ;
#177434=CARTESIAN_POINT('Ctrl Pts',(-25.8206456678488,-14.4093444300335,
113.83969383373)) ;
#177435=CARTESIAN_POINT('Ctrl Pts',(-25.8110049285776,-14.3400077238797,
113.810329695576)) ;
#177436=CARTESIAN_POINT('Ctrl Pts',(-25.7372011124802,-14.3400076836513,
113.834560820481)) ;
#177437=CARTESIAN_POINT('Ctrl Pts',(-25.6633972963827,-14.340007643423,
113.858791945387)) ;
#177438=CARTESIAN_POINT('Ctrl Pts',(-25.6730380356538,-14.4093443495768,
113.888156083541)) ;
#177439=CARTESIAN_POINT('Ctrl Pts',(-25.6826787749249,-14.4786810557306,
113.917520221696)) ;
#177440=CARTESIAN_POINT('Ctrl Pts',(-25.7564825910224,-14.4786810959589,
113.89328909679)) ;
#177441=CARTESIAN_POINT('Ctrl Pts',(-25.8302864071199,-14.4786811361873,
113.869057971885)) ;
#177442=CARTESIAN_POINT('Ctrl Pts',(-25.8206456678488,-14.4093444300335,
113.83969383373)) ;
#177443=CARTESIAN_POINT('Ctrl Pts',(-25.8872186639727,-14.2544052422715,
114.077996994067)) ;
#177444=CARTESIAN_POINT('Ctrl Pts',(-25.872180153682,-14.1957815883073,
114.032192116431)) ;
#177445=CARTESIAN_POINT('Ctrl Pts',(-25.7983763318251,-14.1957815301846,
114.056423223795)) ;
#177446=CARTESIAN_POINT('Ctrl Pts',(-25.7245725099682,-14.1957814720619,
114.080654331158)) ;
#177447=CARTESIAN_POINT('Ctrl Pts',(-25.739611020259,-14.2544051260261,
114.126459208794)) ;
#177448=CARTESIAN_POINT('Ctrl Pts',(-25.7546495305497,-14.3130287799903,
114.17226408643)) ;
#177449=CARTESIAN_POINT('Ctrl Pts',(-25.8284533524066,-14.313028838113,
114.148032979066)) ;
#177450=CARTESIAN_POINT('Ctrl Pts',(-25.9022571742635,-14.3130288962357,
114.123801871703)) ;
#177451=CARTESIAN_POINT('Ctrl Pts',(-25.8872186639727,-14.2544052422715,
114.077996994067)) ;
#177452=CARTESIAN_POINT('Ctrl Pts',(-25.9379469965569,-14.0410991720381,
114.267799990034)) ;
#177453=CARTESIAN_POINT('Ctrl Pts',(-25.9186138483298,-13.9972803376337,
114.20891433828)) ;
#177454=CARTESIAN_POINT('Ctrl Pts',(-25.8448100199794,-13.9972802674836,
114.233145425866)) ;
#177455=CARTESIAN_POINT('Ctrl Pts',(-25.771006191629,-13.9972801973335,
114.257376513451)) ;
#177456=CARTESIAN_POINT('Ctrl Pts',(-25.790339339856,-14.0410990317379,
114.316262165205)) ;
#177457=CARTESIAN_POINT('Ctrl Pts',(-25.8096724880831,-14.0849178661423,
114.375147816958)) ;
#177458=CARTESIAN_POINT('Ctrl Pts',(-25.8834763164336,-14.0849179362924,
114.350916729373)) ;
#177459=CARTESIAN_POINT('Ctrl Pts',(-25.957280144784,-14.0849180064424,
114.326685641788)) ;
#177460=CARTESIAN_POINT('Ctrl Pts',(-25.9379469965569,-14.0410991720381,
114.267799990034)) ;
#177461=CARTESIAN_POINT('Ctrl Pts',(-25.9690716034183,-13.7816895970119,
114.398141043581)) ;
#177462=CARTESIAN_POINT('Ctrl Pts',(-25.9468006981219,-13.7559161217153,
114.330307457948)) ;
#177463=CARTESIAN_POINT('Ctrl Pts',(-25.872996862596,-13.7559160484501,
114.354538523678)) ;
#177464=CARTESIAN_POINT('Ctrl Pts',(-25.7991930270701,-13.7559159751849,
114.378769589408)) ;
#177465=CARTESIAN_POINT('Ctrl Pts',(-25.8214639323665,-13.7816894504815,
114.446603175041)) ;
#177466=CARTESIAN_POINT('Ctrl Pts',(-25.843734837663,-13.8074629257781,
114.514436760674)) ;
#177467=CARTESIAN_POINT('Ctrl Pts',(-25.9175386731889,-13.8074629990433,
114.490205694944)) ;
#177468=CARTESIAN_POINT('Ctrl Pts',(-25.9913425087147,-13.8074630723084,
114.465974629214)) ;
#177469=CARTESIAN_POINT('Ctrl Pts',(-25.9690716034183,-13.7816895970119,
114.398141043581)) ;
#177470=CARTESIAN_POINT('Ctrl Pts',(-25.977202611184,-13.4976199910735,
114.4582556851)) ;
#177471=CARTESIAN_POINT('Ctrl Pts',(-25.9535989487719,-13.4916413053213,
114.386362736462)) ;
#177472=CARTESIAN_POINT('Ctrl Pts',(-25.8797951067563,-13.4916412347082,
114.410593782425)) ;
#177473=CARTESIAN_POINT('Ctrl Pts',(-25.8059912647407,-13.4916411640951,
114.434824828388)) ;
#177474=CARTESIAN_POINT('Ctrl Pts',(-25.8295949271528,-13.4976198498473,
114.506717777026)) ;
#177475=CARTESIAN_POINT('Ctrl Pts',(-25.8531985895649,-13.5035985355994,
114.578610725664)) ;
#177476=CARTESIAN_POINT('Ctrl Pts',(-25.9270024315805,-13.5035986062125,
114.554379679701)) ;
#177477=CARTESIAN_POINT('Ctrl Pts',(-26.0008062735961,-13.5035986768257,
114.530148633738)) ;
#177478=CARTESIAN_POINT('Ctrl Pts',(-25.977202611184,-13.4976199910735,
114.4582556851)) ;
#177479=CARTESIAN_POINT('Ctrl Pts',(-25.9611123344456,-13.2063007087737,
114.444798177741)) ;
#177480=CARTESIAN_POINT('Ctrl Pts',(-25.9378606125945,-13.2206528794354,
114.37397718344)) ;
#177481=CARTESIAN_POINT('Ctrl Pts',(-25.864056765183,-13.2206528189828,
114.398208212968)) ;
#177482=CARTESIAN_POINT('Ctrl Pts',(-25.7902529177715,-13.2206527585302,
114.422439242497)) ;
#177483=CARTESIAN_POINT('Ctrl Pts',(-25.8135046396226,-13.2063005878686,
114.493260236797)) ;
#177484=CARTESIAN_POINT('Ctrl Pts',(-25.8367563614737,-13.1919484172069,
114.564081231098)) ;
#177485=CARTESIAN_POINT('Ctrl Pts',(-25.9105602088852,-13.1919484776594,
114.53985020157)) ;
#177486=CARTESIAN_POINT('Ctrl Pts',(-25.9843640562967,-13.191948538112,
114.515619172042)) ;
#177487=CARTESIAN_POINT('Ctrl Pts',(-25.9611123344456,-13.2063007087737,
114.444798177741)) ;
#177488=CARTESIAN_POINT('Ctrl Pts',(-25.9211552662506,-12.9308185504047,
114.358558160609)) ;
#177489=CARTESIAN_POINT('Ctrl Pts',(-25.8999242910296,-12.9644269321628,
114.293892034663)) ;
#177490=CARTESIAN_POINT('Ctrl Pts',(-25.8261204399611,-12.9644268849646,
114.318123053053)) ;
#177491=CARTESIAN_POINT('Ctrl Pts',(-25.7523165888926,-12.9644268377663,
114.342354071442)) ;
#177492=CARTESIAN_POINT('Ctrl Pts',(-25.7735475641136,-12.9308184560083,
114.407020197389)) ;
#177493=CARTESIAN_POINT('Ctrl Pts',(-25.7947785393346,-12.8972100742503,
114.471686323335)) ;
#177494=CARTESIAN_POINT('Ctrl Pts',(-25.8685823904031,-12.8972101214485,
114.447455304946)) ;
#177495=CARTESIAN_POINT('Ctrl Pts',(-25.9423862414716,-12.8972101686467,
114.423224286556)) ;
#177496=CARTESIAN_POINT('Ctrl Pts',(-25.9211552662506,-12.9308185504047,
114.358558160609)) ;
#177497=CARTESIAN_POINT('Ctrl Pts',(-25.8593713827175,-12.690040453889,
114.205882675566)) ;
#177498=CARTESIAN_POINT('Ctrl Pts',(-25.8416872490551,-12.7405114660654,
114.152019656903)) ;
#177499=CARTESIAN_POINT('Ctrl Pts',(-25.7678833962727,-12.7405114337976,
114.176250670072)) ;
#177500=CARTESIAN_POINT('Ctrl Pts',(-25.6940795434902,-12.7405114015298,
114.200481683241)) ;
#177501=CARTESIAN_POINT('Ctrl Pts',(-25.7117636771525,-12.6900403893535,
114.254344701904)) ;
#177502=CARTESIAN_POINT('Ctrl Pts',(-25.7294478108148,-12.6395693771771,
114.308207720567)) ;
#177503=CARTESIAN_POINT('Ctrl Pts',(-25.8032516635973,-12.6395694094449,
114.283976707398)) ;
#177504=CARTESIAN_POINT('Ctrl Pts',(-25.8770555163798,-12.6395694417127,
114.259745694229)) ;
#177505=CARTESIAN_POINT('Ctrl Pts',(-25.8593713827175,-12.690040453889,
114.205882675566)) ;
#177506=CARTESIAN_POINT('Ctrl Pts',(-25.7799037685495,-12.5021903792694,
113.999176989546)) ;
#177507=CARTESIAN_POINT('Ctrl Pts',(-25.7670102007119,-12.5658538076965,
113.959905261575)) ;
#177508=CARTESIAN_POINT('Ctrl Pts',(-25.6932063475663,-12.5658537885695,
113.984136273638)) ;
#177509=CARTESIAN_POINT('Ctrl Pts',(-25.6194024944207,-12.5658537694425,
114.008367285701)) ;
#177510=CARTESIAN_POINT('Ctrl Pts',(-25.6322960622582,-12.5021903410154,
114.047639013672)) ;
#177511=CARTESIAN_POINT('Ctrl Pts',(-25.6451896300958,-12.4385269125883,
114.086910741644)) ;
#177512=CARTESIAN_POINT('Ctrl Pts',(-25.7189934832414,-12.4385269317153,
114.06267972958)) ;
#177513=CARTESIAN_POINT('Ctrl Pts',(-25.792797336387,-12.4385269508424,
114.038448717517)) ;
#177514=CARTESIAN_POINT('Ctrl Pts',(-25.7799037685495,-12.5021903792694,
113.999176989546)) ;
#177515=CARTESIAN_POINT('Ctrl Pts',(-25.6868876116915,-12.3790435207342,
113.751397700364)) ;
#177516=CARTESIAN_POINT('Ctrl Pts',(-25.6797338653771,-12.4514021719633,
113.729608542811)) ;
#177517=CARTESIAN_POINT('Ctrl Pts',(-25.6059300136845,-12.4514021645019,
113.7538395593)) ;
#177518=CARTESIAN_POINT('Ctrl Pts',(-25.5321261619918,-12.4514021570405,
113.778070575788)) ;
#177519=CARTESIAN_POINT('Ctrl Pts',(-25.5392799083062,-12.3790435058114,
113.799859733342)) ;
#177520=CARTESIAN_POINT('Ctrl Pts',(-25.5464336546206,-12.3066848545823,
113.821648890895)) ;
#177521=CARTESIAN_POINT('Ctrl Pts',(-25.6202375063133,-12.3066848620437,
113.797417874406)) ;
#177522=CARTESIAN_POINT('Ctrl Pts',(-25.6940413580059,-12.3066848695051,
113.773186857918)) ;
#177523=CARTESIAN_POINT('Ctrl Pts',(-25.6868876116915,-12.3790435207342,
113.751397700364)) ;
#177524=CARTESIAN_POINT('Ctrl Pts',(-25.5868978508818,-12.3305042760163,
113.482273898361)) ;
#177525=CARTESIAN_POINT('Ctrl Pts',(-25.5859817904188,-12.4063616289538,
113.479483725613)) ;
#177526=CARTESIAN_POINT('Ctrl Pts',(-25.5121779408216,-12.4063616290811,
113.503714748484)) ;
#177527=CARTESIAN_POINT('Ctrl Pts',(-25.4383740912243,-12.4063616292084,
113.527945771355)) ;
#177528=CARTESIAN_POINT('Ctrl Pts',(-25.4392901516873,-12.3305042762709,
113.530735944103)) ;
#177529=CARTESIAN_POINT('Ctrl Pts',(-25.4402062121503,-12.2546469233334,
113.533526116851)) ;
#177530=CARTESIAN_POINT('Ctrl Pts',(-25.5140100617475,-12.2546469232061,
113.50929509398)) ;
#177531=CARTESIAN_POINT('Ctrl Pts',(-25.5878139113448,-12.2546469230788,
113.48506407111)) ;
#177532=CARTESIAN_POINT('Ctrl Pts',(-25.5868978508818,-12.3305042760163,
113.482273898361)) ;
#177533=CARTESIAN_POINT('Ctrl Pts',(-25.4854179660145,-12.3604684800267,
113.208869990196)) ;
#177534=CARTESIAN_POINT('Ctrl Pts',(-25.4908479731161,-12.434348796245,
113.225408915486)) ;
#177535=CARTESIAN_POINT('Ctrl Pts',(-25.4170441264006,-12.4343487994094,
113.249639947135)) ;
#177536=CARTESIAN_POINT('Ctrl Pts',(-25.3432402796852,-12.4343488025737,
113.273870978783)) ;
#177537=CARTESIAN_POINT('Ctrl Pts',(-25.3378102725836,-12.3604684863554,
113.257332053493)) ;
#177538=CARTESIAN_POINT('Ctrl Pts',(-25.332380265482,-12.2865881701371,
113.240793128203)) ;
#177539=CARTESIAN_POINT('Ctrl Pts',(-25.4061841121974,-12.2865881669728,
113.216562096555)) ;
#177540=CARTESIAN_POINT('Ctrl Pts',(-25.4799879589129,-12.2865881638084,
113.192331064906)) ;
#177541=CARTESIAN_POINT('Ctrl Pts',(-25.4854179660145,-12.3604684800267,
113.208869990196)) ;
#177542=CARTESIAN_POINT('Ctrl Pts',(-25.3908722354269,-12.4650891112354,
112.956114236995)) ;
#177543=CARTESIAN_POINT('Ctrl Pts',(-25.4021832258839,-12.5317749496589,
112.990565688778)) ;
#177544=CARTESIAN_POINT('Ctrl Pts',(-25.3283793807559,-12.5317749532163,
113.014796725262)) ;
#177545=CARTESIAN_POINT('Ctrl Pts',(-25.254575535628,-12.5317749567737,
113.039027761745)) ;
#177546=CARTESIAN_POINT('Ctrl Pts',(-25.2432645451709,-12.4650891183502,
113.004576309962)) ;
#177547=CARTESIAN_POINT('Ctrl Pts',(-25.2319535547139,-12.3984032799266,
112.970124858178)) ;
#177548=CARTESIAN_POINT('Ctrl Pts',(-25.3057573998419,-12.3984032763692,
112.945893821695)) ;
#177549=CARTESIAN_POINT('Ctrl Pts',(-25.3795612449698,-12.3984032728119,
112.921662785211)) ;
#177550=CARTESIAN_POINT('Ctrl Pts',(-25.3908722354269,-12.4650891112354,
112.956114236995)) ;
#177551=CARTESIAN_POINT('Ctrl Pts',(-25.3069218934639,-12.6397680496829,
112.736110244212)) ;
#177552=CARTESIAN_POINT('Ctrl Pts',(-25.3233734025477,-12.6943569653302,
112.786218886429)) ;
#177553=CARTESIAN_POINT('Ctrl Pts',(-25.2495695590936,-12.6943569660359,
112.810449928011)) ;
#177554=CARTESIAN_POINT('Ctrl Pts',(-25.1757657156394,-12.6943569667415,
112.834680969593)) ;
#177555=CARTESIAN_POINT('Ctrl Pts',(-25.1593142065557,-12.6397680510942,
112.784572327376)) ;
#177556=CARTESIAN_POINT('Ctrl Pts',(-25.1428626974719,-12.5851791354469,
112.734463685159)) ;
#177557=CARTESIAN_POINT('Ctrl Pts',(-25.216666540926,-12.5851791347412,
112.710232643577)) ;
#177558=CARTESIAN_POINT('Ctrl Pts',(-25.2904703843801,-12.5851791340356,
112.686001601995)) ;
#177559=CARTESIAN_POINT('Ctrl Pts',(-25.3069218934639,-12.6397680496829,
112.736110244212)) ;
#177560=CARTESIAN_POINT('Ctrl Pts',(-25.2409292762661,-12.8673926753431,
112.570297954244)) ;
#177561=CARTESIAN_POINT('Ctrl Pts',(-25.2612849273591,-12.9061686393151,
112.632297983135)) ;
#177562=CARTESIAN_POINT('Ctrl Pts',(-25.1874810842753,-12.9061686378558,
112.656529025845)) ;
#177563=CARTESIAN_POINT('Ctrl Pts',(-25.1136772411915,-12.9061686363964,
112.680760068555)) ;
#177564=CARTESIAN_POINT('Ctrl Pts',(-25.0933215900984,-12.8673926724244,
112.618760039664)) ;
#177565=CARTESIAN_POINT('Ctrl Pts',(-25.0729659390053,-12.8286167084523,
112.556760010772)) ;
#177566=CARTESIAN_POINT('Ctrl Pts',(-25.1467697820891,-12.8286167099117,
112.532528968062)) ;
#177567=CARTESIAN_POINT('Ctrl Pts',(-25.220573625173,-12.828616711371,112.508297925353)) ;
#177568=CARTESIAN_POINT('Ctrl Pts',(-25.2409292762661,-12.8673926753431,
112.570297954244)) ;
#177569=CARTESIAN_POINT('Ctrl Pts',(-25.1950431269417,-13.138383085188,
112.466309655478)) ;
#177570=CARTESIAN_POINT('Ctrl Pts',(-25.2178932655646,-13.1582932670834,
112.535907490935)) ;
#177571=CARTESIAN_POINT('Ctrl Pts',(-25.1440894224487,-13.15829326372,112.560138533547)) ;
#177572=CARTESIAN_POINT('Ctrl Pts',(-25.0702855793329,-13.1582932603565,
112.58436957616)) ;
#177573=CARTESIAN_POINT('Ctrl Pts',(-25.04743544071,-13.1383830784611,112.514771740703)) ;
#177574=CARTESIAN_POINT('Ctrl Pts',(-25.0245853020871,-13.1184728965658,
112.445173905246)) ;
#177575=CARTESIAN_POINT('Ctrl Pts',(-25.0983891452029,-13.1184728999292,
112.420942862634)) ;
#177576=CARTESIAN_POINT('Ctrl Pts',(-25.1721929883188,-13.1184729032926,
112.396711820022)) ;
#177577=CARTESIAN_POINT('Ctrl Pts',(-25.1950431269417,-13.138383085188,
112.466309655478)) ;
#177578=CARTESIAN_POINT('Ctrl Pts',(-25.1732970592646,-13.4250580301084,
112.435262725168)) ;
#177579=CARTESIAN_POINT('Ctrl Pts',(-25.1969709139446,-13.4249798616491,
112.507369466809)) ;
#177580=CARTESIAN_POINT('Ctrl Pts',(-25.123167070483,-13.4249798591319,
112.531600508368)) ;
#177581=CARTESIAN_POINT('Ctrl Pts',(-25.0493632270214,-13.4249798566146,
112.555831549927)) ;
#177582=CARTESIAN_POINT('Ctrl Pts',(-25.0256893723414,-13.4250580250739,
112.483724808286)) ;
#177583=CARTESIAN_POINT('Ctrl Pts',(-25.0020155176614,-13.4251361935332,
112.411618066645)) ;
#177584=CARTESIAN_POINT('Ctrl Pts',(-25.075819361123,-13.4251361960505,
112.387387025086)) ;
#177585=CARTESIAN_POINT('Ctrl Pts',(-25.1496232045846,-13.4251361985678,
112.363155983527)) ;
#177586=CARTESIAN_POINT('Ctrl Pts',(-25.1732970592646,-13.4250580301084,
112.435262725168)) ;
#177587=CARTESIAN_POINT('Ctrl Pts',(-25.175431424128,-13.713663843469,112.477262712461)) ;
#177588=CARTESIAN_POINT('Ctrl Pts',(-25.1982564463558,-13.6934329579285,
112.546784047362)) ;
#177589=CARTESIAN_POINT('Ctrl Pts',(-25.1244526028314,-13.6934329580841,
112.57101508873)) ;
#177590=CARTESIAN_POINT('Ctrl Pts',(-25.0506487593069,-13.6934329582396,
112.595246130098)) ;
#177591=CARTESIAN_POINT('Ctrl Pts',(-25.0278237370791,-13.7136638437801,
112.525724795196)) ;
#177592=CARTESIAN_POINT('Ctrl Pts',(-25.0049987148513,-13.7338947293205,
112.456203460295)) ;
#177593=CARTESIAN_POINT('Ctrl Pts',(-25.0788025583757,-13.733894729165,
112.431972418927)) ;
#177594=CARTESIAN_POINT('Ctrl Pts',(-25.1526064019001,-13.7338947290095,
112.407741377559)) ;
#177595=CARTESIAN_POINT('Ctrl Pts',(-25.175431424128,-13.713663843469,112.477262712461)) ;
#177596=CARTESIAN_POINT('Ctrl Pts',(-25.2013058612131,-13.9818996954329,
112.591702432285)) ;
#177597=CARTESIAN_POINT('Ctrl Pts',(-25.2216202953023,-13.9429089187137,
112.653576920689)) ;
#177598=CARTESIAN_POINT('Ctrl Pts',(-25.147816452688,-13.9429089238121,
112.677807964829)) ;
#177599=CARTESIAN_POINT('Ctrl Pts',(-25.0740126100738,-13.9429089289105,
112.702039008969)) ;
#177600=CARTESIAN_POINT('Ctrl Pts',(-25.0536981759845,-13.9818997056297,
112.640164520565)) ;
#177601=CARTESIAN_POINT('Ctrl Pts',(-25.0333837418953,-14.0208904823489,
112.578290032162)) ;
#177602=CARTESIAN_POINT('Ctrl Pts',(-25.1071875845096,-14.0208904772505,
112.554058988022)) ;
#177603=CARTESIAN_POINT('Ctrl Pts',(-25.1809914271238,-14.0208904721521,
112.529827943882)) ;
#177604=CARTESIAN_POINT('Ctrl Pts',(-25.2013058612131,-13.9818996954329,
112.591702432285)) ;
#177605=CARTESIAN_POINT('Ctrl Pts',(-25.2475462461254,-14.2073240866329,
112.767809158823)) ;
#177606=CARTESIAN_POINT('Ctrl Pts',(-25.2639316742078,-14.1525370337597,
112.817716528783)) ;
#177607=CARTESIAN_POINT('Ctrl Pts',(-25.1901278330324,-14.1525370412397,
112.841947577306)) ;
#177608=CARTESIAN_POINT('Ctrl Pts',(-25.116323991857,-14.1525370487197,
112.866178625828)) ;
#177609=CARTESIAN_POINT('Ctrl Pts',(-25.0999385637746,-14.2073241015929,
112.816271255868)) ;
#177610=CARTESIAN_POINT('Ctrl Pts',(-25.0835531356922,-14.2621111544661,
112.766363885908)) ;
#177611=CARTESIAN_POINT('Ctrl Pts',(-25.1573569768676,-14.2621111469861,
112.742132837385)) ;
#177612=CARTESIAN_POINT('Ctrl Pts',(-25.2311608180431,-14.2621111395061,
112.717901788863)) ;
#177613=CARTESIAN_POINT('Ctrl Pts',(-25.2475462461254,-14.2073240866329,
112.767809158823)) ;
#177614=CARTESIAN_POINT('Ctrl Pts',(-25.3107801482558,-14.3779496982449,
112.995927736214)) ;
#177615=CARTESIAN_POINT('Ctrl Pts',(-25.3220392060266,-14.3111692669398,
113.030221009202)) ;
#177616=CARTESIAN_POINT('Ctrl Pts',(-25.2482353673534,-14.3111692758398,
113.054452065346)) ;
#177617=CARTESIAN_POINT('Ctrl Pts',(-25.1744315286803,-14.3111692847398,
113.07868312149)) ;
#177618=CARTESIAN_POINT('Ctrl Pts',(-25.1631724709095,-14.3779497160448,
113.044389848502)) ;
#177619=CARTESIAN_POINT('Ctrl Pts',(-25.1519134131387,-14.4447301473499,
113.010096575515)) ;
#177620=CARTESIAN_POINT('Ctrl Pts',(-25.2257172518118,-14.4447301384499,
112.985865519371)) ;
#177621=CARTESIAN_POINT('Ctrl Pts',(-25.299521090485,-14.4447301295499,
112.961634463227)) ;
#177622=CARTESIAN_POINT('Ctrl Pts',(-25.3107801482558,-14.3779496982449,
112.995927736214)) ;
#177623=CARTESIAN_POINT('Ctrl Pts',(-25.3855441089235,-14.4795452062324,
113.25916632019)) ;
#177624=CARTESIAN_POINT('Ctrl Pts',(-25.390864299521,-14.405574238108,113.27537076184)) ;
#177625=CARTESIAN_POINT('Ctrl Pts',(-25.3170604639442,-14.4055742445888,
113.299601827415)) ;
#177626=CARTESIAN_POINT('Ctrl Pts',(-25.2432566283675,-14.4055742510696,
113.32383289299)) ;
#177627=CARTESIAN_POINT('Ctrl Pts',(-25.23793643777,-14.4795452191939,113.30762845134)) ;
#177628=CARTESIAN_POINT('Ctrl Pts',(-25.2326162471725,-14.5535161873183,
113.291424009691)) ;
#177629=CARTESIAN_POINT('Ctrl Pts',(-25.3064200827493,-14.5535161808375,
113.267192944116)) ;
#177630=CARTESIAN_POINT('Ctrl Pts',(-25.3802239183261,-14.5535161743567,
113.242961878541)) ;
#177631=CARTESIAN_POINT('Ctrl Pts',(-25.3855441089235,-14.4795452062324,
113.25916632019)) ;
#177632=CARTESIAN_POINT('Ctrl Pts',(-25.4657056298432,-14.504675613756,
113.538873967324)) ;
#177633=CARTESIAN_POINT('Ctrl Pts',(-25.4647009460347,-14.4288427645242,
113.53581386187)) ;
#177634=CARTESIAN_POINT('Ctrl Pts',(-25.3908971135579,-14.4288427635045,
113.560044936887)) ;
#177635=CARTESIAN_POINT('Ctrl Pts',(-25.3170932810811,-14.4288427624848,
113.584276011904)) ;
#177636=CARTESIAN_POINT('Ctrl Pts',(-25.3180979648896,-14.5046756117167,
113.587336117358)) ;
#177637=CARTESIAN_POINT('Ctrl Pts',(-25.3191026486981,-14.5805084609485,
113.590396222811)) ;
#177638=CARTESIAN_POINT('Ctrl Pts',(-25.3929064811749,-14.5805084619682,
113.566165147794)) ;
#177639=CARTESIAN_POINT('Ctrl Pts',(-25.4667103136517,-14.5805084629879,
113.541934072777)) ;
#177640=CARTESIAN_POINT('Ctrl Pts',(-25.4657056298432,-14.504675613756,
113.538873967324)) ;
#177641=CARTESIAN_POINT('Ctrl Pts',(-25.5441348471131,-14.4524935600785,
113.813035826526)) ;
#177642=CARTESIAN_POINT('Ctrl Pts',(-25.5369228144404,-14.3801950254555,
113.791069137853)) ;
#177643=CARTESIAN_POINT('Ctrl Pts',(-25.4631189835325,-14.3801950131856,
113.815300217648)) ;
#177644=CARTESIAN_POINT('Ctrl Pts',(-25.3893151526246,-14.3801950009157,
113.839531297444)) ;
#177645=CARTESIAN_POINT('Ctrl Pts',(-25.3965271852974,-14.4524935355387,
113.861497986118)) ;
#177646=CARTESIAN_POINT('Ctrl Pts',(-25.4037392179702,-14.5247920701618,
113.883464674792)) ;
#177647=CARTESIAN_POINT('Ctrl Pts',(-25.477543048878,-14.5247920824317,
113.859233594996)) ;
#177648=CARTESIAN_POINT('Ctrl Pts',(-25.5513468797859,-14.5247920947016,
113.8350025152)) ;
#177649=CARTESIAN_POINT('Ctrl Pts',(-25.5441348471131,-14.4524935600785,
113.813035826526)) ;
#177650=CARTESIAN_POINT('Ctrl Pts',(-25.6158038670484,-14.3253673837965,
114.066976143731)) ;
#177651=CARTESIAN_POINT('Ctrl Pts',(-25.6028398302001,-14.2618396984513,
114.027489778218)) ;
#177652=CARTESIAN_POINT('Ctrl Pts',(-25.5290360005822,-14.2618396702595,
114.051720861943)) ;
#177653=CARTESIAN_POINT('Ctrl Pts',(-25.4552321709644,-14.2618396420677,
114.075951945668)) ;
#177654=CARTESIAN_POINT('Ctrl Pts',(-25.4681962078127,-14.325367327413,
114.115438311181)) ;
#177655=CARTESIAN_POINT('Ctrl Pts',(-25.481160244661,-14.3888950127582,
114.154924676695)) ;
#177656=CARTESIAN_POINT('Ctrl Pts',(-25.5549640742788,-14.38889504095,114.13069359297)) ;
#177657=CARTESIAN_POINT('Ctrl Pts',(-25.6287679038966,-14.3888950691418,
114.106462509245)) ;
#177658=CARTESIAN_POINT('Ctrl Pts',(-25.6158038670484,-14.3253673837965,
114.066976143731)) ;
#177659=CARTESIAN_POINT('Ctrl Pts',(-25.6735934060056,-14.1335026343525,
114.278447647152)) ;
#177660=CARTESIAN_POINT('Ctrl Pts',(-25.6558422293983,-14.0832788793335,
114.224380426171)) ;
#177661=CARTESIAN_POINT('Ctrl Pts',(-25.5820383986289,-14.0832788338596,
114.248611506388)) ;
#177662=CARTESIAN_POINT('Ctrl Pts',(-25.5082345678594,-14.0832787883857,
114.272842586606)) ;
#177663=CARTESIAN_POINT('Ctrl Pts',(-25.5259857444668,-14.1335025434047,
114.326909807587)) ;
#177664=CARTESIAN_POINT('Ctrl Pts',(-25.5437369210741,-14.1837262984236,
114.380977028568)) ;
#177665=CARTESIAN_POINT('Ctrl Pts',(-25.6175407518436,-14.1837263438975,
114.356745948351)) ;
#177666=CARTESIAN_POINT('Ctrl Pts',(-25.691344582613,-14.1837263893715,
114.332514868133)) ;
#177667=CARTESIAN_POINT('Ctrl Pts',(-25.6735934060056,-14.1335026343525,
114.278447647152)) ;
#177668=CARTESIAN_POINT('Ctrl Pts',(-25.713031726844,-13.8914689377216,
114.433910815975)) ;
#177669=CARTESIAN_POINT('Ctrl Pts',(-25.6917702020142,-13.8580710694063,
114.369151640563)) ;
#177670=CARTESIAN_POINT('Ctrl Pts',(-25.6179663680164,-13.8580710084392,
114.393382710947)) ;
#177671=CARTESIAN_POINT('Ctrl Pts',(-25.5441625340186,-13.8580709474722,
114.417613781332)) ;
#177672=CARTESIAN_POINT('Ctrl Pts',(-25.5654240588485,-13.8914688157875,
114.482372956744)) ;
#177673=CARTESIAN_POINT('Ctrl Pts',(-25.5866855836783,-13.9248666841028,
114.547132132156)) ;
#177674=CARTESIAN_POINT('Ctrl Pts',(-25.6604894176761,-13.9248667450698,
114.522901061771)) ;
#177675=CARTESIAN_POINT('Ctrl Pts',(-25.7342932516738,-13.9248668060369,
114.498669991387)) ;
#177676=CARTESIAN_POINT('Ctrl Pts',(-25.713031726844,-13.8914689377216,
114.433910815975)) ;
#177677=CARTESIAN_POINT('Ctrl Pts',(-25.7307687812816,-13.6147208150664,
114.523401386807)) ;
#177678=CARTESIAN_POINT('Ctrl Pts',(-25.7075042451934,-13.6005963890855,
114.452541362134)) ;
#177679=CARTESIAN_POINT('Ctrl Pts',(-25.6337004062679,-13.6005963145347,
114.476772417509)) ;
#177680=CARTESIAN_POINT('Ctrl Pts',(-25.5598965673424,-13.600596239984,
114.501003472884)) ;
#177681=CARTESIAN_POINT('Ctrl Pts',(-25.5831611034306,-13.6147206659649,
114.571863497557)) ;
#177682=CARTESIAN_POINT('Ctrl Pts',(-25.6064256395188,-13.6288450919457,
114.64272352223)) ;
#177683=CARTESIAN_POINT('Ctrl Pts',(-25.6802294784443,-13.6288451664965,
114.618492466855)) ;
#177684=CARTESIAN_POINT('Ctrl Pts',(-25.7540333173698,-13.6288452410473,
114.59426141148)) ;
#177685=CARTESIAN_POINT('Ctrl Pts',(-25.7307687812816,-13.6147208150664,
114.523401386807)) ;
#177686=CARTESIAN_POINT('Ctrl Pts',(-25.7245757601632,-13.3237687258409,
114.540012491979)) ;
#177687=CARTESIAN_POINT('Ctrl Pts',(-25.7009758198009,-13.3299371797537,
114.468130879862)) ;
#177688=CARTESIAN_POINT('Ctrl Pts',(-25.6271719743241,-13.3299370967314,
114.492361915283)) ;
#177689=CARTESIAN_POINT('Ctrl Pts',(-25.5533681288474,-13.329937013709,
114.516592950705)) ;
#177690=CARTESIAN_POINT('Ctrl Pts',(-25.5769680692097,-13.3237685597962,
114.588474562821)) ;
#177691=CARTESIAN_POINT('Ctrl Pts',(-25.600568009572,-13.3176001058834,
114.660356174938)) ;
#177692=CARTESIAN_POINT('Ctrl Pts',(-25.6743718550487,-13.3176001889057,
114.636125139517)) ;
#177693=CARTESIAN_POINT('Ctrl Pts',(-25.7481757005255,-13.3176002719281,
114.611894104095)) ;
#177694=CARTESIAN_POINT('Ctrl Pts',(-25.7245757601632,-13.3237687258409,
114.540012491979)) ;
#177695=CARTESIAN_POINT('Ctrl Pts',(-25.6941237439954,-13.0396242352637,
114.482736350999)) ;
#177696=CARTESIAN_POINT('Ctrl Pts',(-25.671881485573,-13.0656396906541,
114.414990018884)) ;
#177697=CARTESIAN_POINT('Ctrl Pts',(-25.598077632554,-13.0656396062825,
114.439221031332)) ;
#177698=CARTESIAN_POINT('Ctrl Pts',(-25.5242737795349,-13.0656395219109,
114.463452043781)) ;
#177699=CARTESIAN_POINT('Ctrl Pts',(-25.5465160379572,-13.0396240665205,
114.531198375896)) ;
#177700=CARTESIAN_POINT('Ctrl Pts',(-25.5687582963795,-13.0136086111301,
114.598944708012)) ;
#177701=CARTESIAN_POINT('Ctrl Pts',(-25.6425621493986,-13.0136086955017,
114.574713695563)) ;
#177702=CARTESIAN_POINT('Ctrl Pts',(-25.7163660024177,-13.0136087798733,
114.550482683115)) ;
#177703=CARTESIAN_POINT('Ctrl Pts',(-25.6941237439954,-13.0396242352637,
114.482736350999)) ;
#177704=CARTESIAN_POINT('Ctrl Pts',(-25.6410851839242,-12.7830678889279,
114.356574719083)) ;
#177705=CARTESIAN_POINT('Ctrl Pts',(-25.6217813743788,-12.8270330002595,
114.297778428028)) ;
#177706=CARTESIAN_POINT('Ctrl Pts',(-25.5479775137743,-12.8270329227443,
114.322009417373)) ;
#177707=CARTESIAN_POINT('Ctrl Pts',(-25.4741736531698,-12.8270328452292,
114.346240406717)) ;
#177708=CARTESIAN_POINT('Ctrl Pts',(-25.4934774627152,-12.7830677338975,
114.405036697772)) ;
#177709=CARTESIAN_POINT('Ctrl Pts',(-25.5127812722606,-12.7391026225659,
114.463832988827)) ;
#177710=CARTESIAN_POINT('Ctrl Pts',(-25.5865851328651,-12.739102700081,
114.439601999483)) ;
#177711=CARTESIAN_POINT('Ctrl Pts',(-25.6603889934697,-12.7391027775962,
114.415371010139)) ;
#177712=CARTESIAN_POINT('Ctrl Pts',(-25.6410851839242,-12.7830678889279,
114.356574719083)) ;
#177713=CARTESIAN_POINT('Ctrl Pts',(-25.5676997033759,-12.5704752635878,
114.168721963641)) ;
#177714=CARTESIAN_POINT('Ctrl Pts',(-25.5527529624881,-12.6293473017033,
114.123196600596)) ;
#177715=CARTESIAN_POINT('Ctrl Pts',(-25.4789490946422,-12.6293472382111,
114.147427567884)) ;
#177716=CARTESIAN_POINT('Ctrl Pts',(-25.4051452267963,-12.6293471747189,
114.171658535172)) ;
#177717=CARTESIAN_POINT('Ctrl Pts',(-25.4200919676841,-12.5704751366034,
114.217183898218)) ;
#177718=CARTESIAN_POINT('Ctrl Pts',(-25.4350387085718,-12.5116030984879,
114.262709261263)) ;
#177719=CARTESIAN_POINT('Ctrl Pts',(-25.5088425764177,-12.5116031619801,
114.238478293975)) ;
#177720=CARTESIAN_POINT('Ctrl Pts',(-25.5826464442636,-12.5116032254723,
114.214247326686)) ;
#177721=CARTESIAN_POINT('Ctrl Pts',(-25.5676997033759,-12.5704752635878,
114.168721963641)) ;
#177722=CARTESIAN_POINT('Ctrl Pts',(-25.4799422590946,-12.4206416986158,
113.936696566694)) ;
#177723=CARTESIAN_POINT('Ctrl Pts',(-25.4703708909182,-12.490060480766,
113.90754372156)) ;
#177724=CARTESIAN_POINT('Ctrl Pts',(-25.3965670178971,-12.4900604392227,
113.931774673086)) ;
#177725=CARTESIAN_POINT('Ctrl Pts',(-25.3227631448761,-12.4900603976793,
113.956005624611)) ;
#177726=CARTESIAN_POINT('Ctrl Pts',(-25.3323345130525,-12.4206416155292,
113.985158469745)) ;
#177727=CARTESIAN_POINT('Ctrl Pts',(-25.341905881229,-12.351222833379,114.014311314878)) ;
#177728=CARTESIAN_POINT('Ctrl Pts',(-25.41570975425,-12.3512228749223,113.990080363353)) ;
#177729=CARTESIAN_POINT('Ctrl Pts',(-25.4895136272711,-12.3512229164656,
113.965849411827)) ;
#177730=CARTESIAN_POINT('Ctrl Pts',(-25.4799422590946,-12.4206416986158,
113.936696566694)) ;
#177731=CARTESIAN_POINT('Ctrl Pts',(-25.381998179666,-12.3408954926335,
113.673866420762)) ;
#177732=CARTESIAN_POINT('Ctrl Pts',(-25.3785163984105,-12.4159838825569,
113.663261474782)) ;
#177733=CARTESIAN_POINT('Ctrl Pts',(-25.3047125221132,-12.4159838672949,
113.687492416329)) ;
#177734=CARTESIAN_POINT('Ctrl Pts',(-25.2309086458159,-12.4159838520328,
113.711723357875)) ;
#177735=CARTESIAN_POINT('Ctrl Pts',(-25.2343904270714,-12.3408954621094,
113.722328303855)) ;
#177736=CARTESIAN_POINT('Ctrl Pts',(-25.2378722083269,-12.265807072186,
113.732933249835)) ;
#177737=CARTESIAN_POINT('Ctrl Pts',(-25.3116760846242,-12.265807087448,
113.708702308288)) ;
#177738=CARTESIAN_POINT('Ctrl Pts',(-25.3854799609215,-12.26580710271,113.684471366741)) ;
#177739=CARTESIAN_POINT('Ctrl Pts',(-25.381998179666,-12.3408954926335,
113.673866420762)) ;
#177740=CARTESIAN_POINT('Ctrl Pts',(-25.2803675767541,-12.3388375024718,
113.399883536457)) ;
#177741=CARTESIAN_POINT('Ctrl Pts',(-25.2832401365507,-12.4141806587766,
113.408632888022)) ;
#177742=CARTESIAN_POINT('Ctrl Pts',(-25.2094362596863,-12.414180672439,
113.432863827842)) ;
#177743=CARTESIAN_POINT('Ctrl Pts',(-25.1356323828219,-12.4141806861015,
113.457094767661)) ;
#177744=CARTESIAN_POINT('Ctrl Pts',(-25.1327598230253,-12.3388375297967,
113.448345416096)) ;
#177745=CARTESIAN_POINT('Ctrl Pts',(-25.1298872632288,-12.263494373492,
113.439596064531)) ;
#177746=CARTESIAN_POINT('Ctrl Pts',(-25.2036911400932,-12.2634943598295,
113.415365124712)) ;
#177747=CARTESIAN_POINT('Ctrl Pts',(-25.2774950169575,-12.2634943461671,
113.391134184892)) ;
#177748=CARTESIAN_POINT('Ctrl Pts',(-25.2803675767541,-12.3388375024718,
113.399883536457)) ;
#177749=CARTESIAN_POINT('Ctrl Pts',(-25.1823213194761,-12.413706142133,
113.136628920894)) ;
#177750=CARTESIAN_POINT('Ctrl Pts',(-25.1913113188617,-12.4839334398815,
113.164011006395)) ;
#177751=CARTESIAN_POINT('Ctrl Pts',(-25.1175074442267,-12.4839334817003,
113.188241953004)) ;
#177752=CARTESIAN_POINT('Ctrl Pts',(-25.0437035695917,-12.4839335235192,
113.212472899614)) ;
#177753=CARTESIAN_POINT('Ctrl Pts',(-25.0347135702062,-12.4137062257707,
113.185090814114)) ;
#177754=CARTESIAN_POINT('Ctrl Pts',(-25.0257235708206,-12.3434789280223,
113.157708728613)) ;
#177755=CARTESIAN_POINT('Ctrl Pts',(-25.0995274454556,-12.3434788862035,
113.133477782003)) ;
#177756=CARTESIAN_POINT('Ctrl Pts',(-25.1733313200905,-12.3434788443846,
113.109246835393)) ;
#177757=CARTESIAN_POINT('Ctrl Pts',(-25.1823213194761,-12.413706142133,
113.136628920894)) ;
#177758=CARTESIAN_POINT('Ctrl Pts',(-25.092980715359,-12.5617183582742,
112.900167957605)) ;
#177759=CARTESIAN_POINT('Ctrl Pts',(-25.1074837531034,-12.6217168854957,
112.944341868443)) ;
#177760=CARTESIAN_POINT('Ctrl Pts',(-25.0336798833631,-12.6217169518503,
112.968572829961)) ;
#177761=CARTESIAN_POINT('Ctrl Pts',(-24.9598760136228,-12.6217170182048,
112.992803791479)) ;
#177762=CARTESIAN_POINT('Ctrl Pts',(-24.9453729758784,-12.5617184909834,
112.948629880641)) ;
#177763=CARTESIAN_POINT('Ctrl Pts',(-24.930869938134,-12.501719963762,112.904455969803)) ;
#177764=CARTESIAN_POINT('Ctrl Pts',(-25.0046738078743,-12.5017198974074,
112.880225008285)) ;
#177765=CARTESIAN_POINT('Ctrl Pts',(-25.0784776776146,-12.5017198310528,
112.855994046767)) ;
#177766=CARTESIAN_POINT('Ctrl Pts',(-25.092980715359,-12.5617183582742,
112.900167957605)) ;
#177767=CARTESIAN_POINT('Ctrl Pts',(-25.0195846393668,-12.7688407831079,
112.711834010416)) ;
#177768=CARTESIAN_POINT('Ctrl Pts',(-25.0385047320968,-12.8144672602671,
112.76946155808)) ;
#177769=CARTESIAN_POINT('Ctrl Pts',(-24.964700869039,-12.8144673453734,
112.793692539952)) ;
#177770=CARTESIAN_POINT('Ctrl Pts',(-24.8908970059813,-12.8144674304797,
112.817923521824)) ;
#177771=CARTESIAN_POINT('Ctrl Pts',(-24.8719769132512,-12.7688409533206,
112.76029597416)) ;
#177772=CARTESIAN_POINT('Ctrl Pts',(-24.8530568205212,-12.7232144761614,
112.702668426497)) ;
#177773=CARTESIAN_POINT('Ctrl Pts',(-24.926860683579,-12.7232143910551,
112.678437444625)) ;
#177774=CARTESIAN_POINT('Ctrl Pts',(-25.0006645466367,-12.7232143059487,
112.654206462753)) ;
#177775=CARTESIAN_POINT('Ctrl Pts',(-25.0195846393668,-12.7688407831079,
112.711834010416)) ;
#177776=CARTESIAN_POINT('Ctrl Pts',(-24.9649866794184,-13.0241117816514,
112.581077125632)) ;
#177777=CARTESIAN_POINT('Ctrl Pts',(-24.9870115430439,-13.0519843902153,
112.648161304551)) ;
#177778=CARTESIAN_POINT('Ctrl Pts',(-24.9132076881355,-13.0519844861314,
112.672392311245)) ;
#177779=CARTESIAN_POINT('Ctrl Pts',(-24.839403833227,-13.0519845820475,
112.696623317938)) ;
#177780=CARTESIAN_POINT('Ctrl Pts',(-24.8173789696015,-13.0241119734836,
112.629539139019)) ;
#177781=CARTESIAN_POINT('Ctrl Pts',(-24.795354105976,-12.9962393649197,
112.5624549601)) ;
#177782=CARTESIAN_POINT('Ctrl Pts',(-24.8691579608845,-12.9962392690036,
112.538223953407)) ;
#177783=CARTESIAN_POINT('Ctrl Pts',(-24.9429618157929,-12.9962391730874,
112.513992946713)) ;
#177784=CARTESIAN_POINT('Ctrl Pts',(-24.9649866794184,-13.0241117816514,
112.581077125632)) ;
#177785=CARTESIAN_POINT('Ctrl Pts',(-24.9332536836434,-13.3070010234793,
112.51985755415)) ;
#177786=CARTESIAN_POINT('Ctrl Pts',(-24.9567938392213,-13.31516473517,112.591557067941)) ;
#177787=CARTESIAN_POINT('Ctrl Pts',(-24.8829899928049,-13.3151648334865,
112.6157881005)) ;
#177788=CARTESIAN_POINT('Ctrl Pts',(-24.8091861463885,-13.315164931803,
112.640019133059)) ;
#177789=CARTESIAN_POINT('Ctrl Pts',(-24.7856459908106,-13.3070012201123,
112.568319619268)) ;
#177790=CARTESIAN_POINT('Ctrl Pts',(-24.7621058352326,-13.2988375084216,
112.496620105477)) ;
#177791=CARTESIAN_POINT('Ctrl Pts',(-24.8359096816491,-13.2988374101051,
112.472389072918)) ;
#177792=CARTESIAN_POINT('Ctrl Pts',(-24.9097135280655,-13.2988373117886,
112.448158040359)) ;
#177793=CARTESIAN_POINT('Ctrl Pts',(-24.9332536836434,-13.3070010234793,
112.51985755415)) ;
#177794=CARTESIAN_POINT('Ctrl Pts',(-24.925629722327,-13.5985554109386,
112.532164471356)) ;
#177795=CARTESIAN_POINT('Ctrl Pts',(-24.9490024367954,-13.5863758262572,
112.603353986648)) ;
#177796=CARTESIAN_POINT('Ctrl Pts',(-24.8751985984021,-13.5863759182584,
112.627585043645)) ;
#177797=CARTESIAN_POINT('Ctrl Pts',(-24.8013947600088,-13.5863760102596,
112.651816100641)) ;
#177798=CARTESIAN_POINT('Ctrl Pts',(-24.7780220455404,-13.5985555949411,
112.580626585349)) ;
#177799=CARTESIAN_POINT('Ctrl Pts',(-24.754649331072,-13.6107351796225,
112.509437070056)) ;
#177800=CARTESIAN_POINT('Ctrl Pts',(-24.8284531694653,-13.6107350876213,
112.48520601306)) ;
#177801=CARTESIAN_POINT('Ctrl Pts',(-24.9022570078586,-13.6107349956201,
112.460974956064)) ;
#177802=CARTESIAN_POINT('Ctrl Pts',(-24.925629722327,-13.5985554109386,
112.532164471356)) ;
#177803=CARTESIAN_POINT('Ctrl Pts',(-24.9421245854702,-13.8770852609277,
112.617931075453)) ;
#177804=CARTESIAN_POINT('Ctrl Pts',(-24.9636458203389,-13.8454408144546,
112.683481282746)) ;
#177805=CARTESIAN_POINT('Ctrl Pts',(-24.8898419885264,-13.8454408929621,
112.707712359786)) ;
#177806=CARTESIAN_POINT('Ctrl Pts',(-24.8160381567138,-13.8454409714697,
112.731943436827)) ;
#177807=CARTESIAN_POINT('Ctrl Pts',(-24.7945169218452,-13.8770854179428,
112.666393229534)) ;
#177808=CARTESIAN_POINT('Ctrl Pts',(-24.7729956869765,-13.9087298644159,
112.600843022241)) ;
#177809=CARTESIAN_POINT('Ctrl Pts',(-24.846799518789,-13.9087297859083,
112.576611945201)) ;
#177810=CARTESIAN_POINT('Ctrl Pts',(-24.9206033506015,-13.9087297074008,
112.552380868161)) ;
#177811=CARTESIAN_POINT('Ctrl Pts',(-24.9421245854702,-13.8770852609277,
112.617931075453)) ;
#177812=CARTESIAN_POINT('Ctrl Pts',(-24.9804514510273,-14.1214182763711,
112.770005884966)) ;
#177813=CARTESIAN_POINT('Ctrl Pts',(-24.9985978942237,-14.0726671201406,
112.825277021458)) ;
#177814=CARTESIAN_POINT('Ctrl Pts',(-24.9247940672919,-14.0726671815673,
112.849508113365)) ;
#177815=CARTESIAN_POINT('Ctrl Pts',(-24.8509902403602,-14.072667242994,
112.873739205271)) ;
#177816=CARTESIAN_POINT('Ctrl Pts',(-24.8328437971638,-14.1214183992245,
112.818468068778)) ;
#177817=CARTESIAN_POINT('Ctrl Pts',(-24.8146973539674,-14.170169555455,
112.763196932286)) ;
#177818=CARTESIAN_POINT('Ctrl Pts',(-24.8885011808991,-14.1701694940283,
112.738965840379)) ;
#177819=CARTESIAN_POINT('Ctrl Pts',(-24.9623050078308,-14.1701694326015,
112.714734748473)) ;
#177820=CARTESIAN_POINT('Ctrl Pts',(-24.9804514510273,-14.1214182763711,
112.770005884966)) ;
#177821=CARTESIAN_POINT('Ctrl Pts',(-25.0373635997591,-14.3164119676812,
112.978804934412)) ;
#177822=CARTESIAN_POINT('Ctrl Pts',(-25.0508302922444,-14.2539728440819,
113.019822305455)) ;
#177823=CARTESIAN_POINT('Ctrl Pts',(-24.9770264679556,-14.2539728850066,
113.044053405412)) ;
#177824=CARTESIAN_POINT('Ctrl Pts',(-24.9032226436669,-14.2539729259314,
113.068284505368)) ;
#177825=CARTESIAN_POINT('Ctrl Pts',(-24.8897559511816,-14.3164120495308,
113.027267134325)) ;
#177826=CARTESIAN_POINT('Ctrl Pts',(-24.8762892586964,-14.3788511731302,
112.986249763282)) ;
#177827=CARTESIAN_POINT('Ctrl Pts',(-24.9500930829851,-14.3788511322054,
112.962018663326)) ;
#177828=CARTESIAN_POINT('Ctrl Pts',(-25.0238969072739,-14.3788510912806,
112.937787563369)) ;
#177829=CARTESIAN_POINT('Ctrl Pts',(-25.0373635997591,-14.3164119676812,
112.978804934412)) ;
#177830=CARTESIAN_POINT('Ctrl Pts',(-25.1082654742619,-14.4472714989735,
113.230330811616)) ;
#177831=CARTESIAN_POINT('Ctrl Pts',(-25.1160662154225,-14.3756009231922,
113.254090609297)) ;
#177832=CARTESIAN_POINT('Ctrl Pts',(-25.042262391181,-14.3756009434077,
113.278321709397)) ;
#177833=CARTESIAN_POINT('Ctrl Pts',(-24.9684585669394,-14.3756009636232,
113.302552809497)) ;
#177834=CARTESIAN_POINT('Ctrl Pts',(-24.9606578257788,-14.4472715394045,
113.278793011817)) ;
#177835=CARTESIAN_POINT('Ctrl Pts',(-24.9528570846181,-14.5189421151858,
113.255033214136)) ;
#177836=CARTESIAN_POINT('Ctrl Pts',(-25.0266609088597,-14.5189420949703,
113.230802114036)) ;
#177837=CARTESIAN_POINT('Ctrl Pts',(-25.1004647331012,-14.5189420747548,
113.206571013936)) ;
#177838=CARTESIAN_POINT('Ctrl Pts',(-25.1082654742619,-14.4472714989735,
113.230330811616)) ;
#177839=CARTESIAN_POINT('Ctrl Pts',(-25.1868459524037,-14.5039655219921,
113.505134344491)) ;
#177840=CARTESIAN_POINT('Ctrl Pts',(-25.1884382106034,-14.4282278620231,
113.509984104971)) ;
#177841=CARTESIAN_POINT('Ctrl Pts',(-25.1146343847165,-14.4282278646451,
113.534215200059)) ;
#177842=CARTESIAN_POINT('Ctrl Pts',(-25.0408305588296,-14.4282278672671,
113.558446295148)) ;
#177843=CARTESIAN_POINT('Ctrl Pts',(-25.0392383006299,-14.5039655272361,
113.553596534669)) ;
#177844=CARTESIAN_POINT('Ctrl Pts',(-25.0376460424301,-14.5797031872051,
113.548746774189)) ;
#177845=CARTESIAN_POINT('Ctrl Pts',(-25.111449868317,-14.5797031845831,
113.5245156791)) ;
#177846=CARTESIAN_POINT('Ctrl Pts',(-25.1852536942039,-14.5797031819611,
113.500284584012)) ;
#177847=CARTESIAN_POINT('Ctrl Pts',(-25.1868459524037,-14.5039655219921,
113.505134344491)) ;
#177848=CARTESIAN_POINT('Ctrl Pts',(-25.267129516287,-14.4826373105238,
113.785223901541)) ;
#177849=CARTESIAN_POINT('Ctrl Pts',(-25.2623828413335,-14.4082736216989,
113.770766294605)) ;
#177850=CARTESIAN_POINT('Ctrl Pts',(-25.188579012109,-14.4082736113454,
113.794997379528)) ;
#177851=CARTESIAN_POINT('Ctrl Pts',(-25.1147751828845,-14.4082736009919,
113.819228464451)) ;
#177852=CARTESIAN_POINT('Ctrl Pts',(-25.1195218578379,-14.4826372898169,
113.833686071387)) ;
#177853=CARTESIAN_POINT('Ctrl Pts',(-25.1242685327913,-14.5570009786418,
113.848143678323)) ;
#177854=CARTESIAN_POINT('Ctrl Pts',(-25.1980723620159,-14.5570009889953,
113.8239125934)) ;
#177855=CARTESIAN_POINT('Ctrl Pts',(-25.2718761912404,-14.5570009993487,
113.799681508477)) ;
#177856=CARTESIAN_POINT('Ctrl Pts',(-25.267129516287,-14.4826373105238,
113.785223901541)) ;
#177857=CARTESIAN_POINT('Ctrl Pts',(-25.3418916496393,-14.3855815012644,
114.048250710986)) ;
#177858=CARTESIAN_POINT('Ctrl Pts',(-25.3311870097103,-14.3178820902551,
114.015646104187)) ;
#177859=CARTESIAN_POINT('Ctrl Pts',(-25.2573831771349,-14.3178820716342,
114.039877178904)) ;
#177860=CARTESIAN_POINT('Ctrl Pts',(-25.1835793445595,-14.3178820530132,
114.064108253621)) ;
#177861=CARTESIAN_POINT('Ctrl Pts',(-25.1942839844885,-14.3855814640225,
114.096712860419)) ;
#177862=CARTESIAN_POINT('Ctrl Pts',(-25.2049886244175,-14.4532808750318,
114.129317467217)) ;
#177863=CARTESIAN_POINT('Ctrl Pts',(-25.2787924569929,-14.4532808936528,
114.105086392501)) ;
#177864=CARTESIAN_POINT('Ctrl Pts',(-25.3525962895683,-14.4532809122737,
114.080855317784)) ;
#177865=CARTESIAN_POINT('Ctrl Pts',(-25.3418916496393,-14.3855815012644,
114.048250710986)) ;
#177866=CARTESIAN_POINT('Ctrl Pts',(-25.4059102519348,-14.2190969785884,
114.278710495903)) ;
#177867=CARTESIAN_POINT('Ctrl Pts',(-25.3899854352774,-14.1629192872983,
114.230206073229)) ;
#177868=CARTESIAN_POINT('Ctrl Pts',(-25.3161815987738,-14.1629192658567,
114.254437135981)) ;
#177869=CARTESIAN_POINT('Ctrl Pts',(-25.2423777622703,-14.1629192444152,
114.278668198734)) ;
#177870=CARTESIAN_POINT('Ctrl Pts',(-25.2583025789277,-14.2190969357053,
114.327172621408)) ;
#177871=CARTESIAN_POINT('Ctrl Pts',(-25.2742273955851,-14.2752746269954,
114.375677044082)) ;
#177872=CARTESIAN_POINT('Ctrl Pts',(-25.3480312320887,-14.275274648437,
114.35144598133)) ;
#177873=CARTESIAN_POINT('Ctrl Pts',(-25.4218350685922,-14.2752746698786,
114.327214918577)) ;
#177874=CARTESIAN_POINT('Ctrl Pts',(-25.4059102519348,-14.2190969785884,
114.278710495903)) ;
#177875=CARTESIAN_POINT('Ctrl Pts',(-25.4534572816173,-13.9949296481822,
114.4590197693)) ;
#177876=CARTESIAN_POINT('Ctrl Pts',(-25.4334540036049,-13.9543190677503,
114.398093011557)) ;
#177877=CARTESIAN_POINT('Ctrl Pts',(-25.35965016373,-13.9543190483412,114.42232406404)) ;
#177878=CARTESIAN_POINT('Ctrl Pts',(-25.285846323855,-13.9543190289321,
114.446555116524)) ;
#177879=CARTESIAN_POINT('Ctrl Pts',(-25.3058496018674,-13.9949296093639,
114.507481874267)) ;
#177880=CARTESIAN_POINT('Ctrl Pts',(-25.3258528798797,-14.0355401897957,
114.568408632009)) ;
#177881=CARTESIAN_POINT('Ctrl Pts',(-25.3996567197547,-14.0355402092049,
114.544177579526)) ;
#177882=CARTESIAN_POINT('Ctrl Pts',(-25.4734605596297,-14.035540228614,
114.519946527043)) ;
#177883=CARTESIAN_POINT('Ctrl Pts',(-25.4534572816173,-13.9949296481822,
114.4590197693)) ;
#177884=CARTESIAN_POINT('Ctrl Pts',(-25.4803949407615,-13.7298783707897,
114.576500255508)) ;
#177885=CARTESIAN_POINT('Ctrl Pts',(-25.457747280991,-13.7077134495774,
114.507519137741)) ;
#177886=CARTESIAN_POINT('Ctrl Pts',(-25.3839434387268,-13.7077134348718,
114.531750182947)) ;
#177887=CARTESIAN_POINT('Ctrl Pts',(-25.3101395964625,-13.7077134201661,
114.555981228153)) ;
#177888=CARTESIAN_POINT('Ctrl Pts',(-25.332787256233,-13.7298783413784,
114.624962345921)) ;
#177889=CARTESIAN_POINT('Ctrl Pts',(-25.3554349160035,-13.7520432625907,
114.693943463688)) ;
#177890=CARTESIAN_POINT('Ctrl Pts',(-25.4292387582677,-13.7520432772964,
114.669712418482)) ;
#177891=CARTESIAN_POINT('Ctrl Pts',(-25.5030426005319,-13.752043292002,
114.645481373276)) ;
#177892=CARTESIAN_POINT('Ctrl Pts',(-25.4803949407615,-13.7298783707897,
114.576500255508)) ;
#177893=CARTESIAN_POINT('Ctrl Pts',(-25.4839639384194,-13.4411780607526,
114.622967439281)) ;
#177894=CARTESIAN_POINT('Ctrl Pts',(-25.4602961356255,-13.4391385958436,
114.550879130608)) ;
#177895=CARTESIAN_POINT('Ctrl Pts',(-25.3864922921103,-13.4391385881017,
114.575110172003)) ;
#177896=CARTESIAN_POINT('Ctrl Pts',(-25.312688448595,-13.4391385803598,
114.599341213399)) ;
#177897=CARTESIAN_POINT('Ctrl Pts',(-25.336356251389,-13.4411780452688,
114.671429522073)) ;
#177898=CARTESIAN_POINT('Ctrl Pts',(-25.3600240541829,-13.4432175101778,
114.743517830747)) ;
#177899=CARTESIAN_POINT('Ctrl Pts',(-25.4338278976981,-13.4432175179197,
114.719286789351)) ;
#177900=CARTESIAN_POINT('Ctrl Pts',(-25.5076317412133,-13.4432175256616,
114.695055747955)) ;
#177901=CARTESIAN_POINT('Ctrl Pts',(-25.4839639384194,-13.4411780607526,
114.622967439281)) ;
#177902=CARTESIAN_POINT('Ctrl Pts',(-25.4634405619125,-13.1535366585443,
114.595704133561)) ;
#177903=CARTESIAN_POINT('Ctrl Pts',(-25.4404409966477,-13.1715786657878,
114.525651168662)) ;
#177904=CARTESIAN_POINT('Ctrl Pts',(-25.3666371528437,-13.1715786624699,
114.549882209178)) ;
#177905=CARTESIAN_POINT('Ctrl Pts',(-25.2928333090395,-13.1715786591521,
114.574113249694)) ;
#177906=CARTESIAN_POINT('Ctrl Pts',(-25.3158328743043,-13.1535366519086,
114.644166214593)) ;
#177907=CARTESIAN_POINT('Ctrl Pts',(-25.3388324395691,-13.1354946446651,
114.714219179492)) ;
#177908=CARTESIAN_POINT('Ctrl Pts',(-25.4126362833732,-13.1354946479829,
114.689988138976)) ;
#177909=CARTESIAN_POINT('Ctrl Pts',(-25.4864401271773,-13.1354946513008,
114.66575709846)) ;
#177910=CARTESIAN_POINT('Ctrl Pts',(-25.4634405619125,-13.1535366585443,
114.595704133561)) ;
#177911=CARTESIAN_POINT('Ctrl Pts',(-25.4188861853407,-12.8812078446008,
114.495722751362)) ;
#177912=CARTESIAN_POINT('Ctrl Pts',(-25.3982238139182,-12.9182937200929,
114.432788501901)) ;
#177913=CARTESIAN_POINT('Ctrl Pts',(-25.3244199706641,-12.9182937216163,
114.457019544092)) ;
#177914=CARTESIAN_POINT('Ctrl Pts',(-25.2506161274099,-12.9182937231397,
114.481250586283)) ;
#177915=CARTESIAN_POINT('Ctrl Pts',(-25.2712784988323,-12.8812078476476,
114.544184835744)) ;
#177916=CARTESIAN_POINT('Ctrl Pts',(-25.2919408702547,-12.8441219721555,
114.607119085205)) ;
#177917=CARTESIAN_POINT('Ctrl Pts',(-25.3657447135089,-12.8441219706321,
114.582888043014)) ;
#177918=CARTESIAN_POINT('Ctrl Pts',(-25.4395485567631,-12.8441219691087,
114.558657000823)) ;
#177919=CARTESIAN_POINT('Ctrl Pts',(-25.4188861853407,-12.8812078446008,
114.495722751362)) ;
#177920=CARTESIAN_POINT('Ctrl Pts',(-25.3535678038264,-12.6502697095916,
114.332121264411)) ;
#177921=CARTESIAN_POINT('Ctrl Pts',(-25.336704301178,-12.7035365652379,
114.280757756318)) ;
#177922=CARTESIAN_POINT('Ctrl Pts',(-25.2629004584182,-12.7035365674139,
114.304988800015)) ;
#177923=CARTESIAN_POINT('Ctrl Pts',(-25.1890966156585,-12.7035365695899,
114.329219843711)) ;
#177924=CARTESIAN_POINT('Ctrl Pts',(-25.2059601183069,-12.6502697139436,
114.380583351805)) ;
#177925=CARTESIAN_POINT('Ctrl Pts',(-25.2228236209554,-12.5970028582972,
114.431946859898)) ;
#177926=CARTESIAN_POINT('Ctrl Pts',(-25.2966274637151,-12.5970028561212,
114.407715816201)) ;
#177927=CARTESIAN_POINT('Ctrl Pts',(-25.3704313064749,-12.5970028539452,
114.383484772504)) ;
#177928=CARTESIAN_POINT('Ctrl Pts',(-25.3535678038264,-12.6502697095916,
114.332121264411)) ;
#177929=CARTESIAN_POINT('Ctrl Pts',(-25.271268624716,-12.4736381112203,
114.116796974903)) ;
#177930=CARTESIAN_POINT('Ctrl Pts',(-25.2593955331649,-12.5393175291298,
114.080633453818)) ;
#177931=CARTESIAN_POINT('Ctrl Pts',(-25.1855916906662,-12.5393175306857,
114.10486449831)) ;
#177932=CARTESIAN_POINT('Ctrl Pts',(-25.1117878481675,-12.5393175322416,
114.129095542802)) ;
#177933=CARTESIAN_POINT('Ctrl Pts',(-25.1236609397186,-12.473638114332,
114.165259063887)) ;
#177934=CARTESIAN_POINT('Ctrl Pts',(-25.1355340312698,-12.4079586964224,
114.201422584972)) ;
#177935=CARTESIAN_POINT('Ctrl Pts',(-25.2093378737685,-12.4079586948666,
114.17719154048)) ;
#177936=CARTESIAN_POINT('Ctrl Pts',(-25.2831417162671,-12.4079586933107,
114.152960495988)) ;
#177937=CARTESIAN_POINT('Ctrl Pts',(-25.271268624716,-12.4736381112203,
114.116796974903)) ;
#177938=CARTESIAN_POINT('Ctrl Pts',(-25.1760059663422,-12.3636957343507,
113.862315910691)) ;
#177939=CARTESIAN_POINT('Ctrl Pts',(-25.17002920577,-12.4371496799271,113.844111662346)) ;
#177940=CARTESIAN_POINT('Ctrl Pts',(-25.0962253625595,-12.4371496797509,
113.86834270467)) ;
#177941=CARTESIAN_POINT('Ctrl Pts',(-25.0224215193491,-12.4371496795748,
113.892573746994)) ;
#177942=CARTESIAN_POINT('Ctrl Pts',(-25.0283982799213,-12.3636957339984,
113.910777995339)) ;
#177943=CARTESIAN_POINT('Ctrl Pts',(-25.0343750404935,-12.290241788422,
113.928982243684)) ;
#177944=CARTESIAN_POINT('Ctrl Pts',(-25.1081788837039,-12.2902417885981,
113.90475120136)) ;
#177945=CARTESIAN_POINT('Ctrl Pts',(-25.1819827269144,-12.2902417887743,
113.880520159036)) ;
#177946=CARTESIAN_POINT('Ctrl Pts',(-25.1760059663422,-12.3636957343507,
113.862315910691)) ;
#177947=CARTESIAN_POINT('Ctrl Pts',(-25.0755208022999,-12.3303161657527,
113.59162885322)) ;
#177948=CARTESIAN_POINT('Ctrl Pts',(-25.0758197046939,-12.4062080741742,
113.592539261621)) ;
#177949=CARTESIAN_POINT('Ctrl Pts',(-25.0020158602591,-12.4062080738796,
113.616770300216)) ;
#177950=CARTESIAN_POINT('Ctrl Pts',(-24.9282120158242,-12.406208073585,
113.64100133881)) ;
#177951=CARTESIAN_POINT('Ctrl Pts',(-24.9279131134302,-12.3303161651636,
113.64009093041)) ;
#177952=CARTESIAN_POINT('Ctrl Pts',(-24.9276142110362,-12.2544242567421,
113.639180522009)) ;
#177953=CARTESIAN_POINT('Ctrl Pts',(-25.0014180554711,-12.2544242570367,
113.614949483414)) ;
#177954=CARTESIAN_POINT('Ctrl Pts',(-25.0752218999059,-12.2544242573313,
113.590718444819)) ;
#177955=CARTESIAN_POINT('Ctrl Pts',(-25.0755208022999,-12.3303161657527,
113.59162885322)) ;
#177956=CARTESIAN_POINT('Ctrl Pts',(-24.975387420301,-12.3741418831008,
113.322042926048)) ;
#177957=CARTESIAN_POINT('Ctrl Pts',(-24.9819458583715,-12.4470842325009,
113.342018870052)) ;
#177958=CARTESIAN_POINT('Ctrl Pts',(-24.90814201245,-12.447084234237,113.366249904119)) ;
#177959=CARTESIAN_POINT('Ctrl Pts',(-24.8343381665285,-12.4470842359731,
113.390480938186)) ;
#177960=CARTESIAN_POINT('Ctrl Pts',(-24.827779728458,-12.374141886573,113.370504994182)) ;
#177961=CARTESIAN_POINT('Ctrl Pts',(-24.8212212903875,-12.3011995371729,
113.350529050178)) ;
#177962=CARTESIAN_POINT('Ctrl Pts',(-24.895025136309,-12.3011995354367,
113.326298016111)) ;
#177963=CARTESIAN_POINT('Ctrl Pts',(-24.9688289822304,-12.3011995337006,
113.302066982044)) ;
#177964=CARTESIAN_POINT('Ctrl Pts',(-24.975387420301,-12.3741418831008,
113.322042926048)) ;
#177965=CARTESIAN_POINT('Ctrl Pts',(-24.8815379026335,-12.4937241519796,
113.071825125992)) ;
#177966=CARTESIAN_POINT('Ctrl Pts',(-24.893921544422,-12.5584232360499,
113.109543700474)) ;
#177967=CARTESIAN_POINT('Ctrl Pts',(-24.8201176966158,-12.5584232440279,
113.1337747288)) ;
#177968=CARTESIAN_POINT('Ctrl Pts',(-24.7463138488095,-12.558423252006,
113.158005757126)) ;
#177969=CARTESIAN_POINT('Ctrl Pts',(-24.7339302070211,-12.4937241679357,
113.120287182645)) ;
#177970=CARTESIAN_POINT('Ctrl Pts',(-24.7215465652326,-12.4290250838654,
113.082568608163)) ;
#177971=CARTESIAN_POINT('Ctrl Pts',(-24.7953504130388,-12.4290250758873,
113.058337579837)) ;
#177972=CARTESIAN_POINT('Ctrl Pts',(-24.869154260845,-12.4290250679093,
113.034106551511)) ;
#177973=CARTESIAN_POINT('Ctrl Pts',(-24.8815379026335,-12.4937241519796,
113.071825125992)) ;
#177974=CARTESIAN_POINT('Ctrl Pts',(-24.8012449463837,-12.6783961032596,
112.862605193765)) ;
#177975=CARTESIAN_POINT('Ctrl Pts',(-24.8185213903701,-12.7302945007164,
112.915226454164)) ;
#177976=CARTESIAN_POINT('Ctrl Pts',(-24.7447175419959,-12.7302945169849,
112.93945748076)) ;
#177977=CARTESIAN_POINT('Ctrl Pts',(-24.6709136936216,-12.7302945332533,
112.963688507356)) ;
#177978=CARTESIAN_POINT('Ctrl Pts',(-24.6536372496352,-12.6783961357965,
112.911067246957)) ;
#177979=CARTESIAN_POINT('Ctrl Pts',(-24.6363608056488,-12.6264977383397,
112.858445986558)) ;
#177980=CARTESIAN_POINT('Ctrl Pts',(-24.7101646540231,-12.6264977220713,
112.834214959962)) ;
#177981=CARTESIAN_POINT('Ctrl Pts',(-24.7839685023973,-12.6264977058028,
112.809983933366)) ;
#177982=CARTESIAN_POINT('Ctrl Pts',(-24.8012449463837,-12.6783961032596,
112.862605193765)) ;
#177983=CARTESIAN_POINT('Ctrl Pts',(-24.738447605087,-12.9163766433386,
112.706791373276)) ;
#177984=CARTESIAN_POINT('Ctrl Pts',(-24.7593999334311,-12.951734042377,
112.770608784171)) ;
#177985=CARTESIAN_POINT('Ctrl Pts',(-24.6855960853926,-12.9517340693484,
112.79483981179)) ;
#177986=CARTESIAN_POINT('Ctrl Pts',(-24.611792237354,-12.9517340963197,
112.819070839409)) ;
#177987=CARTESIAN_POINT('Ctrl Pts',(-24.5908399090099,-12.9163766972813,
112.755253428513)) ;
#177988=CARTESIAN_POINT('Ctrl Pts',(-24.5698875806658,-12.8810192982428,
112.691436017618)) ;
#177989=CARTESIAN_POINT('Ctrl Pts',(-24.6436914287043,-12.8810192712715,
112.667204989999)) ;
#177990=CARTESIAN_POINT('Ctrl Pts',(-24.7174952767428,-12.8810192443002,
112.642973962381)) ;
#177991=CARTESIAN_POINT('Ctrl Pts',(-24.738447605087,-12.9163766433386,
112.706791373276)) ;
#177992=CARTESIAN_POINT('Ctrl Pts',(-24.697217131185,-13.1903758945546,
112.616669578636)) ;
#177993=CARTESIAN_POINT('Ctrl Pts',(-24.720344718258,-13.2066536724704,
112.687112476478)) ;
#177994=CARTESIAN_POINT('Ctrl Pts',(-24.6465408720429,-13.206653710727,
112.711343509651)) ;
#177995=CARTESIAN_POINT('Ctrl Pts',(-24.5727370258278,-13.2066537489837,
112.735574542823)) ;
#177996=CARTESIAN_POINT('Ctrl Pts',(-24.5496094387548,-13.1903759710679,
112.66513164498)) ;
#177997=CARTESIAN_POINT('Ctrl Pts',(-24.5264818516818,-13.1740981931521,
112.594688747138)) ;
#177998=CARTESIAN_POINT('Ctrl Pts',(-24.6002856978969,-13.1740981548955,
112.570457713965)) ;
#177999=CARTESIAN_POINT('Ctrl Pts',(-24.674089544112,-13.1740981166388,
112.546226680793)) ;
#178000=CARTESIAN_POINT('Ctrl Pts',(-24.697217131185,-13.1903758945546,
112.616669578636)) ;
#178001=CARTESIAN_POINT('Ctrl Pts',(-24.679735225327,-13.481432819081,112.598974089601)) ;
#178002=CARTESIAN_POINT('Ctrl Pts',(-24.7033812444506,-13.4774126955136,
112.670996047636)) ;
#178003=CARTESIAN_POINT('Ctrl Pts',(-24.62957740167,-13.4774127443564,112.695227091269)) ;
#178004=CARTESIAN_POINT('Ctrl Pts',(-24.5557735588893,-13.4774127931991,
112.719458134902)) ;
#178005=CARTESIAN_POINT('Ctrl Pts',(-24.5321275397657,-13.4814329167664,
112.647436176867)) ;
#178006=CARTESIAN_POINT('Ctrl Pts',(-24.5084815206421,-13.4854530403338,
112.575414218832)) ;
#178007=CARTESIAN_POINT('Ctrl Pts',(-24.5822853634227,-13.4854529914911,
112.551183175199)) ;
#178008=CARTESIAN_POINT('Ctrl Pts',(-24.6560892062034,-13.4854529426483,
112.526952131566)) ;
#178009=CARTESIAN_POINT('Ctrl Pts',(-24.679735225327,-13.481432819081,112.598974089601)) ;
#178010=CARTESIAN_POINT('Ctrl Pts',(-24.6866566649467,-13.7673558416161,
112.655538950219)) ;
#178011=CARTESIAN_POINT('Ctrl Pts',(-24.709119400258,-13.7433670881258,
112.723956816513)) ;
#178012=CARTESIAN_POINT('Ctrl Pts',(-24.6353155624356,-13.7433671429839,
112.748187875248)) ;
#178013=CARTESIAN_POINT('Ctrl Pts',(-24.5615117246133,-13.7433671978421,
112.772418933983)) ;
#178014=CARTESIAN_POINT('Ctrl Pts',(-24.5390489893019,-13.7673559513324,
112.704001067689)) ;
#178015=CARTESIAN_POINT('Ctrl Pts',(-24.5165862539907,-13.7913447048227,
112.635583201395)) ;
#178016=CARTESIAN_POINT('Ctrl Pts',(-24.590390091813,-13.7913446499646,
112.61135214266)) ;
#178017=CARTESIAN_POINT('Ctrl Pts',(-24.6641939296354,-13.7913445951064,
112.587121083925)) ;
#178018=CARTESIAN_POINT('Ctrl Pts',(-24.6866566649467,-13.7673558416161,
112.655538950219)) ;
#178019=CARTESIAN_POINT('Ctrl Pts',(-24.7163960105244,-14.0271101613543,
112.781439555252)) ;
#178020=CARTESIAN_POINT('Ctrl Pts',(-24.7360839175633,-13.9849513065541,
112.84140574221)) ;
#178021=CARTESIAN_POINT('Ctrl Pts',(-24.6622800853002,-13.9849513605373,
112.865636817878)) ;
#178022=CARTESIAN_POINT('Ctrl Pts',(-24.5884762530371,-13.9849514145205,
112.889867893545)) ;
#178023=CARTESIAN_POINT('Ctrl Pts',(-24.5687883459981,-14.0271102693206,
112.829901706588)) ;
#178024=CARTESIAN_POINT('Ctrl Pts',(-24.5491004389591,-14.0692691241208,
112.769935519631)) ;
#178025=CARTESIAN_POINT('Ctrl Pts',(-24.6229042712222,-14.0692690701376,
112.745704443963)) ;
#178026=CARTESIAN_POINT('Ctrl Pts',(-24.6967081034854,-14.0692690161544,
112.721473368295)) ;
#178027=CARTESIAN_POINT('Ctrl Pts',(-24.7163960105244,-14.0271101613543,
112.781439555252)) ;
#178028=CARTESIAN_POINT('Ctrl Pts',(-24.7663270399,-14.2445027860115,112.968989653976)) ;
#178029=CARTESIAN_POINT('Ctrl Pts',(-24.7818234876689,-14.187105106811,
113.016189332129)) ;
#178030=CARTESIAN_POINT('Ctrl Pts',(-24.7080196613805,-14.1871051547693,
113.040420425995)) ;
#178031=CARTESIAN_POINT('Ctrl Pts',(-24.6342158350921,-14.1871052027276,
113.064651519861)) ;
#178032=CARTESIAN_POINT('Ctrl Pts',(-24.6187193873233,-14.244502881928,
113.017451841708)) ;
#178033=CARTESIAN_POINT('Ctrl Pts',(-24.6032229395544,-14.3019005611285,
112.970252163555)) ;
#178034=CARTESIAN_POINT('Ctrl Pts',(-24.6770267658428,-14.3019005131702,
112.946021069689)) ;
#178035=CARTESIAN_POINT('Ctrl Pts',(-24.7508305921312,-14.3019004652119,
112.921789975823)) ;
#178036=CARTESIAN_POINT('Ctrl Pts',(-24.7663270399,-14.2445027860115,112.968989653976)) ;
#178037=CARTESIAN_POINT('Ctrl Pts',(-24.8322750811479,-14.4028029107363,
113.205401926826)) ;
#178038=CARTESIAN_POINT('Ctrl Pts',(-24.8424542618704,-14.3342697574314,
113.236406067336)) ;
#178039=CARTESIAN_POINT('Ctrl Pts',(-24.7686504412644,-14.3342697924112,
113.260637178509)) ;
#178040=CARTESIAN_POINT('Ctrl Pts',(-24.6948466206583,-14.334269827391,
113.284868289682)) ;
#178041=CARTESIAN_POINT('Ctrl Pts',(-24.6846674399358,-14.402802980696,
113.253864149172)) ;
#178042=CARTESIAN_POINT('Ctrl Pts',(-24.6744882592133,-14.471336134001,
113.222860008663)) ;
#178043=CARTESIAN_POINT('Ctrl Pts',(-24.7482920798194,-14.4713360990211,
113.198628897489)) ;
#178044=CARTESIAN_POINT('Ctrl Pts',(-24.8220959004254,-14.4713360640413,
113.174397786316)) ;
#178045=CARTESIAN_POINT('Ctrl Pts',(-24.8322750811479,-14.4028029107363,
113.205401926826)) ;
#178046=CARTESIAN_POINT('Ctrl Pts',(-24.9082113685337,-14.4900131921161,
113.472067220855)) ;
#178047=CARTESIAN_POINT('Ctrl Pts',(-24.9123716787017,-14.4152919696491,
113.484738852679)) ;
#178048=CARTESIAN_POINT('Ctrl Pts',(-24.8385678620488,-14.4152919849729,
113.508969975893)) ;
#178049=CARTESIAN_POINT('Ctrl Pts',(-24.7647640453958,-14.4152920002968,
113.533201099107)) ;
#178050=CARTESIAN_POINT('Ctrl Pts',(-24.7606037352279,-14.4900132227638,
113.520529467283)) ;
#178051=CARTESIAN_POINT('Ctrl Pts',(-24.7564434250599,-14.5647344452309,
113.507857835459)) ;
#178052=CARTESIAN_POINT('Ctrl Pts',(-24.8302472417128,-14.5647344299071,
113.483626712245)) ;
#178053=CARTESIAN_POINT('Ctrl Pts',(-24.9040510583658,-14.5647344145832,
113.459395589031)) ;
#178054=CARTESIAN_POINT('Ctrl Pts',(-24.9082113685337,-14.4900131921161,
113.472067220855)) ;
#178055=CARTESIAN_POINT('Ctrl Pts',(-24.9884934184206,-14.5009049303826,
113.752069619527)) ;
#178056=CARTESIAN_POINT('Ctrl Pts',(-24.9863207377421,-14.4253144760394,
113.745451982938)) ;
#178057=CARTESIAN_POINT('Ctrl Pts',(-24.9125169233169,-14.4253144674804,
113.769683112938)) ;
#178058=CARTESIAN_POINT('Ctrl Pts',(-24.8387131088918,-14.4253144589214,
113.793914242937)) ;
#178059=CARTESIAN_POINT('Ctrl Pts',(-24.8408857895702,-14.5009049132646,
113.800531879526)) ;
#178060=CARTESIAN_POINT('Ctrl Pts',(-24.8430584702487,-14.5764953676079,
113.807149516115)) ;
#178061=CARTESIAN_POINT('Ctrl Pts',(-24.9168622846738,-14.5764953761669,
113.782918386116)) ;
#178062=CARTESIAN_POINT('Ctrl Pts',(-24.990666099099,-14.5764953847259,
113.758687256117)) ;
#178063=CARTESIAN_POINT('Ctrl Pts',(-24.9884934184206,-14.5009049303826,
113.752069619527)) ;
#178064=CARTESIAN_POINT('Ctrl Pts',(-25.0666037768646,-14.4337694493022,
114.025547084295)) ;
#178065=CARTESIAN_POINT('Ctrl Pts',(-25.0582386564678,-14.3627554397417,
114.000068275361)) ;
#178066=CARTESIAN_POINT('Ctrl Pts',(-24.9844348419182,-14.3627554046461,
114.024299404982)) ;
#178067=CARTESIAN_POINT('Ctrl Pts',(-24.9106310273687,-14.3627553695504,
114.048530534602)) ;
#178068=CARTESIAN_POINT('Ctrl Pts',(-24.9189961477656,-14.4337693791109,
114.074009343536)) ;
#178069=CARTESIAN_POINT('Ctrl Pts',(-24.9273612681624,-14.5047833886713,
114.09948815247)) ;
#178070=CARTESIAN_POINT('Ctrl Pts',(-25.0011650827119,-14.504783423767,
114.075257022849)) ;
#178071=CARTESIAN_POINT('Ctrl Pts',(-25.0749688972614,-14.5047834588626,
114.051025893229)) ;
#178072=CARTESIAN_POINT('Ctrl Pts',(-25.0666037768646,-14.4337694493022,
114.025547084295)) ;
#178073=CARTESIAN_POINT('Ctrl Pts',(-25.1357889459536,-14.2939322119372,
114.271744953977)) ;
#178074=CARTESIAN_POINT('Ctrl Pts',(-25.1218473907092,-14.232577073239,
114.229281224174)) ;
#178075=CARTESIAN_POINT('Ctrl Pts',(-25.0480435732121,-14.2325770123608,
114.253512344817)) ;
#178076=CARTESIAN_POINT('Ctrl Pts',(-24.9742397557151,-14.2325769514826,
114.27774346546)) ;
#178077=CARTESIAN_POINT('Ctrl Pts',(-24.9881813109595,-14.2939320901808,
114.320207195263)) ;
#178078=CARTESIAN_POINT('Ctrl Pts',(-25.0021228662039,-14.3552872288789,
114.362670925066)) ;
#178079=CARTESIAN_POINT('Ctrl Pts',(-25.075926683701,-14.3552872897571,
114.338439804423)) ;
#178080=CARTESIAN_POINT('Ctrl Pts',(-25.149730501198,-14.3552873506354,
114.31420868378)) ;
#178081=CARTESIAN_POINT('Ctrl Pts',(-25.1357889459536,-14.2939322119372,
114.271744953977)) ;
#178082=CARTESIAN_POINT('Ctrl Pts',(-25.1905524181362,-14.0911613446941,
114.474041191823)) ;
#178083=CARTESIAN_POINT('Ctrl Pts',(-25.1720325424193,-14.0438726639187,
114.417632636512)) ;
#178084=CARTESIAN_POINT('Ctrl Pts',(-25.0982287195,-14.0438725807802,114.44186374064)) ;
#178085=CARTESIAN_POINT('Ctrl Pts',(-25.0244248965808,-14.0438724976418,
114.466094844767)) ;
#178086=CARTESIAN_POINT('Ctrl Pts',(-25.0429447722977,-14.0911611784172,
114.522503400078)) ;
#178087=CARTESIAN_POINT('Ctrl Pts',(-25.0614646480147,-14.1384498591927,
114.578911955389)) ;
#178088=CARTESIAN_POINT('Ctrl Pts',(-25.1352684709339,-14.1384499423311,
114.554680851261)) ;
#178089=CARTESIAN_POINT('Ctrl Pts',(-25.2090722938532,-14.1384500254695,
114.530449747134)) ;
#178090=CARTESIAN_POINT('Ctrl Pts',(-25.1905524181362,-14.0911613446941,
114.474041191823)) ;
#178091=CARTESIAN_POINT('Ctrl Pts',(-25.2261345436437,-13.8412394795533,
114.617769466887)) ;
#178092=CARTESIAN_POINT('Ctrl Pts',(-25.2043717963994,-13.8113299936379,
114.551483648106)) ;
#178093=CARTESIAN_POINT('Ctrl Pts',(-25.1305679660697,-13.8113298944944,
114.575714729663)) ;
#178094=CARTESIAN_POINT('Ctrl Pts',(-25.0567641357399,-13.8113297953509,
114.599945811219)) ;
#178095=CARTESIAN_POINT('Ctrl Pts',(-25.0785268829842,-13.8412392812663,
114.666231629999)) ;
#178096=CARTESIAN_POINT('Ctrl Pts',(-25.1002896302284,-13.8711487671817,
114.732517448779)) ;
#178097=CARTESIAN_POINT('Ctrl Pts',(-25.1740934605582,-13.8711488663252,
114.708286367223)) ;
#178098=CARTESIAN_POINT('Ctrl Pts',(-25.2478972908879,-13.8711489654687,
114.684055285667)) ;
#178099=CARTESIAN_POINT('Ctrl Pts',(-25.2261345436437,-13.8412394795533,
114.617769466887)) ;
#178100=CARTESIAN_POINT('Ctrl Pts',(-25.2394283887284,-13.5592605313859,
114.693848406936)) ;
#178101=CARTESIAN_POINT('Ctrl Pts',(-25.2159688790662,-13.5489932748768,
114.622394523587)) ;
#178102=CARTESIAN_POINT('Ctrl Pts',(-25.1421650400429,-13.5489931673576,
114.646625578664)) ;
#178103=CARTESIAN_POINT('Ctrl Pts',(-25.0683612010196,-13.5489930598384,
114.670856633741)) ;
#178104=CARTESIAN_POINT('Ctrl Pts',(-25.0918207106818,-13.5592603163474,
114.74231051709)) ;
#178105=CARTESIAN_POINT('Ctrl Pts',(-25.1152802203441,-13.5695275728564,
114.813764400439)) ;
#178106=CARTESIAN_POINT('Ctrl Pts',(-25.1890840593674,-13.5695276803756,
114.789533345362)) ;
#178107=CARTESIAN_POINT('Ctrl Pts',(-25.2628878983907,-13.5695277878949,
114.765302290285)) ;
#178108=CARTESIAN_POINT('Ctrl Pts',(-25.2394283887284,-13.5592605313859,
114.693848406936)) ;
#178109=CARTESIAN_POINT('Ctrl Pts',(-25.2286664367361,-13.2696223387077,
114.696342245869)) ;
#178110=CARTESIAN_POINT('Ctrl Pts',(-25.2051938392726,-13.279561631404,
114.624848499195)) ;
#178111=CARTESIAN_POINT('Ctrl Pts',(-25.1313899912239,-13.2795615243136,
114.649079526783)) ;
#178112=CARTESIAN_POINT('Ctrl Pts',(-25.0575861431753,-13.2795614172232,
114.67331055437)) ;
#178113=CARTESIAN_POINT('Ctrl Pts',(-25.0810587406387,-13.2696221245269,
114.744804301044)) ;
#178114=CARTESIAN_POINT('Ctrl Pts',(-25.1045313381022,-13.2596828318306,
114.816298047717)) ;
#178115=CARTESIAN_POINT('Ctrl Pts',(-25.1783351861508,-13.259682938921,
114.79206702013)) ;
#178116=CARTESIAN_POINT('Ctrl Pts',(-25.2521390341995,-13.2596830460114,
114.767835992543)) ;
#178117=CARTESIAN_POINT('Ctrl Pts',(-25.2286664367361,-13.2696223387077,
114.696342245869)) ;
#178118=CARTESIAN_POINT('Ctrl Pts',(-25.1937485823441,-12.9883139496615,
114.625551828042)) ;
#178119=CARTESIAN_POINT('Ctrl Pts',(-25.1719429537545,-13.0179078909162,
114.559135399623)) ;
#178120=CARTESIAN_POINT('Ctrl Pts',(-25.09813909715,-13.0179077930937,114.583366401151)) ;
#178121=CARTESIAN_POINT('Ctrl Pts',(-25.0243352405455,-13.0179076952712,
114.607597402679)) ;
#178122=CARTESIAN_POINT('Ctrl Pts',(-25.0461408691352,-12.9883137540165,
114.674013831097)) ;
#178123=CARTESIAN_POINT('Ctrl Pts',(-25.0679464977248,-12.9587198127618,
114.740430259516)) ;
#178124=CARTESIAN_POINT('Ctrl Pts',(-25.1417503543293,-12.9587199105843,
114.716199257988)) ;
#178125=CARTESIAN_POINT('Ctrl Pts',(-25.2155542109338,-12.9587200084068,
114.69196825646)) ;
#178126=CARTESIAN_POINT('Ctrl Pts',(-25.1937485823441,-12.9883139496615,
114.625551828042)) ;
#178127=CARTESIAN_POINT('Ctrl Pts',(-25.1365175245661,-12.7386910562247,
114.486687971447)) ;
#178128=CARTESIAN_POINT('Ctrl Pts',(-25.1179414901368,-12.7857570655332,
114.430108365799)) ;
#178129=CARTESIAN_POINT('Ctrl Pts',(-25.0441376264093,-12.7857569845681,
114.454339345632)) ;
#178130=CARTESIAN_POINT('Ctrl Pts',(-24.9703337626818,-12.785756903603,
114.478570325464)) ;
#178131=CARTESIAN_POINT('Ctrl Pts',(-24.9889097971111,-12.7386908942945,
114.535149931112)) ;
#178132=CARTESIAN_POINT('Ctrl Pts',(-25.0074858315404,-12.691624884986,
114.59172953676)) ;
#178133=CARTESIAN_POINT('Ctrl Pts',(-25.0812896952679,-12.6916249659511,
114.567498556927)) ;
#178134=CARTESIAN_POINT('Ctrl Pts',(-25.1550935589954,-12.6916250469162,
114.543267577095)) ;
#178135=CARTESIAN_POINT('Ctrl Pts',(-25.1365175245661,-12.7386910562247,
114.486687971447)) ;
#178136=CARTESIAN_POINT('Ctrl Pts',(-25.0603010182413,-12.5375785963018,
114.290016712916)) ;
#178137=CARTESIAN_POINT('Ctrl Pts',(-25.046284425511,-12.5987561417494,
114.247324431092)) ;
#178138=CARTESIAN_POINT('Ctrl Pts',(-24.9724805567354,-12.5987560832211,
114.271555395549)) ;
#178139=CARTESIAN_POINT('Ctrl Pts',(-24.8986766879599,-12.5987560246928,
114.295786360006)) ;
#178140=CARTESIAN_POINT('Ctrl Pts',(-24.9126932806902,-12.5375784792451,
114.33847864183)) ;
#178141=CARTESIAN_POINT('Ctrl Pts',(-24.9267098734205,-12.4764009337975,
114.381170923654)) ;
#178142=CARTESIAN_POINT('Ctrl Pts',(-25.0005137421961,-12.4764009923258,
114.356939959197)) ;
#178143=CARTESIAN_POINT('Ctrl Pts',(-25.0743176109717,-12.4764010508541,
114.33270899474)) ;
#178144=CARTESIAN_POINT('Ctrl Pts',(-25.0603010182413,-12.5375785963018,
114.290016712916)) ;
#178145=CARTESIAN_POINT('Ctrl Pts',(-24.9698092052317,-12.3995778757378,
114.049856870399)) ;
#178146=CARTESIAN_POINT('Ctrl Pts',(-24.9613556898593,-12.4704821067912,
114.024108824699)) ;
#178147=CARTESIAN_POINT('Ctrl Pts',(-24.88755181852,-12.4704820736808,114.048339781347)) ;
#178148=CARTESIAN_POINT('Ctrl Pts',(-24.8137479471808,-12.4704820405704,
114.072570737995)) ;
#178149=CARTESIAN_POINT('Ctrl Pts',(-24.8222014625532,-12.399577809517,
114.098318783695)) ;
#178150=CARTESIAN_POINT('Ctrl Pts',(-24.8306549779257,-12.3286735784636,
114.124066829395)) ;
#178151=CARTESIAN_POINT('Ctrl Pts',(-24.9044588492649,-12.328673611574,
114.099835872747)) ;
#178152=CARTESIAN_POINT('Ctrl Pts',(-24.9782627206042,-12.3286736446844,
114.075604916098)) ;
#178153=CARTESIAN_POINT('Ctrl Pts',(-24.9698092052317,-12.3995778757378,
114.049856870399)) ;
#178154=CARTESIAN_POINT('Ctrl Pts',(-24.8707009033833,-12.3345174279643,
113.783475116184)) ;
#178155=CARTESIAN_POINT('Ctrl Pts',(-24.8684199267263,-12.4100708039264,
113.776527627588)) ;
#178156=CARTESIAN_POINT('Ctrl Pts',(-24.794616055458,-12.4100707963706,
113.800758584453)) ;
#178157=CARTESIAN_POINT('Ctrl Pts',(-24.7208121841896,-12.4100707888147,
113.824989541317)) ;
#178158=CARTESIAN_POINT('Ctrl Pts',(-24.7230931608466,-12.3345174128525,
113.831937029912)) ;
#178159=CARTESIAN_POINT('Ctrl Pts',(-24.7253741375036,-12.2589640368904,
113.838884518507)) ;
#178160=CARTESIAN_POINT('Ctrl Pts',(-24.7991780087719,-12.2589640444462,
113.814653561643)) ;
#178161=CARTESIAN_POINT('Ctrl Pts',(-24.8729818800402,-12.2589640520021,
113.790422604779)) ;
#178162=CARTESIAN_POINT('Ctrl Pts',(-24.8707009033833,-12.3345174279643,
113.783475116184)) ;
#178163=CARTESIAN_POINT('Ctrl Pts',(-24.7695605990675,-12.3471393395654,
113.510844338411)) ;
#178164=CARTESIAN_POINT('Ctrl Pts',(-24.773604630639,-12.4219252940087,
113.523161804465)) ;
#178165=CARTESIAN_POINT('Ctrl Pts',(-24.6998007616627,-12.4219253092695,
113.54739276831)) ;
#178166=CARTESIAN_POINT('Ctrl Pts',(-24.6259968926864,-12.4219253245303,
113.571623732156)) ;
#178167=CARTESIAN_POINT('Ctrl Pts',(-24.621952861115,-12.347139370087,113.559306266102)) ;
#178168=CARTESIAN_POINT('Ctrl Pts',(-24.6179088295436,-12.2723534156437,
113.546988800049)) ;
#178169=CARTESIAN_POINT('Ctrl Pts',(-24.6917126985198,-12.272353400383,
113.522757836203)) ;
#178170=CARTESIAN_POINT('Ctrl Pts',(-24.7655165674961,-12.2723533851222,
113.498526872358)) ;
#178171=CARTESIAN_POINT('Ctrl Pts',(-24.7695605990675,-12.3471393395654,
113.510844338411)) ;
#178172=CARTESIAN_POINT('Ctrl Pts',(-24.6727328214046,-12.4360428670471,
113.251326381663)) ;
#178173=CARTESIAN_POINT('Ctrl Pts',(-24.6828107853567,-12.5047344738789,
113.282022232306)) ;
#178174=CARTESIAN_POINT('Ctrl Pts',(-24.6090069204631,-12.5047345075886,
113.306253208587)) ;
#178175=CARTESIAN_POINT('Ctrl Pts',(-24.5352030555695,-12.5047345412984,
113.330484184867)) ;
#178176=CARTESIAN_POINT('Ctrl Pts',(-24.5251250916174,-12.4360429344666,
113.299788334225)) ;
#178177=CARTESIAN_POINT('Ctrl Pts',(-24.5150471276653,-12.3673513276347,
113.269092483582)) ;
#178178=CARTESIAN_POINT('Ctrl Pts',(-24.5888509925589,-12.367351293925,
113.244861507301)) ;
#178179=CARTESIAN_POINT('Ctrl Pts',(-24.6626548574524,-12.3673512602152,
113.220630531021)) ;
#178180=CARTESIAN_POINT('Ctrl Pts',(-24.6727328214046,-12.4360428670471,
113.251326381663)) ;
#178181=CARTESIAN_POINT('Ctrl Pts',(-24.5859199646112,-12.5962612233629,
113.022510647249)) ;
#178182=CARTESIAN_POINT('Ctrl Pts',(-24.6013377912514,-12.6538708074165,
113.069470858232)) ;
#178183=CARTESIAN_POINT('Ctrl Pts',(-24.5275339320715,-12.6538708522854,
113.093701851916)) ;
#178184=CARTESIAN_POINT('Ctrl Pts',(-24.4537300728915,-12.6538708971542,
113.117932845599)) ;
#178185=CARTESIAN_POINT('Ctrl Pts',(-24.4383122462512,-12.5962613131006,
113.070972634616)) ;
#178186=CARTESIAN_POINT('Ctrl Pts',(-24.422894419611,-12.538651729047,113.024012423633)) ;
#178187=CARTESIAN_POINT('Ctrl Pts',(-24.4966982787909,-12.5386516841781,
112.99978142995)) ;
#178188=CARTESIAN_POINT('Ctrl Pts',(-24.5705021379709,-12.5386516393093,
112.975550436267)) ;
#178189=CARTESIAN_POINT('Ctrl Pts',(-24.5859199646112,-12.5962612233629,
113.022510647249)) ;
#178190=CARTESIAN_POINT('Ctrl Pts',(-24.5156431401964,-12.8139558923281,
112.843788818509)) ;
#178191=CARTESIAN_POINT('Ctrl Pts',(-24.5352599429621,-12.8564528958473,
112.903538433404)) ;
#178192=CARTESIAN_POINT('Ctrl Pts',(-24.4614560892477,-12.8564529465473,
112.927769443735)) ;
#178193=CARTESIAN_POINT('Ctrl Pts',(-24.3876522355332,-12.8564529972473,
112.952000454065)) ;
#178194=CARTESIAN_POINT('Ctrl Pts',(-24.3680354327674,-12.8139559937281,
112.89225083917)) ;
#178195=CARTESIAN_POINT('Ctrl Pts',(-24.3484186300016,-12.7714589902089,
112.832501224274)) ;
#178196=CARTESIAN_POINT('Ctrl Pts',(-24.4222224837161,-12.7714589395089,
112.808270213944)) ;
#178197=CARTESIAN_POINT('Ctrl Pts',(-24.4960263374306,-12.7714588888089,
112.784039203613)) ;
#178198=CARTESIAN_POINT('Ctrl Pts',(-24.5156431401964,-12.8139558923281,
112.843788818509)) ;
#178199=CARTESIAN_POINT('Ctrl Pts',(-24.4652008507486,-13.0756188660845,
112.725627916536)) ;
#178200=CARTESIAN_POINT('Ctrl Pts',(-24.4876351956627,-13.0999108300579,
112.793959310375)) ;
#178201=CARTESIAN_POINT('Ctrl Pts',(-24.41383134743,-13.0999108795098,112.818190337402)) ;
#178202=CARTESIAN_POINT('Ctrl Pts',(-24.3400274991972,-13.0999109289618,
112.842421364429)) ;
#178203=CARTESIAN_POINT('Ctrl Pts',(-24.3175931542831,-13.0756189649884,
112.77408997059)) ;
#178204=CARTESIAN_POINT('Ctrl Pts',(-24.2951588093689,-13.051327001015,
112.705758576751)) ;
#178205=CARTESIAN_POINT('Ctrl Pts',(-24.3689626576016,-13.0513269515631,
112.681527549724)) ;
#178206=CARTESIAN_POINT('Ctrl Pts',(-24.4427665058344,-13.0513269021111,
112.657296522697)) ;
#178207=CARTESIAN_POINT('Ctrl Pts',(-24.4652008507486,-13.0756188660845,
112.725627916536)) ;
#178208=CARTESIAN_POINT('Ctrl Pts',(-24.4379052691479,-13.3624251132735,
112.678030789951)) ;
#178209=CARTESIAN_POINT('Ctrl Pts',(-24.4615441067479,-13.3667285784785,
112.75003087435)) ;
#178210=CARTESIAN_POINT('Ctrl Pts',(-24.3877402628968,-13.3667286208057,
112.774261914723)) ;
#178211=CARTESIAN_POINT('Ctrl Pts',(-24.3139364190456,-13.3667286631328,
112.798492955095)) ;
#178212=CARTESIAN_POINT('Ctrl Pts',(-24.2902975814456,-13.3624251979278,
112.726492870696)) ;
#178213=CARTESIAN_POINT('Ctrl Pts',(-24.2666587438456,-13.3581217327227,
112.654492786297)) ;
#178214=CARTESIAN_POINT('Ctrl Pts',(-24.3404625876968,-13.3581216903956,
112.630261745925)) ;
#178215=CARTESIAN_POINT('Ctrl Pts',(-24.4142664315479,-13.3581216480684,
112.606030705552)) ;
#178216=CARTESIAN_POINT('Ctrl Pts',(-24.4379052691479,-13.3624251132735,
112.678030789951)) ;
#178217=CARTESIAN_POINT('Ctrl Pts',(-24.4348796019806,-13.651982180129,
112.704196399724)) ;
#178218=CARTESIAN_POINT('Ctrl Pts',(-24.4580333293247,-13.6360746304586,
112.774718916708)) ;
#178219=CARTESIAN_POINT('Ctrl Pts',(-24.3842294884877,-13.6360746639262,
112.798949966261)) ;
#178220=CARTESIAN_POINT('Ctrl Pts',(-24.3104256476508,-13.6360746973937,
112.823181015814)) ;
#178221=CARTESIAN_POINT('Ctrl Pts',(-24.2872719203067,-13.651982247064,
112.752658498831)) ;
#178222=CARTESIAN_POINT('Ctrl Pts',(-24.2641181929626,-13.6678897967344,
112.682135981847)) ;
#178223=CARTESIAN_POINT('Ctrl Pts',(-24.3379220337996,-13.6678897632668,
112.657904932294)) ;
#178224=CARTESIAN_POINT('Ctrl Pts',(-24.4117258746365,-13.6678897297993,
112.63367388274)) ;
#178225=CARTESIAN_POINT('Ctrl Pts',(-24.4348796019806,-13.651982180129,
112.704196399724)) ;
#178226=CARTESIAN_POINT('Ctrl Pts',(-24.4558001085789,-13.9268736432231,
112.803588355088)) ;
#178227=CARTESIAN_POINT('Ctrl Pts',(-24.4767901805327,-13.8917477253801,
112.867520727055)) ;
#178228=CARTESIAN_POINT('Ctrl Pts',(-24.4029863408681,-13.8917477464933,
112.891751780179)) ;
#178229=CARTESIAN_POINT('Ctrl Pts',(-24.3291825012035,-13.8917477676065,
112.915982833304)) ;
#178230=CARTESIAN_POINT('Ctrl Pts',(-24.3081924292497,-13.9268736854496,
112.852050461337)) ;
#178231=CARTESIAN_POINT('Ctrl Pts',(-24.2872023572959,-13.9619996032926,
112.78811808937)) ;
#178232=CARTESIAN_POINT('Ctrl Pts',(-24.3610061969605,-13.9619995821794,
112.763887036245)) ;
#178233=CARTESIAN_POINT('Ctrl Pts',(-24.4348100366251,-13.9619995610662,
112.739655983121)) ;
#178234=CARTESIAN_POINT('Ctrl Pts',(-24.4558001085789,-13.9268736432231,
112.803588355088)) ;
#178235=CARTESIAN_POINT('Ctrl Pts',(-24.4978634283469,-14.1624927779437,
112.966970517185)) ;
#178236=CARTESIAN_POINT('Ctrl Pts',(-24.515218335732,-14.1108622061885,
113.019830764522)) ;
#178237=CARTESIAN_POINT('Ctrl Pts',(-24.4414144963545,-14.1108622190925,
113.044061818521)) ;
#178238=CARTESIAN_POINT('Ctrl Pts',(-24.367610656977,-14.1108622319965,
113.06829287252)) ;
#178239=CARTESIAN_POINT('Ctrl Pts',(-24.3502557495919,-14.1624928037518,
113.015432625182)) ;
#178240=CARTESIAN_POINT('Ctrl Pts',(-24.3329008422068,-14.214123375507,
112.962572377844)) ;
#178241=CARTESIAN_POINT('Ctrl Pts',(-24.4067046815843,-14.214123362603,
112.938341323845)) ;
#178242=CARTESIAN_POINT('Ctrl Pts',(-24.4805085209618,-14.214123349699,
112.914110269847)) ;
#178243=CARTESIAN_POINT('Ctrl Pts',(-24.4978634283469,-14.1624927779437,
112.966970517185)) ;
#178244=CARTESIAN_POINT('Ctrl Pts',(-24.5579911299017,-14.3467872124729,
113.185684905417)) ;
#178245=CARTESIAN_POINT('Ctrl Pts',(-24.5704376669349,-14.28220994504,113.223595048778)) ;
#178246=CARTESIAN_POINT('Ctrl Pts',(-24.496633826401,-14.2822099499131,
113.247826099254)) ;
#178247=CARTESIAN_POINT('Ctrl Pts',(-24.4228299858672,-14.2822099547862,
113.272057149731)) ;
#178248=CARTESIAN_POINT('Ctrl Pts',(-24.410383448834,-14.346787222219,113.23414700637)) ;
#178249=CARTESIAN_POINT('Ctrl Pts',(-24.3979369118009,-14.4113644896518,
113.19623686301)) ;
#178250=CARTESIAN_POINT('Ctrl Pts',(-24.4717407523347,-14.4113644847787,
113.172005812533)) ;
#178251=CARTESIAN_POINT('Ctrl Pts',(-24.5455445928685,-14.4113644799057,
113.147774762056)) ;
#178252=CARTESIAN_POINT('Ctrl Pts',(-24.5579911299017,-14.3467872124729,
113.185684905417)) ;
#178253=CARTESIAN_POINT('Ctrl Pts',(-24.6305363548121,-14.4636106389172,
113.442047638809)) ;
#178254=CARTESIAN_POINT('Ctrl Pts',(-24.6372034400423,-14.3907789878482,
113.462354504594)) ;
#178255=CARTESIAN_POINT('Ctrl Pts',(-24.5633995981574,-14.3907789888133,
113.486585550955)) ;
#178256=CARTESIAN_POINT('Ctrl Pts',(-24.4895957562725,-14.3907789897784,
113.510816597317)) ;
#178257=CARTESIAN_POINT('Ctrl Pts',(-24.4829286710424,-14.4636106408474,
113.490509731532)) ;
#178258=CARTESIAN_POINT('Ctrl Pts',(-24.4762615858122,-14.5364422919164,
113.470202865748)) ;
#178259=CARTESIAN_POINT('Ctrl Pts',(-24.5500654276971,-14.5364422909513,
113.445971819386)) ;
#178260=CARTESIAN_POINT('Ctrl Pts',(-24.623869269582,-14.5364422899862,
113.421740773025)) ;
#178261=CARTESIAN_POINT('Ctrl Pts',(-24.6305363548121,-14.4636106389172,
113.442047638809)) ;
#178262=CARTESIAN_POINT('Ctrl Pts',(-24.7098618797107,-14.505904926533,
113.719115599711)) ;
#178263=CARTESIAN_POINT('Ctrl Pts',(-24.710266161591,-14.4300107624531,
113.72034697708)) ;
#178264=CARTESIAN_POINT('Ctrl Pts',(-24.6364623183247,-14.430010762108,
113.744578019233)) ;
#178265=CARTESIAN_POINT('Ctrl Pts',(-24.5626584750583,-14.430010761763,
113.768809061387)) ;
#178266=CARTESIAN_POINT('Ctrl Pts',(-24.562254193178,-14.5059049258428,
113.767577684019)) ;
#178267=CARTESIAN_POINT('Ctrl Pts',(-24.5618499112976,-14.5817990899227,
113.766346306651)) ;
#178268=CARTESIAN_POINT('Ctrl Pts',(-24.635653754564,-14.5817990902678,
113.742115264497)) ;
#178269=CARTESIAN_POINT('Ctrl Pts',(-24.7094575978303,-14.5817990906128,
113.717884222343)) ;
#178270=CARTESIAN_POINT('Ctrl Pts',(-24.7098618797107,-14.505904926533,
113.719115599711)) ;
#178271=CARTESIAN_POINT('Ctrl Pts',(-24.789457567232,-14.4703681622542,
113.996992018783)) ;
#178272=CARTESIAN_POINT('Ctrl Pts',(-24.7835710155258,-14.3968421199682,
113.979062532125)) ;
#178273=CARTESIAN_POINT('Ctrl Pts',(-24.709767171351,-14.3968421204311,
114.003293571512)) ;
#178274=CARTESIAN_POINT('Ctrl Pts',(-24.6359633271762,-14.3968421208941,
114.027524610899)) ;
#178275=CARTESIAN_POINT('Ctrl Pts',(-24.6418498788825,-14.4703681631801,
114.045454097557)) ;
#178276=CARTESIAN_POINT('Ctrl Pts',(-24.6477364305887,-14.5438942054661,
114.063383584214)) ;
#178277=CARTESIAN_POINT('Ctrl Pts',(-24.7215402747635,-14.5438942050032,
114.039152544827)) ;
#178278=CARTESIAN_POINT('Ctrl Pts',(-24.7953441189382,-14.5438942045402,
114.01492150544)) ;
#178279=CARTESIAN_POINT('Ctrl Pts',(-24.789457567232,-14.4703681622542,
113.996992018783)) ;
#178280=CARTESIAN_POINT('Ctrl Pts',(-24.8630886166822,-14.359008640194,
114.256813432633)) ;
#178281=CARTESIAN_POINT('Ctrl Pts',(-24.8513157988554,-14.2931494608221,
114.220955329136)) ;
#178282=CARTESIAN_POINT('Ctrl Pts',(-24.7775119545306,-14.293149462549,
114.245186368066)) ;
#178283=CARTESIAN_POINT('Ctrl Pts',(-24.7037081102058,-14.2931494642759,
114.269417406996)) ;
#178284=CARTESIAN_POINT('Ctrl Pts',(-24.7154809280326,-14.3590086436478,
114.305275510493)) ;
#178285=CARTESIAN_POINT('Ctrl Pts',(-24.7272537458594,-14.4248678230197,
114.341133613991)) ;
#178286=CARTESIAN_POINT('Ctrl Pts',(-24.8010575901842,-14.4248678212928,
114.316902575061)) ;
#178287=CARTESIAN_POINT('Ctrl Pts',(-24.874861434509,-14.4248678195659,
114.292671536131)) ;
#178288=CARTESIAN_POINT('Ctrl Pts',(-24.8630886166822,-14.359008640194,
114.256813432633)) ;
#178289=CARTESIAN_POINT('Ctrl Pts',(-24.9242076077781,-14.1808823670753,
114.478358262173)) ;
#178290=CARTESIAN_POINT('Ctrl Pts',(-24.9074173310337,-14.1273644575797,
114.42721778835)) ;
#178291=CARTESIAN_POINT('Ctrl Pts',(-24.8336134872222,-14.1273644591981,
114.451448828844)) ;
#178292=CARTESIAN_POINT('Ctrl Pts',(-24.7598096434107,-14.1273644608165,
114.475679869337)) ;
#178293=CARTESIAN_POINT('Ctrl Pts',(-24.7765999201551,-14.1808823703121,
114.52682034316)) ;
#178294=CARTESIAN_POINT('Ctrl Pts',(-24.7933901968995,-14.2344002798077,
114.577960816982)) ;
#178295=CARTESIAN_POINT('Ctrl Pts',(-24.867194040711,-14.2344002781893,
114.553729776489)) ;
#178296=CARTESIAN_POINT('Ctrl Pts',(-24.9409978845225,-14.2344002765709,
114.529498735995)) ;
#178297=CARTESIAN_POINT('Ctrl Pts',(-24.9242076077781,-14.1808823670753,
114.478358262173)) ;
#178298=CARTESIAN_POINT('Ctrl Pts',(-24.9681883548515,-13.9476582149858,
114.647809634132)) ;
#178299=CARTESIAN_POINT('Ctrl Pts',(-24.9475678449893,-13.9103470808531,
114.585002888174)) ;
#178300=CARTESIAN_POINT('Ctrl Pts',(-24.8737640018743,-13.9103470799281,
114.609233930789)) ;
#178301=CARTESIAN_POINT('Ctrl Pts',(-24.7999601587592,-13.910347079003,
114.633464973403)) ;
#178302=CARTESIAN_POINT('Ctrl Pts',(-24.8205806686214,-13.9476582131357,
114.696271719361)) ;
#178303=CARTESIAN_POINT('Ctrl Pts',(-24.8412011784836,-13.9849693472685,
114.759078465319)) ;
#178304=CARTESIAN_POINT('Ctrl Pts',(-24.9150050215986,-13.9849693481935,
114.734847422704)) ;
#178305=CARTESIAN_POINT('Ctrl Pts',(-24.9888088647137,-13.9849693491186,
114.71061638009)) ;
#178306=CARTESIAN_POINT('Ctrl Pts',(-24.9681883548515,-13.9476582149858,
114.647809634132)) ;
#178307=CARTESIAN_POINT('Ctrl Pts',(-24.9908627448388,-13.6767014389998,
114.75232403868)) ;
#178308=CARTESIAN_POINT('Ctrl Pts',(-24.9678952272064,-13.6582555044241,
114.682368685648)) ;
#178309=CARTESIAN_POINT('Ctrl Pts',(-24.8940913843963,-13.6582554985914,
114.706599729192)) ;
#178310=CARTESIAN_POINT('Ctrl Pts',(-24.8202875415862,-13.6582554927588,
114.730830772735)) ;
#178311=CARTESIAN_POINT('Ctrl Pts',(-24.8432550592186,-13.6767014273345,
114.800786125767)) ;
#178312=CARTESIAN_POINT('Ctrl Pts',(-24.866222576851,-13.6951473619102,
114.870741478798)) ;
#178313=CARTESIAN_POINT('Ctrl Pts',(-24.9400264196611,-13.6951473677429,
114.846510435255)) ;
#178314=CARTESIAN_POINT('Ctrl Pts',(-25.0138302624712,-13.6951473735755,
114.822279391711)) ;
#178315=CARTESIAN_POINT('Ctrl Pts',(-24.9908627448388,-13.6767014389998,
114.75232403868)) ;
#178316=CARTESIAN_POINT('Ctrl Pts',(-24.9899695835005,-13.3872299120028,
114.785058404499)) ;
#178317=CARTESIAN_POINT('Ctrl Pts',(-24.966297312444,-13.3889692104813,
114.712956486132)) ;
#178318=CARTESIAN_POINT('Ctrl Pts',(-24.8924934691212,-13.388969198278,
114.737187528114)) ;
#178319=CARTESIAN_POINT('Ctrl Pts',(-24.8186896257984,-13.3889691860747,
114.761418570096)) ;
#178320=CARTESIAN_POINT('Ctrl Pts',(-24.8423618968549,-13.3872298875961,
114.833520488463)) ;
#178321=CARTESIAN_POINT('Ctrl Pts',(-24.8660341679114,-13.3854905891176,
114.90562240683)) ;
#178322=CARTESIAN_POINT('Ctrl Pts',(-24.9398380112342,-13.385490601321,
114.881391364848)) ;
#178323=CARTESIAN_POINT('Ctrl Pts',(-25.013641854557,-13.3854906135243,
114.857160322866)) ;
#178324=CARTESIAN_POINT('Ctrl Pts',(-24.9899695835005,-13.3872299120028,
114.785058404499)) ;
#178325=CARTESIAN_POINT('Ctrl Pts',(-24.9646913454561,-13.0993467868879,
114.743596413779)) ;
#178326=CARTESIAN_POINT('Ctrl Pts',(-24.9420143908797,-13.1211895488815,
114.674526068666)) ;
#178327=CARTESIAN_POINT('Ctrl Pts',(-24.8682105458579,-13.1211895296054,
114.698757105473)) ;
#178328=CARTESIAN_POINT('Ctrl Pts',(-24.7944067008361,-13.1211895103292,
114.722988142281)) ;
#178329=CARTESIAN_POINT('Ctrl Pts',(-24.8170836554125,-13.0993467483356,
114.792058487393)) ;
#178330=CARTESIAN_POINT('Ctrl Pts',(-24.8397606099889,-13.077503986342,
114.861128832505)) ;
#178331=CARTESIAN_POINT('Ctrl Pts',(-24.9135644550107,-13.0775040056182,
114.836897795698)) ;
#178332=CARTESIAN_POINT('Ctrl Pts',(-24.9873683000325,-13.0775040248944,
114.812666758891)) ;
#178333=CARTESIAN_POINT('Ctrl Pts',(-24.9646913454561,-13.0993467868879,
114.743596413779)) ;
#178334=CARTESIAN_POINT('Ctrl Pts',(-24.9162024965776,-12.8349662721153,
114.631357615901)) ;
#178335=CARTESIAN_POINT('Ctrl Pts',(-24.8961447139292,-12.8753001510476,
114.570264845728)) ;
#178336=CARTESIAN_POINT('Ctrl Pts',(-24.8223408660553,-12.8753001272113,
114.594495873848)) ;
#178337=CARTESIAN_POINT('Ctrl Pts',(-24.7485370181815,-12.875300103375,
114.618726901968)) ;
#178338=CARTESIAN_POINT('Ctrl Pts',(-24.7685948008298,-12.8349662244428,
114.679819672141)) ;
#178339=CARTESIAN_POINT('Ctrl Pts',(-24.7886525834782,-12.7946323455105,
114.740912442314)) ;
#178340=CARTESIAN_POINT('Ctrl Pts',(-24.8624564313521,-12.7946323693468,
114.716681414194)) ;
#178341=CARTESIAN_POINT('Ctrl Pts',(-24.936260279226,-12.7946323931831,
114.692450386074)) ;
#178342=CARTESIAN_POINT('Ctrl Pts',(-24.9162024965776,-12.8349662721153,
114.631357615901)) ;
#178343=CARTESIAN_POINT('Ctrl Pts',(-24.847245455251,-12.6123125745559,
114.45676980248)) ;
#178344=CARTESIAN_POINT('Ctrl Pts',(-24.8312398686168,-12.6682505751424,
114.408019367388)) ;
#178345=CARTESIAN_POINT('Ctrl Pts',(-24.7574360170475,-12.6682505503797,
114.432250384252)) ;
#178346=CARTESIAN_POINT('Ctrl Pts',(-24.6836321654782,-12.6682505256169,
114.456481401117)) ;
#178347=CARTESIAN_POINT('Ctrl Pts',(-24.6996377521124,-12.6123125250304,
114.505231836208)) ;
#178348=CARTESIAN_POINT('Ctrl Pts',(-24.7156433387467,-12.5563745244438,
114.5539822713)) ;
#178349=CARTESIAN_POINT('Ctrl Pts',(-24.7894471903159,-12.5563745492066,
114.529751254436)) ;
#178350=CARTESIAN_POINT('Ctrl Pts',(-24.8632510418852,-12.5563745739693,
114.505520237572)) ;
#178351=CARTESIAN_POINT('Ctrl Pts',(-24.847245455251,-12.6123125745559,
114.45676980248)) ;
#178352=CARTESIAN_POINT('Ctrl Pts',(-24.7618055368288,-12.447065748415,
114.232038687256)) ;
#178353=CARTESIAN_POINT('Ctrl Pts',(-24.7510075081186,-12.5146221963664,
114.199149633188)) ;
#178354=CARTESIAN_POINT('Ctrl Pts',(-24.6772036522679,-12.5146221752964,
114.223380637012)) ;
#178355=CARTESIAN_POINT('Ctrl Pts',(-24.6033997964171,-12.5146221542264,
114.247611640836)) ;
#178356=CARTESIAN_POINT('Ctrl Pts',(-24.6141978251274,-12.4470657062751,
114.280500694904)) ;
#178357=CARTESIAN_POINT('Ctrl Pts',(-24.6249958538377,-12.3795092583237,
114.313389748971)) ;
#178358=CARTESIAN_POINT('Ctrl Pts',(-24.6987997096884,-12.3795092793937,
114.289158745147)) ;
#178359=CARTESIAN_POINT('Ctrl Pts',(-24.7726035655391,-12.3795093004636,
114.264927741324)) ;
#178360=CARTESIAN_POINT('Ctrl Pts',(-24.7618055368288,-12.447065748415,
114.232038687256)) ;
#178361=CARTESIAN_POINT('Ctrl Pts',(-24.6654288827052,-12.3516677675638,
113.973971864171)) ;
#178362=CARTESIAN_POINT('Ctrl Pts',(-24.6606099935128,-12.4259824807609,
113.959294304173)) ;
#178363=CARTESIAN_POINT('Ctrl Pts',(-24.5868061336476,-12.4259824693785,
113.983525295769)) ;
#178364=CARTESIAN_POINT('Ctrl Pts',(-24.5130022737824,-12.425982457996,
114.007756287365)) ;
#178365=CARTESIAN_POINT('Ctrl Pts',(-24.5178211629749,-12.3516677447989,
114.022433847364)) ;
#178366=CARTESIAN_POINT('Ctrl Pts',(-24.5226400521673,-12.2773530316018,
114.037111407362)) ;
#178367=CARTESIAN_POINT('Ctrl Pts',(-24.5964439120325,-12.2773530429843,
114.012880415766)) ;
#178368=CARTESIAN_POINT('Ctrl Pts',(-24.6702477718977,-12.2773530543667,
113.988649424169)) ;
#178369=CARTESIAN_POINT('Ctrl Pts',(-24.6654288827052,-12.3516677675638,
113.973971864171)) ;
#178370=CARTESIAN_POINT('Ctrl Pts',(-24.5645423752006,-12.3325934792249,
113.702063110992)) ;
#178371=CARTESIAN_POINT('Ctrl Pts',(-24.566028277542,-12.4083470766961,
113.706588928583)) ;
#178372=CARTESIAN_POINT('Ctrl Pts',(-24.4922244149365,-12.4083470802209,
113.730819911833)) ;
#178373=CARTESIAN_POINT('Ctrl Pts',(-24.418420552331,-12.4083470837456,
113.755050895082)) ;
#178374=CARTESIAN_POINT('Ctrl Pts',(-24.4169346499896,-12.3325934862743,
113.750525077491)) ;
#178375=CARTESIAN_POINT('Ctrl Pts',(-24.4154487476482,-12.256839888803,
113.7459992599)) ;
#178376=CARTESIAN_POINT('Ctrl Pts',(-24.4892526102537,-12.2568398852783,
113.72176827665)) ;
#178377=CARTESIAN_POINT('Ctrl Pts',(-24.5630564728592,-12.2568398817536,
113.697537293401)) ;
#178378=CARTESIAN_POINT('Ctrl Pts',(-24.5645423752006,-12.3325934792249,
113.702063110992)) ;
#178379=CARTESIAN_POINT('Ctrl Pts',(-24.4649295396859,-12.3910918553195,
113.434163508363)) ;
#178380=CARTESIAN_POINT('Ctrl Pts',(-24.4726376582911,-12.4628709667284,
113.457641192575)) ;
#178381=CARTESIAN_POINT('Ctrl Pts',(-24.3988337941039,-12.4628709892207,
113.481872171008)) ;
#178382=CARTESIAN_POINT('Ctrl Pts',(-24.3250299299166,-12.4628710117129,
113.50610314944)) ;
#178383=CARTESIAN_POINT('Ctrl Pts',(-24.3173218113114,-12.3910919003041,
113.482625465227)) ;
#178384=CARTESIAN_POINT('Ctrl Pts',(-24.3096136927062,-12.3193127888952,
113.459147781014)) ;
#178385=CARTESIAN_POINT('Ctrl Pts',(-24.3834175568935,-12.319312766403,
113.434916802582)) ;
#178386=CARTESIAN_POINT('Ctrl Pts',(-24.4572214210807,-12.3193127439107,
113.41068582415)) ;
#178387=CARTESIAN_POINT('Ctrl Pts',(-24.4649295396859,-12.3910918553195,
113.434163508363)) ;
#178388=CARTESIAN_POINT('Ctrl Pts',(-24.37322692579,-12.5239274893633,113.190432787571)) ;
#178389=CARTESIAN_POINT('Ctrl Pts',(-24.3866124525482,-12.5865367592055,
113.231202940804)) ;
#178390=CARTESIAN_POINT('Ctrl Pts',(-24.3128085888032,-12.5865368036991,
113.255433920583)) ;
#178391=CARTESIAN_POINT('Ctrl Pts',(-24.2390047250582,-12.5865368481928,
113.279664900362)) ;
#178392=CARTESIAN_POINT('Ctrl Pts',(-24.2256191983,-12.5239275783507,113.238894747129)) ;
#178393=CARTESIAN_POINT('Ctrl Pts',(-24.2122336715418,-12.4613183085085,
113.198124593896)) ;
#178394=CARTESIAN_POINT('Ctrl Pts',(-24.2860375352869,-12.4613182640148,
113.173893614117)) ;
#178395=CARTESIAN_POINT('Ctrl Pts',(-24.3598413990319,-12.4613182195212,
113.149662634338)) ;
#178396=CARTESIAN_POINT('Ctrl Pts',(-24.37322692579,-12.5239274893633,113.190432787571)) ;
#178397=CARTESIAN_POINT('Ctrl Pts',(-24.2960054560042,-12.7192927751428,
112.990520520361)) ;
#178398=CARTESIAN_POINT('Ctrl Pts',(-24.3140714527538,-12.7683526424801,
113.045546629888)) ;
#178399=CARTESIAN_POINT('Ctrl Pts',(-24.2402675922761,-12.7683527070147,
113.069777619618)) ;
#178400=CARTESIAN_POINT('Ctrl Pts',(-24.1664637317984,-12.7683527715494,
113.094008609349)) ;
#178401=CARTESIAN_POINT('Ctrl Pts',(-24.1483977350488,-12.719292904212,
113.038982499823)) ;
#178402=CARTESIAN_POINT('Ctrl Pts',(-24.1303317382993,-12.6702330368747,
112.983956390296)) ;
#178403=CARTESIAN_POINT('Ctrl Pts',(-24.2041355987769,-12.67023297234,112.959725400566)) ;
#178404=CARTESIAN_POINT('Ctrl Pts',(-24.2779394592546,-12.6702329078054,
112.935494410835)) ;
#178405=CARTESIAN_POINT('Ctrl Pts',(-24.2960054560042,-12.7192927751428,
112.990520520361)) ;
#178406=CARTESIAN_POINT('Ctrl Pts',(-24.2369143117434,-12.9658343070978,
112.84605739491)) ;
#178407=CARTESIAN_POINT('Ctrl Pts',(-24.2583972142561,-12.9977530103242,
112.911490847945)) ;
#178408=CARTESIAN_POINT('Ctrl Pts',(-24.1845933588617,-12.9977530931819,
112.935721853159)) ;
#178409=CARTESIAN_POINT('Ctrl Pts',(-24.1107895034674,-12.9977531760396,
112.959952858372)) ;
#178410=CARTESIAN_POINT('Ctrl Pts',(-24.0893066009546,-12.9658344728131,
112.894519405337)) ;
#178411=CARTESIAN_POINT('Ctrl Pts',(-24.0678236984419,-12.9339157695866,
112.829085952303)) ;
#178412=CARTESIAN_POINT('Ctrl Pts',(-24.1416275538363,-12.9339156867289,
112.804854947089)) ;
#178413=CARTESIAN_POINT('Ctrl Pts',(-24.2154314092307,-12.9339156038712,
112.780623941875)) ;
#178414=CARTESIAN_POINT('Ctrl Pts',(-24.2369143117434,-12.9658343070978,
112.84605739491)) ;
#178415=CARTESIAN_POINT('Ctrl Pts',(-24.2000431301647,-13.2443245338218,
112.769193829695)) ;
#178416=CARTESIAN_POINT('Ctrl Pts',(-24.2233982405961,-13.2568466102088,
112.840329725867)) ;
#178417=CARTESIAN_POINT('Ctrl Pts',(-24.149594392237,-13.2568467056125,
112.864560752509)) ;
#178418=CARTESIAN_POINT('Ctrl Pts',(-24.0757905438778,-13.2568468010161,
112.888791779151)) ;
#178419=CARTESIAN_POINT('Ctrl Pts',(-24.0524354334464,-13.2443247246291,
112.817655882979)) ;
#178420=CARTESIAN_POINT('Ctrl Pts',(-24.029080323015,-13.2318026482422,
112.746519986807)) ;
#178421=CARTESIAN_POINT('Ctrl Pts',(-24.1028841713741,-13.2318025528385,
112.722288960165)) ;
#178422=CARTESIAN_POINT('Ctrl Pts',(-24.1766880197333,-13.2318024574349,
112.698057933523)) ;
#178423=CARTESIAN_POINT('Ctrl Pts',(-24.2000431301647,-13.2443245338218,
112.769193829695)) ;
#178424=CARTESIAN_POINT('Ctrl Pts',(-24.187186648989,-13.5367809605308,
112.765670474547)) ;
#178425=CARTESIAN_POINT('Ctrl Pts',(-24.210736331474,-13.5289033830346,
112.8373990057)) ;
#178426=CARTESIAN_POINT('Ctrl Pts',(-24.1369324914405,-13.5289034843527,
112.8616300577)) ;
#178427=CARTESIAN_POINT('Ctrl Pts',(-24.063128651407,-13.5289035856708,
112.885861109701)) ;
#178428=CARTESIAN_POINT('Ctrl Pts',(-24.039578968922,-13.536781163167,112.814132578548)) ;
#178429=CARTESIAN_POINT('Ctrl Pts',(-24.0160292864371,-13.5446587406632,
112.742404047396)) ;
#178430=CARTESIAN_POINT('Ctrl Pts',(-24.0898331264706,-13.5446586393451,
112.718172995395)) ;
#178431=CARTESIAN_POINT('Ctrl Pts',(-24.1636369665041,-13.544658538027,
112.693941943395)) ;
#178432=CARTESIAN_POINT('Ctrl Pts',(-24.187186648989,-13.5367809605308,
112.765670474547)) ;
#178433=CARTESIAN_POINT('Ctrl Pts',(-24.198485812454,-13.8179726435299,
112.835367593194)) ;
#178434=CARTESIAN_POINT('Ctrl Pts',(-24.2205509613614,-13.790451684124,
112.902574474547)) ;
#178435=CARTESIAN_POINT('Ctrl Pts',(-24.146747129892,-13.7904517814122,
112.926805552632)) ;
#178436=CARTESIAN_POINT('Ctrl Pts',(-24.0729432984226,-13.7904518787005,
112.951036630717)) ;
#178437=CARTESIAN_POINT('Ctrl Pts',(-24.0508781495152,-13.8179728381065,
112.883829749365)) ;
#178438=CARTESIAN_POINT('Ctrl Pts',(-24.0288130006078,-13.8454937975124,
112.816622868012)) ;
#178439=CARTESIAN_POINT('Ctrl Pts',(-24.1026168320772,-13.8454937002241,
112.792391789926)) ;
#178440=CARTESIAN_POINT('Ctrl Pts',(-24.1764206635466,-13.8454936029358,
112.768160711841)) ;
#178441=CARTESIAN_POINT('Ctrl Pts',(-24.198485812454,-13.8179726435299,
112.835367593194)) ;
#178442=CARTESIAN_POINT('Ctrl Pts',(-24.2324273152291,-14.0724753431544,
112.974281755024)) ;
#178443=CARTESIAN_POINT('Ctrl Pts',(-24.2514200932839,-14.0271455372004,
113.032130690435)) ;
#178444=CARTESIAN_POINT('Ctrl Pts',(-24.1776162699435,-14.0271456228523,
113.056361793279)) ;
#178445=CARTESIAN_POINT('Ctrl Pts',(-24.103812446603,-14.0271457085042,
113.080592896124)) ;
#178446=CARTESIAN_POINT('Ctrl Pts',(-24.0848196685482,-14.0724755144583,
113.022743960713)) ;
#178447=CARTESIAN_POINT('Ctrl Pts',(-24.0658268904934,-14.1178053204124,
112.964895025302)) ;
#178448=CARTESIAN_POINT('Ctrl Pts',(-24.1396307138339,-14.1178052347605,
112.940663922457)) ;
#178449=CARTESIAN_POINT('Ctrl Pts',(-24.2134345371743,-14.1178051491085,
112.916432819612)) ;
#178450=CARTESIAN_POINT('Ctrl Pts',(-24.2324273152291,-14.0724753431544,
112.974281755024)) ;
#178451=CARTESIAN_POINT('Ctrl Pts',(-24.2856593105687,-14.279096140685,
113.171804870744)) ;
#178452=CARTESIAN_POINT('Ctrl Pts',(-24.3002313758955,-14.2192740208291,
113.216189028444)) ;
#178453=CARTESIAN_POINT('Ctrl Pts',(-24.2264275591958,-14.219274086963,
113.240420151515)) ;
#178454=CARTESIAN_POINT('Ctrl Pts',(-24.152623742496,-14.219274153097,113.264651274587)) ;
#178455=CARTESIAN_POINT('Ctrl Pts',(-24.1380516771692,-14.2790962729529,
113.220267116886)) ;
#178456=CARTESIAN_POINT('Ctrl Pts',(-24.1234796118424,-14.3389183928089,
113.175882959185)) ;
#178457=CARTESIAN_POINT('Ctrl Pts',(-24.1972834285421,-14.3389183266749,
113.151651836114)) ;
#178458=CARTESIAN_POINT('Ctrl Pts',(-24.2710872452418,-14.3389182605409,
113.127420713043)) ;
#178459=CARTESIAN_POINT('Ctrl Pts',(-24.2856593105687,-14.279096140685,
113.171804870744)) ;
#178460=CARTESIAN_POINT('Ctrl Pts',(-24.3538376843237,-14.4248617955916,
113.414949069186)) ;
#178461=CARTESIAN_POINT('Ctrl Pts',(-24.3629371876036,-14.3547743304939,
113.442664685881)) ;
#178462=CARTESIAN_POINT('Ctrl Pts',(-24.2891333755111,-14.3547743715158,
113.466895822985)) ;
#178463=CARTESIAN_POINT('Ctrl Pts',(-24.2153295634186,-14.3547744125376,
113.491126960089)) ;
#178464=CARTESIAN_POINT('Ctrl Pts',(-24.2062300601387,-14.4248618776352,
113.463411343394)) ;
#178465=CARTESIAN_POINT('Ctrl Pts',(-24.1971305568588,-14.4949493427329,
113.435695726699)) ;
#178466=CARTESIAN_POINT('Ctrl Pts',(-24.2709343689513,-14.494949301711,
113.411464589595)) ;
#178467=CARTESIAN_POINT('Ctrl Pts',(-24.3447381810438,-14.4949492606892,
113.387233452491)) ;
#178468=CARTESIAN_POINT('Ctrl Pts',(-24.3538376843237,-14.4248617955916,
113.414949069186)) ;
#178469=CARTESIAN_POINT('Ctrl Pts',(-24.4316472822689,-14.4982152843021,
113.687591297354)) ;
#178470=CARTESIAN_POINT('Ctrl Pts',(-24.4345904335442,-14.4229018669145,
113.696555659197)) ;
#178471=CARTESIAN_POINT('Ctrl Pts',(-24.3607866232635,-14.4229018794509,
113.720786801819)) ;
#178472=CARTESIAN_POINT('Ctrl Pts',(-24.2869828129827,-14.4229018919873,
113.745017944441)) ;
#178473=CARTESIAN_POINT('Ctrl Pts',(-24.2840396617074,-14.4982153093749,
113.736053582599)) ;
#178474=CARTESIAN_POINT('Ctrl Pts',(-24.2810965104321,-14.5735287267625,
113.727089220757)) ;
#178475=CARTESIAN_POINT('Ctrl Pts',(-24.3549003207128,-14.5735287142261,
113.702858078135)) ;
#178476=CARTESIAN_POINT('Ctrl Pts',(-24.4287041309936,-14.5735287016897,
113.678626935512)) ;
#178477=CARTESIAN_POINT('Ctrl Pts',(-24.4316472822689,-14.4982152843021,
113.687591297354)) ;
#178478=CARTESIAN_POINT('Ctrl Pts',(-24.511415885813,-14.4941260357652,
113.965774681427)) ;
#178479=CARTESIAN_POINT('Ctrl Pts',(-24.5080653532222,-14.4189866403318,
113.955569497726)) ;
#178480=CARTESIAN_POINT('Ctrl Pts',(-24.4342615422946,-14.4189866245763,
113.979800638379)) ;
#178481=CARTESIAN_POINT('Ctrl Pts',(-24.360457731367,-14.4189866088209,
114.004031779031)) ;
#178482=CARTESIAN_POINT('Ctrl Pts',(-24.3638082639579,-14.4941260042543,
114.014236962732)) ;
#178483=CARTESIAN_POINT('Ctrl Pts',(-24.3671587965487,-14.5692653996877,
114.024442146433)) ;
#178484=CARTESIAN_POINT('Ctrl Pts',(-24.4409626074762,-14.5692654154432,
114.00021100578)) ;
#178485=CARTESIAN_POINT('Ctrl Pts',(-24.5147664184038,-14.5692654311986,
113.975979865128)) ;
#178486=CARTESIAN_POINT('Ctrl Pts',(-24.511415885813,-14.4941260357652,
113.965774681427)) ;
#178487=CARTESIAN_POINT('Ctrl Pts',(-24.588572932717,-14.4126782343137,
114.236447003153)) ;
#178488=CARTESIAN_POINT('Ctrl Pts',(-24.5790926098734,-14.3431123024057,
114.207571467457)) ;
#178489=CARTESIAN_POINT('Ctrl Pts',(-24.5052887953129,-14.3431122609052,
114.231802597044)) ;
#178490=CARTESIAN_POINT('Ctrl Pts',(-24.4314849807525,-14.3431122194047,
114.256033726631)) ;
#178491=CARTESIAN_POINT('Ctrl Pts',(-24.440965303596,-14.4126781513128,
114.284909262327)) ;
#178492=CARTESIAN_POINT('Ctrl Pts',(-24.4504456264396,-14.4822440832209,
114.313784798023)) ;
#178493=CARTESIAN_POINT('Ctrl Pts',(-24.5242494410001,-14.4822441247213,
114.289553668436)) ;
#178494=CARTESIAN_POINT('Ctrl Pts',(-24.5980532555605,-14.4822441662218,
114.265322538849)) ;
#178495=CARTESIAN_POINT('Ctrl Pts',(-24.588572932717,-14.4126782343137,
114.236447003153)) ;
#178496=CARTESIAN_POINT('Ctrl Pts',(-24.6553633361676,-14.2599648668114,
114.475326275185)) ;
#178497=CARTESIAN_POINT('Ctrl Pts',(-24.6404721795823,-14.2009567428221,
114.429970213033)) ;
#178498=CARTESIAN_POINT('Ctrl Pts',(-24.5666683594676,-14.2009566811552,
114.454201325703)) ;
#178499=CARTESIAN_POINT('Ctrl Pts',(-24.492864539353,-14.2009566194882,
114.478432438373)) ;
#178500=CARTESIAN_POINT('Ctrl Pts',(-24.5077556959384,-14.2599647434775,
114.523788500525)) ;
#178501=CARTESIAN_POINT('Ctrl Pts',(-24.5226468525237,-14.3189728674668,
114.569144562677)) ;
#178502=CARTESIAN_POINT('Ctrl Pts',(-24.5964506726383,-14.3189729291337,
114.544913450007)) ;
#178503=CARTESIAN_POINT('Ctrl Pts',(-24.670254492753,-14.3189729908007,
114.520682337336)) ;
#178504=CARTESIAN_POINT('Ctrl Pts',(-24.6553633361676,-14.2599648668114,
114.475326275185)) ;
#178505=CARTESIAN_POINT('Ctrl Pts',(-24.7066777082595,-14.0478524029628,
114.666975267341)) ;
#178506=CARTESIAN_POINT('Ctrl Pts',(-24.6874500195782,-14.0035651769701,
114.608410828212)) ;
#178507=CARTESIAN_POINT('Ctrl Pts',(-24.6136461926996,-14.0035651015323,
114.63264192028)) ;
#178508=CARTESIAN_POINT('Ctrl Pts',(-24.5398423658211,-14.0035650260945,
114.656873012349)) ;
#178509=CARTESIAN_POINT('Ctrl Pts',(-24.5590700545024,-14.0478522520872,
114.715437451478)) ;
#178510=CARTESIAN_POINT('Ctrl Pts',(-24.5782977431838,-14.0921394780799,
114.774001890607)) ;
#178511=CARTESIAN_POINT('Ctrl Pts',(-24.6521015700623,-14.0921395535177,
114.749770798538)) ;
#178512=CARTESIAN_POINT('Ctrl Pts',(-24.7259053969409,-14.0921396289556,
114.72553970647)) ;
#178513=CARTESIAN_POINT('Ctrl Pts',(-24.7066777082595,-14.0478524029628,
114.666975267341)) ;
#178514=CARTESIAN_POINT('Ctrl Pts',(-24.7383886959719,-13.7904112840523,
114.79898244504)) ;
#178515=CARTESIAN_POINT('Ctrl Pts',(-24.7161851481836,-13.764031497392,
114.731354019336)) ;
#178516=CARTESIAN_POINT('Ctrl Pts',(-24.6423813137988,-13.7640314159743,
114.755585088541)) ;
#178517=CARTESIAN_POINT('Ctrl Pts',(-24.5685774794139,-13.7640313345566,
114.779816157747)) ;
#178518=CARTESIAN_POINT('Ctrl Pts',(-24.5907810272022,-13.7904111212169,
114.84744458345)) ;
#178519=CARTESIAN_POINT('Ctrl Pts',(-24.6129845749905,-13.8167909078772,
114.915073009154)) ;
#178520=CARTESIAN_POINT('Ctrl Pts',(-24.6867884093753,-13.8167909892949,
114.890841939949)) ;
#178521=CARTESIAN_POINT('Ctrl Pts',(-24.7605922437602,-13.8167910707126,
114.866610870743)) ;
#178522=CARTESIAN_POINT('Ctrl Pts',(-24.7383886959719,-13.7904112840523,
114.79898244504)) ;
#178523=CARTESIAN_POINT('Ctrl Pts',(-24.7472587412919,-13.5044552055669,
114.861642887694)) ;
#178524=CARTESIAN_POINT('Ctrl Pts',(-24.7236646551396,-13.4980004286212,
114.789779106659)) ;
#178525=CARTESIAN_POINT('Ctrl Pts',(-24.6498608134184,-13.498000350832,
114.814010153519)) ;
#178526=CARTESIAN_POINT('Ctrl Pts',(-24.5760569716972,-13.4980002730428,
114.838241200379)) ;
#178527=CARTESIAN_POINT('Ctrl Pts',(-24.5996510578494,-13.5044550499884,
114.910104981414)) ;
#178528=CARTESIAN_POINT('Ctrl Pts',(-24.6232451440017,-13.5109098269341,
114.981968762449)) ;
#178529=CARTESIAN_POINT('Ctrl Pts',(-24.6970489857229,-13.5109099047233,
114.957737715589)) ;
#178530=CARTESIAN_POINT('Ctrl Pts',(-24.7708528274441,-13.5109099825126,
114.933506668729)) ;
#178531=CARTESIAN_POINT('Ctrl Pts',(-24.7472587412919,-13.5044552055669,
114.861642887694)) ;
#178532=CARTESIAN_POINT('Ctrl Pts',(-24.7317360628477,-13.2137879040768,
114.849818087154)) ;
#178533=CARTESIAN_POINT('Ctrl Pts',(-24.708456421361,-13.227617723032,114.778912053983)) ;
#178534=CARTESIAN_POINT('Ctrl Pts',(-24.6346525736394,-13.2276176541368,
114.803143082567)) ;
#178535=CARTESIAN_POINT('Ctrl Pts',(-24.5608487259178,-13.2276175852417,
114.827374111151)) ;
#178536=CARTESIAN_POINT('Ctrl Pts',(-24.5841283674045,-13.2137877662865,
114.898280144321)) ;
#178537=CARTESIAN_POINT('Ctrl Pts',(-24.6074080088912,-13.1999579473313,
114.969186177492)) ;
#178538=CARTESIAN_POINT('Ctrl Pts',(-24.6812118566128,-13.1999580162265,
114.944955148908)) ;
#178539=CARTESIAN_POINT('Ctrl Pts',(-24.7550157043344,-13.1999580851216,
114.920724120324)) ;
#178540=CARTESIAN_POINT('Ctrl Pts',(-24.7317360628477,-13.2137879040768,
114.849818087154)) ;
#178541=CARTESIAN_POINT('Ctrl Pts',(-24.6925768386914,-12.9385963486889,
114.765886618446)) ;
#178542=CARTESIAN_POINT('Ctrl Pts',(-24.6712648539298,-12.9716609792406,
114.700973750315)) ;
#178543=CARTESIAN_POINT('Ctrl Pts',(-24.5974610016299,-12.9716609227663,
114.725204764954)) ;
#178544=CARTESIAN_POINT('Ctrl Pts',(-24.52365714933,-12.9716608662921,114.749435779593)) ;
#178545=CARTESIAN_POINT('Ctrl Pts',(-24.5449691340916,-12.9385962357404,
114.814348647724)) ;
#178546=CARTESIAN_POINT('Ctrl Pts',(-24.5662811188531,-12.9055316051888,
114.879261515854)) ;
#178547=CARTESIAN_POINT('Ctrl Pts',(-24.640084971153,-12.905531661663,114.855030501215)) ;
#178548=CARTESIAN_POINT('Ctrl Pts',(-24.7138888234529,-12.9055317181373,
114.830799486576)) ;
#178549=CARTESIAN_POINT('Ctrl Pts',(-24.6925768386914,-12.9385963486889,
114.765886618446)) ;
#178550=CARTESIAN_POINT('Ctrl Pts',(-24.6315155721698,-12.6966955833364,
114.615366123145)) ;
#178551=CARTESIAN_POINT('Ctrl Pts',(-24.613700797823,-12.746700030026,114.561105193829)) ;
#178552=CARTESIAN_POINT('Ctrl Pts',(-24.539896942895,-12.7466999895666,
114.585336200463)) ;
#178553=CARTESIAN_POINT('Ctrl Pts',(-24.4660930879669,-12.7466999491071,
114.609567207097)) ;
#178554=CARTESIAN_POINT('Ctrl Pts',(-24.4839078623137,-12.6966955024176,
114.663828136413)) ;
#178555=CARTESIAN_POINT('Ctrl Pts',(-24.5017226366605,-12.646691055728,
114.718089065729)) ;
#178556=CARTESIAN_POINT('Ctrl Pts',(-24.5755264915885,-12.6466910961874,
114.693858059095)) ;
#178557=CARTESIAN_POINT('Ctrl Pts',(-24.6493303465166,-12.6466911366469,
114.66962705246)) ;
#178558=CARTESIAN_POINT('Ctrl Pts',(-24.6315155721698,-12.6966955833364,
114.615366123145)) ;
#178559=CARTESIAN_POINT('Ctrl Pts',(-24.5521621899109,-12.5064217313258,
114.409158146371)) ;
#178560=CARTESIAN_POINT('Ctrl Pts',(-24.5391265658637,-12.5697873341699,
114.369453737928)) ;
#178561=CARTESIAN_POINT('Ctrl Pts',(-24.4653227103417,-12.5697873098007,
114.393684742753)) ;
#178562=CARTESIAN_POINT('Ctrl Pts',(-24.3915188548197,-12.5697872854314,
114.417915747578)) ;
#178563=CARTESIAN_POINT('Ctrl Pts',(-24.4045544788668,-12.5064216825873,
114.457620156021)) ;
#178564=CARTESIAN_POINT('Ctrl Pts',(-24.417590102914,-12.4430560797432,
114.497324564464)) ;
#178565=CARTESIAN_POINT('Ctrl Pts',(-24.491393958436,-12.4430561041124,
114.473093559639)) ;
#178566=CARTESIAN_POINT('Ctrl Pts',(-24.5651978139581,-12.4430561284817,
114.448862554814)) ;
#178567=CARTESIAN_POINT('Ctrl Pts',(-24.5521621899109,-12.5064217313258,
114.409158146371)) ;
#178568=CARTESIAN_POINT('Ctrl Pts',(-24.4595930056771,-12.3814205030376,
114.162674429355)) ;
#178569=CARTESIAN_POINT('Ctrl Pts',(-24.4522670503864,-12.45361013115,114.140360750861)) ;
#178570=CARTESIAN_POINT('Ctrl Pts',(-24.3784631958779,-12.4536101207451,
114.164591758773)) ;
#178571=CARTESIAN_POINT('Ctrl Pts',(-24.3046593413694,-12.4536101103402,
114.188822766685)) ;
#178572=CARTESIAN_POINT('Ctrl Pts',(-24.3119852966601,-12.3814204822278,
114.211136445179)) ;
#178573=CARTESIAN_POINT('Ctrl Pts',(-24.3193112519507,-12.3092308541153,
114.233450123673)) ;
#178574=CARTESIAN_POINT('Ctrl Pts',(-24.3931151064593,-12.3092308645202,
114.209219115761)) ;
#178575=CARTESIAN_POINT('Ctrl Pts',(-24.4669189609677,-12.3092308749251,
114.184988107849)) ;
#178576=CARTESIAN_POINT('Ctrl Pts',(-24.4595930056771,-12.3814205030376,
114.162674429355)) ;
#178577=CARTESIAN_POINT('Ctrl Pts',(-24.3591960058421,-12.3309490204366,
113.892499417778)) ;
#178578=CARTESIAN_POINT('Ctrl Pts',(-24.3581319519906,-12.4067726596542,
113.889258480905)) ;
#178579=CARTESIAN_POINT('Ctrl Pts',(-24.2843281000817,-12.4067726592374,
113.913489496735)) ;
#178580=CARTESIAN_POINT('Ctrl Pts',(-24.2105242481727,-12.4067726588207,
113.937720512564)) ;
#178581=CARTESIAN_POINT('Ctrl Pts',(-24.2115883020242,-12.330949019603,
113.940961449438)) ;
#178582=CARTESIAN_POINT('Ctrl Pts',(-24.2126523558756,-12.2551253803854,
113.944202386311)) ;
#178583=CARTESIAN_POINT('Ctrl Pts',(-24.2864562077845,-12.2551253808022,
113.919971370481)) ;
#178584=CARTESIAN_POINT('Ctrl Pts',(-24.3602600596935,-12.255125381219,
113.895740354651)) ;
#178585=CARTESIAN_POINT('Ctrl Pts',(-24.3591960058421,-12.3309490204366,
113.892499417778)) ;
#178586=CARTESIAN_POINT('Ctrl Pts',(-24.2590492512348,-12.3579787522632,
113.62264874675)) ;
#178587=CARTESIAN_POINT('Ctrl Pts',(-24.2642481311498,-12.4320290416833,
113.638483695714)) ;
#178588=CARTESIAN_POINT('Ctrl Pts',(-24.1904442811735,-12.4320290471933,
113.66271471743)) ;
#178589=CARTESIAN_POINT('Ctrl Pts',(-24.1166404311972,-12.4320290527033,
113.686945739147)) ;
#178590=CARTESIAN_POINT('Ctrl Pts',(-24.1114415512822,-12.3579787632832,
113.671110790183)) ;
#178591=CARTESIAN_POINT('Ctrl Pts',(-24.1062426713672,-12.2839284738631,
113.655275841219)) ;
#178592=CARTESIAN_POINT('Ctrl Pts',(-24.1800465213435,-12.2839284683531,
113.631044819503)) ;
#178593=CARTESIAN_POINT('Ctrl Pts',(-24.2538503713199,-12.2839284628431,
113.606813797786)) ;
#178594=CARTESIAN_POINT('Ctrl Pts',(-24.2590492512348,-12.3579787522632,
113.62264874675)) ;
#178595=CARTESIAN_POINT('Ctrl Pts',(-24.1631094563438,-12.461461206882,
113.36607630111)) ;
#178596=CARTESIAN_POINT('Ctrl Pts',(-24.1742776481116,-12.5283982631063,
113.400092811004)) ;
#178597=CARTESIAN_POINT('Ctrl Pts',(-24.1004738012582,-12.5283982698858,
113.424323842232)) ;
#178598=CARTESIAN_POINT('Ctrl Pts',(-24.0266699544049,-12.5283982766654,
113.44855487346)) ;
#178599=CARTESIAN_POINT('Ctrl Pts',(-24.0155017626371,-12.4614612204411,
113.414538363566)) ;
#178600=CARTESIAN_POINT('Ctrl Pts',(-24.0043335708694,-12.3945241642168,
113.380521853673)) ;
#178601=CARTESIAN_POINT('Ctrl Pts',(-24.0781374177227,-12.3945241574372,
113.356290822444)) ;
#178602=CARTESIAN_POINT('Ctrl Pts',(-24.1519412645761,-12.3945241506577,
113.332059791216)) ;
#178603=CARTESIAN_POINT('Ctrl Pts',(-24.1631094563438,-12.461461206882,
113.36607630111)) ;
#178604=CARTESIAN_POINT('Ctrl Pts',(-24.0794846118896,-12.6327579824641,
113.146729045038)) ;
#178605=CARTESIAN_POINT('Ctrl Pts',(-24.0957769767799,-12.6878348099754,
113.196352959588)) ;
#178606=CARTESIAN_POINT('Ctrl Pts',(-24.0219731318251,-12.6878348153818,
113.220583996599)) ;
#178607=CARTESIAN_POINT('Ctrl Pts',(-23.9481692868703,-12.6878348207882,
113.24481503361)) ;
#178608=CARTESIAN_POINT('Ctrl Pts',(-23.9318769219801,-12.632757993277,
113.19519111906)) ;
#178609=CARTESIAN_POINT('Ctrl Pts',(-23.9155845570898,-12.5776811657657,
113.145567204509)) ;
#178610=CARTESIAN_POINT('Ctrl Pts',(-23.9893884020446,-12.5776811603593,
113.121336167498)) ;
#178611=CARTESIAN_POINT('Ctrl Pts',(-24.0631922469993,-12.5776811549529,
113.097105130487)) ;
#178612=CARTESIAN_POINT('Ctrl Pts',(-24.0794846118896,-12.6327579824641,
113.146729045038)) ;
#178613=CARTESIAN_POINT('Ctrl Pts',(-24.0122990421959,-12.8610649262646,
112.977629767465)) ;
#178614=CARTESIAN_POINT('Ctrl Pts',(-24.0325718885268,-12.9002826126032,
113.039377586343)) ;
#178615=CARTESIAN_POINT('Ctrl Pts',(-23.9587680449403,-12.9002826143644,
113.063608627522)) ;
#178616=CARTESIAN_POINT('Ctrl Pts',(-23.8849642013539,-12.9002826161256,
113.0878396687)) ;
#178617=CARTESIAN_POINT('Ctrl Pts',(-23.8646913550231,-12.861064929787,
113.026091849823)) ;
#178618=CARTESIAN_POINT('Ctrl Pts',(-23.8444185086923,-12.8218472434483,
112.964344030946)) ;
#178619=CARTESIAN_POINT('Ctrl Pts',(-23.9182223522787,-12.8218472416871,
112.940112989767)) ;
#178620=CARTESIAN_POINT('Ctrl Pts',(-23.9920261958651,-12.8218472399259,
112.915881948588)) ;
#178621=CARTESIAN_POINT('Ctrl Pts',(-24.0122990421959,-12.8610649262646,
112.977629767465)) ;
#178622=CARTESIAN_POINT('Ctrl Pts',(-23.9662485633249,-13.1282120035714,
112.872739576532)) ;
#178623=CARTESIAN_POINT('Ctrl Pts',(-23.9890352233381,-13.1488341330094,
112.942144066345)) ;
#178624=CARTESIAN_POINT('Ctrl Pts',(-23.9152313801124,-13.1488341316972,
112.966375108623)) ;
#178625=CARTESIAN_POINT('Ctrl Pts',(-23.8414275368868,-13.148834130385,
112.990606150901)) ;
#178626=CARTESIAN_POINT('Ctrl Pts',(-23.8186408768736,-13.1282120009471,
112.921201661087)) ;
#178627=CARTESIAN_POINT('Ctrl Pts',(-23.7958542168604,-13.1075898715092,
112.851797171274)) ;
#178628=CARTESIAN_POINT('Ctrl Pts',(-23.869658060086,-13.1075898728214,
112.827566128996)) ;
#178629=CARTESIAN_POINT('Ctrl Pts',(-23.9434619033117,-13.1075898741335,
112.803335086719)) ;
#178630=CARTESIAN_POINT('Ctrl Pts',(-23.9662485633249,-13.1282120035714,
112.872739576532)) ;
#178631=CARTESIAN_POINT('Ctrl Pts',(-23.9434524616525,-13.4170777357306,
112.838817161117)) ;
#178632=CARTESIAN_POINT('Ctrl Pts',(-23.9671300237859,-13.4175593372615,
112.91093519508)) ;
#178633=CARTESIAN_POINT('Ctrl Pts',(-23.8933261804059,-13.4175593339228,
112.935166236887)) ;
#178634=CARTESIAN_POINT('Ctrl Pts',(-23.8195223370259,-13.4175593305841,
112.959397278695)) ;
#178635=CARTESIAN_POINT('Ctrl Pts',(-23.7958447748924,-13.4170777290533,
112.887279244733)) ;
#178636=CARTESIAN_POINT('Ctrl Pts',(-23.772167212759,-13.4165961275224,
112.81516121077)) ;
#178637=CARTESIAN_POINT('Ctrl Pts',(-23.845971056139,-13.4165961308611,
112.790930168963)) ;
#178638=CARTESIAN_POINT('Ctrl Pts',(-23.919774899519,-13.4165961341998,
112.766699127155)) ;
#178639=CARTESIAN_POINT('Ctrl Pts',(-23.9434524616525,-13.4170777357306,
112.838817161117)) ;
#178640=CARTESIAN_POINT('Ctrl Pts',(-23.9449981053748,-13.7056413839055,
112.878978183992)) ;
#178641=CARTESIAN_POINT('Ctrl Pts',(-23.967869039491,-13.6859734009019,
112.948639359155)) ;
#178642=CARTESIAN_POINT('Ctrl Pts',(-23.8940651957832,-13.6859733981245,
112.972870399964)) ;
#178643=CARTESIAN_POINT('Ctrl Pts',(-23.8202613520754,-13.6859733953471,
112.997101440773)) ;
#178644=CARTESIAN_POINT('Ctrl Pts',(-23.7973904179592,-13.7056413783507,
112.92744026561)) ;
#178645=CARTESIAN_POINT('Ctrl Pts',(-23.7745194838429,-13.7253093613543,
112.857779090447)) ;
#178646=CARTESIAN_POINT('Ctrl Pts',(-23.8483233275508,-13.7253093641317,
112.833548049638)) ;
#178647=CARTESIAN_POINT('Ctrl Pts',(-23.9221271712586,-13.725309366909,
112.809317008829)) ;
#178648=CARTESIAN_POINT('Ctrl Pts',(-23.9449981053748,-13.7056413839055,
112.878978183992)) ;
#178649=CARTESIAN_POINT('Ctrl Pts',(-23.9701821735012,-13.9747406301587,
112.991309111019)) ;
#178650=CARTESIAN_POINT('Ctrl Pts',(-23.9905910336019,-13.9362526969778,
113.053471205922)) ;
#178651=CARTESIAN_POINT('Ctrl Pts',(-23.9167871901567,-13.9362526974253,
113.077702247531)) ;
#178652=CARTESIAN_POINT('Ctrl Pts',(-23.8429833467115,-13.9362526978728,
113.10193328914)) ;
#178653=CARTESIAN_POINT('Ctrl Pts',(-23.8225744866109,-13.9747406310537,
113.039771194237)) ;
#178654=CARTESIAN_POINT('Ctrl Pts',(-23.8021656265102,-14.0132285642346,
112.977609099335)) ;
#178655=CARTESIAN_POINT('Ctrl Pts',(-23.8759694699554,-14.0132285637871,
112.953378057726)) ;
#178656=CARTESIAN_POINT('Ctrl Pts',(-23.9497733134006,-14.0132285633396,
112.929147016116)) ;
#178657=CARTESIAN_POINT('Ctrl Pts',(-23.9701821735012,-13.9747406301587,
112.991309111019)) ;
#178658=CARTESIAN_POINT('Ctrl Pts',(-24.0160072122531,-14.201974810105,
113.166223946965)) ;
#178659=CARTESIAN_POINT('Ctrl Pts',(-24.0325147694804,-14.1475641696475,
113.216503302712)) ;
#178660=CARTESIAN_POINT('Ctrl Pts',(-23.9587109269328,-14.1475641728961,
113.240734347056)) ;
#178661=CARTESIAN_POINT('Ctrl Pts',(-23.8849070843852,-14.1475641761448,
113.264965391399)) ;
#178662=CARTESIAN_POINT('Ctrl Pts',(-23.8683995271579,-14.2019748166024,
113.214686035651)) ;
#178663=CARTESIAN_POINT('Ctrl Pts',(-23.8518919699306,-14.2563854570598,
113.164406679903)) ;
#178664=CARTESIAN_POINT('Ctrl Pts',(-23.9256958124782,-14.2563854538112,
113.14017563556)) ;
#178665=CARTESIAN_POINT('Ctrl Pts',(-23.9994996550258,-14.2563854505624,
113.115944591217)) ;
#178666=CARTESIAN_POINT('Ctrl Pts',(-24.0160072122531,-14.201974810105,
113.166223946965)) ;
#178667=CARTESIAN_POINT('Ctrl Pts',(-24.0787453413408,-14.3739130003505,
113.392766421991)) ;
#178668=CARTESIAN_POINT('Ctrl Pts',(-24.0901626436676,-14.3074175885929,
113.427541682514)) ;
#178669=CARTESIAN_POINT('Ctrl Pts',(-24.0163588028729,-14.3074175937146,
113.451772732196)) ;
#178670=CARTESIAN_POINT('Ctrl Pts',(-23.9425549620781,-14.3074175988363,
113.476003781877)) ;
#178671=CARTESIAN_POINT('Ctrl Pts',(-23.9311376597514,-14.3739130105938,
113.441228521355)) ;
#178672=CARTESIAN_POINT('Ctrl Pts',(-23.9197203574246,-14.4404084223513,
113.406453260833)) ;
#178673=CARTESIAN_POINT('Ctrl Pts',(-23.9935241982193,-14.4404084172297,
113.382222211151)) ;
#178674=CARTESIAN_POINT('Ctrl Pts',(-24.067328039014,-14.440408412108,113.357991161469)) ;
#178675=CARTESIAN_POINT('Ctrl Pts',(-24.0787453413408,-14.3739130003505,
113.392766421991)) ;
#178676=CARTESIAN_POINT('Ctrl Pts',(-24.153021958778,-14.4775305035498,
113.654416785986)) ;
#178677=CARTESIAN_POINT('Ctrl Pts',(-24.1585367352309,-14.4037037065639,
113.671213904943)) ;
#178678=CARTESIAN_POINT('Ctrl Pts',(-24.0847328966993,-14.403703711016,
113.695444961518)) ;
#178679=CARTESIAN_POINT('Ctrl Pts',(-24.0109290581677,-14.4037037154681,
113.719676018093)) ;
#178680=CARTESIAN_POINT('Ctrl Pts',(-24.0054142817148,-14.477530512454,
113.702878899137)) ;
#178681=CARTESIAN_POINT('Ctrl Pts',(-23.999899505262,-14.5513573094398,
113.686081780181)) ;
#178682=CARTESIAN_POINT('Ctrl Pts',(-24.0737033437936,-14.5513573049878,
113.661850723605)) ;
#178683=CARTESIAN_POINT('Ctrl Pts',(-24.1475071823252,-14.5513573005357,
113.63761966703)) ;
#178684=CARTESIAN_POINT('Ctrl Pts',(-24.153021958778,-14.4775305035498,
113.654416785986)) ;
#178685=CARTESIAN_POINT('Ctrl Pts',(-24.2334081776458,-14.5050608269986,
113.934939965511)) ;
#178686=CARTESIAN_POINT('Ctrl Pts',(-24.2325798290723,-14.4292041443238,
113.93241694891)) ;
#178687=CARTESIAN_POINT('Ctrl Pts',(-24.1587759937175,-14.4292041439296,
113.956648015161)) ;
#178688=CARTESIAN_POINT('Ctrl Pts',(-24.0849721583626,-14.4292041435354,
113.980879081412)) ;
#178689=CARTESIAN_POINT('Ctrl Pts',(-24.0858005069361,-14.5050608262101,
113.983402098013)) ;
#178690=CARTESIAN_POINT('Ctrl Pts',(-24.0866288555096,-14.5809175088849,
113.985925114614)) ;
#178691=CARTESIAN_POINT('Ctrl Pts',(-24.1604326908644,-14.5809175092791,
113.961694048363)) ;
#178692=CARTESIAN_POINT('Ctrl Pts',(-24.2342365262193,-14.5809175096733,
113.937462982112)) ;
#178693=CARTESIAN_POINT('Ctrl Pts',(-24.2334081776458,-14.5050608269986,
113.934939965511)) ;
#178694=CARTESIAN_POINT('Ctrl Pts',(-24.3118138425738,-14.4551363613954,
114.208959708269)) ;
#178695=CARTESIAN_POINT('Ctrl Pts',(-24.3047814448191,-14.3826564737513,
114.187540158768)) ;
#178696=CARTESIAN_POINT('Ctrl Pts',(-24.2309776109259,-14.3826564648488,
114.211771229471)) ;
#178697=CARTESIAN_POINT('Ctrl Pts',(-24.1571737770328,-14.3826564559462,
114.236002300174)) ;
#178698=CARTESIAN_POINT('Ctrl Pts',(-24.1642061747875,-14.4551363435903,
114.257421849676)) ;
#178699=CARTESIAN_POINT('Ctrl Pts',(-24.1712385725423,-14.5276162312344,
114.278841399177)) ;
#178700=CARTESIAN_POINT('Ctrl Pts',(-24.2450424064354,-14.5276162401369,
114.254610328474)) ;
#178701=CARTESIAN_POINT('Ctrl Pts',(-24.3188462403286,-14.5276162490395,
114.230379257771)) ;
#178702=CARTESIAN_POINT('Ctrl Pts',(-24.3118138425738,-14.4551363613954,
114.208959708269)) ;
#178703=CARTESIAN_POINT('Ctrl Pts',(-24.3838624730078,-14.3298705824412,
114.464102745858)) ;
#178704=CARTESIAN_POINT('Ctrl Pts',(-24.3710507387794,-14.2660313750253,
114.425080269742)) ;
#178705=CARTESIAN_POINT('Ctrl Pts',(-24.2972469066288,-14.2660313525063,
114.449311345752)) ;
#178706=CARTESIAN_POINT('Ctrl Pts',(-24.2234430744781,-14.2660313299873,
114.473542421763)) ;
#178707=CARTESIAN_POINT('Ctrl Pts',(-24.2362548087065,-14.3298705374032,
114.512564897879)) ;
#178708=CARTESIAN_POINT('Ctrl Pts',(-24.2490665429349,-14.3937097448191,
114.551587373996)) ;
#178709=CARTESIAN_POINT('Ctrl Pts',(-24.3228703750855,-14.3937097673381,
114.527356297985)) ;
#178710=CARTESIAN_POINT('Ctrl Pts',(-24.3966742072362,-14.3937097898571,
114.503125221975)) ;
#178711=CARTESIAN_POINT('Ctrl Pts',(-24.3838624730078,-14.3298705824412,
114.464102745858)) ;
#178712=CARTESIAN_POINT('Ctrl Pts',(-24.4418657884039,-14.1407879039854,
114.676048055119)) ;
#178713=CARTESIAN_POINT('Ctrl Pts',(-24.4242559427528,-14.0900585571138,
114.622411305648)) ;
#178714=CARTESIAN_POINT('Ctrl Pts',(-24.3504521097342,-14.090058520559,
114.646642379015)) ;
#178715=CARTESIAN_POINT('Ctrl Pts',(-24.2766482767156,-14.0900584840042,
114.670873452382)) ;
#178716=CARTESIAN_POINT('Ctrl Pts',(-24.2942581223667,-14.1407878308758,
114.724510201853)) ;
#178717=CARTESIAN_POINT('Ctrl Pts',(-24.3118679680179,-14.1915171777474,
114.778146951323)) ;
#178718=CARTESIAN_POINT('Ctrl Pts',(-24.3856718010364,-14.1915172143022,
114.753915877957)) ;
#178719=CARTESIAN_POINT('Ctrl Pts',(-24.459475634055,-14.191517250857,114.72968480459)) ;
#178720=CARTESIAN_POINT('Ctrl Pts',(-24.4418657884039,-14.1407879039854,
114.676048055119)) ;
#178721=CARTESIAN_POINT('Ctrl Pts',(-24.4821519623665,-13.8991517087972,
114.83424842299)) ;
#178722=CARTESIAN_POINT('Ctrl Pts',(-24.460969456234,-13.8652196589451,
114.769729925967)) ;
#178723=CARTESIAN_POINT('Ctrl Pts',(-24.3871656211141,-13.8652196069501,
114.793960992934)) ;
#178724=CARTESIAN_POINT('Ctrl Pts',(-24.3133617859942,-13.865219554955,
114.8181920599)) ;
#178725=CARTESIAN_POINT('Ctrl Pts',(-24.3345442921267,-13.8991516048072,
114.882710556924)) ;
#178726=CARTESIAN_POINT('Ctrl Pts',(-24.3557267982592,-13.9330836546593,
114.947229053947)) ;
#178727=CARTESIAN_POINT('Ctrl Pts',(-24.4295306333791,-13.9330837066543,
114.922997986981)) ;
#178728=CARTESIAN_POINT('Ctrl Pts',(-24.503334468499,-13.9330837586493,
114.898766920014)) ;
#178729=CARTESIAN_POINT('Ctrl Pts',(-24.4821519623665,-13.8991517087972,
114.83424842299)) ;
#178730=CARTESIAN_POINT('Ctrl Pts',(-24.5005313129686,-13.622377664187,
114.925775683021)) ;
#178731=CARTESIAN_POINT('Ctrl Pts',(-24.4772993502077,-13.6077202458349,
114.855014871609)) ;
#178732=CARTESIAN_POINT('Ctrl Pts',(-24.4034955109649,-13.6077201796241,
114.879245926018)) ;
#178733=CARTESIAN_POINT('Ctrl Pts',(-24.3296916717221,-13.6077201134133,
114.903476980426)) ;
#178734=CARTESIAN_POINT('Ctrl Pts',(-24.352923634483,-13.6223775317654,
114.974237791838)) ;
#178735=CARTESIAN_POINT('Ctrl Pts',(-24.3761555972439,-13.6370349501174,
115.04499860325)) ;
#178736=CARTESIAN_POINT('Ctrl Pts',(-24.4499594364868,-13.6370350163283,
115.020767548841)) ;
#178737=CARTESIAN_POINT('Ctrl Pts',(-24.5237632757296,-13.6370350825391,
114.996536494432)) ;
#178738=CARTESIAN_POINT('Ctrl Pts',(-24.5005313129686,-13.622377664187,
114.925775683021)) ;
#178739=CARTESIAN_POINT('Ctrl Pts',(-24.49501436777,-13.3324243748073,114.944342617232)) ;
#178740=CARTESIAN_POINT('Ctrl Pts',(-24.4714021470043,-13.3379896350766,
114.872423601156)) ;
#178741=CARTESIAN_POINT('Ctrl Pts',(-24.39759830194,-13.3379895606869,114.896654637833)) ;
#178742=CARTESIAN_POINT('Ctrl Pts',(-24.3237944568757,-13.3379894862972,
114.92088567451)) ;
#178743=CARTESIAN_POINT('Ctrl Pts',(-24.3474066776414,-13.3324242260279,
114.992804690587)) ;
#178744=CARTESIAN_POINT('Ctrl Pts',(-24.371018898407,-13.3268589657586,
115.064723706663)) ;
#178745=CARTESIAN_POINT('Ctrl Pts',(-24.4448227434714,-13.3268590401483,
115.040492669985)) ;
#178746=CARTESIAN_POINT('Ctrl Pts',(-24.5186265885357,-13.326859114538,
115.016261633308)) ;
#178747=CARTESIAN_POINT('Ctrl Pts',(-24.49501436777,-13.3324243748073,114.944342617232)) ;
#178748=CARTESIAN_POINT('Ctrl Pts',(-24.4653775774576,-13.0478498918573,
114.889526808152)) ;
#178749=CARTESIAN_POINT('Ctrl Pts',(-24.443066690919,-13.0732913047775,
114.821571446019)) ;
#178750=CARTESIAN_POINT('Ctrl Pts',(-24.3692628390167,-13.073291227464,
114.845802461869)) ;
#178751=CARTESIAN_POINT('Ctrl Pts',(-24.2954589871145,-13.0732911501505,
114.870033477719)) ;
#178752=CARTESIAN_POINT('Ctrl Pts',(-24.3177698736531,-13.0478497372302,
114.937988839852)) ;
#178753=CARTESIAN_POINT('Ctrl Pts',(-24.3400807601917,-13.02240832431,115.005944201984)) ;
#178754=CARTESIAN_POINT('Ctrl Pts',(-24.413884612094,-13.0224084016235,
114.981713186134)) ;
#178755=CARTESIAN_POINT('Ctrl Pts',(-24.4876884639962,-13.022408478937,
114.957482170284)) ;
#178756=CARTESIAN_POINT('Ctrl Pts',(-24.4653775774576,-13.0478498918573,
114.889526808152)) ;
#178757=CARTESIAN_POINT('Ctrl Pts',(-24.4124318331185,-12.7884262570381,
114.76392923946)) ;
#178758=CARTESIAN_POINT('Ctrl Pts',(-24.3930468030307,-12.8320168743516,
114.704885563836)) ;
#178759=CARTESIAN_POINT('Ctrl Pts',(-24.319242943509,-12.8320168006288,
114.729116556479)) ;
#178760=CARTESIAN_POINT('Ctrl Pts',(-24.2454390839874,-12.8320167269059,
114.753347549122)) ;
#178761=CARTESIAN_POINT('Ctrl Pts',(-24.2648241140752,-12.7884261095925,
114.812391224746)) ;
#178762=CARTESIAN_POINT('Ctrl Pts',(-24.284209144163,-12.744835492279,114.87143490037)) ;
#178763=CARTESIAN_POINT('Ctrl Pts',(-24.3580130036846,-12.7448355660018,
114.847203907727)) ;
#178764=CARTESIAN_POINT('Ctrl Pts',(-24.4318168632063,-12.7448356397246,
114.822972915085)) ;
#178765=CARTESIAN_POINT('Ctrl Pts',(-24.4124318331185,-12.7884262570381,
114.76392923946)) ;
#178766=CARTESIAN_POINT('Ctrl Pts',(-24.3401997969462,-12.5764203972658,
114.57925123095)) ;
#178767=CARTESIAN_POINT('Ctrl Pts',(-24.3250986174262,-12.6348758868913,
114.533255472867)) ;
#178768=CARTESIAN_POINT('Ctrl Pts',(-24.2512947512124,-12.6348758265582,
114.557486445126)) ;
#178769=CARTESIAN_POINT('Ctrl Pts',(-24.1774908849985,-12.6348757662251,
114.581717417385)) ;
#178770=CARTESIAN_POINT('Ctrl Pts',(-24.1925920645185,-12.5764202765996,
114.627713175469)) ;
#178771=CARTESIAN_POINT('Ctrl Pts',(-24.2076932440385,-12.517964786974,
114.673708933552)) ;
#178772=CARTESIAN_POINT('Ctrl Pts',(-24.2814971102523,-12.5179648473072,
114.649477961293)) ;
#178773=CARTESIAN_POINT('Ctrl Pts',(-24.3553009764662,-12.5179649076403,
114.625246989034)) ;
#178774=CARTESIAN_POINT('Ctrl Pts',(-24.3401997969462,-12.5764203972658,
114.57925123095)) ;
#178775=CARTESIAN_POINT('Ctrl Pts',(-24.2523979814976,-12.4236100991773,
114.347280755597)) ;
#178776=CARTESIAN_POINT('Ctrl Pts',(-24.2426710134567,-12.4928195575656,
114.317653978459)) ;
#178777=CARTESIAN_POINT('Ctrl Pts',(-24.1688671416776,-12.4928195167555,
114.341884933767)) ;
#178778=CARTESIAN_POINT('Ctrl Pts',(-24.0950632698985,-12.4928194759453,
114.366115889076)) ;
#178779=CARTESIAN_POINT('Ctrl Pts',(-24.1047902379394,-12.423610017557,
114.395742666214)) ;
#178780=CARTESIAN_POINT('Ctrl Pts',(-24.1145172059802,-12.3544005591686,
114.425369443353)) ;
#178781=CARTESIAN_POINT('Ctrl Pts',(-24.1883210777593,-12.3544005999788,
114.401138488044)) ;
#178782=CARTESIAN_POINT('Ctrl Pts',(-24.2621249495384,-12.354400640789,
114.376907532736)) ;
#178783=CARTESIAN_POINT('Ctrl Pts',(-24.2523979814976,-12.4236100991773,
114.347280755597)) ;
#178784=CARTESIAN_POINT('Ctrl Pts',(-24.1544007543503,-12.3419562515338,
114.084359044048)) ;
#178785=CARTESIAN_POINT('Ctrl Pts',(-24.1507654132783,-12.4169681280718,
114.073286379695)) ;
#178786=CARTESIAN_POINT('Ctrl Pts',(-24.0769615378214,-12.4169681124147,
114.097517323801)) ;
#178787=CARTESIAN_POINT('Ctrl Pts',(-24.0031576623645,-12.4169680967576,
114.121748267908)) ;
#178788=CARTESIAN_POINT('Ctrl Pts',(-24.0067930034366,-12.3419562202195,
114.132820932261)) ;
#178789=CARTESIAN_POINT('Ctrl Pts',(-24.0104283445086,-12.2669443436815,
114.143893596615)) ;
#178790=CARTESIAN_POINT('Ctrl Pts',(-24.0842322199655,-12.2669443593386,
114.119662652508)) ;
#178791=CARTESIAN_POINT('Ctrl Pts',(-24.1580360954224,-12.2669443749958,
114.095431708402)) ;
#178792=CARTESIAN_POINT('Ctrl Pts',(-24.1544007543503,-12.3419562515338,
114.084359044048)) ;
#178793=CARTESIAN_POINT('Ctrl Pts',(-24.0529879307825,-12.3379525743983,
113.810967700911)) ;
#178794=CARTESIAN_POINT('Ctrl Pts',(-24.0556930383593,-12.4133543694812,
113.819207020064)) ;
#178795=CARTESIAN_POINT('Ctrl Pts',(-23.9818891619565,-12.4133543821139,
113.843437961289)) ;
#178796=CARTESIAN_POINT('Ctrl Pts',(-23.9080852855538,-12.4133543947465,
113.867668902515)) ;
#178797=CARTESIAN_POINT('Ctrl Pts',(-23.905380177977,-12.3379525996635,
113.859429583362)) ;
#178798=CARTESIAN_POINT('Ctrl Pts',(-23.9026750704002,-12.2625508045805,
113.85119026421)) ;
#178799=CARTESIAN_POINT('Ctrl Pts',(-23.9764789468029,-12.2625507919479,
113.826959322984)) ;
#178800=CARTESIAN_POINT('Ctrl Pts',(-24.0502828232057,-12.2625507793153,
113.802728381759)) ;
#178801=CARTESIAN_POINT('Ctrl Pts',(-24.0529879307825,-12.3379525743983,
113.810967700911)) ;
#178802=CARTESIAN_POINT('Ctrl Pts',(-23.9551105454002,-12.4104778611719,
113.54810794873)) ;
#178803=CARTESIAN_POINT('Ctrl Pts',(-23.9639235340744,-12.4809266819483,
113.574950888178)) ;
#178804=CARTESIAN_POINT('Ctrl Pts',(-23.8901196595169,-12.4809267225878,
113.599181835023)) ;
#178805=CARTESIAN_POINT('Ctrl Pts',(-23.8163157849594,-12.4809267632273,
113.623412781869)) ;
#178806=CARTESIAN_POINT('Ctrl Pts',(-23.8075027962851,-12.4104779424509,
113.596569842421)) ;
#178807=CARTESIAN_POINT('Ctrl Pts',(-23.7986898076108,-12.3400291216744,
113.569726902974)) ;
#178808=CARTESIAN_POINT('Ctrl Pts',(-23.8724936821683,-12.3400290810349,
113.545495956128)) ;
#178809=CARTESIAN_POINT('Ctrl Pts',(-23.9462975567259,-12.3400290403954,
113.521265009282)) ;
#178810=CARTESIAN_POINT('Ctrl Pts',(-23.9551105454002,-12.4104778611719,
113.54810794873)) ;
#178811=CARTESIAN_POINT('Ctrl Pts',(-23.8656364276719,-12.5557718304403,
113.311130140898)) ;
#178812=CARTESIAN_POINT('Ctrl Pts',(-23.8799736924216,-12.6161812209366,
113.35479913392)) ;
#178813=CARTESIAN_POINT('Ctrl Pts',(-23.8061698222053,-12.6161812871028,
113.379030093989)) ;
#178814=CARTESIAN_POINT('Ctrl Pts',(-23.7323659519891,-12.6161813532691,
113.403261054057)) ;
#178815=CARTESIAN_POINT('Ctrl Pts',(-23.7180286872394,-12.5557719627728,
113.359592061035)) ;
#178816=CARTESIAN_POINT('Ctrl Pts',(-23.7036914224898,-12.4953625722765,
113.315923068013)) ;
#178817=CARTESIAN_POINT('Ctrl Pts',(-23.777495292706,-12.4953625061102,
113.291692107944)) ;
#178818=CARTESIAN_POINT('Ctrl Pts',(-23.8512991629223,-12.495362439944,
113.267461147876)) ;
#178819=CARTESIAN_POINT('Ctrl Pts',(-23.8656364276719,-12.5557718304403,
113.311130140898)) ;
#178820=CARTESIAN_POINT('Ctrl Pts',(-23.7913251487216,-12.7621800376528,
113.120181789862)) ;
#178821=CARTESIAN_POINT('Ctrl Pts',(-23.810139487679,-12.8082681507132,
113.177487228558)) ;
#178822=CARTESIAN_POINT('Ctrl Pts',(-23.7363356240177,-12.8082682369313,
113.201718208592)) ;
#178823=CARTESIAN_POINT('Ctrl Pts',(-23.6625317603564,-12.8082683231495,
113.225949188626)) ;
#178824=CARTESIAN_POINT('Ctrl Pts',(-23.643717421399,-12.7621802100891,
113.16864374993)) ;
#178825=CARTESIAN_POINT('Ctrl Pts',(-23.6249030824416,-12.7160920970287,
113.111338311234)) ;
#178826=CARTESIAN_POINT('Ctrl Pts',(-23.6987069461029,-12.7160920108106,
113.0871073312)) ;
#178827=CARTESIAN_POINT('Ctrl Pts',(-23.7725108097643,-12.7160919245924,
113.062876351166)) ;
#178828=CARTESIAN_POINT('Ctrl Pts',(-23.7913251487216,-12.7621800376528,
113.120181789862)) ;
#178829=CARTESIAN_POINT('Ctrl Pts',(-23.7361036954528,-13.0168738808962,
112.987578292511)) ;
#178830=CARTESIAN_POINT('Ctrl Pts',(-23.7580650338874,-13.0452490763117,
113.054468983887)) ;
#178831=CARTESIAN_POINT('Ctrl Pts',(-23.6842611783686,-13.0452491748441,
113.078699988721)) ;
#178832=CARTESIAN_POINT('Ctrl Pts',(-23.6104573228497,-13.0452492733765,
113.102930993556)) ;
#178833=CARTESIAN_POINT('Ctrl Pts',(-23.5884959844151,-13.0168740779611,
113.03604030218)) ;
#178834=CARTESIAN_POINT('Ctrl Pts',(-23.5665346459805,-12.9884988825456,
112.969149610803)) ;
#178835=CARTESIAN_POINT('Ctrl Pts',(-23.6403385014994,-12.9884987840132,
112.944918605969)) ;
#178836=CARTESIAN_POINT('Ctrl Pts',(-23.7141423570182,-12.9884986854807,
112.920687601134)) ;
#178837=CARTESIAN_POINT('Ctrl Pts',(-23.7361036954528,-13.0168738808962,
112.987578292511)) ;
#178838=CARTESIAN_POINT('Ctrl Pts',(-23.703804074422,-13.2984278863564,
112.924531497575)) ;
#178839=CARTESIAN_POINT('Ctrl Pts',(-23.7273220652697,-13.3071879031459,
112.996163501084)) ;
#178840=CARTESIAN_POINT('Ctrl Pts',(-23.6535182184119,-13.3071880059568,
113.020394532299)) ;
#178841=CARTESIAN_POINT('Ctrl Pts',(-23.579714371554,-13.3071881087676,
113.044625563513)) ;
#178842=CARTESIAN_POINT('Ctrl Pts',(-23.5561963807064,-13.2984280919781,
112.972993560004)) ;
#178843=CARTESIAN_POINT('Ctrl Pts',(-23.5326783898587,-13.2896680751886,
112.901361556494)) ;
#178844=CARTESIAN_POINT('Ctrl Pts',(-23.6064822367166,-13.2896679723777,
112.87713052528)) ;
#178845=CARTESIAN_POINT('Ctrl Pts',(-23.6802860835744,-13.2896678695669,
112.852899494065)) ;
#178846=CARTESIAN_POINT('Ctrl Pts',(-23.703804074422,-13.2984278863564,
112.924531497575)) ;
#178847=CARTESIAN_POINT('Ctrl Pts',(-23.6954444130968,-13.5897265030932,
112.93456078648)) ;
#178848=CARTESIAN_POINT('Ctrl Pts',(-23.7188468988158,-13.5781620490211,
113.005840980081)) ;
#178849=CARTESIAN_POINT('Ctrl Pts',(-23.6450430604439,-13.5781621471943,
113.030072037142)) ;
#178850=CARTESIAN_POINT('Ctrl Pts',(-23.571239222072,-13.5781622453675,
113.054303094203)) ;
#178851=CARTESIAN_POINT('Ctrl Pts',(-23.547836736353,-13.5897266994396,
112.983022900603)) ;
#178852=CARTESIAN_POINT('Ctrl Pts',(-23.524434250634,-13.6012911535118,
112.911742707003)) ;
#178853=CARTESIAN_POINT('Ctrl Pts',(-23.5982380890059,-13.6012910553386,
112.887511649942)) ;
#178854=CARTESIAN_POINT('Ctrl Pts',(-23.6720419273778,-13.6012909571654,
112.86328059288)) ;
#178855=CARTESIAN_POINT('Ctrl Pts',(-23.6954444130968,-13.5897265030932,
112.93456078648)) ;
#178856=CARTESIAN_POINT('Ctrl Pts',(-23.7111888510481,-13.8688372211758,
113.018021310344)) ;
#178857=CARTESIAN_POINT('Ctrl Pts',(-23.7327926044286,-13.8377685346258,
113.083822855566)) ;
#178858=CARTESIAN_POINT('Ctrl Pts',(-23.6589887733588,-13.8377686202372,
113.108053934868)) ;
#178859=CARTESIAN_POINT('Ctrl Pts',(-23.585184942289,-13.8377687058487,
113.13228501417)) ;
#178860=CARTESIAN_POINT('Ctrl Pts',(-23.5635811889085,-13.8688373923986,
113.066483468949)) ;
#178861=CARTESIAN_POINT('Ctrl Pts',(-23.5419774355281,-13.8999060789486,
113.000681923728)) ;
#178862=CARTESIAN_POINT('Ctrl Pts',(-23.6157812665979,-13.8999059933372,
112.976450844425)) ;
#178863=CARTESIAN_POINT('Ctrl Pts',(-23.6895850976677,-13.8999059077257,
112.952219765123)) ;
#178864=CARTESIAN_POINT('Ctrl Pts',(-23.7111888510481,-13.8688372211758,
113.018021310344)) ;
#178865=CARTESIAN_POINT('Ctrl Pts',(-23.7490277618584,-14.1152016754008,
113.168722954981)) ;
#178866=CARTESIAN_POINT('Ctrl Pts',(-23.7672886351906,-14.0668854985442,
113.224342627059)) ;
#178867=CARTESIAN_POINT('Ctrl Pts',(-23.6934848096128,-14.0668855661399,
113.248573723089)) ;
#178868=CARTESIAN_POINT('Ctrl Pts',(-23.6196809840351,-14.0668856337355,
113.272804819119)) ;
#178869=CARTESIAN_POINT('Ctrl Pts',(-23.6014201107028,-14.1152018105922,
113.217185147041)) ;
#178870=CARTESIAN_POINT('Ctrl Pts',(-23.5831592373706,-14.1635179874488,
113.161565474963)) ;
#178871=CARTESIAN_POINT('Ctrl Pts',(-23.6569630629483,-14.1635179198531,
113.137334378933)) ;
#178872=CARTESIAN_POINT('Ctrl Pts',(-23.7307668885261,-14.1635178522575,
113.113103282903)) ;
#178873=CARTESIAN_POINT('Ctrl Pts',(-23.7490277618584,-14.1152016754008,
113.168722954981)) ;
#178874=CARTESIAN_POINT('Ctrl Pts',(-23.8054647064364,-14.3116011164225,
113.376051058603)) ;
#178875=CARTESIAN_POINT('Ctrl Pts',(-23.8190796168698,-14.2494997572639,
113.417519877438)) ;
#178876=CARTESIAN_POINT('Ctrl Pts',(-23.7452757946167,-14.249499803588,
113.441750983595)) ;
#178877=CARTESIAN_POINT('Ctrl Pts',(-23.6714719723636,-14.249499849912,
113.465982089752)) ;
#178878=CARTESIAN_POINT('Ctrl Pts',(-23.6578570619302,-14.3116012090706,
113.424513270916)) ;
#178879=CARTESIAN_POINT('Ctrl Pts',(-23.6442421514968,-14.3737025682292,
113.383044452081)) ;
#178880=CARTESIAN_POINT('Ctrl Pts',(-23.7180459737499,-14.3737025219051,
113.358813345924)) ;
#178881=CARTESIAN_POINT('Ctrl Pts',(-23.7918497960029,-14.3737024755811,
113.334582239768)) ;
#178882=CARTESIAN_POINT('Ctrl Pts',(-23.8054647064364,-14.3116011164225,
113.376051058603)) ;
#178883=CARTESIAN_POINT('Ctrl Pts',(-23.8758475364015,-14.4442909382302,
113.625906113769)) ;
#178884=CARTESIAN_POINT('Ctrl Pts',(-23.8838347972143,-14.3728313741273,
113.650234020023)) ;
#178885=CARTESIAN_POINT('Ctrl Pts',(-23.8100309758451,-14.3728313982058,
113.674465128872)) ;
#178886=CARTESIAN_POINT('Ctrl Pts',(-23.7362271544759,-14.3728314222843,
113.698696237721)) ;
#178887=CARTESIAN_POINT('Ctrl Pts',(-23.7282398936631,-14.4442909863872,
113.674368331467)) ;
#178888=CARTESIAN_POINT('Ctrl Pts',(-23.7202526328503,-14.5157505504901,
113.650040425214)) ;
#178889=CARTESIAN_POINT('Ctrl Pts',(-23.7940564542195,-14.5157505264116,
113.625809316365)) ;
#178890=CARTESIAN_POINT('Ctrl Pts',(-23.8678602755887,-14.5157505023331,
113.601578207516)) ;
#178891=CARTESIAN_POINT('Ctrl Pts',(-23.8758475364015,-14.4442909382302,
113.625906113769)) ;
#178892=CARTESIAN_POINT('Ctrl Pts',(-23.9543884340958,-14.5033545209173,
113.900640311808)) ;
#178893=CARTESIAN_POINT('Ctrl Pts',(-23.9561692678758,-14.4276627971391,
113.906064442885)) ;
#178894=CARTESIAN_POINT('Ctrl Pts',(-23.8823654450948,-14.4276628009884,
113.930295547434)) ;
#178895=CARTESIAN_POINT('Ctrl Pts',(-23.8085616223137,-14.4276628048377,
113.954526651983)) ;
#178896=CARTESIAN_POINT('Ctrl Pts',(-23.8067807885338,-14.5033545286159,
113.949102520905)) ;
#178897=CARTESIAN_POINT('Ctrl Pts',(-23.8049999547538,-14.5790462523942,
113.943678389828)) ;
#178898=CARTESIAN_POINT('Ctrl Pts',(-23.8788037775349,-14.5790462485448,
113.91944728528)) ;
#178899=CARTESIAN_POINT('Ctrl Pts',(-23.9526076003159,-14.5790462446955,
113.895216180731)) ;
#178900=CARTESIAN_POINT('Ctrl Pts',(-23.9543884340958,-14.5033545209173,
113.900640311808)) ;
#178901=CARTESIAN_POINT('Ctrl Pts',(-24.034459322074,-14.4845849990311,
114.179961742102)) ;
#178902=CARTESIAN_POINT('Ctrl Pts',(-24.0299189346052,-14.4100891125331,
114.166132453338)) ;
#178903=CARTESIAN_POINT('Ctrl Pts',(-23.9561151089116,-14.4100891003362,
114.190363549015)) ;
#178904=CARTESIAN_POINT('Ctrl Pts',(-23.8823112832179,-14.4100890881394,
114.214594644693)) ;
#178905=CARTESIAN_POINT('Ctrl Pts',(-23.8868516706868,-14.4845849746373,
114.228423933456)) ;
#178906=CARTESIAN_POINT('Ctrl Pts',(-23.8913920581557,-14.5590808611353,
114.24225322222)) ;
#178907=CARTESIAN_POINT('Ctrl Pts',(-23.9651958838493,-14.5590808733321,
114.218022126543)) ;
#178908=CARTESIAN_POINT('Ctrl Pts',(-24.0389997095429,-14.559080885529,
114.193791030865)) ;
#178909=CARTESIAN_POINT('Ctrl Pts',(-24.034459322074,-14.4845849990311,
114.179961742102)) ;
#178910=CARTESIAN_POINT('Ctrl Pts',(-24.1098198340275,-14.3894948595566,
114.444970199635)) ;
#178911=CARTESIAN_POINT('Ctrl Pts',(-24.0992767680653,-14.3215252408879,
114.412857720877)) ;
#178912=CARTESIAN_POINT('Ctrl Pts',(-24.0254729382836,-14.3215252179033,
114.437088804104)) ;
#178913=CARTESIAN_POINT('Ctrl Pts',(-23.951669108502,-14.3215251949188,
114.46131988733)) ;
#178914=CARTESIAN_POINT('Ctrl Pts',(-23.9622121744642,-14.3894948135875,
114.493432366087)) ;
#178915=CARTESIAN_POINT('Ctrl Pts',(-23.9727552404264,-14.4574644322562,
114.525544844844)) ;
#178916=CARTESIAN_POINT('Ctrl Pts',(-24.0465590702081,-14.4574644552408,
114.501313761618)) ;
#178917=CARTESIAN_POINT('Ctrl Pts',(-24.1203628999897,-14.4574644782253,
114.477082678392)) ;
#178918=CARTESIAN_POINT('Ctrl Pts',(-24.1098198340275,-14.3894948595566,
114.444970199635)) ;
#178919=CARTESIAN_POINT('Ctrl Pts',(-24.1743167962616,-14.2243477865837,
114.676951586264)) ;
#178920=CARTESIAN_POINT('Ctrl Pts',(-24.1585190622833,-14.1678057740267,
114.628834236749)) ;
#178921=CARTESIAN_POINT('Ctrl Pts',(-24.0847152279406,-14.1678057466232,
114.653065306083)) ;
#178922=CARTESIAN_POINT('Ctrl Pts',(-24.0109113935979,-14.1678057192196,
114.677296375417)) ;
#178923=CARTESIAN_POINT('Ctrl Pts',(-24.0267091275762,-14.2243477317766,
114.725413724931)) ;
#178924=CARTESIAN_POINT('Ctrl Pts',(-24.0425068615545,-14.2808897443336,
114.773531074446)) ;
#178925=CARTESIAN_POINT('Ctrl Pts',(-24.1163106958972,-14.2808897717371,
114.749300005113)) ;
#178926=CARTESIAN_POINT('Ctrl Pts',(-24.1901145302398,-14.2808897991407,
114.725068935779)) ;
#178927=CARTESIAN_POINT('Ctrl Pts',(-24.1743167962616,-14.2243477865837,
114.676951586264)) ;
#178928=CARTESIAN_POINT('Ctrl Pts',(-24.222244696456,-14.0022176408066,
114.858320300605)) ;
#178929=CARTESIAN_POINT('Ctrl Pts',(-24.2023442920191,-13.9610998254784,
114.797706878987)) ;
#178930=CARTESIAN_POINT('Ctrl Pts',(-24.128540453823,-13.9610997980143,
114.821937936584)) ;
#178931=CARTESIAN_POINT('Ctrl Pts',(-24.0547366156269,-13.9610997705502,
114.846168994181)) ;
#178932=CARTESIAN_POINT('Ctrl Pts',(-24.0746370200638,-14.0022175858784,
114.906782415799)) ;
#178933=CARTESIAN_POINT('Ctrl Pts',(-24.0945374245007,-14.0433354012065,
114.967395837416)) ;
#178934=CARTESIAN_POINT('Ctrl Pts',(-24.1683412626968,-14.0433354286706,
114.943164779819)) ;
#178935=CARTESIAN_POINT('Ctrl Pts',(-24.2421451008929,-14.0433354561347,
114.918933722222)) ;
#178936=CARTESIAN_POINT('Ctrl Pts',(-24.222244696456,-14.0022176408066,
114.858320300605)) ;
#178937=CARTESIAN_POINT('Ctrl Pts',(-24.249840889695,-13.738467096939,114.977769983769)) ;
#178938=CARTESIAN_POINT('Ctrl Pts',(-24.2272510577212,-13.7157029540504,
114.90896499996)) ;
#178939=CARTESIAN_POINT('Ctrl Pts',(-24.1534472163186,-13.7157029304284,
114.933196047791)) ;
#178940=CARTESIAN_POINT('Ctrl Pts',(-24.0796433749161,-13.7157029068064,
114.957427095621)) ;
#178941=CARTESIAN_POINT('Ctrl Pts',(-24.1022332068898,-13.7384670496951,
115.02623207943)) ;
#178942=CARTESIAN_POINT('Ctrl Pts',(-24.1248230388635,-13.7612311925838,
115.09503706324)) ;
#178943=CARTESIAN_POINT('Ctrl Pts',(-24.1986268802661,-13.7612312162057,
115.070806015409)) ;
#178944=CARTESIAN_POINT('Ctrl Pts',(-24.2724307216687,-13.7612312398277,
115.046574967579)) ;
#178945=CARTESIAN_POINT('Ctrl Pts',(-24.249840889695,-13.738467096939,114.977769983769)) ;
#178946=CARTESIAN_POINT('Ctrl Pts',(-24.2541673118349,-13.4497089979361,
115.026595498721)) ;
#178947=CARTESIAN_POINT('Ctrl Pts',(-24.2305033326588,-13.4470729422015,
114.954518836024)) ;
#178948=CARTESIAN_POINT('Ctrl Pts',(-24.1566994891785,-13.4470729268746,
114.978749877526)) ;
#178949=CARTESIAN_POINT('Ctrl Pts',(-24.0828956456982,-13.4470729115476,
115.002980919029)) ;
#178950=CARTESIAN_POINT('Ctrl Pts',(-24.1065596248743,-13.4497089672822,
115.075057581726)) ;
#178951=CARTESIAN_POINT('Ctrl Pts',(-24.1302236040503,-13.4523450230167,
115.147134244423)) ;
#178952=CARTESIAN_POINT('Ctrl Pts',(-24.2040274475306,-13.4523450383437,
115.122903202921)) ;
#178953=CARTESIAN_POINT('Ctrl Pts',(-24.2778312910109,-13.4523450536706,
115.098672161419)) ;
#178954=CARTESIAN_POINT('Ctrl Pts',(-24.2541673118349,-13.4497089979361,
115.026595498721)) ;
#178955=CARTESIAN_POINT('Ctrl Pts',(-24.2342295189752,-13.1612741016994,
115.001189108722)) ;
#178956=CARTESIAN_POINT('Ctrl Pts',(-24.2111911927436,-13.1787740076572,
114.931018084053)) ;
#178957=CARTESIAN_POINT('Ctrl Pts',(-24.1373873484711,-13.1787739983459,
114.955249123143)) ;
#178958=CARTESIAN_POINT('Ctrl Pts',(-24.0635835041986,-13.1787739890347,
114.979480162232)) ;
#178959=CARTESIAN_POINT('Ctrl Pts',(-24.0866218304302,-13.161274083077,
115.049651186901)) ;
#178960=CARTESIAN_POINT('Ctrl Pts',(-24.1096601566617,-13.1437741771192,
115.11982221157)) ;
#178961=CARTESIAN_POINT('Ctrl Pts',(-24.1834640009343,-13.1437741864305,
115.095591172481)) ;
#178962=CARTESIAN_POINT('Ctrl Pts',(-24.2572678452068,-13.1437741957417,
115.071360133392)) ;
#178963=CARTESIAN_POINT('Ctrl Pts',(-24.2342295189752,-13.1612741016994,
115.001189108722)) ;
#178964=CARTESIAN_POINT('Ctrl Pts',(-24.190640216784,-12.8897094409154,
114.903930822118)) ;
#178965=CARTESIAN_POINT('Ctrl Pts',(-24.1698760482874,-12.9261981229531,
114.840686515092)) ;
#178966=CARTESIAN_POINT('Ctrl Pts',(-24.0960722041816,-12.9261981199508,
114.864917554689)) ;
#178967=CARTESIAN_POINT('Ctrl Pts',(-24.0222683600759,-12.9261981169484,
114.889148594286)) ;
#178968=CARTESIAN_POINT('Ctrl Pts',(-24.0430325285724,-12.8897094349106,
114.952392901312)) ;
#178969=CARTESIAN_POINT('Ctrl Pts',(-24.063796697069,-12.8532207528728,
115.015637208338)) ;
#178970=CARTESIAN_POINT('Ctrl Pts',(-24.1376005411748,-12.8532207558752,
114.991406168741)) ;
#178971=CARTESIAN_POINT('Ctrl Pts',(-24.2114043852805,-12.8532207588776,
114.967175129144)) ;
#178972=CARTESIAN_POINT('Ctrl Pts',(-24.190640216784,-12.8897094409154,
114.903930822118)) ;
#178973=CARTESIAN_POINT('Ctrl Pts',(-24.12571950388,-12.6562456914582,114.741683307062)) ;
#178974=CARTESIAN_POINT('Ctrl Pts',(-24.1087229981294,-12.7090913672215,
114.689914692932)) ;
#178975=CARTESIAN_POINT('Ctrl Pts',(-24.0349191547742,-12.7090913678115,
114.714145734815)) ;
#178976=CARTESIAN_POINT('Ctrl Pts',(-23.9611153114191,-12.7090913684014,
114.738376776699)) ;
#178977=CARTESIAN_POINT('Ctrl Pts',(-23.9781118171697,-12.6562456926381,
114.790145390829)) ;
#178978=CARTESIAN_POINT('Ctrl Pts',(-23.9951083229202,-12.6034000168748,
114.841914004959)) ;
#178979=CARTESIAN_POINT('Ctrl Pts',(-24.0689121662754,-12.6034000162848,
114.817682963075)) ;
#178980=CARTESIAN_POINT('Ctrl Pts',(-24.1427160096306,-12.6034000156949,
114.793451921192)) ;
#178981=CARTESIAN_POINT('Ctrl Pts',(-24.12571950388,-12.6562456914582,114.741683307062)) ;
#178982=CARTESIAN_POINT('Ctrl Pts',(-24.0436220945344,-12.4776727385034,
114.527047044572)) ;
#178983=CARTESIAN_POINT('Ctrl Pts',(-24.0315999579,-12.5430665367951,114.490429556204)) ;
#178984=CARTESIAN_POINT('Ctrl Pts',(-23.9577961152497,-12.5430665383516,
114.514660600234)) ;
#178985=CARTESIAN_POINT('Ctrl Pts',(-23.8839922725995,-12.543066539908,
114.538891644265)) ;
#178986=CARTESIAN_POINT('Ctrl Pts',(-23.896014409234,-12.4776727416163,
114.575509132633)) ;
#178987=CARTESIAN_POINT('Ctrl Pts',(-23.9080365458684,-12.4122789433245,
114.612126621002)) ;
#178988=CARTESIAN_POINT('Ctrl Pts',(-23.9818403885187,-12.4122789417681,
114.587895576971)) ;
#178989=CARTESIAN_POINT('Ctrl Pts',(-24.0556442311689,-12.4122789402116,
114.563664532941)) ;
#178990=CARTESIAN_POINT('Ctrl Pts',(-24.0436220945344,-12.4776727385034,
114.527047044572)) ;
#178991=CARTESIAN_POINT('Ctrl Pts',(-23.949166950014,-12.3662041520314,
114.27482871689)) ;
#178992=CARTESIAN_POINT('Ctrl Pts',(-23.9429885673847,-12.439478800866,
114.256010360343)) ;
#178993=CARTESIAN_POINT('Ctrl Pts',(-23.8691847249648,-12.4394788016548,
114.280241405074)) ;
#178994=CARTESIAN_POINT('Ctrl Pts',(-23.7953808825448,-12.4394788024435,
114.304472449806)) ;
#178995=CARTESIAN_POINT('Ctrl Pts',(-23.8015592651741,-12.3662041536089,
114.323290806354)) ;
#178996=CARTESIAN_POINT('Ctrl Pts',(-23.8077376478033,-12.2929295047743,
114.342109162901)) ;
#178997=CARTESIAN_POINT('Ctrl Pts',(-23.8815414902233,-12.2929295039855,
114.317878118169)) ;
#178998=CARTESIAN_POINT('Ctrl Pts',(-23.9553453326433,-12.2929295031968,
114.293647073438)) ;
#178999=CARTESIAN_POINT('Ctrl Pts',(-23.949166950014,-12.3662041520314,
114.27482871689)) ;
#179000=CARTESIAN_POINT('Ctrl Pts',(-23.8486819494618,-12.3300379060018,
114.004176603024)) ;
#179001=CARTESIAN_POINT('Ctrl Pts',(-23.8487783311831,-12.4059457816004,
114.004470166228)) ;
#179002=CARTESIAN_POINT('Ctrl Pts',(-23.7749744882838,-12.405945781314,
114.0287012095)) ;
#179003=CARTESIAN_POINT('Ctrl Pts',(-23.7011706453844,-12.4059457810276,
114.052932252771)) ;
#179004=CARTESIAN_POINT('Ctrl Pts',(-23.7010742636631,-12.330037905429,
114.052638689568)) ;
#179005=CARTESIAN_POINT('Ctrl Pts',(-23.7009778819417,-12.2541300298303,
114.052345126364)) ;
#179006=CARTESIAN_POINT('Ctrl Pts',(-23.7747817248411,-12.2541300301167,
114.028114083092)) ;
#179007=CARTESIAN_POINT('Ctrl Pts',(-23.8485855677404,-12.2541300304032,
114.00388303982)) ;
#179008=CARTESIAN_POINT('Ctrl Pts',(-23.8486819494618,-12.3300379060018,
114.004176603024)) ;
#179009=CARTESIAN_POINT('Ctrl Pts',(-23.7479716280047,-12.3719948524369,
113.733003975022)) ;
#179010=CARTESIAN_POINT('Ctrl Pts',(-23.7543642990967,-12.4450845928375,
113.752475019667)) ;
#179011=CARTESIAN_POINT('Ctrl Pts',(-23.6805604549014,-12.4450845931213,
113.776706058991)) ;
#179012=CARTESIAN_POINT('Ctrl Pts',(-23.606756610706,-12.4450845934052,
113.800937098315)) ;
#179013=CARTESIAN_POINT('Ctrl Pts',(-23.600363939614,-12.3719948530046,
113.781466053671)) ;
#179014=CARTESIAN_POINT('Ctrl Pts',(-23.593971268522,-12.298905112604,113.761995009026)) ;
#179015=CARTESIAN_POINT('Ctrl Pts',(-23.6677751127173,-12.2989051123201,
113.737763969702)) ;
#179016=CARTESIAN_POINT('Ctrl Pts',(-23.7415789569127,-12.2989051120363,
113.713532930378)) ;
#179017=CARTESIAN_POINT('Ctrl Pts',(-23.7479716280047,-12.3719948524369,
113.733003975022)) ;
#179018=CARTESIAN_POINT('Ctrl Pts',(-23.6544815761993,-12.4886302946211,
113.483633344995)) ;
#179019=CARTESIAN_POINT('Ctrl Pts',(-23.6666792066729,-12.5536824070631,
113.520785359195)) ;
#179020=CARTESIAN_POINT('Ctrl Pts',(-23.5928753612354,-12.5536824104958,
113.545016394736)) ;
#179021=CARTESIAN_POINT('Ctrl Pts',(-23.519071515798,-12.5536824139286,
113.569247430277)) ;
#179022=CARTESIAN_POINT('Ctrl Pts',(-23.5068738853244,-12.4886303014866,
113.532095416077)) ;
#179023=CARTESIAN_POINT('Ctrl Pts',(-23.4946762548508,-12.4235781890446,
113.494943401877)) ;
#179024=CARTESIAN_POINT('Ctrl Pts',(-23.5684801002883,-12.4235781856119,
113.470712366336)) ;
#179025=CARTESIAN_POINT('Ctrl Pts',(-23.6422839457257,-12.4235781821791,
113.446481330795)) ;
#179026=CARTESIAN_POINT('Ctrl Pts',(-23.6544815761993,-12.4886302946211,
113.483633344995)) ;
#179027=CARTESIAN_POINT('Ctrl Pts',(-23.5734119895845,-12.6716133926028,
113.272144861852)) ;
#179028=CARTESIAN_POINT('Ctrl Pts',(-23.5905546162055,-12.7239835426952,
113.324358536327)) ;
#179029=CARTESIAN_POINT('Ctrl Pts',(-23.5167507697617,-12.7239835519862,
113.348589568803)) ;
#179030=CARTESIAN_POINT('Ctrl Pts',(-23.4429469233179,-12.7239835612772,
113.372820601279)) ;
#179031=CARTESIAN_POINT('Ctrl Pts',(-23.425804296697,-12.6716134111847,
113.320606926803)) ;
#179032=CARTESIAN_POINT('Ctrl Pts',(-23.408661670076,-12.6192432610923,
113.268393252328)) ;
#179033=CARTESIAN_POINT('Ctrl Pts',(-23.4824655165198,-12.6192432518013,
113.244162219852)) ;
#179034=CARTESIAN_POINT('Ctrl Pts',(-23.5562693629636,-12.6192432425104,
113.219931187376)) ;
#179035=CARTESIAN_POINT('Ctrl Pts',(-23.5734119895845,-12.6716133926028,
113.272144861852)) ;
#179036=CARTESIAN_POINT('Ctrl Pts',(-23.5097546848615,-12.9096205473869,
113.113892958082)) ;
#179037=CARTESIAN_POINT('Ctrl Pts',(-23.5306295961467,-12.9454485292725,
113.177474569271)) ;
#179038=CARTESIAN_POINT('Ctrl Pts',(-23.4568257492868,-12.9454485486713,
113.201705600479)) ;
#179039=CARTESIAN_POINT('Ctrl Pts',(-23.3830219024269,-12.9454485680701,
113.225936631688)) ;
#179040=CARTESIAN_POINT('Ctrl Pts',(-23.3621469911418,-12.9096205861845,
113.162355020499)) ;
#179041=CARTESIAN_POINT('Ctrl Pts',(-23.3412720798566,-12.8737926042989,
113.098773409311)) ;
#179042=CARTESIAN_POINT('Ctrl Pts',(-23.4150759267165,-12.8737925849001,
113.074542378102)) ;
#179043=CARTESIAN_POINT('Ctrl Pts',(-23.4888797735763,-12.8737925655013,
113.050311346893)) ;
#179044=CARTESIAN_POINT('Ctrl Pts',(-23.5097546848615,-12.9096205473869,
113.113892958082)) ;
#179045=CARTESIAN_POINT('Ctrl Pts',(-23.4680736791357,-13.1819739695916,
113.02227623672)) ;
#179046=CARTESIAN_POINT('Ctrl Pts',(-23.4911576828605,-13.1988376121803,
113.09258638691)) ;
#179047=CARTESIAN_POINT('Ctrl Pts',(-23.4173538372792,-13.1988376406376,
113.116817422013)) ;
#179048=CARTESIAN_POINT('Ctrl Pts',(-23.3435499916979,-13.198837669095,
113.141048457116)) ;
#179049=CARTESIAN_POINT('Ctrl Pts',(-23.3204659879731,-13.1819740265063,
113.070738306926)) ;
#179050=CARTESIAN_POINT('Ctrl Pts',(-23.2973819842482,-13.1651103839176,
113.000428156736)) ;
#179051=CARTESIAN_POINT('Ctrl Pts',(-23.3711858298295,-13.1651103554602,
112.976197121633)) ;
#179052=CARTESIAN_POINT('Ctrl Pts',(-23.4449896754108,-13.1651103270029,
112.951966086531)) ;
#179053=CARTESIAN_POINT('Ctrl Pts',(-23.4680736791357,-13.1819739695916,
113.02227623672)) ;
#179054=CARTESIAN_POINT('Ctrl Pts',(-23.4498548257593,-13.4720244815185,
113.002241777348)) ;
#179055=CARTESIAN_POINT('Ctrl Pts',(-23.4735105433531,-13.4686610544737,
113.074293275574)) ;
#179056=CARTESIAN_POINT('Ctrl Pts',(-23.399706700273,-13.4686610921263,
113.098524318295)) ;
#179057=CARTESIAN_POINT('Ctrl Pts',(-23.3259028571929,-13.4686611297789,
113.122755361017)) ;
#179058=CARTESIAN_POINT('Ctrl Pts',(-23.3022471395991,-13.4720245568238,
113.05070386279)) ;
#179059=CARTESIAN_POINT('Ctrl Pts',(-23.2785914220053,-13.4753879838686,
112.978652364563)) ;
#179060=CARTESIAN_POINT('Ctrl Pts',(-23.3523952650854,-13.475387946216,
112.954421321842)) ;
#179061=CARTESIAN_POINT('Ctrl Pts',(-23.4261991081655,-13.4753879085634,
112.930190279121)) ;
#179062=CARTESIAN_POINT('Ctrl Pts',(-23.4498548257593,-13.4720244815185,
113.002241777348)) ;
#179063=CARTESIAN_POINT('Ctrl Pts',(-23.4559991647249,-13.7591219512168,
113.056520534112)) ;
#179064=CARTESIAN_POINT('Ctrl Pts',(-23.4785242563665,-13.7357085596368,
113.125128327926)) ;
#179065=CARTESIAN_POINT('Ctrl Pts',(-23.4047204173389,-13.7357086049052,
113.14935938299)) ;
#179066=CARTESIAN_POINT('Ctrl Pts',(-23.3309165783112,-13.7357086501736,
113.173590438055)) ;
#179067=CARTESIAN_POINT('Ctrl Pts',(-23.3083914866696,-13.7591220417536,
113.10498264424)) ;
#179068=CARTESIAN_POINT('Ctrl Pts',(-23.285866395028,-13.7825354333337,
113.036374850426)) ;
#179069=CARTESIAN_POINT('Ctrl Pts',(-23.3596702340557,-13.7825353880653,
113.012143795361)) ;
#179070=CARTESIAN_POINT('Ctrl Pts',(-23.4334740730833,-13.7825353427969,
112.987912740297)) ;
#179071=CARTESIAN_POINT('Ctrl Pts',(-23.4559991647249,-13.7591219512168,
113.056520534112)) ;
#179072=CARTESIAN_POINT('Ctrl Pts',(-23.4853259386765,-14.0209982570872,
113.181335126666)) ;
#179073=CARTESIAN_POINT('Ctrl Pts',(-23.5051016687503,-13.9792670582561,
113.241568808581)) ;
#179074=CARTESIAN_POINT('Ctrl Pts',(-23.4312978349103,-13.9792671054372,
113.265799879446)) ;
#179075=CARTESIAN_POINT('Ctrl Pts',(-23.3574940010702,-13.9792671526183,
113.29003095031)) ;
#179076=CARTESIAN_POINT('Ctrl Pts',(-23.3377182709964,-14.0209983514494,
113.229797268396)) ;
#179077=CARTESIAN_POINT('Ctrl Pts',(-23.3179425409226,-14.0627295502805,
113.169563586481)) ;
#179078=CARTESIAN_POINT('Ctrl Pts',(-23.3917463747627,-14.0627295030994,
113.145332515616)) ;
#179079=CARTESIAN_POINT('Ctrl Pts',(-23.4655502086028,-14.0627294559183,
113.121101444752)) ;
#179080=CARTESIAN_POINT('Ctrl Pts',(-23.4853259386765,-14.0209982570872,
113.181335126666)) ;
#179081=CARTESIAN_POINT('Ctrl Pts',(-23.5345041189141,-14.2386408615737,
113.36640397491)) ;
#179082=CARTESIAN_POINT('Ctrl Pts',(-23.5501447454779,-14.1816542557546,
113.4140427986)) ;
#179083=CARTESIAN_POINT('Ctrl Pts',(-23.4763409167572,-14.1816542976557,
113.438273885057)) ;
#179084=CARTESIAN_POINT('Ctrl Pts',(-23.4025370880364,-14.1816543395568,
113.462504971515)) ;
#179085=CARTESIAN_POINT('Ctrl Pts',(-23.3868964614725,-14.2386409453758,
113.414866147825)) ;
#179086=CARTESIAN_POINT('Ctrl Pts',(-23.3712558349086,-14.2956275511949,
113.367227324135)) ;
#179087=CARTESIAN_POINT('Ctrl Pts',(-23.4450596636294,-14.2956275092938,
113.342996237677)) ;
#179088=CARTESIAN_POINT('Ctrl Pts',(-23.5188634923502,-14.2956274673927,
113.31876515122)) ;
#179089=CARTESIAN_POINT('Ctrl Pts',(-23.5345041189141,-14.2386408615737,
113.36640397491)) ;
#179090=CARTESIAN_POINT('Ctrl Pts',(-23.6001054827243,-14.3991847031552,
113.601804261301)) ;
#179091=CARTESIAN_POINT('Ctrl Pts',(-23.6104522949311,-14.3309065513588,
113.633318980433)) ;
#179092=CARTESIAN_POINT('Ctrl Pts',(-23.5366484717624,-14.330906583244,
113.657550083801)) ;
#179093=CARTESIAN_POINT('Ctrl Pts',(-23.4628446485939,-14.3309066151293,
113.68178118717)) ;
#179094=CARTESIAN_POINT('Ctrl Pts',(-23.4524978363872,-14.3991847669257,
113.650266468038)) ;
#179095=CARTESIAN_POINT('Ctrl Pts',(-23.4421510241805,-14.4674629187221,
113.618751748905)) ;
#179096=CARTESIAN_POINT('Ctrl Pts',(-23.515954847349,-14.4674628868368,
113.594520645537)) ;
#179097=CARTESIAN_POINT('Ctrl Pts',(-23.5897586705176,-14.4674628549516,
113.570289542169)) ;
#179098=CARTESIAN_POINT('Ctrl Pts',(-23.6001054827243,-14.3991847031552,
113.601804261301)) ;
#179099=CARTESIAN_POINT('Ctrl Pts',(-23.6758396635348,-14.4885294284138,
113.867853985645)) ;
#179100=CARTESIAN_POINT('Ctrl Pts',(-23.6801818892424,-14.4139147342441,
113.881079703006)) ;
#179101=CARTESIAN_POINT('Ctrl Pts',(-23.6063780700887,-14.4139147488746,
113.905310818603)) ;
#179102=CARTESIAN_POINT('Ctrl Pts',(-23.5325742509351,-14.4139147635052,
113.929541934201)) ;
#179103=CARTESIAN_POINT('Ctrl Pts',(-23.5282320252275,-14.4885294576749,
113.91631621684)) ;
#179104=CARTESIAN_POINT('Ctrl Pts',(-23.52388979952,-14.5631441518446,113.903090499479)) ;
#179105=CARTESIAN_POINT('Ctrl Pts',(-23.5976936186736,-14.563144137214,
113.878859383882)) ;
#179106=CARTESIAN_POINT('Ctrl Pts',(-23.6714974378272,-14.5631441225835,
113.854628268285)) ;
#179107=CARTESIAN_POINT('Ctrl Pts',(-23.6758396635348,-14.4885294284138,
113.867853985645)) ;
#179108=CARTESIAN_POINT('Ctrl Pts',(-23.7560787132041,-14.5016597743674,
114.147723270265)) ;
#179109=CARTESIAN_POINT('Ctrl Pts',(-23.7540912036683,-14.4260199965907,
114.141669635237)) ;
#179110=CARTESIAN_POINT('Ctrl Pts',(-23.6802873870442,-14.4260199894703,
114.165900758539)) ;
#179111=CARTESIAN_POINT('Ctrl Pts',(-23.60648357042,-14.4260199823499,114.19013188184)) ;
#179112=CARTESIAN_POINT('Ctrl Pts',(-23.6084710799558,-14.5016597601266,
114.196185516868)) ;
#179113=CARTESIAN_POINT('Ctrl Pts',(-23.6104585894916,-14.5772995379034,
114.202239151896)) ;
#179114=CARTESIAN_POINT('Ctrl Pts',(-23.6842624061158,-14.5772995450237,
114.178008028595)) ;
#179115=CARTESIAN_POINT('Ctrl Pts',(-23.7580662227399,-14.5772995521441,
114.153776905293)) ;
#179116=CARTESIAN_POINT('Ctrl Pts',(-23.7560787132041,-14.5016597743674,
114.147723270265)) ;
#179117=CARTESIAN_POINT('Ctrl Pts',(-23.8342305464961,-14.437009415365,
114.421263368043)) ;
#179118=CARTESIAN_POINT('Ctrl Pts',(-23.8260492739451,-14.3657730764766,
114.396344530107)) ;
#179119=CARTESIAN_POINT('Ctrl Pts',(-23.7522454576535,-14.3657730444813,
114.420575654421)) ;
#179120=CARTESIAN_POINT('Ctrl Pts',(-23.678441641362,-14.365773012486,114.444806778735)) ;
#179121=CARTESIAN_POINT('Ctrl Pts',(-23.6866229139129,-14.4370093513744,
114.469725616672)) ;
#179122=CARTESIAN_POINT('Ctrl Pts',(-23.6948041864639,-14.5082456902627,
114.494644454609)) ;
#179123=CARTESIAN_POINT('Ctrl Pts',(-23.7686080027555,-14.508245722258,
114.470413330295)) ;
#179124=CARTESIAN_POINT('Ctrl Pts',(-23.8424118190471,-14.5082457542533,
114.44618220598)) ;
#179125=CARTESIAN_POINT('Ctrl Pts',(-23.8342305464961,-14.437009415365,
114.421263368043)) ;
#179126=CARTESIAN_POINT('Ctrl Pts',(-23.9038790142128,-14.2988734246617,
114.668946179201)) ;
#179127=CARTESIAN_POINT('Ctrl Pts',(-23.8900877080365,-14.2371769971241,
114.626940083908)) ;
#179128=CARTESIAN_POINT('Ctrl Pts',(-23.8162838894959,-14.237176939765,
114.651171201373)) ;
#179129=CARTESIAN_POINT('Ctrl Pts',(-23.7424800709552,-14.2371768824059,
114.675402318837)) ;
#179130=CARTESIAN_POINT('Ctrl Pts',(-23.7562713771315,-14.2988733099436,
114.717408414129)) ;
#179131=CARTESIAN_POINT('Ctrl Pts',(-23.7700626833078,-14.3605697374812,
114.759414509421)) ;
#179132=CARTESIAN_POINT('Ctrl Pts',(-23.8438665018485,-14.3605697948403,
114.735183391957)) ;
#179133=CARTESIAN_POINT('Ctrl Pts',(-23.9176703203892,-14.3605698521993,
114.710952274493)) ;
#179134=CARTESIAN_POINT('Ctrl Pts',(-23.9038790142128,-14.2988734246617,
114.668946179201)) ;
#179135=CARTESIAN_POINT('Ctrl Pts',(-23.9589267388881,-14.0989764690058,
114.871924271344)) ;
#179136=CARTESIAN_POINT('Ctrl Pts',(-23.9405414467477,-14.0511462695814,
114.815925635974)) ;
#179137=CARTESIAN_POINT('Ctrl Pts',(-23.8667376232761,-14.0511461903864,
114.840156738419)) ;
#179138=CARTESIAN_POINT('Ctrl Pts',(-23.7929337998045,-14.0511461111915,
114.864387840864)) ;
#179139=CARTESIAN_POINT('Ctrl Pts',(-23.8113190919448,-14.0989763106159,
114.920386476235)) ;
#179140=CARTESIAN_POINT('Ctrl Pts',(-23.8297043840852,-14.1468065100403,
114.976385111605)) ;
#179141=CARTESIAN_POINT('Ctrl Pts',(-23.9035082075568,-14.1468065892353,
114.95215400916)) ;
#179142=CARTESIAN_POINT('Ctrl Pts',(-23.9773120310284,-14.1468066684302,
114.927922906715)) ;
#179143=CARTESIAN_POINT('Ctrl Pts',(-23.9589267388881,-14.0989764690058,
114.871924271344)) ;
#179144=CARTESIAN_POINT('Ctrl Pts',(-23.9954157212117,-13.8484694868484,
115.01867831934)) ;
#179145=CARTESIAN_POINT('Ctrl Pts',(-23.973718935146,-13.8180580458534,
114.952593407707)) ;
#179146=CARTESIAN_POINT('Ctrl Pts',(-23.8999151048323,-13.8180579489714,
114.976824489312)) ;
#179147=CARTESIAN_POINT('Ctrl Pts',(-23.8261112745187,-13.8180578520894,
115.001055570918)) ;
#179148=CARTESIAN_POINT('Ctrl Pts',(-23.8478080605844,-13.8484692930843,
115.067140482551)) ;
#179149=CARTESIAN_POINT('Ctrl Pts',(-23.8695048466502,-13.8788807340793,
115.133225394185)) ;
#179150=CARTESIAN_POINT('Ctrl Pts',(-23.9433086769638,-13.8788808309613,
115.108994312579)) ;
#179151=CARTESIAN_POINT('Ctrl Pts',(-24.0171125072775,-13.8788809278433,
115.084763230974)) ;
#179152=CARTESIAN_POINT('Ctrl Pts',(-23.9954157212117,-13.8484694868484,
115.01867831934)) ;
#179153=CARTESIAN_POINT('Ctrl Pts',(-24.0092992091124,-13.5679794956402,
115.096428165126)) ;
#179154=CARTESIAN_POINT('Ctrl Pts',(-23.9858673863467,-13.5571060309524,
115.025058611615)) ;
#179155=CARTESIAN_POINT('Ctrl Pts',(-23.9120635475771,-13.5571059245038,
115.049289667465)) ;
#179156=CARTESIAN_POINT('Ctrl Pts',(-23.8382597088075,-13.5571058180553,
115.073520723315)) ;
#179157=CARTESIAN_POINT('Ctrl Pts',(-23.8616915315733,-13.567979282743,
115.144890276826)) ;
#179158=CARTESIAN_POINT('Ctrl Pts',(-23.885123354339,-13.5788527474308,
115.216259830337)) ;
#179159=CARTESIAN_POINT('Ctrl Pts',(-23.9589271931086,-13.5788528538794,
115.192028774487)) ;
#179160=CARTESIAN_POINT('Ctrl Pts',(-24.0327310318782,-13.578852960328,
115.167797718637)) ;
#179161=CARTESIAN_POINT('Ctrl Pts',(-24.0092992091124,-13.5679794956402,
115.096428165126)) ;
#179162=CARTESIAN_POINT('Ctrl Pts',(-23.9992431261541,-13.2778704302602,
115.101136556638)) ;
#179163=CARTESIAN_POINT('Ctrl Pts',(-23.9757477130597,-13.2872353982741,
115.02957331723)) ;
#179164=CARTESIAN_POINT('Ctrl Pts',(-23.9019438652982,-13.2872352908657,
115.053804345692)) ;
#179165=CARTESIAN_POINT('Ctrl Pts',(-23.8281400175367,-13.2872351834573,
115.078035374154)) ;
#179166=CARTESIAN_POINT('Ctrl Pts',(-23.8516354306311,-13.2778702154433,
115.149598613562)) ;
#179167=CARTESIAN_POINT('Ctrl Pts',(-23.8751308437256,-13.2685052474294,
115.22116185297)) ;
#179168=CARTESIAN_POINT('Ctrl Pts',(-23.9489346914871,-13.2685053548378,
115.196930824508)) ;
#179169=CARTESIAN_POINT('Ctrl Pts',(-24.0227385392486,-13.2685054622462,
115.172699796046)) ;
#179170=CARTESIAN_POINT('Ctrl Pts',(-23.9992431261541,-13.2778704302602,
115.101136556638)) ;
#179171=CARTESIAN_POINT('Ctrl Pts',(-23.9651195032617,-12.9966579805532,
115.03267001783)) ;
#179172=CARTESIAN_POINT('Ctrl Pts',(-23.9432377697369,-13.0256699682594,
114.966021786025)) ;
#179173=CARTESIAN_POINT('Ctrl Pts',(-23.8694339132126,-13.025669868452,
114.990252787797)) ;
#179174=CARTESIAN_POINT('Ctrl Pts',(-23.7956300566882,-13.0256697686447,
115.014483789568)) ;
#179175=CARTESIAN_POINT('Ctrl Pts',(-23.817511790213,-12.9966577809386,
115.081132021373)) ;
#179176=CARTESIAN_POINT('Ctrl Pts',(-23.8393935237377,-12.9676457932324,
115.147780253178)) ;
#179177=CARTESIAN_POINT('Ctrl Pts',(-23.9131973802621,-12.9676458930398,
115.123549251406)) ;
#179178=CARTESIAN_POINT('Ctrl Pts',(-23.9870012367865,-12.9676459928471,
115.099318249634)) ;
#179179=CARTESIAN_POINT('Ctrl Pts',(-23.9651195032617,-12.9966579805532,
115.03267001783)) ;
#179180=CARTESIAN_POINT('Ctrl Pts',(-23.9083188929157,-12.7449733317735,
114.895243151894)) ;
#179181=CARTESIAN_POINT('Ctrl Pts',(-23.8896339516894,-12.7916002389954,
114.838331833659)) ;
#179182=CARTESIAN_POINT('Ctrl Pts',(-23.8158300876213,-12.7916001552318,
114.862562812454)) ;
#179183=CARTESIAN_POINT('Ctrl Pts',(-23.7420262235532,-12.7916000714681,
114.886793791249)) ;
#179184=CARTESIAN_POINT('Ctrl Pts',(-23.7607111647796,-12.7449731642463,
114.943705109484)) ;
#179185=CARTESIAN_POINT('Ctrl Pts',(-23.7793961060059,-12.6983462570244,
115.000616427718)) ;
#179186=CARTESIAN_POINT('Ctrl Pts',(-23.8531999700739,-12.698346340788,
114.976385448923)) ;
#179187=CARTESIAN_POINT('Ctrl Pts',(-23.927003834142,-12.6983464245516,
114.952154470128)) ;
#179188=CARTESIAN_POINT('Ctrl Pts',(-23.9083188929157,-12.7449733317735,
114.895243151894)) ;
#179189=CARTESIAN_POINT('Ctrl Pts',(-23.8326075291051,-12.5424420519023,
114.700085714252)) ;
#179190=CARTESIAN_POINT('Ctrl Pts',(-23.81844720302,-12.6032785791417,114.656955643741)) ;
#179191=CARTESIAN_POINT('Ctrl Pts',(-23.7446433333702,-12.6032785174952,
114.681186605535)) ;
#179192=CARTESIAN_POINT('Ctrl Pts',(-23.6708394637203,-12.6032784558487,
114.705417567328)) ;
#179193=CARTESIAN_POINT('Ctrl Pts',(-23.6849997898054,-12.5424419286094,
114.748547637839)) ;
#179194=CARTESIAN_POINT('Ctrl Pts',(-23.6991601158905,-12.48160540137,114.79167770835)) ;
#179195=CARTESIAN_POINT('Ctrl Pts',(-23.7729639855403,-12.4816054630165,
114.767446746556)) ;
#179196=CARTESIAN_POINT('Ctrl Pts',(-23.8467678551901,-12.481605524663,
114.743215784762)) ;
#179197=CARTESIAN_POINT('Ctrl Pts',(-23.8326075291051,-12.5424420519023,
114.700085714252)) ;
#179198=CARTESIAN_POINT('Ctrl Pts',(-23.7423558200825,-12.4024494998622,
114.460690641158)) ;
#179199=CARTESIAN_POINT('Ctrl Pts',(-23.7337409088041,-12.4731509953254,
114.434451009471)) ;
#179200=CARTESIAN_POINT('Ctrl Pts',(-23.6599370360758,-12.4731509596195,
114.458681961889)) ;
#179201=CARTESIAN_POINT('Ctrl Pts',(-23.5861331633476,-12.4731509239136,
114.482912914306)) ;
#179202=CARTESIAN_POINT('Ctrl Pts',(-23.594748074626,-12.4024494284505,
114.509152545993)) ;
#179203=CARTESIAN_POINT('Ctrl Pts',(-23.6033629859044,-12.3317479329873,
114.535392177679)) ;
#179204=CARTESIAN_POINT('Ctrl Pts',(-23.6771668586326,-12.3317479686932,
114.511161225262)) ;
#179205=CARTESIAN_POINT('Ctrl Pts',(-23.7509707313608,-12.331748004399,
114.486930272844)) ;
#179206=CARTESIAN_POINT('Ctrl Pts',(-23.7423558200825,-12.4024494998622,
114.460690641158)) ;
#179207=CARTESIAN_POINT('Ctrl Pts',(-23.6437350301605,-12.33540698977,114.195676204108)) ;
#179208=CARTESIAN_POINT('Ctrl Pts',(-23.6412608759413,-12.4108950254445,
114.188140327696)) ;
#179209=CARTESIAN_POINT('Ctrl Pts',(-23.5674570025814,-12.4108950163572,
114.212371278189)) ;
#179210=CARTESIAN_POINT('Ctrl Pts',(-23.4936531292215,-12.4108950072698,
114.236602228683)) ;
#179211=CARTESIAN_POINT('Ctrl Pts',(-23.4961272834406,-12.3354069715953,
114.244138105095)) ;
#179212=CARTESIAN_POINT('Ctrl Pts',(-23.4986014376598,-12.2599189359207,
114.251673981507)) ;
#179213=CARTESIAN_POINT('Ctrl Pts',(-23.5724053110197,-12.2599189450081,
114.227443031014)) ;
#179214=CARTESIAN_POINT('Ctrl Pts',(-23.6462091843796,-12.2599189540954,
114.20321208052)) ;
#179215=CARTESIAN_POINT('Ctrl Pts',(-23.6437350301605,-12.33540698977,114.195676204108)) ;
#179216=CARTESIAN_POINT('Ctrl Pts',(-23.54230497616,-12.3455818235887,113.922252265825)) ;
#179217=CARTESIAN_POINT('Ctrl Pts',(-23.5461738202571,-12.4204731523851,
113.934036138957)) ;
#179218=CARTESIAN_POINT('Ctrl Pts',(-23.4723699490057,-12.4204731683141,
113.958267095873)) ;
#179219=CARTESIAN_POINT('Ctrl Pts',(-23.3985660777543,-12.4204731842432,
113.982498052789)) ;
#179220=CARTESIAN_POINT('Ctrl Pts',(-23.3946972336572,-12.3455818554468,
113.970714179657)) ;
#179221=CARTESIAN_POINT('Ctrl Pts',(-23.3908283895601,-12.2706905266504,
113.958930306525)) ;
#179222=CARTESIAN_POINT('Ctrl Pts',(-23.4646322608115,-12.2706905107213,
113.934699349609)) ;
#179223=CARTESIAN_POINT('Ctrl Pts',(-23.5384361320628,-12.2706904947923,
113.910468392693)) ;
#179224=CARTESIAN_POINT('Ctrl Pts',(-23.54230497616,-12.3455818235887,113.922252265825)) ;
#179225=CARTESIAN_POINT('Ctrl Pts',(-23.4449159493085,-12.433061741337,
113.661165866049)) ;
#179226=CARTESIAN_POINT('Ctrl Pts',(-23.4548546920134,-12.5019585481824,
113.691437671103)) ;
#179227=CARTESIAN_POINT('Ctrl Pts',(-23.3810508250872,-12.5019585842902,
113.715668641192)) ;
#179228=CARTESIAN_POINT('Ctrl Pts',(-23.307246958161,-12.501958620398,113.739899611282)) ;
#179229=CARTESIAN_POINT('Ctrl Pts',(-23.2973082154561,-12.4330618135526,
113.709627806229)) ;
#179230=CARTESIAN_POINT('Ctrl Pts',(-23.2873694727513,-12.3641650067072,
113.679356001175)) ;
#179231=CARTESIAN_POINT('Ctrl Pts',(-23.3611733396774,-12.3641649705994,
113.655125031086)) ;
#179232=CARTESIAN_POINT('Ctrl Pts',(-23.4349772066036,-12.3641649344917,
113.630894060996)) ;
#179233=CARTESIAN_POINT('Ctrl Pts',(-23.4449159493085,-12.433061741337,
113.661165866049)) ;
#179234=CARTESIAN_POINT('Ctrl Pts',(-23.3581859160956,-12.5907670484714,
113.432424558756)) ;
#179235=CARTESIAN_POINT('Ctrl Pts',(-23.3734620758896,-12.6487569748398,
113.478953275208)) ;
#179236=CARTESIAN_POINT('Ctrl Pts',(-23.2996582144225,-12.6487570251188,
113.503184261925)) ;
#179237=CARTESIAN_POINT('Ctrl Pts',(-23.2258543529553,-12.6487570753977,
113.527415248642)) ;
#179238=CARTESIAN_POINT('Ctrl Pts',(-23.2105781931613,-12.5907671490293,
113.48088653219)) ;
#179239=CARTESIAN_POINT('Ctrl Pts',(-23.1953020333673,-12.5327772226608,
113.434357815739)) ;
#179240=CARTESIAN_POINT('Ctrl Pts',(-23.2691058948344,-12.5327771723819,
113.410126829022)) ;
#179241=CARTESIAN_POINT('Ctrl Pts',(-23.3429097563016,-12.5327771221029,
113.385895842305)) ;
#179242=CARTESIAN_POINT('Ctrl Pts',(-23.3581859160956,-12.5907670484714,
113.432424558756)) ;
#179243=CARTESIAN_POINT('Ctrl Pts',(-23.2872506370322,-12.8072730343164,
113.25175834982)) ;
#179244=CARTESIAN_POINT('Ctrl Pts',(-23.3067702142274,-12.8502341493777,
113.31121183114)) ;
#179245=CARTESIAN_POINT('Ctrl Pts',(-23.2329663588169,-12.8502342073388,
113.335442836304)) ;
#179246=CARTESIAN_POINT('Ctrl Pts',(-23.1591625034065,-12.8502342652999,
113.359673841469)) ;
#179247=CARTESIAN_POINT('Ctrl Pts',(-23.1396429262112,-12.8072731502386,
113.300220360149)) ;
#179248=CARTESIAN_POINT('Ctrl Pts',(-23.120123349016,-12.7643120351774,
113.240766878829)) ;
#179249=CARTESIAN_POINT('Ctrl Pts',(-23.1939272044265,-12.7643119772163,
113.216535873664)) ;
#179250=CARTESIAN_POINT('Ctrl Pts',(-23.267731059837,-12.7643119192552,
113.192304868499)) ;
#179251=CARTESIAN_POINT('Ctrl Pts',(-23.2872506370322,-12.8072730343164,
113.25175834982)) ;
#179252=CARTESIAN_POINT('Ctrl Pts',(-23.2361882931638,-13.0681776762317,
113.131728504028)) ;
#179253=CARTESIAN_POINT('Ctrl Pts',(-23.2585681123116,-13.0929875781858,
113.199893821003)) ;
#179254=CARTESIAN_POINT('Ctrl Pts',(-23.1847642630524,-13.0929876362341,
113.224124844904)) ;
#179255=CARTESIAN_POINT('Ctrl Pts',(-23.1109604137933,-13.0929876942824,
113.248355868804)) ;
#179256=CARTESIAN_POINT('Ctrl Pts',(-23.0885805946455,-13.0681777923284,
113.18019055183)) ;
#179257=CARTESIAN_POINT('Ctrl Pts',(-23.0662007754978,-13.0433678903743,
113.112025234855)) ;
#179258=CARTESIAN_POINT('Ctrl Pts',(-23.1400046247569,-13.043367832326,
113.087794210954)) ;
#179259=CARTESIAN_POINT('Ctrl Pts',(-23.2138084740161,-13.0433677742776,
113.063563187054)) ;
#179260=CARTESIAN_POINT('Ctrl Pts',(-23.2361882931638,-13.0681776762317,
113.131728504028)) ;
#179261=CARTESIAN_POINT('Ctrl Pts',(-23.2082374843446,-13.3550287065478,
113.082188386664)) ;
#179262=CARTESIAN_POINT('Ctrl Pts',(-23.2318663981751,-13.3598480286535,
113.154158244693)) ;
#179263=CARTESIAN_POINT('Ctrl Pts',(-23.1580625540699,-13.3598480797462,
113.178389284292)) ;
#179264=CARTESIAN_POINT('Ctrl Pts',(-23.0842587099647,-13.3598481308389,
113.202620323891)) ;
#179265=CARTESIAN_POINT('Ctrl Pts',(-23.0606297961342,-13.3550288087332,
113.130650465862)) ;
#179266=CARTESIAN_POINT('Ctrl Pts',(-23.0370008823037,-13.3502094866275,
113.058680607834)) ;
#179267=CARTESIAN_POINT('Ctrl Pts',(-23.1108047264089,-13.3502094355348,
113.034449568235)) ;
#179268=CARTESIAN_POINT('Ctrl Pts',(-23.1846085705141,-13.3502093844422,
113.010218528636)) ;
#179269=CARTESIAN_POINT('Ctrl Pts',(-23.2082374843446,-13.3550287065478,
113.082188386664)) ;
#179270=CARTESIAN_POINT('Ctrl Pts',(-23.2046137347424,-13.6436167217993,
113.106398539743)) ;
#179271=CARTESIAN_POINT('Ctrl Pts',(-23.2278019241114,-13.6282936387258,
113.177026022299)) ;
#179272=CARTESIAN_POINT('Ctrl Pts',(-23.1539980837884,-13.6282936821549,
113.201257073418)) ;
#179273=CARTESIAN_POINT('Ctrl Pts',(-23.0801942434654,-13.6282937255841,
113.225488124537)) ;
#179274=CARTESIAN_POINT('Ctrl Pts',(-23.0570060540965,-13.6436168086577,
113.154860641981)) ;
#179275=CARTESIAN_POINT('Ctrl Pts',(-23.0338178647275,-13.6589398917312,
113.084233159425)) ;
#179276=CARTESIAN_POINT('Ctrl Pts',(-23.1076217050505,-13.6589398483021,
113.060002108306)) ;
#179277=CARTESIAN_POINT('Ctrl Pts',(-23.1814255453735,-13.6589398048729,
113.035771057187)) ;
#179278=CARTESIAN_POINT('Ctrl Pts',(-23.2046137347424,-13.6436167217993,
113.106398539743)) ;
#179279=CARTESIAN_POINT('Ctrl Pts',(-23.2246473462219,-13.9180811572707,
113.202915786182)) ;
#179280=CARTESIAN_POINT('Ctrl Pts',(-23.2457373765754,-13.8835710604602,
113.267152615087)) ;
#179281=CARTESIAN_POINT('Ctrl Pts',(-23.1719335384956,-13.8835710916854,
113.291383673039)) ;
#179282=CARTESIAN_POINT('Ctrl Pts',(-23.0981297004159,-13.8835711229105,
113.31561473099)) ;
#179283=CARTESIAN_POINT('Ctrl Pts',(-23.0770396700624,-13.918081219721,
113.251377902085)) ;
#179284=CARTESIAN_POINT('Ctrl Pts',(-23.055949639709,-13.9525913165315,
113.187141073179)) ;
#179285=CARTESIAN_POINT('Ctrl Pts',(-23.1297534777888,-13.9525912853064,
113.162910015228)) ;
#179286=CARTESIAN_POINT('Ctrl Pts',(-23.2035573158685,-13.9525912540812,
113.138678957277)) ;
#179287=CARTESIAN_POINT('Ctrl Pts',(-23.2246473462219,-13.9180811572707,
113.202915786182)) ;
#179288=CARTESIAN_POINT('Ctrl Pts',(-23.2663198478807,-14.156549136634,
113.365316344901)) ;
#179289=CARTESIAN_POINT('Ctrl Pts',(-23.2837980929174,-14.1053360637856,
113.418552258655)) ;
#179290=CARTESIAN_POINT('Ctrl Pts',(-23.2099942554152,-14.1053360831036,
113.442783318366)) ;
#179291=CARTESIAN_POINT('Ctrl Pts',(-23.1361904179131,-14.1053361024216,
113.467014378076)) ;
#179292=CARTESIAN_POINT('Ctrl Pts',(-23.1187121728764,-14.1565491752701,
113.413778464322)) ;
#179293=CARTESIAN_POINT('Ctrl Pts',(-23.1012339278397,-14.2077622481185,
113.360542550568)) ;
#179294=CARTESIAN_POINT('Ctrl Pts',(-23.1750377653419,-14.2077622288005,
113.336311490857)) ;
#179295=CARTESIAN_POINT('Ctrl Pts',(-23.248841602844,-14.2077622094825,
113.312080431146)) ;
#179296=CARTESIAN_POINT('Ctrl Pts',(-23.2663198478807,-14.156549136634,
113.365316344901)) ;
#179297=CARTESIAN_POINT('Ctrl Pts',(-23.3260277991125,-14.3423727651068,
113.58274099428)) ;
#179298=CARTESIAN_POINT('Ctrl Pts',(-23.3386275164003,-14.2781068691163,
113.621117699827)) ;
#179299=CARTESIAN_POINT('Ctrl Pts',(-23.2648236779677,-14.2781068782219,
113.645348756703)) ;
#179300=CARTESIAN_POINT('Ctrl Pts',(-23.191019839535,-14.2781068873274,
113.66957981358)) ;
#179301=CARTESIAN_POINT('Ctrl Pts',(-23.1784201222473,-14.342372783318,
113.631203108033)) ;
#179302=CARTESIAN_POINT('Ctrl Pts',(-23.1658204049595,-14.4066386793085,
113.592826402486)) ;
#179303=CARTESIAN_POINT('Ctrl Pts',(-23.2396242433921,-14.406638670203,
113.568595345609)) ;
#179304=CARTESIAN_POINT('Ctrl Pts',(-23.3134280818248,-14.4066386610974,
113.544364288733)) ;
#179305=CARTESIAN_POINT('Ctrl Pts',(-23.3260277991125,-14.3423727651068,
113.58274099428)) ;
#179306=CARTESIAN_POINT('Ctrl Pts',(-23.3982430302962,-14.4613427108393,
113.838084052962)) ;
#179307=CARTESIAN_POINT('Ctrl Pts',(-23.4050870415736,-14.3886728717829,
113.858929806808)) ;
#179308=CARTESIAN_POINT('Ctrl Pts',(-23.3312832017508,-14.3886728745372,
113.88316085945)) ;
#179309=CARTESIAN_POINT('Ctrl Pts',(-23.2574793619279,-14.3886728772916,
113.907391912092)) ;
#179310=CARTESIAN_POINT('Ctrl Pts',(-23.2506353506505,-14.461342716348,
113.886546158247)) ;
#179311=CARTESIAN_POINT('Ctrl Pts',(-23.243791339373,-14.5340125554044,
113.865700404401)) ;
#179312=CARTESIAN_POINT('Ctrl Pts',(-23.3175951791959,-14.5340125526501,
113.841469351759)) ;
#179313=CARTESIAN_POINT('Ctrl Pts',(-23.3913990190187,-14.5340125498957,
113.817238299117)) ;
#179314=CARTESIAN_POINT('Ctrl Pts',(-23.3982430302962,-14.4613427108393,
113.838084052962)) ;
#179315=CARTESIAN_POINT('Ctrl Pts',(-23.4778308247352,-14.5057889124528,
114.116110858595)) ;
#179316=CARTESIAN_POINT('Ctrl Pts',(-23.4783907365172,-14.4299056340327,
114.117816259447)) ;
#179317=CARTESIAN_POINT('Ctrl Pts',(-23.4045868946325,-14.4299056336396,
114.142047305809)) ;
#179318=CARTESIAN_POINT('Ctrl Pts',(-23.3307830527477,-14.4299056332465,
114.166278352171)) ;
#179319=CARTESIAN_POINT('Ctrl Pts',(-23.3302231409656,-14.5057889116665,
114.164572951319)) ;
#179320=CARTESIAN_POINT('Ctrl Pts',(-23.3296632291836,-14.5816721900866,
114.162867550466)) ;
#179321=CARTESIAN_POINT('Ctrl Pts',(-23.4034670710684,-14.5816721904797,
114.138636504104)) ;
#179322=CARTESIAN_POINT('Ctrl Pts',(-23.4772709129532,-14.5816721908728,
114.114405457742)) ;
#179323=CARTESIAN_POINT('Ctrl Pts',(-23.4778308247352,-14.5057889124528,
114.116110858595)) ;
#179324=CARTESIAN_POINT('Ctrl Pts',(-23.5571252249388,-14.4724226584541,
114.392900262027)) ;
#179325=CARTESIAN_POINT('Ctrl Pts',(-23.5514192768126,-14.3987559090156,
114.375520864663)) ;
#179326=CARTESIAN_POINT('Ctrl Pts',(-23.4776154337327,-14.3987559084173,
114.399751907385)) ;
#179327=CARTESIAN_POINT('Ctrl Pts',(-23.4038115906528,-14.3987559078189,
114.423982950107)) ;
#179328=CARTESIAN_POINT('Ctrl Pts',(-23.4095175387789,-14.4724226572574,
114.44136234747)) ;
#179329=CARTESIAN_POINT('Ctrl Pts',(-23.4152234869051,-14.5460894066958,
114.458741744834)) ;
#179330=CARTESIAN_POINT('Ctrl Pts',(-23.489027329985,-14.5460894072942,
114.434510702113)) ;
#179331=CARTESIAN_POINT('Ctrl Pts',(-23.5628311730649,-14.5460894078926,
114.410279659391)) ;
#179332=CARTESIAN_POINT('Ctrl Pts',(-23.5571252249388,-14.4724226584541,
114.392900262027)) ;
#179333=CARTESIAN_POINT('Ctrl Pts',(-23.6311473330998,-14.3630839653471,
114.653969620511)) ;
#179334=CARTESIAN_POINT('Ctrl Pts',(-23.6195269569882,-14.2969416918189,
114.618575829864)) ;
#179335=CARTESIAN_POINT('Ctrl Pts',(-23.5457231128652,-14.2969416928651,
114.642806869409)) ;
#179336=CARTESIAN_POINT('Ctrl Pts',(-23.4719192687422,-14.2969416939113,
114.667037908954)) ;
#179337=CARTESIAN_POINT('Ctrl Pts',(-23.4835396448539,-14.3630839674395,
114.702431699601)) ;
#179338=CARTESIAN_POINT('Ctrl Pts',(-23.4951600209655,-14.4292262409677,
114.737825490247)) ;
#179339=CARTESIAN_POINT('Ctrl Pts',(-23.5689638650885,-14.4292262399216,
114.713594450703)) ;
#179340=CARTESIAN_POINT('Ctrl Pts',(-23.6427677092115,-14.4292262388754,
114.689363411158)) ;
#179341=CARTESIAN_POINT('Ctrl Pts',(-23.6311473330998,-14.3630839653471,
114.653969620511)) ;
#179342=CARTESIAN_POINT('Ctrl Pts',(-23.6926670750486,-14.1865023299291,
114.87674421223)) ;
#179343=CARTESIAN_POINT('Ctrl Pts',(-23.6760010931989,-14.132592518795,
114.825982320627)) ;
#179344=CARTESIAN_POINT('Ctrl Pts',(-23.6021972490565,-14.1325925211688,
114.850213360112)) ;
#179345=CARTESIAN_POINT('Ctrl Pts',(-23.528393404914,-14.1325925235426,
114.874444399598)) ;
#179346=CARTESIAN_POINT('Ctrl Pts',(-23.5450593867637,-14.1865023346767,
114.925206291201)) ;
#179347=CARTESIAN_POINT('Ctrl Pts',(-23.5617253686134,-14.2404121458108,
114.975968182805)) ;
#179348=CARTESIAN_POINT('Ctrl Pts',(-23.6355292127559,-14.240412143437,
114.95173714332)) ;
#179349=CARTESIAN_POINT('Ctrl Pts',(-23.7093330568983,-14.2404121410632,
114.927506103834)) ;
#179350=CARTESIAN_POINT('Ctrl Pts',(-23.6926670750486,-14.1865023299291,
114.87674421223)) ;
#179351=CARTESIAN_POINT('Ctrl Pts',(-23.737109657086,-13.9552367476643,
115.047514669265)) ;
#179352=CARTESIAN_POINT('Ctrl Pts',(-23.7165830285528,-13.91739633188,114.98499387076)) ;
#179353=CARTESIAN_POINT('Ctrl Pts',(-23.6427791848163,-13.917396334111,
115.009224911482)) ;
#179354=CARTESIAN_POINT('Ctrl Pts',(-23.5689753410797,-13.9173963363419,
115.033455952203)) ;
#179355=CARTESIAN_POINT('Ctrl Pts',(-23.5895019696129,-13.9552367521262,
115.095976750709)) ;
#179356=CARTESIAN_POINT('Ctrl Pts',(-23.6100285981462,-13.9930771679105,
115.158497549214)) ;
#179357=CARTESIAN_POINT('Ctrl Pts',(-23.6838324418827,-13.9930771656796,
115.134266508492)) ;
#179358=CARTESIAN_POINT('Ctrl Pts',(-23.7576362856192,-13.9930771634486,
115.110035467771)) ;
#179359=CARTESIAN_POINT('Ctrl Pts',(-23.737109657086,-13.9552367476643,
115.047514669265)) ;
#179360=CARTESIAN_POINT('Ctrl Pts',(-23.7605010634612,-13.6844063432408,
115.1543055001)) ;
#179361=CARTESIAN_POINT('Ctrl Pts',(-23.7375752646493,-13.6654217630373,
115.084477215966)) ;
#179362=CARTESIAN_POINT('Ctrl Pts',(-23.6637714214189,-13.6654217622708,
115.10870825823)) ;
#179363=CARTESIAN_POINT('Ctrl Pts',(-23.5899675781886,-13.6654217615044,
115.132939300493)) ;
#179364=CARTESIAN_POINT('Ctrl Pts',(-23.6128933770005,-13.6844063417079,
115.202767584627)) ;
#179365=CARTESIAN_POINT('Ctrl Pts',(-23.6358191758124,-13.7033909219114,
115.272595868762)) ;
#179366=CARTESIAN_POINT('Ctrl Pts',(-23.7096230190428,-13.7033909226779,
115.248364826498)) ;
#179367=CARTESIAN_POINT('Ctrl Pts',(-23.7834268622731,-13.7033909234443,
115.224133784235)) ;
#179368=CARTESIAN_POINT('Ctrl Pts',(-23.7605010634612,-13.6844063432408,
115.1543055001)) ;
#179369=CARTESIAN_POINT('Ctrl Pts',(-23.760236922336,-13.395616216205,115.188901213406)) ;
#179370=CARTESIAN_POINT('Ctrl Pts',(-23.7365635501868,-13.3967687826649,
115.116795941421)) ;
#179371=CARTESIAN_POINT('Ctrl Pts',(-23.6627597068722,-13.3967687773501,
115.141026983428)) ;
#179372=CARTESIAN_POINT('Ctrl Pts',(-23.5889558635576,-13.3967687720353,
115.165258025435)) ;
#179373=CARTESIAN_POINT('Ctrl Pts',(-23.6126292357068,-13.3956162055754,
115.23736329742)) ;
#179374=CARTESIAN_POINT('Ctrl Pts',(-23.6363026078559,-13.3944636391155,
115.309468569405)) ;
#179375=CARTESIAN_POINT('Ctrl Pts',(-23.7101064511705,-13.3944636444303,
115.285237527398)) ;
#179376=CARTESIAN_POINT('Ctrl Pts',(-23.7839102944851,-13.3944636497451,
115.261006485391)) ;
#179377=CARTESIAN_POINT('Ctrl Pts',(-23.760236922336,-13.395616216205,115.188901213406)) ;
#179378=CARTESIAN_POINT('Ctrl Pts',(-23.7358042656124,-13.1080920804484,
115.149918807693)) ;
#179379=CARTESIAN_POINT('Ctrl Pts',(-23.7130691272017,-13.1293224287734,
115.080671244182)) ;
#179380=CARTESIAN_POINT('Ctrl Pts',(-23.6392652830181,-13.1293224180304,
115.104902283542)) ;
#179381=CARTESIAN_POINT('Ctrl Pts',(-23.5654614388346,-13.1293224072874,
115.129133322903)) ;
#179382=CARTESIAN_POINT('Ctrl Pts',(-23.5881965772453,-13.1080920589624,
115.198380886413)) ;
#179383=CARTESIAN_POINT('Ctrl Pts',(-23.610931715656,-13.0868617106374,
115.267628449924)) ;
#179384=CARTESIAN_POINT('Ctrl Pts',(-23.6847355598396,-13.0868617213805,
115.243397410564)) ;
#179385=CARTESIAN_POINT('Ctrl Pts',(-23.7585394040231,-13.0868617321235,
115.219166371203)) ;
#179386=CARTESIAN_POINT('Ctrl Pts',(-23.7358042656124,-13.1080920804484,
115.149918807693)) ;
#179387=CARTESIAN_POINT('Ctrl Pts',(-23.6876957397051,-12.8414911099526,
115.039017564153)) ;
#179388=CARTESIAN_POINT('Ctrl Pts',(-23.6675492663887,-12.8813675737048,
114.977654656676)) ;
#179389=CARTESIAN_POINT('Ctrl Pts',(-23.5937454199294,-12.8813675568765,
115.001885689105)) ;
#179390=CARTESIAN_POINT('Ctrl Pts',(-23.5199415734701,-12.8813675400482,
115.026116721534)) ;
#179391=CARTESIAN_POINT('Ctrl Pts',(-23.5400880467865,-12.8414910762961,
115.08747962901)) ;
#179392=CARTESIAN_POINT('Ctrl Pts',(-23.5602345201028,-12.8016146125439,
115.148842536487)) ;
#179393=CARTESIAN_POINT('Ctrl Pts',(-23.6340383665621,-12.8016146293722,
115.124611504058)) ;
#179394=CARTESIAN_POINT('Ctrl Pts',(-23.7078422130214,-12.8016146462005,
115.10038047163)) ;
#179395=CARTESIAN_POINT('Ctrl Pts',(-23.6876957397051,-12.8414911099526,
115.039017564153)) ;
#179396=CARTESIAN_POINT('Ctrl Pts',(-23.6196197911873,-12.6185827250958,
114.866926329754)) ;
#179397=CARTESIAN_POINT('Ctrl Pts',(-23.6034678707082,-12.6740802978787,
114.817730185585)) ;
#179398=CARTESIAN_POINT('Ctrl Pts',(-23.5296640215903,-12.6740802801009,
114.841961209916)) ;
#179399=CARTESIAN_POINT('Ctrl Pts',(-23.4558601724725,-12.674080262323,
114.866192234247)) ;
#179400=CARTESIAN_POINT('Ctrl Pts',(-23.4720120929516,-12.6185826895401,
114.915388378416)) ;
#179401=CARTESIAN_POINT('Ctrl Pts',(-23.4881640134308,-12.5630851167572,
114.964584522586)) ;
#179402=CARTESIAN_POINT('Ctrl Pts',(-23.5619678625486,-12.563085134535,
114.940353498254)) ;
#179403=CARTESIAN_POINT('Ctrl Pts',(-23.6357717116664,-12.5630851523128,
114.916122473923)) ;
#179404=CARTESIAN_POINT('Ctrl Pts',(-23.6196197911873,-12.6185827250958,
114.866926329754)) ;
#179405=CARTESIAN_POINT('Ctrl Pts',(-23.5344644232555,-12.4509854490646,
114.643132785995)) ;
#179406=CARTESIAN_POINT('Ctrl Pts',(-23.5234985411404,-12.518265407944,
114.609732477738)) ;
#179407=CARTESIAN_POINT('Ctrl Pts',(-23.4496946881903,-12.5182653912533,
114.633963490396)) ;
#179408=CARTESIAN_POINT('Ctrl Pts',(-23.3758908352401,-12.5182653745627,
114.658194503055)) ;
#179409=CARTESIAN_POINT('Ctrl Pts',(-23.3868567173552,-12.4509854156833,
114.691594811312)) ;
#179410=CARTESIAN_POINT('Ctrl Pts',(-23.3978225994702,-12.383705456804,
114.72499511957)) ;
#179411=CARTESIAN_POINT('Ctrl Pts',(-23.4716264524203,-12.3837054734946,
114.700764106911)) ;
#179412=CARTESIAN_POINT('Ctrl Pts',(-23.5454303053705,-12.3837054901852,
114.676533094252)) ;
#179413=CARTESIAN_POINT('Ctrl Pts',(-23.5344644232555,-12.4509854490646,
114.643132785995)) ;
#179414=CARTESIAN_POINT('Ctrl Pts',(-23.4384531446303,-12.3534810644787,
114.386130027561)) ;
#179415=CARTESIAN_POINT('Ctrl Pts',(-23.4334417543044,-12.427665920119,
114.370866140378)) ;
#179416=CARTESIAN_POINT('Ctrl Pts',(-23.3596378977513,-12.4276659104835,
114.395097142063)) ;
#179417=CARTESIAN_POINT('Ctrl Pts',(-23.2858340411983,-12.4276659008479,
114.419328143747)) ;
#179418=CARTESIAN_POINT('Ctrl Pts',(-23.2908454315242,-12.3534810452076,
114.43459203093)) ;
#179419=CARTESIAN_POINT('Ctrl Pts',(-23.2958568218501,-12.2792961895673,
114.449855918113)) ;
#179420=CARTESIAN_POINT('Ctrl Pts',(-23.3696606784032,-12.2792961992029,
114.425624916429)) ;
#179421=CARTESIAN_POINT('Ctrl Pts',(-23.4434645349562,-12.2792962088384,
114.401393914744)) ;
#179422=CARTESIAN_POINT('Ctrl Pts',(-23.4384531446303,-12.3534810644787,
114.386130027561)) ;
#179423=CARTESIAN_POINT('Ctrl Pts',(-23.3373005505562,-12.3320089256095,
114.113522831925)) ;
#179424=CARTESIAN_POINT('Ctrl Pts',(-23.3386099896682,-12.407800207037,
114.117511171175)) ;
#179425=CARTESIAN_POINT('Ctrl Pts',(-23.2648061300108,-12.407800209429,
114.141742163405)) ;
#179426=CARTESIAN_POINT('Ctrl Pts',(-23.1910022703534,-12.4078002118209,
114.165973155634)) ;
#179427=CARTESIAN_POINT('Ctrl Pts',(-23.1896928312415,-12.3320089303934,
114.161984816384)) ;
#179428=CARTESIAN_POINT('Ctrl Pts',(-23.1883833921295,-12.2562176489658,
114.157996477134)) ;
#179429=CARTESIAN_POINT('Ctrl Pts',(-23.2621872517869,-12.2562176465738,
114.133765484905)) ;
#179430=CARTESIAN_POINT('Ctrl Pts',(-23.3359911114443,-12.2562176441819,
114.109534492675)) ;
#179431=CARTESIAN_POINT('Ctrl Pts',(-23.3373005505562,-12.3320089256095,
114.113522831925)) ;
#179432=CARTESIAN_POINT('Ctrl Pts',(-23.2376722572993,-12.3884256006082,
113.845536510079)) ;
#179433=CARTESIAN_POINT('Ctrl Pts',(-23.2452056301701,-12.4603875127443,
113.868481947164)) ;
#179434=CARTESIAN_POINT('Ctrl Pts',(-23.1714017687528,-12.4603875316984,
113.892712934033)) ;
#179435=CARTESIAN_POINT('Ctrl Pts',(-23.0975979073355,-12.4603875506525,
113.916943920902)) ;
#179436=CARTESIAN_POINT('Ctrl Pts',(-23.0900645344648,-12.3884256385165,
113.893998483817)) ;
#179437=CARTESIAN_POINT('Ctrl Pts',(-23.0825311615941,-12.3164637263805,
113.871053046732)) ;
#179438=CARTESIAN_POINT('Ctrl Pts',(-23.1563350230114,-12.3164637074263,
113.846822059863)) ;
#179439=CARTESIAN_POINT('Ctrl Pts',(-23.2301388844286,-12.3164636884722,
113.822591072994)) ;
#179440=CARTESIAN_POINT('Ctrl Pts',(-23.2376722572993,-12.3884256006082,
113.845536510079)) ;
#179441=CARTESIAN_POINT('Ctrl Pts',(-23.1459449956219,-12.5185566369419,
113.601605269859)) ;
#179442=CARTESIAN_POINT('Ctrl Pts',(-23.1591598321752,-12.5815371501028,
113.641855528462)) ;
#179443=CARTESIAN_POINT('Ctrl Pts',(-23.0853559708827,-12.5815371883386,
113.666086515711)) ;
#179444=CARTESIAN_POINT('Ctrl Pts',(-23.0115521095902,-12.5815372265744,
113.69031750296)) ;
#179445=CARTESIAN_POINT('Ctrl Pts',(-22.9983372730369,-12.5185567134136,
113.650067244357)) ;
#179446=CARTESIAN_POINT('Ctrl Pts',(-22.9851224364836,-12.4555762002527,
113.609816985754)) ;
#179447=CARTESIAN_POINT('Ctrl Pts',(-23.0589262977762,-12.4555761620169,
113.585585998505)) ;
#179448=CARTESIAN_POINT('Ctrl Pts',(-23.1327301590687,-12.4555761237811,
113.561355011256)) ;
#179449=CARTESIAN_POINT('Ctrl Pts',(-23.1459449956219,-12.5185566369419,
113.601605269859)) ;
#179450=CARTESIAN_POINT('Ctrl Pts',(-23.0678884204578,-12.7128146761132,
113.399287149443)) ;
#179451=CARTESIAN_POINT('Ctrl Pts',(-23.0858389718743,-12.7623237651114,
113.453961631268)) ;
#179452=CARTESIAN_POINT('Ctrl Pts',(-23.0120351128278,-12.7623238229043,
113.478192625358)) ;
#179453=CARTESIAN_POINT('Ctrl Pts',(-22.9382312537813,-12.7623238806971,
113.502423619448)) ;
#179454=CARTESIAN_POINT('Ctrl Pts',(-22.9202807023649,-12.7128147916989,
113.447749137622)) ;
#179455=CARTESIAN_POINT('Ctrl Pts',(-22.9023301509484,-12.6633057027007,
113.393074655797)) ;
#179456=CARTESIAN_POINT('Ctrl Pts',(-22.9761340099949,-12.6633056449079,
113.368843661707)) ;
#179457=CARTESIAN_POINT('Ctrl Pts',(-23.0499378690414,-12.663305587115,
113.344612667617)) ;
#179458=CARTESIAN_POINT('Ctrl Pts',(-23.0678884204578,-12.7128146761132,
113.399287149443)) ;
#179459=CARTESIAN_POINT('Ctrl Pts',(-23.0080726213499,-12.9591843124397,
113.25274040277)) ;
#179460=CARTESIAN_POINT('Ctrl Pts',(-23.0294880013055,-12.9915649142031,
113.317968193112)) ;
#179461=CARTESIAN_POINT('Ctrl Pts',(-22.9556841465484,-12.9915649910661,
113.342199200267)) ;
#179462=CARTESIAN_POINT('Ctrl Pts',(-22.8818802917913,-12.9915650679292,
113.366430207422)) ;
#179463=CARTESIAN_POINT('Ctrl Pts',(-22.8604649118357,-12.9591844661657,
113.30120241708)) ;
#179464=CARTESIAN_POINT('Ctrl Pts',(-22.8390495318801,-12.9268038644023,
113.235974626737)) ;
#179465=CARTESIAN_POINT('Ctrl Pts',(-22.9128533866372,-12.9268037875393,
113.211743619582)) ;
#179466=CARTESIAN_POINT('Ctrl Pts',(-22.9866572413943,-12.9268037106763,
113.187512612428)) ;
#179467=CARTESIAN_POINT('Ctrl Pts',(-23.0080726213499,-12.9591843124397,
113.25274040277)) ;
#179468=CARTESIAN_POINT('Ctrl Pts',(-22.9707781839292,-13.2359003760254,
113.174438606138)) ;
#179469=CARTESIAN_POINT('Ctrl Pts',(-22.9940981173892,-13.2490083473187,
113.245467359058)) ;
#179470=CARTESIAN_POINT('Ctrl Pts',(-22.9202942691491,-13.24900843612,113.269698386062)) ;
#179471=CARTESIAN_POINT('Ctrl Pts',(-22.8464904209091,-13.2490085249213,
113.293929413067)) ;
#179472=CARTESIAN_POINT('Ctrl Pts',(-22.8231704874491,-13.235900553628,
113.222900660147)) ;
#179473=CARTESIAN_POINT('Ctrl Pts',(-22.7998505539891,-13.2227925823347,
113.151871907227)) ;
#179474=CARTESIAN_POINT('Ctrl Pts',(-22.8736544022292,-13.2227924935334,
113.127640880223)) ;
#179475=CARTESIAN_POINT('Ctrl Pts',(-22.9474582504692,-13.2227924047321,
113.103409853218)) ;
#179476=CARTESIAN_POINT('Ctrl Pts',(-22.9707781839292,-13.2359003760254,
113.174438606138)) ;
#179477=CARTESIAN_POINT('Ctrl Pts',(-22.9571487392571,-13.5269168879405,
113.168395654949)) ;
#179478=CARTESIAN_POINT('Ctrl Pts',(-22.9807202921007,-13.5197262961672,
113.240190799802)) ;
#179479=CARTESIAN_POINT('Ctrl Pts',(-22.9069164515481,-13.5197263915446,
113.264421850221)) ;
#179480=CARTESIAN_POINT('Ctrl Pts',(-22.8331126109954,-13.5197264869221,
113.28865290064)) ;
#179481=CARTESIAN_POINT('Ctrl Pts',(-22.8095410581518,-13.5269170786954,
113.216857755787)) ;
#179482=CARTESIAN_POINT('Ctrl Pts',(-22.7859695053082,-13.5341076704686,
113.145062610933)) ;
#179483=CARTESIAN_POINT('Ctrl Pts',(-22.8597733458609,-13.5341075750912,
113.120831560514)) ;
#179484=CARTESIAN_POINT('Ctrl Pts',(-22.9335771864135,-13.5341074797137,
113.096600510095)) ;
#179485=CARTESIAN_POINT('Ctrl Pts',(-22.9571487392571,-13.5269168879405,
113.168395654949)) ;
#179486=CARTESIAN_POINT('Ctrl Pts',(-22.9677330810903,-13.8100818853549,
113.236088284649)) ;
#179487=CARTESIAN_POINT('Ctrl Pts',(-22.9898665157146,-13.7831112951298,
113.303503153356)) ;
#179488=CARTESIAN_POINT('Ctrl Pts',(-22.9160626835003,-13.7831113889682,
113.327734229173)) ;
#179489=CARTESIAN_POINT('Ctrl Pts',(-22.8422588512859,-13.7831114828066,
113.351965304989)) ;
#179490=CARTESIAN_POINT('Ctrl Pts',(-22.8201254166616,-13.8100820730318,
113.284550436281)) ;
#179491=CARTESIAN_POINT('Ctrl Pts',(-22.7979919820373,-13.837052663257,
113.217135567573)) ;
#179492=CARTESIAN_POINT('Ctrl Pts',(-22.8717958142516,-13.8370525694185,
113.192904491757)) ;
#179493=CARTESIAN_POINT('Ctrl Pts',(-22.945599646466,-13.8370524755801,
113.168673415941)) ;
#179494=CARTESIAN_POINT('Ctrl Pts',(-22.9677330810903,-13.8100818853549,
113.236088284649)) ;
#179495=CARTESIAN_POINT('Ctrl Pts',(-23.0011086677166,-14.0658493622321,
113.373303697314)) ;
#179496=CARTESIAN_POINT('Ctrl Pts',(-23.0202087390422,-14.0209825335161,
113.431479430768)) ;
#179497=CARTESIAN_POINT('Ctrl Pts',(-22.9464049149718,-14.0209826175788,
113.455710531389)) ;
#179498=CARTESIAN_POINT('Ctrl Pts',(-22.8726010909013,-14.0209827016415,
113.479941632011)) ;
#179499=CARTESIAN_POINT('Ctrl Pts',(-22.8535010195757,-14.0658495303575,
113.421765898557)) ;
#179500=CARTESIAN_POINT('Ctrl Pts',(-22.8344009482501,-14.1107163590735,
113.363590165103)) ;
#179501=CARTESIAN_POINT('Ctrl Pts',(-22.9082047723206,-14.1107162750108,
113.339359064481)) ;
#179502=CARTESIAN_POINT('Ctrl Pts',(-22.982008596391,-14.1107161909481,
113.31512796386)) ;
#179503=CARTESIAN_POINT('Ctrl Pts',(-23.0011086677166,-14.0658493622321,
113.373303697314)) ;
#179504=CARTESIAN_POINT('Ctrl Pts',(-23.0539725203832,-14.2744004374724,
113.569778136137)) ;
#179505=CARTESIAN_POINT('Ctrl Pts',(-23.0686762202321,-14.2149073780421,
113.614563231378)) ;
#179506=CARTESIAN_POINT('Ctrl Pts',(-22.9948724030358,-14.2149074440193,
113.638794352937)) ;
#179507=CARTESIAN_POINT('Ctrl Pts',(-22.9210685858396,-14.2149075099964,
113.663025474496)) ;
#179508=CARTESIAN_POINT('Ctrl Pts',(-22.9063648859907,-14.2744005694268,
113.618240379255)) ;
#179509=CARTESIAN_POINT('Ctrl Pts',(-22.8916611861419,-14.3338936288571,
113.573455284013)) ;
#179510=CARTESIAN_POINT('Ctrl Pts',(-22.9654650033381,-14.3338935628799,
113.549224162454)) ;
#179511=CARTESIAN_POINT('Ctrl Pts',(-23.0392688205343,-14.3338934969028,
113.524993040895)) ;
#179512=CARTESIAN_POINT('Ctrl Pts',(-23.0539725203832,-14.2744004374724,
113.569778136137)) ;
#179513=CARTESIAN_POINT('Ctrl Pts',(-23.1216893204055,-14.4215076088756,
113.811439149396)) ;
#179514=CARTESIAN_POINT('Ctrl Pts',(-23.1309543238125,-14.3516564443396,
113.839658852781)) ;
#179515=CARTESIAN_POINT('Ctrl Pts',(-23.0571505115092,-14.3516564861261,
113.863889989243)) ;
#179516=CARTESIAN_POINT('Ctrl Pts',(-22.9833466992058,-14.3516565279127,
113.888121125705)) ;
#179517=CARTESIAN_POINT('Ctrl Pts',(-22.9740816957989,-14.4215076924487,
113.85990142232)) ;
#179518=CARTESIAN_POINT('Ctrl Pts',(-22.9648166923919,-14.4913588569847,
113.831681718935)) ;
#179519=CARTESIAN_POINT('Ctrl Pts',(-23.0386205046952,-14.4913588151982,
113.807450582473)) ;
#179520=CARTESIAN_POINT('Ctrl Pts',(-23.1124243169985,-14.4913587734116,
113.783219446011)) ;
#179521=CARTESIAN_POINT('Ctrl Pts',(-23.1216893204055,-14.4215076088756,
113.811439149396)) ;
#179522=CARTESIAN_POINT('Ctrl Pts',(-23.1988440710271,-14.4970287487176,
114.081882466236)) ;
#179523=CARTESIAN_POINT('Ctrl Pts',(-23.2020027620207,-14.421801684016,
114.091503327255)) ;
#179524=CARTESIAN_POINT('Ctrl Pts',(-23.1281989521545,-14.42180169783,114.11573447114)) ;
#179525=CARTESIAN_POINT('Ctrl Pts',(-23.0543951422883,-14.421801711644,
114.139965615025)) ;
#179526=CARTESIAN_POINT('Ctrl Pts',(-23.0512364512947,-14.4970287763456,
114.130344754007)) ;
#179527=CARTESIAN_POINT('Ctrl Pts',(-23.0480777603011,-14.5722558410471,
114.120723892988)) ;
#179528=CARTESIAN_POINT('Ctrl Pts',(-23.1218815701673,-14.5722558272332,
114.096492749103)) ;
#179529=CARTESIAN_POINT('Ctrl Pts',(-23.1956853800335,-14.5722558134192,
114.072261605218)) ;
#179530=CARTESIAN_POINT('Ctrl Pts',(-23.1988440710271,-14.4970287487176,
114.081882466236)) ;
#179531=CARTESIAN_POINT('Ctrl Pts',(-23.2792349709217,-14.495364180026,
114.362233916425)) ;
#179532=CARTESIAN_POINT('Ctrl Pts',(-23.2760513537556,-14.420141562785,
114.352537130133)) ;
#179533=CARTESIAN_POINT('Ctrl Pts',(-23.202247543564,-14.4201415475385,
114.376768273027)) ;
#179534=CARTESIAN_POINT('Ctrl Pts',(-23.1284437333723,-14.420141532292,
114.400999415921)) ;
#179535=CARTESIAN_POINT('Ctrl Pts',(-23.1316273505383,-14.495364149533,
114.410696202213)) ;
#179536=CARTESIAN_POINT('Ctrl Pts',(-23.1348109677044,-14.570586766774,
114.420392988505)) ;
#179537=CARTESIAN_POINT('Ctrl Pts',(-23.2086147778961,-14.5705867820204,
114.396161845611)) ;
#179538=CARTESIAN_POINT('Ctrl Pts',(-23.2824185880877,-14.5705867972669,
114.371930702717)) ;
#179539=CARTESIAN_POINT('Ctrl Pts',(-23.2792349709217,-14.495364180026,
114.362233916425)) ;
#179540=CARTESIAN_POINT('Ctrl Pts',(-23.3563637359517,-14.4159600881982,
114.632728072821)) ;
#179541=CARTESIAN_POINT('Ctrl Pts',(-23.3470544555899,-14.3461687677575,
114.604373504854)) ;
#179542=CARTESIAN_POINT('Ctrl Pts',(-23.2732506422362,-14.346168725633,
114.628604638116)) ;
#179543=CARTESIAN_POINT('Ctrl Pts',(-23.1994468288825,-14.3461686835086,
114.652835771379)) ;
#179544=CARTESIAN_POINT('Ctrl Pts',(-23.2087561092442,-14.4159600039494,
114.681190339346)) ;
#179545=CARTESIAN_POINT('Ctrl Pts',(-23.2180653896059,-14.4857513243901,
114.709544907314)) ;
#179546=CARTESIAN_POINT('Ctrl Pts',(-23.2918692029597,-14.4857513665145,
114.685313774051)) ;
#179547=CARTESIAN_POINT('Ctrl Pts',(-23.3656730163134,-14.485751408639,
114.661082640788)) ;
#179548=CARTESIAN_POINT('Ctrl Pts',(-23.3563637359517,-14.4159600881982,
114.632728072821)) ;
#179549=CARTESIAN_POINT('Ctrl Pts',(-23.4233024681412,-14.2660479877099,
114.871922390373)) ;
#179550=CARTESIAN_POINT('Ctrl Pts',(-23.4085752084141,-14.2066193411526,
114.827065531498)) ;
#179551=CARTESIAN_POINT('Ctrl Pts',(-23.3347713898697,-14.206619276698,
114.85129664895)) ;
#179552=CARTESIAN_POINT('Ctrl Pts',(-23.2609675713253,-14.2066192122434,
114.875527766403)) ;
#179553=CARTESIAN_POINT('Ctrl Pts',(-23.2756948310523,-14.2660478588008,
114.920384625278)) ;
#179554=CARTESIAN_POINT('Ctrl Pts',(-23.2904220907793,-14.3254765053581,
114.965241484154)) ;
#179555=CARTESIAN_POINT('Ctrl Pts',(-23.3642259093238,-14.3254765698126,
114.941010366701)) ;
#179556=CARTESIAN_POINT('Ctrl Pts',(-23.4380297278682,-14.3254766342672,
114.916779249248)) ;
#179557=CARTESIAN_POINT('Ctrl Pts',(-23.4233024681412,-14.2660479877099,
114.871922390373)) ;
#179558=CARTESIAN_POINT('Ctrl Pts',(-23.4754105644669,-14.0549162780305,
115.066119893745)) ;
#179559=CARTESIAN_POINT('Ctrl Pts',(-23.4562889637978,-14.010139153776,
115.007878581465)) ;
#179560=CARTESIAN_POINT('Ctrl Pts',(-23.3824851382236,-14.0101390737133,
115.032109677506)) ;
#179561=CARTESIAN_POINT('Ctrl Pts',(-23.3086813126494,-14.0101389936507,
115.056340773547)) ;
#179562=CARTESIAN_POINT('Ctrl Pts',(-23.3278029133185,-14.0549161179053,
115.114582085827)) ;
#179563=CARTESIAN_POINT('Ctrl Pts',(-23.3469245139876,-14.0996932421598,
115.172823398108)) ;
#179564=CARTESIAN_POINT('Ctrl Pts',(-23.4207283395618,-14.0996933222224,
115.148592302067)) ;
#179565=CARTESIAN_POINT('Ctrl Pts',(-23.494532165136,-14.0996934022851,
115.124361206026)) ;
#179566=CARTESIAN_POINT('Ctrl Pts',(-23.4754105644669,-14.0549162780305,
115.066119893745)) ;
#179567=CARTESIAN_POINT('Ctrl Pts',(-23.5077572471595,-13.7973888984154,
115.200198351239)) ;
#179568=CARTESIAN_POINT('Ctrl Pts',(-23.4856127499084,-13.7705242930268,
115.132749783824)) ;
#179569=CARTESIAN_POINT('Ctrl Pts',(-23.4118089164229,-13.7705242060614,
115.156980855769)) ;
#179570=CARTESIAN_POINT('Ctrl Pts',(-23.3380050829375,-13.770524119096,
115.181211927714)) ;
#179571=CARTESIAN_POINT('Ctrl Pts',(-23.3601495801886,-13.7973887244846,
115.248660495129)) ;
#179572=CARTESIAN_POINT('Ctrl Pts',(-23.3822940774398,-13.8242533298732,
115.316109062544)) ;
#179573=CARTESIAN_POINT('Ctrl Pts',(-23.4560979109252,-13.8242534168386,
115.291877990599)) ;
#179574=CARTESIAN_POINT('Ctrl Pts',(-23.5299017444107,-13.824253503804,
115.267646918654)) ;
#179575=CARTESIAN_POINT('Ctrl Pts',(-23.5077572471595,-13.7973888984154,
115.200198351239)) ;
#179576=CARTESIAN_POINT('Ctrl Pts',(-23.5172572061641,-13.5143192821472,
115.264479052943)) ;
#179577=CARTESIAN_POINT('Ctrl Pts',(-23.4936848178715,-13.5071778533561,
115.192681359907)) ;
#179578=CARTESIAN_POINT('Ctrl Pts',(-23.4198809766881,-13.507177766311,
115.216912408405)) ;
#179579=CARTESIAN_POINT('Ctrl Pts',(-23.3460771355048,-13.5071776792659,
115.241143456903)) ;
#179580=CARTESIAN_POINT('Ctrl Pts',(-23.3696495237974,-13.514319108057,
115.312941149939)) ;
#179581=CARTESIAN_POINT('Ctrl Pts',(-23.39322191209,-13.5214605368481,115.384738842976)) ;
#179582=CARTESIAN_POINT('Ctrl Pts',(-23.4670257532734,-13.5214606238932,
115.360507794478)) ;
#179583=CARTESIAN_POINT('Ctrl Pts',(-23.5408295944568,-13.5214607109383,
115.33627674598)) ;
#179584=CARTESIAN_POINT('Ctrl Pts',(-23.5172572061641,-13.5143192821472,
115.264479052943)) ;
#179585=CARTESIAN_POINT('Ctrl Pts',(-23.5025567461663,-13.2228141005811,
115.255249135668)) ;
#179586=CARTESIAN_POINT('Ctrl Pts',(-23.4792395565044,-13.236014362639,
115.184228736629)) ;
#179587=CARTESIAN_POINT('Ctrl Pts',(-23.4054357084178,-13.2360142841561,
115.208459764101)) ;
#179588=CARTESIAN_POINT('Ctrl Pts',(-23.3316318603313,-13.2360142056732,
115.232690791573)) ;
#179589=CARTESIAN_POINT('Ctrl Pts',(-23.3549490499933,-13.2228139436153,
115.303711190613)) ;
#179590=CARTESIAN_POINT('Ctrl Pts',(-23.3782662396552,-13.2096136815574,
115.374731589652)) ;
#179591=CARTESIAN_POINT('Ctrl Pts',(-23.4520700877417,-13.2096137600403,
115.35050056218)) ;
#179592=CARTESIAN_POINT('Ctrl Pts',(-23.5258739358282,-13.2096138385232,
115.326269534708)) ;
#179593=CARTESIAN_POINT('Ctrl Pts',(-23.5025567461663,-13.2228141005811,
115.255249135668)) ;
#179594=CARTESIAN_POINT('Ctrl Pts',(-23.4640229788602,-12.9463122499942,
115.173287772294)) ;
#179595=CARTESIAN_POINT('Ctrl Pts',(-23.4426283410456,-12.9788376519378,
115.108123156115)) ;
#179596=CARTESIAN_POINT('Ctrl Pts',(-23.3688244875743,-12.978837586653,
115.132354167186)) ;
#179597=CARTESIAN_POINT('Ctrl Pts',(-23.295020634103,-12.9788375213682,
115.156585178257)) ;
#179598=CARTESIAN_POINT('Ctrl Pts',(-23.3164152719176,-12.9463121194246,
115.221749794436)) ;
#179599=CARTESIAN_POINT('Ctrl Pts',(-23.3378099097322,-12.913786717481,
115.286914410615)) ;
#179600=CARTESIAN_POINT('Ctrl Pts',(-23.4116137632035,-12.9137867827658,
115.262683399543)) ;
#179601=CARTESIAN_POINT('Ctrl Pts',(-23.4854176166749,-12.9137868480506,
115.238452388472)) ;
#179602=CARTESIAN_POINT('Ctrl Pts',(-23.4640229788602,-12.9463122499942,
115.173287772294)) ;
#179603=CARTESIAN_POINT('Ctrl Pts',(-23.4033068584606,-12.7025112775513,
115.023933887441)) ;
#179604=CARTESIAN_POINT('Ctrl Pts',(-23.38538272599,-12.7521082971811,114.969339870752)) ;
#179605=CARTESIAN_POINT('Ctrl Pts',(-23.3115788693362,-12.7521082496802,
114.99357087213)) ;
#179606=CARTESIAN_POINT('Ctrl Pts',(-23.2377750126825,-12.7521082021794,
115.017801873508)) ;
#179607=CARTESIAN_POINT('Ctrl Pts',(-23.2556991451531,-12.7025111825496,
115.072395890197)) ;
#179608=CARTESIAN_POINT('Ctrl Pts',(-23.2736232776238,-12.6529141629198,
115.126989906885)) ;
#179609=CARTESIAN_POINT('Ctrl Pts',(-23.3474271342775,-12.6529142104206,
115.102758905507)) ;
#179610=CARTESIAN_POINT('Ctrl Pts',(-23.4212309909313,-12.6529142579215,
115.078527904129)) ;
#179611=CARTESIAN_POINT('Ctrl Pts',(-23.4033068584606,-12.7025112775513,
115.023933887441)) ;
#179612=CARTESIAN_POINT('Ctrl Pts',(-23.3247469439269,-12.5113386435153,
114.819989036996)) ;
#179613=CARTESIAN_POINT('Ctrl Pts',(-23.3115496393032,-12.5743584257443,
114.779792175398)) ;
#179614=CARTESIAN_POINT('Ctrl Pts',(-23.2377457810958,-12.5743583951879,
114.804023172044)) ;
#179615=CARTESIAN_POINT('Ctrl Pts',(-23.1639419228884,-12.5743583646314,
114.82825416869)) ;
#179616=CARTESIAN_POINT('Ctrl Pts',(-23.1771392275121,-12.5113385824024,
114.868451030287)) ;
#179617=CARTESIAN_POINT('Ctrl Pts',(-23.1903365321358,-12.4483188001733,
114.908647891885)) ;
#179618=CARTESIAN_POINT('Ctrl Pts',(-23.2641403903432,-12.4483188307298,
114.884416895239)) ;
#179619=CARTESIAN_POINT('Ctrl Pts',(-23.3379442485506,-12.4483188612862,
114.860185898593)) ;
#179620=CARTESIAN_POINT('Ctrl Pts',(-23.3247469439269,-12.5113386435153,
114.819989036996)) ;
#179621=CARTESIAN_POINT('Ctrl Pts',(-23.2322554152184,-12.3839986409936,
114.573835678973)) ;
#179622=CARTESIAN_POINT('Ctrl Pts',(-23.2247600633501,-12.45600534241,114.551006045648)) ;
#179623=CARTESIAN_POINT('Ctrl Pts',(-23.1509562059776,-12.4560053286552,
114.575237044837)) ;
#179624=CARTESIAN_POINT('Ctrl Pts',(-23.0771523486052,-12.4560053149005,
114.599468044026)) ;
#179625=CARTESIAN_POINT('Ctrl Pts',(-23.0846477004735,-12.3839986134842,
114.622297677351)) ;
#179626=CARTESIAN_POINT('Ctrl Pts',(-23.0921430523418,-12.3119919120679,
114.645127310676)) ;
#179627=CARTESIAN_POINT('Ctrl Pts',(-23.1659469097142,-12.3119919258226,
114.620896311487)) ;
#179628=CARTESIAN_POINT('Ctrl Pts',(-23.2397507670867,-12.3119919395773,
114.596665312298)) ;
#179629=CARTESIAN_POINT('Ctrl Pts',(-23.2322554152184,-12.3839986409936,
114.573835678973)) ;
#179630=CARTESIAN_POINT('Ctrl Pts',(-23.1325124738357,-12.3313598679509,
114.305463729675)) ;
#179631=CARTESIAN_POINT('Ctrl Pts',(-23.1312369108758,-12.4071510797427,
114.301578569967)) ;
#179632=CARTESIAN_POINT('Ctrl Pts',(-23.0574330554719,-12.4071510785913,
114.325809575152)) ;
#179633=CARTESIAN_POINT('Ctrl Pts',(-22.983629200068,-12.4071510774399,
114.350040580336)) ;
#179634=CARTESIAN_POINT('Ctrl Pts',(-22.9849047630278,-12.3313598656482,
114.353925740044)) ;
#179635=CARTESIAN_POINT('Ctrl Pts',(-22.9861803259877,-12.2555686538564,
114.357810899752)) ;
#179636=CARTESIAN_POINT('Ctrl Pts',(-23.0599841813916,-12.2555686550078,
114.333579894567)) ;
#179637=CARTESIAN_POINT('Ctrl Pts',(-23.1337880367955,-12.2555686561592,
114.309348889382)) ;
#179638=CARTESIAN_POINT('Ctrl Pts',(-23.1325124738357,-12.3313598679509,
114.305463729675)) ;
#179639=CARTESIAN_POINT('Ctrl Pts',(-23.0315695868954,-12.3561484752169,
114.033447032347)) ;
#179640=CARTESIAN_POINT('Ctrl Pts',(-23.0366068410836,-12.4303237529548,
114.048789695264)) ;
#179641=CARTESIAN_POINT('Ctrl Pts',(-22.9628029885546,-12.4303237603732,
114.073020709205)) ;
#179642=CARTESIAN_POINT('Ctrl Pts',(-22.8889991360256,-12.4303237677915,
114.097251723146)) ;
#179643=CARTESIAN_POINT('Ctrl Pts',(-22.8839618818374,-12.3561484900536,
114.08190906023)) ;
#179644=CARTESIAN_POINT('Ctrl Pts',(-22.8789246276492,-12.2819732123158,
114.066566397313)) ;
#179645=CARTESIAN_POINT('Ctrl Pts',(-22.9527284801782,-12.2819732048974,
114.042335383372)) ;
#179646=CARTESIAN_POINT('Ctrl Pts',(-23.0265323327071,-12.2819731974791,
114.018104369431)) ;
#179647=CARTESIAN_POINT('Ctrl Pts',(-23.0315695868954,-12.3561484752169,
114.033447032347)) ;
#179648=CARTESIAN_POINT('Ctrl Pts',(-22.9354487583315,-12.4578681360596,
113.776309520322)) ;
#179649=CARTESIAN_POINT('Ctrl Pts',(-22.9464679447324,-12.5250537220818,
113.809872183762)) ;
#179650=CARTESIAN_POINT('Ctrl Pts',(-22.8726640957551,-12.5250537323896,
113.834103208521)) ;
#179651=CARTESIAN_POINT('Ctrl Pts',(-22.7988602467779,-12.5250537426973,
113.85833423328)) ;
#179652=CARTESIAN_POINT('Ctrl Pts',(-22.787841060377,-12.4578681566752,
113.82477156984)) ;
#179653=CARTESIAN_POINT('Ctrl Pts',(-22.7768218739761,-12.390682570653,
113.7912089064)) ;
#179654=CARTESIAN_POINT('Ctrl Pts',(-22.8506257229533,-12.3906825603452,
113.766977881641)) ;
#179655=CARTESIAN_POINT('Ctrl Pts',(-22.9244295719306,-12.3906825500374,
113.742746856882)) ;
#179656=CARTESIAN_POINT('Ctrl Pts',(-22.9354487583315,-12.4578681360596,
113.776309520322)) ;
#179657=CARTESIAN_POINT('Ctrl Pts',(-22.8516194022014,-12.6270814220524,
113.556268256684)) ;
#179658=CARTESIAN_POINT('Ctrl Pts',(-22.8677782073947,-12.6825528988753,
113.605485369805)) ;
#179659=CARTESIAN_POINT('Ctrl Pts',(-22.7939743607582,-12.6825529093536,
113.629716401694)) ;
#179660=CARTESIAN_POINT('Ctrl Pts',(-22.7201705141217,-12.6825529198319,
113.653947433583)) ;
#179661=CARTESIAN_POINT('Ctrl Pts',(-22.7040117089284,-12.627081443009,
113.604730320462)) ;
#179662=CARTESIAN_POINT('Ctrl Pts',(-22.6878529037351,-12.5716099661861,
113.555513207342)) ;
#179663=CARTESIAN_POINT('Ctrl Pts',(-22.7616567503716,-12.5716099557078,
113.531282175453)) ;
#179664=CARTESIAN_POINT('Ctrl Pts',(-22.8354605970081,-12.5716099452296,
113.507051143564)) ;
#179665=CARTESIAN_POINT('Ctrl Pts',(-22.8516194022014,-12.6270814220524,
113.556268256684)) ;
#179666=CARTESIAN_POINT('Ctrl Pts',(-22.7839838450555,-12.8533401319523,
113.385716322209)) ;
#179667=CARTESIAN_POINT('Ctrl Pts',(-22.8041559831465,-12.8930967028274,
113.447157399914)) ;
#179668=CARTESIAN_POINT('Ctrl Pts',(-22.7303521385785,-12.8930967101103,
113.471388438103)) ;
#179669=CARTESIAN_POINT('Ctrl Pts',(-22.6565482940104,-12.8930967173931,
113.495619476292)) ;
#179670=CARTESIAN_POINT('Ctrl Pts',(-22.6363761559194,-12.853340146518,
113.434178398587)) ;
#179671=CARTESIAN_POINT('Ctrl Pts',(-22.6162040178284,-12.8135835756429,
113.372737320882)) ;
#179672=CARTESIAN_POINT('Ctrl Pts',(-22.6900078623964,-12.8135835683601,
113.348506282693)) ;
#179673=CARTESIAN_POINT('Ctrl Pts',(-22.7638117069645,-12.8135835610772,
113.324275244504)) ;
#179674=CARTESIAN_POINT('Ctrl Pts',(-22.7839838450555,-12.8533401319523,
113.385716322209)) ;
#179675=CARTESIAN_POINT('Ctrl Pts',(-22.737057523416,-13.1210491167834,
113.278349913962)) ;
#179676=CARTESIAN_POINT('Ctrl Pts',(-22.7598008408309,-13.1421721692445,
113.347622389144)) ;
#179677=CARTESIAN_POINT('Ctrl Pts',(-22.6859969973566,-13.1421721715333,
113.371853430664)) ;
#179678=CARTESIAN_POINT('Ctrl Pts',(-22.6121931538823,-13.1421721738222,
113.396084472184)) ;
#179679=CARTESIAN_POINT('Ctrl Pts',(-22.5894498364674,-13.121049121361,
113.326811997003)) ;
#179680=CARTESIAN_POINT('Ctrl Pts',(-22.5667065190524,-13.0999260688999,
113.257539521822)) ;
#179681=CARTESIAN_POINT('Ctrl Pts',(-22.6405103625268,-13.0999260666111,
113.233308480301)) ;
#179682=CARTESIAN_POINT('Ctrl Pts',(-22.7143142060011,-13.0999260643223,
113.209077438781)) ;
#179683=CARTESIAN_POINT('Ctrl Pts',(-22.737057523416,-13.1210491167834,
113.278349913962)) ;
#179684=CARTESIAN_POINT('Ctrl Pts',(-22.7137114782824,-13.40900770729,113.242669521787)) ;
#179685=CARTESIAN_POINT('Ctrl Pts',(-22.7373858208915,-13.410054885097,
113.314777749557)) ;
#179686=CARTESIAN_POINT('Ctrl Pts',(-22.663581977556,-13.4100548838608,
113.339008791501)) ;
#179687=CARTESIAN_POINT('Ctrl Pts',(-22.5897781342205,-13.4100548826247,
113.363239833444)) ;
#179688=CARTESIAN_POINT('Ctrl Pts',(-22.5661037916114,-13.4090077048177,
113.291131605674)) ;
#179689=CARTESIAN_POINT('Ctrl Pts',(-22.5424294490023,-13.4079605270107,
113.219023377904)) ;
#179690=CARTESIAN_POINT('Ctrl Pts',(-22.6162332923378,-13.4079605282469,
113.19479233596)) ;
#179691=CARTESIAN_POINT('Ctrl Pts',(-22.6900371356733,-13.407960529483,
113.170561294017)) ;
#179692=CARTESIAN_POINT('Ctrl Pts',(-22.7137114782824,-13.40900770729,113.242669521787)) ;
#179693=CARTESIAN_POINT('Ctrl Pts',(-22.7145790475153,-13.6972694862933,
113.280702081642)) ;
#179694=CARTESIAN_POINT('Ctrl Pts',(-22.7374956175448,-13.6781895282422,
113.350502256437)) ;
#179695=CARTESIAN_POINT('Ctrl Pts',(-22.6636917739189,-13.6781895252059,
113.374733297496)) ;
#179696=CARTESIAN_POINT('Ctrl Pts',(-22.5898879302931,-13.6781895221696,
113.398964338555)) ;
#179697=CARTESIAN_POINT('Ctrl Pts',(-22.5669713602635,-13.6972694802207,
113.32916416376)) ;
#179698=CARTESIAN_POINT('Ctrl Pts',(-22.544054790234,-13.7163494382719,
113.259363988965)) ;
#179699=CARTESIAN_POINT('Ctrl Pts',(-22.6178586338598,-13.7163494413082,
113.235132947906)) ;
#179700=CARTESIAN_POINT('Ctrl Pts',(-22.6916624774857,-13.7163494443445,
113.210901906847)) ;
#179701=CARTESIAN_POINT('Ctrl Pts',(-22.7145790475153,-13.6972694862933,
113.280702081642)) ;
#179702=CARTESIAN_POINT('Ctrl Pts',(-22.73888971428,-13.9663054532962,113.390221067271)) ;
#179703=CARTESIAN_POINT('Ctrl Pts',(-22.7594085131034,-13.9284104742122,
113.452718017853)) ;
#179704=CARTESIAN_POINT('Ctrl Pts',(-22.6856046691513,-13.9284104715145,
113.476949057918)) ;
#179705=CARTESIAN_POINT('Ctrl Pts',(-22.6118008251992,-13.9284104688168,
113.501180097983)) ;
#179706=CARTESIAN_POINT('Ctrl Pts',(-22.5912820263757,-13.9663054479008,
113.438683147401)) ;
#179707=CARTESIAN_POINT('Ctrl Pts',(-22.5707632275523,-14.0042004269848,
113.376186196819)) ;
#179708=CARTESIAN_POINT('Ctrl Pts',(-22.6445670715044,-14.0042004296825,
113.351955156754)) ;
#179709=CARTESIAN_POINT('Ctrl Pts',(-22.7183709154566,-14.0042004323802,
113.327724116689)) ;
#179710=CARTESIAN_POINT('Ctrl Pts',(-22.73888971428,-13.9663054532962,113.390221067271)) ;
#179711=CARTESIAN_POINT('Ctrl Pts',(-22.7845308373615,-14.1969043333081,
113.564878486232)) ;
#179712=CARTESIAN_POINT('Ctrl Pts',(-22.8011552397315,-14.1428507400375,
113.615513733517)) ;
#179713=CARTESIAN_POINT('Ctrl Pts',(-22.7273513962051,-14.1428507401224,
113.639744774879)) ;
#179714=CARTESIAN_POINT('Ctrl Pts',(-22.6535475526786,-14.1428507402074,
113.663975816241)) ;
#179715=CARTESIAN_POINT('Ctrl Pts',(-22.6369231503086,-14.196904333478,
113.613340568955)) ;
#179716=CARTESIAN_POINT('Ctrl Pts',(-22.6202987479386,-14.2509579267487,
113.56270532167)) ;
#179717=CARTESIAN_POINT('Ctrl Pts',(-22.6941025914651,-14.2509579266637,
113.538474280308)) ;
#179718=CARTESIAN_POINT('Ctrl Pts',(-22.7679064349915,-14.2509579265788,
113.514243238946)) ;
#179719=CARTESIAN_POINT('Ctrl Pts',(-22.7845308373615,-14.1969043333081,
113.564878486232)) ;
#179720=CARTESIAN_POINT('Ctrl Pts',(-22.8467313080852,-14.3698914257013,
113.789672047739)) ;
#179721=CARTESIAN_POINT('Ctrl Pts',(-22.8583054400605,-14.3036801668695,
113.824924986188)) ;
#179722=CARTESIAN_POINT('Ctrl Pts',(-22.7845015975603,-14.3036801689092,
113.849156030675)) ;
#179723=CARTESIAN_POINT('Ctrl Pts',(-22.71069775506,-14.303680170949,113.873387075162)) ;
#179724=CARTESIAN_POINT('Ctrl Pts',(-22.6991236230846,-14.3698914297808,
113.838134136713)) ;
#179725=CARTESIAN_POINT('Ctrl Pts',(-22.6875494911093,-14.4361026886127,
113.802881198264)) ;
#179726=CARTESIAN_POINT('Ctrl Pts',(-22.7613533336096,-14.4361026865729,
113.778650153777)) ;
#179727=CARTESIAN_POINT('Ctrl Pts',(-22.8351571761099,-14.4361026845332,
113.75441910929)) ;
#179728=CARTESIAN_POINT('Ctrl Pts',(-22.8467313080852,-14.3698914257013,
113.789672047739)) ;
#179729=CARTESIAN_POINT('Ctrl Pts',(-22.9207425971933,-14.4755193866787,
114.050515802976)) ;
#179730=CARTESIAN_POINT('Ctrl Pts',(-22.9264328703088,-14.4018362726686,
114.067847456596)) ;
#179731=CARTESIAN_POINT('Ctrl Pts',(-22.8526290294858,-14.4018362752404,
114.092078506192)) ;
#179732=CARTESIAN_POINT('Ctrl Pts',(-22.7788251886628,-14.4018362778122,
114.116309555787)) ;
#179733=CARTESIAN_POINT('Ctrl Pts',(-22.7731349155474,-14.4755193918222,
114.098977902168)) ;
#179734=CARTESIAN_POINT('Ctrl Pts',(-22.7674446424319,-14.5492025058322,
114.081646248548)) ;
#179735=CARTESIAN_POINT('Ctrl Pts',(-22.8412484832549,-14.5492025032605,
114.057415198952)) ;
#179736=CARTESIAN_POINT('Ctrl Pts',(-22.9150523240779,-14.5492025006887,
114.033184149356)) ;
#179737=CARTESIAN_POINT('Ctrl Pts',(-22.9207425971933,-14.4755193866787,
114.050515802976)) ;
#179738=CARTESIAN_POINT('Ctrl Pts',(-23.0006816978968,-14.5054697818126,
114.329505017033)) ;
#179739=CARTESIAN_POINT('Ctrl Pts',(-23.0000638124603,-14.4295881889502,
114.327623037386)) ;
#179740=CARTESIAN_POINT('Ctrl Pts',(-22.9262599739428,-14.4295881891086,
114.351854094004)) ;
#179741=CARTESIAN_POINT('Ctrl Pts',(-22.8524561354252,-14.429588189267,
114.376085150622)) ;
#179742=CARTESIAN_POINT('Ctrl Pts',(-22.8530740208617,-14.5054697821294,
114.377967130269)) ;
#179743=CARTESIAN_POINT('Ctrl Pts',(-22.8536919062982,-14.5813513749918,
114.379849109916)) ;
#179744=CARTESIAN_POINT('Ctrl Pts',(-22.9274957448158,-14.5813513748333,
114.355618053298)) ;
#179745=CARTESIAN_POINT('Ctrl Pts',(-23.0012995833333,-14.5813513746749,
114.33138699668)) ;
#179746=CARTESIAN_POINT('Ctrl Pts',(-23.0006816978968,-14.5054697818126,
114.329505017033)) ;
#179747=CARTESIAN_POINT('Ctrl Pts',(-23.0797492263395,-14.4574393177702,
114.6057916227)) ;
#179748=CARTESIAN_POINT('Ctrl Pts',(-23.0728759886018,-14.384801335134,
114.584856849095)) ;
#179749=CARTESIAN_POINT('Ctrl Pts',(-22.9990721521764,-14.384801328945,
114.609087912085)) ;
#179750=CARTESIAN_POINT('Ctrl Pts',(-22.9252683157509,-14.384801322756,
114.633318975075)) ;
#179751=CARTESIAN_POINT('Ctrl Pts',(-22.9321415534886,-14.4574393053923,
114.65425374868)) ;
#179752=CARTESIAN_POINT('Ctrl Pts',(-22.9390147912263,-14.5300772880285,
114.675188522285)) ;
#179753=CARTESIAN_POINT('Ctrl Pts',(-23.0128186276518,-14.5300772942175,
114.650957459295)) ;
#179754=CARTESIAN_POINT('Ctrl Pts',(-23.0866224640773,-14.5300773004065,
114.626726396305)) ;
#179755=CARTESIAN_POINT('Ctrl Pts',(-23.0797492263395,-14.4574393177702,
114.6057916227)) ;
#179756=CARTESIAN_POINT('Ctrl Pts',(-23.1516520346911,-14.3349211938034,
114.860267274073)) ;
#179757=CARTESIAN_POINT('Ctrl Pts',(-23.1390144923335,-14.2707324518497,
114.821775358504)) ;
#179758=CARTESIAN_POINT('Ctrl Pts',(-23.0652106573152,-14.2707324355109,
114.84600642578)) ;
#179759=CARTESIAN_POINT('Ctrl Pts',(-22.9914068222969,-14.2707324191721,
114.870237493056)) ;
#179760=CARTESIAN_POINT('Ctrl Pts',(-23.0040443646544,-14.3349211611258,
114.908729408625)) ;
#179761=CARTESIAN_POINT('Ctrl Pts',(-23.0166819070119,-14.3991099030794,
114.947221324195)) ;
#179762=CARTESIAN_POINT('Ctrl Pts',(-23.0904857420302,-14.3991099194182,
114.922990256919)) ;
#179763=CARTESIAN_POINT('Ctrl Pts',(-23.1642895770486,-14.399109935757,
114.898759189643)) ;
#179764=CARTESIAN_POINT('Ctrl Pts',(-23.1516520346911,-14.3349211938034,
114.860267274073)) ;
#179765=CARTESIAN_POINT('Ctrl Pts',(-23.2103873638468,-14.1470800055845,
115.074578542204)) ;
#179766=CARTESIAN_POINT('Ctrl Pts',(-23.1928978798013,-14.0959137214437,
115.021308394955)) ;
#179767=CARTESIAN_POINT('Ctrl Pts',(-23.1190940448238,-14.0959136926008,
115.045539462355)) ;
#179768=CARTESIAN_POINT('Ctrl Pts',(-23.0452902098462,-14.095913663758,
115.069770529756)) ;
#179769=CARTESIAN_POINT('Ctrl Pts',(-23.0627796938917,-14.1470799478988,
115.123040677004)) ;
#179770=CARTESIAN_POINT('Ctrl Pts',(-23.0802691779372,-14.1982462320397,
115.176310824253)) ;
#179771=CARTESIAN_POINT('Ctrl Pts',(-23.1540730129147,-14.1982462608825,
115.152079756853)) ;
#179772=CARTESIAN_POINT('Ctrl Pts',(-23.2278768478922,-14.1982462897254,
115.127848689452)) ;
#179773=CARTESIAN_POINT('Ctrl Pts',(-23.2103873638468,-14.1470800055845,
115.074578542204)) ;
#179774=CARTESIAN_POINT('Ctrl Pts',(-23.2512289756988,-13.9065331674936,
115.234478316148)) ;
#179775=CARTESIAN_POINT('Ctrl Pts',(-23.2301280118323,-13.8720877275132,
115.170208183899)) ;
#179776=CARTESIAN_POINT('Ctrl Pts',(-23.1563241754642,-13.8720876844338,
115.194439247064)) ;
#179777=CARTESIAN_POINT('Ctrl Pts',(-23.0825203390961,-13.8720876413544,
115.218670310229)) ;
#179778=CARTESIAN_POINT('Ctrl Pts',(-23.1036213029626,-13.9065330813348,
115.282940442478)) ;
#179779=CARTESIAN_POINT('Ctrl Pts',(-23.1247222668291,-13.9409785213152,
115.347210574727)) ;
#179780=CARTESIAN_POINT('Ctrl Pts',(-23.1985261031972,-13.9409785643945,
115.322979511562)) ;
#179781=CARTESIAN_POINT('Ctrl Pts',(-23.2723299395653,-13.9409786074739,
115.298748448398)) ;
#179782=CARTESIAN_POINT('Ctrl Pts',(-23.2512289756988,-13.9065331674936,
115.234478316148)) ;
#179783=CARTESIAN_POINT('Ctrl Pts',(-23.2702582801817,-13.630738678715,
115.327956236279)) ;
#179784=CARTESIAN_POINT('Ctrl Pts',(-23.2470632296834,-13.6154990346672,
115.257307853852)) ;
#179785=CARTESIAN_POINT('Ctrl Pts',(-23.1732593900141,-13.6154989781254,
115.281538906962)) ;
#179786=CARTESIAN_POINT('Ctrl Pts',(-23.0994555503449,-13.6154989215836,
115.305769960072)) ;
#179787=CARTESIAN_POINT('Ctrl Pts',(-23.1226506008432,-13.6307385656315,
115.376418342499)) ;
#179788=CARTESIAN_POINT('Ctrl Pts',(-23.1458456513416,-13.6459782096793,
115.447066724927)) ;
#179789=CARTESIAN_POINT('Ctrl Pts',(-23.2196494910108,-13.6459782662211,
115.422835671817)) ;
#179790=CARTESIAN_POINT('Ctrl Pts',(-23.29345333068,-13.6459783227629,115.398604618707)) ;
#179791=CARTESIAN_POINT('Ctrl Pts',(-23.2702582801817,-13.630738678715,
115.327956236279)) ;
#179792=CARTESIAN_POINT('Ctrl Pts',(-23.2654718156878,-13.3408270196336,
115.34875619149)) ;
#179793=CARTESIAN_POINT('Ctrl Pts',(-23.2418454296788,-13.3458064636332,
115.276794030546)) ;
#179794=CARTESIAN_POINT('Ctrl Pts',(-23.1680415850337,-13.3458063983403,
115.301025068501)) ;
#179795=CARTESIAN_POINT('Ctrl Pts',(-23.0942377403886,-13.3458063330474,
115.325256106455)) ;
#179796=CARTESIAN_POINT('Ctrl Pts',(-23.1178641263977,-13.3408268890478,
115.397218267399)) ;
#179797=CARTESIAN_POINT('Ctrl Pts',(-23.1414905124067,-13.3358474450482,
115.469180428343)) ;
#179798=CARTESIAN_POINT('Ctrl Pts',(-23.2152943570518,-13.3358475103411,
115.444949390389)) ;
#179799=CARTESIAN_POINT('Ctrl Pts',(-23.2890982016969,-13.335847575634,
115.420718352435)) ;
#179800=CARTESIAN_POINT('Ctrl Pts',(-23.2654718156878,-13.3408270196336,
115.34875619149)) ;
#179801=CARTESIAN_POINT('Ctrl Pts',(-23.2364052797184,-13.0553492265632,
115.295741122605)) ;
#179802=CARTESIAN_POINT('Ctrl Pts',(-23.2140390795287,-13.0802672240232,
115.227617284172)) ;
#179803=CARTESIAN_POINT('Ctrl Pts',(-23.1402352286369,-13.0802671541192,
115.2518483031)) ;
#179804=CARTESIAN_POINT('Ctrl Pts',(-23.066431377745,-13.0802670842153,
115.276079322027)) ;
#179805=CARTESIAN_POINT('Ctrl Pts',(-23.0887975779347,-13.0553490867554,
115.34420316046)) ;
#179806=CARTESIAN_POINT('Ctrl Pts',(-23.1111637781244,-13.0304310892955,
115.412326998893)) ;
#179807=CARTESIAN_POINT('Ctrl Pts',(-23.1849676290162,-13.0304311591994,
115.388095979966)) ;
#179808=CARTESIAN_POINT('Ctrl Pts',(-23.2587714799081,-13.0304312291033,
115.363864961038)) ;
#179809=CARTESIAN_POINT('Ctrl Pts',(-23.2364052797184,-13.0553492265632,
115.295741122605)) ;
#179810=CARTESIAN_POINT('Ctrl Pts',(-23.184450119502,-12.7963986353394,
115.172941175961)) ;
#179811=CARTESIAN_POINT('Ctrl Pts',(-23.1649453982512,-12.8394319369363,
115.113532940537)) ;
#179812=CARTESIAN_POINT('Ctrl Pts',(-23.0911415405192,-12.8394318699613,
115.137763938631)) ;
#179813=CARTESIAN_POINT('Ctrl Pts',(-23.0173376827871,-12.8394318029862,
115.161994936724)) ;
#179814=CARTESIAN_POINT('Ctrl Pts',(-23.0368424040378,-12.7963985013893,
115.221403172148)) ;
#179815=CARTESIAN_POINT('Ctrl Pts',(-23.0563471252886,-12.7533651997924,
115.280811407572)) ;
#179816=CARTESIAN_POINT('Ctrl Pts',(-23.1301509830206,-12.7533652667675,
115.256580409478)) ;
#179817=CARTESIAN_POINT('Ctrl Pts',(-23.2039548407527,-12.7533653337425,
115.232349411385)) ;
#179818=CARTESIAN_POINT('Ctrl Pts',(-23.184450119502,-12.7963986353394,
115.172941175961)) ;
#179819=CARTESIAN_POINT('Ctrl Pts',(-23.112508885965,-12.581755675213,114.98929825524)) ;
#179820=CARTESIAN_POINT('Ctrl Pts',(-23.097264403479,-12.6398371824031,
114.942866019574)) ;
#179821=CARTESIAN_POINT('Ctrl Pts',(-23.0234605390643,-12.6398371256695,
114.967096997313)) ;
#179822=CARTESIAN_POINT('Ctrl Pts',(-22.9496566746497,-12.639837068936,
114.991327975052)) ;
#179823=CARTESIAN_POINT('Ctrl Pts',(-22.9649011571356,-12.581755561746,
115.037760210718)) ;
#179824=CARTESIAN_POINT('Ctrl Pts',(-22.9801456396215,-12.5236740545559,
115.084192446384)) ;
#179825=CARTESIAN_POINT('Ctrl Pts',(-23.0539495040362,-12.5236741112895,
115.059961468645)) ;
#179826=CARTESIAN_POINT('Ctrl Pts',(-23.1277533684509,-12.523674168023,
115.035730490905)) ;
#179827=CARTESIAN_POINT('Ctrl Pts',(-23.112508885965,-12.581755675213,114.98929825524)) ;
#179828=CARTESIAN_POINT('Ctrl Pts',(-23.0250710503237,-12.4271874700909,
114.758426315697)) ;
#179829=CARTESIAN_POINT('Ctrl Pts',(-23.0151754699224,-12.4961449438695,
114.728285972627)) ;
#179830=CARTESIAN_POINT('Ctrl Pts',(-22.9413715999022,-12.4961449047111,
114.752516933292)) ;
#179831=CARTESIAN_POINT('Ctrl Pts',(-22.8675677298821,-12.4961448655528,
114.776747893958)) ;
#179832=CARTESIAN_POINT('Ctrl Pts',(-22.8774633102834,-12.4271873917741,
114.806888237029)) ;
#179833=CARTESIAN_POINT('Ctrl Pts',(-22.8873588906847,-12.3582299179955,
114.837028580099)) ;
#179834=CARTESIAN_POINT('Ctrl Pts',(-22.9611627607048,-12.3582299571538,
114.812797619433)) ;
#179835=CARTESIAN_POINT('Ctrl Pts',(-23.034966630725,-12.3582299963122,
114.788566658768)) ;
#179836=CARTESIAN_POINT('Ctrl Pts',(-23.0250710503237,-12.4271874700909,
114.758426315697)) ;
#179837=CARTESIAN_POINT('Ctrl Pts',(-22.9276247608224,-12.3434882644401,
114.49706508371)) ;
#179838=CARTESIAN_POINT('Ctrl Pts',(-22.9237846766469,-12.4183899253302,
114.485368804997)) ;
#179839=CARTESIAN_POINT('Ctrl Pts',(-22.8499808028187,-12.4183899094731,
114.509599754064)) ;
#179840=CARTESIAN_POINT('Ctrl Pts',(-22.7761769289905,-12.418389893616,
114.533830703132)) ;
#179841=CARTESIAN_POINT('Ctrl Pts',(-22.780017013166,-12.3434882327259,
114.545526981844)) ;
#179842=CARTESIAN_POINT('Ctrl Pts',(-22.7838570973414,-12.2685865718357,
114.557223260557)) ;
#179843=CARTESIAN_POINT('Ctrl Pts',(-22.8576609711696,-12.2685865876929,
114.53299231149)) ;
#179844=CARTESIAN_POINT('Ctrl Pts',(-22.9314648449978,-12.26858660355,114.508761362422)) ;
#179845=CARTESIAN_POINT('Ctrl Pts',(-22.9276247608224,-12.3434882644401,
114.49706508371)) ;
#179846=CARTESIAN_POINT('Ctrl Pts',(-22.826190770514,-12.3367187774922,
114.223618478407)) ;
#179847=CARTESIAN_POINT('Ctrl Pts',(-22.8286921174986,-12.412202858538,
114.23123717574)) ;
#179848=CARTESIAN_POINT('Ctrl Pts',(-22.7548882421407,-12.4122028696992,
114.255468120148)) ;
#179849=CARTESIAN_POINT('Ctrl Pts',(-22.6810843667827,-12.4122028808603,
114.279699064556)) ;
#179850=CARTESIAN_POINT('Ctrl Pts',(-22.678583019798,-12.3367187998145,
114.272080367222)) ;
#179851=CARTESIAN_POINT('Ctrl Pts',(-22.6760816728134,-12.2612347187686,
114.264461669889)) ;
#179852=CARTESIAN_POINT('Ctrl Pts',(-22.7498855481713,-12.2612347076075,
114.240230725481)) ;
#179853=CARTESIAN_POINT('Ctrl Pts',(-22.8236894235293,-12.2612346964463,
114.215999781074)) ;
#179854=CARTESIAN_POINT('Ctrl Pts',(-22.826190770514,-12.3367187774922,
114.223618478407)) ;
#179855=CARTESIAN_POINT('Ctrl Pts',(-22.7275355764204,-12.4076100218016,
113.958611864948)) ;
#179856=CARTESIAN_POINT('Ctrl Pts',(-22.7361941637396,-12.478255694811,
113.984984522816)) ;
#179857=CARTESIAN_POINT('Ctrl Pts',(-22.662390289618,-12.4782557339545,
114.00921547099)) ;
#179858=CARTESIAN_POINT('Ctrl Pts',(-22.5885864154965,-12.4782557730979,
114.033446419164)) ;
#179859=CARTESIAN_POINT('Ctrl Pts',(-22.5799278281774,-12.4076101000885,
114.007073761295)) ;
#179860=CARTESIAN_POINT('Ctrl Pts',(-22.5712692408582,-12.3369644270791,
113.980701103427)) ;
#179861=CARTESIAN_POINT('Ctrl Pts',(-22.6450731149797,-12.3369643879356,
113.956470155253)) ;
#179862=CARTESIAN_POINT('Ctrl Pts',(-22.7188769891013,-12.3369643487922,
113.93223920708)) ;
#179863=CARTESIAN_POINT('Ctrl Pts',(-22.7275355764204,-12.4076100218016,
113.958611864948)) ;
#179864=CARTESIAN_POINT('Ctrl Pts',(-22.6381489586998,-12.5503272886106,
113.721728947846)) ;
#179865=CARTESIAN_POINT('Ctrl Pts',(-22.6523289736193,-12.6111127645847,
113.764918983274)) ;
#179866=CARTESIAN_POINT('Ctrl Pts',(-22.5785251034211,-12.6111128294537,
113.789149943397)) ;
#179867=CARTESIAN_POINT('Ctrl Pts',(-22.5047212332228,-12.6111128943226,
113.81338090352)) ;
#179868=CARTESIAN_POINT('Ctrl Pts',(-22.4905412183032,-12.5503274183485,
113.770190868092)) ;
#179869=CARTESIAN_POINT('Ctrl Pts',(-22.4763612033837,-12.4895419423743,
113.727000832665)) ;
#179870=CARTESIAN_POINT('Ctrl Pts',(-22.550165073582,-12.4895418775054,
113.702769872541)) ;
#179871=CARTESIAN_POINT('Ctrl Pts',(-22.6239689437803,-12.4895418126364,
113.678538912418)) ;
#179872=CARTESIAN_POINT('Ctrl Pts',(-22.6381489586998,-12.5503272886106,
113.721728947846)) ;
#179873=CARTESIAN_POINT('Ctrl Pts',(-22.5630668542689,-12.7556871760659,
113.528549608634)) ;
#179874=CARTESIAN_POINT('Ctrl Pts',(-22.5817750440793,-12.8022252144536,
113.585531734144)) ;
#179875=CARTESIAN_POINT('Ctrl Pts',(-22.5079711800751,-12.8022253005655,
113.609762713133)) ;
#179876=CARTESIAN_POINT('Ctrl Pts',(-22.434167316071,-12.8022253866775,
113.633993692123)) ;
#179877=CARTESIAN_POINT('Ctrl Pts',(-22.4154591262606,-12.7556873482899,
113.577011566613)) ;
#179878=CARTESIAN_POINT('Ctrl Pts',(-22.3967509364503,-12.7091493099022,
113.520029441103)) ;
#179879=CARTESIAN_POINT('Ctrl Pts',(-22.4705548004545,-12.7091492237902,
113.495798462113)) ;
#179880=CARTESIAN_POINT('Ctrl Pts',(-22.5443586644586,-12.7091491376783,
113.471567483124)) ;
#179881=CARTESIAN_POINT('Ctrl Pts',(-22.5630668542689,-12.7556871760659,
113.528549608634)) ;
#179882=CARTESIAN_POINT('Ctrl Pts',(-22.5073121196337,-13.0091921750313,
113.394296840887)) ;
#179883=CARTESIAN_POINT('Ctrl Pts',(-22.5292047849245,-13.038100701856,
113.460978364909)) ;
#179884=CARTESIAN_POINT('Ctrl Pts',(-22.4554009289081,-13.03810080188,113.485209368228)) ;
#179885=CARTESIAN_POINT('Ctrl Pts',(-22.3815970728916,-13.038100901904,
113.509440371547)) ;
#179886=CARTESIAN_POINT('Ctrl Pts',(-22.3597044076008,-13.0091923750794,
113.442758847525)) ;
#179887=CARTESIAN_POINT('Ctrl Pts',(-22.3378117423101,-12.9802838482547,
113.376077323502)) ;
#179888=CARTESIAN_POINT('Ctrl Pts',(-22.4116155983265,-12.9802837482307,
113.351846320183)) ;
#179889=CARTESIAN_POINT('Ctrl Pts',(-22.4854194543429,-12.9802836482067,
113.327615316865)) ;
#179890=CARTESIAN_POINT('Ctrl Pts',(-22.5073121196337,-13.0091921750313,
113.394296840887)) ;
#179891=CARTESIAN_POINT('Ctrl Pts',(-22.4743110003687,-13.2902503547293,
113.32912295841)) ;
#179892=CARTESIAN_POINT('Ctrl Pts',(-22.497808872614,-13.2995791016308,
113.400693683843)) ;
#179893=CARTESIAN_POINT('Ctrl Pts',(-22.424005025375,-13.2995792074157,
113.424924713897)) ;
#179894=CARTESIAN_POINT('Ctrl Pts',(-22.3502011781361,-13.2995793132006,
113.449155743951)) ;
#179895=CARTESIAN_POINT('Ctrl Pts',(-22.3267033058907,-13.2902505662991,
113.377585018517)) ;
#179896=CARTESIAN_POINT('Ctrl Pts',(-22.3032054336454,-13.2809218193976,
113.306014293084)) ;
#179897=CARTESIAN_POINT('Ctrl Pts',(-22.3770092808844,-13.2809217136127,
113.28178326303)) ;
#179898=CARTESIAN_POINT('Ctrl Pts',(-22.4508131281233,-13.2809216078278,
113.257552232976)) ;
#179899=CARTESIAN_POINT('Ctrl Pts',(-22.4743110003687,-13.2902503547293,
113.32912295841)) ;
#179900=CARTESIAN_POINT('Ctrl Pts',(-22.4652747457874,-13.5823834440121,
113.337185548665)) ;
#179901=CARTESIAN_POINT('Ctrl Pts',(-22.4887023578516,-13.5713305139235,
113.408542272981)) ;
#179902=CARTESIAN_POINT('Ctrl Pts',(-22.4148985194354,-13.5713306161393,
113.432773329908)) ;
#179903=CARTESIAN_POINT('Ctrl Pts',(-22.3410946810191,-13.5713307183552,
113.457004386834)) ;
#179904=CARTESIAN_POINT('Ctrl Pts',(-22.317667068955,-13.5823836484438,
113.385647662517)) ;
#179905=CARTESIAN_POINT('Ctrl Pts',(-22.2942394568908,-13.5934365785324,
113.3142909382)) ;
#179906=CARTESIAN_POINT('Ctrl Pts',(-22.368043295307,-13.5934364763166,
113.290059881274)) ;
#179907=CARTESIAN_POINT('Ctrl Pts',(-22.4418471337233,-13.5934363741007,
113.265828824348)) ;
#179908=CARTESIAN_POINT('Ctrl Pts',(-22.4652747457874,-13.5823834440121,
113.337185548665)) ;
#179909=CARTESIAN_POINT('Ctrl Pts',(-22.4804477896373,-13.8618181146796,
113.418880666887)) ;
#179910=CARTESIAN_POINT('Ctrl Pts',(-22.5021170027006,-13.8312391943693,
113.484881591642)) ;
#179911=CARTESIAN_POINT('Ctrl Pts',(-22.428313172045,-13.8312392849538,
113.509112672206)) ;
#179912=CARTESIAN_POINT('Ctrl Pts',(-22.3545093413895,-13.8312393755383,
113.53334375277)) ;
#179913=CARTESIAN_POINT('Ctrl Pts',(-22.3328401283261,-13.8618182958485,
113.467342828015)) ;
#179914=CARTESIAN_POINT('Ctrl Pts',(-22.3111709152628,-13.8923972161587,
113.401341903259)) ;
#179915=CARTESIAN_POINT('Ctrl Pts',(-22.3849747459184,-13.8923971255743,
113.377110822695)) ;
#179916=CARTESIAN_POINT('Ctrl Pts',(-22.4587785765739,-13.8923970349898,
113.352879742131)) ;
#179917=CARTESIAN_POINT('Ctrl Pts',(-22.4804477896373,-13.8618181146796,
113.418880666887)) ;
#179918=CARTESIAN_POINT('Ctrl Pts',(-22.517518476082,-14.1083106024044,
113.567088552821)) ;
#179919=CARTESIAN_POINT('Ctrl Pts',(-22.5359014970355,-14.0604763693046,
113.623080266709)) ;
#179920=CARTESIAN_POINT('Ctrl Pts',(-22.4620976726408,-14.0604764428427,
113.647311366343)) ;
#179921=CARTESIAN_POINT('Ctrl Pts',(-22.3882938482461,-14.0604765163808,
113.671542465977)) ;
#179922=CARTESIAN_POINT('Ctrl Pts',(-22.3699108272926,-14.1083107494807,
113.615550752088)) ;
#179923=CARTESIAN_POINT('Ctrl Pts',(-22.3515278063391,-14.1561449825805,
113.559559038199)) ;
#179924=CARTESIAN_POINT('Ctrl Pts',(-22.4253316307338,-14.1561449090424,
113.535327938566)) ;
#179925=CARTESIAN_POINT('Ctrl Pts',(-22.4991354551285,-14.1561448355042,
113.511096838932)) ;
#179926=CARTESIAN_POINT('Ctrl Pts',(-22.517518476082,-14.1083106024044,
113.567088552821)) ;
#179927=CARTESIAN_POINT('Ctrl Pts',(-22.5736052210533,-14.3070623418306,
113.773452298608)) ;
#179928=CARTESIAN_POINT('Ctrl Pts',(-22.5873648692715,-14.2452796350311,
113.81536196524)) ;
#179929=CARTESIAN_POINT('Ctrl Pts',(-22.5135610487874,-14.2452796860699,
113.839593076785)) ;
#179930=CARTESIAN_POINT('Ctrl Pts',(-22.4397572283033,-14.2452797371086,
113.86382418833)) ;
#179931=CARTESIAN_POINT('Ctrl Pts',(-22.4259975800851,-14.3070624439081,
113.821914521697)) ;
#179932=CARTESIAN_POINT('Ctrl Pts',(-22.412237931867,-14.3688451507076,
113.780004855065)) ;
#179933=CARTESIAN_POINT('Ctrl Pts',(-22.4860417523511,-14.3688450996689,
113.75577374352)) ;
#179934=CARTESIAN_POINT('Ctrl Pts',(-22.5598455728352,-14.3688450486301,
113.731542631975)) ;
#179935=CARTESIAN_POINT('Ctrl Pts',(-22.5736052210533,-14.3070623418306,
113.773452298608)) ;
#179936=CARTESIAN_POINT('Ctrl Pts',(-22.6439238545744,-14.4418892785907,
114.023216814566)) ;
#179937=CARTESIAN_POINT('Ctrl Pts',(-22.652058457175,-14.370599628049,114.047993499991)) ;
#179938=CARTESIAN_POINT('Ctrl Pts',(-22.57825463788,-14.3705996550827,114.072224615158)) ;
#179939=CARTESIAN_POINT('Ctrl Pts',(-22.504450818585,-14.3705996821164,
114.096455730324)) ;
#179940=CARTESIAN_POINT('Ctrl Pts',(-22.4963162159844,-14.4418893326581,
114.071679044899)) ;
#179941=CARTESIAN_POINT('Ctrl Pts',(-22.4881816133838,-14.5131789831999,
114.046902359473)) ;
#179942=CARTESIAN_POINT('Ctrl Pts',(-22.5619854326788,-14.5131789561661,
114.022671244307)) ;
#179943=CARTESIAN_POINT('Ctrl Pts',(-22.6357892519738,-14.5131789291324,
113.99844012914)) ;
#179944=CARTESIAN_POINT('Ctrl Pts',(-22.6439238545744,-14.4418892785907,
114.023216814566)) ;
#179945=CARTESIAN_POINT('Ctrl Pts',(-22.7221906575843,-14.502692884587,
114.29704932502)) ;
#179946=CARTESIAN_POINT('Ctrl Pts',(-22.7241395691929,-14.4270502382033,
114.302985393882)) ;
#179947=CARTESIAN_POINT('Ctrl Pts',(-22.6503357490113,-14.4270502433144,
114.327216506348)) ;
#179948=CARTESIAN_POINT('Ctrl Pts',(-22.5765319288297,-14.4270502484255,
114.351447618814)) ;
#179949=CARTESIAN_POINT('Ctrl Pts',(-22.5745830172211,-14.5026928948091,
114.345511549952)) ;
#179950=CARTESIAN_POINT('Ctrl Pts',(-22.5726341056125,-14.5783355411928,
114.339575481091)) ;
#179951=CARTESIAN_POINT('Ctrl Pts',(-22.6464379257941,-14.5783355360817,
114.315344368625)) ;
#179952=CARTESIAN_POINT('Ctrl Pts',(-22.7202417459757,-14.5783355309706,
114.291113256159)) ;
#179953=CARTESIAN_POINT('Ctrl Pts',(-22.7221906575843,-14.502692884587,
114.29704932502)) ;
#179954=CARTESIAN_POINT('Ctrl Pts',(-22.8020413108005,-14.4862255258319,
114.575584821507)) ;
#179955=CARTESIAN_POINT('Ctrl Pts',(-22.7976870656786,-14.4116185668452,
114.562322492106)) ;
#179956=CARTESIAN_POINT('Ctrl Pts',(-22.7238832430576,-14.4116185533067,
114.586553597142)) ;
#179957=CARTESIAN_POINT('Ctrl Pts',(-22.6500794204367,-14.4116185397681,
114.610784702179)) ;
#179958=CARTESIAN_POINT('Ctrl Pts',(-22.6544336655587,-14.4862254987549,
114.62404703158)) ;
#179959=CARTESIAN_POINT('Ctrl Pts',(-22.6587879106807,-14.5608324577416,
114.637309360981)) ;
#179960=CARTESIAN_POINT('Ctrl Pts',(-22.7325917333016,-14.5608324712802,
114.613078255944)) ;
#179961=CARTESIAN_POINT('Ctrl Pts',(-22.8063955559225,-14.5608324848187,
114.588847150908)) ;
#179962=CARTESIAN_POINT('Ctrl Pts',(-22.8020413108005,-14.4862255258319,
114.575584821507)) ;
#179963=CARTESIAN_POINT('Ctrl Pts',(-22.877609829832,-14.3934141564473,
114.841215988645)) ;
#179964=CARTESIAN_POINT('Ctrl Pts',(-22.867238975887,-14.3251742595679,
114.809628039706)) ;
#179965=CARTESIAN_POINT('Ctrl Pts',(-22.7934351490755,-14.325174232371,
114.833859131978)) ;
#179966=CARTESIAN_POINT('Ctrl Pts',(-22.719631322264,-14.3251742051741,
114.858090224251)) ;
#179967=CARTESIAN_POINT('Ctrl Pts',(-22.730002176209,-14.3934141020535,
114.889678173191)) ;
#179968=CARTESIAN_POINT('Ctrl Pts',(-22.7403730301541,-14.4616539989329,
114.921266122131)) ;
#179969=CARTESIAN_POINT('Ctrl Pts',(-22.8141768569656,-14.4616540261298,
114.897035029858)) ;
#179970=CARTESIAN_POINT('Ctrl Pts',(-22.8879806837771,-14.4616540533267,
114.872803937585)) ;
#179971=CARTESIAN_POINT('Ctrl Pts',(-22.877609829832,-14.3934141564473,
114.841215988645)) ;
#179972=CARTESIAN_POINT('Ctrl Pts',(-22.9425681516689,-14.2302607448999,
115.074611405796)) ;
#179973=CARTESIAN_POINT('Ctrl Pts',(-22.9269105859837,-14.1733086335148,
115.026920986085)) ;
#179974=CARTESIAN_POINT('Ctrl Pts',(-22.8531067540947,-14.1733085993244,
115.051152062893)) ;
#179975=CARTESIAN_POINT('Ctrl Pts',(-22.7793029222056,-14.173308565134,
115.0753831397)) ;
#179976=CARTESIAN_POINT('Ctrl Pts',(-22.7949604878908,-14.2302606765191,
115.123073559411)) ;
#179977=CARTESIAN_POINT('Ctrl Pts',(-22.810618053576,-14.2872127879042,
115.170763979122)) ;
#179978=CARTESIAN_POINT('Ctrl Pts',(-22.884421885465,-14.2872128220946,
115.146532902315)) ;
#179979=CARTESIAN_POINT('Ctrl Pts',(-22.9582257173541,-14.287212856285,
115.122301825507)) ;
#179980=CARTESIAN_POINT('Ctrl Pts',(-22.9425681516689,-14.2302607448999,
115.074611405796)) ;
#179981=CARTESIAN_POINT('Ctrl Pts',(-22.9912511714667,-14.0081666908763,
115.258483536822)) ;
#179982=CARTESIAN_POINT('Ctrl Pts',(-22.9714340856062,-13.9666350467411,
115.198123889987)) ;
#179983=CARTESIAN_POINT('Ctrl Pts',(-22.8976302488478,-13.9666350124539,
115.222354951962)) ;
#179984=CARTESIAN_POINT('Ctrl Pts',(-22.8238264120893,-13.9666349781666,
115.246586013938)) ;
#179985=CARTESIAN_POINT('Ctrl Pts',(-22.8436434979498,-14.0081666223018,
115.306945660774)) ;
#179986=CARTESIAN_POINT('Ctrl Pts',(-22.8634605838102,-14.0496982664369,
115.36730530761)) ;
#179987=CARTESIAN_POINT('Ctrl Pts',(-22.9372644205687,-14.0496983007242,
115.343074245634)) ;
#179988=CARTESIAN_POINT('Ctrl Pts',(-23.0110682573271,-14.0496983350115,
115.318843183658)) ;
#179989=CARTESIAN_POINT('Ctrl Pts',(-22.9912511714667,-14.0081666908763,
115.258483536822)) ;
#179990=CARTESIAN_POINT('Ctrl Pts',(-23.0192337790016,-13.7466548362381,
115.378918754356)) ;
#179991=CARTESIAN_POINT('Ctrl Pts',(-22.9967045463713,-13.7233199580348,
115.31029834618)) ;
#179992=CARTESIAN_POINT('Ctrl Pts',(-22.9229007059932,-13.7233199251522,
115.334529397131)) ;
#179993=CARTESIAN_POINT('Ctrl Pts',(-22.849096865615,-13.7233198922696,
115.358760448081)) ;
#179994=CARTESIAN_POINT('Ctrl Pts',(-22.8716260982453,-13.7466547704729,
115.427380856258)) ;
#179995=CARTESIAN_POINT('Ctrl Pts',(-22.8941553308756,-13.7699896486762,
115.496001264434)) ;
#179996=CARTESIAN_POINT('Ctrl Pts',(-22.9679591712538,-13.7699896815587,
115.471770213484)) ;
#179997=CARTESIAN_POINT('Ctrl Pts',(-23.041763011632,-13.7699897144413,
115.447539162533)) ;
#179998=CARTESIAN_POINT('Ctrl Pts',(-23.0192337790016,-13.7466548362381,
115.378918754356)) ;
#179999=CARTESIAN_POINT('Ctrl Pts',(-23.0243744063994,-13.4587847124533,
115.430169417964)) ;
#180000=CARTESIAN_POINT('Ctrl Pts',(-23.0007154115326,-13.4555144548359,
115.358107936487)) ;
#180001=CARTESIAN_POINT('Ctrl Pts',(-22.9269115681353,-13.4555144300918,
115.382338978242)) ;
#180002=CARTESIAN_POINT('Ctrl Pts',(-22.8531077247379,-13.4555144053477,
115.406570019997)) ;
#180003=CARTESIAN_POINT('Ctrl Pts',(-22.8767667196047,-13.4587846629652,
115.478631501474)) ;
#180004=CARTESIAN_POINT('Ctrl Pts',(-22.9004257144714,-13.4620549205826,
115.550692982951)) ;
#180005=CARTESIAN_POINT('Ctrl Pts',(-22.9742295578688,-13.4620549453267,
115.526461941196)) ;
#180006=CARTESIAN_POINT('Ctrl Pts',(-23.0480334012661,-13.4620549700708,
115.502230899441)) ;
#180007=CARTESIAN_POINT('Ctrl Pts',(-23.0243744063994,-13.4587847124533,
115.430169417964)) ;
#180008=CARTESIAN_POINT('Ctrl Pts',(-23.0049652251957,-13.1685102080527,
115.4065743669)) ;
#180009=CARTESIAN_POINT('Ctrl Pts',(-22.9818905294018,-13.1855034690251,
115.336292566279)) ;
#180010=CARTESIAN_POINT('Ctrl Pts',(-22.908086684634,-13.1855034529917,
115.36052360386)) ;
#180011=CARTESIAN_POINT('Ctrl Pts',(-22.8342828398661,-13.1855034369582,
115.38475464144)) ;
#180012=CARTESIAN_POINT('Ctrl Pts',(-22.85735753566,-13.1685101759858,115.455036442061)) ;
#180013=CARTESIAN_POINT('Ctrl Pts',(-22.8804322314538,-13.1515169150133,
115.525318242682)) ;
#180014=CARTESIAN_POINT('Ctrl Pts',(-22.9542360762216,-13.1515169310468,
115.501087205101)) ;
#180015=CARTESIAN_POINT('Ctrl Pts',(-23.0280399209895,-13.1515169470802,
115.476856167521)) ;
#180016=CARTESIAN_POINT('Ctrl Pts',(-23.0049652251957,-13.1685102080527,
115.4065743669)) ;
#180017=CARTESIAN_POINT('Ctrl Pts',(-22.9622751071858,-12.8978336872395,
115.311834565575)) ;
#180018=CARTESIAN_POINT('Ctrl Pts',(-22.9414163104123,-12.9337522455578,
115.248302035944)) ;
#180019=CARTESIAN_POINT('Ctrl Pts',(-22.8676124651999,-12.9337522361366,
115.272533072171)) ;
#180020=CARTESIAN_POINT('Ctrl Pts',(-22.7938086199876,-12.9337522267154,
115.296764108397)) ;
#180021=CARTESIAN_POINT('Ctrl Pts',(-22.814667416761,-12.897833668397,115.360296638028)) ;
#180022=CARTESIAN_POINT('Ctrl Pts',(-22.8355262135344,-12.8619151100786,
115.423829167659)) ;
#180023=CARTESIAN_POINT('Ctrl Pts',(-22.9093300587468,-12.8619151194999,
115.399598131433)) ;
#180024=CARTESIAN_POINT('Ctrl Pts',(-22.9831339039592,-12.8619151289211,
115.375367095206)) ;
#180025=CARTESIAN_POINT('Ctrl Pts',(-22.9622751071858,-12.8978336872395,
115.311834565575)) ;
#180026=CARTESIAN_POINT('Ctrl Pts',(-22.8977448880343,-12.6619537350285,
115.150913911777)) ;
#180027=CARTESIAN_POINT('Ctrl Pts',(-22.8806231861635,-12.7143974709413,
115.098763970377)) ;
#180028=CARTESIAN_POINT('Ctrl Pts',(-22.8068193417578,-12.714397468419,
115.12299500906)) ;
#180029=CARTESIAN_POINT('Ctrl Pts',(-22.7330154973522,-12.7143974658967,
115.147226047744)) ;
#180030=CARTESIAN_POINT('Ctrl Pts',(-22.750137199223,-12.6619537299839,
115.199375989144)) ;
#180031=CARTESIAN_POINT('Ctrl Pts',(-22.7672589010938,-12.6095099940711,
115.251525930544)) ;
#180032=CARTESIAN_POINT('Ctrl Pts',(-22.8410627454994,-12.6095099965934,
115.22729489186)) ;
#180033=CARTESIAN_POINT('Ctrl Pts',(-22.9148665899051,-12.6095099991157,
115.203063853177)) ;
#180034=CARTESIAN_POINT('Ctrl Pts',(-22.8977448880343,-12.6619537350285,
115.150913911777)) ;
#180035=CARTESIAN_POINT('Ctrl Pts',(-22.8158701194052,-12.4816257056073,
114.937014037923)) ;
#180036=CARTESIAN_POINT('Ctrl Pts',(-22.803705693731,-12.5467399887244,
114.899963160045)) ;
#180037=CARTESIAN_POINT('Ctrl Pts',(-22.7299018503216,-12.5467399890346,
114.924194201763)) ;
#180038=CARTESIAN_POINT('Ctrl Pts',(-22.6560980069122,-12.5467399893448,
114.948425243481)) ;
#180039=CARTESIAN_POINT('Ctrl Pts',(-22.6682624325864,-12.4816257062277,
114.985476121359)) ;
#180040=CARTESIAN_POINT('Ctrl Pts',(-22.6804268582606,-12.4165114231106,
115.022526999237)) ;
#180041=CARTESIAN_POINT('Ctrl Pts',(-22.75423070167,-12.4165114228005,114.998295957519)) ;
#180042=CARTESIAN_POINT('Ctrl Pts',(-22.8280345450794,-12.4165114224903,
114.974064915801)) ;
#180043=CARTESIAN_POINT('Ctrl Pts',(-22.8158701194052,-12.4816257056073,
114.937014037923)) ;
#180044=CARTESIAN_POINT('Ctrl Pts',(-22.7221314995921,-12.3684889471066,
114.686813418536)) ;
#180045=CARTESIAN_POINT('Ctrl Pts',(-22.7157636589691,-12.441600008621,
114.667418003494)) ;
#180046=CARTESIAN_POINT('Ctrl Pts',(-22.6419598163146,-12.441600009445,
114.691649047512)) ;
#180047=CARTESIAN_POINT('Ctrl Pts',(-22.5681559736601,-12.4416000102689,
114.715880091529)) ;
#180048=CARTESIAN_POINT('Ctrl Pts',(-22.5745238142832,-12.3684889487544,
114.735275506571)) ;
#180049=CARTESIAN_POINT('Ctrl Pts',(-22.5808916549062,-12.2953778872399,
114.754670921612)) ;
#180050=CARTESIAN_POINT('Ctrl Pts',(-22.6546954975606,-12.295377886416,
114.730439877594)) ;
#180051=CARTESIAN_POINT('Ctrl Pts',(-22.7284993402151,-12.2953778855921,
114.706208833577)) ;
#180052=CARTESIAN_POINT('Ctrl Pts',(-22.7221314995921,-12.3684889471066,
114.686813418536)) ;
#180053=CARTESIAN_POINT('Ctrl Pts',(-22.6211642213523,-12.3299903879882,
114.414896154153)) ;
#180054=CARTESIAN_POINT('Ctrl Pts',(-22.6211005272298,-12.4058988295515,
114.414702152198)) ;
#180055=CARTESIAN_POINT('Ctrl Pts',(-22.547296684874,-12.4058988295036,
114.438933197125)) ;
#180056=CARTESIAN_POINT('Ctrl Pts',(-22.4734928425182,-12.4058988294557,
114.463164242052)) ;
#180057=CARTESIAN_POINT('Ctrl Pts',(-22.4735565366407,-12.3299903878923,
114.463358244007)) ;
#180058=CARTESIAN_POINT('Ctrl Pts',(-22.4736202307632,-12.254081946329,
114.463552245962)) ;
#180059=CARTESIAN_POINT('Ctrl Pts',(-22.547424073119,-12.2540819463769,
114.439321201035)) ;
#180060=CARTESIAN_POINT('Ctrl Pts',(-22.6212279154748,-12.2540819464249,
114.415090156108)) ;
#180061=CARTESIAN_POINT('Ctrl Pts',(-22.6211642213523,-12.3299903879882,
114.414896154153)) ;
#180062=CARTESIAN_POINT('Ctrl Pts',(-22.5210459323926,-12.3696139932957,
114.145284395622)) ;
#180063=CARTESIAN_POINT('Ctrl Pts',(-22.5272419402638,-12.4428670872802,
114.164156435911)) ;
#180064=CARTESIAN_POINT('Ctrl Pts',(-22.4534380974035,-12.4428670865975,
114.188387479302)) ;
#180065=CARTESIAN_POINT('Ctrl Pts',(-22.3796342545432,-12.4428670859149,
114.212618522693)) ;
#180066=CARTESIAN_POINT('Ctrl Pts',(-22.373438246672,-12.3696139919303,
114.193746482403)) ;
#180067=CARTESIAN_POINT('Ctrl Pts',(-22.3672422388009,-12.2963608979458,
114.174874442114)) ;
#180068=CARTESIAN_POINT('Ctrl Pts',(-22.4410460816612,-12.2963608986285,
114.150643398723)) ;
#180069=CARTESIAN_POINT('Ctrl Pts',(-22.5148499245215,-12.2963608993112,
114.126412355333)) ;
#180070=CARTESIAN_POINT('Ctrl Pts',(-22.5210459323926,-12.3696139932957,
114.145284395622)) ;
#180071=CARTESIAN_POINT('Ctrl Pts',(-22.4270329126327,-12.4839372794238,
113.894388923213)) ;
#180072=CARTESIAN_POINT('Ctrl Pts',(-22.4390689464251,-12.5493150647165,
113.931048740115)) ;
#180073=CARTESIAN_POINT('Ctrl Pts',(-22.3652651026278,-12.5493150649477,
113.955279780652)) ;
#180074=CARTESIAN_POINT('Ctrl Pts',(-22.2914612588304,-12.549315065179,
113.979510821188)) ;
#180075=CARTESIAN_POINT('Ctrl Pts',(-22.279425225038,-12.4839372798862,
113.942851004286)) ;
#180076=CARTESIAN_POINT('Ctrl Pts',(-22.2673891912455,-12.4185594945934,
113.906191187384)) ;
#180077=CARTESIAN_POINT('Ctrl Pts',(-22.3411930350429,-12.4185594943622,
113.881960146848)) ;
#180078=CARTESIAN_POINT('Ctrl Pts',(-22.4149968788402,-12.418559494131,
113.857729106311)) ;
#180079=CARTESIAN_POINT('Ctrl Pts',(-22.4270329126327,-12.4839372794238,
113.894388923213)) ;
#180080=CARTESIAN_POINT('Ctrl Pts',(-22.3450439580957,-12.6667316342934,
113.680343028654)) ;
#180081=CARTESIAN_POINT('Ctrl Pts',(-22.3620843484137,-12.7194414647668,
113.73224530796)) ;
#180082=CARTESIAN_POINT('Ctrl Pts',(-22.2882805032508,-12.7194414698136,
113.756476344337)) ;
#180083=CARTESIAN_POINT('Ctrl Pts',(-22.2144766580878,-12.7194414748605,
113.780707380714)) ;
#180084=CARTESIAN_POINT('Ctrl Pts',(-22.1974362677697,-12.6667316443871,
113.728805101408)) ;
#180085=CARTESIAN_POINT('Ctrl Pts',(-22.1803958774517,-12.6140218139138,
113.676902822102)) ;
#180086=CARTESIAN_POINT('Ctrl Pts',(-22.2541997226147,-12.6140218088669,
113.652671785725)) ;
#180087=CARTESIAN_POINT('Ctrl Pts',(-22.3280035677777,-12.6140218038201,
113.628440749348)) ;
#180088=CARTESIAN_POINT('Ctrl Pts',(-22.3450439580957,-12.6667316342934,
113.680343028654)) ;
#180089=CARTESIAN_POINT('Ctrl Pts',(-22.2812994602008,-12.9020313562946,
113.521591306162)) ;
#180090=CARTESIAN_POINT('Ctrl Pts',(-22.3020828222175,-12.9383882322268,
113.584894073218)) ;
#180091=CARTESIAN_POINT('Ctrl Pts',(-22.2282789766405,-12.9383882439588,
113.609125108335)) ;
#180092=CARTESIAN_POINT('Ctrl Pts',(-22.1544751310636,-12.9383882556908,
113.633356143451)) ;
#180093=CARTESIAN_POINT('Ctrl Pts',(-22.133691769047,-12.9020313797586,
113.570053376394)) ;
#180094=CARTESIAN_POINT('Ctrl Pts',(-22.1129084070303,-12.8656745038264,
113.506750609338)) ;
#180095=CARTESIAN_POINT('Ctrl Pts',(-22.1867122526073,-12.8656744920944,
113.482519574222)) ;
#180096=CARTESIAN_POINT('Ctrl Pts',(-22.2605160981842,-12.8656744803624,
113.458288539106)) ;
#180097=CARTESIAN_POINT('Ctrl Pts',(-22.2812994602008,-12.9020313562946,
113.521591306162)) ;
#180098=CARTESIAN_POINT('Ctrl Pts',(-22.2388473261469,-13.1740426154344,
113.427694180976)) ;
#180099=CARTESIAN_POINT('Ctrl Pts',(-22.2618922493966,-13.1914596717363,
113.497885298515)) ;
#180100=CARTESIAN_POINT('Ctrl Pts',(-22.1880884043741,-13.1914596914773,
113.52211633532)) ;
#180101=CARTESIAN_POINT('Ctrl Pts',(-22.1142845593517,-13.1914597112182,
113.546347372125)) ;
#180102=CARTESIAN_POINT('Ctrl Pts',(-22.091239636102,-13.1740426549163,
113.476156254586)) ;
#180103=CARTESIAN_POINT('Ctrl Pts',(-22.0681947128524,-13.1566255986144,
113.405965137047)) ;
#180104=CARTESIAN_POINT('Ctrl Pts',(-22.1419985578748,-13.1566255788734,
113.381734100242)) ;
#180105=CARTESIAN_POINT('Ctrl Pts',(-22.2158024028973,-13.1566255591325,
113.357503063437)) ;
#180106=CARTESIAN_POINT('Ctrl Pts',(-22.2388473261469,-13.1740426154344,
113.427694180976)) ;
#180107=CARTESIAN_POINT('Ctrl Pts',(-22.2199943655419,-13.4634545824485,
113.40566955685)) ;
#180108=CARTESIAN_POINT('Ctrl Pts',(-22.243656437071,-13.4606896668886,
113.47774040833)) ;
#180109=CARTESIAN_POINT('Ctrl Pts',(-22.1698525937983,-13.4606896946661,
113.501971450465)) ;
#180110=CARTESIAN_POINT('Ctrl Pts',(-22.0960487505255,-13.4606897224437,
113.526202492599)) ;
#180111=CARTESIAN_POINT('Ctrl Pts',(-22.0723866789964,-13.4634546380036,
113.454131641119)) ;
#180112=CARTESIAN_POINT('Ctrl Pts',(-22.0487246074673,-13.4662195535635,
113.382060789639)) ;
#180113=CARTESIAN_POINT('Ctrl Pts',(-22.12252845074,-13.466219525786,113.357829747505)) ;
#180114=CARTESIAN_POINT('Ctrl Pts',(-22.1963322940127,-13.4662194980085,
113.33359870537)) ;
#180115=CARTESIAN_POINT('Ctrl Pts',(-22.2199943655419,-13.4634545824485,
113.40566955685)) ;
#180116=CARTESIAN_POINT('Ctrl Pts',(-22.2254048356507,-13.7505708131454,
113.45766775839)) ;
#180117=CARTESIAN_POINT('Ctrl Pts',(-22.2479884314305,-13.7277551955946,
113.526453746576)) ;
#180118=CARTESIAN_POINT('Ctrl Pts',(-22.1741845912889,-13.7277552307989,
113.550684798247)) ;
#180119=CARTESIAN_POINT('Ctrl Pts',(-22.1003807511473,-13.7277552660031,
113.574915849919)) ;
#180120=CARTESIAN_POINT('Ctrl Pts',(-22.0777971553675,-13.7505708835539,
113.506129861733)) ;
#180121=CARTESIAN_POINT('Ctrl Pts',(-22.0552135595877,-13.7733865011047,
113.437343873547)) ;
#180122=CARTESIAN_POINT('Ctrl Pts',(-22.1290173997293,-13.7733864659004,
113.413112821876)) ;
#180123=CARTESIAN_POINT('Ctrl Pts',(-22.2028212398709,-13.7733864306961,
113.388881770204)) ;
#180124=CARTESIAN_POINT('Ctrl Pts',(-22.2254048356507,-13.7505708131454,
113.45766775839)) ;
#180125=CARTESIAN_POINT('Ctrl Pts',(-22.253988225315,-14.0133363300327,
113.580184190739)) ;
#180126=CARTESIAN_POINT('Ctrl Pts',(-22.2738750852953,-13.9721415095329,
113.64075635663)) ;
#180127=CARTESIAN_POINT('Ctrl Pts',(-22.2000712494337,-13.9721415478717,
113.664987421337)) ;
#180128=CARTESIAN_POINT('Ctrl Pts',(-22.126267413572,-13.9721415862106,
113.689218486045)) ;
#180129=CARTESIAN_POINT('Ctrl Pts',(-22.1063805535917,-14.0133364067105,
113.628646320154)) ;
#180130=CARTESIAN_POINT('Ctrl Pts',(-22.0864936936113,-14.0545312272103,
113.568074154263)) ;
#180131=CARTESIAN_POINT('Ctrl Pts',(-22.160297529473,-14.0545311888715,
113.543843089555)) ;
#180132=CARTESIAN_POINT('Ctrl Pts',(-22.2341013653346,-14.0545311505326,
113.519612024848)) ;
#180133=CARTESIAN_POINT('Ctrl Pts',(-22.253988225315,-14.0133363300327,
113.580184190739)) ;
#180134=CARTESIAN_POINT('Ctrl Pts',(-22.302884463881,-14.2335678065818,
113.764575325811)) ;
#180135=CARTESIAN_POINT('Ctrl Pts',(-22.3186524020933,-14.1769371406859,
113.812601920414)) ;
#180136=CARTESIAN_POINT('Ctrl Pts',(-22.2448485711463,-14.1769371770333,
113.836833000091)) ;
#180137=CARTESIAN_POINT('Ctrl Pts',(-22.1710447401993,-14.1769372133807,
113.861064079767)) ;
#180138=CARTESIAN_POINT('Ctrl Pts',(-22.155276801987,-14.2335678792767,
113.813037485163)) ;
#180139=CARTESIAN_POINT('Ctrl Pts',(-22.1395088637747,-14.2901985451726,
113.76501089056)) ;
#180140=CARTESIAN_POINT('Ctrl Pts',(-22.2133126947217,-14.2901985088252,
113.740779810884)) ;
#180141=CARTESIAN_POINT('Ctrl Pts',(-22.2871165256687,-14.2901984724778,
113.716548731207)) ;
#180142=CARTESIAN_POINT('Ctrl Pts',(-22.302884463881,-14.2335678065818,
113.764575325811)) ;
#180143=CARTESIAN_POINT('Ctrl Pts',(-22.3681132301931,-14.3958087768564,
113.998825699408)) ;
#180144=CARTESIAN_POINT('Ctrl Pts',(-22.3786137764085,-14.3277685970779,
114.030808667693)) ;
#180145=CARTESIAN_POINT('Ctrl Pts',(-22.304809950723,-14.3277686257104,
114.055039763396)) ;
#180146=CARTESIAN_POINT('Ctrl Pts',(-22.2310061250376,-14.327768654343,
114.079270859098)) ;
#180147=CARTESIAN_POINT('Ctrl Pts',(-22.2205055788222,-14.3958088341215,
114.047287890812)) ;
#180148=CARTESIAN_POINT('Ctrl Pts',(-22.2100050326069,-14.4638490139001,
114.015304922527)) ;
#180149=CARTESIAN_POINT('Ctrl Pts',(-22.2838088582923,-14.4638489852675,
113.991073826824)) ;
#180150=CARTESIAN_POINT('Ctrl Pts',(-22.3576126839778,-14.463848956635,
113.966842731122)) ;
#180151=CARTESIAN_POINT('Ctrl Pts',(-22.3681132301931,-14.3958087768564,
113.998825699408)) ;
#180152=CARTESIAN_POINT('Ctrl Pts',(-22.443875331704,-14.4872051600084,
114.265066140511)) ;
#180153=CARTESIAN_POINT('Ctrl Pts',(-22.4483673589723,-14.4126853477426,
114.278748129396)) ;
#180154=CARTESIAN_POINT('Ctrl Pts',(-22.3745635375518,-14.4126853615341,
114.302979238089)) ;
#180155=CARTESIAN_POINT('Ctrl Pts',(-22.3007597161312,-14.4126853753255,
114.327210346781)) ;
#180156=CARTESIAN_POINT('Ctrl Pts',(-22.2962676888629,-14.4872051875913,
114.313528357897)) ;
#180157=CARTESIAN_POINT('Ctrl Pts',(-22.2917756615946,-14.561724999857,
114.299846369012)) ;
#180158=CARTESIAN_POINT('Ctrl Pts',(-22.3655794830151,-14.5617249860656,
114.275615260319)) ;
#180159=CARTESIAN_POINT('Ctrl Pts',(-22.4393833044357,-14.5617249722742,
114.251384151627)) ;
#180160=CARTESIAN_POINT('Ctrl Pts',(-22.443875331704,-14.4872051600084,
114.265066140511)) ;
#180161=CARTESIAN_POINT('Ctrl Pts',(-22.5236867142171,-14.5023836342265,
114.543451391417)) ;
#180162=CARTESIAN_POINT('Ctrl Pts',(-22.5218827377138,-14.4266966491582,
114.53795676855)) ;
#180163=CARTESIAN_POINT('Ctrl Pts',(-22.4480789185891,-14.4266966434283,
114.562187884235)) ;
#180164=CARTESIAN_POINT('Ctrl Pts',(-22.3742750994644,-14.4266966376984,
114.586418999921)) ;
#180165=CARTESIAN_POINT('Ctrl Pts',(-22.3760790759678,-14.5023836227667,
114.591913622788)) ;
#180166=CARTESIAN_POINT('Ctrl Pts',(-22.3778830524711,-14.5780706078349,
114.597408245655)) ;
#180167=CARTESIAN_POINT('Ctrl Pts',(-22.4516868715958,-14.5780706135648,
114.573177129969)) ;
#180168=CARTESIAN_POINT('Ctrl Pts',(-22.5254906907205,-14.5780706192947,
114.548946014284)) ;
#180169=CARTESIAN_POINT('Ctrl Pts',(-22.5236867142171,-14.5023836342265,
114.543451391417)) ;
#180170=CARTESIAN_POINT('Ctrl Pts',(-22.6023114828813,-14.4395233841403,
114.8185888207)) ;
#180171=CARTESIAN_POINT('Ctrl Pts',(-22.5942777325874,-14.3681145695168,
114.794119311872)) ;
#180172=CARTESIAN_POINT('Ctrl Pts',(-22.5204739146049,-14.3681145402781,
114.818350431036)) ;
#180173=CARTESIAN_POINT('Ctrl Pts',(-22.4466700966224,-14.3681145110395,
114.8425815502)) ;
#180174=CARTESIAN_POINT('Ctrl Pts',(-22.4547038469163,-14.4395233256629,
114.867051059028)) ;
#180175=CARTESIAN_POINT('Ctrl Pts',(-22.4627375972102,-14.5109321402864,
114.891520567857)) ;
#180176=CARTESIAN_POINT('Ctrl Pts',(-22.5365414151927,-14.510932169525,
114.867289448692)) ;
#180177=CARTESIAN_POINT('Ctrl Pts',(-22.6103452331752,-14.5109321987637,
114.843058329528)) ;
#180178=CARTESIAN_POINT('Ctrl Pts',(-22.6023114828813,-14.4395233841403,
114.8185888207)) ;
#180179=CARTESIAN_POINT('Ctrl Pts',(-22.6719122092473,-14.3038981389521,
115.065942143316)) ;
#180180=CARTESIAN_POINT('Ctrl Pts',(-22.6582758145708,-14.2418546197311,
115.024407883578)) ;
#180181=CARTESIAN_POINT('Ctrl Pts',(-22.5844719945869,-14.2418545666607,
115.048638996647)) ;
#180182=CARTESIAN_POINT('Ctrl Pts',(-22.5106681746031,-14.2418545135903,
115.072870109715)) ;
#180183=CARTESIAN_POINT('Ctrl Pts',(-22.5243045692795,-14.3038980328113,
115.114404369452)) ;
#180184=CARTESIAN_POINT('Ctrl Pts',(-22.5379409639559,-14.3659415520323,
115.15593862919)) ;
#180185=CARTESIAN_POINT('Ctrl Pts',(-22.6117447839398,-14.3659416051027,
115.131707516122)) ;
#180186=CARTESIAN_POINT('Ctrl Pts',(-22.6855486039237,-14.3659416581731,
115.107476403053)) ;
#180187=CARTESIAN_POINT('Ctrl Pts',(-22.6719122092473,-14.3038981389521,
115.065942143316)) ;
#180188=CARTESIAN_POINT('Ctrl Pts',(-22.7275755368524,-14.1052991872385,
115.270872462987)) ;
#180189=CARTESIAN_POINT('Ctrl Pts',(-22.7093008428281,-14.057030828904,
115.215210691726)) ;
#180190=CARTESIAN_POINT('Ctrl Pts',(-22.6354970186199,-14.0570307540221,
115.239441791928)) ;
#180191=CARTESIAN_POINT('Ctrl Pts',(-22.5616931944116,-14.0570306791401,
115.263672892129)) ;
#180192=CARTESIAN_POINT('Ctrl Pts',(-22.5799678884359,-14.1052990374745,
115.31933466339)) ;
#180193=CARTESIAN_POINT('Ctrl Pts',(-22.5982425824603,-14.1535673958089,
115.37499643465)) ;
#180194=CARTESIAN_POINT('Ctrl Pts',(-22.6720464066685,-14.1535674706909,
115.350765334449)) ;
#180195=CARTESIAN_POINT('Ctrl Pts',(-22.7458502308768,-14.1535675455729,
115.326534234247)) ;
#180196=CARTESIAN_POINT('Ctrl Pts',(-22.7275755368524,-14.1052991872385,
115.270872462987)) ;
#180197=CARTESIAN_POINT('Ctrl Pts',(-22.7645650054977,-13.8563431079666,
115.419085314818)) ;
#180198=CARTESIAN_POINT('Ctrl Pts',(-22.742945507972,-13.8253850611036,
115.353235811681)) ;
#180199=CARTESIAN_POINT('Ctrl Pts',(-22.6691416774397,-13.8253849680989,
115.377466892621)) ;
#180200=CARTESIAN_POINT('Ctrl Pts',(-22.5953378469074,-13.8253848750942,
115.40169797356)) ;
#180201=CARTESIAN_POINT('Ctrl Pts',(-22.616957344433,-13.8563429219572,
115.467547476697)) ;
#180202=CARTESIAN_POINT('Ctrl Pts',(-22.6385768419586,-13.8873009688202,
115.533396979833)) ;
#180203=CARTESIAN_POINT('Ctrl Pts',(-22.712380672491,-13.8873010618249,
115.509165898894)) ;
#180204=CARTESIAN_POINT('Ctrl Pts',(-22.7861845030233,-13.8873011548297,
115.484934817954)) ;
#180205=CARTESIAN_POINT('Ctrl Pts',(-22.7645650054977,-13.8563431079666,
115.419085314818)) ;
#180206=CARTESIAN_POINT('Ctrl Pts',(-22.7791798044281,-13.5768529523028,
115.499023031472)) ;
#180207=CARTESIAN_POINT('Ctrl Pts',(-22.7557753098736,-13.5653624857166,
115.427736715333)) ;
#180208=CARTESIAN_POINT('Ctrl Pts',(-22.6819714713014,-13.56536238196,115.451967771784)) ;
#180209=CARTESIAN_POINT('Ctrl Pts',(-22.6081676327291,-13.5653622782034,
115.476198828235)) ;
#180210=CARTESIAN_POINT('Ctrl Pts',(-22.6315721272836,-13.5768527447896,
115.547485144374)) ;
#180211=CARTESIAN_POINT('Ctrl Pts',(-22.6549766218381,-13.5883432113757,
115.618771460513)) ;
#180212=CARTESIAN_POINT('Ctrl Pts',(-22.7287804604104,-13.5883433151323,
115.594540404062)) ;
#180213=CARTESIAN_POINT('Ctrl Pts',(-22.8025842989826,-13.5883434188889,
115.570309347611)) ;
#180214=CARTESIAN_POINT('Ctrl Pts',(-22.7791798044281,-13.5768529523028,
115.499023031472)) ;
#180215=CARTESIAN_POINT('Ctrl Pts',(-22.7697827423378,-13.2855121533732,
115.505888509514)) ;
#180216=CARTESIAN_POINT('Ctrl Pts',(-22.7462655648333,-13.2943449974089,
115.434258979246)) ;
#180217=CARTESIAN_POINT('Ctrl Pts',(-22.6724617173834,-13.2943448909631,
115.458490008657)) ;
#180218=CARTESIAN_POINT('Ctrl Pts',(-22.5986578699334,-13.2943447845173,
115.482721038068)) ;
#180219=CARTESIAN_POINT('Ctrl Pts',(-22.6221750474379,-13.2855119404815,
115.554350568336)) ;
#180220=CARTESIAN_POINT('Ctrl Pts',(-22.6456922249424,-13.2766790964458,
115.625980098605)) ;
#180221=CARTESIAN_POINT('Ctrl Pts',(-22.7194960723924,-13.2766792028916,
115.601749069194)) ;
#180222=CARTESIAN_POINT('Ctrl Pts',(-22.7932999198423,-13.2766793093374,
115.577518039783)) ;
#180223=CARTESIAN_POINT('Ctrl Pts',(-22.7697827423378,-13.2855121533732,
115.505888509514)) ;
#180224=CARTESIAN_POINT('Ctrl Pts',(-22.736267599059,-13.0041275578471,
115.439237761638)) ;
#180225=CARTESIAN_POINT('Ctrl Pts',(-22.714322517485,-13.0326186796293,
115.372396581896)) ;
#180226=CARTESIAN_POINT('Ctrl Pts',(-22.6405186612293,-13.0326185795002,
115.396627584487)) ;
#180227=CARTESIAN_POINT('Ctrl Pts',(-22.5667148049737,-13.0326184793711,
115.420858587077)) ;
#180228=CARTESIAN_POINT('Ctrl Pts',(-22.5886598865477,-13.0041273575889,
115.487699766818)) ;
#180229=CARTESIAN_POINT('Ctrl Pts',(-22.6106049681218,-12.9756362358068,
115.554540946559)) ;
#180230=CARTESIAN_POINT('Ctrl Pts',(-22.6844088243775,-12.9756363359359,
115.530309943969)) ;
#180231=CARTESIAN_POINT('Ctrl Pts',(-22.7582126806331,-12.975636436065,
115.506078941379)) ;
#180232=CARTESIAN_POINT('Ctrl Pts',(-22.736267599059,-13.0041275578471,
115.439237761638)) ;
#180233=CARTESIAN_POINT('Ctrl Pts',(-22.6804050530378,-12.7524010633512,
115.304496989377)) ;
#180234=CARTESIAN_POINT('Ctrl Pts',(-22.6615950142437,-12.798508919761,
115.247204644104)) ;
#180235=CARTESIAN_POINT('Ctrl Pts',(-22.5877911501292,-12.798508834093,
115.271435622758)) ;
#180236=CARTESIAN_POINT('Ctrl Pts',(-22.5139872860148,-12.7985087484251,
115.295666601412)) ;
#180237=CARTESIAN_POINT('Ctrl Pts',(-22.5327973248089,-12.7524008920153,
115.352958946684)) ;
#180238=CARTESIAN_POINT('Ctrl Pts',(-22.551607363603,-12.7062930356055,
115.410251291957)) ;
#180239=CARTESIAN_POINT('Ctrl Pts',(-22.6254112277175,-12.7062931212734,
115.386020313304)) ;
#180240=CARTESIAN_POINT('Ctrl Pts',(-22.6992150918319,-12.7062932069414,
115.36178933465)) ;
#180241=CARTESIAN_POINT('Ctrl Pts',(-22.6804050530378,-12.7524010633512,
115.304496989377)) ;
#180242=CARTESIAN_POINT('Ctrl Pts',(-22.6049368462365,-12.5474082659178,
115.110214285938)) ;
#180243=CARTESIAN_POINT('Ctrl Pts',(-22.5906314344715,-12.6078966446447,
115.066642307803)) ;
#180244=CARTESIAN_POINT('Ctrl Pts',(-22.5168275643,-12.6078965805878,115.090873268007)) ;
#180245=CARTESIAN_POINT('Ctrl Pts',(-22.4430236941285,-12.6078965165309,
115.115104228212)) ;
#180246=CARTESIAN_POINT('Ctrl Pts',(-22.4573291058934,-12.5474081378039,
115.158676206348)) ;
#180247=CARTESIAN_POINT('Ctrl Pts',(-22.4716345176584,-12.4869197590769,
115.202248184483)) ;
#180248=CARTESIAN_POINT('Ctrl Pts',(-22.5454383878299,-12.4869198231338,
115.178017224278)) ;
#180249=CARTESIAN_POINT('Ctrl Pts',(-22.6192422580014,-12.4869198871908,
115.153786264074)) ;
#180250=CARTESIAN_POINT('Ctrl Pts',(-22.6049368462365,-12.5474082659178,
115.110214285938)) ;
#180251=CARTESIAN_POINT('Ctrl Pts',(-22.5152721436028,-12.4057612857423,
114.872509443197)) ;
#180252=CARTESIAN_POINT('Ctrl Pts',(-22.506473096668,-12.4762290506085,
114.845708963927)) ;
#180253=CARTESIAN_POINT('Ctrl Pts',(-22.432669222784,-12.4762290124344,
114.869939912825)) ;
#180254=CARTESIAN_POINT('Ctrl Pts',(-22.3588653489,-12.4762289742604,114.894170861722)) ;
#180255=CARTESIAN_POINT('Ctrl Pts',(-22.3676643958349,-12.4057612093942,
114.920971340992)) ;
#180256=CARTESIAN_POINT('Ctrl Pts',(-22.3764634427698,-12.3352934445281,
114.947771820262)) ;
#180257=CARTESIAN_POINT('Ctrl Pts',(-22.4502673166537,-12.3352934827021,
114.923540871364)) ;
#180258=CARTESIAN_POINT('Ctrl Pts',(-22.5240711905377,-12.3352935208762,
114.899309922467)) ;
#180259=CARTESIAN_POINT('Ctrl Pts',(-22.5152721436028,-12.4057612857423,
114.872509443197)) ;
#180260=CARTESIAN_POINT('Ctrl Pts',(-22.416477982246,-12.3361751661113,
114.607093665793)) ;
#180261=CARTESIAN_POINT('Ctrl Pts',(-22.413828814936,-12.4116066467127,
114.599024727648)) ;
#180262=CARTESIAN_POINT('Ctrl Pts',(-22.3400249400517,-12.4116066363173,
114.623255673499)) ;
#180263=CARTESIAN_POINT('Ctrl Pts',(-22.2662210651673,-12.4116066259219,
114.647486619349)) ;
#180264=CARTESIAN_POINT('Ctrl Pts',(-22.2688702324773,-12.3361751453206,
114.655555557494)) ;
#180265=CARTESIAN_POINT('Ctrl Pts',(-22.2715193997872,-12.2607436647193,
114.663624495639)) ;
#180266=CARTESIAN_POINT('Ctrl Pts',(-22.3453232746716,-12.2607436751146,
114.639393549788)) ;
#180267=CARTESIAN_POINT('Ctrl Pts',(-22.4191271495559,-12.26074368551,114.615162603938)) ;
#180268=CARTESIAN_POINT('Ctrl Pts',(-22.416477982246,-12.3361751661113,
114.607093665793)) ;
#180269=CARTESIAN_POINT('Ctrl Pts',(-22.3151654199719,-12.3442704255669,
114.333978009921)) ;
#180270=CARTESIAN_POINT('Ctrl Pts',(-22.318851814107,-12.4192498359007,
114.345206169785)) ;
#180271=CARTESIAN_POINT('Ctrl Pts',(-22.2450479408706,-12.4192498519891,
114.369437120655)) ;
#180272=CARTESIAN_POINT('Ctrl Pts',(-22.1712440676341,-12.4192498680774,
114.393668071524)) ;
#180273=CARTESIAN_POINT('Ctrl Pts',(-22.1675576734989,-12.3442704577436,
114.38243991166)) ;
#180274=CARTESIAN_POINT('Ctrl Pts',(-22.1638712793637,-12.2692910474097,
114.371211751796)) ;
#180275=CARTESIAN_POINT('Ctrl Pts',(-22.2376751526002,-12.2692910313214,
114.346980800926)) ;
#180276=CARTESIAN_POINT('Ctrl Pts',(-22.3114790258367,-12.269291015233,
114.322749850057)) ;
#180277=CARTESIAN_POINT('Ctrl Pts',(-22.3151654199719,-12.3442704255669,
114.333978009921)) ;
#180278=CARTESIAN_POINT('Ctrl Pts',(-22.2178317346334,-12.4291570429794,
114.072959782331)) ;
#180279=CARTESIAN_POINT('Ctrl Pts',(-22.2275858904983,-12.4983225025168,
114.102669365496)) ;
#180280=CARTESIAN_POINT('Ctrl Pts',(-22.1537820211615,-12.4983225412537,
114.126900328243)) ;
#180281=CARTESIAN_POINT('Ctrl Pts',(-22.0799781518247,-12.4983225799905,
114.15113129099)) ;
#180282=CARTESIAN_POINT('Ctrl Pts',(-22.0702239959598,-12.429157120453,
114.121421707825)) ;
#180283=CARTESIAN_POINT('Ctrl Pts',(-22.0604698400949,-12.3599916609156,
114.09171212466)) ;
#180284=CARTESIAN_POINT('Ctrl Pts',(-22.1342737094317,-12.3599916221787,
114.067481161913)) ;
#180285=CARTESIAN_POINT('Ctrl Pts',(-22.2080775787685,-12.3599915834419,
114.043250199166)) ;
#180286=CARTESIAN_POINT('Ctrl Pts',(-22.2178317346334,-12.4291570429794,
114.072959782331)) ;
#180287=CARTESIAN_POINT('Ctrl Pts',(-22.1305576720065,-12.5849331529663,
113.842608904662)) ;
#180288=CARTESIAN_POINT('Ctrl Pts',(-22.1456858757499,-12.6433268351206,
113.888686970688)) ;
#180289=CARTESIAN_POINT('Ctrl Pts',(-22.0718820120717,-12.6433268905322,
113.91291795067)) ;
#180290=CARTESIAN_POINT('Ctrl Pts',(-21.9980781483935,-12.6433269459438,
113.937148930652)) ;
#180291=CARTESIAN_POINT('Ctrl Pts',(-21.98294994465,-12.5849332637895,113.891070864627)) ;
#180292=CARTESIAN_POINT('Ctrl Pts',(-21.9678217409065,-12.5265395816352,
113.844992798601)) ;
#180293=CARTESIAN_POINT('Ctrl Pts',(-22.0416256045847,-12.5265395262236,
113.820761818619)) ;
#180294=CARTESIAN_POINT('Ctrl Pts',(-22.115429468263,-12.526539470812,113.796530838636)) ;
#180295=CARTESIAN_POINT('Ctrl Pts',(-22.1305576720065,-12.5849331529663,
113.842608904662)) ;
#180296=CARTESIAN_POINT('Ctrl Pts',(-22.0589049961337,-12.8005108515807,
113.659850775532)) ;
#180297=CARTESIAN_POINT('Ctrl Pts',(-22.0783245226493,-12.8439413739947,
113.718999518458)) ;
#180298=CARTESIAN_POINT('Ctrl Pts',(-22.0045206655792,-12.8439414387627,
113.743230518568)) ;
#180299=CARTESIAN_POINT('Ctrl Pts',(-21.9307168085092,-12.8439415035308,
113.767461518678)) ;
#180300=CARTESIAN_POINT('Ctrl Pts',(-21.9112972819936,-12.8005109811168,
113.708312775751)) ;
#180301=CARTESIAN_POINT('Ctrl Pts',(-21.8918777554779,-12.7570804587029,
113.649164032825)) ;
#180302=CARTESIAN_POINT('Ctrl Pts',(-21.965681612548,-12.7570803939349,
113.624933032715)) ;
#180303=CARTESIAN_POINT('Ctrl Pts',(-22.039485469618,-12.7570803291668,
113.600702032605)) ;
#180304=CARTESIAN_POINT('Ctrl Pts',(-22.0589049961337,-12.8005108515807,
113.659850775532)) ;
#180305=CARTESIAN_POINT('Ctrl Pts',(-22.0073169664416,-13.060269126664,
113.538192775077)) ;
#180306=CARTESIAN_POINT('Ctrl Pts',(-22.0296337589836,-13.0856291470037,
113.606166122998)) ;
#180307=CARTESIAN_POINT('Ctrl Pts',(-21.9558299085615,-13.0856292137402,
113.630397143356)) ;
#180308=CARTESIAN_POINT('Ctrl Pts',(-21.8820260581393,-13.0856292804768,
113.654628163715)) ;
#180309=CARTESIAN_POINT('Ctrl Pts',(-21.8597092655973,-13.0602692601371,
113.586654815794)) ;
#180310=CARTESIAN_POINT('Ctrl Pts',(-21.8373924730553,-13.0349092397974,
113.518681467873)) ;
#180311=CARTESIAN_POINT('Ctrl Pts',(-21.9111963234774,-13.0349091730608,
113.494450447515)) ;
#180312=CARTESIAN_POINT('Ctrl Pts',(-21.9850001738996,-13.0349091063243,
113.470219427156)) ;
#180313=CARTESIAN_POINT('Ctrl Pts',(-22.0073169664416,-13.060269126664,
113.538192775077)) ;
#180314=CARTESIAN_POINT('Ctrl Pts',(-21.978691089474,-13.3453693583979,
113.486439374298)) ;
#180315=CARTESIAN_POINT('Ctrl Pts',(-22.0023070600683,-13.3508620232142,
113.558369809098)) ;
#180316=CARTESIAN_POINT('Ctrl Pts',(-21.9285032156018,-13.3508620856039,
113.582600847596)) ;
#180317=CARTESIAN_POINT('Ctrl Pts',(-21.8546993711354,-13.3508621479936,
113.606831886095)) ;
#180318=CARTESIAN_POINT('Ctrl Pts',(-21.8310834005412,-13.3453694831773,
113.534901451295)) ;
#180319=CARTESIAN_POINT('Ctrl Pts',(-21.8074674299469,-13.3398768183609,
113.462971016496)) ;
#180320=CARTESIAN_POINT('Ctrl Pts',(-21.8812712744133,-13.3398767559712,
113.438739977997)) ;
#180321=CARTESIAN_POINT('Ctrl Pts',(-21.9550751188797,-13.3398766935815,
113.414508939498)) ;
#180322=CARTESIAN_POINT('Ctrl Pts',(-21.978691089474,-13.3453693583979,
113.486439374298)) ;
#180323=CARTESIAN_POINT('Ctrl Pts',(-21.9743140972656,-13.6361640667827,
113.508607131723)) ;
#180324=CARTESIAN_POINT('Ctrl Pts',(-21.9975369390037,-13.6213614987656,
113.57934015963)) ;
#180325=CARTESIAN_POINT('Ctrl Pts',(-21.9237330991818,-13.6213615511211,
113.603571212275)) ;
#180326=CARTESIAN_POINT('Ctrl Pts',(-21.84992925936,-13.6213616034766,113.62780226492)) ;
#180327=CARTESIAN_POINT('Ctrl Pts',(-21.8267064176218,-13.6361641714938,
113.557069237013)) ;
#180328=CARTESIAN_POINT('Ctrl Pts',(-21.8034835758837,-13.6509667395109,
113.486336209106)) ;
#180329=CARTESIAN_POINT('Ctrl Pts',(-21.8772874157056,-13.6509666871554,
113.462105156461)) ;
#180330=CARTESIAN_POINT('Ctrl Pts',(-21.9510912555274,-13.6509666347999,
113.437874103816)) ;
#180331=CARTESIAN_POINT('Ctrl Pts',(-21.9743140972656,-13.6361640667827,
113.508607131723)) ;
#180332=CARTESIAN_POINT('Ctrl Pts',(-21.9936997725589,-13.9104324089111,
113.603035067072)) ;
#180333=CARTESIAN_POINT('Ctrl Pts',(-22.0148720614655,-13.8764575771015,
113.667522442062)) ;
#180334=CARTESIAN_POINT('Ctrl Pts',(-21.9410682247111,-13.8764576175232,
113.69175350405)) ;
#180335=CARTESIAN_POINT('Ctrl Pts',(-21.8672643879568,-13.8764576579448,
113.715984566039)) ;
#180336=CARTESIAN_POINT('Ctrl Pts',(-21.8460920990502,-13.9104324897545,
113.651497191049)) ;
#180337=CARTESIAN_POINT('Ctrl Pts',(-21.8249198101436,-13.9444073215641,
113.587009816059)) ;
#180338=CARTESIAN_POINT('Ctrl Pts',(-21.8987236468979,-13.9444072811424,
113.56277875407)) ;
#180339=CARTESIAN_POINT('Ctrl Pts',(-21.9725274836523,-13.9444072407208,
113.538547692082)) ;
#180340=CARTESIAN_POINT('Ctrl Pts',(-21.9936997725589,-13.9104324089111,
113.603035067072)) ;
#180341=CARTESIAN_POINT('Ctrl Pts',(-22.0347431039267,-14.1501784561149,
113.763511943349)) ;
#180342=CARTESIAN_POINT('Ctrl Pts',(-22.0523478858651,-14.0994124816197,
113.817133267897)) ;
#180343=CARTESIAN_POINT('Ctrl Pts',(-21.9785440504179,-14.0994125084155,
113.841364333867)) ;
#180344=CARTESIAN_POINT('Ctrl Pts',(-21.9047402149707,-14.0994125352114,
113.865595399836)) ;
#180345=CARTESIAN_POINT('Ctrl Pts',(-21.8871354330323,-14.1501785097066,
113.811974075288)) ;
#180346=CARTESIAN_POINT('Ctrl Pts',(-21.8695306510939,-14.2009444842018,
113.75835275074)) ;
#180347=CARTESIAN_POINT('Ctrl Pts',(-21.9433344865411,-14.200944457406,
113.73412168477)) ;
#180348=CARTESIAN_POINT('Ctrl Pts',(-22.0171383219884,-14.2009444306102,
113.709890618801)) ;
#180349=CARTESIAN_POINT('Ctrl Pts',(-22.0347431039267,-14.1501784561149,
113.763511943349)) ;
#180350=CARTESIAN_POINT('Ctrl Pts',(-22.0939751521265,-14.3377944456025,
113.979478469494)) ;
#180351=CARTESIAN_POINT('Ctrl Pts',(-22.1067351330108,-14.273851283079,
114.018343311917)) ;
#180352=CARTESIAN_POINT('Ctrl Pts',(-22.0329312970307,-14.2738512972119,
114.042574376263)) ;
#180353=CARTESIAN_POINT('Ctrl Pts',(-21.9591274610505,-14.2738513113447,
114.06680544061)) ;
#180354=CARTESIAN_POINT('Ctrl Pts',(-21.9463674801662,-14.3377944738682,
114.027940598186)) ;
#180355=CARTESIAN_POINT('Ctrl Pts',(-21.9336074992819,-14.4017376363917,
113.989075755763)) ;
#180356=CARTESIAN_POINT('Ctrl Pts',(-22.0074113352621,-14.4017376222589,
113.964844691417)) ;
#180357=CARTESIAN_POINT('Ctrl Pts',(-22.0812151712422,-14.4017376081261,
113.94061362707)) ;
#180358=CARTESIAN_POINT('Ctrl Pts',(-22.0939751521265,-14.3377944456025,
113.979478469494)) ;
#180359=CARTESIAN_POINT('Ctrl Pts',(-22.1659929301065,-14.4588735568458,
114.234265903067)) ;
#180360=CARTESIAN_POINT('Ctrl Pts',(-22.1730103976931,-14.3863794182977,
114.255639976685)) ;
#180361=CARTESIAN_POINT('Ctrl Pts',(-22.0992065603188,-14.3863794234914,
114.279871036785)) ;
#180362=CARTESIAN_POINT('Ctrl Pts',(-22.0254027229444,-14.3863794286851,
114.304102096885)) ;
#180363=CARTESIAN_POINT('Ctrl Pts',(-22.0183852553577,-14.4588735672332,
114.282728023267)) ;
#180364=CARTESIAN_POINT('Ctrl Pts',(-22.011367787771,-14.5313677057812,
114.261353949649)) ;
#180365=CARTESIAN_POINT('Ctrl Pts',(-22.0851716251454,-14.5313677005875,
114.237122889549)) ;
#180366=CARTESIAN_POINT('Ctrl Pts',(-22.1589754625198,-14.5313676953939,
114.212891829449)) ;
#180367=CARTESIAN_POINT('Ctrl Pts',(-22.1659929301065,-14.4588735568458,
114.234265903067)) ;
#180368=CARTESIAN_POINT('Ctrl Pts',(-22.2451385688619,-14.5056122473976,
114.510797193633)) ;
#180369=CARTESIAN_POINT('Ctrl Pts',(-22.2459063570101,-14.4297450127553,
114.513135752203)) ;
#180370=CARTESIAN_POINT('Ctrl Pts',(-22.1721025175833,-14.4297450124761,
114.537366806052)) ;
#180371=CARTESIAN_POINT('Ctrl Pts',(-22.0982986781565,-14.4297450121969,
114.5615978599)) ;
#180372=CARTESIAN_POINT('Ctrl Pts',(-22.0975308900083,-14.5056122468393,
114.55925930133)) ;
#180373=CARTESIAN_POINT('Ctrl Pts',(-22.0967631018602,-14.5814794814817,
114.556920742759)) ;
#180374=CARTESIAN_POINT('Ctrl Pts',(-22.170566941287,-14.5814794817608,
114.532689688911)) ;
#180375=CARTESIAN_POINT('Ctrl Pts',(-22.2443707807138,-14.58147948204,114.508458635062)) ;
#180376=CARTESIAN_POINT('Ctrl Pts',(-22.2451385688619,-14.5056122473976,
114.510797193633)) ;
#180377=CARTESIAN_POINT('Ctrl Pts',(-22.324940686415,-14.4743736272664,
114.789329071983)) ;
#180378=CARTESIAN_POINT('Ctrl Pts',(-22.3194033900936,-14.4005733067483,
114.772463360702)) ;
#180379=CARTESIAN_POINT('Ctrl Pts',(-22.2455995486149,-14.4005733047048,
114.7966944083)) ;
#180380=CARTESIAN_POINT('Ctrl Pts',(-22.1717957071361,-14.4005733026613,
114.820925455899)) ;
#180381=CARTESIAN_POINT('Ctrl Pts',(-22.1773330034575,-14.4743736231794,
114.83779116718)) ;
#180382=CARTESIAN_POINT('Ctrl Pts',(-22.1828702997789,-14.5481739436975,
114.854656878461)) ;
#180383=CARTESIAN_POINT('Ctrl Pts',(-22.2566741412577,-14.548173945741,
114.830425830863)) ;
#180384=CARTESIAN_POINT('Ctrl Pts',(-22.3304779827364,-14.5481739477846,
114.806194783264)) ;
#180385=CARTESIAN_POINT('Ctrl Pts',(-22.324940686415,-14.4743736272664,
114.789329071983)) ;
#180386=CARTESIAN_POINT('Ctrl Pts',(-22.3988824387203,-14.3676054099568,
115.049984802301)) ;
#180387=CARTESIAN_POINT('Ctrl Pts',(-22.3874402811753,-14.3011495694392,
115.015133836573)) ;
#180388=CARTESIAN_POINT('Ctrl Pts',(-22.3136364381479,-14.3011495683314,
115.039364879455)) ;
#180389=CARTESIAN_POINT('Ctrl Pts',(-22.2398325951206,-14.3011495672236,
115.063595922336)) ;
#180390=CARTESIAN_POINT('Ctrl Pts',(-22.2512747526657,-14.3676054077411,
115.098446888065)) ;
#180391=CARTESIAN_POINT('Ctrl Pts',(-22.2627169102107,-14.4340612482587,
115.133297853793)) ;
#180392=CARTESIAN_POINT('Ctrl Pts',(-22.3365207532381,-14.4340612493665,
115.109066810911)) ;
#180393=CARTESIAN_POINT('Ctrl Pts',(-22.4103245962654,-14.4340612504743,
115.084835768029)) ;
#180394=CARTESIAN_POINT('Ctrl Pts',(-22.3988824387203,-14.3676054099568,
115.049984802301)) ;
#180395=CARTESIAN_POINT('Ctrl Pts',(-22.4609934584054,-14.1926642104704,
115.274637530722)) ;
#180396=CARTESIAN_POINT('Ctrl Pts',(-22.4444629941387,-14.1383247775165,
115.22428840378)) ;
#180397=CARTESIAN_POINT('Ctrl Pts',(-22.3706591502841,-14.1383247785838,
115.248519444142)) ;
#180398=CARTESIAN_POINT('Ctrl Pts',(-22.2968553064295,-14.1383247796511,
115.272750484504)) ;
#180399=CARTESIAN_POINT('Ctrl Pts',(-22.3133857706962,-14.192664212605,
115.323099611446)) ;
#180400=CARTESIAN_POINT('Ctrl Pts',(-22.3299162349628,-14.2470036455589,
115.373448738388)) ;
#180401=CARTESIAN_POINT('Ctrl Pts',(-22.4037200788174,-14.2470036444916,
115.349217698026)) ;
#180402=CARTESIAN_POINT('Ctrl Pts',(-22.477523922672,-14.2470036434243,
115.324986657664)) ;
#180403=CARTESIAN_POINT('Ctrl Pts',(-22.4609934584054,-14.1926642104704,
115.274637530722)) ;
#180404=CARTESIAN_POINT('Ctrl Pts',(-22.5060098471497,-13.9629645552833,
115.447132030502)) ;
#180405=CARTESIAN_POINT('Ctrl Pts',(-22.485579189812,-13.9245838600997,
115.384903544793)) ;
#180406=CARTESIAN_POINT('Ctrl Pts',(-22.411775345856,-13.9245838630912,
115.409134584846)) ;
#180407=CARTESIAN_POINT('Ctrl Pts',(-22.3379715019,-13.9245838660827,115.433365624899)) ;
#180408=CARTESIAN_POINT('Ctrl Pts',(-22.3584021592378,-13.9629645612662,
115.495594110609)) ;
#180409=CARTESIAN_POINT('Ctrl Pts',(-22.3788328165755,-14.0013452564497,
115.557822596318)) ;
#180410=CARTESIAN_POINT('Ctrl Pts',(-22.4526366605315,-14.0013452534583,
115.533591556265)) ;
#180411=CARTESIAN_POINT('Ctrl Pts',(-22.5264405044875,-14.0013452504668,
115.509360516212)) ;
#180412=CARTESIAN_POINT('Ctrl Pts',(-22.5060098471497,-13.9629645552833,
115.447132030502)) ;
#180413=CARTESIAN_POINT('Ctrl Pts',(-22.5301282053753,-13.6916669453695,
115.556308146258)) ;
#180414=CARTESIAN_POINT('Ctrl Pts',(-22.5072437313959,-13.6721744570857,
115.486605730959)) ;
#180415=CARTESIAN_POINT('Ctrl Pts',(-22.4334398878541,-13.6721744593942,
115.510836772273)) ;
#180416=CARTESIAN_POINT('Ctrl Pts',(-22.3596360443124,-13.6721744617026,
115.535067813588)) ;
#180417=CARTESIAN_POINT('Ctrl Pts',(-22.3825205182917,-13.6916669499864,
115.604770228888)) ;
#180418=CARTESIAN_POINT('Ctrl Pts',(-22.4054049922711,-13.7111594382702,
115.674472644188)) ;
#180419=CARTESIAN_POINT('Ctrl Pts',(-22.4792088358129,-13.7111594359618,
115.650241602873)) ;
#180420=CARTESIAN_POINT('Ctrl Pts',(-22.5530126793547,-13.7111594336534,
115.626010561558)) ;
#180421=CARTESIAN_POINT('Ctrl Pts',(-22.5301282053753,-13.6916669453695,
115.556308146258)) ;
#180422=CARTESIAN_POINT('Ctrl Pts',(-22.5305152960144,-13.4042886281479,
115.592739547311)) ;
#180423=CARTESIAN_POINT('Ctrl Pts',(-22.5068408787418,-13.4048339669214,
115.520631092151)) ;
#180424=CARTESIAN_POINT('Ctrl Pts',(-22.4330370354201,-13.4048339668837,
115.544862134136)) ;
#180425=CARTESIAN_POINT('Ctrl Pts',(-22.3592331920984,-13.404833966846,
115.569093176121)) ;
#180426=CARTESIAN_POINT('Ctrl Pts',(-22.382907609371,-13.4042886280725,
115.641201631281)) ;
#180427=CARTESIAN_POINT('Ctrl Pts',(-22.4065820266436,-13.403743289299,
115.713310086441)) ;
#180428=CARTESIAN_POINT('Ctrl Pts',(-22.4803858699653,-13.4037432893367,
115.689079044456)) ;
#180429=CARTESIAN_POINT('Ctrl Pts',(-22.554189713287,-13.4037432893744,
115.664848002471)) ;
#180430=CARTESIAN_POINT('Ctrl Pts',(-22.5305152960144,-13.4042886281479,
115.592739547311)) ;
#180431=CARTESIAN_POINT('Ctrl Pts',(-22.5067605017534,-13.1160881842174,
115.55586845108)) ;
#180432=CARTESIAN_POINT('Ctrl Pts',(-22.4839758365331,-13.1367582104912,
115.486470037027)) ;
#180433=CARTESIAN_POINT('Ctrl Pts',(-22.4101719928964,-13.1367582061789,
115.510701078053)) ;
#180434=CARTESIAN_POINT('Ctrl Pts',(-22.3363681492598,-13.1367582018666,
115.534932119079)) ;
#180435=CARTESIAN_POINT('Ctrl Pts',(-22.3591528144801,-13.1160881755929,
115.604330533131)) ;
#180436=CARTESIAN_POINT('Ctrl Pts',(-22.3819374797004,-13.0954181493191,
115.673728947184)) ;
#180437=CARTESIAN_POINT('Ctrl Pts',(-22.455741323337,-13.0954181536314,
115.649497906158)) ;
#180438=CARTESIAN_POINT('Ctrl Pts',(-22.5295451669737,-13.0954181579436,
115.625266865132)) ;
#180439=CARTESIAN_POINT('Ctrl Pts',(-22.5067605017534,-13.1160881842174,
115.55586845108)) ;
#180440=CARTESIAN_POINT('Ctrl Pts',(-22.4595154178549,-12.8495738757798,
115.447455103037)) ;
#180441=CARTESIAN_POINT('Ctrl Pts',(-22.4392620419425,-12.8888833461409,
115.385766587677)) ;
#180442=CARTESIAN_POINT('Ctrl Pts',(-22.365458196973,-12.8888833370438,
115.409997624643)) ;
#180443=CARTESIAN_POINT('Ctrl Pts',(-22.2916543520035,-12.8888833279467,
115.434228661609)) ;
#180444=CARTESIAN_POINT('Ctrl Pts',(-22.311907727916,-12.8495738575856,
115.495917176969)) ;
#180445=CARTESIAN_POINT('Ctrl Pts',(-22.3321611038284,-12.8102643872246,
115.557605692329)) ;
#180446=CARTESIAN_POINT('Ctrl Pts',(-22.4059649487979,-12.8102643963217,
115.533374655363)) ;
#180447=CARTESIAN_POINT('Ctrl Pts',(-22.4797687937674,-12.8102644054188,
115.509143618397)) ;
#180448=CARTESIAN_POINT('Ctrl Pts',(-22.4595154178549,-12.8495738757798,
115.447455103037)) ;
#180449=CARTESIAN_POINT('Ctrl Pts',(-22.3918481625051,-12.6242652876755,
115.276723191289)) ;
#180450=CARTESIAN_POINT('Ctrl Pts',(-22.3755581859856,-12.6793633695142,
115.22710655087)) ;
#180451=CARTESIAN_POINT('Ctrl Pts',(-22.3017543389936,-12.6793633576824,
115.251337581676)) ;
#180452=CARTESIAN_POINT('Ctrl Pts',(-22.2279504920016,-12.6793633458506,
115.275568612482)) ;
#180453=CARTESIAN_POINT('Ctrl Pts',(-22.244240468521,-12.6242652640119,
115.325185252901)) ;
#180454=CARTESIAN_POINT('Ctrl Pts',(-22.2605304450405,-12.5691671821732,
115.374801893319)) ;
#180455=CARTESIAN_POINT('Ctrl Pts',(-22.3343342920325,-12.569167194005,
115.350570862513)) ;
#180456=CARTESIAN_POINT('Ctrl Pts',(-22.4081381390246,-12.5691672058369,
115.326339831707)) ;
#180457=CARTESIAN_POINT('Ctrl Pts',(-22.3918481625051,-12.6242652876755,
115.276723191289)) ;
#180458=CARTESIAN_POINT('Ctrl Pts',(-22.3066463098264,-12.4543477917217,
115.052950743928)) ;
#180459=CARTESIAN_POINT('Ctrl Pts',(-22.2955420650032,-12.5213905408383,
115.019129005345)) ;
#180460=CARTESIAN_POINT('Ctrl Pts',(-22.2217382143452,-12.5213905278412,
115.043360024985)) ;
#180461=CARTESIAN_POINT('Ctrl Pts',(-22.1479343636872,-12.521390514844,
115.067591044625)) ;
#180462=CARTESIAN_POINT('Ctrl Pts',(-22.1590386085103,-12.4543477657274,
115.101412783208)) ;
#180463=CARTESIAN_POINT('Ctrl Pts',(-22.1701428533335,-12.3873050166108,
115.135234521791)) ;
#180464=CARTESIAN_POINT('Ctrl Pts',(-22.2439467039915,-12.387305029608,
115.111003502151)) ;
#180465=CARTESIAN_POINT('Ctrl Pts',(-22.3177505546495,-12.3873050426051,
115.086772482511)) ;
#180466=CARTESIAN_POINT('Ctrl Pts',(-22.3066463098264,-12.4543477917217,
115.052950743928)) ;
#180467=CARTESIAN_POINT('Ctrl Pts',(-22.2113534668614,-12.3553371823295,
114.797951573092)) ;
#180468=CARTESIAN_POINT('Ctrl Pts',(-22.2061572714321,-12.4293892510952,
114.78212479958)) ;
#180469=CARTESIAN_POINT('Ctrl Pts',(-22.1323534180165,-12.4293892433542,
114.806355810821)) ;
#180470=CARTESIAN_POINT('Ctrl Pts',(-22.058549564601,-12.4293892356132,
114.830586822062)) ;
#180471=CARTESIAN_POINT('Ctrl Pts',(-22.0637457600304,-12.3553371668475,
114.846413595574)) ;
#180472=CARTESIAN_POINT('Ctrl Pts',(-22.0689419554598,-12.2812850980819,
114.862240369086)) ;
#180473=CARTESIAN_POINT('Ctrl Pts',(-22.1427458088753,-12.2812851058229,
114.838009357845)) ;
#180474=CARTESIAN_POINT('Ctrl Pts',(-22.2165496622908,-12.2812851135639,
114.813778346604)) ;
#180475=CARTESIAN_POINT('Ctrl Pts',(-22.2113534668614,-12.3553371823295,
114.797951573092)) ;
#180476=CARTESIAN_POINT('Ctrl Pts',(-22.1099317335009,-12.3315537600446,
114.524642057895)) ;
#180477=CARTESIAN_POINT('Ctrl Pts',(-22.1110725413318,-12.4073738615737,
114.52811677365)) ;
#180478=CARTESIAN_POINT('Ctrl Pts',(-22.0372686845444,-12.4073738630853,
114.552347774621)) ;
#180479=CARTESIAN_POINT('Ctrl Pts',(-21.963464827757,-12.4073738645969,
114.576578775592)) ;
#180480=CARTESIAN_POINT('Ctrl Pts',(-21.9623240199261,-12.3315537630678,
114.573104059837)) ;
#180481=CARTESIAN_POINT('Ctrl Pts',(-21.9611832120952,-12.2557336615386,
114.569629344082)) ;
#180482=CARTESIAN_POINT('Ctrl Pts',(-22.0349870688826,-12.255733660027,
114.545398343111)) ;
#180483=CARTESIAN_POINT('Ctrl Pts',(-22.1087909256699,-12.2557336585155,
114.521167342141)) ;
#180484=CARTESIAN_POINT('Ctrl Pts',(-22.1099317335009,-12.3315537600446,
114.524642057895)) ;
#180485=CARTESIAN_POINT('Ctrl Pts',(-22.010593220664,-12.3856473127391,
114.257389293014)) ;
#180486=CARTESIAN_POINT('Ctrl Pts',(-22.0179406256113,-12.4577997306566,
114.279768302014)) ;
#180487=CARTESIAN_POINT('Ctrl Pts',(-21.9441367672794,-12.4577997458788,
114.30399929828)) ;
#180488=CARTESIAN_POINT('Ctrl Pts',(-21.8703329089475,-12.457799761101,
114.328230294547)) ;
#180489=CARTESIAN_POINT('Ctrl Pts',(-21.8629855040001,-12.3856473431835,
114.305851285547)) ;
#180490=CARTESIAN_POINT('Ctrl Pts',(-21.8556380990528,-12.3134949252661,
114.283472276546)) ;
#180491=CARTESIAN_POINT('Ctrl Pts',(-21.9294419573847,-12.3134949100439,
114.25924128028)) ;
#180492=CARTESIAN_POINT('Ctrl Pts',(-22.0032458157166,-12.3134948948217,
114.235010284013)) ;
#180493=CARTESIAN_POINT('Ctrl Pts',(-22.010593220664,-12.3856473127391,
114.257389293014)) ;
#180494=CARTESIAN_POINT('Ctrl Pts',(-21.9183564548921,-12.513656004823,
114.011961870334)) ;
#180495=CARTESIAN_POINT('Ctrl Pts',(-21.9314195210671,-12.5769754722421,
114.051749861039)) ;
#180496=CARTESIAN_POINT('Ctrl Pts',(-21.8576156621307,-12.5769755044901,
114.075980855464)) ;
#180497=CARTESIAN_POINT('Ctrl Pts',(-21.7838118031943,-12.576975536738,
114.10021184989)) ;
#180498=CARTESIAN_POINT('Ctrl Pts',(-21.7707487370193,-12.5136560693188,
114.060423859185)) ;
#180499=CARTESIAN_POINT('Ctrl Pts',(-21.7576856708444,-12.4503366018996,
114.02063586848)) ;
#180500=CARTESIAN_POINT('Ctrl Pts',(-21.8314895297808,-12.4503365696517,
113.996404874054)) ;
#180501=CARTESIAN_POINT('Ctrl Pts',(-21.9052933887172,-12.4503365374038,
113.972173879629)) ;
#180502=CARTESIAN_POINT('Ctrl Pts',(-21.9183564548921,-12.513656004823,
114.011961870334)) ;
#180503=CARTESIAN_POINT('Ctrl Pts',(-21.839571054505,-12.707439556573,113.807586885716)) ;
#180504=CARTESIAN_POINT('Ctrl Pts',(-21.8574172488463,-12.7573213774984,
113.861943512876)) ;
#180505=CARTESIAN_POINT('Ctrl Pts',(-21.7836133912687,-12.7573214291752,
113.88617451144)) ;
#180506=CARTESIAN_POINT('Ctrl Pts',(-21.709809533691,-12.7573214808521,
113.910405510004)) ;
#180507=CARTESIAN_POINT('Ctrl Pts',(-21.6919633393498,-12.7074396599266,
113.856048882843)) ;
#180508=CARTESIAN_POINT('Ctrl Pts',(-21.6741171450086,-12.6575578390012,
113.801692255683)) ;
#180509=CARTESIAN_POINT('Ctrl Pts',(-21.7479210025862,-12.6575577873243,
113.777461257119)) ;
#180510=CARTESIAN_POINT('Ctrl Pts',(-21.8217248601638,-12.6575577356475,
113.753230258555)) ;
#180511=CARTESIAN_POINT('Ctrl Pts',(-21.839571054505,-12.707439556573,113.807586885716)) ;
#180512=CARTESIAN_POINT('Ctrl Pts',(-21.7797609837458,-12.9500051005904,
113.660688819678)) ;
#180513=CARTESIAN_POINT('Ctrl Pts',(-21.8010788020931,-12.9830234168188,
113.725619453298)) ;
#180514=CARTESIAN_POINT('Ctrl Pts',(-21.7272749484766,-12.9830234842415,
113.749850463927)) ;
#180515=CARTESIAN_POINT('Ctrl Pts',(-21.65347109486,-12.9830235516642,113.774081474556)) ;
#180516=CARTESIAN_POINT('Ctrl Pts',(-21.6321532765127,-12.9500052354358,
113.709150840935)) ;
#180517=CARTESIAN_POINT('Ctrl Pts',(-21.6108354581654,-12.9169869192073,
113.644220207315)) ;
#180518=CARTESIAN_POINT('Ctrl Pts',(-21.6846393117819,-12.9169868517846,
113.619989196687)) ;
#180519=CARTESIAN_POINT('Ctrl Pts',(-21.7584431653985,-12.9169867843619,
113.595758186058)) ;
#180520=CARTESIAN_POINT('Ctrl Pts',(-21.7797609837458,-12.9500051005904,
113.660688819678)) ;
#180521=CARTESIAN_POINT('Ctrl Pts',(-21.741415490494,-13.2274462581565,
113.579389468672)) ;
#180522=CARTESIAN_POINT('Ctrl Pts',(-21.7647069644902,-13.2411424706592,
113.650331538803)) ;
#180523=CARTESIAN_POINT('Ctrl Pts',(-21.6909031163578,-13.2411425518727,
113.674562566135)) ;
#180524=CARTESIAN_POINT('Ctrl Pts',(-21.6170992682254,-13.2411426330862,
113.698793593467)) ;
#180525=CARTESIAN_POINT('Ctrl Pts',(-21.5938077942292,-13.2274464205834,
113.627851523337)) ;
#180526=CARTESIAN_POINT('Ctrl Pts',(-21.570516320233,-13.2137502080807,
113.556909453206)) ;
#180527=CARTESIAN_POINT('Ctrl Pts',(-21.6443201683654,-13.2137501268672,
113.532678425874)) ;
#180528=CARTESIAN_POINT('Ctrl Pts',(-21.7181240164978,-13.2137500456537,
113.508447398542)) ;
#180529=CARTESIAN_POINT('Ctrl Pts',(-21.741415490494,-13.2274462581565,
113.579389468672)) ;
#180530=CARTESIAN_POINT('Ctrl Pts',(-21.7271451352815,-13.5192262317475,
113.571491516801)) ;
#180531=CARTESIAN_POINT('Ctrl Pts',(-21.750730941216,-13.5125713400262,
113.643330074385)) ;
#180532=CARTESIAN_POINT('Ctrl Pts',(-21.6769271002671,-13.5125714295465,
113.667561123597)) ;
#180533=CARTESIAN_POINT('Ctrl Pts',(-21.6031232593182,-13.5125715190667,
113.691792172809)) ;
#180534=CARTESIAN_POINT('Ctrl Pts',(-21.5795374533838,-13.519226410788,
113.619953615225)) ;
#180535=CARTESIAN_POINT('Ctrl Pts',(-21.5559516474493,-13.5258813025093,
113.548115057642)) ;
#180536=CARTESIAN_POINT('Ctrl Pts',(-21.6297554883982,-13.525881212989,
113.523884008429)) ;
#180537=CARTESIAN_POINT('Ctrl Pts',(-21.7035593293471,-13.5258811234688,
113.499652959217)) ;
#180538=CARTESIAN_POINT('Ctrl Pts',(-21.7271451352815,-13.5192262317475,
113.571491516801)) ;
#180539=CARTESIAN_POINT('Ctrl Pts',(-21.7370271436767,-13.8018769048648,
113.636919707644)) ;
#180540=CARTESIAN_POINT('Ctrl Pts',(-21.7592262395528,-13.7754786172954,
113.704534570041)) ;
#180541=CARTESIAN_POINT('Ctrl Pts',(-21.6854224064523,-13.7754787060709,
113.728765643158)) ;
#180542=CARTESIAN_POINT('Ctrl Pts',(-21.6116185733517,-13.7754787948464,
113.752996716275)) ;
#180543=CARTESIAN_POINT('Ctrl Pts',(-21.5894194774756,-13.8018770824157,
113.685381853878)) ;
#180544=CARTESIAN_POINT('Ctrl Pts',(-21.5672203815995,-13.8282753699851,
113.617766991481)) ;
#180545=CARTESIAN_POINT('Ctrl Pts',(-21.6410242147001,-13.8282752812096,
113.593535918364)) ;
#180546=CARTESIAN_POINT('Ctrl Pts',(-21.7148280478006,-13.8282751924341,
113.569304845247)) ;
#180547=CARTESIAN_POINT('Ctrl Pts',(-21.7370271436767,-13.8018769048648,
113.636919707644)) ;
#180548=CARTESIAN_POINT('Ctrl Pts',(-21.7697376558309,-14.058784271986,
113.772109441117)) ;
#180549=CARTESIAN_POINT('Ctrl Pts',(-21.7889497969748,-14.0144111213973,
113.830626521239)) ;
#180550=CARTESIAN_POINT('Ctrl Pts',(-21.7151459718567,-14.0144112025132,
113.854857618669)) ;
#180551=CARTESIAN_POINT('Ctrl Pts',(-21.6413421467386,-14.014411283629,
113.879088716099)) ;
#180552=CARTESIAN_POINT('Ctrl Pts',(-21.6221300055947,-14.0587844342176,
113.820571635977)) ;
#180553=CARTESIAN_POINT('Ctrl Pts',(-21.6029178644509,-14.1031575848063,
113.762054555855)) ;
#180554=CARTESIAN_POINT('Ctrl Pts',(-21.676721689569,-14.1031575036904,
113.737823458425)) ;
#180555=CARTESIAN_POINT('Ctrl Pts',(-21.7505255146871,-14.1031574225746,
113.713592360994)) ;
#180556=CARTESIAN_POINT('Ctrl Pts',(-21.7697376558309,-14.058784271986,
113.772109441117)) ;
#180557=CARTESIAN_POINT('Ctrl Pts',(-21.8220819037483,-14.2690401451517,
113.967006518844)) ;
#180558=CARTESIAN_POINT('Ctrl Pts',(-21.8369339115327,-14.2099227100526,
114.012243336187)) ;
#180559=CARTESIAN_POINT('Ctrl Pts',(-21.7631300934121,-14.2099227749143,
114.03647445493)) ;
#180560=CARTESIAN_POINT('Ctrl Pts',(-21.6893262752916,-14.209922839776,
114.060705573674)) ;
#180561=CARTESIAN_POINT('Ctrl Pts',(-21.6744742675071,-14.2690402748751,
114.015468756331)) ;
#180562=CARTESIAN_POINT('Ctrl Pts',(-21.6596222597227,-14.3281577099741,
113.970231938989)) ;
#180563=CARTESIAN_POINT('Ctrl Pts',(-21.7334260778433,-14.3281576451124,
113.946000820246)) ;
#180564=CARTESIAN_POINT('Ctrl Pts',(-21.8072298959639,-14.3281575802507,
113.921769701502)) ;
#180565=CARTESIAN_POINT('Ctrl Pts',(-21.8220819037483,-14.2690401451517,
113.967006518844)) ;
#180566=CARTESIAN_POINT('Ctrl Pts',(-21.8895943124559,-14.418345814643,
114.208124022186)) ;
#180567=CARTESIAN_POINT('Ctrl Pts',(-21.8990204669094,-14.3487174926443,
114.236834565689)) ;
#180568=CARTESIAN_POINT('Ctrl Pts',(-21.8252166540276,-14.3487175346435,
114.261065700389)) ;
#180569=CARTESIAN_POINT('Ctrl Pts',(-21.7514128411458,-14.3487175766427,
114.285296835089)) ;
#180570=CARTESIAN_POINT('Ctrl Pts',(-21.7419866866923,-14.4183458986414,
114.256586291586)) ;
#180571=CARTESIAN_POINT('Ctrl Pts',(-21.7325605322388,-14.48797422064,114.227875748084)) ;
#180572=CARTESIAN_POINT('Ctrl Pts',(-21.8063643451206,-14.4879741786408,
114.203644613384)) ;
#180573=CARTESIAN_POINT('Ctrl Pts',(-21.8801681580024,-14.4879741366417,
114.179413478684)) ;
#180574=CARTESIAN_POINT('Ctrl Pts',(-21.8895943124559,-14.418345814643,
114.208124022186)) ;
#180575=CARTESIAN_POINT('Ctrl Pts',(-21.966477791396,-14.4960013207205,
114.477695371654)) ;
#180576=CARTESIAN_POINT('Ctrl Pts',(-21.9698176997642,-14.4208489309484,
114.487868191563)) ;
#180577=CARTESIAN_POINT('Ctrl Pts',(-21.8960138897414,-14.4208489456351,
114.512099334971)) ;
#180578=CARTESIAN_POINT('Ctrl Pts',(-21.8222100797186,-14.4208489603219,
114.536330478379)) ;
#180579=CARTESIAN_POINT('Ctrl Pts',(-21.8188701713504,-14.496001350094,
114.52615765847)) ;
#180580=CARTESIAN_POINT('Ctrl Pts',(-21.8155302629822,-14.5711537398661,
114.51598483856)) ;
#180581=CARTESIAN_POINT('Ctrl Pts',(-21.889334073005,-14.5711537251794,
114.491753695152)) ;
#180582=CARTESIAN_POINT('Ctrl Pts',(-21.9631378830277,-14.5711537104926,
114.467522551744)) ;
#180583=CARTESIAN_POINT('Ctrl Pts',(-21.966477791396,-14.4960013207205,
114.477695371654)) ;
#180584=CARTESIAN_POINT('Ctrl Pts',(-22.0471672488081,-14.4962457299704,
114.759096539096)) ;
#180585=CARTESIAN_POINT('Ctrl Pts',(-22.0441414094765,-14.4209645456079,
114.749880318615)) ;
#180586=CARTESIAN_POINT('Ctrl Pts',(-21.9703375995745,-14.4209645311187,
114.774111462391)) ;
#180587=CARTESIAN_POINT('Ctrl Pts',(-21.8965337896726,-14.4209645166296,
114.798342606167)) ;
#180588=CARTESIAN_POINT('Ctrl Pts',(-21.8995596290041,-14.4962457009921,
114.807558826648)) ;
#180589=CARTESIAN_POINT('Ctrl Pts',(-21.9025854683358,-14.5715268853546,
114.81677504713)) ;
#180590=CARTESIAN_POINT('Ctrl Pts',(-21.9763892782377,-14.5715268998438,
114.792543903354)) ;
#180591=CARTESIAN_POINT('Ctrl Pts',(-22.0501930881397,-14.5715269143329,
114.768312759578)) ;
#180592=CARTESIAN_POINT('Ctrl Pts',(-22.0471672488081,-14.4962457299704,
114.759096539096)) ;
#180593=CARTESIAN_POINT('Ctrl Pts',(-22.1237856140213,-14.4198799151553,
115.027702043525)) ;
#180594=CARTESIAN_POINT('Ctrl Pts',(-22.1146768854847,-14.3498193552219,
114.999958324006)) ;
#180595=CARTESIAN_POINT('Ctrl Pts',(-22.0408730730278,-14.3498193130492,
115.02418946)) ;
#180596=CARTESIAN_POINT('Ctrl Pts',(-21.967069260571,-14.3498192708765,
115.048420595995)) ;
#180597=CARTESIAN_POINT('Ctrl Pts',(-21.9761779891077,-14.4198798308098,
115.076164315514)) ;
#180598=CARTESIAN_POINT('Ctrl Pts',(-21.9852867176444,-14.4899403907432,
115.103908035032)) ;
#180599=CARTESIAN_POINT('Ctrl Pts',(-22.0590905301012,-14.4899404329159,
115.079676899038)) ;
#180600=CARTESIAN_POINT('Ctrl Pts',(-22.132894342558,-14.4899404750886,
115.055445763043)) ;
#180601=CARTESIAN_POINT('Ctrl Pts',(-22.1237856140213,-14.4198799151553,
115.027702043525)) ;
#180602=CARTESIAN_POINT('Ctrl Pts',(-22.1916978524243,-14.2709014086462,
115.270163302908)) ;
#180603=CARTESIAN_POINT('Ctrl Pts',(-22.1770973048726,-14.2111372247694,
115.225692388811)) ;
#180604=CARTESIAN_POINT('Ctrl Pts',(-22.1032934872705,-14.2111371588843,
115.249923509134)) ;
#180605=CARTESIAN_POINT('Ctrl Pts',(-22.0294896696684,-14.2111370929992,
115.274154629457)) ;
#180606=CARTESIAN_POINT('Ctrl Pts',(-22.0440902172201,-14.270901276876,
115.318625543554)) ;
#180607=CARTESIAN_POINT('Ctrl Pts',(-22.0586907647718,-14.3306654607528,
115.36309645765)) ;
#180608=CARTESIAN_POINT('Ctrl Pts',(-22.1324945823739,-14.3306655266379,
115.338865337328)) ;
#180609=CARTESIAN_POINT('Ctrl Pts',(-22.206298399976,-14.330665592523,115.314634217005)) ;
#180610=CARTESIAN_POINT('Ctrl Pts',(-22.1916978524243,-14.2709014086462,
115.270163302908)) ;
#180611=CARTESIAN_POINT('Ctrl Pts',(-22.244095479827,-14.0614284920593,
115.465166551261)) ;
#180612=CARTESIAN_POINT('Ctrl Pts',(-22.2250822225662,-14.016200017183,
115.407255235435)) ;
#180613=CARTESIAN_POINT('Ctrl Pts',(-22.1512783980525,-14.01619993407,115.431486334706)) ;
#180614=CARTESIAN_POINT('Ctrl Pts',(-22.0774745735387,-14.016199850957,
115.455717433977)) ;
#180615=CARTESIAN_POINT('Ctrl Pts',(-22.0964878307995,-14.0614283258333,
115.513628749803)) ;
#180616=CARTESIAN_POINT('Ctrl Pts',(-22.1155010880602,-14.1066568007097,
115.571540065629)) ;
#180617=CARTESIAN_POINT('Ctrl Pts',(-22.189304912574,-14.1066568838226,
115.547308966358)) ;
#180618=CARTESIAN_POINT('Ctrl Pts',(-22.2631087370878,-14.1066569669356,
115.523077867087)) ;
#180619=CARTESIAN_POINT('Ctrl Pts',(-22.244095479827,-14.0614284920593,
115.465166551261)) ;
#180620=CARTESIAN_POINT('Ctrl Pts',(-22.2770600984898,-13.8059370930909,
115.601015529285)) ;
#180621=CARTESIAN_POINT('Ctrl Pts',(-22.2549834954965,-13.778478597832,
115.5337737567)) ;
#180622=CARTESIAN_POINT('Ctrl Pts',(-22.1811796629507,-13.7784785051367,
115.558004831507)) ;
#180623=CARTESIAN_POINT('Ctrl Pts',(-22.1073758304049,-13.7784784124414,
115.582235906314)) ;
#180624=CARTESIAN_POINT('Ctrl Pts',(-22.1294524333982,-13.8059369077003,
115.649477678899)) ;
#180625=CARTESIAN_POINT('Ctrl Pts',(-22.1515290363916,-13.8333954029592,
115.716719451483)) ;
#180626=CARTESIAN_POINT('Ctrl Pts',(-22.2253328689374,-13.8333954956545,
115.692488376677)) ;
#180627=CARTESIAN_POINT('Ctrl Pts',(-22.2991367014832,-13.8333955883498,
115.66825730187)) ;
#180628=CARTESIAN_POINT('Ctrl Pts',(-22.2770600984898,-13.8059370930909,
115.601015529285)) ;
#180629=CARTESIAN_POINT('Ctrl Pts',(-22.2872367367097,-13.5211628984478,
115.667631143365)) ;
#180630=CARTESIAN_POINT('Ctrl Pts',(-22.2636792886074,-13.5135452087457,
115.595878955628)) ;
#180631=CARTESIAN_POINT('Ctrl Pts',(-22.1898754477952,-13.5135451161284,
115.620110005257)) ;
#180632=CARTESIAN_POINT('Ctrl Pts',(-22.116071606983,-13.513545023511,115.644341054886)) ;
#180633=CARTESIAN_POINT('Ctrl Pts',(-22.1396290550854,-13.5211627132132,
115.716093242622)) ;
#180634=CARTESIAN_POINT('Ctrl Pts',(-22.1631865031877,-13.5287804029153,
115.787845430359)) ;
#180635=CARTESIAN_POINT('Ctrl Pts',(-22.2369903439999,-13.5287804955326,
115.76361438073)) ;
#180636=CARTESIAN_POINT('Ctrl Pts',(-22.3107941848121,-13.52878058815,115.739383331101)) ;
#180637=CARTESIAN_POINT('Ctrl Pts',(-22.2872367367097,-13.5211628984478,
115.667631143365)) ;
#180638=CARTESIAN_POINT('Ctrl Pts',(-22.2733014770103,-13.2317212421624,
115.660460390471)) ;
#180639=CARTESIAN_POINT('Ctrl Pts',(-22.2499517872738,-13.244300576159,
115.589341001286)) ;
#180640=CARTESIAN_POINT('Ctrl Pts',(-22.1761479389709,-13.2443004892996,
115.613572028099)) ;
#180641=CARTESIAN_POINT('Ctrl Pts',(-22.102344090668,-13.2443004024403,
115.637803054912)) ;
#180642=CARTESIAN_POINT('Ctrl Pts',(-22.1256937804045,-13.2317210684437,
115.708922444097)) ;
#180643=CARTESIAN_POINT('Ctrl Pts',(-22.1490434701409,-13.2191417344471,
115.780041833282)) ;
#180644=CARTESIAN_POINT('Ctrl Pts',(-22.2228473184438,-13.2191418213064,
115.755810806469)) ;
#180645=CARTESIAN_POINT('Ctrl Pts',(-22.2966511667467,-13.2191419081658,
115.731579779656)) ;
#180646=CARTESIAN_POINT('Ctrl Pts',(-22.2733014770103,-13.2317212421624,
115.660460390471)) ;
#180647=CARTESIAN_POINT('Ctrl Pts',(-22.2352493339622,-12.953209842425,
115.580148172852)) ;
#180648=CARTESIAN_POINT('Ctrl Pts',(-22.2137846357895,-12.9852534588735,
115.514770163977)) ;
#180649=CARTESIAN_POINT('Ctrl Pts',(-22.1399807814508,-12.9852533862488,
115.539001172406)) ;
#180650=CARTESIAN_POINT('Ctrl Pts',(-22.0661769271121,-12.9852533136241,
115.563232180835)) ;
#180651=CARTESIAN_POINT('Ctrl Pts',(-22.0876416252848,-12.9532096971755,
115.62861018971)) ;
#180652=CARTESIAN_POINT('Ctrl Pts',(-22.1091063234574,-12.921166080727,
115.693988198586)) ;
#180653=CARTESIAN_POINT('Ctrl Pts',(-22.1829101777961,-12.9211661533517,
115.669757190157)) ;
#180654=CARTESIAN_POINT('Ctrl Pts',(-22.2567140321349,-12.9211662259765,
115.645526181728)) ;
#180655=CARTESIAN_POINT('Ctrl Pts',(-22.2352493339622,-12.953209842425,
115.580148172852)) ;
#180656=CARTESIAN_POINT('Ctrl Pts',(-22.1754856836276,-12.7094642616823,
115.433485637688)) ;
#180657=CARTESIAN_POINT('Ctrl Pts',(-22.1574294209425,-12.7585743721417,
115.378489173487)) ;
#180658=CARTESIAN_POINT('Ctrl Pts',(-22.0836255623272,-12.7585743165694,
115.402720168891)) ;
#180659=CARTESIAN_POINT('Ctrl Pts',(-22.009821703712,-12.7585742609971,
115.426951164294)) ;
#180660=CARTESIAN_POINT('Ctrl Pts',(-22.027877966397,-12.7094641505378,
115.481947628495)) ;
#180661=CARTESIAN_POINT('Ctrl Pts',(-22.0459342290821,-12.6603540400784,
115.536944092696)) ;
#180662=CARTESIAN_POINT('Ctrl Pts',(-22.1197380876974,-12.6603540956507,
115.512713097292)) ;
#180663=CARTESIAN_POINT('Ctrl Pts',(-22.1935419463127,-12.660354151223,
115.488482101889)) ;
#180664=CARTESIAN_POINT('Ctrl Pts',(-22.1754856836276,-12.7094642616823,
115.433485637688)) ;
#180665=CARTESIAN_POINT('Ctrl Pts',(-22.0966448910796,-12.5150572905195,
115.22901210739)) ;
#180666=CARTESIAN_POINT('Ctrl Pts',(-22.0833278506864,-12.5778156836835,
115.18845054981)) ;
#180667=CARTESIAN_POINT('Ctrl Pts',(-22.0095239905601,-12.5778156484991,
115.212681540611)) ;
#180668=CARTESIAN_POINT('Ctrl Pts',(-21.9357201304339,-12.5778156133148,
115.236912531413)) ;
#180669=CARTESIAN_POINT('Ctrl Pts',(-21.9490371708272,-12.5150572201508,
115.277474088992)) ;
#180670=CARTESIAN_POINT('Ctrl Pts',(-21.9623542112205,-12.4522988269869,
115.318035646572)) ;
#180671=CARTESIAN_POINT('Ctrl Pts',(-22.0361580713467,-12.4522988621712,
115.293804655771)) ;
#180672=CARTESIAN_POINT('Ctrl Pts',(-22.1099619314729,-12.4522988973556,
115.269573664969)) ;
#180673=CARTESIAN_POINT('Ctrl Pts',(-22.0966448910796,-12.5150572905195,
115.22901210739)) ;
#180674=CARTESIAN_POINT('Ctrl Pts',(-22.0054187277231,-12.3871819681861,
114.986327553014)) ;
#180675=CARTESIAN_POINT('Ctrl Pts',(-21.997723242732,-12.4589631112732,
114.962888346264)) ;
#180676=CARTESIAN_POINT('Ctrl Pts',(-21.9239193820062,-12.4589630933021,
114.987119335239)) ;
#180677=CARTESIAN_POINT('Ctrl Pts',(-21.8501155212804,-12.458963075331,
115.011350324214)) ;
#180678=CARTESIAN_POINT('Ctrl Pts',(-21.8578110062715,-12.3871819322439,
115.034789530964)) ;
#180679=CARTESIAN_POINT('Ctrl Pts',(-21.8655064912626,-12.3154007891568,
115.058228737713)) ;
#180680=CARTESIAN_POINT('Ctrl Pts',(-21.9393103519884,-12.3154008071279,
115.033997748738)) ;
#180681=CARTESIAN_POINT('Ctrl Pts',(-22.0131142127142,-12.315400825099,
115.009766759763)) ;
#180682=CARTESIAN_POINT('Ctrl Pts',(-22.0054187277231,-12.3871819681861,
114.986327553014)) ;
#180683=CARTESIAN_POINT('Ctrl Pts',(-21.905263733452,-12.3316884564228,
114.716909806915)) ;
#180684=CARTESIAN_POINT('Ctrl Pts',(-21.9038120156515,-12.4074536121107,
114.7124881078)) ;
#180685=CARTESIAN_POINT('Ctrl Pts',(-21.8300081572495,-12.4074536102533,
114.736719103853)) ;
#180686=CARTESIAN_POINT('Ctrl Pts',(-21.7562042988474,-12.407453608396,
114.760950099906)) ;
#180687=CARTESIAN_POINT('Ctrl Pts',(-21.7576560166478,-12.3316884527082,
114.765371799021)) ;
#180688=CARTESIAN_POINT('Ctrl Pts',(-21.7591077344482,-12.2559232970203,
114.769793498135)) ;
#180689=CARTESIAN_POINT('Ctrl Pts',(-21.8329115928503,-12.2559232988777,
114.745562502083)) ;
#180690=CARTESIAN_POINT('Ctrl Pts',(-21.9067154512524,-12.255923300735,
114.72133150603)) ;
#180691=CARTESIAN_POINT('Ctrl Pts',(-21.905263733452,-12.3316884564228,
114.716909806915)) ;
#180692=CARTESIAN_POINT('Ctrl Pts',(-21.8045903005962,-12.3542922095437,
114.445593550072)) ;
#180693=CARTESIAN_POINT('Ctrl Pts',(-21.809434740059,-12.4285936621951,
114.46034893024)) ;
#180694=CARTESIAN_POINT('Ctrl Pts',(-21.7356308842862,-12.428593671534,
114.484579934302)) ;
#180695=CARTESIAN_POINT('Ctrl Pts',(-21.6618270285135,-12.428593680873,
114.508810938363)) ;
#180696=CARTESIAN_POINT('Ctrl Pts',(-21.6569825890507,-12.3542922282216,
114.494055558194)) ;
#180697=CARTESIAN_POINT('Ctrl Pts',(-21.6521381495879,-12.2799907755701,
114.479300178026)) ;
#180698=CARTESIAN_POINT('Ctrl Pts',(-21.7259420053606,-12.2799907662312,
114.455069173964)) ;
#180699=CARTESIAN_POINT('Ctrl Pts',(-21.7997458611334,-12.2799907568923,
114.430838169903)) ;
#180700=CARTESIAN_POINT('Ctrl Pts',(-21.8045903005962,-12.3542922095437,
114.445593550072)) ;
#180701=CARTESIAN_POINT('Ctrl Pts',(-21.7081146500002,-12.4537268763868,
114.187411168182)) ;
#180702=CARTESIAN_POINT('Ctrl Pts',(-21.7189646587714,-12.5211987643482,
114.220458543672)) ;
#180703=CARTESIAN_POINT('Ctrl Pts',(-21.6451608071161,-12.5211987790939,
114.244689560275)) ;
#180704=CARTESIAN_POINT('Ctrl Pts',(-21.5713569554607,-12.5211987938395,
114.268920576877)) ;
#180705=CARTESIAN_POINT('Ctrl Pts',(-21.5605069466895,-12.4537269058781,
114.235873201386)) ;
#180706=CARTESIAN_POINT('Ctrl Pts',(-21.5496569379183,-12.3862550179166,
114.202825825896)) ;
#180707=CARTESIAN_POINT('Ctrl Pts',(-21.6234607895737,-12.386255003171,
114.178594809294)) ;
#180708=CARTESIAN_POINT('Ctrl Pts',(-21.697264641229,-12.3862549884253,
114.154363792692)) ;
#180709=CARTESIAN_POINT('Ctrl Pts',(-21.7081146500002,-12.4537268763868,
114.187411168182)) ;
#180710=CARTESIAN_POINT('Ctrl Pts',(-21.6237862011861,-12.6212675456056,
113.965882774821)) ;
#180711=CARTESIAN_POINT('Ctrl Pts',(-21.6398097461159,-12.6771429779521,
114.014687906835)) ;
#180712=CARTESIAN_POINT('Ctrl Pts',(-21.5660058974906,-12.6771429943205,
114.038918932666)) ;
#180713=CARTESIAN_POINT('Ctrl Pts',(-21.4922020488653,-12.6771430106889,
114.063149958497)) ;
#180714=CARTESIAN_POINT('Ctrl Pts',(-21.4761785039354,-12.6212675783423,
114.014344826483)) ;
#180715=CARTESIAN_POINT('Ctrl Pts',(-21.4601549590056,-12.5653921459958,
113.965539694469)) ;
#180716=CARTESIAN_POINT('Ctrl Pts',(-21.5339588076309,-12.5653921296274,
113.941308668638)) ;
#180717=CARTESIAN_POINT('Ctrl Pts',(-21.6077626562563,-12.565392113259,
113.917077642806)) ;
#180718=CARTESIAN_POINT('Ctrl Pts',(-21.6237862011861,-12.6212675456056,
113.965882774821)) ;
#180719=CARTESIAN_POINT('Ctrl Pts',(-21.5556046478956,-12.846192059173,
113.793679096726)) ;
#180720=CARTESIAN_POINT('Ctrl Pts',(-21.5756792298815,-12.8864467914097,
113.854823034128)) ;
#180721=CARTESIAN_POINT('Ctrl Pts',(-21.5018753840635,-12.8864468052169,
113.87905406851)) ;
#180722=CARTESIAN_POINT('Ctrl Pts',(-21.4280715382456,-12.8864468190241,
113.903285102892)) ;
#180723=CARTESIAN_POINT('Ctrl Pts',(-21.4079969562597,-12.8461920867874,
113.84214116549)) ;
#180724=CARTESIAN_POINT('Ctrl Pts',(-21.3879223742738,-12.8059373545508,
113.780997228088)) ;
#180725=CARTESIAN_POINT('Ctrl Pts',(-21.4617262200917,-12.8059373407436,
113.756766193706)) ;
#180726=CARTESIAN_POINT('Ctrl Pts',(-21.5355300659097,-12.8059373269364,
113.732535159324)) ;
#180727=CARTESIAN_POINT('Ctrl Pts',(-21.5556046478956,-12.846192059173,
113.793679096726)) ;
#180728=CARTESIAN_POINT('Ctrl Pts',(-21.5080827888729,-13.1124184461725,
113.684427311798)) ;
#180729=CARTESIAN_POINT('Ctrl Pts',(-21.5307714606436,-13.1341445509028,
113.753533345037)) ;
#180730=CARTESIAN_POINT('Ctrl Pts',(-21.4569676166366,-13.1341445595333,
113.777764384935)) ;
#180731=CARTESIAN_POINT('Ctrl Pts',(-21.3831637726296,-13.1341445681639,
113.801995424833)) ;
#180732=CARTESIAN_POINT('Ctrl Pts',(-21.3604751008589,-13.1124184634336,
113.732889391594)) ;
#180733=CARTESIAN_POINT('Ctrl Pts',(-21.3377864290883,-13.0906923587033,
113.663783358355)) ;
#180734=CARTESIAN_POINT('Ctrl Pts',(-21.4115902730953,-13.0906923500727,
113.639552318457)) ;
#180735=CARTESIAN_POINT('Ctrl Pts',(-21.4853941171023,-13.0906923414422,
113.615321278559)) ;
#180736=CARTESIAN_POINT('Ctrl Pts',(-21.5080827888729,-13.1124184461725,
113.684427311798)) ;
#180737=CARTESIAN_POINT('Ctrl Pts',(-21.483971454148,-13.400879749144,113.646523677771)) ;
#180738=CARTESIAN_POINT('Ctrl Pts',(-21.5076425326459,-13.4024961126535,
113.718621963503)) ;
#180739=CARTESIAN_POINT('Ctrl Pts',(-21.4338386893524,-13.4024961156936,
113.742853005574)) ;
#180740=CARTESIAN_POINT('Ctrl Pts',(-21.360034846059,-13.4024961187337,
113.767084047645)) ;
#180741=CARTESIAN_POINT('Ctrl Pts',(-21.3363637675611,-13.4008797552242,
113.694985761914)) ;
#180742=CARTESIAN_POINT('Ctrl Pts',(-21.3126926890632,-13.3992633917147,
113.622887476182)) ;
#180743=CARTESIAN_POINT('Ctrl Pts',(-21.3864965323567,-13.3992633886746,
113.598656434111)) ;
#180744=CARTESIAN_POINT('Ctrl Pts',(-21.4603003756501,-13.3992633856344,
113.57442539204)) ;
#180745=CARTESIAN_POINT('Ctrl Pts',(-21.483971454148,-13.400879749144,113.646523677771)) ;
#180746=CARTESIAN_POINT('Ctrl Pts',(-21.4841119720974,-13.6891262166377,
113.682294540054)) ;
#180747=CARTESIAN_POINT('Ctrl Pts',(-21.5070772034444,-13.6706178186388,
113.752242929323)) ;
#180748=CARTESIAN_POINT('Ctrl Pts',(-21.4332733600708,-13.6706178179427,
113.77647397115)) ;
#180749=CARTESIAN_POINT('Ctrl Pts',(-21.3594695166973,-13.6706178172465,
113.800705012978)) ;
#180750=CARTESIAN_POINT('Ctrl Pts',(-21.3365042853503,-13.6891262152454,
113.730756623709)) ;
#180751=CARTESIAN_POINT('Ctrl Pts',(-21.3135390540032,-13.7076346132443,
113.66080823444)) ;
#180752=CARTESIAN_POINT('Ctrl Pts',(-21.3873428973768,-13.7076346139405,
113.636577192613)) ;
#180753=CARTESIAN_POINT('Ctrl Pts',(-21.4611467407504,-13.7076346146366,
113.612346150785)) ;
#180754=CARTESIAN_POINT('Ctrl Pts',(-21.4841119720974,-13.6891262166377,
113.682294540054)) ;
#180755=CARTESIAN_POINT('Ctrl Pts',(-21.5080695511385,-13.9605413879786,
113.790974309993)) ;
#180756=CARTESIAN_POINT('Ctrl Pts',(-21.5286572198407,-13.9230519796462,
113.853681027115)) ;
#180757=CARTESIAN_POINT('Ctrl Pts',(-21.4548533759605,-13.9230519767635,
113.877912067399)) ;
#180758=CARTESIAN_POINT('Ctrl Pts',(-21.3810495320804,-13.9230519738809,
113.902143107683)) ;
#180759=CARTESIAN_POINT('Ctrl Pts',(-21.3604618633781,-13.9605413822133,
113.839436390562)) ;
#180760=CARTESIAN_POINT('Ctrl Pts',(-21.3398741946759,-13.9980307905457,
113.77672967344)) ;
#180761=CARTESIAN_POINT('Ctrl Pts',(-21.413678038556,-13.9980307934284,
113.752498633156)) ;
#180762=CARTESIAN_POINT('Ctrl Pts',(-21.4874818824362,-13.9980307963111,
113.728267592871)) ;
#180763=CARTESIAN_POINT('Ctrl Pts',(-21.5080695511385,-13.9605413879786,
113.790974309993)) ;
#180764=CARTESIAN_POINT('Ctrl Pts',(-21.5525393505442,-14.1894540736428,
113.961580396736)) ;
#180765=CARTESIAN_POINT('Ctrl Pts',(-21.569324495808,-14.1359254038344,
114.012705240998)) ;
#180766=CARTESIAN_POINT('Ctrl Pts',(-21.4955206516589,-14.1359254016367,
114.036936280463)) ;
#180767=CARTESIAN_POINT('Ctrl Pts',(-21.4217168075098,-14.135925399439,
114.061167319929)) ;
#180768=CARTESIAN_POINT('Ctrl Pts',(-21.404931662246,-14.1894540692474,
114.010042475666)) ;
#180769=CARTESIAN_POINT('Ctrl Pts',(-21.3881465169822,-14.2429827390558,
113.958917631403)) ;
#180770=CARTESIAN_POINT('Ctrl Pts',(-21.4619503611313,-14.2429827412535,
113.934686591938)) ;
#180771=CARTESIAN_POINT('Ctrl Pts',(-21.5357542052804,-14.2429827434512,
113.910455552473)) ;
#180772=CARTESIAN_POINT('Ctrl Pts',(-21.5525393505442,-14.1894540736428,
113.961580396736)) ;
#180773=CARTESIAN_POINT('Ctrl Pts',(-21.6146814088062,-14.3660067048925,
114.186472926776)) ;
#180774=CARTESIAN_POINT('Ctrl Pts',(-21.6264149208127,-14.3000702425711,
114.222211311175)) ;
#180775=CARTESIAN_POINT('Ctrl Pts',(-21.5526110770569,-14.3000702422313,
114.246442351837)) ;
#180776=CARTESIAN_POINT('Ctrl Pts',(-21.478807233301,-14.3000702418915,
114.2706733925)) ;
#180777=CARTESIAN_POINT('Ctrl Pts',(-21.4670737212945,-14.3660067042129,
114.234935008102)) ;
#180778=CARTESIAN_POINT('Ctrl Pts',(-21.4553402092879,-14.4319431665342,
114.199196623703)) ;
#180779=CARTESIAN_POINT('Ctrl Pts',(-21.5291440530438,-14.431943166874,
114.174965583041)) ;
#180780=CARTESIAN_POINT('Ctrl Pts',(-21.6029478967997,-14.4319431672138,
114.150734542378)) ;
#180781=CARTESIAN_POINT('Ctrl Pts',(-21.6146814088062,-14.3660067048925,
114.186472926776)) ;
#180782=CARTESIAN_POINT('Ctrl Pts',(-21.6884351663154,-14.4734792612079,
114.446508526122)) ;
#180783=CARTESIAN_POINT('Ctrl Pts',(-21.6943034555198,-14.3999420243742,
114.464382388145)) ;
#180784=CARTESIAN_POINT('Ctrl Pts',(-21.6204996128377,-14.3999420254069,
114.488613432078)) ;
#180785=CARTESIAN_POINT('Ctrl Pts',(-21.5466957701556,-14.3999420264397,
114.512844476011)) ;
#180786=CARTESIAN_POINT('Ctrl Pts',(-21.5408274809512,-14.4734792632734,
114.494970613988)) ;
#180787=CARTESIAN_POINT('Ctrl Pts',(-21.5349591917469,-14.5470165001072,
114.477096751966)) ;
#180788=CARTESIAN_POINT('Ctrl Pts',(-21.608763034429,-14.5470164990744,
114.452865708032)) ;
#180789=CARTESIAN_POINT('Ctrl Pts',(-21.6825668771111,-14.5470164980416,
114.428634664099)) ;
#180790=CARTESIAN_POINT('Ctrl Pts',(-21.6884351663154,-14.4734792612079,
114.446508526122)) ;
#180791=CARTESIAN_POINT('Ctrl Pts',(-21.7683784809354,-14.5056975632985,
114.725551946228)) ;
#180792=CARTESIAN_POINT('Ctrl Pts',(-21.7679376011022,-14.4298031115965,
114.724209097231)) ;
#180793=CARTESIAN_POINT('Ctrl Pts',(-21.6941337602889,-14.4298031119292,
114.748440146856)) ;
#180794=CARTESIAN_POINT('Ctrl Pts',(-21.6203299194757,-14.4298031122619,
114.772671196482)) ;
#180795=CARTESIAN_POINT('Ctrl Pts',(-21.6207707993088,-14.5056975639639,
114.774014045479)) ;
#180796=CARTESIAN_POINT('Ctrl Pts',(-21.621211679142,-14.5815920156659,
114.775356894476)) ;
#180797=CARTESIAN_POINT('Ctrl Pts',(-21.6950155199553,-14.5815920153332,
114.75112584485)) ;
#180798=CARTESIAN_POINT('Ctrl Pts',(-21.7688193607686,-14.5815920150005,
114.726894795225)) ;
#180799=CARTESIAN_POINT('Ctrl Pts',(-21.7683784809354,-14.5056975632985,
114.725551946228)) ;
#180800=CARTESIAN_POINT('Ctrl Pts',(-21.8474157178673,-14.4599236721213,
115.001679784935)) ;
#180801=CARTESIAN_POINT('Ctrl Pts',(-21.8407231446936,-14.387115192455,
114.981295286612)) ;
#180802=CARTESIAN_POINT('Ctrl Pts',(-21.7669193056391,-14.3871151888849,
115.005526341595)) ;
#180803=CARTESIAN_POINT('Ctrl Pts',(-21.6931154665847,-14.3871151853148,
115.029757396577)) ;
#180804=CARTESIAN_POINT('Ctrl Pts',(-21.6998080397583,-14.4599236649811,
115.0501418949)) ;
#180805=CARTESIAN_POINT('Ctrl Pts',(-21.706500612932,-14.5327321446473,
115.070526393222)) ;
#180806=CARTESIAN_POINT('Ctrl Pts',(-21.7803044519865,-14.5327321482174,
115.04629533824)) ;
#180807=CARTESIAN_POINT('Ctrl Pts',(-21.854108291041,-14.5327321517875,
115.022064283257)) ;
#180808=CARTESIAN_POINT('Ctrl Pts',(-21.8474157178673,-14.4599236721213,
115.001679784935)) ;
#180809=CARTESIAN_POINT('Ctrl Pts',(-21.9195991566158,-14.3395761921465,
115.257002682461)) ;
#180810=CARTESIAN_POINT('Ctrl Pts',(-21.9071229816857,-14.27506508821,115.219002266226)) ;
#180811=CARTESIAN_POINT('Ctrl Pts',(-21.8333191441344,-14.2750650771765,
115.243233325787)) ;
#180812=CARTESIAN_POINT('Ctrl Pts',(-21.7595153065832,-14.2750650661431,
115.267464385348)) ;
#180813=CARTESIAN_POINT('Ctrl Pts',(-21.7719914815133,-14.3395761700796,
115.305464801583)) ;
#180814=CARTESIAN_POINT('Ctrl Pts',(-21.7844676564434,-14.4040872740161,
115.343465217818)) ;
#180815=CARTESIAN_POINT('Ctrl Pts',(-21.8582714939946,-14.4040872850496,
115.319234158257)) ;
#180816=CARTESIAN_POINT('Ctrl Pts',(-21.9320753315458,-14.404087296083,
115.295003098696)) ;
#180817=CARTESIAN_POINT('Ctrl Pts',(-21.9195991566158,-14.3395761921465,
115.257002682461)) ;
#180818=CARTESIAN_POINT('Ctrl Pts',(-21.9788462429372,-14.1535350418836,
115.472880057577)) ;
#180819=CARTESIAN_POINT('Ctrl Pts',(-21.9614823731304,-14.101920284912,
115.419992511226)) ;
#180820=CARTESIAN_POINT('Ctrl Pts',(-21.8876785361283,-14.1019202637606,
115.44422357246)) ;
#180821=CARTESIAN_POINT('Ctrl Pts',(-21.8138746991261,-14.1019202426092,
115.468454633693)) ;
#180822=CARTESIAN_POINT('Ctrl Pts',(-21.8312385689329,-14.1535349995808,
115.521342180044)) ;
#180823=CARTESIAN_POINT('Ctrl Pts',(-21.8486024387397,-14.2051497565524,
115.574229726395)) ;
#180824=CARTESIAN_POINT('Ctrl Pts',(-21.9224062757418,-14.2051497777038,
115.549998665161)) ;
#180825=CARTESIAN_POINT('Ctrl Pts',(-21.996210112744,-14.2051497988552,
115.525767603927)) ;
#180826=CARTESIAN_POINT('Ctrl Pts',(-21.9788462429372,-14.1535350418836,
115.472880057577)) ;
#180827=CARTESIAN_POINT('Ctrl Pts',(-22.0203775008148,-13.9130985111844,
115.635036561647)) ;
#180828=CARTESIAN_POINT('Ctrl Pts',(-21.99935074439,-13.8781962453412,115.570992453461)) ;
#180829=CARTESIAN_POINT('Ctrl Pts',(-21.9255469068525,-13.8781962102056,
115.595223513064)) ;
#180830=CARTESIAN_POINT('Ctrl Pts',(-21.851743069315,-13.87819617507,115.619454572667)) ;
#180831=CARTESIAN_POINT('Ctrl Pts',(-21.8727698257398,-13.9130984409133,
115.683498680853)) ;
#180832=CARTESIAN_POINT('Ctrl Pts',(-21.8937965821645,-13.9480007067565,
115.747542789039)) ;
#180833=CARTESIAN_POINT('Ctrl Pts',(-21.967600419702,-13.9480007418921,
115.723311729436)) ;
#180834=CARTESIAN_POINT('Ctrl Pts',(-22.0414042572395,-13.9480007770277,
115.699080669833)) ;
#180835=CARTESIAN_POINT('Ctrl Pts',(-22.0203775008148,-13.9130985111844,
115.635036561647)) ;
#180836=CARTESIAN_POINT('Ctrl Pts',(-22.0399483640035,-13.6395736822347,
115.72995984664)) ;
#180837=CARTESIAN_POINT('Ctrl Pts',(-22.0167942098363,-13.6237185301076,
115.659436028045)) ;
#180838=CARTESIAN_POINT('Ctrl Pts',(-21.9429903696287,-13.6237184841126,
115.683667079515)) ;
#180839=CARTESIAN_POINT('Ctrl Pts',(-21.8691865294211,-13.6237184381175,
115.707898130985)) ;
#180840=CARTESIAN_POINT('Ctrl Pts',(-21.8923406835883,-13.6395735902447,
115.77842194958)) ;
#180841=CARTESIAN_POINT('Ctrl Pts',(-21.9154948377555,-13.6554287423718,
115.848945768175)) ;
#180842=CARTESIAN_POINT('Ctrl Pts',(-21.9892986779631,-13.6554287883668,
115.824714716705)) ;
#180843=CARTESIAN_POINT('Ctrl Pts',(-22.0631025181708,-13.6554288343619,
115.800483665235)) ;
#180844=CARTESIAN_POINT('Ctrl Pts',(-22.0399483640035,-13.6395736822347,
115.72995984664)) ;
#180845=CARTESIAN_POINT('Ctrl Pts',(-22.0358686869632,-13.3487006076146,
115.75305462755)) ;
#180846=CARTESIAN_POINT('Ctrl Pts',(-22.0122308536401,-13.3531309210736,
115.68105760011)) ;
#180847=CARTESIAN_POINT('Ctrl Pts',(-21.9384270093491,-13.3531308648212,
115.705288639143)) ;
#180848=CARTESIAN_POINT('Ctrl Pts',(-21.8646231650582,-13.3531308085687,
115.729519678176)) ;
#180849=CARTESIAN_POINT('Ctrl Pts',(-21.8882609983813,-13.3487004951098,
115.801516705617)) ;
#180850=CARTESIAN_POINT('Ctrl Pts',(-21.9118988317044,-13.3442701816508,
115.873513733057)) ;
#180851=CARTESIAN_POINT('Ctrl Pts',(-21.9857026759953,-13.3442702379032,
115.849282694024)) ;
#180852=CARTESIAN_POINT('Ctrl Pts',(-22.0595065202863,-13.3442702941557,
115.825051654991)) ;
#180853=CARTESIAN_POINT('Ctrl Pts',(-22.0358686869632,-13.3487006076146,
115.75305462755)) ;
#180854=CARTESIAN_POINT('Ctrl Pts',(-22.0075438310689,-13.0636371844073,
115.70218883906)) ;
#180855=CARTESIAN_POINT('Ctrl Pts',(-21.9851168187077,-13.0879765100876,
115.633879776751)) ;
#180856=CARTESIAN_POINT('Ctrl Pts',(-21.9113129689696,-13.0879764491053,
115.658110799193)) ;
#180857=CARTESIAN_POINT('Ctrl Pts',(-21.8375091192314,-13.0879763881229,
115.682341821635)) ;
#180858=CARTESIAN_POINT('Ctrl Pts',(-21.8599361315927,-13.0636370624426,
115.750650883944)) ;
#180859=CARTESIAN_POINT('Ctrl Pts',(-21.882363143954,-13.0392977367622,
115.818959946253)) ;
#180860=CARTESIAN_POINT('Ctrl Pts',(-21.9561669936921,-13.0392977977446,
115.794728923811)) ;
#180861=CARTESIAN_POINT('Ctrl Pts',(-22.0299708434302,-13.0392978587269,
115.77049790137)) ;
#180862=CARTESIAN_POINT('Ctrl Pts',(-22.0075438310689,-13.0636371844073,
115.70218883906)) ;
#180863=CARTESIAN_POINT('Ctrl Pts',(-21.9561819767785,-12.803286823163,
115.581244291729)) ;
#180864=CARTESIAN_POINT('Ctrl Pts',(-21.9365739681163,-12.8458384350668,
115.521521459681)) ;
#180865=CARTESIAN_POINT('Ctrl Pts',(-21.8627701120826,-12.8458383747554,
115.545752462947)) ;
#180866=CARTESIAN_POINT('Ctrl Pts',(-21.788966256049,-12.8458383144439,
115.569983466214)) ;
#180867=CARTESIAN_POINT('Ctrl Pts',(-21.8085742647111,-12.8032867025401,
115.629706298262)) ;
#180868=CARTESIAN_POINT('Ctrl Pts',(-21.8281822733732,-12.7607350906363,
115.68942913031)) ;
#180869=CARTESIAN_POINT('Ctrl Pts',(-21.9019861294069,-12.7607351509478,
115.665198127044)) ;
#180870=CARTESIAN_POINT('Ctrl Pts',(-21.9757899854406,-12.7607352112592,
115.640967123777)) ;
#180871=CARTESIAN_POINT('Ctrl Pts',(-21.9561819767785,-12.803286823163,
115.581244291729)) ;
#180872=CARTESIAN_POINT('Ctrl Pts',(-21.8847933182746,-12.5872505028287,
115.399264233317)) ;
#180873=CARTESIAN_POINT('Ctrl Pts',(-21.8694073476483,-12.644946835435,
115.352401047758)) ;
#180874=CARTESIAN_POINT('Ctrl Pts',(-21.7956034852775,-12.6449467832351,
115.376632031723)) ;
#180875=CARTESIAN_POINT('Ctrl Pts',(-21.7217996229066,-12.6449467310352,
115.400863015687)) ;
#180876=CARTESIAN_POINT('Ctrl Pts',(-21.7371855935328,-12.5872503984288,
115.447726201246)) ;
#180877=CARTESIAN_POINT('Ctrl Pts',(-21.752571564159,-12.5295540658224,
115.494589386805)) ;
#180878=CARTESIAN_POINT('Ctrl Pts',(-21.8263754265299,-12.5295541180224,
115.47035840284)) ;
#180879=CARTESIAN_POINT('Ctrl Pts',(-21.9001792889008,-12.5295541702223,
115.446127418876)) ;
#180880=CARTESIAN_POINT('Ctrl Pts',(-21.8847933182746,-12.5872505028287,
115.399264233317)) ;
#180881=CARTESIAN_POINT('Ctrl Pts',(-21.7976012004924,-12.4304809457012,
115.169196272267)) ;
#180882=CARTESIAN_POINT('Ctrl Pts',(-21.7875456541485,-12.4992062995871,
115.138568698872)) ;
#180883=CARTESIAN_POINT('Ctrl Pts',(-21.7137417860944,-12.4992062624081,
115.162799665526)) ;
#180884=CARTESIAN_POINT('Ctrl Pts',(-21.6399379180403,-12.4992062252292,
115.187030632181)) ;
#180885=CARTESIAN_POINT('Ctrl Pts',(-21.6499934643842,-12.4304808713433,
115.217658205575)) ;
#180886=CARTESIAN_POINT('Ctrl Pts',(-21.6600490107281,-12.3617555174574,
115.24828577897)) ;
#180887=CARTESIAN_POINT('Ctrl Pts',(-21.7338528787822,-12.3617555546364,
115.224054812315)) ;
#180888=CARTESIAN_POINT('Ctrl Pts',(-21.8076567468363,-12.3617555918153,
115.199823845661)) ;
#180889=CARTESIAN_POINT('Ctrl Pts',(-21.7976012004924,-12.4304809457012,
115.169196272267)) ;
#180890=CARTESIAN_POINT('Ctrl Pts',(-21.700169966331,-12.3447676693836,
114.907940821846)) ;
#180891=CARTESIAN_POINT('Ctrl Pts',(-21.6961674254043,-12.4195774199376,
114.895749726183)) ;
#180892=CARTESIAN_POINT('Ctrl Pts',(-21.6223635532352,-12.4195774042201,
114.919980680304)) ;
#180893=CARTESIAN_POINT('Ctrl Pts',(-21.548559681066,-12.4195773885026,
114.944211634424)) ;
#180894=CARTESIAN_POINT('Ctrl Pts',(-21.5525622219927,-12.3447676379485,
114.956402730087)) ;
#180895=CARTESIAN_POINT('Ctrl Pts',(-21.5565647629194,-12.2699578873945,
114.96859382575)) ;
#180896=CARTESIAN_POINT('Ctrl Pts',(-21.6303686350885,-12.269957903112,
114.944362871629)) ;
#180897=CARTESIAN_POINT('Ctrl Pts',(-21.7041725072576,-12.2699579188295,
114.920131917509)) ;
#180898=CARTESIAN_POINT('Ctrl Pts',(-21.700169966331,-12.3447676693836,
114.907940821846)) ;
#180899=CARTESIAN_POINT('Ctrl Pts',(-21.5992738440407,-12.3358385329225,
114.635951321801)) ;
#180900=CARTESIAN_POINT('Ctrl Pts',(-21.6015788063553,-12.4113804397121,
114.642971863216)) ;
#180901=CARTESIAN_POINT('Ctrl Pts',(-21.5277749325704,-12.4113804494303,
114.667202812415)) ;
#180902=CARTESIAN_POINT('Ctrl Pts',(-21.4539710587855,-12.4113804591485,
114.691433761613)) ;
#180903=CARTESIAN_POINT('Ctrl Pts',(-21.4516660964708,-12.335838552359,
114.684413220199)) ;
#180904=CARTESIAN_POINT('Ctrl Pts',(-21.4493611341561,-12.2602966455695,
114.677392678784)) ;
#180905=CARTESIAN_POINT('Ctrl Pts',(-21.523165007941,-12.2602966358513,
114.653161729585)) ;
#180906=CARTESIAN_POINT('Ctrl Pts',(-21.596968881726,-12.260296626133,114.628930780386)) ;
#180907=CARTESIAN_POINT('Ctrl Pts',(-21.5992738440407,-12.3358385329225,
114.635951321801)) ;
#180908=CARTESIAN_POINT('Ctrl Pts',(-21.5003785782672,-12.4042599768703,
114.370232214751)) ;
#180909=CARTESIAN_POINT('Ctrl Pts',(-21.5088568368988,-12.4751356263476,
114.396055620604)) ;
#180910=CARTESIAN_POINT('Ctrl Pts',(-21.4350529637228,-12.4751356632063,
114.420286571658)) ;
#180911=CARTESIAN_POINT('Ctrl Pts',(-21.3612490905468,-12.4751357000651,
114.444517522711)) ;
#180912=CARTESIAN_POINT('Ctrl Pts',(-21.3527708319152,-12.4042600505878,
114.418694116858)) ;
#180913=CARTESIAN_POINT('Ctrl Pts',(-21.3442925732836,-12.3333844011106,
114.392870711006)) ;
#180914=CARTESIAN_POINT('Ctrl Pts',(-21.4180964464596,-12.3333843642518,
114.368639759952)) ;
#180915=CARTESIAN_POINT('Ctrl Pts',(-21.4919003196355,-12.3333843273931,
114.344408808898)) ;
#180916=CARTESIAN_POINT('Ctrl Pts',(-21.5003785782672,-12.4042599768703,
114.370232214751)) ;
#180917=CARTESIAN_POINT('Ctrl Pts',(-21.4104042015346,-12.5454038835963,
114.131652978612)) ;
#180918=CARTESIAN_POINT('Ctrl Pts',(-21.4244426778221,-12.6065294802411,
114.174411910246)) ;
#180919=CARTESIAN_POINT('Ctrl Pts',(-21.3506388079976,-12.6065295430782,
114.198642871508)) ;
#180920=CARTESIAN_POINT('Ctrl Pts',(-21.2768349381732,-12.6065296059152,
114.22287383277)) ;
#180921=CARTESIAN_POINT('Ctrl Pts',(-21.2627964618856,-12.5454040092703,
114.180114901136)) ;
#180922=CARTESIAN_POINT('Ctrl Pts',(-21.2487579855981,-12.4842784126255,
114.137355969502)) ;
#180923=CARTESIAN_POINT('Ctrl Pts',(-21.3225618554226,-12.4842783497885,
114.11312500824)) ;
#180924=CARTESIAN_POINT('Ctrl Pts',(-21.3963657252471,-12.4842782869515,
114.088894046978)) ;
#180925=CARTESIAN_POINT('Ctrl Pts',(-21.4104042015346,-12.5454038835963,
114.131652978612)) ;
#180926=CARTESIAN_POINT('Ctrl Pts',(-21.3349456169578,-12.7490645526663,
113.9372922249)) ;
#180927=CARTESIAN_POINT('Ctrl Pts',(-21.3535389852584,-12.796061398436,
113.993924622637)) ;
#180928=CARTESIAN_POINT('Ctrl Pts',(-21.2797351212098,-12.7960614831609,
114.018155601491)) ;
#180929=CARTESIAN_POINT('Ctrl Pts',(-21.2059312571613,-12.7960615678859,
114.042386580345)) ;
#180930=CARTESIAN_POINT('Ctrl Pts',(-21.1873378888607,-12.7490647221162,
113.985754182609)) ;
#180931=CARTESIAN_POINT('Ctrl Pts',(-21.1687445205602,-12.7020678763465,
113.929121784872)) ;
#180932=CARTESIAN_POINT('Ctrl Pts',(-21.2425483846087,-12.7020677916216,
113.904890806017)) ;
#180933=CARTESIAN_POINT('Ctrl Pts',(-21.3163522486572,-12.7020677068967,
113.880659827163)) ;
#180934=CARTESIAN_POINT('Ctrl Pts',(-21.3349456169578,-12.7490645526663,
113.9372922249)) ;
#180935=CARTESIAN_POINT('Ctrl Pts',(-21.278705237238,-13.0004109945635,
113.801433245637)) ;
#180936=CARTESIAN_POINT('Ctrl Pts',(-21.300519235436,-13.0299291555683,
113.867875162378)) ;
#180937=CARTESIAN_POINT('Ctrl Pts',(-21.2267153790532,-13.0299292556675,
113.892106164581)) ;
#180938=CARTESIAN_POINT('Ctrl Pts',(-21.1529115226705,-13.0299293557667,
113.916337166784)) ;
#180939=CARTESIAN_POINT('Ctrl Pts',(-21.1310975244725,-13.0004111947619,
113.849895250044)) ;
#180940=CARTESIAN_POINT('Ctrl Pts',(-21.1092835262744,-12.9708930337571,
113.783453333303)) ;
#180941=CARTESIAN_POINT('Ctrl Pts',(-21.1830873826572,-12.9708929336578,
113.7592223311)) ;
#180942=CARTESIAN_POINT('Ctrl Pts',(-21.25689123904,-12.9708928335586,113.734991328897)) ;
#180943=CARTESIAN_POINT('Ctrl Pts',(-21.278705237238,-13.0004109945635,
113.801433245637)) ;
#180944=CARTESIAN_POINT('Ctrl Pts',(-21.2448570719353,-13.281956740539,
113.733818494743)) ;
#180945=CARTESIAN_POINT('Ctrl Pts',(-21.2683324030269,-13.2918622013087,
113.805320563426)) ;
#180946=CARTESIAN_POINT('Ctrl Pts',(-21.1945285554331,-13.2918623086419,
113.8295515924)) ;
#180947=CARTESIAN_POINT('Ctrl Pts',(-21.1207247078394,-13.2918624159751,
113.853782621373)) ;
#180948=CARTESIAN_POINT('Ctrl Pts',(-21.0972493767479,-13.2819569552054,
113.782280552689)) ;
#180949=CARTESIAN_POINT('Ctrl Pts',(-21.0737740456563,-13.2720514944356,
113.710778484005)) ;
#180950=CARTESIAN_POINT('Ctrl Pts',(-21.14757789325,-13.2720513871025,113.686547455032)) ;
#180951=CARTESIAN_POINT('Ctrl Pts',(-21.2213817408438,-13.2720512797693,
113.662316426059)) ;
#180952=CARTESIAN_POINT('Ctrl Pts',(-21.2448570719353,-13.281956740539,
113.733818494743)) ;
#180953=CARTESIAN_POINT('Ctrl Pts',(-21.2351498447256,-13.573019683806,
113.739702682927)) ;
#180954=CARTESIAN_POINT('Ctrl Pts',(-21.2586042557794,-13.5626188486144,
113.811141032577)) ;
#180955=CARTESIAN_POINT('Ctrl Pts',(-21.1848004171839,-13.5626189543087,
113.835372088957)) ;
#180956=CARTESIAN_POINT('Ctrl Pts',(-21.1109965785883,-13.5626190600031,
113.859603145337)) ;
#180957=CARTESIAN_POINT('Ctrl Pts',(-21.0875421675344,-13.5730198951947,
113.788164795687)) ;
#180958=CARTESIAN_POINT('Ctrl Pts',(-21.0640877564806,-13.5834207303863,
113.716726446036)) ;
#180959=CARTESIAN_POINT('Ctrl Pts',(-21.1378915950762,-13.583420624692,
113.692495389656)) ;
#180960=CARTESIAN_POINT('Ctrl Pts',(-21.2116954336718,-13.5834205189976,
113.668264333277)) ;
#180961=CARTESIAN_POINT('Ctrl Pts',(-21.2351498447256,-13.573019683806,
113.739702682927)) ;
#180962=CARTESIAN_POINT('Ctrl Pts',(-21.2495046916565,-13.8532505028034,
113.818910957215)) ;
#180963=CARTESIAN_POINT('Ctrl Pts',(-21.2712576372625,-13.823269355178,
113.885166917691)) ;
#180964=CARTESIAN_POINT('Ctrl Pts',(-21.1974538069553,-13.823269450611,
113.909397999316)) ;
#180965=CARTESIAN_POINT('Ctrl Pts',(-21.1236499766481,-13.8232695460439,
113.933629080941)) ;
#180966=CARTESIAN_POINT('Ctrl Pts',(-21.101897031042,-13.8532506936693,
113.867373120465)) ;
#180967=CARTESIAN_POINT('Ctrl Pts',(-21.080144085436,-13.8832318412947,
113.801117159989)) ;
#180968=CARTESIAN_POINT('Ctrl Pts',(-21.1539479157432,-13.8832317458617,
113.776886078364)) ;
#180969=CARTESIAN_POINT('Ctrl Pts',(-21.2277517460505,-13.8832316504288,
113.752654996739)) ;
#180970=CARTESIAN_POINT('Ctrl Pts',(-21.2495046916565,-13.8532505028034,
113.818910957215)) ;
#180971=CARTESIAN_POINT('Ctrl Pts',(-21.2861585371864,-14.1021597581384,
113.966023254985)) ;
#180972=CARTESIAN_POINT('Ctrl Pts',(-21.3046510157037,-14.0547556097992,
114.022348358853)) ;
#180973=CARTESIAN_POINT('Ctrl Pts',(-21.2308471921295,-14.0547556877835,
114.046579460986)) ;
#180974=CARTESIAN_POINT('Ctrl Pts',(-21.1570433685553,-14.0547557657678,
114.070810563118)) ;
#180975=CARTESIAN_POINT('Ctrl Pts',(-21.138550890038,-14.102159914107,114.01448545925)) ;
#180976=CARTESIAN_POINT('Ctrl Pts',(-21.1200584115207,-14.1495640624461,
113.958160355381)) ;
#180977=CARTESIAN_POINT('Ctrl Pts',(-21.1938622350949,-14.1495639844619,
113.933929253249)) ;
#180978=CARTESIAN_POINT('Ctrl Pts',(-21.2676660586691,-14.1495639064776,
113.909698151116)) ;
#180979=CARTESIAN_POINT('Ctrl Pts',(-21.2861585371864,-14.1021597581384,
113.966023254985)) ;
#180980=CARTESIAN_POINT('Ctrl Pts',(-21.3416525533176,-14.3018608409922,
114.170484973414)) ;
#180981=CARTESIAN_POINT('Ctrl Pts',(-21.3555650519419,-14.240442969134,
114.212860197592)) ;
#180982=CARTESIAN_POINT('Ctrl Pts',(-21.2817612329827,-14.2404430248273,
114.237091313781)) ;
#180983=CARTESIAN_POINT('Ctrl Pts',(-21.2079574140235,-14.2404430805207,
114.261322429971)) ;
#180984=CARTESIAN_POINT('Ctrl Pts',(-21.1940449153992,-14.3018609523788,
114.218947205793)) ;
#180985=CARTESIAN_POINT('Ctrl Pts',(-21.1801324167749,-14.3632788242369,
114.176571981615)) ;
#180986=CARTESIAN_POINT('Ctrl Pts',(-21.2539362357341,-14.3632787685436,
114.152340865426)) ;
#180987=CARTESIAN_POINT('Ctrl Pts',(-21.3277400546933,-14.3632787128503,
114.128109749236)) ;
#180988=CARTESIAN_POINT('Ctrl Pts',(-21.3416525533176,-14.3018608409922,
114.170484973414)) ;
#180989=CARTESIAN_POINT('Ctrl Pts',(-21.411315277641,-14.4384983198451,
114.418115610093)) ;
#180990=CARTESIAN_POINT('Ctrl Pts',(-21.4196514727048,-14.3674483770308,
114.443506313464)) ;
#180991=CARTESIAN_POINT('Ctrl Pts',(-21.3458476559104,-14.3674484079295,
114.467737436247)) ;
#180992=CARTESIAN_POINT('Ctrl Pts',(-21.2720438391161,-14.3674484388281,
114.49196855903)) ;
#180993=CARTESIAN_POINT('Ctrl Pts',(-21.2637076440523,-14.4384983816424,
114.466577855659)) ;
#180994=CARTESIAN_POINT('Ctrl Pts',(-21.2553714489885,-14.5095483244567,
114.441187152289)) ;
#180995=CARTESIAN_POINT('Ctrl Pts',(-21.3291752657829,-14.509548293558,
114.416956029506)) ;
#180996=CARTESIAN_POINT('Ctrl Pts',(-21.4029790825773,-14.5095482626594,
114.392724906723)) ;
#180997=CARTESIAN_POINT('Ctrl Pts',(-21.411315277641,-14.4384983198451,
114.418115610093)) ;
#180998=CARTESIAN_POINT('Ctrl Pts',(-21.4896790967479,-14.5020770602936,
114.692365991293)) ;
#180999=CARTESIAN_POINT('Ctrl Pts',(-21.4918207117146,-14.4264807176174,
114.698889003319)) ;
#181000=CARTESIAN_POINT('Ctrl Pts',(-21.4180168942886,-14.4264807240547,
114.723120124178)) ;
#181001=CARTESIAN_POINT('Ctrl Pts',(-21.3442130768625,-14.426480730492,
114.747351245037)) ;
#181002=CARTESIAN_POINT('Ctrl Pts',(-21.3420714618958,-14.5020770731682,
114.740828233011)) ;
#181003=CARTESIAN_POINT('Ctrl Pts',(-21.339929846929,-14.5776734158445,
114.734305220985)) ;
#181004=CARTESIAN_POINT('Ctrl Pts',(-21.4137336643551,-14.5776734094072,
114.710074100126)) ;
#181005=CARTESIAN_POINT('Ctrl Pts',(-21.4875374817811,-14.5776734029699,
114.685842979267)) ;
#181006=CARTESIAN_POINT('Ctrl Pts',(-21.4896790967479,-14.5020770602936,
114.692365991293)) ;
#181007=CARTESIAN_POINT('Ctrl Pts',(-21.5697542529171,-14.48777877411,114.971664919752)) ;
#181008=CARTESIAN_POINT('Ctrl Pts',(-21.5655757371925,-14.4130666847603,
114.958937833571)) ;
#181009=CARTESIAN_POINT('Ctrl Pts',(-21.4917719173005,-14.413066670136,
114.98316894692)) ;
#181010=CARTESIAN_POINT('Ctrl Pts',(-21.4179680974086,-14.4130666555116,
115.007400060268)) ;
#181011=CARTESIAN_POINT('Ctrl Pts',(-21.4221466131332,-14.4877787448612,
115.020127146449)) ;
#181012=CARTESIAN_POINT('Ctrl Pts',(-21.4263251288578,-14.5624908342109,
115.032854232629)) ;
#181013=CARTESIAN_POINT('Ctrl Pts',(-21.5001289487497,-14.5624908488352,
115.008623119281)) ;
#181014=CARTESIAN_POINT('Ctrl Pts',(-21.5739327686417,-14.5624908634596,
114.984392005932)) ;
#181015=CARTESIAN_POINT('Ctrl Pts',(-21.5697542529171,-14.48777877411,114.971664919752)) ;
#181016=CARTESIAN_POINT('Ctrl Pts',(-21.6455150626232,-14.3970097456745,
115.237875186916)) ;
#181017=CARTESIAN_POINT('Ctrl Pts',(-21.6353069764491,-14.3285220925645,
115.206783002163)) ;
#181018=CARTESIAN_POINT('Ctrl Pts',(-21.5615031523443,-14.3285220617789,
115.231014102679)) ;
#181019=CARTESIAN_POINT('Ctrl Pts',(-21.4876993282394,-14.3285220309933,
115.255245203196)) ;
#181020=CARTESIAN_POINT('Ctrl Pts',(-21.4979074144135,-14.3970096841033,
115.286337387949)) ;
#181021=CARTESIAN_POINT('Ctrl Pts',(-21.5081155005876,-14.4654973372134,
115.317429572702)) ;
#181022=CARTESIAN_POINT('Ctrl Pts',(-21.5819193246924,-14.465497367999,
115.293198472186)) ;
#181023=CARTESIAN_POINT('Ctrl Pts',(-21.6557231487973,-14.4654973987846,
115.268967371669)) ;
#181024=CARTESIAN_POINT('Ctrl Pts',(-21.6455150626232,-14.3970097456745,
115.237875186916)) ;
#181025=CARTESIAN_POINT('Ctrl Pts',(-21.7106846353234,-14.2362612997962,
115.471811422078)) ;
#181026=CARTESIAN_POINT('Ctrl Pts',(-21.6951775844478,-14.1788934065685,
115.424579445984)) ;
#181027=CARTESIAN_POINT('Ctrl Pts',(-21.6213737551867,-14.1788933656858,
115.448810530796)) ;
#181028=CARTESIAN_POINT('Ctrl Pts',(-21.5475699259256,-14.178893324803,
115.473041615607)) ;
#181029=CARTESIAN_POINT('Ctrl Pts',(-21.5630769768012,-14.2362612180308,
115.520273591701)) ;
#181030=CARTESIAN_POINT('Ctrl Pts',(-21.5785840276768,-14.2936291112585,
115.567505567795)) ;
#181031=CARTESIAN_POINT('Ctrl Pts',(-21.6523878569379,-14.2936291521412,
115.543274482984)) ;
#181032=CARTESIAN_POINT('Ctrl Pts',(-21.726191686199,-14.293629193024,115.519043398172)) ;
#181033=CARTESIAN_POINT('Ctrl Pts',(-21.7106846353234,-14.2362612997962,
115.471811422078)) ;
#181034=CARTESIAN_POINT('Ctrl Pts',(-21.7599663610644,-14.0159101115065,
115.65749922043)) ;
#181035=CARTESIAN_POINT('Ctrl Pts',(-21.740258470966,-13.973840125215,115.597472166055)) ;
#181036=CARTESIAN_POINT('Ctrl Pts',(-21.666454636156,-13.97384008191,115.621703233965)) ;
#181037=CARTESIAN_POINT('Ctrl Pts',(-21.592650801346,-13.973840038605,115.645934301876)) ;
#181038=CARTESIAN_POINT('Ctrl Pts',(-21.6123586914444,-14.0159100248966,
115.705961356251)) ;
#181039=CARTESIAN_POINT('Ctrl Pts',(-21.6320665815428,-14.0579800111881,
115.765988410626)) ;
#181040=CARTESIAN_POINT('Ctrl Pts',(-21.7058704163528,-14.0579800544931,
115.741757342715)) ;
#181041=CARTESIAN_POINT('Ctrl Pts',(-21.7796742511628,-14.0579800977981,
115.717526274805)) ;
#181042=CARTESIAN_POINT('Ctrl Pts',(-21.7599663610644,-14.0159101115065,
115.65749922043)) ;
#181043=CARTESIAN_POINT('Ctrl Pts',(-21.7887254354454,-13.7543350935969,
115.7804395058)) ;
#181044=CARTESIAN_POINT('Ctrl Pts',(-21.7662483401476,-13.7304650573216,
115.711977899343)) ;
#181045=CARTESIAN_POINT('Ctrl Pts',(-21.6924445007129,-13.730465015473,
115.736208953168)) ;
#181046=CARTESIAN_POINT('Ctrl Pts',(-21.6186406612782,-13.7304649736245,
115.760440006992)) ;
#181047=CARTESIAN_POINT('Ctrl Pts',(-21.6411177565759,-13.7543350098997,
115.828901613449)) ;
#181048=CARTESIAN_POINT('Ctrl Pts',(-21.6635948518736,-13.778205046175,
115.897363219905)) ;
#181049=CARTESIAN_POINT('Ctrl Pts',(-21.7373986913083,-13.7782050880236,
115.873132166081)) ;
#181050=CARTESIAN_POINT('Ctrl Pts',(-21.8112025307431,-13.7782051298721,
115.848901112257)) ;
#181051=CARTESIAN_POINT('Ctrl Pts',(-21.7887254354454,-13.7543350935969,
115.7804395058)) ;
#181052=CARTESIAN_POINT('Ctrl Pts',(-21.7944517107035,-13.4665595551094,
115.833506874945)) ;
#181053=CARTESIAN_POINT('Ctrl Pts',(-21.7708033171206,-13.4627465020412,
115.761477683097)) ;
#181054=CARTESIAN_POINT('Ctrl Pts',(-21.6969994739287,-13.4627464684725,
115.785708725478)) ;
#181055=CARTESIAN_POINT('Ctrl Pts',(-21.6231956307368,-13.4627464349037,
115.809939767858)) ;
#181056=CARTESIAN_POINT('Ctrl Pts',(-21.6468440243196,-13.4665594879718,
115.881968959706)) ;
#181057=CARTESIAN_POINT('Ctrl Pts',(-21.6704924179025,-13.4703725410399,
115.953998151553)) ;
#181058=CARTESIAN_POINT('Ctrl Pts',(-21.7442962610944,-13.4703725746087,
115.929767109173)) ;
#181059=CARTESIAN_POINT('Ctrl Pts',(-21.8181001042863,-13.4703726081775,
115.905536066792)) ;
#181060=CARTESIAN_POINT('Ctrl Pts',(-21.7944517107035,-13.4665595551094,
115.833506874945)) ;
#181061=CARTESIAN_POINT('Ctrl Pts',(-21.7759076496093,-13.1776643244991,
115.812347038779)) ;
#181062=CARTESIAN_POINT('Ctrl Pts',(-21.7527874084242,-13.1940170948714,
115.741926514053)) ;
#181063=CARTESIAN_POINT('Ctrl Pts',(-21.6789835629887,-13.1940170691323,
115.7661575496)) ;
#181064=CARTESIAN_POINT('Ctrl Pts',(-21.6051797175531,-13.1940170433932,
115.790388585147)) ;
#181065=CARTESIAN_POINT('Ctrl Pts',(-21.6282999587382,-13.1776642730209,
115.860809109873)) ;
#181066=CARTESIAN_POINT('Ctrl Pts',(-21.6514201999233,-13.1613115026485,
115.931229634599)) ;
#181067=CARTESIAN_POINT('Ctrl Pts',(-21.7252240453588,-13.1613115283877,
115.906998599052)) ;
#181068=CARTESIAN_POINT('Ctrl Pts',(-21.7990278907943,-13.1613115541268,
115.882767563505)) ;
#181069=CARTESIAN_POINT('Ctrl Pts',(-21.7759076496093,-13.1776643244991,
115.812347038779)) ;
#181070=CARTESIAN_POINT('Ctrl Pts',(-21.7336480522878,-12.90467088677,115.719119626664)) ;
#181071=CARTESIAN_POINT('Ctrl Pts',(-21.7127091437857,-12.9401099840166,
115.655343089489)) ;
#181072=CARTESIAN_POINT('Ctrl Pts',(-21.6389052974629,-12.9401099680248,
115.679574122334)) ;
#181073=CARTESIAN_POINT('Ctrl Pts',(-21.5651014511401,-12.9401099520331,
115.703805155178)) ;
#181074=CARTESIAN_POINT('Ctrl Pts',(-21.5860403596422,-12.9046708547865,
115.767581692352)) ;
#181075=CARTESIAN_POINT('Ctrl Pts',(-21.6069792681442,-12.86923175754,115.831358229527)) ;
#181076=CARTESIAN_POINT('Ctrl Pts',(-21.680783114467,-12.8692317735317,
115.807127196682)) ;
#181077=CARTESIAN_POINT('Ctrl Pts',(-21.7545869607898,-12.8692317895235,
115.782896163838)) ;
#181078=CARTESIAN_POINT('Ctrl Pts',(-21.7336480522878,-12.90467088677,115.719119626664)) ;
#181079=CARTESIAN_POINT('Ctrl Pts',(-21.670032619818,-12.6688603640825,
115.560779753081)) ;
#181080=CARTESIAN_POINT('Ctrl Pts',(-21.6527710229661,-12.7208184006723,
115.508203713992)) ;
#181081=CARTESIAN_POINT('Ctrl Pts',(-21.5789671769035,-12.7208183925847,
115.532434747629)) ;
#181082=CARTESIAN_POINT('Ctrl Pts',(-21.505163330841,-12.7208183844972,
115.556665781266)) ;
#181083=CARTESIAN_POINT('Ctrl Pts',(-21.5224249276929,-12.6688603479075,
115.609241820356)) ;
#181084=CARTESIAN_POINT('Ctrl Pts',(-21.5396865245448,-12.6169023113178,
115.661817859445)) ;
#181085=CARTESIAN_POINT('Ctrl Pts',(-21.6134903706073,-12.6169023194053,
115.637586825808)) ;
#181086=CARTESIAN_POINT('Ctrl Pts',(-21.6872942166699,-12.6169023274928,
115.613355792171)) ;
#181087=CARTESIAN_POINT('Ctrl Pts',(-21.670032619818,-12.6688603640825,
115.560779753081)) ;
#181088=CARTESIAN_POINT('Ctrl Pts',(-21.5885287279957,-12.48602188738,115.348081223403)) ;
#181089=CARTESIAN_POINT('Ctrl Pts',(-21.5761965323051,-12.5508253721629,
115.310519345023)) ;
#181090=CARTESIAN_POINT('Ctrl Pts',(-21.5023926874474,-12.5508253699932,
115.33475038233)) ;
#181091=CARTESIAN_POINT('Ctrl Pts',(-21.4285888425897,-12.5508253678235,
115.358981419637)) ;
#181092=CARTESIAN_POINT('Ctrl Pts',(-21.4409210382802,-12.4860218830405,
115.396543298016)) ;
#181093=CARTESIAN_POINT('Ctrl Pts',(-21.4532532339708,-12.4212183982575,
115.434105176396)) ;
#181094=CARTESIAN_POINT('Ctrl Pts',(-21.5270570788285,-12.4212184004273,
115.409874139089)) ;
#181095=CARTESIAN_POINT('Ctrl Pts',(-21.6008609236862,-12.421218402597,
115.385643101782)) ;
#181096=CARTESIAN_POINT('Ctrl Pts',(-21.5885287279957,-12.48602188738,115.348081223403)) ;
#181097=CARTESIAN_POINT('Ctrl Pts',(-21.4945267923872,-12.3704601308902,
115.097266800152)) ;
#181098=CARTESIAN_POINT('Ctrl Pts',(-21.4880053381033,-12.4434303508523,
115.077403502628)) ;
#181099=CARTESIAN_POINT('Ctrl Pts',(-21.4142014945595,-12.4434303510562,
115.101634543937)) ;
#181100=CARTESIAN_POINT('Ctrl Pts',(-21.3403976510158,-12.4434303512601,
115.125865585246)) ;
#181101=CARTESIAN_POINT('Ctrl Pts',(-21.3469191052998,-12.370460131298,
115.14572888277)) ;
#181102=CARTESIAN_POINT('Ctrl Pts',(-21.3534405595837,-12.297489911336,
115.165592180293)) ;
#181103=CARTESIAN_POINT('Ctrl Pts',(-21.4272444031274,-12.2974899111321,
115.141361138984)) ;
#181104=CARTESIAN_POINT('Ctrl Pts',(-21.5010482466712,-12.2974899109282,
115.117130097675)) ;
#181105=CARTESIAN_POINT('Ctrl Pts',(-21.4945267923872,-12.3704601308902,
115.097266800152)) ;
#181106=CARTESIAN_POINT('Ctrl Pts',(-21.3942570657881,-12.3301504850153,
114.827261741778)) ;
#181107=CARTESIAN_POINT('Ctrl Pts',(-21.3939948822089,-12.406044193393,
114.826463172943)) ;
#181108=CARTESIAN_POINT('Ctrl Pts',(-21.3201910395033,-12.4060441935951,
114.850694216804)) ;
#181109=CARTESIAN_POINT('Ctrl Pts',(-21.2463871967976,-12.4060441937972,
114.874925260666)) ;
#181110=CARTESIAN_POINT('Ctrl Pts',(-21.2466493803768,-12.3301504854195,
114.875723829501)) ;
#181111=CARTESIAN_POINT('Ctrl Pts',(-21.2469115639559,-12.2542567770418,
114.876522398337)) ;
#181112=CARTESIAN_POINT('Ctrl Pts',(-21.3207154066615,-12.2542567768397,
114.852291354475)) ;
#181113=CARTESIAN_POINT('Ctrl Pts',(-21.3945192493672,-12.2542567766376,
114.828060310614)) ;
#181114=CARTESIAN_POINT('Ctrl Pts',(-21.3942570657881,-12.3301504850153,
114.827261741778)) ;
#181115=CARTESIAN_POINT('Ctrl Pts',(-21.2939223840727,-12.3670848663884,
114.557023720825)) ;
#181116=CARTESIAN_POINT('Ctrl Pts',(-21.299934115299,-12.440512077599,114.57533448422)) ;
#181117=CARTESIAN_POINT('Ctrl Pts',(-21.2261302729601,-12.4405120766493,
114.599565529198)) ;
#181118=CARTESIAN_POINT('Ctrl Pts',(-21.1523264306211,-12.4405120756996,
114.623796574177)) ;
#181119=CARTESIAN_POINT('Ctrl Pts',(-21.1463146993948,-12.367084864489,
114.605485810782)) ;
#181120=CARTESIAN_POINT('Ctrl Pts',(-21.1403029681685,-12.2936576532783,
114.587175047387)) ;
#181121=CARTESIAN_POINT('Ctrl Pts',(-21.2141068105074,-12.293657654228,
114.562944002409)) ;
#181122=CARTESIAN_POINT('Ctrl Pts',(-21.2879106528464,-12.2936576551777,
114.53871295743)) ;
#181123=CARTESIAN_POINT('Ctrl Pts',(-21.2939223840727,-12.3670848663884,
114.557023720825)) ;
#181124=CARTESIAN_POINT('Ctrl Pts',(-21.1989536269659,-12.4806961242678,
114.303499956068)) ;
#181125=CARTESIAN_POINT('Ctrl Pts',(-21.2108665545281,-12.5462988180666,
114.339784811313)) ;
#181126=CARTESIAN_POINT('Ctrl Pts',(-21.1370627115663,-12.5462988169735,
114.364015854394)) ;
#181127=CARTESIAN_POINT('Ctrl Pts',(-21.0632588686045,-12.5462988158804,
114.388246897476)) ;
#181128=CARTESIAN_POINT('Ctrl Pts',(-21.0513459410423,-12.4806961220815,
114.351962042231)) ;
#181129=CARTESIAN_POINT('Ctrl Pts',(-21.0394330134802,-12.4150934282827,
114.315677186986)) ;
#181130=CARTESIAN_POINT('Ctrl Pts',(-21.113236856442,-12.4150934293758,
114.291446143904)) ;
#181131=CARTESIAN_POINT('Ctrl Pts',(-21.1870406994037,-12.415093430469,
114.267215100823)) ;
#181132=CARTESIAN_POINT('Ctrl Pts',(-21.1989536269659,-12.4806961242678,
114.303499956068)) ;
#181133=CARTESIAN_POINT('Ctrl Pts',(-21.1174616220678,-12.659847054779,
114.090572179847)) ;
#181134=CARTESIAN_POINT('Ctrl Pts',(-21.1343519658611,-12.7130362017687,
114.142017441774)) ;
#181135=CARTESIAN_POINT('Ctrl Pts',(-21.0605481221497,-12.7130362022566,
114.166248482573)) ;
#181136=CARTESIAN_POINT('Ctrl Pts',(-20.9867442784384,-12.7130362027444,
114.190479523371)) ;
#181137=CARTESIAN_POINT('Ctrl Pts',(-20.9698539346452,-12.6598470557547,
114.139034261444)) ;
#181138=CARTESIAN_POINT('Ctrl Pts',(-20.9529635908519,-12.606657908765,
114.087588999516)) ;
#181139=CARTESIAN_POINT('Ctrl Pts',(-21.0267674345633,-12.6066579082772,
114.063357958718)) ;
#181140=CARTESIAN_POINT('Ctrl Pts',(-21.1005712782746,-12.6066579077893,
114.039126917919)) ;
#181141=CARTESIAN_POINT('Ctrl Pts',(-21.1174616220678,-12.659847054779,
114.090572179847)) ;
#181142=CARTESIAN_POINT('Ctrl Pts',(-21.0527943299023,-12.8944266812495,
113.929149642183)) ;
#181143=CARTESIAN_POINT('Ctrl Pts',(-21.0734893261191,-12.9313139586903,
113.992183261414)) ;
#181144=CARTESIAN_POINT('Ctrl Pts',(-20.9996854816442,-12.9313139638645,
114.016414299887)) ;
#181145=CARTESIAN_POINT('Ctrl Pts',(-20.9258816371693,-12.9313139690387,
114.04064533836)) ;
#181146=CARTESIAN_POINT('Ctrl Pts',(-20.9051866409525,-12.8944266915978,
113.977611719129)) ;
#181147=CARTESIAN_POINT('Ctrl Pts',(-20.8844916447358,-12.8575394141569,
113.914578099897)) ;
#181148=CARTESIAN_POINT('Ctrl Pts',(-20.9582954892107,-12.8575394089827,
113.890347061425)) ;
#181149=CARTESIAN_POINT('Ctrl Pts',(-21.0320993336856,-12.8575394038086,
113.866116022952)) ;
#181150=CARTESIAN_POINT('Ctrl Pts',(-21.0527943299023,-12.8944266812495,
113.929149642183)) ;
#181151=CARTESIAN_POINT('Ctrl Pts',(-21.009715412858,-13.1656332510844,
113.833333116255)) ;
#181152=CARTESIAN_POINT('Ctrl Pts',(-21.0327159486317,-13.183637429578,
113.903389036868)) ;
#181153=CARTESIAN_POINT('Ctrl Pts',(-20.9589121041979,-13.1836374410536,
113.927620075466)) ;
#181154=CARTESIAN_POINT('Ctrl Pts',(-20.885108259764,-13.1836374525291,
113.951851114064)) ;
#181155=CARTESIAN_POINT('Ctrl Pts',(-20.8621077239903,-13.1656332740355,
113.88179519345)) ;
#181156=CARTESIAN_POINT('Ctrl Pts',(-20.8391071882165,-13.1476290955419,
113.811739272837)) ;
#181157=CARTESIAN_POINT('Ctrl Pts',(-20.9129110326504,-13.1476290840664,
113.787508234239)) ;
#181158=CARTESIAN_POINT('Ctrl Pts',(-20.9867148770842,-13.1476290725908,
113.763277195641)) ;
#181159=CARTESIAN_POINT('Ctrl Pts',(-21.009715412858,-13.1656332510844,
113.833333116255)) ;
#181160=CARTESIAN_POINT('Ctrl Pts',(-20.9901169836703,-13.455130793988,
113.809077738093)) ;
#181161=CARTESIAN_POINT('Ctrl Pts',(-21.0137859653004,-13.4529475727115,
113.8811696368)) ;
#181162=CARTESIAN_POINT('Ctrl Pts',(-20.9399821218703,-13.452947591497,
113.905400678454)) ;
#181163=CARTESIAN_POINT('Ctrl Pts',(-20.8661782784401,-13.4529476102826,
113.929631720109)) ;
#181164=CARTESIAN_POINT('Ctrl Pts',(-20.84250929681,-13.4551308315591,113.857539821403)) ;
#181165=CARTESIAN_POINT('Ctrl Pts',(-20.8188403151799,-13.4573140528355,
113.785447922696)) ;
#181166=CARTESIAN_POINT('Ctrl Pts',(-20.89264415861,-13.45731403405,113.761216881042)) ;
#181167=CARTESIAN_POINT('Ctrl Pts',(-20.9664480020402,-13.4573140152645,
113.736985839387)) ;
#181168=CARTESIAN_POINT('Ctrl Pts',(-20.9901169836703,-13.455130793988,
113.809077738093)) ;
#181169=CARTESIAN_POINT('Ctrl Pts',(-20.9948751859287,-13.7427936624919,
113.859110662264)) ;
#181170=CARTESIAN_POINT('Ctrl Pts',(-21.0175108531374,-13.7205220170914,
113.928055251801)) ;
#181171=CARTESIAN_POINT('Ctrl Pts',(-20.9437070120615,-13.7205220434154,
113.952286300627)) ;
#181172=CARTESIAN_POINT('Ctrl Pts',(-20.8699031709856,-13.7205220697394,
113.976517349452)) ;
#181173=CARTESIAN_POINT('Ctrl Pts',(-20.847267503777,-13.7427937151399,
113.907572759915)) ;
#181174=CARTESIAN_POINT('Ctrl Pts',(-20.8246318365683,-13.7650653605404,
113.838628170377)) ;
#181175=CARTESIAN_POINT('Ctrl Pts',(-20.8984356776442,-13.7650653342164,
113.814397121552)) ;
#181176=CARTESIAN_POINT('Ctrl Pts',(-20.9722395187201,-13.7650653078924,
113.790166072726)) ;
#181177=CARTESIAN_POINT('Ctrl Pts',(-20.9948751859287,-13.7427936624919,
113.859110662264)) ;
#181178=CARTESIAN_POINT('Ctrl Pts',(-21.0227622802631,-14.0059776158613,
113.979433797495)) ;
#181179=CARTESIAN_POINT('Ctrl Pts',(-21.0427513300967,-13.9652981717702,
114.040317217391)) ;
#181180=CARTESIAN_POINT('Ctrl Pts',(-20.9689474924063,-13.9652982015733,
114.064548276528)) ;
#181181=CARTESIAN_POINT('Ctrl Pts',(-20.895143654716,-13.9652982313764,
114.088779335666)) ;
#181182=CARTESIAN_POINT('Ctrl Pts',(-20.8751546048824,-14.0059776754674,
114.02789591577)) ;
#181183=CARTESIAN_POINT('Ctrl Pts',(-20.8551655550488,-14.0466571195585,
113.967012495875)) ;
#181184=CARTESIAN_POINT('Ctrl Pts',(-20.9289693927392,-14.0466570897554,
113.942781436737)) ;
#181185=CARTESIAN_POINT('Ctrl Pts',(-21.0027732304295,-14.0466570599524,
113.9185503776)) ;
#181186=CARTESIAN_POINT('Ctrl Pts',(-21.0227622802631,-14.0059776158613,
113.979433797495)) ;
#181187=CARTESIAN_POINT('Ctrl Pts',(-21.0711237055155,-14.2279037819529,
114.162216793604)) ;
#181188=CARTESIAN_POINT('Ctrl Pts',(-21.0870308603311,-14.1716706622332,
114.210667419716)) ;
#181189=CARTESIAN_POINT('Ctrl Pts',(-21.0132270269163,-14.1716706921349,
114.234898491876)) ;
#181190=CARTESIAN_POINT('Ctrl Pts',(-20.9394231935014,-14.1716707220365,
114.259129564036)) ;
#181191=CARTESIAN_POINT('Ctrl Pts',(-20.9235160386858,-14.2279038417561,
114.210678937924)) ;
#181192=CARTESIAN_POINT('Ctrl Pts',(-20.9076088838701,-14.2841369614758,
114.162228311812)) ;
#181193=CARTESIAN_POINT('Ctrl Pts',(-20.981412717285,-14.2841369315741,
114.137997239652)) ;
#181194=CARTESIAN_POINT('Ctrl Pts',(-21.0552165506998,-14.2841369016725,
114.113766167492)) ;
#181195=CARTESIAN_POINT('Ctrl Pts',(-21.0711237055155,-14.2279037819529,
114.162216793604)) ;
#181196=CARTESIAN_POINT('Ctrl Pts',(-21.1359737665809,-14.3919406672911,
114.39531754647)) ;
#181197=CARTESIAN_POINT('Ctrl Pts',(-21.1466400020903,-14.3241730854154,
114.427805177804)) ;
#181198=CARTESIAN_POINT('Ctrl Pts',(-21.0728361735549,-14.3241731099825,
114.452036264826)) ;
#181199=CARTESIAN_POINT('Ctrl Pts',(-20.9990323450195,-14.3241731345496,
114.476267351848)) ;
#181200=CARTESIAN_POINT('Ctrl Pts',(-20.98836610951,-14.3919407164252,114.443779720514)) ;
#181201=CARTESIAN_POINT('Ctrl Pts',(-20.9776998740006,-14.4597082983009,
114.41129208918)) ;
#181202=CARTESIAN_POINT('Ctrl Pts',(-21.051503702536,-14.4597082737338,
114.387061002158)) ;
#181203=CARTESIAN_POINT('Ctrl Pts',(-21.1253075310714,-14.4597082491667,
114.362829915136)) ;
#181204=CARTESIAN_POINT('Ctrl Pts',(-21.1359737665809,-14.3919406672911,
114.39531754647)) ;
#181205=CARTESIAN_POINT('Ctrl Pts',(-21.211254131552,-14.4855253459423,
114.659978503316)) ;
#181206=CARTESIAN_POINT('Ctrl Pts',(-21.215947932786,-14.4111261442654,
114.674275063348)) ;
#181207=CARTESIAN_POINT('Ctrl Pts',(-21.142144108098,-14.4111261567896,
114.698506162089)) ;
#181208=CARTESIAN_POINT('Ctrl Pts',(-21.0683402834099,-14.4111261693137,
114.722737260829)) ;
#181209=CARTESIAN_POINT('Ctrl Pts',(-21.0636464821759,-14.4855253709906,
114.708440700797)) ;
#181210=CARTESIAN_POINT('Ctrl Pts',(-21.058952680942,-14.5599245726675,
114.694144140765)) ;
#181211=CARTESIAN_POINT('Ctrl Pts',(-21.13275650563,-14.5599245601434,114.669913042024)) ;
#181212=CARTESIAN_POINT('Ctrl Pts',(-21.206560330318,-14.5599245476192,
114.645681943284)) ;
#181213=CARTESIAN_POINT('Ctrl Pts',(-21.211254131552,-14.4855253459423,
114.659978503316)) ;
#181214=CARTESIAN_POINT('Ctrl Pts',(-21.2915339470349,-14.5029122651219,
114.940022641269)) ;
#181215=CARTESIAN_POINT('Ctrl Pts',(-21.2898945125984,-14.4271913157213,
114.935029187143)) ;
#181216=CARTESIAN_POINT('Ctrl Pts',(-21.2160906909928,-14.4271913111352,
114.959260295272)) ;
#181217=CARTESIAN_POINT('Ctrl Pts',(-21.1422868693872,-14.427191306549,
114.983491403401)) ;
#181218=CARTESIAN_POINT('Ctrl Pts',(-21.1439263038237,-14.5029122559496,
114.988484857527)) ;
#181219=CARTESIAN_POINT('Ctrl Pts',(-21.1455657382602,-14.5786332053501,
114.993478311653)) ;
#181220=CARTESIAN_POINT('Ctrl Pts',(-21.2193695598658,-14.5786332099363,
114.969247203524)) ;
#181221=CARTESIAN_POINT('Ctrl Pts',(-21.2931733814714,-14.5786332145224,
114.945016095395)) ;
#181222=CARTESIAN_POINT('Ctrl Pts',(-21.2915339470349,-14.5029122651219,
114.940022641269)) ;
#181223=CARTESIAN_POINT('Ctrl Pts',(-21.3695938610987,-14.4429567945224,
115.213104290298)) ;
#181224=CARTESIAN_POINT('Ctrl Pts',(-21.3617712091174,-14.3713125211074,
115.189277753062)) ;
#181225=CARTESIAN_POINT('Ctrl Pts',(-21.2879673882971,-14.3713124959872,
115.213508863583)) ;
#181226=CARTESIAN_POINT('Ctrl Pts',(-21.2141635674768,-14.371312470867,
115.237739974103)) ;
#181227=CARTESIAN_POINT('Ctrl Pts',(-21.2219862194581,-14.4429567442819,
115.261566511339)) ;
#181228=CARTESIAN_POINT('Ctrl Pts',(-21.2298088714394,-14.5146010176969,
115.285393048575)) ;
#181229=CARTESIAN_POINT('Ctrl Pts',(-21.3036126922597,-14.5146010428171,
115.261161938054)) ;
#181230=CARTESIAN_POINT('Ctrl Pts',(-21.37741651308,-14.5146010679373,115.236930827533)) ;
#181231=CARTESIAN_POINT('Ctrl Pts',(-21.3695938610987,-14.4429567945224,
115.213104290298)) ;
#181232=CARTESIAN_POINT('Ctrl Pts',(-21.4400444498509,-14.3088313127917,
115.463288416723)) ;
#181233=CARTESIAN_POINT('Ctrl Pts',(-21.4265550909516,-14.2464468463962,
115.422202004376)) ;
#181234=CARTESIAN_POINT('Ctrl Pts',(-21.352751269324,-14.2464467981566,
115.446433112437)) ;
#181235=CARTESIAN_POINT('Ctrl Pts',(-21.2789474476964,-14.2464467499169,
115.470664220499)) ;
#181236=CARTESIAN_POINT('Ctrl Pts',(-21.2924368065957,-14.3088312163124,
115.511750632847)) ;
#181237=CARTESIAN_POINT('Ctrl Pts',(-21.3059261654949,-14.3712156827079,
115.552837045195)) ;
#181238=CARTESIAN_POINT('Ctrl Pts',(-21.3797299871225,-14.3712157309476,
115.528605937133)) ;
#181239=CARTESIAN_POINT('Ctrl Pts',(-21.4535338087501,-14.3712157791872,
115.504374829071)) ;
#181240=CARTESIAN_POINT('Ctrl Pts',(-21.4400444498509,-14.3088313127917,
115.463288416723)) ;
#181241=CARTESIAN_POINT('Ctrl Pts',(-21.4961500025639,-14.1118280044828,
115.669548634659)) ;
#181242=CARTESIAN_POINT('Ctrl Pts',(-21.4779920712133,-14.0631071534286,
115.614242503785)) ;
#181243=CARTESIAN_POINT('Ctrl Pts',(-21.4041882459561,-14.0631070839309,
115.638473600791)) ;
#181244=CARTESIAN_POINT('Ctrl Pts',(-21.3303844206988,-14.0631070144332,
115.662704697798)) ;
#181245=CARTESIAN_POINT('Ctrl Pts',(-21.3485423520494,-14.1118278654874,
115.718010828672)) ;
#181246=CARTESIAN_POINT('Ctrl Pts',(-21.3667002834,-14.1605487165416,115.773316959545)) ;
#181247=CARTESIAN_POINT('Ctrl Pts',(-21.4405041086572,-14.1605487860393,
115.749085862539)) ;
#181248=CARTESIAN_POINT('Ctrl Pts',(-21.5143079339144,-14.160548855537,
115.724854765532)) ;
#181249=CARTESIAN_POINT('Ctrl Pts',(-21.4961500025639,-14.1118280044828,
115.669548634659)) ;
#181250=CARTESIAN_POINT('Ctrl Pts',(-21.5338004050003,-13.8633524569287,
115.819871913818)) ;
#181251=CARTESIAN_POINT('Ctrl Pts',(-21.5122496905878,-13.8319077248758,
115.754231913034)) ;
#181252=CARTESIAN_POINT('Ctrl Pts',(-21.4384458597035,-13.8319076363894,
115.778462992901)) ;
#181253=CARTESIAN_POINT('Ctrl Pts',(-21.3646420288192,-13.8319075479029,
115.802694072769)) ;
#181254=CARTESIAN_POINT('Ctrl Pts',(-21.3861927432316,-13.8633522799557,
115.868334073552)) ;
#181255=CARTESIAN_POINT('Ctrl Pts',(-21.407743457644,-13.8947970120086,
115.933974074336)) ;
#181256=CARTESIAN_POINT('Ctrl Pts',(-21.4815472885284,-13.894797100495,
115.909742994468)) ;
#181257=CARTESIAN_POINT('Ctrl Pts',(-21.5553511194127,-13.8947971889815,
115.885511914601)) ;
#181258=CARTESIAN_POINT('Ctrl Pts',(-21.5338004050003,-13.8633524569287,
115.819871913818)) ;
#181259=CARTESIAN_POINT('Ctrl Pts',(-21.5489972331909,-13.5856086171591,
115.901434129162)) ;
#181260=CARTESIAN_POINT('Ctrl Pts',(-21.5256242740484,-13.5735093381459,
115.830243864882)) ;
#181261=CARTESIAN_POINT('Ctrl Pts',(-21.4518204355535,-13.5735092387167,
115.854474921568)) ;
#181262=CARTESIAN_POINT('Ctrl Pts',(-21.3780165970586,-13.5735091392875,
115.878705978255)) ;
#181263=CARTESIAN_POINT('Ctrl Pts',(-21.401389556201,-13.5856084183006,
115.949896242535)) ;
#181264=CARTESIAN_POINT('Ctrl Pts',(-21.4247625153435,-13.5977076973138,
116.021086506816)) ;
#181265=CARTESIAN_POINT('Ctrl Pts',(-21.4985663538384,-13.597707796743,
115.996855450129)) ;
#181266=CARTESIAN_POINT('Ctrl Pts',(-21.5723701923333,-13.5977078961722,
115.972624393442)) ;
#181267=CARTESIAN_POINT('Ctrl Pts',(-21.5489972331909,-13.5856086171591,
115.901434129162)) ;
#181268=CARTESIAN_POINT('Ctrl Pts',(-21.540363783719,-13.29429050433,115.910632149051)) ;
#181269=CARTESIAN_POINT('Ctrl Pts',(-21.5168248652678,-13.3025120940468,
115.838936399422)) ;
#181270=CARTESIAN_POINT('Ctrl Pts',(-21.4430210182317,-13.3025119902988,
115.863167430093)) ;
#181271=CARTESIAN_POINT('Ctrl Pts',(-21.3692171711956,-13.3025118865508,
115.887398460765)) ;
#181272=CARTESIAN_POINT('Ctrl Pts',(-21.3927560896468,-13.294290296834,
115.959094210394)) ;
#181273=CARTESIAN_POINT('Ctrl Pts',(-21.4162950080979,-13.2860687071171,
116.030789960024)) ;
#181274=CARTESIAN_POINT('Ctrl Pts',(-21.4900988551341,-13.2860688108651,
116.006558929353)) ;
#181275=CARTESIAN_POINT('Ctrl Pts',(-21.5639027021702,-13.2860689146131,
115.982327898681)) ;
#181276=CARTESIAN_POINT('Ctrl Pts',(-21.540363783719,-13.29429050433,115.910632149051)) ;
#181277=CARTESIAN_POINT('Ctrl Pts',(-21.5075688559681,-13.0122145331766,
115.846182232389)) ;
#181278=CARTESIAN_POINT('Ctrl Pts',(-21.4855516918688,-13.0401416634717,
115.779121500935)) ;
#181279=CARTESIAN_POINT('Ctrl Pts',(-21.4117478360689,-13.0401415643198,
115.803352504913)) ;
#181280=CARTESIAN_POINT('Ctrl Pts',(-21.3379439802689,-13.0401414651678,
115.827583508891)) ;
#181281=CARTESIAN_POINT('Ctrl Pts',(-21.3599611443683,-13.0122143348728,
115.894644240346)) ;
#181282=CARTESIAN_POINT('Ctrl Pts',(-21.3819783084676,-12.9842872045777,
115.9617049718)) ;
#181283=CARTESIAN_POINT('Ctrl Pts',(-21.4557821642676,-12.9842873037296,
115.937473967822)) ;
#181284=CARTESIAN_POINT('Ctrl Pts',(-21.5295860200675,-12.9842874028816,
115.913242963844)) ;
#181285=CARTESIAN_POINT('Ctrl Pts',(-21.5075688559681,-13.0122145331766,
115.846182232389)) ;
#181286=CARTESIAN_POINT('Ctrl Pts',(-21.4520578760768,-12.7583429519339,
115.712662082996)) ;
#181287=CARTESIAN_POINT('Ctrl Pts',(-21.4331479501616,-12.8040356004971,
115.65506549767)) ;
#181288=CARTESIAN_POINT('Ctrl Pts',(-21.3593440862728,-12.8040355143443,
115.679296477011)) ;
#181289=CARTESIAN_POINT('Ctrl Pts',(-21.2855402223839,-12.8040354281915,
115.703527456352)) ;
#181290=CARTESIAN_POINT('Ctrl Pts',(-21.3044501482991,-12.7583427796283,
115.761124041677)) ;
#181291=CARTESIAN_POINT('Ctrl Pts',(-21.3233600742142,-12.7126501310651,
115.818720627003)) ;
#181292=CARTESIAN_POINT('Ctrl Pts',(-21.3971639381031,-12.7126502172179,
115.794489647662)) ;
#181293=CARTESIAN_POINT('Ctrl Pts',(-21.4709678019919,-12.7126503033707,
115.770258668321)) ;
#181294=CARTESIAN_POINT('Ctrl Pts',(-21.4520578760768,-12.7583429519339,
115.712662082996)) ;
#181295=CARTESIAN_POINT('Ctrl Pts',(-21.377127791228,-12.5522896132778,
115.51996437081)) ;
#181296=CARTESIAN_POINT('Ctrl Pts',(-21.3626860354123,-12.6124359304363,
115.475977110671)) ;
#181297=CARTESIAN_POINT('Ctrl Pts',(-21.2888821651091,-12.6124358649261,
115.500208070475)) ;
#181298=CARTESIAN_POINT('Ctrl Pts',(-21.2150782948059,-12.6124357994159,
115.524439030279)) ;
#181299=CARTESIAN_POINT('Ctrl Pts',(-21.2295200506216,-12.5522894822574,
115.568426290417)) ;
#181300=CARTESIAN_POINT('Ctrl Pts',(-21.2439618064373,-12.4921431650989,
115.612413550556)) ;
#181301=CARTESIAN_POINT('Ctrl Pts',(-21.3177656767405,-12.4921432306091,
115.588182590752)) ;
#181302=CARTESIAN_POINT('Ctrl Pts',(-21.3915695470436,-12.4921432961193,
115.563951630948)) ;
#181303=CARTESIAN_POINT('Ctrl Pts',(-21.377127791228,-12.5522896132778,
115.51996437081)) ;
#181304=CARTESIAN_POINT('Ctrl Pts',(-21.2880636112646,-12.4090180636989,
115.283992249369)) ;
#181305=CARTESIAN_POINT('Ctrl Pts',(-21.2790882199127,-12.4792560944464,
115.256654653408)) ;
#181306=CARTESIAN_POINT('Ctrl Pts',(-21.2052843453941,-12.4792560544209,
115.280885600373)) ;
#181307=CARTESIAN_POINT('Ctrl Pts',(-21.1314804708756,-12.4792560143955,
115.305116547337)) ;
#181308=CARTESIAN_POINT('Ctrl Pts',(-21.1404558622274,-12.409017983648,
115.332454143298)) ;
#181309=CARTESIAN_POINT('Ctrl Pts',(-21.1494312535792,-12.3387799529005,
115.359791739258)) ;
#181310=CARTESIAN_POINT('Ctrl Pts',(-21.2232351280978,-12.3387799929259,
115.335560792294)) ;
#181311=CARTESIAN_POINT('Ctrl Pts',(-21.2970390026164,-12.3387800329514,
115.31132984533)) ;
#181312=CARTESIAN_POINT('Ctrl Pts',(-21.2880636112646,-12.4090180636989,
115.283992249369)) ;
#181313=CARTESIAN_POINT('Ctrl Pts',(-21.1893528871873,-12.3371174607651,
115.018865437518)) ;
#181314=CARTESIAN_POINT('Ctrl Pts',(-21.1865205563104,-12.4124801362831,
115.010238612627)) ;
#181315=CARTESIAN_POINT('Ctrl Pts',(-21.1127166802678,-12.4124801245382,
115.03446955495)) ;
#181316=CARTESIAN_POINT('Ctrl Pts',(-21.0389128042251,-12.4124801127933,
115.058700497272)) ;
#181317=CARTESIAN_POINT('Ctrl Pts',(-21.041745135102,-12.3371174372753,
115.067327322162)) ;
#181318=CARTESIAN_POINT('Ctrl Pts',(-21.0445774659788,-12.2617547617574,
115.075954147053)) ;
#181319=CARTESIAN_POINT('Ctrl Pts',(-21.1183813420215,-12.2617547735023,
115.05172320473)) ;
#181320=CARTESIAN_POINT('Ctrl Pts',(-21.1921852180641,-12.2617547852472,
115.027492262408)) ;
#181321=CARTESIAN_POINT('Ctrl Pts',(-21.1893528871873,-12.3371174607651,
115.018865437518)) ;
#181322=CARTESIAN_POINT('Ctrl Pts',(-21.0881345102603,-12.3428658905722,
114.745994676073)) ;
#181323=CARTESIAN_POINT('Ctrl Pts',(-21.0916317451865,-12.4179397314328,
114.756646687407)) ;
#181324=CARTESIAN_POINT('Ctrl Pts',(-21.0178278702962,-12.4179397474679,
114.780877633239)) ;
#181325=CARTESIAN_POINT('Ctrl Pts',(-20.9440239954059,-12.4179397635031,
114.805108579071)) ;
#181326=CARTESIAN_POINT('Ctrl Pts',(-20.9405267604797,-12.3428659226425,
114.794456567738)) ;
#181327=CARTESIAN_POINT('Ctrl Pts',(-20.9370295255536,-12.267792081782,
114.783804556404)) ;
#181328=CARTESIAN_POINT('Ctrl Pts',(-21.0108334004439,-12.2677920657468,
114.759573610572)) ;
#181329=CARTESIAN_POINT('Ctrl Pts',(-21.0846372753342,-12.2677920497116,
114.73534266474)) ;
#181330=CARTESIAN_POINT('Ctrl Pts',(-21.0881345102603,-12.3428658905722,
114.745994676073)) ;
#181331=CARTESIAN_POINT('Ctrl Pts',(-20.9904482281693,-12.4257351119528,
114.483961462618)) ;
#181332=CARTESIAN_POINT('Ctrl Pts',(-21.000036278797,-12.4951358678153,
114.513165115915)) ;
#181333=CARTESIAN_POINT('Ctrl Pts',(-20.9262324076312,-12.4951359082695,
114.537396073091)) ;
#181334=CARTESIAN_POINT('Ctrl Pts',(-20.8524285364653,-12.4951359487237,
114.561627030267)) ;
#181335=CARTESIAN_POINT('Ctrl Pts',(-20.8428404858377,-12.4257351928613,
114.532423376971)) ;
#181336=CARTESIAN_POINT('Ctrl Pts',(-20.8332524352101,-12.3563344369988,
114.503219723674)) ;
#181337=CARTESIAN_POINT('Ctrl Pts',(-20.9070563063759,-12.3563343965446,
114.478988766498)) ;
#181338=CARTESIAN_POINT('Ctrl Pts',(-20.9808601775417,-12.3563343560904,
114.454757809322)) ;
#181339=CARTESIAN_POINT('Ctrl Pts',(-20.9904482281693,-12.4257351119528,
114.483961462618)) ;
#181340=CARTESIAN_POINT('Ctrl Pts',(-20.9030223342738,-12.5790185234623,
114.253042471409)) ;
#181341=CARTESIAN_POINT('Ctrl Pts',(-20.9179968510548,-12.6378213476739,
114.298652431594)) ;
#181342=CARTESIAN_POINT('Ctrl Pts',(-20.8441929853562,-12.6378214074388,
114.322883405423)) ;
#181343=CARTESIAN_POINT('Ctrl Pts',(-20.7703891196576,-12.6378214672038,
114.347114379252)) ;
#181344=CARTESIAN_POINT('Ctrl Pts',(-20.7554146028766,-12.5790186429921,
114.301504419066)) ;
#181345=CARTESIAN_POINT('Ctrl Pts',(-20.7404400860955,-12.5202158187805,
114.255894458881)) ;
#181346=CARTESIAN_POINT('Ctrl Pts',(-20.8142439517941,-12.5202157590156,
114.231663485053)) ;
#181347=CARTESIAN_POINT('Ctrl Pts',(-20.8880478174927,-12.5202156992507,
114.207432511224)) ;
#181348=CARTESIAN_POINT('Ctrl Pts',(-20.9030223342738,-12.5790185234623,
114.253042471409)) ;
#181349=CARTESIAN_POINT('Ctrl Pts',(-20.8305192061514,-12.7940406828703,
114.067860324909)) ;
#181350=CARTESIAN_POINT('Ctrl Pts',(-20.8498407335462,-12.837920143464,
114.12671057818)) ;
#181351=CARTESIAN_POINT('Ctrl Pts',(-20.7760368749615,-12.8379202140664,
114.150941573677)) ;
#181352=CARTESIAN_POINT('Ctrl Pts',(-20.7022330163768,-12.8379202846688,
114.175172569173)) ;
#181353=CARTESIAN_POINT('Ctrl Pts',(-20.6829114889821,-12.7940408240752,
114.116322315902)) ;
#181354=CARTESIAN_POINT('Ctrl Pts',(-20.6635899615873,-12.7501613634815,
114.057472062632)) ;
#181355=CARTESIAN_POINT('Ctrl Pts',(-20.7373938201719,-12.7501612928791,
114.033241067135)) ;
#181356=CARTESIAN_POINT('Ctrl Pts',(-20.8111976787566,-12.7501612222767,
114.009010071638)) ;
#181357=CARTESIAN_POINT('Ctrl Pts',(-20.8305192061514,-12.7940406828703,
114.067860324909)) ;
#181358=CARTESIAN_POINT('Ctrl Pts',(-20.7785061884323,-13.0518842131347,
113.944776920917)) ;
#181359=CARTESIAN_POINT('Ctrl Pts',(-20.8007570400159,-13.0778272755866,
114.012549423138)) ;
#181360=CARTESIAN_POINT('Ctrl Pts',(-20.7269531884297,-13.0778273508396,
114.036780439951)) ;
#181361=CARTESIAN_POINT('Ctrl Pts',(-20.6531493368435,-13.0778274260925,
114.061011456764)) ;
#181362=CARTESIAN_POINT('Ctrl Pts',(-20.6308984852599,-13.0518843636406,
113.993238954542)) ;
#181363=CARTESIAN_POINT('Ctrl Pts',(-20.6086476336763,-13.0259413011886,
113.92546645232)) ;
#181364=CARTESIAN_POINT('Ctrl Pts',(-20.6824514852625,-13.0259412259357,
113.901235435508)) ;
#181365=CARTESIAN_POINT('Ctrl Pts',(-20.7562553368487,-13.0259411506828,
113.877004418695)) ;
#181366=CARTESIAN_POINT('Ctrl Pts',(-20.7785061884323,-13.0518842131347,
113.944776920917)) ;
#181367=CARTESIAN_POINT('Ctrl Pts',(-20.74911735469,-13.3370763555055,113.890776267983)) ;
#181368=CARTESIAN_POINT('Ctrl Pts',(-20.7727189618692,-13.343146769627,
113.96266295396)) ;
#181369=CARTESIAN_POINT('Ctrl Pts',(-20.698915117013,-13.3431468412151,
113.986893991271)) ;
#181370=CARTESIAN_POINT('Ctrl Pts',(-20.6251112721567,-13.3431469128033,
114.011125028582)) ;
#181371=CARTESIAN_POINT('Ctrl Pts',(-20.6015096649775,-13.3370764986818,
113.939238342606)) ;
#181372=CARTESIAN_POINT('Ctrl Pts',(-20.5779080577983,-13.3310060845603,
113.867351656629)) ;
#181373=CARTESIAN_POINT('Ctrl Pts',(-20.6517119026545,-13.3310060129721,
113.843120619318)) ;
#181374=CARTESIAN_POINT('Ctrl Pts',(-20.7255157475108,-13.3310059413839,
113.818889582007)) ;
#181375=CARTESIAN_POINT('Ctrl Pts',(-20.74911735469,-13.3370763555055,113.890776267983)) ;
#181376=CARTESIAN_POINT('Ctrl Pts',(-20.7440079729999,-13.6270297095458,
113.910587476447)) ;
#181377=CARTESIAN_POINT('Ctrl Pts',(-20.767270009811,-13.6128647269904,
113.981439886012)) ;
#181378=CARTESIAN_POINT('Ctrl Pts',(-20.6934661705013,-13.6128647900771,
114.005670940217)) ;
#181379=CARTESIAN_POINT('Ctrl Pts',(-20.6196623311916,-13.6128648531639,
114.029901994422)) ;
#181380=CARTESIAN_POINT('Ctrl Pts',(-20.5964002943804,-13.6270298357193,
113.959049584857)) ;
#181381=CARTESIAN_POINT('Ctrl Pts',(-20.5731382575693,-13.6411948182747,
113.888197175291)) ;
#181382=CARTESIAN_POINT('Ctrl Pts',(-20.646942096879,-13.6411947551879,
113.863966121086)) ;
#181383=CARTESIAN_POINT('Ctrl Pts',(-20.7207459361887,-13.6411946921012,
113.839735066881)) ;
#181384=CARTESIAN_POINT('Ctrl Pts',(-20.7440079729999,-13.6270297095458,
113.910587476447)) ;
#181385=CARTESIAN_POINT('Ctrl Pts',(-20.7628136407268,-13.9038567932623,
114.003478096107)) ;
#181386=CARTESIAN_POINT('Ctrl Pts',(-20.7840611677085,-13.8703419963818,
114.068194633963)) ;
#181387=CARTESIAN_POINT('Ctrl Pts',(-20.7102573321534,-13.8703420447739,
114.092425699604)) ;
#181388=CARTESIAN_POINT('Ctrl Pts',(-20.6364534965982,-13.8703420931661,
114.116656765245)) ;
#181389=CARTESIAN_POINT('Ctrl Pts',(-20.6152059696165,-13.9038568900467,
114.051940227388)) ;
#181390=CARTESIAN_POINT('Ctrl Pts',(-20.5939584426348,-13.9373716869272,
113.987223689532)) ;
#181391=CARTESIAN_POINT('Ctrl Pts',(-20.66776227819,-13.9373716385351,113.962992623891)) ;
#181392=CARTESIAN_POINT('Ctrl Pts',(-20.7415661137451,-13.9373715901429,
113.93876155825)) ;
#181393=CARTESIAN_POINT('Ctrl Pts',(-20.7628136407268,-13.9038567932623,
114.003478096107)) ;
#181394=CARTESIAN_POINT('Ctrl Pts',(-20.8034569028155,-14.1447030861545,
114.162759758855)) ;
#181395=CARTESIAN_POINT('Ctrl Pts',(-20.821164521826,-14.0943210410225,
114.216694308367)) ;
#181396=CARTESIAN_POINT('Ctrl Pts',(-20.7473606880735,-14.0943210744769,
114.240925379498)) ;
#181397=CARTESIAN_POINT('Ctrl Pts',(-20.673556854321,-14.0943211079313,
114.26515645063)) ;
#181398=CARTESIAN_POINT('Ctrl Pts',(-20.6558492353105,-14.1447031530633,
114.211221901118)) ;
#181399=CARTESIAN_POINT('Ctrl Pts',(-20.6381416163,-14.1950851981953,114.157287351607)) ;
#181400=CARTESIAN_POINT('Ctrl Pts',(-20.7119454500525,-14.1950851647409,
114.133056280476)) ;
#181401=CARTESIAN_POINT('Ctrl Pts',(-20.785749283805,-14.1950851312865,
114.108825209344)) ;
#181402=CARTESIAN_POINT('Ctrl Pts',(-20.8034569028155,-14.1447030861545,
114.162759758855)) ;
#181403=CARTESIAN_POINT('Ctrl Pts',(-20.8618372427062,-14.332817774621,
114.375897727997)) ;
#181404=CARTESIAN_POINT('Ctrl Pts',(-20.8747644917741,-14.2692250612684,
114.415272042114)) ;
#181405=CARTESIAN_POINT('Ctrl Pts',(-20.8009606585353,-14.2692250813647,
114.43950311481)) ;
#181406=CARTESIAN_POINT('Ctrl Pts',(-20.7271568252965,-14.269225101461,
114.463734187506)) ;
#181407=CARTESIAN_POINT('Ctrl Pts',(-20.7142295762286,-14.3328178148136,
114.424359873389)) ;
#181408=CARTESIAN_POINT('Ctrl Pts',(-20.7013023271606,-14.3964105281663,
114.384985559272)) ;
#181409=CARTESIAN_POINT('Ctrl Pts',(-20.7751061603994,-14.3964105080699,
114.360754486576)) ;
#181410=CARTESIAN_POINT('Ctrl Pts',(-20.8489099936382,-14.3964104879736,
114.33652341388)) ;
#181411=CARTESIAN_POINT('Ctrl Pts',(-20.8618372427062,-14.332817774621,
114.375897727997)) ;
#181412=CARTESIAN_POINT('Ctrl Pts',(-20.9337388829321,-14.45646682902,114.630435787986)) ;
#181413=CARTESIAN_POINT('Ctrl Pts',(-20.9409299779606,-14.3841439170352,
114.652338702601)) ;
#181414=CARTESIAN_POINT('Ctrl Pts',(-20.8671261432927,-14.3841439249686,
114.676569770944)) ;
#181415=CARTESIAN_POINT('Ctrl Pts',(-20.7933223086247,-14.3841439329019,
114.700800839287)) ;
#181416=CARTESIAN_POINT('Ctrl Pts',(-20.7861312135962,-14.4564668448866,
114.678897924672)) ;
#181417=CARTESIAN_POINT('Ctrl Pts',(-20.7789401185677,-14.5287897568713,
114.656995010056)) ;
#181418=CARTESIAN_POINT('Ctrl Pts',(-20.8527439532357,-14.528789748938,
114.632763941713)) ;
#181419=CARTESIAN_POINT('Ctrl Pts',(-20.9265477879036,-14.5287897410047,
114.60853287337)) ;
#181420=CARTESIAN_POINT('Ctrl Pts',(-20.9337388829321,-14.45646682902,114.630435787986)) ;
#181421=CARTESIAN_POINT('Ctrl Pts',(-21.0127215247643,-14.5053560860543,
114.906444434635)) ;
#181422=CARTESIAN_POINT('Ctrl Pts',(-21.0136752367889,-14.4295100560536,
114.90934928717)) ;
#181423=CARTESIAN_POINT('Ctrl Pts',(-20.9398714000126,-14.4295100560703,
114.933580349091)) ;
#181424=CARTESIAN_POINT('Ctrl Pts',(-20.8660675632364,-14.429510056087,
114.957811411013)) ;
#181425=CARTESIAN_POINT('Ctrl Pts',(-20.8651138512118,-14.5053560860877,
114.954906558478)) ;
#181426=CARTESIAN_POINT('Ctrl Pts',(-20.8641601391871,-14.5812021160883,
114.952001705943)) ;
#181427=CARTESIAN_POINT('Ctrl Pts',(-20.9379639759634,-14.5812021160717,
114.927770644021)) ;
#181428=CARTESIAN_POINT('Ctrl Pts',(-21.0117678127397,-14.581202116055,
114.903539582099)) ;
#181429=CARTESIAN_POINT('Ctrl Pts',(-21.0127215247643,-14.5053560860543,
114.906444434635)) ;
#181430=CARTESIAN_POINT('Ctrl Pts',(-21.0928080257603,-14.4762759602464,
115.185935827809)) ;
#181431=CARTESIAN_POINT('Ctrl Pts',(-21.0874352126605,-14.4023454887856,
115.169571105754)) ;
#181432=CARTESIAN_POINT('Ctrl Pts',(-21.0136313731792,-14.4023454850915,
115.193802159437)) ;
#181433=CARTESIAN_POINT('Ctrl Pts',(-20.9398275336979,-14.4023454813974,
115.218033213119)) ;
#181434=CARTESIAN_POINT('Ctrl Pts',(-20.9452003467976,-14.4762759528582,
115.234397935174)) ;
#181435=CARTESIAN_POINT('Ctrl Pts',(-20.9505731598973,-14.5502064243191,
115.250762657229)) ;
#181436=CARTESIAN_POINT('Ctrl Pts',(-21.0243769993787,-14.5502064280132,
115.226531603546)) ;
#181437=CARTESIAN_POINT('Ctrl Pts',(-21.09818083886,-14.5502064317073,115.202300549864)) ;
#181438=CARTESIAN_POINT('Ctrl Pts',(-21.0928080257603,-14.4762759602464,
115.185935827809)) ;
#181439=CARTESIAN_POINT('Ctrl Pts',(-21.166945453464,-14.3712943997113,
115.44718234613)) ;
#181440=CARTESIAN_POINT('Ctrl Pts',(-21.1556545074881,-14.3045830394382,
115.412791946338)) ;
#181441=CARTESIAN_POINT('Ctrl Pts',(-21.0818506659481,-14.3045830356426,
115.43702299375)) ;
#181442=CARTESIAN_POINT('Ctrl Pts',(-21.008046824408,-14.3045830318471,
115.461254041162)) ;
#181443=CARTESIAN_POINT('Ctrl Pts',(-21.0193377703839,-14.3712943921201,
115.495644440954)) ;
#181444=CARTESIAN_POINT('Ctrl Pts',(-21.0306287163597,-14.4380057523932,
115.530034840746)) ;
#181445=CARTESIAN_POINT('Ctrl Pts',(-21.1044325578998,-14.4380057561888,
115.505803793334)) ;
#181446=CARTESIAN_POINT('Ctrl Pts',(-21.1782363994398,-14.4380057599843,
115.481572745922)) ;
#181447=CARTESIAN_POINT('Ctrl Pts',(-21.166945453464,-14.3712943997113,
115.44718234613)) ;
#181448=CARTESIAN_POINT('Ctrl Pts',(-21.22925533612,-14.1990455522355,115.672287786187)) ;
#181449=CARTESIAN_POINT('Ctrl Pts',(-21.2128657588445,-14.1442616573657,
115.622367778204)) ;
#181450=CARTESIAN_POINT('Ctrl Pts',(-21.1390619159356,-14.1442616552479,
115.646598821446)) ;
#181451=CARTESIAN_POINT('Ctrl Pts',(-21.0652580730266,-14.1442616531301,
115.670829864688)) ;
#181452=CARTESIAN_POINT('Ctrl Pts',(-21.0816476503021,-14.1990455479999,
115.720749872672)) ;
#181453=CARTESIAN_POINT('Ctrl Pts',(-21.0980372275776,-14.2538294428697,
115.770669880655)) ;
#181454=CARTESIAN_POINT('Ctrl Pts',(-21.1718410704865,-14.2538294449875,
115.746438837413)) ;
#181455=CARTESIAN_POINT('Ctrl Pts',(-21.2456449133955,-14.2538294471053,
115.722207794171)) ;
#181456=CARTESIAN_POINT('Ctrl Pts',(-21.22925533612,-14.1990455522355,115.672287786187)) ;
#181457=CARTESIAN_POINT('Ctrl Pts',(-21.275036309889,-13.969268231171,115.847326008971)) ;
#181458=CARTESIAN_POINT('Ctrl Pts',(-21.2546885946839,-13.9304471194496,
115.785350151579)) ;
#181459=CARTESIAN_POINT('Ctrl Pts',(-21.1808847509395,-13.9304471207081,
115.809581192277)) ;
#181460=CARTESIAN_POINT('Ctrl Pts',(-21.107080907195,-13.9304471219666,
115.833812232975)) ;
#181461=CARTESIAN_POINT('Ctrl Pts',(-21.1274286224002,-13.9692682336881,
115.895788090367)) ;
#181462=CARTESIAN_POINT('Ctrl Pts',(-21.1477763376053,-14.0080893454095,
115.957763947758)) ;
#181463=CARTESIAN_POINT('Ctrl Pts',(-21.2215801813498,-14.008089344151,
115.933532907061)) ;
#181464=CARTESIAN_POINT('Ctrl Pts',(-21.2953840250942,-14.0080893428925,
115.909301866363)) ;
#181465=CARTESIAN_POINT('Ctrl Pts',(-21.275036309889,-13.969268231171,115.847326008971)) ;
#181466=CARTESIAN_POINT('Ctrl Pts',(-21.2996282826531,-13.7012052922517,
115.957629225369)) ;
#181467=CARTESIAN_POINT('Ctrl Pts',(-21.2768004959632,-13.6810448607135,
115.888099470425)) ;
#181468=CARTESIAN_POINT('Ctrl Pts',(-21.2029966522746,-13.6810448639026,
115.912330511293)) ;
#181469=CARTESIAN_POINT('Ctrl Pts',(-21.1291928085861,-13.6810448670916,
115.936561552161)) ;
#181470=CARTESIAN_POINT('Ctrl Pts',(-21.152020595276,-13.7012052986298,
116.006091307105)) ;
#181471=CARTESIAN_POINT('Ctrl Pts',(-21.174848381966,-13.7213657301679,
116.075621062049)) ;
#181472=CARTESIAN_POINT('Ctrl Pts',(-21.2486522256545,-13.7213657269789,
116.051390021181)) ;
#181473=CARTESIAN_POINT('Ctrl Pts',(-21.3224560693431,-13.7213657237898,
116.027158980313)) ;
#181474=CARTESIAN_POINT('Ctrl Pts',(-21.2996282826531,-13.7012052922517,
115.957629225369)) ;
#181475=CARTESIAN_POINT('Ctrl Pts',(-21.300776790549,-13.4115854195081,
115.996699140416)) ;
#181476=CARTESIAN_POINT('Ctrl Pts',(-21.2770987495347,-13.4116194662379,
115.924579647977)) ;
#181477=CARTESIAN_POINT('Ctrl Pts',(-21.20329490617,-13.4116194689939,115.948810689832)) ;
#181478=CARTESIAN_POINT('Ctrl Pts',(-21.1294910628053,-13.41161947175,115.973041731686)) ;
#181479=CARTESIAN_POINT('Ctrl Pts',(-21.1531691038196,-13.4115854250202,
116.045161224125)) ;
#181480=CARTESIAN_POINT('Ctrl Pts',(-21.176847144834,-13.4115513782904,
116.117280716563)) ;
#181481=CARTESIAN_POINT('Ctrl Pts',(-21.2506509881987,-13.4115513755344,
116.093049674709)) ;
#181482=CARTESIAN_POINT('Ctrl Pts',(-21.3244548315633,-13.4115513727784,
116.068818632855)) ;
#181483=CARTESIAN_POINT('Ctrl Pts',(-21.300776790549,-13.4115854195081,
115.996699140416)) ;
#181484=CARTESIAN_POINT('Ctrl Pts',(-21.2776657782434,-13.1240520278943,
115.961667884177)) ;
#181485=CARTESIAN_POINT('Ctrl Pts',(-21.2548350128594,-13.1441635924048,
115.892129056556)) ;
#181486=CARTESIAN_POINT('Ctrl Pts',(-21.1810311695779,-13.144163592711,
115.916360098664)) ;
#181487=CARTESIAN_POINT('Ctrl Pts',(-21.1072273262965,-13.1441635930171,
115.940591140771)) ;
#181488=CARTESIAN_POINT('Ctrl Pts',(-21.1300580916804,-13.1240520285066,
116.010129968393)) ;
#181489=CARTESIAN_POINT('Ctrl Pts',(-21.1528888570643,-13.103940463996,
116.079668796014)) ;
#181490=CARTESIAN_POINT('Ctrl Pts',(-21.2266927003458,-13.1039404636899,
116.055437753906)) ;
#181491=CARTESIAN_POINT('Ctrl Pts',(-21.3004965436273,-13.1039404633837,
116.031206711798)) ;
#181492=CARTESIAN_POINT('Ctrl Pts',(-21.2776657782434,-13.1240520278943,
115.961667884177)) ;
#181493=CARTESIAN_POINT('Ctrl Pts',(-21.2310997495999,-12.8565945311091,
115.85532524094)) ;
#181494=CARTESIAN_POINT('Ctrl Pts',(-21.2107526317274,-12.895411134357,
115.79335120282)) ;
#181495=CARTESIAN_POINT('Ctrl Pts',(-21.1369487878002,-12.8954111308149,
115.817582242961)) ;
#181496=CARTESIAN_POINT('Ctrl Pts',(-21.0631449438729,-12.8954111272728,
115.841813283102)) ;
#181497=CARTESIAN_POINT('Ctrl Pts',(-21.0834920617454,-12.8565945240249,
115.903787321221)) ;
#181498=CARTESIAN_POINT('Ctrl Pts',(-21.1038391796179,-12.817777920777,
115.965761359341)) ;
#181499=CARTESIAN_POINT('Ctrl Pts',(-21.1776430235452,-12.8177779243191,
115.9415303192)) ;
#181500=CARTESIAN_POINT('Ctrl Pts',(-21.2514468674724,-12.8177779278612,
115.917299279059)) ;
#181501=CARTESIAN_POINT('Ctrl Pts',(-21.2310997495999,-12.8565945311091,
115.85532524094)) ;
#181502=CARTESIAN_POINT('Ctrl Pts',(-21.1639038965067,-12.6299321000607,
115.686042104693)) ;
#181503=CARTESIAN_POINT('Ctrl Pts',(-21.1474868349835,-12.6846316848106,
115.636038384002)) ;
#181504=CARTESIAN_POINT('Ctrl Pts',(-21.0736829896652,-12.6846316781894,
115.660269419906)) ;
#181505=CARTESIAN_POINT('Ctrl Pts',(-20.9998791443469,-12.6846316715683,
115.68450045581)) ;
#181506=CARTESIAN_POINT('Ctrl Pts',(-21.0162962058702,-12.6299320868185,
115.7345041765)) ;
#181507=CARTESIAN_POINT('Ctrl Pts',(-21.0327132673934,-12.5752325020687,
115.784507897191)) ;
#181508=CARTESIAN_POINT('Ctrl Pts',(-21.1065171127117,-12.5752325086898,
115.760276861287)) ;
#181509=CARTESIAN_POINT('Ctrl Pts',(-21.18032095803,-12.5752325153109,115.736045825383)) ;
#181510=CARTESIAN_POINT('Ctrl Pts',(-21.1639038965067,-12.6299321000607,
115.686042104693)) ;
#181511=CARTESIAN_POINT('Ctrl Pts',(-21.0795308737286,-12.458754218581,
115.464633703423)) ;
#181512=CARTESIAN_POINT('Ctrl Pts',(-21.0682449006004,-12.5254858902144,
115.430258449939)) ;
#181513=CARTESIAN_POINT('Ctrl Pts',(-20.9944410527263,-12.5254858817945,
115.454489478058)) ;
#181514=CARTESIAN_POINT('Ctrl Pts',(-20.9206372048521,-12.5254858733746,
115.478720506177)) ;
#181515=CARTESIAN_POINT('Ctrl Pts',(-20.9319231779803,-12.4587542017412,
115.513095759661)) ;
#181516=CARTESIAN_POINT('Ctrl Pts',(-20.9432091511085,-12.3920225301078,
115.547471013146)) ;
#181517=CARTESIAN_POINT('Ctrl Pts',(-21.0170129989826,-12.3920225385277,
115.523239985027)) ;
#181518=CARTESIAN_POINT('Ctrl Pts',(-21.0908168468568,-12.3920225469476,
115.499008956907)) ;
#181519=CARTESIAN_POINT('Ctrl Pts',(-21.0795308737286,-12.458754218581,
115.464633703423)) ;
#181520=CARTESIAN_POINT('Ctrl Pts',(-20.9840008114821,-12.3569969390507,
115.209096703892)) ;
#181521=CARTESIAN_POINT('Ctrl Pts',(-20.978635400475,-12.4309301429408,
115.192754527206)) ;
#181522=CARTESIAN_POINT('Ctrl Pts',(-20.9048315498076,-12.4309301369064,
115.216985546818)) ;
#181523=CARTESIAN_POINT('Ctrl Pts',(-20.8310276991402,-12.430930130872,
115.241216566429)) ;
#181524=CARTESIAN_POINT('Ctrl Pts',(-20.8363931101473,-12.356996926982,
115.257558743115)) ;
#181525=CARTESIAN_POINT('Ctrl Pts',(-20.8417585211544,-12.283063723092,
115.273900919801)) ;
#181526=CARTESIAN_POINT('Ctrl Pts',(-20.9155623718218,-12.2830637291264,
115.249669900189)) ;
#181527=CARTESIAN_POINT('Ctrl Pts',(-20.9893662224891,-12.2830637351607,
115.225438880578)) ;
#181528=CARTESIAN_POINT('Ctrl Pts',(-20.9840008114821,-12.3569969390507,
115.209096703892)) ;
#181529=CARTESIAN_POINT('Ctrl Pts',(-20.8827940549326,-12.3311725454961,
114.936383442419)) ;
#181530=CARTESIAN_POINT('Ctrl Pts',(-20.8837517075036,-12.4070160661621,
114.939300296995)) ;
#181531=CARTESIAN_POINT('Ctrl Pts',(-20.8099478537991,-12.4070160669481,
114.963531307356)) ;
#181532=CARTESIAN_POINT('Ctrl Pts',(-20.7361440000946,-12.4070160677341,
114.987762317717)) ;
#181533=CARTESIAN_POINT('Ctrl Pts',(-20.7351863475235,-12.3311725470681,
114.984845463141)) ;
#181534=CARTESIAN_POINT('Ctrl Pts',(-20.7342286949525,-12.2553290264021,
114.981928608564)) ;
#181535=CARTESIAN_POINT('Ctrl Pts',(-20.808032548657,-12.2553290256161,
114.957697598203)) ;
#181536=CARTESIAN_POINT('Ctrl Pts',(-20.8818364023615,-12.2553290248301,
114.933466587842)) ;
#181537=CARTESIAN_POINT('Ctrl Pts',(-20.8827940549326,-12.3311725454961,
114.936383442419)) ;
#181538=CARTESIAN_POINT('Ctrl Pts',(-20.7831194155453,-12.3830921654557,
114.668177530527)) ;
#181539=CARTESIAN_POINT('Ctrl Pts',(-20.7903054822259,-12.4554200435771,
114.690065129378)) ;
#181540=CARTESIAN_POINT('Ctrl Pts',(-20.716501626603,-12.4554200554495,
114.714296133896)) ;
#181541=CARTESIAN_POINT('Ctrl Pts',(-20.6426977709801,-12.4554200673219,
114.738527138414)) ;
#181542=CARTESIAN_POINT('Ctrl Pts',(-20.6355117042995,-12.3830921892004,
114.716639539563)) ;
#181543=CARTESIAN_POINT('Ctrl Pts',(-20.6283256376189,-12.310764311079,
114.694751940711)) ;
#181544=CARTESIAN_POINT('Ctrl Pts',(-20.7021294932418,-12.3107642992066,
114.670520936193)) ;
#181545=CARTESIAN_POINT('Ctrl Pts',(-20.7759333488647,-12.3107642873342,
114.646289931676)) ;
#181546=CARTESIAN_POINT('Ctrl Pts',(-20.7831194155453,-12.3830921654557,
114.668177530527)) ;
#181547=CARTESIAN_POINT('Ctrl Pts',(-20.6905057252182,-12.5097082549453,
114.421659452315)) ;
#181548=CARTESIAN_POINT('Ctrl Pts',(-20.7034324595095,-12.5733006688363,
114.461032198267)) ;
#181549=CARTESIAN_POINT('Ctrl Pts',(-20.6296286028042,-12.5733006960963,
114.485263199488)) ;
#181550=CARTESIAN_POINT('Ctrl Pts',(-20.555824746099,-12.5733007233563,
114.509494200709)) ;
#181551=CARTESIAN_POINT('Ctrl Pts',(-20.5428980118077,-12.5097083094653,
114.470121454757)) ;
#181552=CARTESIAN_POINT('Ctrl Pts',(-20.5299712775163,-12.4461158955744,
114.430748708805)) ;
#181553=CARTESIAN_POINT('Ctrl Pts',(-20.6037751342216,-12.4461158683144,
114.406517707584)) ;
#181554=CARTESIAN_POINT('Ctrl Pts',(-20.6775789909268,-12.4461158410544,
114.382286706363)) ;
#181555=CARTESIAN_POINT('Ctrl Pts',(-20.6905057252182,-12.5097082549453,
114.421659452315)) ;
#181556=CARTESIAN_POINT('Ctrl Pts',(-20.611889484645,-12.6999655173835,
114.217488910924)) ;
#181557=CARTESIAN_POINT('Ctrl Pts',(-20.6295936140436,-12.7503658770991,
114.271412831411)) ;
#181558=CARTESIAN_POINT('Ctrl Pts',(-20.5557897586328,-12.7503659198469,
114.295643836575)) ;
#181559=CARTESIAN_POINT('Ctrl Pts',(-20.481985903222,-12.7503659625947,
114.319874841739)) ;
#181560=CARTESIAN_POINT('Ctrl Pts',(-20.4642817738234,-12.699965602879,
114.265950921252)) ;
#181561=CARTESIAN_POINT('Ctrl Pts',(-20.4465776444248,-12.6495652431633,
114.212027000766)) ;
#181562=CARTESIAN_POINT('Ctrl Pts',(-20.5203814998356,-12.6495652004156,
114.187795995602)) ;
#181563=CARTESIAN_POINT('Ctrl Pts',(-20.5941853552464,-12.6495651576678,
114.163564990438)) ;
#181564=CARTESIAN_POINT('Ctrl Pts',(-20.611889484645,-12.6999655173835,
114.217488910924)) ;
#181565=CARTESIAN_POINT('Ctrl Pts',(-20.5509672408573,-12.9431519741363,
114.067493771152)) ;
#181566=CARTESIAN_POINT('Ctrl Pts',(-20.5722146237278,-12.9766466266446,
114.132209869832)) ;
#181567=CARTESIAN_POINT('Ctrl Pts',(-20.4984107710343,-12.9766466864281,
114.156440883272)) ;
#181568=CARTESIAN_POINT('Ctrl Pts',(-20.4246069183407,-12.9766467462115,
114.180671896712)) ;
#181569=CARTESIAN_POINT('Ctrl Pts',(-20.4033595354702,-12.9431520937032,
114.115955798032)) ;
#181570=CARTESIAN_POINT('Ctrl Pts',(-20.3821121525996,-12.9096574411949,
114.051239699352)) ;
#181571=CARTESIAN_POINT('Ctrl Pts',(-20.4559160052932,-12.9096573814114,
114.027008685912)) ;
#181572=CARTESIAN_POINT('Ctrl Pts',(-20.5297198579867,-12.9096573216279,
114.002777672472)) ;
#181573=CARTESIAN_POINT('Ctrl Pts',(-20.5509672408573,-12.9431519741363,
114.067493771152)) ;
#181574=CARTESIAN_POINT('Ctrl Pts',(-20.5121852559406,-13.2187420743147,
113.984700488241)) ;
#181575=CARTESIAN_POINT('Ctrl Pts',(-20.535439895788,-13.233044020348,114.055530367671)) ;
#181576=CARTESIAN_POINT('Ctrl Pts',(-20.4616360479609,-13.2330440926295,
114.079761395933)) ;
#181577=CARTESIAN_POINT('Ctrl Pts',(-20.3878322001338,-13.2330441649111,
114.103992424196)) ;
#181578=CARTESIAN_POINT('Ctrl Pts',(-20.3645775602864,-13.2187422188778,
114.033162544766)) ;
#181579=CARTESIAN_POINT('Ctrl Pts',(-20.341322920439,-13.2044402728445,
113.962332665335)) ;
#181580=CARTESIAN_POINT('Ctrl Pts',(-20.4151267682661,-13.204440200563,
113.938101637073)) ;
#181581=CARTESIAN_POINT('Ctrl Pts',(-20.4889306160931,-13.2044401282814,
113.913870608811)) ;
#181582=CARTESIAN_POINT('Ctrl Pts',(-20.5121852559406,-13.2187420743147,
113.984700488241)) ;
#181583=CARTESIAN_POINT('Ctrl Pts',(-20.4971344280026,-13.5111774969548,
113.974526122815)) ;
#181584=CARTESIAN_POINT('Ctrl Pts',(-20.5207357628537,-13.505083397222,
114.046411979112)) ;
#181585=CARTESIAN_POINT('Ctrl Pts',(-20.4469319214645,-13.5050834796266,
114.070643026983)) ;
#181586=CARTESIAN_POINT('Ctrl Pts',(-20.3731280800753,-13.5050835620312,
114.094874074854)) ;
#181587=CARTESIAN_POINT('Ctrl Pts',(-20.3495267452242,-13.511177661764,
114.022988218557)) ;
#181588=CARTESIAN_POINT('Ctrl Pts',(-20.3259254103731,-13.5172717614969,
113.95110236226)) ;
#181589=CARTESIAN_POINT('Ctrl Pts',(-20.3997292517623,-13.5172716790923,
113.926871314389)) ;
#181590=CARTESIAN_POINT('Ctrl Pts',(-20.4735330931515,-13.5172715966877,
113.902640266518)) ;
#181591=CARTESIAN_POINT('Ctrl Pts',(-20.4971344280026,-13.5111774969548,
113.974526122815)) ;
#181592=CARTESIAN_POINT('Ctrl Pts',(-20.5063387268511,-13.7940494918521,
114.037849430853)) ;
#181593=CARTESIAN_POINT('Ctrl Pts',(-20.5286013967457,-13.7681973144643,
114.105657929582)) ;
#181594=CARTESIAN_POINT('Ctrl Pts',(-20.4547975626805,-13.7681973972875,
114.129888999761)) ;
#181595=CARTESIAN_POINT('Ctrl Pts',(-20.3809937286154,-13.7681974801107,
114.15412006994)) ;
#181596=CARTESIAN_POINT('Ctrl Pts',(-20.3587310587208,-13.7940496574985,
114.086311571211)) ;
#181597=CARTESIAN_POINT('Ctrl Pts',(-20.3364683888263,-13.8199018348862,
114.018503072482)) ;
#181598=CARTESIAN_POINT('Ctrl Pts',(-20.4102722228914,-13.819901752063,
113.994272002303)) ;
#181599=CARTESIAN_POINT('Ctrl Pts',(-20.4840760569565,-13.8199016692398,
113.970040932124)) ;
#181600=CARTESIAN_POINT('Ctrl Pts',(-20.5063387268511,-13.7940494918521,
114.037849430853)) ;
#181601=CARTESIAN_POINT('Ctrl Pts',(-20.5386101711866,-14.0529110285333,
114.171842551174)) ;
#181602=CARTESIAN_POINT('Ctrl Pts',(-20.5579137638,-14.0089483158053,114.230638177808)) ;
#181603=CARTESIAN_POINT('Ctrl Pts',(-20.4841099376321,-14.0089483935527,
114.25486927204)) ;
#181604=CARTESIAN_POINT('Ctrl Pts',(-20.4103061114642,-14.0089484713001,
114.279100366273)) ;
#181605=CARTESIAN_POINT('Ctrl Pts',(-20.3910025188508,-14.0529111840282,
114.22030473964)) ;
#181606=CARTESIAN_POINT('Ctrl Pts',(-20.3716989262374,-14.0968738967562,
114.161509113006)) ;
#181607=CARTESIAN_POINT('Ctrl Pts',(-20.4455027524053,-14.0968738190088,
114.137278018774)) ;
#181608=CARTESIAN_POINT('Ctrl Pts',(-20.5193065785732,-14.0968737412614,
114.113046924541)) ;
#181609=CARTESIAN_POINT('Ctrl Pts',(-20.5386101711866,-14.0529110285333,
114.171842551174)) ;
#181610=CARTESIAN_POINT('Ctrl Pts',(-20.5902344604345,-14.2634870650102,
114.364365229605)) ;
#181611=CARTESIAN_POINT('Ctrl Pts',(-20.6052317953266,-14.2047586746315,
114.410044689958)) ;
#181612=CARTESIAN_POINT('Ctrl Pts',(-20.531427975912,-14.2047587372463,
114.43427580476)) ;
#181613=CARTESIAN_POINT('Ctrl Pts',(-20.4576241564973,-14.204758799861,
114.458506919562)) ;
#181614=CARTESIAN_POINT('Ctrl Pts',(-20.4426268216052,-14.2634871902397,
114.412827459209)) ;
#181615=CARTESIAN_POINT('Ctrl Pts',(-20.4276294867131,-14.3222155806184,
114.367147998855)) ;
#181616=CARTESIAN_POINT('Ctrl Pts',(-20.5014333061278,-14.3222155180036,
114.342916884053)) ;
#181617=CARTESIAN_POINT('Ctrl Pts',(-20.5752371255424,-14.3222154553889,
114.318685769251)) ;
#181618=CARTESIAN_POINT('Ctrl Pts',(-20.5902344604345,-14.2634870650102,
114.364365229605)) ;
#181619=CARTESIAN_POINT('Ctrl Pts',(-20.6572920468694,-14.4148461022599,
114.60407461122)) ;
#181620=CARTESIAN_POINT('Ctrl Pts',(-20.6668958738474,-14.3454644446965,
114.633326316629)) ;
#181621=CARTESIAN_POINT('Ctrl Pts',(-20.5930920598847,-14.3454644862781,
114.657557448037)) ;
#181622=CARTESIAN_POINT('Ctrl Pts',(-20.519288245922,-14.3454645278597,
114.681788579445)) ;
#181623=CARTESIAN_POINT('Ctrl Pts',(-20.509684418944,-14.414846185423,114.652536874035)) ;
#181624=CARTESIAN_POINT('Ctrl Pts',(-20.500080591966,-14.4842278429864,
114.623285168626)) ;
#181625=CARTESIAN_POINT('Ctrl Pts',(-20.5738844059287,-14.4842278014048,
114.599054037218)) ;
#181626=CARTESIAN_POINT('Ctrl Pts',(-20.6476882198914,-14.4842277598232,
114.57482290581)) ;
#181627=CARTESIAN_POINT('Ctrl Pts',(-20.6572920468694,-14.4148461022599,
114.60407461122)) ;
#181628=CARTESIAN_POINT('Ctrl Pts',(-20.7340710302273,-14.494780073978,
114.873368689738)) ;
#181629=CARTESIAN_POINT('Ctrl Pts',(-20.7375952932734,-14.4197159016166,
114.88410302429)) ;
#181630=CARTESIAN_POINT('Ctrl Pts',(-20.6637914825865,-14.4197159169921,
114.908334165676)) ;
#181631=CARTESIAN_POINT('Ctrl Pts',(-20.5899876718997,-14.4197159323676,
114.932565307061)) ;
#181632=CARTESIAN_POINT('Ctrl Pts',(-20.5864634088536,-14.4947801047291,
114.921830972509)) ;
#181633=CARTESIAN_POINT('Ctrl Pts',(-20.5829391458075,-14.5698442770905,
114.911096637957)) ;
#181634=CARTESIAN_POINT('Ctrl Pts',(-20.6567429564944,-14.5698442617149,
114.886865496572)) ;
#181635=CARTESIAN_POINT('Ctrl Pts',(-20.7305467671812,-14.5698442463394,
114.862634355187)) ;
#181636=CARTESIAN_POINT('Ctrl Pts',(-20.7340710302273,-14.494780073978,
114.873368689738)) ;
#181637=CARTESIAN_POINT('Ctrl Pts',(-20.814667921946,-14.4974507314962,
115.154444310866)) ;
#181638=CARTESIAN_POINT('Ctrl Pts',(-20.8118340578012,-14.4220890720825,
115.145812815837)) ;
#181639=CARTESIAN_POINT('Ctrl Pts',(-20.7380302478058,-14.4220890586317,
115.170043959328)) ;
#181640=CARTESIAN_POINT('Ctrl Pts',(-20.6642264378103,-14.4220890451809,
115.194275102819)) ;
#181641=CARTESIAN_POINT('Ctrl Pts',(-20.6670603019551,-14.4974507045946,
115.202906597848)) ;
#181642=CARTESIAN_POINT('Ctrl Pts',(-20.6698941660999,-14.5728123640084,
115.211538092878)) ;
#181643=CARTESIAN_POINT('Ctrl Pts',(-20.7436979760954,-14.5728123774592,
115.187306949387)) ;
#181644=CARTESIAN_POINT('Ctrl Pts',(-20.8175017860908,-14.57281239091,115.163075805895)) ;
#181645=CARTESIAN_POINT('Ctrl Pts',(-20.814667921946,-14.4974507314962,
115.154444310866)) ;
#181646=CARTESIAN_POINT('Ctrl Pts',(-20.8916746371351,-14.4229495346006,
115.424337435555)) ;
#181647=CARTESIAN_POINT('Ctrl Pts',(-20.8827289243665,-14.3526782474262,
115.397090235752)) ;
#181648=CARTESIAN_POINT('Ctrl Pts',(-20.8089251121826,-14.3526782058987,
115.421321372578)) ;
#181649=CARTESIAN_POINT('Ctrl Pts',(-20.7351212999988,-14.3526781643712,
115.445552509404)) ;
#181650=CARTESIAN_POINT('Ctrl Pts',(-20.7440670127673,-14.4229494515456,
115.472799709206)) ;
#181651=CARTESIAN_POINT('Ctrl Pts',(-20.7530127255359,-14.49322073872,115.500046909008)) ;
#181652=CARTESIAN_POINT('Ctrl Pts',(-20.8268165377198,-14.4932207802475,
115.475815772183)) ;
#181653=CARTESIAN_POINT('Ctrl Pts',(-20.9006203499037,-14.493220821775,
115.451584635357)) ;
#181654=CARTESIAN_POINT('Ctrl Pts',(-20.8916746371351,-14.4229495346006,
115.424337435555)) ;
#181655=CARTESIAN_POINT('Ctrl Pts',(-20.9596595247132,-14.2768020033666,
115.6668461103)) ;
#181656=CARTESIAN_POINT('Ctrl Pts',(-20.9452208674078,-14.2166300695752,
115.622868287728)) ;
#181657=CARTESIAN_POINT('Ctrl Pts',(-20.8714170505769,-14.2166300030693,
115.647099410399)) ;
#181658=CARTESIAN_POINT('Ctrl Pts',(-20.7976132337459,-14.2166299365633,
115.671330533071)) ;
#181659=CARTESIAN_POINT('Ctrl Pts',(-20.8120518910512,-14.2768018703547,
115.715308355643)) ;
#181660=CARTESIAN_POINT('Ctrl Pts',(-20.8264905483566,-14.336973804146,
115.759286178215)) ;
#181661=CARTESIAN_POINT('Ctrl Pts',(-20.9002943651876,-14.336973870652,
115.735055055544)) ;
#181662=CARTESIAN_POINT('Ctrl Pts',(-20.9740981820186,-14.3369739371579,
115.710823932872)) ;
#181663=CARTESIAN_POINT('Ctrl Pts',(-20.9596595247132,-14.2768020033666,
115.6668461103)) ;
#181664=CARTESIAN_POINT('Ctrl Pts',(-21.012974127338,-14.0672719747909,
115.864923528027)) ;
#181665=CARTESIAN_POINT('Ctrl Pts',(-20.9940531582264,-14.0216384576254,
115.807293306955)) ;
#181666=CARTESIAN_POINT('Ctrl Pts',(-20.9202493344567,-14.0216383725684,
115.831524408492)) ;
#181667=CARTESIAN_POINT('Ctrl Pts',(-20.8464455106869,-14.0216382875114,
115.855755510029)) ;
#181668=CARTESIAN_POINT('Ctrl Pts',(-20.8653664797985,-14.067271804677,
115.913385731101)) ;
#181669=CARTESIAN_POINT('Ctrl Pts',(-20.88428744891,-14.1129053218425,115.971015952173)) ;
#181670=CARTESIAN_POINT('Ctrl Pts',(-20.9580912726798,-14.1129054068995,
115.946784850636)) ;
#181671=CARTESIAN_POINT('Ctrl Pts',(-21.0318950964495,-14.1129054919565,
115.922553749099)) ;
#181672=CARTESIAN_POINT('Ctrl Pts',(-21.012974127338,-14.0672719747909,
115.864923528027)) ;
#181673=CARTESIAN_POINT('Ctrl Pts',(-21.0462752479574,-13.8140437794069,
116.001605423442)) ;
#181674=CARTESIAN_POINT('Ctrl Pts',(-21.0242717527116,-13.786022349902,
115.934586325172)) ;
#181675=CARTESIAN_POINT('Ctrl Pts',(-20.9504679209727,-13.7860222533108,
115.958817402436)) ;
#181676=CARTESIAN_POINT('Ctrl Pts',(-20.8766640892339,-13.7860221567197,
115.983048479701)) ;
#181677=CARTESIAN_POINT('Ctrl Pts',(-20.8986675844797,-13.8140435862246,
116.050067577971)) ;
#181678=CARTESIAN_POINT('Ctrl Pts',(-20.9206710797256,-13.8420650157295,
116.117086676241)) ;
#181679=CARTESIAN_POINT('Ctrl Pts',(-20.9944749114644,-13.8420651123206,
116.092855598977)) ;
#181680=CARTESIAN_POINT('Ctrl Pts',(-21.0682787432033,-13.8420652089118,
116.068624521712)) ;
#181681=CARTESIAN_POINT('Ctrl Pts',(-21.0462752479574,-13.8140437794069,
116.001605423442)) ;
#181682=CARTESIAN_POINT('Ctrl Pts',(-21.057235818105,-13.5305545368903,
116.070529359299)) ;
#181683=CARTESIAN_POINT('Ctrl Pts',(-21.0336987141124,-13.5222834200997,
115.998839136312)) ;
#181684=CARTESIAN_POINT('Ctrl Pts',(-20.9598948737852,-13.5222833210965,
116.023070187418)) ;
#181685=CARTESIAN_POINT('Ctrl Pts',(-20.8860910334581,-13.5222832220932,
116.047301238524)) ;
#181686=CARTESIAN_POINT('Ctrl Pts',(-20.9096281374507,-13.5305543388838,
116.11899146151)) ;
#181687=CARTESIAN_POINT('Ctrl Pts',(-20.9331652414433,-13.5388254556744,
116.190681684497)) ;
#181688=CARTESIAN_POINT('Ctrl Pts',(-21.0069690817705,-13.5388255546776,
116.166450633391)) ;
#181689=CARTESIAN_POINT('Ctrl Pts',(-21.0807729220976,-13.5388256536809,
116.142219582285)) ;
#181690=CARTESIAN_POINT('Ctrl Pts',(-21.057235818105,-13.5305545368903,
116.070529359299)) ;
#181691=CARTESIAN_POINT('Ctrl Pts',(-21.0439982208835,-13.2400469135056,
116.065602507524)) ;
#181692=CARTESIAN_POINT('Ctrl Pts',(-21.0206177244586,-13.2520460162367,
115.994389286006)) ;
#181693=CARTESIAN_POINT('Ctrl Pts',(-20.9468138760363,-13.2520459225966,
116.018620312456)) ;
#181694=CARTESIAN_POINT('Ctrl Pts',(-20.873010027614,-13.2520458289565,
116.042851338905)) ;
#181695=CARTESIAN_POINT('Ctrl Pts',(-20.8963905240389,-13.2400467262255,
116.114064560423)) ;
#181696=CARTESIAN_POINT('Ctrl Pts',(-20.9197710204638,-13.2280476234944,
116.18527778194)) ;
#181697=CARTESIAN_POINT('Ctrl Pts',(-20.9935748688861,-13.2280477171344,
116.161046755491)) ;
#181698=CARTESIAN_POINT('Ctrl Pts',(-21.0673787173084,-13.2280478107745,
116.136815729041)) ;
#181699=CARTESIAN_POINT('Ctrl Pts',(-21.0439982208835,-13.2400469135056,
116.065602507524)) ;
#181700=CARTESIAN_POINT('Ctrl Pts',(-21.0066020047252,-12.9607801917685,
115.987295334548)) ;
#181701=CARTESIAN_POINT('Ctrl Pts',(-20.9850605701347,-12.9922952069383,
115.921683598776)) ;
#181702=CARTESIAN_POINT('Ctrl Pts',(-20.911256714969,-12.9922951270176,
115.945914604686)) ;
#181703=CARTESIAN_POINT('Ctrl Pts',(-20.8374528598033,-12.9922950470968,
115.970145610596)) ;
#181704=CARTESIAN_POINT('Ctrl Pts',(-20.8589942943938,-12.960780031927,
116.035757346369)) ;
#181705=CARTESIAN_POINT('Ctrl Pts',(-20.8805357289843,-12.9292650167572,
116.101369082141)) ;
#181706=CARTESIAN_POINT('Ctrl Pts',(-20.95433958415,-12.929265096678,116.077138076231)) ;
#181707=CARTESIAN_POINT('Ctrl Pts',(-21.0281434393157,-12.9292651765987,
116.052907070321)) ;
#181708=CARTESIAN_POINT('Ctrl Pts',(-21.0066020047252,-12.9607801917685,
115.987295334548)) ;
#181709=CARTESIAN_POINT('Ctrl Pts',(-20.9473443980316,-12.7157522020321,
115.842202222821)) ;
#181710=CARTESIAN_POINT('Ctrl Pts',(-20.929175396646,-12.7644222769748,
115.786862374571)) ;
#181711=CARTESIAN_POINT('Ctrl Pts',(-20.8553715365486,-12.7644222146516,
115.81109336546)) ;
#181712=CARTESIAN_POINT('Ctrl Pts',(-20.7815676764512,-12.7644221523283,
115.835324356349)) ;
#181713=CARTESIAN_POINT('Ctrl Pts',(-20.7997366778369,-12.7157520773856,
115.8906642046)) ;
#181714=CARTESIAN_POINT('Ctrl Pts',(-20.8179056792225,-12.6670820024428,
115.946004052851)) ;
#181715=CARTESIAN_POINT('Ctrl Pts',(-20.8917095393199,-12.6670820647661,
115.921773061961)) ;
#181716=CARTESIAN_POINT('Ctrl Pts',(-20.9655133994172,-12.6670821270893,
115.897542071072)) ;
#181717=CARTESIAN_POINT('Ctrl Pts',(-20.9473443980316,-12.7157522020321,
115.842202222821)) ;
#181718=CARTESIAN_POINT('Ctrl Pts',(-20.8694399766873,-12.5205021117526,
115.640390114338)) ;
#181719=CARTESIAN_POINT('Ctrl Pts',(-20.8559487341846,-12.5828779756765,
115.599297965034)) ;
#181720=CARTESIAN_POINT('Ctrl Pts',(-20.7821448714235,-12.5828779339693,
115.62352894781)) ;
#181721=CARTESIAN_POINT('Ctrl Pts',(-20.7083410086625,-12.582877892262,
115.647759930586)) ;
#181722=CARTESIAN_POINT('Ctrl Pts',(-20.7218322511651,-12.5205020283381,
115.688852079889)) ;
#181723=CARTESIAN_POINT('Ctrl Pts',(-20.7353234936678,-12.4581261644142,
115.729944229193)) ;
#181724=CARTESIAN_POINT('Ctrl Pts',(-20.8091273564289,-12.4581262061215,
115.705713246417)) ;
#181725=CARTESIAN_POINT('Ctrl Pts',(-20.88293121919,-12.4581262478287,115.681482263641)) ;
#181726=CARTESIAN_POINT('Ctrl Pts',(-20.8694399766873,-12.5205021117526,
115.640390114338)) ;
#181727=CARTESIAN_POINT('Ctrl Pts',(-20.7779765651367,-12.3896091910669,
115.397208988666)) ;
#181728=CARTESIAN_POINT('Ctrl Pts',(-20.7701183297895,-12.4612182427459,
115.373274070417)) ;
#181729=CARTESIAN_POINT('Ctrl Pts',(-20.6963144664325,-12.4612182215385,
115.397505051378)) ;
#181730=CARTESIAN_POINT('Ctrl Pts',(-20.6225106030756,-12.461218200331,
115.421736032339)) ;
#181731=CARTESIAN_POINT('Ctrl Pts',(-20.6303688384228,-12.389609148652,
115.445670950587)) ;
#181732=CARTESIAN_POINT('Ctrl Pts',(-20.6382270737699,-12.318000096973,
115.469605868836)) ;
#181733=CARTESIAN_POINT('Ctrl Pts',(-20.7120309371269,-12.3180001181804,
115.445374887875)) ;
#181734=CARTESIAN_POINT('Ctrl Pts',(-20.7858348004839,-12.3180001393879,
115.421143906914)) ;
#181735=CARTESIAN_POINT('Ctrl Pts',(-20.7779765651367,-12.3896091910669,
115.397208988666)) ;
#181736=CARTESIAN_POINT('Ctrl Pts',(-20.6779561212234,-12.3322116649338,
115.128190401515)) ;
#181737=CARTESIAN_POINT('Ctrl Pts',(-20.6763321849345,-12.4079372852091,
115.123244152491)) ;
#181738=CARTESIAN_POINT('Ctrl Pts',(-20.6025283236232,-12.4079372823359,
115.147475139682)) ;
#181739=CARTESIAN_POINT('Ctrl Pts',(-20.5287244623119,-12.4079372794628,
115.171706126874)) ;
#181740=CARTESIAN_POINT('Ctrl Pts',(-20.5303483986008,-12.3322116591875,
115.176652375899)) ;
#181741=CARTESIAN_POINT('Ctrl Pts',(-20.5319723348897,-12.2564860389122,
115.181598624924)) ;
#181742=CARTESIAN_POINT('Ctrl Pts',(-20.605776196201,-12.2564860417854,
115.157367637732)) ;
#181743=CARTESIAN_POINT('Ctrl Pts',(-20.6795800575123,-12.2564860446585,
115.13313665054)) ;
#181744=CARTESIAN_POINT('Ctrl Pts',(-20.6779561212234,-12.3322116649338,
115.128190401515)) ;
#181745=CARTESIAN_POINT('Ctrl Pts',(-20.5774147689211,-12.3526193896652,
114.857217210318)) ;
#181746=CARTESIAN_POINT('Ctrl Pts',(-20.582078673644,-12.4270343562084,
114.871422710604)) ;
#181747=CARTESIAN_POINT('Ctrl Pts',(-20.5082748147709,-12.4270343671983,
114.895653705222)) ;
#181748=CARTESIAN_POINT('Ctrl Pts',(-20.4344709558978,-12.4270343781882,
114.919884699841)) ;
#181749=CARTESIAN_POINT('Ctrl Pts',(-20.4298070511749,-12.352619411645,
114.905679199554)) ;
#181750=CARTESIAN_POINT('Ctrl Pts',(-20.4251431464519,-12.2782044451017,
114.891473699268)) ;
#181751=CARTESIAN_POINT('Ctrl Pts',(-20.498947005325,-12.2782044341118,
114.86724270465)) ;
#181752=CARTESIAN_POINT('Ctrl Pts',(-20.5727508641981,-12.2782044231219,
114.843011710032)) ;
#181753=CARTESIAN_POINT('Ctrl Pts',(-20.5774147689211,-12.3526193896652,
114.857217210318)) ;
#181754=CARTESIAN_POINT('Ctrl Pts',(-20.480876963674,-12.4495335034968,
114.598771665885)) ;
#181755=CARTESIAN_POINT('Ctrl Pts',(-20.4915518909879,-12.5172950398371,
114.631285771301)) ;
#181756=CARTESIAN_POINT('Ctrl Pts',(-20.4177480363705,-12.517295059255,
114.655516778881)) ;
#181757=CARTESIAN_POINT('Ctrl Pts',(-20.343944181753,-12.5172950786729,
114.679747786462)) ;
#181758=CARTESIAN_POINT('Ctrl Pts',(-20.333269254439,-12.4495335423326,
114.647233681045)) ;
#181759=CARTESIAN_POINT('Ctrl Pts',(-20.3225943271251,-12.3817720059923,
114.614719575629)) ;
#181760=CARTESIAN_POINT('Ctrl Pts',(-20.3963981817425,-12.3817719865744,
114.590488568049)) ;
#181761=CARTESIAN_POINT('Ctrl Pts',(-20.47020203636,-12.3817719671566,114.566257560468)) ;
#181762=CARTESIAN_POINT('Ctrl Pts',(-20.480876963674,-12.4495335034968,
114.598771665885)) ;
#181763=CARTESIAN_POINT('Ctrl Pts',(-20.3957540886572,-12.6159519111974,
114.374983031782)) ;
#181764=CARTESIAN_POINT('Ctrl Pts',(-20.411654514387,-12.6721964554001,
114.423413162412)) ;
#181765=CARTESIAN_POINT('Ctrl Pts',(-20.337850663774,-12.6721964775936,
114.447644182189)) ;
#181766=CARTESIAN_POINT('Ctrl Pts',(-20.264046813161,-12.6721964997871,
114.471875201966)) ;
#181767=CARTESIAN_POINT('Ctrl Pts',(-20.2481463874312,-12.6159519555843,
114.423445071337)) ;
#181768=CARTESIAN_POINT('Ctrl Pts',(-20.2322459617013,-12.5597074113816,
114.375014940707)) ;
#181769=CARTESIAN_POINT('Ctrl Pts',(-20.3060498123144,-12.5597073891882,
114.35078392093)) ;
#181770=CARTESIAN_POINT('Ctrl Pts',(-20.3798536629274,-12.5597073669947,
114.326552901153)) ;
#181771=CARTESIAN_POINT('Ctrl Pts',(-20.3957540886572,-12.6159519111974,
114.374983031782)) ;
#181772=CARTESIAN_POINT('Ctrl Pts',(-20.3271536623197,-12.8395609374739,
114.201485817632)) ;
#181773=CARTESIAN_POINT('Ctrl Pts',(-20.3471345416621,-12.8802774256323,
114.262344351742)) ;
#181774=CARTESIAN_POINT('Ctrl Pts',(-20.2733306944363,-12.8802774463099,
114.286575381836)) ;
#181775=CARTESIAN_POINT('Ctrl Pts',(-20.1995268472104,-12.8802774669874,
114.31080641193)) ;
#181776=CARTESIAN_POINT('Ctrl Pts',(-20.179545967868,-12.839560978829,114.24994787782)) ;
#181777=CARTESIAN_POINT('Ctrl Pts',(-20.1595650885256,-12.7988444906705,
114.189089343709)) ;
#181778=CARTESIAN_POINT('Ctrl Pts',(-20.2333689357514,-12.798844469993,
114.164858313616)) ;
#181779=CARTESIAN_POINT('Ctrl Pts',(-20.3071727829772,-12.7988444493154,
114.140627283522)) ;
#181780=CARTESIAN_POINT('Ctrl Pts',(-20.3271536623197,-12.8395609374739,
114.201485817632)) ;
#181781=CARTESIAN_POINT('Ctrl Pts',(-20.2791583118047,-13.1036924153161,
114.090643871318)) ;
#181782=CARTESIAN_POINT('Ctrl Pts',(-20.3017891444804,-13.126027690226,
114.159573735842)) ;
#181783=CARTESIAN_POINT('Ctrl Pts',(-20.2279852997255,-13.1260277069746,
114.183804773462)) ;
#181784=CARTESIAN_POINT('Ctrl Pts',(-20.1541814549706,-13.1260277237232,
114.208035811082)) ;
#181785=CARTESIAN_POINT('Ctrl Pts',(-20.1315506222949,-13.1036924488133,
114.139105946557)) ;
#181786=CARTESIAN_POINT('Ctrl Pts',(-20.1089197896193,-13.0813571739034,
114.070176082033)) ;
#181787=CARTESIAN_POINT('Ctrl Pts',(-20.1827236343742,-13.0813571571548,
114.045945044413)) ;
#181788=CARTESIAN_POINT('Ctrl Pts',(-20.2565274791291,-13.0813571404062,
114.021714006793)) ;
#181789=CARTESIAN_POINT('Ctrl Pts',(-20.2791583118047,-13.1036924153161,
114.090643871318)) ;
#181790=CARTESIAN_POINT('Ctrl Pts',(-20.2542197759365,-13.3927905140901,
114.05034234162)) ;
#181791=CARTESIAN_POINT('Ctrl Pts',(-20.277888414452,-13.3949729390862,
114.122433195443)) ;
#181792=CARTESIAN_POINT('Ctrl Pts',(-20.204084571161,-13.3949729481192,
114.146664237522)) ;
#181793=CARTESIAN_POINT('Ctrl Pts',(-20.1302807278701,-13.3949729571521,
114.170895279601)) ;
#181794=CARTESIAN_POINT('Ctrl Pts',(-20.1066120893547,-13.392790532156,
114.098804425778)) ;
#181795=CARTESIAN_POINT('Ctrl Pts',(-20.0829434508393,-13.3906081071599,
114.026713571955)) ;
#181796=CARTESIAN_POINT('Ctrl Pts',(-20.1567472941302,-13.390608098127,
114.002482529876)) ;
#181797=CARTESIAN_POINT('Ctrl Pts',(-20.2305511374211,-13.3906080890941,
113.978251487797)) ;
#181798=CARTESIAN_POINT('Ctrl Pts',(-20.2542197759365,-13.3927905140901,
114.05034234162)) ;
#181799=CARTESIAN_POINT('Ctrl Pts',(-20.2537651631048,-13.6807940128297,
114.084250210379)) ;
#181800=CARTESIAN_POINT('Ctrl Pts',(-20.2767706334503,-13.6628697332101,
114.154321161045)) ;
#181801=CARTESIAN_POINT('Ctrl Pts',(-20.2029667904965,-13.6628697375112,
114.178552204151)) ;
#181802=CARTESIAN_POINT('Ctrl Pts',(-20.1291629475428,-13.6628697418123,
114.202783247257)) ;
#181803=CARTESIAN_POINT('Ctrl Pts',(-20.1061574771973,-13.680794021432,
114.132712296591)) ;
#181804=CARTESIAN_POINT('Ctrl Pts',(-20.0831520068518,-13.6987183010517,
114.062641345926)) ;
#181805=CARTESIAN_POINT('Ctrl Pts',(-20.1569558498055,-13.6987182967505,
114.03841030282)) ;
#181806=CARTESIAN_POINT('Ctrl Pts',(-20.2307596927593,-13.6987182924494,
114.014179259714)) ;
#181807=CARTESIAN_POINT('Ctrl Pts',(-20.2537651631048,-13.6807940128297,
114.084250210379)) ;
#181808=CARTESIAN_POINT('Ctrl Pts',(-20.2767369580529,-13.9516407801447,
114.189702183706)) ;
#181809=CARTESIAN_POINT('Ctrl Pts',(-20.2974385928997,-13.9147771638665,
114.252756023256)) ;
#181810=CARTESIAN_POINT('Ctrl Pts',(-20.2236347495658,-13.9147771635359,
114.276987065204)) ;
#181811=CARTESIAN_POINT('Ctrl Pts',(-20.1498309062319,-13.9147771632054,
114.301218107152)) ;
#181812=CARTESIAN_POINT('Ctrl Pts',(-20.1291292713852,-13.9516407794836,
114.238164267602)) ;
#181813=CARTESIAN_POINT('Ctrl Pts',(-20.1084276365384,-13.9885043957617,
114.175110428052)) ;
#181814=CARTESIAN_POINT('Ctrl Pts',(-20.1822314798723,-13.9885043960923,
114.150879386104)) ;
#181815=CARTESIAN_POINT('Ctrl Pts',(-20.2560353232062,-13.9885043964229,
114.126648344155)) ;
#181816=CARTESIAN_POINT('Ctrl Pts',(-20.2767369580529,-13.9516407801447,
114.189702183706)) ;
#181817=CARTESIAN_POINT('Ctrl Pts',(-20.3212515827195,-14.1848191645832,
114.360909549778)) ;
#181818=CARTESIAN_POINT('Ctrl Pts',(-20.3381385223981,-14.1316174193291,
114.412344443398)) ;
#181819=CARTESIAN_POINT('Ctrl Pts',(-20.2643346783687,-14.1316174171336,
114.436575483228)) ;
#181820=CARTESIAN_POINT('Ctrl Pts',(-20.1905308343394,-14.1316174149382,
114.460806523058)) ;
#181821=CARTESIAN_POINT('Ctrl Pts',(-20.1736438946608,-14.1848191601922,
114.409371629438)) ;
#181822=CARTESIAN_POINT('Ctrl Pts',(-20.1567569549822,-14.2380209054463,
114.357936735817)) ;
#181823=CARTESIAN_POINT('Ctrl Pts',(-20.2305607990116,-14.2380209076418,
114.333705695988)) ;
#181824=CARTESIAN_POINT('Ctrl Pts',(-20.304364643041,-14.2380209098372,
114.309474656158)) ;
#181825=CARTESIAN_POINT('Ctrl Pts',(-20.3212515827195,-14.1848191645832,
114.360909549778)) ;
#181826=CARTESIAN_POINT('Ctrl Pts',(-20.3823727653949,-14.3611535147467,
114.582313485388)) ;
#181827=CARTESIAN_POINT('Ctrl Pts',(-20.3942874125168,-14.2955603830771,
114.618603578166)) ;
#181828=CARTESIAN_POINT('Ctrl Pts',(-20.3204835681855,-14.2955603814556,
114.642834617076)) ;
#181829=CARTESIAN_POINT('Ctrl Pts',(-20.2466797238541,-14.2955603798341,
114.667065655986)) ;
#181830=CARTESIAN_POINT('Ctrl Pts',(-20.2347650767322,-14.3611535115037,
114.630775563208)) ;
#181831=CARTESIAN_POINT('Ctrl Pts',(-20.2228504296103,-14.4267466431733,
114.594485470431)) ;
#181832=CARTESIAN_POINT('Ctrl Pts',(-20.2966542739417,-14.4267466447948,
114.570254431521)) ;
#181833=CARTESIAN_POINT('Ctrl Pts',(-20.370458118273,-14.4267466464163,
114.546023392611)) ;
#181834=CARTESIAN_POINT('Ctrl Pts',(-20.3823727653949,-14.3611535147467,
114.582313485388)) ;
#181835=CARTESIAN_POINT('Ctrl Pts',(-20.4563210601665,-14.4717132500286,
114.843190270097)) ;
#181836=CARTESIAN_POINT('Ctrl Pts',(-20.4623519080848,-14.3983025037114,
114.861559259812)) ;
#181837=CARTESIAN_POINT('Ctrl Pts',(-20.3885480641969,-14.3983025035885,
114.885790300072)) ;
#181838=CARTESIAN_POINT('Ctrl Pts',(-20.314744220309,-14.3983025034657,
114.910021340333)) ;
#181839=CARTESIAN_POINT('Ctrl Pts',(-20.3087133723907,-14.4717132497829,
114.891652350619)) ;
#181840=CARTESIAN_POINT('Ctrl Pts',(-20.3026825244725,-14.5451239961002,
114.873283360904)) ;
#181841=CARTESIAN_POINT('Ctrl Pts',(-20.3764863683604,-14.545123996223,
114.849052320643)) ;
#181842=CARTESIAN_POINT('Ctrl Pts',(-20.4502902122482,-14.5451239963458,
114.824821280383)) ;
#181843=CARTESIAN_POINT('Ctrl Pts',(-20.4563210601665,-14.4717132500286,
114.843190270097)) ;
#181844=CARTESIAN_POINT('Ctrl Pts',(-20.5359913410577,-14.5058049610956,
115.121300978399)) ;
#181845=CARTESIAN_POINT('Ctrl Pts',(-20.5357343387305,-14.4299061959812,
115.120518190733)) ;
#181846=CARTESIAN_POINT('Ctrl Pts',(-20.4619304960325,-14.4299061963414,
115.144749234618)) ;
#181847=CARTESIAN_POINT('Ctrl Pts',(-20.3881266533344,-14.4299061967016,
115.168980278503)) ;
#181848=CARTESIAN_POINT('Ctrl Pts',(-20.3883836556616,-14.505804961816,
115.169763066168)) ;
#181849=CARTESIAN_POINT('Ctrl Pts',(-20.3886406579888,-14.5817037269304,
115.170545853834)) ;
#181850=CARTESIAN_POINT('Ctrl Pts',(-20.4624445006868,-14.5817037265702,
115.146314809949)) ;
#181851=CARTESIAN_POINT('Ctrl Pts',(-20.5362483433849,-14.58170372621,115.122083766064)) ;
#181852=CARTESIAN_POINT('Ctrl Pts',(-20.5359913410577,-14.5058049610956,
115.121300978399)) ;
#181853=CARTESIAN_POINT('Ctrl Pts',(-20.6152285993297,-14.4622432474708,
115.398086166475)) ;
#181854=CARTESIAN_POINT('Ctrl Pts',(-20.6087050569855,-14.389275462024,
115.378216508923)) ;
#181855=CARTESIAN_POINT('Ctrl Pts',(-20.5349012157987,-14.3892754604599,
115.402447557411)) ;
#181856=CARTESIAN_POINT('Ctrl Pts',(-20.4610973746118,-14.3892754588959,
115.426678605899)) ;
#181857=CARTESIAN_POINT('Ctrl Pts',(-20.4676209169561,-14.4622432443427,
115.44654826345)) ;
#181858=CARTESIAN_POINT('Ctrl Pts',(-20.4741444593003,-14.5352110297894,
115.466417921002)) ;
#181859=CARTESIAN_POINT('Ctrl Pts',(-20.5479483004871,-14.5352110313535,
115.442186872514)) ;
#181860=CARTESIAN_POINT('Ctrl Pts',(-20.621752141674,-14.5352110329176,
115.417955824026)) ;
#181861=CARTESIAN_POINT('Ctrl Pts',(-20.6152285993297,-14.4622432474708,
115.398086166475)) ;
#181862=CARTESIAN_POINT('Ctrl Pts',(-20.6876764922037,-14.343914063795,
115.654200032397)) ;
#181863=CARTESIAN_POINT('Ctrl Pts',(-20.6753512998401,-14.2791023763225,
115.616659484858)) ;
#181864=CARTESIAN_POINT('Ctrl Pts',(-20.6015474601322,-14.2791023697226,
115.64089053785)) ;
#181865=CARTESIAN_POINT('Ctrl Pts',(-20.5277436204242,-14.2791023631227,
115.665121590843)) ;
#181866=CARTESIAN_POINT('Ctrl Pts',(-20.5400688127878,-14.3439140505953,
115.702662138382)) ;
#181867=CARTESIAN_POINT('Ctrl Pts',(-20.5523940051514,-14.4087257380679,
115.740202685921)) ;
#181868=CARTESIAN_POINT('Ctrl Pts',(-20.6261978448593,-14.4087257446678,
115.715971632929)) ;
#181869=CARTESIAN_POINT('Ctrl Pts',(-20.7000016845672,-14.4087257512676,
115.691740579936)) ;
#181870=CARTESIAN_POINT('Ctrl Pts',(-20.6876764922037,-14.343914063795,
115.654200032397)) ;
#181871=CARTESIAN_POINT('Ctrl Pts',(-20.7473748229597,-14.1592285094383,
115.871492526232)) ;
#181872=CARTESIAN_POINT('Ctrl Pts',(-20.7301296462246,-14.1072180552491,
115.818966499993)) ;
#181873=CARTESIAN_POINT('Ctrl Pts',(-20.6563258073989,-14.1072180404113,
115.843197555672)) ;
#181874=CARTESIAN_POINT('Ctrl Pts',(-20.5825219685731,-14.1072180255735,
115.867428611351)) ;
#181875=CARTESIAN_POINT('Ctrl Pts',(-20.5997671453082,-14.1592284797627,
115.91995463759)) ;
#181876=CARTESIAN_POINT('Ctrl Pts',(-20.6170123220432,-14.2112389339519,
115.97248066383)) ;
#181877=CARTESIAN_POINT('Ctrl Pts',(-20.690816160869,-14.2112389487897,
115.948249608151)) ;
#181878=CARTESIAN_POINT('Ctrl Pts',(-20.7646199996947,-14.2112389636275,
115.924018552472)) ;
#181879=CARTESIAN_POINT('Ctrl Pts',(-20.7473748229597,-14.1592285094383,
115.871492526232)) ;
#181880=CARTESIAN_POINT('Ctrl Pts',(-20.7892502687807,-13.9218383285055,
116.034450676081)) ;
#181881=CARTESIAN_POINT('Ctrl Pts',(-20.7683235711504,-13.8863275964736,
115.97071133106)) ;
#181882=CARTESIAN_POINT('Ctrl Pts',(-20.6945197320421,-13.8863275716233,
115.994942385878)) ;
#181883=CARTESIAN_POINT('Ctrl Pts',(-20.6207158929338,-13.886327546773,
116.019173440697)) ;
#181884=CARTESIAN_POINT('Ctrl Pts',(-20.6416425905641,-13.9218382788049,
116.082912785718)) ;
#181885=CARTESIAN_POINT('Ctrl Pts',(-20.6625692881944,-13.9573490108368,
116.146652130738)) ;
#181886=CARTESIAN_POINT('Ctrl Pts',(-20.7363731273027,-13.9573490356871,
116.12242107592)) ;
#181887=CARTESIAN_POINT('Ctrl Pts',(-20.810176966411,-13.9573490605374,
116.098190021101)) ;
#181888=CARTESIAN_POINT('Ctrl Pts',(-20.7892502687807,-13.9218383285055,
116.034450676081)) ;
#181889=CARTESIAN_POINT('Ctrl Pts',(-20.8096697160064,-13.6477929587425,
116.132141353103)) ;
#181890=CARTESIAN_POINT('Ctrl Pts',(-20.7865525111925,-13.6313648712608,
116.061730076469)) ;
#181891=CARTESIAN_POINT('Ctrl Pts',(-20.7127486704703,-13.6313648350965,
116.085961126372)) ;
#181892=CARTESIAN_POINT('Ctrl Pts',(-20.638944829748,-13.6313647989322,
116.110192176274)) ;
#181893=CARTESIAN_POINT('Ctrl Pts',(-20.6620620345618,-13.6477928864138,
116.180603452908)) ;
#181894=CARTESIAN_POINT('Ctrl Pts',(-20.6851792393755,-13.6642209738955,
116.251014729542)) ;
#181895=CARTESIAN_POINT('Ctrl Pts',(-20.7589830800978,-13.6642210100599,
116.22678367964)) ;
#181896=CARTESIAN_POINT('Ctrl Pts',(-20.8327869208201,-13.6642210462242,
116.202552629737)) ;
#181897=CARTESIAN_POINT('Ctrl Pts',(-20.8096697160064,-13.6477929587425,
116.132141353103)) ;
#181898=CARTESIAN_POINT('Ctrl Pts',(-20.8062757150026,-13.3573882946602,
116.157281504951)) ;
#181899=CARTESIAN_POINT('Ctrl Pts',(-20.7826279371143,-13.3612124494826,
116.085254188169)) ;
#181900=CARTESIAN_POINT('Ctrl Pts',(-20.7088240931421,-13.3612124035114,
116.109485228173)) ;
#181901=CARTESIAN_POINT('Ctrl Pts',(-20.6350202491699,-13.3612123575402,
116.133716268177)) ;
#181902=CARTESIAN_POINT('Ctrl Pts',(-20.6586680270582,-13.3573882027177,
116.205743584959)) ;
#181903=CARTESIAN_POINT('Ctrl Pts',(-20.6823158049464,-13.3535640478952,
116.277770901741)) ;
#181904=CARTESIAN_POINT('Ctrl Pts',(-20.7561196489186,-13.3535640938664,
116.253539861737)) ;
#181905=CARTESIAN_POINT('Ctrl Pts',(-20.8299234928908,-13.3535641398377,
116.229308821733)) ;
#181906=CARTESIAN_POINT('Ctrl Pts',(-20.8062757150026,-13.3573882946602,
116.157281504951)) ;
#181907=CARTESIAN_POINT('Ctrl Pts',(-20.7786075112858,-13.0713760146383,
116.108481462324)) ;
#181908=CARTESIAN_POINT('Ctrl Pts',(-20.7561233059056,-13.0951747720227,
116.03999819949)) ;
#181909=CARTESIAN_POINT('Ctrl Pts',(-20.682319457276,-13.0951747198527,
116.064229225309)) ;
#181910=CARTESIAN_POINT('Ctrl Pts',(-20.6085156086464,-13.0951746676827,
116.088460251127)) ;
#181911=CARTESIAN_POINT('Ctrl Pts',(-20.6309998140267,-13.0713759102982,
116.156943513961)) ;
#181912=CARTESIAN_POINT('Ctrl Pts',(-20.6534840194069,-13.0475771529138,
116.225426776795)) ;
#181913=CARTESIAN_POINT('Ctrl Pts',(-20.7272878680365,-13.0475772050838,
116.201195750976)) ;
#181914=CARTESIAN_POINT('Ctrl Pts',(-20.8010917166661,-13.0475772572539,
116.176964725158)) ;
#181915=CARTESIAN_POINT('Ctrl Pts',(-20.7786075112858,-13.0713760146383,
116.108481462324)) ;
#181916=CARTESIAN_POINT('Ctrl Pts',(-20.727862298227,-12.8101300373193,
115.989403245096)) ;
#181917=CARTESIAN_POINT('Ctrl Pts',(-20.7081542834235,-12.852202961782,
115.929375810654)) ;
#181918=CARTESIAN_POINT('Ctrl Pts',(-20.634350429137,-12.8522029087301,
115.953606819242)) ;
#181919=CARTESIAN_POINT('Ctrl Pts',(-20.5605465748504,-12.8522028556782,
115.97783782783)) ;
#181920=CARTESIAN_POINT('Ctrl Pts',(-20.5802545896539,-12.8101299312156,
116.037865262272)) ;
#181921=CARTESIAN_POINT('Ctrl Pts',(-20.5999626044573,-12.7680570067529,
116.097892696714)) ;
#181922=CARTESIAN_POINT('Ctrl Pts',(-20.6737664587439,-12.7680570598048,
116.073661688126)) ;
#181923=CARTESIAN_POINT('Ctrl Pts',(-20.7475703130304,-12.7680571128567,
116.049430679538)) ;
#181924=CARTESIAN_POINT('Ctrl Pts',(-20.727862298227,-12.8101300373193,
115.989403245096)) ;
#181925=CARTESIAN_POINT('Ctrl Pts',(-20.6569850715304,-12.5926203368979,
115.808983189136)) ;
#181926=CARTESIAN_POINT('Ctrl Pts',(-20.6414632766714,-12.6499401722223,
115.761706305044)) ;
#181927=CARTESIAN_POINT('Ctrl Pts',(-20.5676594164585,-12.6499401250942,
115.785937295581)) ;
#181928=CARTESIAN_POINT('Ctrl Pts',(-20.4938555562457,-12.6499400779661,
115.810168286119)) ;
#181929=CARTESIAN_POINT('Ctrl Pts',(-20.5093773511048,-12.5926202426416,
115.857445170211)) ;
#181930=CARTESIAN_POINT('Ctrl Pts',(-20.5248991459638,-12.5353004073172,
115.904722054302)) ;
#181931=CARTESIAN_POINT('Ctrl Pts',(-20.5987030061767,-12.5353004544453,
115.880491063765)) ;
#181932=CARTESIAN_POINT('Ctrl Pts',(-20.6725068663895,-12.5353005015734,
115.856260073227)) ;
#181933=CARTESIAN_POINT('Ctrl Pts',(-20.6569850715304,-12.5926203368979,
115.808983189136)) ;
#181934=CARTESIAN_POINT('Ctrl Pts',(-20.5702654370651,-12.4341144288436,
115.580315447972)) ;
#181935=CARTESIAN_POINT('Ctrl Pts',(-20.5600417992635,-12.5025837722115,
115.549175895275)) ;
#181936=CARTESIAN_POINT('Ctrl Pts',(-20.4862379335849,-12.5025837377898,
115.573406869165)) ;
#181937=CARTESIAN_POINT('Ctrl Pts',(-20.4124340679063,-12.502583703368,
115.597637843054)) ;
#181938=CARTESIAN_POINT('Ctrl Pts',(-20.4226577057078,-12.4341143600001,
115.628777395751)) ;
#181939=CARTESIAN_POINT('Ctrl Pts',(-20.4328813435093,-12.3656450166321,
115.659916948448)) ;
#181940=CARTESIAN_POINT('Ctrl Pts',(-20.506685209188,-12.3656450510539,
115.635685974559)) ;
#181941=CARTESIAN_POINT('Ctrl Pts',(-20.5804890748666,-12.3656450854756,
115.611455000669)) ;
#181942=CARTESIAN_POINT('Ctrl Pts',(-20.5702654370651,-12.4341144288436,
115.580315447972)) ;
#181943=CARTESIAN_POINT('Ctrl Pts',(-20.4730652679923,-12.346259851331,
115.319760267267)) ;
#181944=CARTESIAN_POINT('Ctrl Pts',(-20.4688784108342,-12.4209624752005,
115.30700777424)) ;
#181945=CARTESIAN_POINT('Ctrl Pts',(-20.3950745409072,-12.4209624599237,
115.33123873519)) ;
#181946=CARTESIAN_POINT('Ctrl Pts',(-20.3212706709801,-12.4209624446469,
115.355469696139)) ;
#181947=CARTESIAN_POINT('Ctrl Pts',(-20.3254575281383,-12.3462598207773,
115.368222189166)) ;
#181948=CARTESIAN_POINT('Ctrl Pts',(-20.3296443852964,-12.2715571969078,
115.380974682192)) ;
#181949=CARTESIAN_POINT('Ctrl Pts',(-20.4034482552235,-12.2715572121846,
115.356743721243)) ;
#181950=CARTESIAN_POINT('Ctrl Pts',(-20.4772521251505,-12.2715572274614,
115.332512760293)) ;
#181951=CARTESIAN_POINT('Ctrl Pts',(-20.4730652679923,-12.346259851331,
115.319760267267)) ;
#181952=CARTESIAN_POINT('Ctrl Pts',(-20.372232841033,-12.3348158852733,
115.047945482228)) ;
#181953=CARTESIAN_POINT('Ctrl Pts',(-20.3743491903962,-12.4104256805368,
115.054391539147)) ;
#181954=CARTESIAN_POINT('Ctrl Pts',(-20.3005453185203,-12.4104256886821,
115.078622494161)) ;
#181955=CARTESIAN_POINT('Ctrl Pts',(-20.2267414466445,-12.4104256968275,
115.102853449174)) ;
#181956=CARTESIAN_POINT('Ctrl Pts',(-20.2246250972813,-12.334815901564,
115.096407392256)) ;
#181957=CARTESIAN_POINT('Ctrl Pts',(-20.2225087479182,-12.2592061063006,
115.089961335338)) ;
#181958=CARTESIAN_POINT('Ctrl Pts',(-20.296312619794,-12.2592060981552,
115.065730380324)) ;
#181959=CARTESIAN_POINT('Ctrl Pts',(-20.3701164916698,-12.2592060900098,
115.04149942531)) ;
#181960=CARTESIAN_POINT('Ctrl Pts',(-20.372232841033,-12.3348158852733,
115.047945482228)) ;
#181961=CARTESIAN_POINT('Ctrl Pts',(-20.272459099619,-12.4019396871859,
114.779822675992)) ;
#181962=CARTESIAN_POINT('Ctrl Pts',(-20.2808041605409,-12.4729745049504,
114.805240383184)) ;
#181963=CARTESIAN_POINT('Ctrl Pts',(-20.2070002883668,-12.4729745398318,
114.829471337289)) ;
#181964=CARTESIAN_POINT('Ctrl Pts',(-20.1331964161927,-12.4729745747131,
114.853702291394)) ;
#181965=CARTESIAN_POINT('Ctrl Pts',(-20.1248513552708,-12.4019397569486,
114.828284584203)) ;
#181966=CARTESIAN_POINT('Ctrl Pts',(-20.1165062943488,-12.330904939184,
114.802866877011)) ;
#181967=CARTESIAN_POINT('Ctrl Pts',(-20.1903101665229,-12.3309049043027,
114.778635922906)) ;
#181968=CARTESIAN_POINT('Ctrl Pts',(-20.2641140386971,-12.3309048694214,
114.7544049688)) ;
#181969=CARTESIAN_POINT('Ctrl Pts',(-20.272459099619,-12.4019396871859,
114.779822675992)) ;
#181970=CARTESIAN_POINT('Ctrl Pts',(-20.1830070427554,-12.5400212389952,
114.542504031555)) ;
#181971=CARTESIAN_POINT('Ctrl Pts',(-20.1968824352242,-12.6015185806479,
114.584766236272)) ;
#181972=CARTESIAN_POINT('Ctrl Pts',(-20.1230785662842,-12.6015186402617,
114.608997200228)) ;
#181973=CARTESIAN_POINT('Ctrl Pts',(-20.0492746973443,-12.6015186998755,
114.633228164184)) ;
#181974=CARTESIAN_POINT('Ctrl Pts',(-20.0353993048755,-12.5400213582228,
114.590965959467)) ;
#181975=CARTESIAN_POINT('Ctrl Pts',(-20.0215239124067,-12.4785240165702,
114.54870375475)) ;
#181976=CARTESIAN_POINT('Ctrl Pts',(-20.0953277813467,-12.4785239569564,
114.524472790794)) ;
#181977=CARTESIAN_POINT('Ctrl Pts',(-20.1691316502866,-12.4785238973426,
114.500241826838)) ;
#181978=CARTESIAN_POINT('Ctrl Pts',(-20.1830070427554,-12.5400212389952,
114.542504031555)) ;
#181979=CARTESIAN_POINT('Ctrl Pts',(-20.1067029971044,-12.7426569389483,
114.345713360105)) ;
#181980=CARTESIAN_POINT('Ctrl Pts',(-20.1251890157944,-12.790097789664,
114.402018788292)) ;
#181981=CARTESIAN_POINT('Ctrl Pts',(-20.0513851519428,-12.7900978720305,
114.426249767746)) ;
#181982=CARTESIAN_POINT('Ctrl Pts',(-19.9775812880912,-12.790097954397,
114.450480747201)) ;
#181983=CARTESIAN_POINT('Ctrl Pts',(-19.9590952694012,-12.7426571036813,
114.394175319013)) ;
#181984=CARTESIAN_POINT('Ctrl Pts',(-19.9406092507112,-12.6952162529655,
114.337869890826)) ;
#181985=CARTESIAN_POINT('Ctrl Pts',(-20.0144131145628,-12.695216170599,
114.313638911372)) ;
#181986=CARTESIAN_POINT('Ctrl Pts',(-20.0882169784144,-12.6952160882325,
114.289407931918)) ;
#181987=CARTESIAN_POINT('Ctrl Pts',(-20.1067029971044,-12.7426569389483,
114.345713360105)) ;
#181988=CARTESIAN_POINT('Ctrl Pts',(-20.0499392060894,-12.9928209893326,
114.208234860581)) ;
#181989=CARTESIAN_POINT('Ctrl Pts',(-20.0716826594989,-13.0228660525859,
114.2744619093)) ;
#181990=CARTESIAN_POINT('Ctrl Pts',(-19.9978788029917,-13.0228661512881,
114.298692911124)) ;
#181991=CARTESIAN_POINT('Ctrl Pts',(-19.9240749464844,-13.0228662499903,
114.322923912948)) ;
#181992=CARTESIAN_POINT('Ctrl Pts',(-19.9023314930749,-12.992821186737,
114.256696864229)) ;
#181993=CARTESIAN_POINT('Ctrl Pts',(-19.8805880396653,-12.9627761234838,
114.190469815509)) ;
#181994=CARTESIAN_POINT('Ctrl Pts',(-19.9543918961725,-12.9627760247816,
114.166238813685)) ;
#181995=CARTESIAN_POINT('Ctrl Pts',(-20.0281957526798,-12.9627759260794,
114.142007811862)) ;
#181996=CARTESIAN_POINT('Ctrl Pts',(-20.0499392060894,-12.9928209893326,
114.208234860581)) ;
#181997=CARTESIAN_POINT('Ctrl Pts',(-20.0153853295519,-13.274121349933,
114.138514811439)) ;
#181998=CARTESIAN_POINT('Ctrl Pts',(-20.0388382801524,-13.2845716251807,
114.209948712753)) ;
#181999=CARTESIAN_POINT('Ctrl Pts',(-19.9650344322706,-13.2845717326201,
114.234179740849)) ;
#182000=CARTESIAN_POINT('Ctrl Pts',(-19.8912305843888,-13.2845718400594,
114.258410768945)) ;
#182001=CARTESIAN_POINT('Ctrl Pts',(-19.8677776337882,-13.2741215648117,
114.18697686763)) ;
#182002=CARTESIAN_POINT('Ctrl Pts',(-19.8443246831877,-13.263671289564,
114.115542966315)) ;
#182003=CARTESIAN_POINT('Ctrl Pts',(-19.9181285310695,-13.2636711821247,
114.09131193822)) ;
#182004=CARTESIAN_POINT('Ctrl Pts',(-19.9919323789513,-13.2636710746853,
114.067080910124)) ;
#182005=CARTESIAN_POINT('Ctrl Pts',(-20.0153853295519,-13.274121349933,
114.138514811439)) ;
#182006=CARTESIAN_POINT('Ctrl Pts',(-20.0050410507883,-13.5650423075934,
114.142439305779)) ;
#182007=CARTESIAN_POINT('Ctrl Pts',(-20.0285177894748,-13.5551969668732,
114.213945661769)) ;
#182008=CARTESIAN_POINT('Ctrl Pts',(-19.95471395066,-13.555197074088,114.238176717481)) ;
#182009=CARTESIAN_POINT('Ctrl Pts',(-19.8809101118452,-13.5551971813029,
114.262407773194)) ;
#182010=CARTESIAN_POINT('Ctrl Pts',(-19.8574333731587,-13.5650425220231,
114.190901417204)) ;
#182011=CARTESIAN_POINT('Ctrl Pts',(-19.8339566344721,-13.5748878627432,
114.119395061214)) ;
#182012=CARTESIAN_POINT('Ctrl Pts',(-19.9077604732869,-13.5748877555284,
114.095164005502)) ;
#182013=CARTESIAN_POINT('Ctrl Pts',(-19.9815643121017,-13.5748876483136,
114.070932949789)) ;
#182014=CARTESIAN_POINT('Ctrl Pts',(-20.0050410507883,-13.5650423075934,
114.142439305779)) ;
#182015=CARTESIAN_POINT('Ctrl Pts',(-20.0186971571549,-13.8454220244642,
114.219462038445)) ;
#182016=CARTESIAN_POINT('Ctrl Pts',(-20.0405222537569,-13.8159869229919,
114.285937759159)) ;
#182017=CARTESIAN_POINT('Ctrl Pts',(-19.9667184235267,-13.8159870213789,
114.310168841019)) ;
#182018=CARTESIAN_POINT('Ctrl Pts',(-19.8929145932964,-13.8159871197658,
114.334399922878)) ;
#182019=CARTESIAN_POINT('Ctrl Pts',(-19.8710894966944,-13.8454222212381,
114.267924202164)) ;
#182020=CARTESIAN_POINT('Ctrl Pts',(-19.8492644000924,-13.8748573227103,
114.20144848145)) ;
#182021=CARTESIAN_POINT('Ctrl Pts',(-19.9230682303227,-13.8748572243234,
114.177217399591)) ;
#182022=CARTESIAN_POINT('Ctrl Pts',(-19.9968720605529,-13.8748571259364,
114.152986317731)) ;
#182023=CARTESIAN_POINT('Ctrl Pts',(-20.0186971571549,-13.8454220244642,
114.219462038445)) ;
#182024=CARTESIAN_POINT('Ctrl Pts',(-20.0547596385372,-14.095635489283,
114.36479225159)) ;
#182025=CARTESIAN_POINT('Ctrl Pts',(-20.0733651925667,-14.0486874017416,
114.421461765146)) ;
#182026=CARTESIAN_POINT('Ctrl Pts',(-19.9995613695628,-14.0486874834364,
114.445692869016)) ;
#182027=CARTESIAN_POINT('Ctrl Pts',(-19.9257575465589,-14.0486875651311,
114.469923972886)) ;
#182028=CARTESIAN_POINT('Ctrl Pts',(-19.9071519925294,-14.0956356526725,
114.41325445933)) ;
#182029=CARTESIAN_POINT('Ctrl Pts',(-19.8885464384999,-14.1425837402138,
114.356584945773)) ;
#182030=CARTESIAN_POINT('Ctrl Pts',(-19.9623502615038,-14.1425836585191,
114.332353841904)) ;
#182031=CARTESIAN_POINT('Ctrl Pts',(-20.0361540845077,-14.1425835768243,
114.308122738034)) ;
#182032=CARTESIAN_POINT('Ctrl Pts',(-20.0547596385372,-14.095635489283,
114.36479225159)) ;
#182033=CARTESIAN_POINT('Ctrl Pts',(-20.1097879472539,-14.2970558104585,
114.56784725279)) ;
#182034=CARTESIAN_POINT('Ctrl Pts',(-20.1238459167263,-14.2359749683573,
114.6106655576)) ;
#182035=CARTESIAN_POINT('Ctrl Pts',(-20.0500420989193,-14.2359750277231,
114.634896677298)) ;
#182036=CARTESIAN_POINT('Ctrl Pts',(-19.9762382811122,-14.2359750870889,
114.659127796997)) ;
#182037=CARTESIAN_POINT('Ctrl Pts',(-19.9621803116398,-14.2970559291901,
114.616309492187)) ;
#182038=CARTESIAN_POINT('Ctrl Pts',(-19.9481223421674,-14.3581367712912,
114.573491187376)) ;
#182039=CARTESIAN_POINT('Ctrl Pts',(-20.0219261599745,-14.3581367119255,
114.549260067678)) ;
#182040=CARTESIAN_POINT('Ctrl Pts',(-20.0957299777816,-14.3581366525597,
114.525028947979)) ;
#182041=CARTESIAN_POINT('Ctrl Pts',(-20.1097879472539,-14.2970558104585,
114.56784725279)) ;
#182042=CARTESIAN_POINT('Ctrl Pts',(-20.1793472667708,-14.4359480747077,
114.815266815336)) ;
#182043=CARTESIAN_POINT('Ctrl Pts',(-20.1878342866457,-14.3650783452255,
114.841116906637)) ;
#182044=CARTESIAN_POINT('Ctrl Pts',(-20.114030471417,-14.3650783787337,
114.865348034189)) ;
#182045=CARTESIAN_POINT('Ctrl Pts',(-20.0402266561884,-14.3650784122419,
114.889579161741)) ;
#182046=CARTESIAN_POINT('Ctrl Pts',(-20.0317396363136,-14.4359481417242,
114.86372907044)) ;
#182047=CARTESIAN_POINT('Ctrl Pts',(-20.0232526164387,-14.5068178712064,
114.837878979139)) ;
#182048=CARTESIAN_POINT('Ctrl Pts',(-20.0970564316673,-14.5068178376981,
114.813647851587)) ;
#182049=CARTESIAN_POINT('Ctrl Pts',(-20.1708602468959,-14.5068178041899,
114.789416724035)) ;
#182050=CARTESIAN_POINT('Ctrl Pts',(-20.1793472667708,-14.4359480747077,
114.815266815336)) ;
#182051=CARTESIAN_POINT('Ctrl Pts',(-20.2575026754292,-14.501304829004,
115.088848135438)) ;
#182052=CARTESIAN_POINT('Ctrl Pts',(-20.2598105850978,-14.4257651981435,
115.095877654163)) ;
#182053=CARTESIAN_POINT('Ctrl Pts',(-20.1860067697474,-14.4257652059426,
115.120108781345)) ;
#182054=CARTESIAN_POINT('Ctrl Pts',(-20.112202954397,-14.4257652137418,
115.144339908526)) ;
#182055=CARTESIAN_POINT('Ctrl Pts',(-20.1098950447284,-14.5013048446024,
115.1373103898)) ;
#182056=CARTESIAN_POINT('Ctrl Pts',(-20.1075871350598,-14.576844475463,
115.130280871074)) ;
#182057=CARTESIAN_POINT('Ctrl Pts',(-20.1813909504102,-14.5768444676638,
115.106049743893)) ;
#182058=CARTESIAN_POINT('Ctrl Pts',(-20.2551947657606,-14.5768444598646,
115.081818616712)) ;
#182059=CARTESIAN_POINT('Ctrl Pts',(-20.2575026754292,-14.501304829004,
115.088848135438)) ;
#182060=CARTESIAN_POINT('Ctrl Pts',(-20.3373604074522,-14.4893139259723,
115.367374582084)) ;
#182061=CARTESIAN_POINT('Ctrl Pts',(-20.3333659245991,-14.4144981524163,
115.355208030175)) ;
#182062=CARTESIAN_POINT('Ctrl Pts',(-20.2595621073134,-14.4144981369881,
115.379439151462)) ;
#182063=CARTESIAN_POINT('Ctrl Pts',(-20.1857582900276,-14.4144981215599,
115.403670272748)) ;
#182064=CARTESIAN_POINT('Ctrl Pts',(-20.1897527728807,-14.4893138951159,
115.415836824657)) ;
#182065=CARTESIAN_POINT('Ctrl Pts',(-20.1937472557339,-14.564129668672,
115.428003376567)) ;
#182066=CARTESIAN_POINT('Ctrl Pts',(-20.2675510730196,-14.5641296841002,
115.40377225528)) ;
#182067=CARTESIAN_POINT('Ctrl Pts',(-20.3413548903053,-14.5641296995284,
115.379541133994)) ;
#182068=CARTESIAN_POINT('Ctrl Pts',(-20.3373604074522,-14.4893139259723,
115.367374582084)) ;
#182069=CARTESIAN_POINT('Ctrl Pts',(-20.4135150495728,-14.4004454436412,
115.63486985746)) ;
#182070=CARTESIAN_POINT('Ctrl Pts',(-20.4034620789504,-14.3317211347541,
115.604250129488)) ;
#182071=CARTESIAN_POINT('Ctrl Pts',(-20.3296582572807,-14.331721100851,
115.628481237421)) ;
#182072=CARTESIAN_POINT('Ctrl Pts',(-20.255854435611,-14.331721066948,115.652712345355)) ;
#182073=CARTESIAN_POINT('Ctrl Pts',(-20.2659074062333,-14.4004453758351,
115.683332073327)) ;
#182074=CARTESIAN_POINT('Ctrl Pts',(-20.2759603768557,-14.4691696847222,
115.713951801299)) ;
#182075=CARTESIAN_POINT('Ctrl Pts',(-20.3497641985254,-14.4691697186253,
115.689720693366)) ;
#182076=CARTESIAN_POINT('Ctrl Pts',(-20.4235680201952,-14.4691697525284,
115.665489585432)) ;
#182077=CARTESIAN_POINT('Ctrl Pts',(-20.4135150495728,-14.4004454436412,
115.63486985746)) ;
#182078=CARTESIAN_POINT('Ctrl Pts',(-20.4788768821726,-14.2418718140722,
115.86930035727)) ;
#182079=CARTESIAN_POINT('Ctrl Pts',(-20.4635137429904,-14.1841154082224,
115.822506712786)) ;
#182080=CARTESIAN_POINT('Ctrl Pts',(-20.3897099161486,-14.1841153614757,
115.846737804967)) ;
#182081=CARTESIAN_POINT('Ctrl Pts',(-20.3159060893068,-14.1841153147289,
115.870968897147)) ;
#182082=CARTESIAN_POINT('Ctrl Pts',(-20.3312692284891,-14.2418717205788,
115.917762541631)) ;
#182083=CARTESIAN_POINT('Ctrl Pts',(-20.3466323676714,-14.2996281264286,
115.964556186114)) ;
#182084=CARTESIAN_POINT('Ctrl Pts',(-20.4204361945131,-14.2996281731753,
115.940325093934)) ;
#182085=CARTESIAN_POINT('Ctrl Pts',(-20.4942400213549,-14.299628219922,
115.916094001753)) ;
#182086=CARTESIAN_POINT('Ctrl Pts',(-20.4788768821726,-14.2418718140722,
115.86930035727)) ;
#182087=CARTESIAN_POINT('Ctrl Pts',(-20.5287019786929,-14.0233785235775,
116.056610441429)) ;
#182088=CARTESIAN_POINT('Ctrl Pts',(-20.5091010771396,-13.9807896305814,
115.996909256697)) ;
#182089=CARTESIAN_POINT('Ctrl Pts',(-20.4352972442419,-13.9807895787785,
116.021140330432)) ;
#182090=CARTESIAN_POINT('Ctrl Pts',(-20.3614934113443,-13.9807895269757,
116.045371404168)) ;
#182091=CARTESIAN_POINT('Ctrl Pts',(-20.3810943128976,-14.0233784199718,
116.105072588899)) ;
#182092=CARTESIAN_POINT('Ctrl Pts',(-20.4006952144509,-14.0659673129679,
116.16477377363)) ;
#182093=CARTESIAN_POINT('Ctrl Pts',(-20.4744990473485,-14.0659673647708,
116.140542699895)) ;
#182094=CARTESIAN_POINT('Ctrl Pts',(-20.5483028802461,-14.0659674165736,
116.11631162616)) ;
#182095=CARTESIAN_POINT('Ctrl Pts',(-20.5287019786929,-14.0233785235775,
116.056610441429)) ;
#182096=CARTESIAN_POINT('Ctrl Pts',(-20.5581714230433,-13.7618917263419,
116.181832379666)) ;
#182097=CARTESIAN_POINT('Ctrl Pts',(-20.5357493769413,-13.7374955038548,
116.113538443995)) ;
#182098=CARTESIAN_POINT('Ctrl Pts',(-20.4619455385341,-13.7374954531261,
116.137769500949)) ;
#182099=CARTESIAN_POINT('Ctrl Pts',(-20.3881417001269,-13.7374954023974,
116.162000557903)) ;
#182100=CARTESIAN_POINT('Ctrl Pts',(-20.4105637462289,-13.7618916248845,
116.230294493574)) ;
#182101=CARTESIAN_POINT('Ctrl Pts',(-20.4329857923308,-13.7862878473716,
116.298588429245)) ;
#182102=CARTESIAN_POINT('Ctrl Pts',(-20.506789630738,-13.7862878981003,
116.274357372291)) ;
#182103=CARTESIAN_POINT('Ctrl Pts',(-20.5805934691452,-13.786287948829,
116.250126315337)) ;
#182104=CARTESIAN_POINT('Ctrl Pts',(-20.5581714230433,-13.7618917263419,
116.181832379666)) ;
#182105=CARTESIAN_POINT('Ctrl Pts',(-20.5645519553757,-13.4754623735639,
116.236774706755)) ;
#182106=CARTESIAN_POINT('Ctrl Pts',(-20.5409155733802,-13.471028133492,
116.164782100062)) ;
#182107=CARTESIAN_POINT('Ctrl Pts',(-20.4671117304669,-13.4710280894286,
116.189013143291)) ;
#182108=CARTESIAN_POINT('Ctrl Pts',(-20.3933078875535,-13.4710280453652,
116.213244186519)) ;
#182109=CARTESIAN_POINT('Ctrl Pts',(-20.4169442695489,-13.4754622854371,
116.285236793213)) ;
#182110=CARTESIAN_POINT('Ctrl Pts',(-20.4405806515443,-13.479896525509,
116.357229399907)) ;
#182111=CARTESIAN_POINT('Ctrl Pts',(-20.5143844944577,-13.4798965695724,
116.332998356678)) ;
#182112=CARTESIAN_POINT('Ctrl Pts',(-20.5881883373711,-13.4798966136358,
116.308767313449)) ;
#182113=CARTESIAN_POINT('Ctrl Pts',(-20.5645519553757,-13.4754623735639,
116.236774706755)) ;
#182114=CARTESIAN_POINT('Ctrl Pts',(-20.5467688213249,-13.1862230579374,
116.217949995558)) ;
#182115=CARTESIAN_POINT('Ctrl Pts',(-20.523607060582,-13.2019774295457,
116.147403008764)) ;
#182116=CARTESIAN_POINT('Ctrl Pts',(-20.4498032145121,-13.2019773939464,
116.171634042378)) ;
#182117=CARTESIAN_POINT('Ctrl Pts',(-20.3759993684423,-13.2019773583471,
116.195865075993)) ;
#182118=CARTESIAN_POINT('Ctrl Pts',(-20.3991611291852,-13.1862229867387,
116.266412062787)) ;
#182119=CARTESIAN_POINT('Ctrl Pts',(-20.4223228899281,-13.1704686151304,
116.336959049582)) ;
#182120=CARTESIAN_POINT('Ctrl Pts',(-20.4961267359979,-13.1704686507297,
116.312728015967)) ;
#182121=CARTESIAN_POINT('Ctrl Pts',(-20.5699305820678,-13.170468686329,
116.288496982352)) ;
#182122=CARTESIAN_POINT('Ctrl Pts',(-20.5467688213249,-13.1862230579374,
116.217949995558)) ;
#182123=CARTESIAN_POINT('Ctrl Pts',(-20.5051147908571,-12.9121173454345,
116.12661145186)) ;
#182124=CARTESIAN_POINT('Ctrl Pts',(-20.4840909773503,-12.9470346448942,
116.062576307566)) ;
#182125=CARTESIAN_POINT('Ctrl Pts',(-20.4102871297331,-12.947034620835,
116.086807336468)) ;
#182126=CARTESIAN_POINT('Ctrl Pts',(-20.3364832821159,-12.9470345967758,
116.111038365369)) ;
#182127=CARTESIAN_POINT('Ctrl Pts',(-20.3575070956226,-12.9121172973162,
116.175073509663)) ;
#182128=CARTESIAN_POINT('Ctrl Pts',(-20.3785309091293,-12.8771999978565,
116.239108653958)) ;
#182129=CARTESIAN_POINT('Ctrl Pts',(-20.4523347567466,-12.8772000219157,
116.214877625056)) ;
#182130=CARTESIAN_POINT('Ctrl Pts',(-20.5261386043638,-12.8772000459749,
116.190646596154)) ;
#182131=CARTESIAN_POINT('Ctrl Pts',(-20.5051147908571,-12.9121173454345,
116.12661145186)) ;
#182132=CARTESIAN_POINT('Ctrl Pts',(-20.4420769531017,-12.6748571224349,
115.970037261179)) ;
#182133=CARTESIAN_POINT('Ctrl Pts',(-20.4246897099179,-12.7263936809792,
115.917078523479)) ;
#182134=CARTESIAN_POINT('Ctrl Pts',(-20.350885862107,-12.7263936670357,
115.941309551791)) ;
#182135=CARTESIAN_POINT('Ctrl Pts',(-20.2770820142961,-12.7263936530922,
115.965540580103)) ;
#182136=CARTESIAN_POINT('Ctrl Pts',(-20.2944692574799,-12.6748570945479,
116.018499317803)) ;
#182137=CARTESIAN_POINT('Ctrl Pts',(-20.3118565006636,-12.6233205360036,
116.071458055503)) ;
#182138=CARTESIAN_POINT('Ctrl Pts',(-20.3856603484746,-12.6233205499471,
116.047227027191)) ;
#182139=CARTESIAN_POINT('Ctrl Pts',(-20.4594641962855,-12.6233205638906,
116.02299599888)) ;
#182140=CARTESIAN_POINT('Ctrl Pts',(-20.4420769531017,-12.6748571224349,
115.970037261179)) ;
#182141=CARTESIAN_POINT('Ctrl Pts',(-20.3606399883835,-12.4898752939566,
115.757680794649)) ;
#182142=CARTESIAN_POINT('Ctrl Pts',(-20.3481742578633,-12.5544068109691,
115.71971219061)) ;
#182143=CARTESIAN_POINT('Ctrl Pts',(-20.274370411419,-12.5544068057079,
115.743943223084)) ;
#182144=CARTESIAN_POINT('Ctrl Pts',(-20.2005665649747,-12.5544068004467,
115.768174255558)) ;
#182145=CARTESIAN_POINT('Ctrl Pts',(-20.2130322954949,-12.4898752834342,
115.806142859598)) ;
#182146=CARTESIAN_POINT('Ctrl Pts',(-20.2254980260151,-12.4253437664217,
115.844111463637)) ;
#182147=CARTESIAN_POINT('Ctrl Pts',(-20.2993018724594,-12.4253437716829,
115.819880431163)) ;
#182148=CARTESIAN_POINT('Ctrl Pts',(-20.3731057189037,-12.4253437769441,
115.795649398689)) ;
#182149=CARTESIAN_POINT('Ctrl Pts',(-20.3606399883835,-12.4898752939566,
115.757680794649)) ;
#182150=CARTESIAN_POINT('Ctrl Pts',(-20.267669228754,-12.3730682967797,
115.5097223699)) ;
#182151=CARTESIAN_POINT('Ctrl Pts',(-20.2609477177173,-12.4458523869168,
115.489249731667)) ;
#182152=CARTESIAN_POINT('Ctrl Pts',(-20.1871438723082,-12.4458523855329,
115.513480767294)) ;
#182153=CARTESIAN_POINT('Ctrl Pts',(-20.113340026899,-12.445852384149,115.537711802922)) ;
#182154=CARTESIAN_POINT('Ctrl Pts',(-20.1200615379358,-12.3730682940119,
115.558184441155)) ;
#182155=CARTESIAN_POINT('Ctrl Pts',(-20.1267830489725,-12.3002842038747,
115.578657079388)) ;
#182156=CARTESIAN_POINT('Ctrl Pts',(-20.2005868943816,-12.3002842052586,
115.55442604376)) ;
#182157=CARTESIAN_POINT('Ctrl Pts',(-20.2743907397907,-12.3002842066425,
115.530195008133)) ;
#182158=CARTESIAN_POINT('Ctrl Pts',(-20.267669228754,-12.3730682967797,
115.5097223699)) ;
#182159=CARTESIAN_POINT('Ctrl Pts',(-20.166688706548,-12.330125354393,115.237846370994)) ;
#182160=CARTESIAN_POINT('Ctrl Pts',(-20.1662696956355,-12.4060180175289,
115.236570131351)) ;
#182161=CARTESIAN_POINT('Ctrl Pts',(-20.092465852039,-12.4060180179283,
115.260801172499)) ;
#182162=CARTESIAN_POINT('Ctrl Pts',(-20.0186620084424,-12.4060180183277,
115.285032213647)) ;
#182163=CARTESIAN_POINT('Ctrl Pts',(-20.0190810193549,-12.3301253551918,
115.286308453291)) ;
#182164=CARTESIAN_POINT('Ctrl Pts',(-20.0195000302674,-12.2542326920559,
115.287584692934)) ;
#182165=CARTESIAN_POINT('Ctrl Pts',(-20.0933038738639,-12.2542326916565,
115.263353651786)) ;
#182166=CARTESIAN_POINT('Ctrl Pts',(-20.1671077174604,-12.2542326912571,
115.239122610638)) ;
#182167=CARTESIAN_POINT('Ctrl Pts',(-20.166688706548,-12.330125354393,115.237846370994)) ;
#182168=CARTESIAN_POINT('Ctrl Pts',(-20.0667473533349,-12.3650026478225,
114.968634787347)) ;
#182169=CARTESIAN_POINT('Ctrl Pts',(-20.0725778668182,-12.4385726507877,
114.986393590701)) ;
#182170=CARTESIAN_POINT('Ctrl Pts',(-19.9987740239603,-12.4385726504867,
115.010624634099)) ;
#182171=CARTESIAN_POINT('Ctrl Pts',(-19.9249701811023,-12.4385726501857,
115.034855677496)) ;
#182172=CARTESIAN_POINT('Ctrl Pts',(-19.9191396676191,-12.3650026472205,
115.017096874142)) ;
#182173=CARTESIAN_POINT('Ctrl Pts',(-19.9133091541358,-12.2914326442552,
114.999338070788)) ;
#182174=CARTESIAN_POINT('Ctrl Pts',(-19.9871129969937,-12.2914326445563,
114.97510702739)) ;
#182175=CARTESIAN_POINT('Ctrl Pts',(-20.0609168398517,-12.2914326448573,
114.950875983992)) ;
#182176=CARTESIAN_POINT('Ctrl Pts',(-20.0667473533349,-12.3650026478225,
114.968634787347)) ;
#182177=CARTESIAN_POINT('Ctrl Pts',(-19.9714448335891,-12.4764750890778,
114.714120708034)) ;
#182178=CARTESIAN_POINT('Ctrl Pts',(-19.9831991431023,-12.5423709931459,
114.749922438328)) ;
#182179=CARTESIAN_POINT('Ctrl Pts',(-19.9093953006452,-12.5423709914641,
114.774153482947)) ;
#182180=CARTESIAN_POINT('Ctrl Pts',(-19.8355914581881,-12.5423709897823,
114.798384527565)) ;
#182181=CARTESIAN_POINT('Ctrl Pts',(-19.8238371486749,-12.4764750857142,
114.762582797271)) ;
#182182=CARTESIAN_POINT('Ctrl Pts',(-19.8120828391616,-12.410579181646,
114.726781066978)) ;
#182183=CARTESIAN_POINT('Ctrl Pts',(-19.8858866816187,-12.4105791833278,
114.702550022359)) ;
#182184=CARTESIAN_POINT('Ctrl Pts',(-19.9596905240758,-12.4105791850096,
114.67831897774)) ;
#182185=CARTESIAN_POINT('Ctrl Pts',(-19.9714448335891,-12.4764750890778,
114.714120708034)) ;
#182186=CARTESIAN_POINT('Ctrl Pts',(-19.8896127307638,-12.6535586984017,
114.500104289073)) ;
#182187=CARTESIAN_POINT('Ctrl Pts',(-19.9063692751628,-12.7071860625279,
114.551142019704)) ;
#182188=CARTESIAN_POINT('Ctrl Pts',(-19.8325654322624,-12.7071860605199,
114.575373062973)) ;
#182189=CARTESIAN_POINT('Ctrl Pts',(-19.758761589362,-12.7071860585118,
114.599604106241)) ;
#182190=CARTESIAN_POINT('Ctrl Pts',(-19.742005044963,-12.6535586943856,
114.54856637561)) ;
#182191=CARTESIAN_POINT('Ctrl Pts',(-19.7252485005639,-12.5999313302593,
114.497528644979)) ;
#182192=CARTESIAN_POINT('Ctrl Pts',(-19.7990523434643,-12.5999313322674,
114.473297601711)) ;
#182193=CARTESIAN_POINT('Ctrl Pts',(-19.8728561863647,-12.5999313342754,
114.449066558443)) ;
#182194=CARTESIAN_POINT('Ctrl Pts',(-19.8896127307638,-12.6535586984017,
114.500104289073)) ;
#182195=CARTESIAN_POINT('Ctrl Pts',(-19.8242138693162,-12.8875907025722,
114.33656955619)) ;
#182196=CARTESIAN_POINT('Ctrl Pts',(-19.8448239027325,-12.9249550568961,
114.399344392539)) ;
#182197=CARTESIAN_POINT('Ctrl Pts',(-19.7710200590923,-12.9249550576415,
114.423575433555)) ;
#182198=CARTESIAN_POINT('Ctrl Pts',(-19.6972162154521,-12.9249550583868,
114.44780647457)) ;
#182199=CARTESIAN_POINT('Ctrl Pts',(-19.6766061820359,-12.887590704063,
114.385031638221)) ;
#182200=CARTESIAN_POINT('Ctrl Pts',(-19.6559961486197,-12.8502263497391,
114.322256801871)) ;
#182201=CARTESIAN_POINT('Ctrl Pts',(-19.7297999922599,-12.8502263489938,
114.298025760856)) ;
#182202=CARTESIAN_POINT('Ctrl Pts',(-19.8036038359,-12.8502263482484,114.273794719841)) ;
#182203=CARTESIAN_POINT('Ctrl Pts',(-19.8242138693162,-12.8875907025722,
114.33656955619)) ;
#182204=CARTESIAN_POINT('Ctrl Pts',(-19.7806786916706,-13.1564738506933,
114.239166113218)) ;
#182205=CARTESIAN_POINT('Ctrl Pts',(-19.8036300452104,-13.1751180004759,
114.30907223283)) ;
#182206=CARTESIAN_POINT('Ctrl Pts',(-19.7298262013386,-13.1751180045343,
114.333303273139)) ;
#182207=CARTESIAN_POINT('Ctrl Pts',(-19.6560223574667,-13.1751180085928,
114.357534313449)) ;
#182208=CARTESIAN_POINT('Ctrl Pts',(-19.633071003927,-13.1564738588101,
114.287628193837)) ;
#182209=CARTESIAN_POINT('Ctrl Pts',(-19.6101196503872,-13.1378297090275,
114.217722074225)) ;
#182210=CARTESIAN_POINT('Ctrl Pts',(-19.6839234942591,-13.1378297049691,
114.193491033915)) ;
#182211=CARTESIAN_POINT('Ctrl Pts',(-19.7577273381309,-13.1378297009107,
114.169259993606)) ;
#182212=CARTESIAN_POINT('Ctrl Pts',(-19.7806786916706,-13.1564738506933,
114.239166113218)) ;
#182213=CARTESIAN_POINT('Ctrl Pts',(-19.7602296026469,-13.4476180482474,
114.212556713675)) ;
#182214=CARTESIAN_POINT('Ctrl Pts',(-19.7839041995415,-13.4459601626287,
114.284665715712)) ;
#182215=CARTESIAN_POINT('Ctrl Pts',(-19.7101003560251,-13.4459601740975,
114.308896757104)) ;
#182216=CARTESIAN_POINT('Ctrl Pts',(-19.6362965125087,-13.4459601855664,
114.333127798496)) ;
#182217=CARTESIAN_POINT('Ctrl Pts',(-19.6126219156141,-13.4476180711851,
114.261018796459)) ;
#182218=CARTESIAN_POINT('Ctrl Pts',(-19.5889473187195,-13.4492759568038,
114.188909794422)) ;
#182219=CARTESIAN_POINT('Ctrl Pts',(-19.6627511622359,-13.4492759453349,
114.16467875303)) ;
#182220=CARTESIAN_POINT('Ctrl Pts',(-19.7365550057523,-13.4492759338661,
114.140447711637)) ;
#182221=CARTESIAN_POINT('Ctrl Pts',(-19.7602296026469,-13.4476180482474,
114.212556713675)) ;
#182222=CARTESIAN_POINT('Ctrl Pts',(-19.7643490688689,-13.7346448783816,
114.260518004658)) ;
#182223=CARTESIAN_POINT('Ctrl Pts',(-19.7870375076896,-13.7129435340765,
114.329623328187)) ;
#182224=CARTESIAN_POINT('Ctrl Pts',(-19.713233665749,-13.7129435517169,
114.353854374379)) ;
#182225=CARTESIAN_POINT('Ctrl Pts',(-19.6394298238083,-13.7129435693573,
114.378085420571)) ;
#182226=CARTESIAN_POINT('Ctrl Pts',(-19.6167413849876,-13.7346449136625,
114.308980097041)) ;
#182227=CARTESIAN_POINT('Ctrl Pts',(-19.5940529461669,-13.7563462579677,
114.239874773512)) ;
#182228=CARTESIAN_POINT('Ctrl Pts',(-19.6678567881075,-13.7563462403272,
114.21564372732)) ;
#182229=CARTESIAN_POINT('Ctrl Pts',(-19.7416606300482,-13.7563462226868,
114.191412681128)) ;
#182230=CARTESIAN_POINT('Ctrl Pts',(-19.7643490688689,-13.7346448783816,
114.260518004658)) ;
#182231=CARTESIAN_POINT('Ctrl Pts',(-19.7916546783398,-13.9993799399049,
114.37915348673)) ;
#182232=CARTESIAN_POINT('Ctrl Pts',(-19.811735534808,-13.9591628378215,
114.440316534995)) ;
#182233=CARTESIAN_POINT('Ctrl Pts',(-19.7379316955588,-13.9591628601971,
114.464547589384)) ;
#182234=CARTESIAN_POINT('Ctrl Pts',(-19.6641278563097,-13.9591628825727,
114.488778643774)) ;
#182235=CARTESIAN_POINT('Ctrl Pts',(-19.6440469998415,-13.9993799846561,
114.427615595509)) ;
#182236=CARTESIAN_POINT('Ctrl Pts',(-19.6239661433733,-14.0395970867396,
114.366452547245)) ;
#182237=CARTESIAN_POINT('Ctrl Pts',(-19.6977699826225,-14.0395970643639,
114.342221492855)) ;
#182238=CARTESIAN_POINT('Ctrl Pts',(-19.7715738218716,-14.0395970419883,
114.317990438466)) ;
#182239=CARTESIAN_POINT('Ctrl Pts',(-19.7916546783398,-13.9993799399049,
114.37915348673)) ;
#182240=CARTESIAN_POINT('Ctrl Pts',(-19.8393939276307,-14.2219559568416,
114.559939768172)) ;
#182241=CARTESIAN_POINT('Ctrl Pts',(-19.8554384541888,-14.1661403968853,
114.608808806644)) ;
#182242=CARTESIAN_POINT('Ctrl Pts',(-19.7816346183794,-14.1661404199882,
114.63303987151)) ;
#182243=CARTESIAN_POINT('Ctrl Pts',(-19.7078307825699,-14.166140443091,
114.657270936377)) ;
#182244=CARTESIAN_POINT('Ctrl Pts',(-19.6917862560118,-14.2219560030472,
114.608401897904)) ;
#182245=CARTESIAN_POINT('Ctrl Pts',(-19.6757417294536,-14.2777715630035,
114.559532859432)) ;
#182246=CARTESIAN_POINT('Ctrl Pts',(-19.7495455652631,-14.2777715399007,
114.535301794566)) ;
#182247=CARTESIAN_POINT('Ctrl Pts',(-19.8233494010725,-14.2777715167979,
114.511070729699)) ;
#182248=CARTESIAN_POINT('Ctrl Pts',(-19.8393939276307,-14.2219559568416,
114.559939768172)) ;
#182249=CARTESIAN_POINT('Ctrl Pts',(-19.9035549276073,-14.3877271051732,
114.790823935463)) ;
#182250=CARTESIAN_POINT('Ctrl Pts',(-19.9144091659851,-14.3202567503196,
114.823884193423)) ;
#182251=CARTESIAN_POINT('Ctrl Pts',(-19.8406053341715,-14.3202567702551,
114.84811527046)) ;
#182252=CARTESIAN_POINT('Ctrl Pts',(-19.7668015023578,-14.3202567901906,
114.872346347496)) ;
#182253=CARTESIAN_POINT('Ctrl Pts',(-19.75594726398,-14.3877271450442,114.839286089537)) ;
#182254=CARTESIAN_POINT('Ctrl Pts',(-19.7450930256021,-14.4551974998978,
114.806225831578)) ;
#182255=CARTESIAN_POINT('Ctrl Pts',(-19.8188968574157,-14.4551974799623,
114.781994754541)) ;
#182256=CARTESIAN_POINT('Ctrl Pts',(-19.8927006892294,-14.4551974600268,
114.757763677504)) ;
#182257=CARTESIAN_POINT('Ctrl Pts',(-19.9035549276073,-14.3877271051732,
114.790823935463)) ;
#182258=CARTESIAN_POINT('Ctrl Pts',(-19.9791956729631,-14.4840522417127,
115.05686055136)) ;
#182259=CARTESIAN_POINT('Ctrl Pts',(-19.9840468444247,-14.4097585017527,
115.07163643588)) ;
#182260=CARTESIAN_POINT('Ctrl Pts',(-19.9102430170675,-14.4097585129656,
115.095867526491)) ;
#182261=CARTESIAN_POINT('Ctrl Pts',(-19.8364391897103,-14.4097585241785,
115.120098617101)) ;
#182262=CARTESIAN_POINT('Ctrl Pts',(-19.8315880182487,-14.4840522641385,
115.105322732581)) ;
#182263=CARTESIAN_POINT('Ctrl Pts',(-19.8267368467871,-14.5583460040984,
115.090546848061)) ;
#182264=CARTESIAN_POINT('Ctrl Pts',(-19.9005406741443,-14.5583459928856,
115.06631575745)) ;
#182265=CARTESIAN_POINT('Ctrl Pts',(-19.9743445015015,-14.5583459816727,
115.04208466684)) ;
#182266=CARTESIAN_POINT('Ctrl Pts',(-19.9791956729631,-14.4840522417127,
115.05686055136)) ;
#182267=CARTESIAN_POINT('Ctrl Pts',(-20.0588167420593,-14.5035551456864,
115.334617178698)) ;
#182268=CARTESIAN_POINT('Ctrl Pts',(-20.057386595992,-14.4277930448145,
115.330261183388)) ;
#182269=CARTESIAN_POINT('Ctrl Pts',(-19.9835827710018,-14.4277930415592,
115.354492281207)) ;
#182270=CARTESIAN_POINT('Ctrl Pts',(-19.9097789460115,-14.427793038304,
115.378723379027)) ;
#182271=CARTESIAN_POINT('Ctrl Pts',(-19.9112090920788,-14.503555139176,
115.383079374337)) ;
#182272=CARTESIAN_POINT('Ctrl Pts',(-19.912639238146,-14.579317240048,115.387435369648)) ;
#182273=CARTESIAN_POINT('Ctrl Pts',(-19.9864430631363,-14.5793172433032,
115.363204271828)) ;
#182274=CARTESIAN_POINT('Ctrl Pts',(-20.0602468881266,-14.5793172465584,
115.338973174008)) ;
#182275=CARTESIAN_POINT('Ctrl Pts',(-20.0588167420593,-14.5035551456864,
115.334617178698)) ;
#182276=CARTESIAN_POINT('Ctrl Pts',(-20.1375552337769,-14.4455933724693,
115.610012047624)) ;
#182277=CARTESIAN_POINT('Ctrl Pts',(-20.1298896565059,-14.3737681183539,
115.58666393477)) ;
#182278=CARTESIAN_POINT('Ctrl Pts',(-20.0560858333493,-14.3737680965987,
115.610895038174)) ;
#182279=CARTESIAN_POINT('Ctrl Pts',(-19.9822820101926,-14.3737680748436,
115.635126141579)) ;
#182280=CARTESIAN_POINT('Ctrl Pts',(-19.9899475874636,-14.445593328959,
115.658474254434)) ;
#182281=CARTESIAN_POINT('Ctrl Pts',(-19.9976131647346,-14.5174185830743,
115.681822367288)) ;
#182282=CARTESIAN_POINT('Ctrl Pts',(-20.0714169878912,-14.5174186048295,
115.657591263883)) ;
#182283=CARTESIAN_POINT('Ctrl Pts',(-20.1452208110478,-14.5174186265847,
115.633360160479)) ;
#182284=CARTESIAN_POINT('Ctrl Pts',(-20.1375552337769,-14.4455933724693,
115.610012047624)) ;
#182285=CARTESIAN_POINT('Ctrl Pts',(-20.2080701569904,-14.3137077173971,
115.860269168483)) ;
#182286=CARTESIAN_POINT('Ctrl Pts',(-20.1947361462872,-14.2509862906075,
115.819655921839)) ;
#182287=CARTESIAN_POINT('Ctrl Pts',(-20.1209323226071,-14.2509862477117,
115.843887023649)) ;
#182288=CARTESIAN_POINT('Ctrl Pts',(-20.0471284989271,-14.2509862048158,
115.86811812546)) ;
#182289=CARTESIAN_POINT('Ctrl Pts',(-20.0604625096304,-14.3137076316054,
115.908731372104)) ;
#182290=CARTESIAN_POINT('Ctrl Pts',(-20.0737965203336,-14.3764290583951,
115.949344618748)) ;
#182291=CARTESIAN_POINT('Ctrl Pts',(-20.1476003440137,-14.3764291012909,
115.925113516938)) ;
#182292=CARTESIAN_POINT('Ctrl Pts',(-20.2214041676937,-14.3764291441867,
115.900882415128)) ;
#182293=CARTESIAN_POINT('Ctrl Pts',(-20.2080701569904,-14.3137077173971,
115.860269168483)) ;
#182294=CARTESIAN_POINT('Ctrl Pts',(-20.2646911851614,-14.118290994482,
116.068126903514)) ;
#182295=CARTESIAN_POINT('Ctrl Pts',(-20.2466522852371,-14.0691221426053,
116.013183323304)) ;
#182296=CARTESIAN_POINT('Ctrl Pts',(-20.1728484586584,-14.0691220793387,
116.037414416285)) ;
#182297=CARTESIAN_POINT('Ctrl Pts',(-20.0990446320796,-14.0691220160722,
116.061645509267)) ;
#182298=CARTESIAN_POINT('Ctrl Pts',(-20.1170835320039,-14.1182908679489,
116.116589089477)) ;
#182299=CARTESIAN_POINT('Ctrl Pts',(-20.1351224319283,-14.1674597198256,
116.171532669688)) ;
#182300=CARTESIAN_POINT('Ctrl Pts',(-20.208926258507,-14.1674597830921,
116.147301576706)) ;
#182301=CARTESIAN_POINT('Ctrl Pts',(-20.2827300850857,-14.1674598463587,
116.123070483725)) ;
#182302=CARTESIAN_POINT('Ctrl Pts',(-20.2646911851614,-14.118290994482,
116.068126903514)) ;
#182303=CARTESIAN_POINT('Ctrl Pts',(-20.3028224443455,-13.8721339097932,
116.21976440383)) ;
#182304=CARTESIAN_POINT('Ctrl Pts',(-20.2813606322499,-13.840079359465,
116.1543951853)) ;
#182305=CARTESIAN_POINT('Ctrl Pts',(-20.2075568006751,-13.8400792780125,
116.178626263064)) ;
#182306=CARTESIAN_POINT('Ctrl Pts',(-20.1337529691003,-13.8400791965599,
116.202857340829)) ;
#182307=CARTESIAN_POINT('Ctrl Pts',(-20.1552147811959,-13.872133746888,
116.268226559358)) ;
#182308=CARTESIAN_POINT('Ctrl Pts',(-20.1766765932915,-13.9041882972162,
116.333595777888)) ;
#182309=CARTESIAN_POINT('Ctrl Pts',(-20.2504804248663,-13.9041883786687,
116.309364700123)) ;
#182310=CARTESIAN_POINT('Ctrl Pts',(-20.3242842564411,-13.9041884601213,
116.285133622359)) ;
#182311=CARTESIAN_POINT('Ctrl Pts',(-20.3028224443455,-13.8721339097932,
116.21976440383)) ;
#182312=CARTESIAN_POINT('Ctrl Pts',(-20.3188675383437,-13.5943341067766,
116.304015063102)) ;
#182313=CARTESIAN_POINT('Ctrl Pts',(-20.2955222534172,-13.5816279445403,
116.232909090126)) ;
#182314=CARTESIAN_POINT('Ctrl Pts',(-20.2217184149583,-13.5816278507647,
116.257140146922)) ;
#182315=CARTESIAN_POINT('Ctrl Pts',(-20.1479145764994,-13.5816277569891,
116.281371203719)) ;
#182316=CARTESIAN_POINT('Ctrl Pts',(-20.1712598614258,-13.5943339192254,
116.352477176694)) ;
#182317=CARTESIAN_POINT('Ctrl Pts',(-20.1946051463523,-13.6070400814617,
116.42358314967)) ;
#182318=CARTESIAN_POINT('Ctrl Pts',(-20.2684089848112,-13.6070401752373,
116.399352092874)) ;
#182319=CARTESIAN_POINT('Ctrl Pts',(-20.3422128232701,-13.6070402690129,
116.375121036078)) ;
#182320=CARTESIAN_POINT('Ctrl Pts',(-20.3188675383437,-13.5943341067766,
116.304015063102)) ;
#182321=CARTESIAN_POINT('Ctrl Pts',(-20.310817084727,-13.3016132059809,
116.315163697483)) ;
#182322=CARTESIAN_POINT('Ctrl Pts',(-20.2872614887352,-13.309324862532,
116.243417150824)) ;
#182323=CARTESIAN_POINT('Ctrl Pts',(-20.2134576420664,-13.3093247622356,
116.267648182615)) ;
#182324=CARTESIAN_POINT('Ctrl Pts',(-20.1396537953975,-13.3093246619392,
116.291879214405)) ;
#182325=CARTESIAN_POINT('Ctrl Pts',(-20.1632093913893,-13.3016130053881,
116.363625761064)) ;
#182326=CARTESIAN_POINT('Ctrl Pts',(-20.1867649873811,-13.293901348837,
116.435372307722)) ;
#182327=CARTESIAN_POINT('Ctrl Pts',(-20.2605688340499,-13.2939014491334,
116.411141275932)) ;
#182328=CARTESIAN_POINT('Ctrl Pts',(-20.3343726807187,-13.2939015494298,
116.386910244142)) ;
#182329=CARTESIAN_POINT('Ctrl Pts',(-20.310817084727,-13.3016132059809,
116.315163697483)) ;
#182330=CARTESIAN_POINT('Ctrl Pts',(-20.2787910861107,-13.0203974601351,
116.252886906067)) ;
#182331=CARTESIAN_POINT('Ctrl Pts',(-20.2567073240818,-13.0477539673653,
116.185623328126)) ;
#182332=CARTESIAN_POINT('Ctrl Pts',(-20.182903468911,-13.0477538708474,
116.209854334021)) ;
#182333=CARTESIAN_POINT('Ctrl Pts',(-20.1090996137403,-13.0477537743296,
116.234085339916)) ;
#182334=CARTESIAN_POINT('Ctrl Pts',(-20.1311833757692,-13.0203972670994,
116.301348917857)) ;
#182335=CARTESIAN_POINT('Ctrl Pts',(-20.1532671377981,-12.9930407598692,
116.368612495798)) ;
#182336=CARTESIAN_POINT('Ctrl Pts',(-20.2270709929689,-12.9930408563871,
116.344381489903)) ;
#182337=CARTESIAN_POINT('Ctrl Pts',(-20.3008748481397,-12.9930409529049,
116.320150484008)) ;
#182338=CARTESIAN_POINT('Ctrl Pts',(-20.2787910861107,-13.0203974601351,
116.252886906067)) ;
#182339=CARTESIAN_POINT('Ctrl Pts',(-20.2240804356435,-12.7657619407627,
116.121738912419)) ;
#182340=CARTESIAN_POINT('Ctrl Pts',(-20.2050494897071,-12.8109362194434,
116.06377371967)) ;
#182341=CARTESIAN_POINT('Ctrl Pts',(-20.1312456264214,-12.8109361340697,
116.088004700848)) ;
#182342=CARTESIAN_POINT('Ctrl Pts',(-20.0574417631357,-12.810936048696,
116.112235682026)) ;
#182343=CARTESIAN_POINT('Ctrl Pts',(-20.076472709072,-12.7657617700153,
116.170200874775)) ;
#182344=CARTESIAN_POINT('Ctrl Pts',(-20.0955036550083,-12.7205874913346,
116.228166067524)) ;
#182345=CARTESIAN_POINT('Ctrl Pts',(-20.1693075182941,-12.7205875767083,
116.203935086346)) ;
#182346=CARTESIAN_POINT('Ctrl Pts',(-20.2431113815798,-12.720587662082,
116.179704105168)) ;
#182347=CARTESIAN_POINT('Ctrl Pts',(-20.2240804356435,-12.7657619407627,
116.121738912419)) ;
#182348=CARTESIAN_POINT('Ctrl Pts',(-20.149613612166,-12.5577255499837,
115.930492489718)) ;
#182349=CARTESIAN_POINT('Ctrl Pts',(-20.1350175403921,-12.6174909098253,
115.886035208073)) ;
#182350=CARTESIAN_POINT('Ctrl Pts',(-20.0612136703226,-12.6174908436088,
115.910266168589)) ;
#182351=CARTESIAN_POINT('Ctrl Pts',(-19.9874098002531,-12.6174907773923,
115.934497129104)) ;
#182352=CARTESIAN_POINT('Ctrl Pts',(-20.002005872027,-12.5577254175507,
115.97895441075)) ;
#182353=CARTESIAN_POINT('Ctrl Pts',(-20.0166019438008,-12.497960057709,
116.023411692395)) ;
#182354=CARTESIAN_POINT('Ctrl Pts',(-20.0904058138703,-12.4979601239256,
115.999180731879)) ;
#182355=CARTESIAN_POINT('Ctrl Pts',(-20.1642096839398,-12.4979601901421,
115.974949771364)) ;
#182356=CARTESIAN_POINT('Ctrl Pts',(-20.149613612166,-12.5577255499837,
115.930492489718)) ;
#182357=CARTESIAN_POINT('Ctrl Pts',(-20.0607208453583,-12.4120606642955,
115.695117936638)) ;
#182358=CARTESIAN_POINT('Ctrl Pts',(-20.0515773677667,-12.4820840248362,
115.667268377092)) ;
#182359=CARTESIAN_POINT('Ctrl Pts',(-19.9777734930595,-12.482083983576,
115.691499323482)) ;
#182360=CARTESIAN_POINT('Ctrl Pts',(-19.9039696183523,-12.4820839423157,
115.715730269872)) ;
#182361=CARTESIAN_POINT('Ctrl Pts',(-19.913113095944,-12.412060581775,115.743579829418)) ;
#182362=CARTESIAN_POINT('Ctrl Pts',(-19.9222565735356,-12.3420372212343,
115.771429388964)) ;
#182363=CARTESIAN_POINT('Ctrl Pts',(-19.9960604482428,-12.3420372624946,
115.747198442574)) ;
#182364=CARTESIAN_POINT('Ctrl Pts',(-20.06986432295,-12.3420373037548,115.722967496184)) ;
#182365=CARTESIAN_POINT('Ctrl Pts',(-20.0607208453583,-12.4120606642955,
115.695117936638)) ;
#182366=CARTESIAN_POINT('Ctrl Pts',(-19.9618159399851,-12.3380220880362,
115.429525652929)) ;
#182367=CARTESIAN_POINT('Ctrl Pts',(-19.9588261722604,-12.4133190427032,
115.420419300761)) ;
#182368=CARTESIAN_POINT('Ctrl Pts',(-19.8850222955982,-12.4133190298849,
115.444650241197)) ;
#182369=CARTESIAN_POINT('Ctrl Pts',(-19.811218418936,-12.4133190170666,
115.468881181632)) ;
#182370=CARTESIAN_POINT('Ctrl Pts',(-19.8142081866607,-12.3380220623996,
115.477987533799)) ;
#182371=CARTESIAN_POINT('Ctrl Pts',(-19.8171979543855,-12.2627251077326,
115.487093885967)) ;
#182372=CARTESIAN_POINT('Ctrl Pts',(-19.8910018310476,-12.2627251205509,
115.462862945531)) ;
#182373=CARTESIAN_POINT('Ctrl Pts',(-19.9648057077098,-12.2627251333692,
115.438632005096)) ;
#182374=CARTESIAN_POINT('Ctrl Pts',(-19.9618159399851,-12.3380220880362,
115.429525652929)) ;
#182375=CARTESIAN_POINT('Ctrl Pts',(-19.8611741252131,-12.3416277493325,
115.158205582033)) ;
#182376=CARTESIAN_POINT('Ctrl Pts',(-19.8644777699935,-12.4167843477481,
115.168267948947)) ;
#182377=CARTESIAN_POINT('Ctrl Pts',(-19.7906738939163,-12.4167843633384,
115.192498891164)) ;
#182378=CARTESIAN_POINT('Ctrl Pts',(-19.7168700178391,-12.4167843789286,
115.216729833381)) ;
#182379=CARTESIAN_POINT('Ctrl Pts',(-19.7135663730587,-12.3416277805131,
115.206667466468)) ;
#182380=CARTESIAN_POINT('Ctrl Pts',(-19.7102627282783,-12.2664711820975,
115.196605099554)) ;
#182381=CARTESIAN_POINT('Ctrl Pts',(-19.7840666043555,-12.2664711665072,
115.172374157337)) ;
#182382=CARTESIAN_POINT('Ctrl Pts',(-19.8578704804326,-12.266471150917,
115.14814321512)) ;
#182383=CARTESIAN_POINT('Ctrl Pts',(-19.8611741252131,-12.3416277493325,
115.158205582033)) ;
#182384=CARTESIAN_POINT('Ctrl Pts',(-19.7631652821149,-12.4221117178776,
114.895226151352)) ;
#182385=CARTESIAN_POINT('Ctrl Pts',(-19.7725811313252,-12.4917616411482,
114.923905306819)) ;
#182386=CARTESIAN_POINT('Ctrl Pts',(-19.6987772586223,-12.4917616828604,
114.948136259314)) ;
#182387=CARTESIAN_POINT('Ctrl Pts',(-19.6249733859194,-12.4917617245726,
114.972367211809)) ;
#182388=CARTESIAN_POINT('Ctrl Pts',(-19.6155575367091,-12.422111801302,
114.943688056342)) ;
#182389=CARTESIAN_POINT('Ctrl Pts',(-19.6061416874989,-12.3524618780314,
114.915008900874)) ;
#182390=CARTESIAN_POINT('Ctrl Pts',(-19.6799455602017,-12.3524618363192,
114.89077794838)) ;
#182391=CARTESIAN_POINT('Ctrl Pts',(-19.7537494329046,-12.3524617946069,
114.866546995885)) ;
#182392=CARTESIAN_POINT('Ctrl Pts',(-19.7631652821149,-12.4221117178776,
114.895226151352)) ;
#182393=CARTESIAN_POINT('Ctrl Pts',(-19.6752313663645,-12.5739000669618,
114.662827645649)) ;
#182394=CARTESIAN_POINT('Ctrl Pts',(-19.6900674408757,-12.6330567654726,
114.708015932909)) ;
#182395=CARTESIAN_POINT('Ctrl Pts',(-19.6162635736451,-12.6330568281404,
114.732246902071)) ;
#182396=CARTESIAN_POINT('Ctrl Pts',(-19.5424597064145,-12.6330568908083,
114.756477871234)) ;
#182397=CARTESIAN_POINT('Ctrl Pts',(-19.5276236319032,-12.5739001922976,
114.711289583973)) ;
#182398=CARTESIAN_POINT('Ctrl Pts',(-19.5127875573919,-12.5147434937868,
114.666101296713)) ;
#182399=CARTESIAN_POINT('Ctrl Pts',(-19.5865914246226,-12.5147434311189,
114.641870327551)) ;
#182400=CARTESIAN_POINT('Ctrl Pts',(-19.6603952918532,-12.5147433684511,
114.617639358388)) ;
#182401=CARTESIAN_POINT('Ctrl Pts',(-19.6752313663645,-12.5739000669618,
114.662827645649)) ;
#182402=CARTESIAN_POINT('Ctrl Pts',(-19.6024167491396,-12.7865530350162,
114.47657434342)) ;
#182403=CARTESIAN_POINT('Ctrl Pts',(-19.62162373082,-12.830951855475,114.535075708779)) ;
#182404=CARTESIAN_POINT('Ctrl Pts',(-19.5478198706535,-12.8309519318751,
114.559306699458)) ;
#182405=CARTESIAN_POINT('Ctrl Pts',(-19.4740160104871,-12.8309520082752,
114.583537690136)) ;
#182406=CARTESIAN_POINT('Ctrl Pts',(-19.4548090288067,-12.7865531878164,
114.525036324778)) ;
#182407=CARTESIAN_POINT('Ctrl Pts',(-19.4356020471263,-12.7421543673576,
114.466534959419)) ;
#182408=CARTESIAN_POINT('Ctrl Pts',(-19.5094059072927,-12.7421542909575,
114.44230396874)) ;
#182409=CARTESIAN_POINT('Ctrl Pts',(-19.5832097674592,-12.7421542145574,
114.418072978062)) ;
#182410=CARTESIAN_POINT('Ctrl Pts',(-19.6024167491396,-12.7865530350162,
114.47657434342)) ;
#182411=CARTESIAN_POINT('Ctrl Pts',(-19.5495231103684,-13.044698151263,
114.350994766483)) ;
#182412=CARTESIAN_POINT('Ctrl Pts',(-19.5717169142585,-13.071140713464,
114.418593510497)) ;
#182413=CARTESIAN_POINT('Ctrl Pts',(-19.4979130617208,-13.0711407952517,
114.442824524411)) ;
#182414=CARTESIAN_POINT('Ctrl Pts',(-19.4241092091832,-13.0711408770393,
114.467055538326)) ;
#182415=CARTESIAN_POINT('Ctrl Pts',(-19.4019154052932,-13.0446983148383,
114.399456794313)) ;
#182416=CARTESIAN_POINT('Ctrl Pts',(-19.3797216014032,-13.0182557526373,
114.3318580503)) ;
#182417=CARTESIAN_POINT('Ctrl Pts',(-19.4535254539408,-13.0182556708497,
114.307627036385)) ;
#182418=CARTESIAN_POINT('Ctrl Pts',(-19.5273293064784,-13.018255589062,
114.28339602247)) ;
#182419=CARTESIAN_POINT('Ctrl Pts',(-19.5495231103684,-13.044698151263,
114.350994766483)) ;
#182420=CARTESIAN_POINT('Ctrl Pts',(-19.5196225512715,-13.328059924083,
114.29525984895)) ;
#182421=CARTESIAN_POINT('Ctrl Pts',(-19.5432061536921,-13.33475818736,114.367091695157)) ;
#182422=CARTESIAN_POINT('Ctrl Pts',(-19.4694023083734,-13.3347582681445,
114.39132273106)) ;
#182423=CARTESIAN_POINT('Ctrl Pts',(-19.3955984630547,-13.334758348929,
114.415553766962)) ;
#182424=CARTESIAN_POINT('Ctrl Pts',(-19.3720148606341,-13.328060085652,
114.343721920755)) ;
#182425=CARTESIAN_POINT('Ctrl Pts',(-19.3484312582135,-13.321361822375,
114.271890074548)) ;
#182426=CARTESIAN_POINT('Ctrl Pts',(-19.4222351035322,-13.3213617415905,
114.247659038646)) ;
#182427=CARTESIAN_POINT('Ctrl Pts',(-19.4960389488509,-13.321361660806,
114.223428002743)) ;
#182428=CARTESIAN_POINT('Ctrl Pts',(-19.5196225512715,-13.328059924083,
114.29525984895)) ;
#182429=CARTESIAN_POINT('Ctrl Pts',(-19.5137354281578,-13.6187777866059,
114.312782448992)) ;
#182430=CARTESIAN_POINT('Ctrl Pts',(-19.5370320865056,-13.6051885128316,
114.383740309993)) ;
#182431=CARTESIAN_POINT('Ctrl Pts',(-19.4632282475792,-13.6051885851199,
114.407971365366)) ;
#182432=CARTESIAN_POINT('Ctrl Pts',(-19.3894244086527,-13.6051886574082,
114.432202420738)) ;
#182433=CARTESIAN_POINT('Ctrl Pts',(-19.3661277503048,-13.6187779311824,
114.361244559737)) ;
#182434=CARTESIAN_POINT('Ctrl Pts',(-19.3428310919569,-13.6323672049567,
114.290286698735)) ;
#182435=CARTESIAN_POINT('Ctrl Pts',(-19.4166349308834,-13.6323671326684,
114.266055643363)) ;
#182436=CARTESIAN_POINT('Ctrl Pts',(-19.4904387698099,-13.6323670603802,
114.241824587991)) ;
#182437=CARTESIAN_POINT('Ctrl Pts',(-19.5137354281578,-13.6187777866059,
114.312782448992)) ;
#182438=CARTESIAN_POINT('Ctrl Pts',(-19.5318785681101,-13.8959727795492,
114.403613733301)) ;
#182439=CARTESIAN_POINT('Ctrl Pts',(-19.5532078201559,-13.863009115872,
114.468579192321)) ;
#182440=CARTESIAN_POINT('Ctrl Pts',(-19.4794039858328,-13.8630091736306,
114.492810261715)) ;
#182441=CARTESIAN_POINT('Ctrl Pts',(-19.4056001515098,-13.8630092313891,
114.517041331108)) ;
#182442=CARTESIAN_POINT('Ctrl Pts',(-19.3842708994639,-13.8959728950663,
114.452075872088)) ;
#182443=CARTESIAN_POINT('Ctrl Pts',(-19.3629416474181,-13.9289365587434,
114.387110413069)) ;
#182444=CARTESIAN_POINT('Ctrl Pts',(-19.4367454817412,-13.9289365009848,
114.362879343675)) ;
#182445=CARTESIAN_POINT('Ctrl Pts',(-19.5105493160643,-13.9289364432263,
114.338648274282)) ;
#182446=CARTESIAN_POINT('Ctrl Pts',(-19.5318785681101,-13.8959727795492,
114.403613733301)) ;
#182447=CARTESIAN_POINT('Ctrl Pts',(-19.5718247752165,-14.1380897314584,
114.560743510385)) ;
#182448=CARTESIAN_POINT('Ctrl Pts',(-19.5896635278032,-14.0881713161907,
114.615077471405)) ;
#182449=CARTESIAN_POINT('Ctrl Pts',(-19.5158596961997,-14.0881713577831,
114.639308549082)) ;
#182450=CARTESIAN_POINT('Ctrl Pts',(-19.4420558645962,-14.0881713993755,
114.663539626758)) ;
#182451=CARTESIAN_POINT('Ctrl Pts',(-19.4242171120094,-14.1380898146432,
114.609205665738)) ;
#182452=CARTESIAN_POINT('Ctrl Pts',(-19.4063783594226,-14.1880082299108,
114.554871704718)) ;
#182453=CARTESIAN_POINT('Ctrl Pts',(-19.4801821910262,-14.1880081883184,
114.530640627041)) ;
#182454=CARTESIAN_POINT('Ctrl Pts',(-19.5539860226297,-14.188008146726,
114.506409549364)) ;
#182455=CARTESIAN_POINT('Ctrl Pts',(-19.5718247752165,-14.1380897314584,
114.560743510385)) ;
#182456=CARTESIAN_POINT('Ctrl Pts',(-19.6301836363791,-14.3289912800735,
114.774053959867)) ;
#182457=CARTESIAN_POINT('Ctrl Pts',(-19.6432389873474,-14.2656678675504,
114.813818451542)) ;
#182458=CARTESIAN_POINT('Ctrl Pts',(-19.5694351562483,-14.2656678924027,
114.838049530756)) ;
#182459=CARTESIAN_POINT('Ctrl Pts',(-19.4956313251491,-14.2656679172549,
114.862280609969)) ;
#182460=CARTESIAN_POINT('Ctrl Pts',(-19.4825759741808,-14.3289913297781,
114.822516118294)) ;
#182461=CARTESIAN_POINT('Ctrl Pts',(-19.4695206232126,-14.3923147423012,
114.782751626618)) ;
#182462=CARTESIAN_POINT('Ctrl Pts',(-19.5433244543117,-14.3923147174489,
114.758520547405)) ;
#182463=CARTESIAN_POINT('Ctrl Pts',(-19.6171282854108,-14.3923146925966,
114.734289468192)) ;
#182464=CARTESIAN_POINT('Ctrl Pts',(-19.6301836363791,-14.3289912800735,
114.774053959867)) ;
#182465=CARTESIAN_POINT('Ctrl Pts',(-19.7013725695596,-14.4536834307714,
115.026197380429)) ;
#182466=CARTESIAN_POINT('Ctrl Pts',(-19.7087463412497,-14.3815580790825,
115.048656698481)) ;
#182467=CARTESIAN_POINT('Ctrl Pts',(-19.6349425096067,-14.381558090492,
115.072887776038)) ;
#182468=CARTESIAN_POINT('Ctrl Pts',(-19.5611386779637,-14.3815581019016,
115.097118853595)) ;
#182469=CARTESIAN_POINT('Ctrl Pts',(-19.5537649062736,-14.4536834535906,
115.074659535542)) ;
#182470=CARTESIAN_POINT('Ctrl Pts',(-19.5463911345834,-14.5258088052795,
115.052200217489)) ;
#182471=CARTESIAN_POINT('Ctrl Pts',(-19.6201949662265,-14.52580879387,115.027969139933)) ;
#182472=CARTESIAN_POINT('Ctrl Pts',(-19.6939987978695,-14.5258087824604,
115.003738062376)) ;
#182473=CARTESIAN_POINT('Ctrl Pts',(-19.7013725695596,-14.4536834307714,
115.026197380429)) ;
#182474=CARTESIAN_POINT('Ctrl Pts',(-19.7802758537962,-14.5050447602448,
115.301993496295)) ;
#182475=CARTESIAN_POINT('Ctrl Pts',(-19.7814175815001,-14.4292238155188,
115.305471014069)) ;
#182476=CARTESIAN_POINT('Ctrl Pts',(-19.7076137477033,-14.4292238160263,
115.329702085066)) ;
#182477=CARTESIAN_POINT('Ctrl Pts',(-19.6338099139064,-14.4292238165338,
115.353933156062)) ;
#182478=CARTESIAN_POINT('Ctrl Pts',(-19.6326681862024,-14.5050447612597,
115.350455638288)) ;
#182479=CARTESIAN_POINT('Ctrl Pts',(-19.6315264584984,-14.5808657059856,
115.346978120514)) ;
#182480=CARTESIAN_POINT('Ctrl Pts',(-19.7053302922953,-14.5808657054781,
115.322747049518)) ;
#182481=CARTESIAN_POINT('Ctrl Pts',(-19.7791341260922,-14.5808657049707,
115.298515978521)) ;
#182482=CARTESIAN_POINT('Ctrl Pts',(-19.7802758537962,-14.5050447602448,
115.301993496295)) ;
#182483=CARTESIAN_POINT('Ctrl Pts',(-19.8602648502565,-14.4782940097224,
115.581115798134)) ;
#182484=CARTESIAN_POINT('Ctrl Pts',(-19.8550887574373,-14.4042259752822,
115.565350254132)) ;
#182485=CARTESIAN_POINT('Ctrl Pts',(-19.781284920809,-14.4042259695799,
115.589581316504)) ;
#182486=CARTESIAN_POINT('Ctrl Pts',(-19.7074810841807,-14.4042259638776,
115.613812378877)) ;
#182487=CARTESIAN_POINT('Ctrl Pts',(-19.712657177,-14.4782939983178,115.629577922879)) ;
#182488=CARTESIAN_POINT('Ctrl Pts',(-19.7178332698193,-14.552362032758,
115.645343466881)) ;
#182489=CARTESIAN_POINT('Ctrl Pts',(-19.7916371064475,-14.5523620384603,
115.621112404509)) ;
#182490=CARTESIAN_POINT('Ctrl Pts',(-19.8654409430758,-14.5523620441626,
115.596881342136)) ;
#182491=CARTESIAN_POINT('Ctrl Pts',(-19.8602648502565,-14.4782940097224,
115.581115798134)) ;
#182492=CARTESIAN_POINT('Ctrl Pts',(-19.9347147614836,-14.3758709565101,
115.843310818207)) ;
#182493=CARTESIAN_POINT('Ctrl Pts',(-19.923599187215,-14.3088425929799,
115.809454572183)) ;
#182494=CARTESIAN_POINT('Ctrl Pts',(-19.8497953478602,-14.3088425851836,
115.83368562625)) ;
#182495=CARTESIAN_POINT('Ctrl Pts',(-19.7759915085054,-14.3088425773873,
115.857916680318)) ;
#182496=CARTESIAN_POINT('Ctrl Pts',(-19.787107082774,-14.3758709409175,
115.891772926342)) ;
#182497=CARTESIAN_POINT('Ctrl Pts',(-19.7982226570426,-14.4428993044478,
115.925629172366)) ;
#182498=CARTESIAN_POINT('Ctrl Pts',(-19.8720264963974,-14.442899312244,
115.901398118298)) ;
#182499=CARTESIAN_POINT('Ctrl Pts',(-19.9458303357523,-14.4428993200403,
115.87716706423)) ;
#182500=CARTESIAN_POINT('Ctrl Pts',(-19.9347147614836,-14.3758709565101,
115.843310818207)) ;
#182501=CARTESIAN_POINT('Ctrl Pts',(-19.9978520690189,-14.2038414128419,
116.071213910054)) ;
#182502=CARTESIAN_POINT('Ctrl Pts',(-19.9815743341015,-14.1487238719563,
116.021634555749)) ;
#182503=CARTESIAN_POINT('Ctrl Pts',(-19.9077704923257,-14.1487238662438,
116.045865602443)) ;
#182504=CARTESIAN_POINT('Ctrl Pts',(-19.8339666505498,-14.1487238605313,
116.070096649137)) ;
#182505=CARTESIAN_POINT('Ctrl Pts',(-19.8502443854672,-14.2038414014169,
116.119676003441)) ;
#182506=CARTESIAN_POINT('Ctrl Pts',(-19.8665221203846,-14.2589589423024,
116.169255357746)) ;
#182507=CARTESIAN_POINT('Ctrl Pts',(-19.9403259621604,-14.2589589480149,
116.145024311053)) ;
#182508=CARTESIAN_POINT('Ctrl Pts',(-20.0141298039363,-14.2589589537274,
116.120793264359)) ;
#182509=CARTESIAN_POINT('Ctrl Pts',(-19.9978520690189,-14.2038414128419,
116.071213910054)) ;
#182510=CARTESIAN_POINT('Ctrl Pts',(-20.0437608055394,-13.9777022974474,
116.246290431743)) ;
#182511=CARTESIAN_POINT('Ctrl Pts',(-20.0235237807075,-13.9382924680263,
116.184651719268)) ;
#182512=CARTESIAN_POINT('Ctrl Pts',(-19.9497199377517,-13.9382924647888,
116.208882762368)) ;
#182513=CARTESIAN_POINT('Ctrl Pts',(-19.8759160947959,-13.9382924615514,
116.233113805468)) ;
#182514=CARTESIAN_POINT('Ctrl Pts',(-19.8961531196278,-13.9777022909725,
116.294752517942)) ;
#182515=CARTESIAN_POINT('Ctrl Pts',(-19.9163901444597,-14.0171121203935,
116.356391230417)) ;
#182516=CARTESIAN_POINT('Ctrl Pts',(-19.9901939874155,-14.017112123631,
116.332160187317)) ;
#182517=CARTESIAN_POINT('Ctrl Pts',(-20.0639978303713,-14.0171121268685,
116.307929144217)) ;
#182518=CARTESIAN_POINT('Ctrl Pts',(-20.0437608055394,-13.9777022974474,
116.246290431743)) ;
#182519=CARTESIAN_POINT('Ctrl Pts',(-20.0692545667737,-13.7081471730545,
116.359670607939)) ;
#182520=CARTESIAN_POINT('Ctrl Pts',(-20.046467328162,-13.6875008672276,
116.290264355866)) ;
#182521=CARTESIAN_POINT('Ctrl Pts',(-19.9726634845246,-13.6875008686463,
116.314495396889)) ;
#182522=CARTESIAN_POINT('Ctrl Pts',(-19.8988596408872,-13.687500870065,
116.338726437913)) ;
#182523=CARTESIAN_POINT('Ctrl Pts',(-19.9216468794989,-13.7081471758919,
116.408132689987)) ;
#182524=CARTESIAN_POINT('Ctrl Pts',(-19.9444341181106,-13.7287934817188,
116.47753894206)) ;
#182525=CARTESIAN_POINT('Ctrl Pts',(-20.018237961748,-13.7287934803001,
116.453307901037)) ;
#182526=CARTESIAN_POINT('Ctrl Pts',(-20.0920418053854,-13.7287934788814,
116.429076860013)) ;
#182527=CARTESIAN_POINT('Ctrl Pts',(-20.0692545667737,-13.7081471730545,
116.359670607939)) ;
#182528=CARTESIAN_POINT('Ctrl Pts',(-20.0710088126816,-13.4207218926891,
116.400338260626)) ;
#182529=CARTESIAN_POINT('Ctrl Pts',(-20.0473342388488,-13.4201152017274,
116.328229328668)) ;
#182530=CARTESIAN_POINT('Ctrl Pts',(-19.9735303954241,-13.4201152047761,
116.35246037034)) ;
#182531=CARTESIAN_POINT('Ctrl Pts',(-19.8997265519995,-13.4201152078248,
116.376691412012)) ;
#182532=CARTESIAN_POINT('Ctrl Pts',(-19.9234011258323,-13.4207218987865,
116.44880034397)) ;
#182533=CARTESIAN_POINT('Ctrl Pts',(-19.9470756996652,-13.4213285897482,
116.520909275928)) ;
#182534=CARTESIAN_POINT('Ctrl Pts',(-20.0208795430899,-13.4213285866995,
116.496678234256)) ;
#182535=CARTESIAN_POINT('Ctrl Pts',(-20.0946833865145,-13.4213285836508,
116.472447192584)) ;
#182536=CARTESIAN_POINT('Ctrl Pts',(-20.0710088126816,-13.4207218926891,
116.400338260626)) ;
#182537=CARTESIAN_POINT('Ctrl Pts',(-20.0486389329938,-13.1323473586493,
116.367635760185)) ;
#182538=CARTESIAN_POINT('Ctrl Pts',(-20.0257581006651,-13.1518767361785,
116.297944436781)) ;
#182539=CARTESIAN_POINT('Ctrl Pts',(-19.9519542575344,-13.1518767392038,
116.322175479348)) ;
#182540=CARTESIAN_POINT('Ctrl Pts',(-19.8781504144038,-13.1518767422291,
116.346406521915)) ;
#182541=CARTESIAN_POINT('Ctrl Pts',(-19.9010312467325,-13.1323473646999,
116.416097845319)) ;
#182542=CARTESIAN_POINT('Ctrl Pts',(-19.9239120790612,-13.1128179871707,
116.485789168723)) ;
#182543=CARTESIAN_POINT('Ctrl Pts',(-19.9977159221919,-13.1128179841454,
116.461558126156)) ;
#182544=CARTESIAN_POINT('Ctrl Pts',(-20.0715197653226,-13.1128179811201,
116.437327083588)) ;
#182545=CARTESIAN_POINT('Ctrl Pts',(-20.0486389329938,-13.1323473586493,
116.367635760185)) ;
#182546=CARTESIAN_POINT('Ctrl Pts',(-20.0027585392029,-12.8640039527127,
116.26336619867)) ;
#182547=CARTESIAN_POINT('Ctrl Pts',(-19.9823136010525,-12.9022999989721,
116.201094215862)) ;
#182548=CARTESIAN_POINT('Ctrl Pts',(-19.9085097578917,-12.9022999996752,
116.225325258337)) ;
#182549=CARTESIAN_POINT('Ctrl Pts',(-19.8347059147309,-12.9023000003783,
116.249556300812)) ;
#182550=CARTESIAN_POINT('Ctrl Pts',(-19.8551508528813,-12.8640039541189,
116.31182828362)) ;
#182551=CARTESIAN_POINT('Ctrl Pts',(-19.8755957910317,-12.8257079078595,
116.374100266428)) ;
#182552=CARTESIAN_POINT('Ctrl Pts',(-19.9493996341925,-12.8257079071564,
116.349869223953)) ;
#182553=CARTESIAN_POINT('Ctrl Pts',(-20.0232034773534,-12.8257079064533,
116.325638181478)) ;
#182554=CARTESIAN_POINT('Ctrl Pts',(-20.0027585392029,-12.8640039527127,
116.26336619867)) ;
#182555=CARTESIAN_POINT('Ctrl Pts',(-19.935788026807,-12.6351955964259,
116.094916391057)) ;
#182556=CARTESIAN_POINT('Ctrl Pts',(-19.9192541332925,-12.6895248162975,
116.044556819081)) ;
#182557=CARTESIAN_POINT('Ctrl Pts',(-19.8454502892082,-12.6895248136964,
116.068787858743)) ;
#182558=CARTESIAN_POINT('Ctrl Pts',(-19.7716464451238,-12.6895248110954,
116.093018898405)) ;
#182559=CARTESIAN_POINT('Ctrl Pts',(-19.7881803386382,-12.6351955912238,
116.143378470382)) ;
#182560=CARTESIAN_POINT('Ctrl Pts',(-19.8047142321527,-12.5808663713523,
116.193738042358)) ;
#182561=CARTESIAN_POINT('Ctrl Pts',(-19.8785180762371,-12.5808663739533,
116.169507002696)) ;
#182562=CARTESIAN_POINT('Ctrl Pts',(-19.9523219203215,-12.5808663765543,
116.145275963034)) ;
#182563=CARTESIAN_POINT('Ctrl Pts',(-19.935788026807,-12.6351955964259,
116.094916391057)) ;
#182564=CARTESIAN_POINT('Ctrl Pts',(-19.8524350019228,-12.4633049543151,
115.876360547653)) ;
#182565=CARTESIAN_POINT('Ctrl Pts',(-19.8409661307527,-12.5297151872054,
115.841428216412)) ;
#182566=CARTESIAN_POINT('Ctrl Pts',(-19.7671622852702,-12.5297151829142,
115.865659251816)) ;
#182567=CARTESIAN_POINT('Ctrl Pts',(-19.6933584397878,-12.529715178623,
115.88989028722)) ;
#182568=CARTESIAN_POINT('Ctrl Pts',(-19.7048273109579,-12.4633049457328,
115.924822618461)) ;
#182569=CARTESIAN_POINT('Ctrl Pts',(-19.7162961821279,-12.3968947128425,
115.959754949702)) ;
#182570=CARTESIAN_POINT('Ctrl Pts',(-19.7901000276104,-12.3968947171337,
115.935523914298)) ;
#182571=CARTESIAN_POINT('Ctrl Pts',(-19.8639038730929,-12.3968947214249,
115.911292878894)) ;
#182572=CARTESIAN_POINT('Ctrl Pts',(-19.8524350019228,-12.4633049543151,
115.876360547653)) ;
#182573=CARTESIAN_POINT('Ctrl Pts',(-19.7565552164464,-12.3586842738095,
115.619991906947)) ;
#182574=CARTESIAN_POINT('Ctrl Pts',(-19.7510262973849,-12.4324967253125,
115.603151711264)) ;
#182575=CARTESIAN_POINT('Ctrl Pts',(-19.6772224491687,-12.432496720994,
115.627382738341)) ;
#182576=CARTESIAN_POINT('Ctrl Pts',(-19.6034186009525,-12.4324967166755,
115.651613765419)) ;
#182577=CARTESIAN_POINT('Ctrl Pts',(-19.6089475200141,-12.3586842651726,
115.668453961102)) ;
#182578=CARTESIAN_POINT('Ctrl Pts',(-19.6144764390756,-12.2848718136696,
115.685294156784)) ;
#182579=CARTESIAN_POINT('Ctrl Pts',(-19.6882802872918,-12.284871817988,
115.661063129707)) ;
#182580=CARTESIAN_POINT('Ctrl Pts',(-19.762084135508,-12.2848718223065,
115.63683210263)) ;
#182581=CARTESIAN_POINT('Ctrl Pts',(-19.7565552164464,-12.3586842738095,
115.619991906947)) ;
#182582=CARTESIAN_POINT('Ctrl Pts',(-19.6559368636795,-12.3308701665295,
115.348879090383)) ;
#182583=CARTESIAN_POINT('Ctrl Pts',(-19.6566937304098,-12.4067313032611,
115.351184383885)) ;
#182584=CARTESIAN_POINT('Ctrl Pts',(-19.5828898799169,-12.4067313035056,
115.375415404028)) ;
#182585=CARTESIAN_POINT('Ctrl Pts',(-19.5090860294241,-12.4067313037501,
115.399646424171)) ;
#182586=CARTESIAN_POINT('Ctrl Pts',(-19.5083291626938,-12.3308701670186,
115.39734113067)) ;
#182587=CARTESIAN_POINT('Ctrl Pts',(-19.5075722959635,-12.2550090302871,
115.395035837168)) ;
#182588=CARTESIAN_POINT('Ctrl Pts',(-19.5813761464564,-12.2550090300425,
115.370804817025)) ;
#182589=CARTESIAN_POINT('Ctrl Pts',(-19.6551799969492,-12.255009029798,
115.346573796882)) ;
#182590=CARTESIAN_POINT('Ctrl Pts',(-19.6559368636795,-12.3308701665295,
115.348879090383)) ;
#182591=CARTESIAN_POINT('Ctrl Pts',(-19.5559630364021,-12.3804185210795,
115.079826490949)) ;
#182592=CARTESIAN_POINT('Ctrl Pts',(-19.5629676944445,-12.4529298980233,
115.101161548555)) ;
#182593=CARTESIAN_POINT('Ctrl Pts',(-19.4891638418352,-12.452929906521,
115.125392562252)) ;
#182594=CARTESIAN_POINT('Ctrl Pts',(-19.415359989226,-12.4529299150187,
115.149623575949)) ;
#182595=CARTESIAN_POINT('Ctrl Pts',(-19.4083553311837,-12.380418538075,
115.128288518343)) ;
#182596=CARTESIAN_POINT('Ctrl Pts',(-19.4013506731413,-12.3079071611312,
115.106953460736)) ;
#182597=CARTESIAN_POINT('Ctrl Pts',(-19.4751545257505,-12.3079071526335,
115.082722447039)) ;
#182598=CARTESIAN_POINT('Ctrl Pts',(-19.5489583783597,-12.3079071441357,
115.058491433342)) ;
#182599=CARTESIAN_POINT('Ctrl Pts',(-19.5559630364021,-12.3804185210795,
115.079826490949)) ;
#182600=CARTESIAN_POINT('Ctrl Pts',(-19.4632285523152,-12.5045865657479,
114.832858816864)) ;
#182601=CARTESIAN_POINT('Ctrl Pts',(-19.4759837989463,-12.5685333529208,
114.871709239288)) ;
#182602=CARTESIAN_POINT('Ctrl Pts',(-19.4021799450906,-12.5685333737573,
114.895940249188)) ;
#182603=CARTESIAN_POINT('Ctrl Pts',(-19.3283760912348,-12.5685333945939,
114.920171259088)) ;
#182604=CARTESIAN_POINT('Ctrl Pts',(-19.3156208446037,-12.504586607421,
114.881320836664)) ;
#182605=CARTESIAN_POINT('Ctrl Pts',(-19.3028655979726,-12.4406398202481,
114.84247041424)) ;
#182606=CARTESIAN_POINT('Ctrl Pts',(-19.3766694518284,-12.4406397994116,
114.81823940434)) ;
#182607=CARTESIAN_POINT('Ctrl Pts',(-19.4504733056841,-12.440639778575,
114.794008394439)) ;
#182608=CARTESIAN_POINT('Ctrl Pts',(-19.4632285523152,-12.5045865657479,
114.832858816864)) ;
#182609=CARTESIAN_POINT('Ctrl Pts',(-19.3838405577288,-12.6936012415773,
114.626458033077)) ;
#182610=CARTESIAN_POINT('Ctrl Pts',(-19.4014244618248,-12.7444433865652,
114.680015766882)) ;
#182611=CARTESIAN_POINT('Ctrl Pts',(-19.3276206083385,-12.7444434214993,
114.704246777907)) ;
#182612=CARTESIAN_POINT('Ctrl Pts',(-19.2538167548521,-12.7444434564334,
114.728477788932)) ;
#182613=CARTESIAN_POINT('Ctrl Pts',(-19.2362328507561,-12.6936013114455,
114.674920055127)) ;
#182614=CARTESIAN_POINT('Ctrl Pts',(-19.2186489466601,-12.6427591664577,
114.621362321322)) ;
#182615=CARTESIAN_POINT('Ctrl Pts',(-19.2924528001464,-12.6427591315236,
114.597131310297)) ;
#182616=CARTESIAN_POINT('Ctrl Pts',(-19.3662566536328,-12.6427590965895,
114.572900299272)) ;
#182617=CARTESIAN_POINT('Ctrl Pts',(-19.3838405577288,-12.6936012415773,
114.626458033077)) ;
#182618=CARTESIAN_POINT('Ctrl Pts',(-19.3222105618298,-12.9362801376937,
114.474398641739)) ;
#182619=CARTESIAN_POINT('Ctrl Pts',(-19.3433851628242,-12.9702525737982,
114.538893058736)) ;
#182620=CARTESIAN_POINT('Ctrl Pts',(-19.2695813111783,-12.9702526255318,
114.563124075367)) ;
#182621=CARTESIAN_POINT('Ctrl Pts',(-19.1957774595324,-12.9702526772653,
114.587355091998)) ;
#182622=CARTESIAN_POINT('Ctrl Pts',(-19.1746028585379,-12.9362802411607,
114.522860675001)) ;
#182623=CARTESIAN_POINT('Ctrl Pts',(-19.1534282575434,-12.9023078050562,
114.458366258004)) ;
#182624=CARTESIAN_POINT('Ctrl Pts',(-19.2272321091894,-12.9023077533226,
114.434135241373)) ;
#182625=CARTESIAN_POINT('Ctrl Pts',(-19.3010359608353,-12.9023077015891,
114.409904224742)) ;
#182626=CARTESIAN_POINT('Ctrl Pts',(-19.3222105618298,-12.9362801376937,
114.474398641739)) ;
#182627=CARTESIAN_POINT('Ctrl Pts',(-19.2828604657008,-13.2112926431605,
114.389881775346)) ;
#182628=CARTESIAN_POINT('Ctrl Pts',(-19.3060817289072,-13.2261131719055,
114.460609995074)) ;
#182629=CARTESIAN_POINT('Ctrl Pts',(-19.2322778814261,-13.2261132359039,
114.48484102439)) ;
#182630=CARTESIAN_POINT('Ctrl Pts',(-19.1584740339449,-13.2261132999022,
114.509072053706)) ;
#182631=CARTESIAN_POINT('Ctrl Pts',(-19.1352527707385,-13.2112927711572,
114.438343833979)) ;
#182632=CARTESIAN_POINT('Ctrl Pts',(-19.1120315075321,-13.1964722424121,
114.367615614251)) ;
#182633=CARTESIAN_POINT('Ctrl Pts',(-19.1858353550133,-13.1964721784138,
114.343384584935)) ;
#182634=CARTESIAN_POINT('Ctrl Pts',(-19.2596392024944,-13.1964721144154,
114.319153555619)) ;
#182635=CARTESIAN_POINT('Ctrl Pts',(-19.2828604657008,-13.2112926431605,
114.389881775346)) ;
#182636=CARTESIAN_POINT('Ctrl Pts',(-19.2671542279157,-13.5026318637497,
114.377588421652)) ;
#182637=CARTESIAN_POINT('Ctrl Pts',(-19.2907702583407,-13.4971333433814,
114.449519038463)) ;
#182638=CARTESIAN_POINT('Ctrl Pts',(-19.2169664165159,-13.4971334172492,
114.473750085008)) ;
#182639=CARTESIAN_POINT('Ctrl Pts',(-19.1431625746911,-13.4971334911169,
114.497981131552)) ;
#182640=CARTESIAN_POINT('Ctrl Pts',(-19.119546544266,-13.5026320114853,
114.426050514741)) ;
#182641=CARTESIAN_POINT('Ctrl Pts',(-19.0959305138409,-13.5081305318536,
114.35411989793)) ;
#182642=CARTESIAN_POINT('Ctrl Pts',(-19.1697343556658,-13.5081304579859,
114.329888851385)) ;
#182643=CARTESIAN_POINT('Ctrl Pts',(-19.2435381974906,-13.5081303841181,
114.305657804841)) ;
#182644=CARTESIAN_POINT('Ctrl Pts',(-19.2671542279157,-13.5026318637497,
114.377588421652)) ;
#182645=CARTESIAN_POINT('Ctrl Pts',(-19.2757419733594,-13.7865927515763,
114.439120363259)) ;
#182646=CARTESIAN_POINT('Ctrl Pts',(-19.2980606185593,-13.7612608950297,
114.507099353878)) ;
#182647=CARTESIAN_POINT('Ctrl Pts',(-19.2242567835297,-13.7612609711619,
114.531330421119)) ;
#182648=CARTESIAN_POINT('Ctrl Pts',(-19.1504529485,-13.7612610472941,114.55556148836)) ;
#182649=CARTESIAN_POINT('Ctrl Pts',(-19.1281343033001,-13.7865929038406,
114.487582497741)) ;
#182650=CARTESIAN_POINT('Ctrl Pts',(-19.1058156581001,-13.8119247603871,
114.419603507123)) ;
#182651=CARTESIAN_POINT('Ctrl Pts',(-19.1796194931298,-13.811924684255,
114.395372439881)) ;
#182652=CARTESIAN_POINT('Ctrl Pts',(-19.2534233281594,-13.8119246081228,
114.37114137264)) ;
#182653=CARTESIAN_POINT('Ctrl Pts',(-19.2757419733594,-13.7865927515763,
114.439120363259)) ;
#182654=CARTESIAN_POINT('Ctrl Pts',(-19.3070927419327,-14.0445932154009,
114.570030945766)) ;
#182655=CARTESIAN_POINT('Ctrl Pts',(-19.3265220349553,-14.0012118501805,
114.629209435722)) ;
#182656=CARTESIAN_POINT('Ctrl Pts',(-19.2527182070799,-14.001211921774,
114.653440524754)) ;
#182657=CARTESIAN_POINT('Ctrl Pts',(-19.1789143792045,-14.0012119933675,
114.677671613786)) ;
#182658=CARTESIAN_POINT('Ctrl Pts',(-19.159485086182,-14.0445933585879,
114.61849312383)) ;
#182659=CARTESIAN_POINT('Ctrl Pts',(-19.1400557931594,-14.0879747238084,
114.559314633874)) ;
#182660=CARTESIAN_POINT('Ctrl Pts',(-19.2138596210347,-14.0879746522149,
114.535083544842)) ;
#182661=CARTESIAN_POINT('Ctrl Pts',(-19.2876634489101,-14.0879745806213,
114.510852455809)) ;
#182662=CARTESIAN_POINT('Ctrl Pts',(-19.3070927419327,-14.0445932154009,
114.570030945766)) ;
#182663=CARTESIAN_POINT('Ctrl Pts',(-19.358347515694,-14.2581092551482,
114.761608730446)) ;
#182664=CARTESIAN_POINT('Ctrl Pts',(-19.3734928699903,-14.199757820622,
114.807739034136)) ;
#182665=CARTESIAN_POINT('Ctrl Pts',(-19.2996890489537,-14.199757880284,
114.831970143998)) ;
#182666=CARTESIAN_POINT('Ctrl Pts',(-19.2258852279171,-14.199757939946,
114.85620125386)) ;
#182667=CARTESIAN_POINT('Ctrl Pts',(-19.2107398736208,-14.2581093744722,
114.81007095017)) ;
#182668=CARTESIAN_POINT('Ctrl Pts',(-19.1955945193246,-14.3164608089984,
114.763940646481)) ;
#182669=CARTESIAN_POINT('Ctrl Pts',(-19.2693983403611,-14.3164607493364,
114.739709536619)) ;
#182670=CARTESIAN_POINT('Ctrl Pts',(-19.3432021613977,-14.3164606896743,
114.715478426757)) ;
#182671=CARTESIAN_POINT('Ctrl Pts',(-19.358347515694,-14.2581092551482,
114.761608730446)) ;
#182672=CARTESIAN_POINT('Ctrl Pts',(-19.4252783091883,-14.4117380229187,
115.001038317045)) ;
#182673=CARTESIAN_POINT('Ctrl Pts',(-19.4350370294147,-14.3425754066096,
115.030761802378)) ;
#182674=CARTESIAN_POINT('Ctrl Pts',(-19.3612332141478,-14.3425754472621,
115.054992929814)) ;
#182675=CARTESIAN_POINT('Ctrl Pts',(-19.287429398881,-14.3425754879145,
115.079224057249)) ;
#182676=CARTESIAN_POINT('Ctrl Pts',(-19.2776706786545,-14.4117381042236,
115.049500571916)) ;
#182677=CARTESIAN_POINT('Ctrl Pts',(-19.2679119584281,-14.4809007205327,
115.019777086582)) ;
#182678=CARTESIAN_POINT('Ctrl Pts',(-19.3417157736949,-14.4809006798802,
114.995545959146)) ;
#182679=CARTESIAN_POINT('Ctrl Pts',(-19.4155195889618,-14.4809006392278,
114.971314831711)) ;
#182680=CARTESIAN_POINT('Ctrl Pts',(-19.4252783091883,-14.4117380229187,
115.001038317045)) ;
#182681=CARTESIAN_POINT('Ctrl Pts',(-19.5019526631148,-14.4936441507055,
115.270046158408)) ;
#182682=CARTESIAN_POINT('Ctrl Pts',(-19.5056386466896,-14.4186618661927,
115.281273067656)) ;
#182683=CARTESIAN_POINT('Ctrl Pts',(-19.4318348350287,-14.4186618819305,
115.305504206074)) ;
#182684=CARTESIAN_POINT('Ctrl Pts',(-19.3580310233677,-14.4186618976683,
115.329735344493)) ;
#182685=CARTESIAN_POINT('Ctrl Pts',(-19.3543450397929,-14.4936441821811,
115.318508435245)) ;
#182686=CARTESIAN_POINT('Ctrl Pts',(-19.350659056218,-14.5686264666939,
115.307281525998)) ;
#182687=CARTESIAN_POINT('Ctrl Pts',(-19.424462867879,-14.5686264509561,
115.283050387579)) ;
#182688=CARTESIAN_POINT('Ctrl Pts',(-19.49826667954,-14.5686264352184,115.258819249161)) ;
#182689=CARTESIAN_POINT('Ctrl Pts',(-19.5019526631148,-14.4936441507055,
115.270046158408)) ;
#182690=CARTESIAN_POINT('Ctrl Pts',(-19.5823198515389,-14.4983888239063,
115.550327419762)) ;
#182691=CARTESIAN_POINT('Ctrl Pts',(-19.5796658758239,-14.422965043811,
115.542243835903)) ;
#182692=CARTESIAN_POINT('Ctrl Pts',(-19.505862065243,-14.4229650315207,
115.566474977611)) ;
#182693=CARTESIAN_POINT('Ctrl Pts',(-19.4320582546622,-14.4229650192305,
115.59070611932)) ;
#182694=CARTESIAN_POINT('Ctrl Pts',(-19.4347122303772,-14.4983887993257,
115.598789703178)) ;
#182695=CARTESIAN_POINT('Ctrl Pts',(-19.4373662060922,-14.573812579421,
115.606873287037)) ;
#182696=CARTESIAN_POINT('Ctrl Pts',(-19.511170016673,-14.5738125917113,
115.582642145328)) ;
#182697=CARTESIAN_POINT('Ctrl Pts',(-19.5849738272539,-14.5738126040015,
115.55841100362)) ;
#182698=CARTESIAN_POINT('Ctrl Pts',(-19.5823198515389,-14.4983888239063,
115.550327419762)) ;
#182699=CARTESIAN_POINT('Ctrl Pts',(-19.6595477418913,-14.426207251784,
115.82090191206)) ;
#182700=CARTESIAN_POINT('Ctrl Pts',(-19.6507666379267,-14.3557121733631,
115.79415608413)) ;
#182701=CARTESIAN_POINT('Ctrl Pts',(-19.5769628256401,-14.355712132954,
115.818387220643)) ;
#182702=CARTESIAN_POINT('Ctrl Pts',(-19.5031590133536,-14.3557120925449,
115.842618357156)) ;
#182703=CARTESIAN_POINT('Ctrl Pts',(-19.5119401173182,-14.4262071709657,
115.869364185087)) ;
#182704=CARTESIAN_POINT('Ctrl Pts',(-19.5207212212828,-14.4967022493866,
115.896110013017)) ;
#182705=CARTESIAN_POINT('Ctrl Pts',(-19.5945250335694,-14.4967022897957,
115.871878876504)) ;
#182706=CARTESIAN_POINT('Ctrl Pts',(-19.6683288458559,-14.4967023302048,
115.847647739991)) ;
#182707=CARTESIAN_POINT('Ctrl Pts',(-19.6595477418913,-14.426207251784,
115.82090191206)) ;
#182708=CARTESIAN_POINT('Ctrl Pts',(-19.7280764038109,-14.2809809264381,
116.065217208955)) ;
#182709=CARTESIAN_POINT('Ctrl Pts',(-19.7137615271889,-14.2205203869784,
116.021616402365)) ;
#182710=CARTESIAN_POINT('Ctrl Pts',(-19.6399577106063,-14.2205203209335,
116.045847525793)) ;
#182711=CARTESIAN_POINT('Ctrl Pts',(-19.5661538940236,-14.2205202548886,
116.070078649221)) ;
#182712=CARTESIAN_POINT('Ctrl Pts',(-19.5804687706457,-14.2809807943484,
116.113679455811)) ;
#182713=CARTESIAN_POINT('Ctrl Pts',(-19.5947836472677,-14.3414413338082,
116.157280262401)) ;
#182714=CARTESIAN_POINT('Ctrl Pts',(-19.6685874638503,-14.3414413998531,
116.133049138973)) ;
#182715=CARTESIAN_POINT('Ctrl Pts',(-19.7423912804329,-14.3414414658979,
116.108818015545)) ;
#182716=CARTESIAN_POINT('Ctrl Pts',(-19.7280764038109,-14.2809809264381,
116.065217208955)) ;
#182717=CARTESIAN_POINT('Ctrl Pts',(-19.7813206021368,-14.0755731076895,
116.262663449883)) ;
#182718=CARTESIAN_POINT('Ctrl Pts',(-19.7625374017033,-14.0293643773253,
116.205452849931)) ;
#182719=CARTESIAN_POINT('Ctrl Pts',(-19.6887335786472,-14.0293642911148,
116.229683953641)) ;
#182720=CARTESIAN_POINT('Ctrl Pts',(-19.614929755591,-14.0293642049043,
116.253915057352)) ;
#182721=CARTESIAN_POINT('Ctrl Pts',(-19.6337129560244,-14.0755729352685,
116.311125657304)) ;
#182722=CARTESIAN_POINT('Ctrl Pts',(-19.6524961564578,-14.1217816656326,
116.368336257255)) ;
#182723=CARTESIAN_POINT('Ctrl Pts',(-19.726299979514,-14.1217817518431,
116.344105153545)) ;
#182724=CARTESIAN_POINT('Ctrl Pts',(-19.8001038025702,-14.1217818380536,
116.319874049834)) ;
#182725=CARTESIAN_POINT('Ctrl Pts',(-19.7813206021368,-14.0755731076895,
116.262663449883)) ;
#182726=CARTESIAN_POINT('Ctrl Pts',(-19.8156285654698,-13.8214647968314,
116.402723704513)) ;
#182727=CARTESIAN_POINT('Ctrl Pts',(-19.7936862540445,-13.7929280082953,
116.33589096223)) ;
#182728=CARTESIAN_POINT('Ctrl Pts',(-19.7198824228961,-13.7929279092314,
116.360122041293)) ;
#182729=CARTESIAN_POINT('Ctrl Pts',(-19.6460785917477,-13.7929278101675,
116.384353120356)) ;
#182730=CARTESIAN_POINT('Ctrl Pts',(-19.668020903173,-13.8214645987035,
116.451185862638)) ;
#182731=CARTESIAN_POINT('Ctrl Pts',(-19.6899632145983,-13.8500013872396,
116.518018604921)) ;
#182732=CARTESIAN_POINT('Ctrl Pts',(-19.7637670457467,-13.8500014863035,
116.493787525858)) ;
#182733=CARTESIAN_POINT('Ctrl Pts',(-19.8375708768951,-13.8500015853674,
116.469556446795)) ;
#182734=CARTESIAN_POINT('Ctrl Pts',(-19.8156285654698,-13.8214647968314,
116.402723704513)) ;
#182735=CARTESIAN_POINT('Ctrl Pts',(-19.8271835709341,-13.5390721929965,
116.473371097639)) ;
#182736=CARTESIAN_POINT('Ctrl Pts',(-19.8036682136408,-13.5302086359891,
116.401747111505)) ;
#182737=CARTESIAN_POINT('Ctrl Pts',(-19.7298643737381,-13.5302085326853,
116.425978163903)) ;
#182738=CARTESIAN_POINT('Ctrl Pts',(-19.6560605338353,-13.5302084293816,
116.450209216302)) ;
#182739=CARTESIAN_POINT('Ctrl Pts',(-19.6795758911286,-13.539071986389,
116.521833202437)) ;
#182740=CARTESIAN_POINT('Ctrl Pts',(-19.7030912484218,-13.5479355433964,
116.593457188571)) ;
#182741=CARTESIAN_POINT('Ctrl Pts',(-19.7768950883246,-13.5479356467002,
116.569226136173)) ;
#182742=CARTESIAN_POINT('Ctrl Pts',(-19.8506989282273,-13.5479357500039,
116.544995083774)) ;
#182743=CARTESIAN_POINT('Ctrl Pts',(-19.8271835709341,-13.5390721929965,
116.473371097639)) ;
#182744=CARTESIAN_POINT('Ctrl Pts',(-19.8146134378266,-13.2479213210197,
116.470556422711)) ;
#182745=CARTESIAN_POINT('Ctrl Pts',(-19.7912065222546,-13.2593718199025,
116.399262732634)) ;
#182746=CARTESIAN_POINT('Ctrl Pts',(-19.7174026738327,-13.2593717210079,
116.423493759085)) ;
#182747=CARTESIAN_POINT('Ctrl Pts',(-19.6435988254109,-13.2593716221134,
116.447724785536)) ;
#182748=CARTESIAN_POINT('Ctrl Pts',(-19.667005740983,-13.2479211232306,
116.519018475613)) ;
#182749=CARTESIAN_POINT('Ctrl Pts',(-19.690412656555,-13.2364706243478,
116.59031216569)) ;
#182750=CARTESIAN_POINT('Ctrl Pts',(-19.7642165049769,-13.2364707232423,
116.566081139239)) ;
#182751=CARTESIAN_POINT('Ctrl Pts',(-19.8380203533987,-13.2364708221369,
116.541850112788)) ;
#182752=CARTESIAN_POINT('Ctrl Pts',(-19.8146134378266,-13.2479213210197,
116.470556422711)) ;
#182753=CARTESIAN_POINT('Ctrl Pts',(-19.7780274303114,-12.9689956696526,
116.394584966036)) ;
#182754=CARTESIAN_POINT('Ctrl Pts',(-19.7564059267676,-12.9999372691398,
116.328729353013)) ;
#182755=CARTESIAN_POINT('Ctrl Pts',(-19.6826020709247,-12.9999371823959,
116.352960356861)) ;
#182756=CARTESIAN_POINT('Ctrl Pts',(-19.6087982150818,-12.9999370956519,
116.377191360708)) ;
#182757=CARTESIAN_POINT('Ctrl Pts',(-19.6304197186256,-12.9689954961647,
116.443046973731)) ;
#182758=CARTESIAN_POINT('Ctrl Pts',(-19.6520412221694,-12.9380538966775,
116.508902586753)) ;
#182759=CARTESIAN_POINT('Ctrl Pts',(-19.7258450780123,-12.9380539834215,
116.484671582906)) ;
#182760=CARTESIAN_POINT('Ctrl Pts',(-19.7996489338551,-12.9380540701654,
116.460440579058)) ;
#182761=CARTESIAN_POINT('Ctrl Pts',(-19.7780274303114,-12.9689956696526,
116.394584966036)) ;
#182762=CARTESIAN_POINT('Ctrl Pts',(-19.7192534733058,-12.7220961737177,
116.251055118297)) ;
#182763=CARTESIAN_POINT('Ctrl Pts',(-19.7009686186426,-12.7703223930981,
116.195362399511)) ;
#182764=CARTESIAN_POINT('Ctrl Pts',(-19.6271647572106,-12.7703223245763,
116.219593386335)) ;
#182765=CARTESIAN_POINT('Ctrl Pts',(-19.5533608957786,-12.7703222560545,
116.243824373159)) ;
#182766=CARTESIAN_POINT('Ctrl Pts',(-19.5716457504418,-12.7220960366741,
116.299517091945)) ;
#182767=CARTESIAN_POINT('Ctrl Pts',(-19.589930605105,-12.6738698172937,
116.355209810731)) ;
#182768=CARTESIAN_POINT('Ctrl Pts',(-19.663734466537,-12.6738698858155,
116.330978823907)) ;
#182769=CARTESIAN_POINT('Ctrl Pts',(-19.737538327969,-12.6738699543374,
116.306747837083)) ;
#182770=CARTESIAN_POINT('Ctrl Pts',(-19.7192534733058,-12.7220961737177,
116.251055118297)) ;
#182771=CARTESIAN_POINT('Ctrl Pts',(-19.6419060205883,-12.5254520180373,
116.050893527524)) ;
#182772=CARTESIAN_POINT('Ctrl Pts',(-19.6282608755407,-12.5874803484278,
116.009332615734)) ;
#182773=CARTESIAN_POINT('Ctrl Pts',(-19.5544570106936,-12.5874803012304,
116.033563592156)) ;
#182774=CARTESIAN_POINT('Ctrl Pts',(-19.4806531458465,-12.5874802540331,
116.057794568578)) ;
#182775=CARTESIAN_POINT('Ctrl Pts',(-19.4942982908941,-12.5254519236426,
116.099355480369)) ;
#182776=CARTESIAN_POINT('Ctrl Pts',(-19.5079434359418,-12.463423593252,
116.140916392159)) ;
#182777=CARTESIAN_POINT('Ctrl Pts',(-19.5817473007888,-12.4634236404494,
116.116685415737)) ;
#182778=CARTESIAN_POINT('Ctrl Pts',(-19.6555511656359,-12.4634236876467,
116.092454439314)) ;
#182779=CARTESIAN_POINT('Ctrl Pts',(-19.6419060205883,-12.5254520180373,
116.050893527524)) ;
#182780=CARTESIAN_POINT('Ctrl Pts',(-19.5507750838464,-12.3924871288094,
115.808727229059)) ;
#182781=CARTESIAN_POINT('Ctrl Pts',(-19.5427394409189,-12.4638924990082,
115.784251955766)) ;
#182782=CARTESIAN_POINT('Ctrl Pts',(-19.4689355748862,-12.4638924741093,
115.808482928577)) ;
#182783=CARTESIAN_POINT('Ctrl Pts',(-19.3951317088534,-12.4638924492103,
115.832713901388)) ;
#182784=CARTESIAN_POINT('Ctrl Pts',(-19.4031673517809,-12.3924870790115,
115.857189174681)) ;
#182785=CARTESIAN_POINT('Ctrl Pts',(-19.4112029947084,-12.3210817088127,
115.881664447974)) ;
#182786=CARTESIAN_POINT('Ctrl Pts',(-19.4850068607412,-12.3210817337116,
115.857433475163)) ;
#182787=CARTESIAN_POINT('Ctrl Pts',(-19.5588107267739,-12.3210817586106,
115.833202502352)) ;
#182788=CARTESIAN_POINT('Ctrl Pts',(-19.5507750838464,-12.3924871288094,
115.808727229059)) ;
#182789=CARTESIAN_POINT('Ctrl Pts',(-19.4509678272437,-12.3327720085306,
115.540332649395)) ;
#182790=CARTESIAN_POINT('Ctrl Pts',(-19.4491517888012,-12.4084551705648,
115.534801288009)) ;
#182791=CARTESIAN_POINT('Ctrl Pts',(-19.3753479243441,-12.4084551665108,
115.55903226562)) ;
#182792=CARTESIAN_POINT('Ctrl Pts',(-19.3015440598871,-12.4084551624567,
115.58326324323)) ;
#182793=CARTESIAN_POINT('Ctrl Pts',(-19.3033600983296,-12.3327720004226,
115.588794604616)) ;
#182794=CARTESIAN_POINT('Ctrl Pts',(-19.3051761367722,-12.2570888383885,
115.594325966001)) ;
#182795=CARTESIAN_POINT('Ctrl Pts',(-19.3789800012292,-12.2570888424425,
115.570094988391)) ;
#182796=CARTESIAN_POINT('Ctrl Pts',(-19.4527838656863,-12.2570888464965,
115.54586401078)) ;
#182797=CARTESIAN_POINT('Ctrl Pts',(-19.4509678272437,-12.3327720085306,
115.540332649395)) ;
#182798=CARTESIAN_POINT('Ctrl Pts',(-19.3501879158993,-12.3509988977752,
115.268703339782)) ;
#182799=CARTESIAN_POINT('Ctrl Pts',(-19.35467457357,-12.4255237330698,115.282368973957)) ;
#182800=CARTESIAN_POINT('Ctrl Pts',(-19.280870711689,-12.4255237455323,
115.306599959414)) ;
#182801=CARTESIAN_POINT('Ctrl Pts',(-19.2070668498081,-12.4255237579948,
115.330830944871)) ;
#182802=CARTESIAN_POINT('Ctrl Pts',(-19.2025801921374,-12.3509989227002,
115.317165310695)) ;
#182803=CARTESIAN_POINT('Ctrl Pts',(-19.1980935344667,-12.2764740874057,
115.303499676519)) ;
#182804=CARTESIAN_POINT('Ctrl Pts',(-19.2718973963476,-12.2764740749432,
115.279268691063)) ;
#182805=CARTESIAN_POINT('Ctrl Pts',(-19.3457012582286,-12.2764740624807,
115.255037705606)) ;
#182806=CARTESIAN_POINT('Ctrl Pts',(-19.3501879158993,-12.3509988977752,
115.268703339782)) ;
#182807=CARTESIAN_POINT('Ctrl Pts',(-19.2537109950385,-12.4453838611795,
115.010328377215)) ;
#182808=CARTESIAN_POINT('Ctrl Pts',(-19.2642064131177,-12.5134317382336,
115.042295726253)) ;
#182809=CARTESIAN_POINT('Ctrl Pts',(-19.1904025553865,-12.5134317622461,
115.066526724349)) ;
#182810=CARTESIAN_POINT('Ctrl Pts',(-19.1165986976553,-12.5134317862586,
115.090757722445)) ;
#182811=CARTESIAN_POINT('Ctrl Pts',(-19.1061032795761,-12.4453839092044,
115.058790373407)) ;
#182812=CARTESIAN_POINT('Ctrl Pts',(-19.0956078614969,-12.3773360321503,
115.026823024368)) ;
#182813=CARTESIAN_POINT('Ctrl Pts',(-19.1694117192281,-12.3773360081379,
115.002592026272)) ;
#182814=CARTESIAN_POINT('Ctrl Pts',(-19.2432155769593,-12.3773359841254,
114.978361028176)) ;
#182815=CARTESIAN_POINT('Ctrl Pts',(-19.2537109950385,-12.4453838611795,
115.010328377215)) ;
#182816=CARTESIAN_POINT('Ctrl Pts',(-19.1680396764701,-12.6100760699984,
114.78492817834)) ;
#182817=CARTESIAN_POINT('Ctrl Pts',(-19.1837973550642,-12.6667282433853,
114.832923524027)) ;
#182818=CARTESIAN_POINT('Ctrl Pts',(-19.109993502002,-12.6667282722992,
114.857154536344)) ;
#182819=CARTESIAN_POINT('Ctrl Pts',(-19.0361896489399,-12.6667283012131,
114.881385548662)) ;
#182820=CARTESIAN_POINT('Ctrl Pts',(-19.0204319703459,-12.6100761278262,
114.833390202975)) ;
#182821=CARTESIAN_POINT('Ctrl Pts',(-19.0046742917518,-12.5534239544393,
114.785394857287)) ;
#182822=CARTESIAN_POINT('Ctrl Pts',(-19.078478144814,-12.5534239255254,
114.76116384497)) ;
#182823=CARTESIAN_POINT('Ctrl Pts',(-19.1522819978761,-12.5534238966115,
114.736932832653)) ;
#182824=CARTESIAN_POINT('Ctrl Pts',(-19.1680396764701,-12.6100760699984,
114.78492817834)) ;
#182825=CARTESIAN_POINT('Ctrl Pts',(-19.0989285208918,-12.8316470477012,
114.609808039742)) ;
#182826=CARTESIAN_POINT('Ctrl Pts',(-19.1188033970976,-12.8729143960197,
114.670343705199)) ;
#182827=CARTESIAN_POINT('Ctrl Pts',(-19.0449995481209,-12.8729144255077,
114.694574729961)) ;
#182828=CARTESIAN_POINT('Ctrl Pts',(-18.9711956991442,-12.8729144549957,
114.718805754722)) ;
#182829=CARTESIAN_POINT('Ctrl Pts',(-18.9513208229384,-12.8316471066773,
114.658270089265)) ;
#182830=CARTESIAN_POINT('Ctrl Pts',(-18.9314459467326,-12.7903797583588,
114.597734423807)) ;
#182831=CARTESIAN_POINT('Ctrl Pts',(-19.0052497957093,-12.7903797288708,
114.573503399046)) ;
#182832=CARTESIAN_POINT('Ctrl Pts',(-19.079053644686,-12.7903796993828,
114.549272374285)) ;
#182833=CARTESIAN_POINT('Ctrl Pts',(-19.0989285208918,-12.8316470477012,
114.609808039742)) ;
#182834=CARTESIAN_POINT('Ctrl Pts',(-19.0499531759888,-13.0973555362981,
114.496308559562)) ;
#182835=CARTESIAN_POINT('Ctrl Pts',(-19.0725398327684,-13.1201328482756,
114.5651038713)) ;
#182836=CARTESIAN_POINT('Ctrl Pts',(-18.9987359873466,-13.1201328716907,
114.589334906889)) ;
#182837=CARTESIAN_POINT('Ctrl Pts',(-18.9249321419248,-13.1201328951058,
114.613565942478)) ;
#182838=CARTESIAN_POINT('Ctrl Pts',(-18.9023454851452,-13.0973555831283,
114.54477063074)) ;
#182839=CARTESIAN_POINT('Ctrl Pts',(-18.8797588283656,-13.0745782711508,
114.475975319001)) ;
#182840=CARTESIAN_POINT('Ctrl Pts',(-18.9535626737874,-13.0745782477357,
114.451744283413)) ;
#182841=CARTESIAN_POINT('Ctrl Pts',(-19.0273665192092,-13.0745782243206,
114.427513247824)) ;
#182842=CARTESIAN_POINT('Ctrl Pts',(-19.0499531759888,-13.0973555362981,
114.496308559562)) ;
#182843=CARTESIAN_POINT('Ctrl Pts',(-19.0246223482772,-13.3829827267331,
114.454418834067)) ;
#182844=CARTESIAN_POINT('Ctrl Pts',(-19.0482819521427,-13.3858507921175,
114.526482169625)) ;
#182845=CARTESIAN_POINT('Ctrl Pts',(-18.9744781087354,-13.3858508103817,
114.55071321135)) ;
#182846=CARTESIAN_POINT('Ctrl Pts',(-18.9006742653281,-13.3858508286459,
114.574944253074)) ;
#182847=CARTESIAN_POINT('Ctrl Pts',(-18.8770146614626,-13.3829827632615,
114.502880917516)) ;
#182848=CARTESIAN_POINT('Ctrl Pts',(-18.8533550575971,-13.380114697877,
114.430817581958)) ;
#182849=CARTESIAN_POINT('Ctrl Pts',(-18.9271589010044,-13.3801146796128,
114.406586540234)) ;
#182850=CARTESIAN_POINT('Ctrl Pts',(-19.0009627444117,-13.3801146613487,
114.382355498509)) ;
#182851=CARTESIAN_POINT('Ctrl Pts',(-19.0246223482772,-13.3829827267331,
114.454418834067)) ;
#182852=CARTESIAN_POINT('Ctrl Pts',(-19.0233599186535,-13.6735145155205,
114.486149491012)) ;
#182853=CARTESIAN_POINT('Ctrl Pts',(-19.0464072958713,-13.6561003398034,
114.556348083136)) ;
#182854=CARTESIAN_POINT('Ctrl Pts',(-18.9726034534189,-13.6561003497692,
114.580579127769)) ;
#182855=CARTESIAN_POINT('Ctrl Pts',(-18.8987996109665,-13.656100359735,
114.604810172402)) ;
#182856=CARTESIAN_POINT('Ctrl Pts',(-18.8757522337487,-13.673514535452,
114.534611580278)) ;
#182857=CARTESIAN_POINT('Ctrl Pts',(-18.8527048565308,-13.690928711169,
114.464412988154)) ;
#182858=CARTESIAN_POINT('Ctrl Pts',(-18.9265086989832,-13.6909287012033,
114.440181943521)) ;
#182859=CARTESIAN_POINT('Ctrl Pts',(-19.0003125414356,-13.6909286912375,
114.415950898888)) ;
#182860=CARTESIAN_POINT('Ctrl Pts',(-19.0233599186535,-13.6735145155205,
114.486149491012)) ;
#182861=CARTESIAN_POINT('Ctrl Pts',(-19.0457709783456,-13.9443960540442,
114.589809022558)) ;
#182862=CARTESIAN_POINT('Ctrl Pts',(-19.0665555634341,-13.9080411308625,
114.65311551506)) ;
#182863=CARTESIAN_POINT('Ctrl Pts',(-18.9927517208893,-13.9080411350017,
114.677346559412)) ;
#182864=CARTESIAN_POINT('Ctrl Pts',(-18.9189478783444,-13.9080411391408,
114.701577603763)) ;
#182865=CARTESIAN_POINT('Ctrl Pts',(-18.898163293256,-13.9443960623225,
114.638271111261)) ;
#182866=CARTESIAN_POINT('Ctrl Pts',(-18.8773787081675,-13.9807509855041,
114.574964618758)) ;
#182867=CARTESIAN_POINT('Ctrl Pts',(-18.9511825507123,-13.980750981365,
114.550733574406)) ;
#182868=CARTESIAN_POINT('Ctrl Pts',(-19.0249863932572,-13.9807509772258,
114.526502530055)) ;
#182869=CARTESIAN_POINT('Ctrl Pts',(-19.0457709783456,-13.9443960540442,
114.589809022558)) ;
#182870=CARTESIAN_POINT('Ctrl Pts',(-19.0894428117511,-14.1780473237906,
114.75829138369)) ;
#182871=CARTESIAN_POINT('Ctrl Pts',(-19.1064751505177,-14.125322660068,
114.810169139406)) ;
#182872=CARTESIAN_POINT('Ctrl Pts',(-19.0326713072854,-14.12532266015,114.834400181664)) ;
#182873=CARTESIAN_POINT('Ctrl Pts',(-18.9588674640532,-14.1253226602321,
114.858631223921)) ;
#182874=CARTESIAN_POINT('Ctrl Pts',(-18.9418351252866,-14.1780473239547,
114.806753468205)) ;
#182875=CARTESIAN_POINT('Ctrl Pts',(-18.9248027865201,-14.2307719876773,
114.754875712489)) ;
#182876=CARTESIAN_POINT('Ctrl Pts',(-18.9986066297524,-14.2307719875953,
114.730644670231)) ;
#182877=CARTESIAN_POINT('Ctrl Pts',(-19.0724104729846,-14.2307719875132,
114.706413627973)) ;
#182878=CARTESIAN_POINT('Ctrl Pts',(-19.0894428117511,-14.1780473237906,
114.75829138369)) ;
#182879=CARTESIAN_POINT('Ctrl Pts',(-19.1503829732197,-14.3571729772058,
114.97930953691)) ;
#182880=CARTESIAN_POINT('Ctrl Pts',(-19.1624527588711,-14.2918617658065,
115.016072156599)) ;
#182881=CARTESIAN_POINT('Ctrl Pts',(-19.088648914819,-14.2918617643923,
115.04030319636)) ;
#182882=CARTESIAN_POINT('Ctrl Pts',(-19.0148450707669,-14.291861762978,
115.064534236121)) ;
#182883=CARTESIAN_POINT('Ctrl Pts',(-19.0027752851155,-14.3571729743773,
115.027771616431)) ;
#182884=CARTESIAN_POINT('Ctrl Pts',(-18.9907054994641,-14.4224841857766,
114.991008996742)) ;
#182885=CARTESIAN_POINT('Ctrl Pts',(-19.0645093435162,-14.4224841871909,
114.966777956981)) ;
#182886=CARTESIAN_POINT('Ctrl Pts',(-19.1383131875683,-14.4224841886051,
114.942546917221)) ;
#182887=CARTESIAN_POINT('Ctrl Pts',(-19.1503829732197,-14.3571729772058,
114.97930953691)) ;
#182888=CARTESIAN_POINT('Ctrl Pts',(-19.2242001392869,-14.4697035049953,
115.239834214336)) ;
#182889=CARTESIAN_POINT('Ctrl Pts',(-19.2303944994986,-14.3964364704153,
115.258701236151)) ;
#182890=CARTESIAN_POINT('Ctrl Pts',(-19.1565906550596,-14.3964364695808,
115.282932274733)) ;
#182891=CARTESIAN_POINT('Ctrl Pts',(-19.0827868106205,-14.3964364687462,
115.307163313314)) ;
#182892=CARTESIAN_POINT('Ctrl Pts',(-19.0765924504088,-14.4697035033262,
115.2882962915)) ;
#182893=CARTESIAN_POINT('Ctrl Pts',(-19.0703980901972,-14.5429705379062,
115.269429269686)) ;
#182894=CARTESIAN_POINT('Ctrl Pts',(-19.1442019346362,-14.5429705387408,
115.245198231104)) ;
#182895=CARTESIAN_POINT('Ctrl Pts',(-19.2180057790753,-14.5429705395753,
115.220967192522)) ;
#182896=CARTESIAN_POINT('Ctrl Pts',(-19.2242001392869,-14.4697035049953,
115.239834214336)) ;
#182897=CARTESIAN_POINT('Ctrl Pts',(-19.3035102564175,-14.5058316151569,
115.516726782394)) ;
#182898=CARTESIAN_POINT('Ctrl Pts',(-19.3034446215456,-14.4299343068103,
115.5165268692)) ;
#182899=CARTESIAN_POINT('Ctrl Pts',(-19.2296407775637,-14.4299343070279,
115.540757909174)) ;
#182900=CARTESIAN_POINT('Ctrl Pts',(-19.1558369335817,-14.4299343072455,
115.564988949148)) ;
#182901=CARTESIAN_POINT('Ctrl Pts',(-19.1559025684536,-14.5058316155922,
115.565188862343)) ;
#182902=CARTESIAN_POINT('Ctrl Pts',(-19.1559682033254,-14.5817289239388,
115.565388775537)) ;
#182903=CARTESIAN_POINT('Ctrl Pts',(-19.2297720473073,-14.5817289237212,
115.541157735563)) ;
#182904=CARTESIAN_POINT('Ctrl Pts',(-19.3035758912893,-14.5817289235035,
115.516926695588)) ;
#182905=CARTESIAN_POINT('Ctrl Pts',(-19.3035102564175,-14.5058316151569,
115.516726782394)) ;
#182906=CARTESIAN_POINT('Ctrl Pts',(-19.3827642308923,-14.4647781183691,
115.793520482864)) ;
#182907=CARTESIAN_POINT('Ctrl Pts',(-19.3764319338488,-14.3916362177671,
115.774233327761)) ;
#182908=CARTESIAN_POINT('Ctrl Pts',(-19.3026280907892,-14.3916362178144,
115.798464370545)) ;
#182909=CARTESIAN_POINT('Ctrl Pts',(-19.2288242477297,-14.3916362178617,
115.822695413328)) ;
#182910=CARTESIAN_POINT('Ctrl Pts',(-19.2351565447731,-14.4647781184637,
115.841982568431)) ;
#182911=CARTESIAN_POINT('Ctrl Pts',(-19.2414888418166,-14.5379200190658,
115.861269723533)) ;
#182912=CARTESIAN_POINT('Ctrl Pts',(-19.3152926848761,-14.5379200190184,
115.83703868075)) ;
#182913=CARTESIAN_POINT('Ctrl Pts',(-19.3890965279357,-14.5379200189711,
115.812807637966)) ;
#182914=CARTESIAN_POINT('Ctrl Pts',(-19.3827642308923,-14.4647781183691,
115.793520482864)) ;
#182915=CARTESIAN_POINT('Ctrl Pts',(-19.4555982839664,-14.3484987257117,
116.050853216229)) ;
#182916=CARTESIAN_POINT('Ctrl Pts',(-19.4434365510196,-14.2833691759875,
116.013810539845)) ;
#182917=CARTESIAN_POINT('Ctrl Pts',(-19.3696327093056,-14.2833691732841,
116.038041586727)) ;
#182918=CARTESIAN_POINT('Ctrl Pts',(-19.2958288675915,-14.2833691705807,
116.062272633608)) ;
#182919=CARTESIAN_POINT('Ctrl Pts',(-19.3079906005384,-14.3484987203049,
116.099315309993)) ;
#182920=CARTESIAN_POINT('Ctrl Pts',(-19.3201523334852,-14.4136282700291,
116.136357986378)) ;
#182921=CARTESIAN_POINT('Ctrl Pts',(-19.3939561751992,-14.4136282727325,
116.112126939496)) ;
#182922=CARTESIAN_POINT('Ctrl Pts',(-19.4677600169133,-14.4136282754358,
116.087895892614)) ;
#182923=CARTESIAN_POINT('Ctrl Pts',(-19.4555982839664,-14.3484987257117,
116.050853216229)) ;
#182924=CARTESIAN_POINT('Ctrl Pts',(-19.5158156777424,-14.1655053892491,
116.26975198964)) ;
#182925=CARTESIAN_POINT('Ctrl Pts',(-19.4986972476325,-14.1130583565086,
116.217612013334)) ;
#182926=CARTESIAN_POINT('Ctrl Pts',(-19.4248934070266,-14.1130583479537,
116.241843063591)) ;
#182927=CARTESIAN_POINT('Ctrl Pts',(-19.3510895664207,-14.1130583393988,
116.266074113848)) ;
#182928=CARTESIAN_POINT('Ctrl Pts',(-19.3682079965306,-14.1655053721393,
116.318214090154)) ;
#182929=CARTESIAN_POINT('Ctrl Pts',(-19.3853264266405,-14.2179524048798,
116.370354066459)) ;
#182930=CARTESIAN_POINT('Ctrl Pts',(-19.4591302672464,-14.2179524134347,
116.346123016202)) ;
#182931=CARTESIAN_POINT('Ctrl Pts',(-19.5329341078523,-14.2179524219896,
116.321891965945)) ;
#182932=CARTESIAN_POINT('Ctrl Pts',(-19.5158156777424,-14.1655053892491,
116.26975198964)) ;
#182933=CARTESIAN_POINT('Ctrl Pts',(-19.5583308176863,-13.9286208259661,
116.434763630565)) ;
#182934=CARTESIAN_POINT('Ctrl Pts',(-19.537483987011,-13.8926376196403,
116.371267547564)) ;
#182935=CARTESIAN_POINT('Ctrl Pts',(-19.4636801467042,-13.8926376022121,
116.395498598732)) ;
#182936=CARTESIAN_POINT('Ctrl Pts',(-19.3898763063974,-13.8926375847838,
116.4197296499)) ;
#182937=CARTESIAN_POINT('Ctrl Pts',(-19.4107231370728,-13.9286207911095,
116.483225732902)) ;
#182938=CARTESIAN_POINT('Ctrl Pts',(-19.4315699677482,-13.9646039974353,
116.546721815903)) ;
#182939=CARTESIAN_POINT('Ctrl Pts',(-19.5053738080549,-13.9646040148635,
116.522490764735)) ;
#182940=CARTESIAN_POINT('Ctrl Pts',(-19.5791776483617,-13.9646040322918,
116.498259713567)) ;
#182941=CARTESIAN_POINT('Ctrl Pts',(-19.5583308176863,-13.9286208259661,
116.434763630565)) ;
#182942=CARTESIAN_POINT('Ctrl Pts',(-19.5793222342617,-13.6565946963034,
116.5340328038)) ;
#182943=CARTESIAN_POINT('Ctrl Pts',(-19.5562485424584,-13.6395527561257,
116.463754060976)) ;
#182944=CARTESIAN_POINT('Ctrl Pts',(-19.4824447011078,-13.6395527301396,
116.487985108965)) ;
#182945=CARTESIAN_POINT('Ctrl Pts',(-19.4086408597573,-13.6395527041535,
116.512216156954)) ;
#182946=CARTESIAN_POINT('Ctrl Pts',(-19.4317145515606,-13.6565946443312,
116.582494899778)) ;
#182947=CARTESIAN_POINT('Ctrl Pts',(-19.4547882433639,-13.6736365845089,
116.652773642602)) ;
#182948=CARTESIAN_POINT('Ctrl Pts',(-19.5285920847144,-13.673636610495,
116.628542594613)) ;
#182949=CARTESIAN_POINT('Ctrl Pts',(-19.6023959260649,-13.6736366364811,
116.604311546624)) ;
#182950=CARTESIAN_POINT('Ctrl Pts',(-19.5793222342617,-13.6565946963034,
116.5340328038)) ;
#182951=CARTESIAN_POINT('Ctrl Pts',(-19.5766443908906,-13.3650274692435,
116.561521687916)) ;
#182952=CARTESIAN_POINT('Ctrl Pts',(-19.5529865212982,-13.3683183370286,
116.489463633607)) ;
#182953=CARTESIAN_POINT('Ctrl Pts',(-19.4791826776011,-13.368318300107,
116.513694674449)) ;
#182954=CARTESIAN_POINT('Ctrl Pts',(-19.4053788339039,-13.3683182631854,
116.537925715291)) ;
#182955=CARTESIAN_POINT('Ctrl Pts',(-19.4290367034963,-13.3650273954003,
116.6099837696)) ;
#182956=CARTESIAN_POINT('Ctrl Pts',(-19.4526945730887,-13.3617365276153,
116.682041823909)) ;
#182957=CARTESIAN_POINT('Ctrl Pts',(-19.5264984167859,-13.3617365645369,
116.657810783067)) ;
#182958=CARTESIAN_POINT('Ctrl Pts',(-19.6003022604831,-13.3617366014585,
116.633579742225)) ;
#182959=CARTESIAN_POINT('Ctrl Pts',(-19.5766443908906,-13.3650274692435,
116.561521687916)) ;
#182960=CARTESIAN_POINT('Ctrl Pts',(-19.5495669925005,-13.0788343995772,
116.514498473725)) ;
#182961=CARTESIAN_POINT('Ctrl Pts',(-19.5270319383932,-13.1021119946019,
116.445860334053)) ;
#182962=CARTESIAN_POINT('Ctrl Pts',(-19.4532280907541,-13.1021119511676,
116.470091362888)) ;
#182963=CARTESIAN_POINT('Ctrl Pts',(-19.379424243115,-13.1021119077334,
116.494322391723)) ;
#182964=CARTESIAN_POINT('Ctrl Pts',(-19.4019592972223,-13.0788343127088,
116.562960531395)) ;
#182965=CARTESIAN_POINT('Ctrl Pts',(-19.4244943513295,-13.0555567176841,
116.631598671068)) ;
#182966=CARTESIAN_POINT('Ctrl Pts',(-19.4982981989686,-13.0555567611183,
116.607367642232)) ;
#182967=CARTESIAN_POINT('Ctrl Pts',(-19.5721020466077,-13.0555568045526,
116.583136613397)) ;
#182968=CARTESIAN_POINT('Ctrl Pts',(-19.5495669925005,-13.0788343995772,
116.514498473725)) ;
#182969=CARTESIAN_POINT('Ctrl Pts',(-19.4996422792964,-12.8175211583994,
116.397794021949)) ;
#182970=CARTESIAN_POINT('Ctrl Pts',(-19.4798288097377,-12.8590768776832,
116.337445389538)) ;
#182971=CARTESIAN_POINT('Ctrl Pts',(-19.4060249573596,-12.8590768329722,
116.361676403939)) ;
#182972=CARTESIAN_POINT('Ctrl Pts',(-19.3322211049816,-12.8590767882613,
116.38590741834)) ;
#182973=CARTESIAN_POINT('Ctrl Pts',(-19.3520345745402,-12.8175210689774,
116.446256050751)) ;
#182974=CARTESIAN_POINT('Ctrl Pts',(-19.3718480440989,-12.7759653496935,
116.506604683163)) ;
#182975=CARTESIAN_POINT('Ctrl Pts',(-19.445651896477,-12.7759653944045,
116.482373668762)) ;
#182976=CARTESIAN_POINT('Ctrl Pts',(-19.519455748855,-12.7759654391155,
116.458142654361)) ;
#182977=CARTESIAN_POINT('Ctrl Pts',(-19.4996422792964,-12.8175211583994,
116.397794021949)) ;
#182978=CARTESIAN_POINT('Ctrl Pts',(-19.4293404722098,-12.5984995679009,
116.219119607498)) ;
#182979=CARTESIAN_POINT('Ctrl Pts',(-19.4136731235186,-12.6554070787726,
116.171399390111)) ;
#182980=CARTESIAN_POINT('Ctrl Pts',(-19.3398692657786,-12.6554070377801,
116.195630388181)) ;
#182981=CARTESIAN_POINT('Ctrl Pts',(-19.2660654080387,-12.6554069967877,
116.21986138625)) ;
#182982=CARTESIAN_POINT('Ctrl Pts',(-19.2817327567299,-12.5984994859161,
116.267581603637)) ;
#182983=CARTESIAN_POINT('Ctrl Pts',(-19.2974001054211,-12.5415919750444,
116.315301821023)) ;
#182984=CARTESIAN_POINT('Ctrl Pts',(-19.3712039631611,-12.5415920160368,
116.291070822954)) ;
#182985=CARTESIAN_POINT('Ctrl Pts',(-19.445007820901,-12.5415920570292,
116.266839824884)) ;
#182986=CARTESIAN_POINT('Ctrl Pts',(-19.4293404722098,-12.5984995679009,
116.219119607498)) ;
#182987=CARTESIAN_POINT('Ctrl Pts',(-19.3431976343271,-12.4381081950322,
115.992149215875)) ;
#182988=CARTESIAN_POINT('Ctrl Pts',(-19.3327893138113,-12.5062960463662,
115.960447149621)) ;
#182989=CARTESIAN_POINT('Ctrl Pts',(-19.2589854510198,-12.5062960154841,
115.984678132304)) ;
#182990=CARTESIAN_POINT('Ctrl Pts',(-19.1851815882283,-12.506295984602,
116.008909114987)) ;
#182991=CARTESIAN_POINT('Ctrl Pts',(-19.1955899087441,-12.4381081332681,
116.040611181242)) ;
#182992=CARTESIAN_POINT('Ctrl Pts',(-19.2059982292598,-12.3699202819341,
116.072313247497)) ;
#182993=CARTESIAN_POINT('Ctrl Pts',(-19.2798020920513,-12.3699203128162,
116.048082264814)) ;
#182994=CARTESIAN_POINT('Ctrl Pts',(-19.3536059548428,-12.3699203436983,
116.02385128213)) ;
#182995=CARTESIAN_POINT('Ctrl Pts',(-19.3431976343271,-12.4381081950322,
115.992149215875)) ;
#182996=CARTESIAN_POINT('Ctrl Pts',(-19.2456411710222,-12.3474840033873,
115.730719198245)) ;
#182997=CARTESIAN_POINT('Ctrl Pts',(-19.2412898424851,-12.4220984887537,
115.717465752075)) ;
#182998=CARTESIAN_POINT('Ctrl Pts',(-19.1674859748129,-12.4220984739895,
115.741696719893)) ;
#182999=CARTESIAN_POINT('Ctrl Pts',(-19.0936821071408,-12.4220984592253,
115.76592768771)) ;
#183000=CARTESIAN_POINT('Ctrl Pts',(-19.0980334356779,-12.3474839738589,
115.779181133881)) ;
#183001=CARTESIAN_POINT('Ctrl Pts',(-19.1023847642151,-12.2728694884925,
115.792434580051)) ;
#183002=CARTESIAN_POINT('Ctrl Pts',(-19.1761886318872,-12.2728695032567,
115.768203612233)) ;
#183003=CARTESIAN_POINT('Ctrl Pts',(-19.2499924995594,-12.2728695180209,
115.743972644416)) ;
#183004=CARTESIAN_POINT('Ctrl Pts',(-19.2456411710222,-12.3474840033873,
115.730719198245)) ;
#183005=CARTESIAN_POINT('Ctrl Pts',(-19.1449743145035,-12.3342746176406,
115.45936107608)) ;
#183006=CARTESIAN_POINT('Ctrl Pts',(-19.1469154659611,-12.4099190416296,
115.465273508583)) ;
#183007=CARTESIAN_POINT('Ctrl Pts',(-19.0731115962662,-12.4099190485564,
115.489504470239)) ;
#183008=CARTESIAN_POINT('Ctrl Pts',(-18.9993077265714,-12.4099190554831,
115.513735431896)) ;
#183009=CARTESIAN_POINT('Ctrl Pts',(-18.9973665751139,-12.3342746314941,
115.507822999394)) ;
#183010=CARTESIAN_POINT('Ctrl Pts',(-18.9954254236563,-12.2586302075051,
115.501910566892)) ;
#183011=CARTESIAN_POINT('Ctrl Pts',(-19.0692292933512,-12.2586302005783,
115.477679605235)) ;
#183012=CARTESIAN_POINT('Ctrl Pts',(-19.143033163046,-12.2586301936515,
115.453448643578)) ;
#183013=CARTESIAN_POINT('Ctrl Pts',(-19.1449743145035,-12.3342746176406,
115.45936107608)) ;
#183014=CARTESIAN_POINT('Ctrl Pts',(-19.0456937210243,-12.3983523506611,
115.192496748361)) ;
#183015=CARTESIAN_POINT('Ctrl Pts',(-19.0538339702952,-12.4696333213927,
115.21729063245)) ;
#183016=CARTESIAN_POINT('Ctrl Pts',(-18.9800301001254,-12.4696333527669,
115.24152159266)) ;
#183017=CARTESIAN_POINT('Ctrl Pts',(-18.9062262299556,-12.4696333841411,
115.26575255287)) ;
#183018=CARTESIAN_POINT('Ctrl Pts',(-18.8980859806847,-12.3983524134095,
115.240958668781)) ;
#183019=CARTESIAN_POINT('Ctrl Pts',(-18.8899457314137,-12.3270714426779,
115.216164784692)) ;
#183020=CARTESIAN_POINT('Ctrl Pts',(-18.9637496015835,-12.3270714113037,
115.191933824481)) ;
#183021=CARTESIAN_POINT('Ctrl Pts',(-19.0375534717533,-12.3270713799295,
115.167702864271)) ;
#183022=CARTESIAN_POINT('Ctrl Pts',(-19.0456937210243,-12.3983523506611,
115.192496748361)) ;
#183023=CARTESIAN_POINT('Ctrl Pts',(-18.9551049831602,-12.5353914606374,
114.952015661837)) ;
#183024=CARTESIAN_POINT('Ctrl Pts',(-18.9688484070963,-12.5972087494759,
114.993875911784)) ;
#183025=CARTESIAN_POINT('Ctrl Pts',(-18.8950445391368,-12.5972088056809,
115.018106878726)) ;
#183026=CARTESIAN_POINT('Ctrl Pts',(-18.8212406711773,-12.5972088618859,
115.042337845668)) ;
#183027=CARTESIAN_POINT('Ctrl Pts',(-18.8074972472412,-12.5353915730474,
115.000477595721)) ;
#183028=CARTESIAN_POINT('Ctrl Pts',(-18.7937538233051,-12.4735742842089,
114.958617345773)) ;
#183029=CARTESIAN_POINT('Ctrl Pts',(-18.8675576912646,-12.4735742280039,
114.934386378831)) ;
#183030=CARTESIAN_POINT('Ctrl Pts',(-18.9413615592241,-12.4735741717989,
114.910155411889)) ;
#183031=CARTESIAN_POINT('Ctrl Pts',(-18.9551049831602,-12.5353914606374,
114.952015661837)) ;
#183032=CARTESIAN_POINT('Ctrl Pts',(-18.8783820413473,-12.7368848040207,
114.753966045534)) ;
#183033=CARTESIAN_POINT('Ctrl Pts',(-18.8967647782412,-12.7847255574639,
114.8099568941)) ;
#183034=CARTESIAN_POINT('Ctrl Pts',(-18.8229609148592,-12.7847256367286,
114.834187874984)) ;
#183035=CARTESIAN_POINT('Ctrl Pts',(-18.7491570514771,-12.7847257159933,
114.858418855869)) ;
#183036=CARTESIAN_POINT('Ctrl Pts',(-18.7307743145832,-12.7368849625501,
114.802428007303)) ;
#183037=CARTESIAN_POINT('Ctrl Pts',(-18.7123915776892,-12.6890442091069,
114.746437158737)) ;
#183038=CARTESIAN_POINT('Ctrl Pts',(-18.7861954410713,-12.6890441298422,
114.722206177853)) ;
#183039=CARTESIAN_POINT('Ctrl Pts',(-18.8599993044534,-12.6890440505775,
114.697975196968)) ;
#183040=CARTESIAN_POINT('Ctrl Pts',(-18.8783820413473,-12.7368848040207,
114.753966045534)) ;
#183041=CARTESIAN_POINT('Ctrl Pts',(-18.8212505018881,-12.9849643669818,
114.615234103962)) ;
#183042=CARTESIAN_POINT('Ctrl Pts',(-18.8429187755215,-13.0155548424745,
114.681232167266)) ;
#183043=CARTESIAN_POINT('Ctrl Pts',(-18.7691149190821,-13.0155549383142,
114.705463169296)) ;
#183044=CARTESIAN_POINT('Ctrl Pts',(-18.6953110626427,-13.0155550341539,
114.729694171327)) ;
#183045=CARTESIAN_POINT('Ctrl Pts',(-18.6736427890092,-12.9849645586612,
114.663696108023)) ;
#183046=CARTESIAN_POINT('Ctrl Pts',(-18.6519745153757,-12.9543740831685,
114.597698044719)) ;
#183047=CARTESIAN_POINT('Ctrl Pts',(-18.7257783718151,-12.9543739873288,
114.573467042688)) ;
#183048=CARTESIAN_POINT('Ctrl Pts',(-18.7995822282546,-12.9543738914891,
114.549236040658)) ;
#183049=CARTESIAN_POINT('Ctrl Pts',(-18.8212505018881,-12.9849643669818,
114.615234103962)) ;
#183050=CARTESIAN_POINT('Ctrl Pts',(-18.785989087223,-13.2657001242146,
114.543367393447)) ;
#183051=CARTESIAN_POINT('Ctrl Pts',(-18.8094158544499,-13.2767359206685,
114.614721544454)) ;
#183052=CARTESIAN_POINT('Ctrl Pts',(-18.7356120063235,-13.2767360267194,
114.638952571805)) ;
#183053=CARTESIAN_POINT('Ctrl Pts',(-18.6618081581972,-13.2767361327703,
114.663183599156)) ;
#183054=CARTESIAN_POINT('Ctrl Pts',(-18.6383813909702,-13.2657003363164,
114.591829448148)) ;
#183055=CARTESIAN_POINT('Ctrl Pts',(-18.6149546237433,-13.2546645398624,
114.52047529714)) ;
#183056=CARTESIAN_POINT('Ctrl Pts',(-18.6887584718697,-13.2546644338116,
114.496244269789)) ;
#183057=CARTESIAN_POINT('Ctrl Pts',(-18.762562319996,-13.2546643277607,
114.472013242439)) ;
#183058=CARTESIAN_POINT('Ctrl Pts',(-18.785989087223,-13.2657001242146,
114.543367393447)) ;
#183059=CARTESIAN_POINT('Ctrl Pts',(-18.7749409518522,-13.5562446654925,
114.545103589634)) ;
#183060=CARTESIAN_POINT('Ctrl Pts',(-18.7984413535009,-13.5470119024509,
114.616682019189)) ;
#183061=CARTESIAN_POINT('Ctrl Pts',(-18.7246375143752,-13.5470120097675,
114.640913073955)) ;
#183062=CARTESIAN_POINT('Ctrl Pts',(-18.6508336752495,-13.5470121170841,
114.66514412872)) ;
#183063=CARTESIAN_POINT('Ctrl Pts',(-18.6273332736008,-13.5562448801257,
114.593565699165)) ;
#183064=CARTESIAN_POINT('Ctrl Pts',(-18.6038328719521,-13.5654776431673,
114.52198726961)) ;
#183065=CARTESIAN_POINT('Ctrl Pts',(-18.6776367110778,-13.5654775358507,
114.497756214844)) ;
#183066=CARTESIAN_POINT('Ctrl Pts',(-18.7514405502036,-13.5654774285341,
114.473525160079)) ;
#183067=CARTESIAN_POINT('Ctrl Pts',(-18.7749409518522,-13.5562446654925,
114.545103589634)) ;
#183068=CARTESIAN_POINT('Ctrl Pts',(-18.7878772786409,-13.837740260252,
114.619989429758)) ;
#183069=CARTESIAN_POINT('Ctrl Pts',(-18.8097751113286,-13.8088409661864,
114.686686692827)) ;
#183070=CARTESIAN_POINT('Ctrl Pts',(-18.7359712810008,-13.8088410662031,
114.710917774389)) ;
#183071=CARTESIAN_POINT('Ctrl Pts',(-18.6621674506729,-13.8088411662199,
114.735148855951)) ;
#183072=CARTESIAN_POINT('Ctrl Pts',(-18.6402696179852,-13.8377404602855,
114.668451592882)) ;
#183073=CARTESIAN_POINT('Ctrl Pts',(-18.6183717852975,-13.8666397543512,
114.601754329814)) ;
#183074=CARTESIAN_POINT('Ctrl Pts',(-18.6921756156254,-13.8666396543344,
114.577523248252)) ;
#183075=CARTESIAN_POINT('Ctrl Pts',(-18.7659794459532,-13.8666395543177,
114.553292166689)) ;
#183076=CARTESIAN_POINT('Ctrl Pts',(-18.7878772786409,-13.837740260252,
114.619989429758)) ;
#183077=CARTESIAN_POINT('Ctrl Pts',(-18.823586104698,-14.0900089023239,
114.76439949876)) ;
#183078=CARTESIAN_POINT('Ctrl Pts',(-18.8422860154947,-14.0434540249531,
114.821356407761)) ;
#183079=CARTESIAN_POINT('Ctrl Pts',(-18.7684821927334,-14.0434541089459,
114.845587512369)) ;
#183080=CARTESIAN_POINT('Ctrl Pts',(-18.694678369972,-14.0434541929387,
114.869818616978)) ;
#183081=CARTESIAN_POINT('Ctrl Pts',(-18.6759784591753,-14.0900090703095,
114.812861707977)) ;
#183082=CARTESIAN_POINT('Ctrl Pts',(-18.6572785483786,-14.1365639476803,
114.755904798977)) ;
#183083=CARTESIAN_POINT('Ctrl Pts',(-18.73108237114,-14.1365638636875,114.731673694368)) ;
#183084=CARTESIAN_POINT('Ctrl Pts',(-18.8048861939013,-14.1365637796947,
114.70744258976)) ;
#183085=CARTESIAN_POINT('Ctrl Pts',(-18.823586104698,-14.0900089023239,
114.76439949876)) ;
#183086=CARTESIAN_POINT('Ctrl Pts',(-18.8778061466655,-14.2916996646196,
114.964766086765)) ;
#183087=CARTESIAN_POINT('Ctrl Pts',(-18.8920194354158,-14.2309943169081,
115.008057468957)) ;
#183088=CARTESIAN_POINT('Ctrl Pts',(-18.8182156184406,-14.230994379438,
115.03228859119)) ;
#183089=CARTESIAN_POINT('Ctrl Pts',(-18.7444118014655,-14.2309944419679,
115.056519713422)) ;
#183090=CARTESIAN_POINT('Ctrl Pts',(-18.7301985127151,-14.2916997896794,
115.01322833123)) ;
#183091=CARTESIAN_POINT('Ctrl Pts',(-18.7159852239648,-14.3524051373909,
114.969936949037)) ;
#183092=CARTESIAN_POINT('Ctrl Pts',(-18.7897890409399,-14.352405074861,
114.945705826805)) ;
#183093=CARTESIAN_POINT('Ctrl Pts',(-18.8635928579151,-14.352405012331,
114.921474704573)) ;
#183094=CARTESIAN_POINT('Ctrl Pts',(-18.8778061466655,-14.2916996646196,
114.964766086765)) ;
#183095=CARTESIAN_POINT('Ctrl Pts',(-18.9472129540579,-14.4330905333239,
115.211832429368)) ;
#183096=CARTESIAN_POINT('Ctrl Pts',(-18.9558639366158,-14.362422601594,
115.23818192445)) ;
#183097=CARTESIAN_POINT('Ctrl Pts',(-18.8820601227543,-14.3624226376889,
115.262413056166)) ;
#183098=CARTESIAN_POINT('Ctrl Pts',(-18.8082563088927,-14.3624226737838,
115.286644187882)) ;
#183099=CARTESIAN_POINT('Ctrl Pts',(-18.7996053263348,-14.4330906055137,
115.2602946928)) ;
#183100=CARTESIAN_POINT('Ctrl Pts',(-18.7909543437769,-14.5037585372437,
115.233945197718)) ;
#183101=CARTESIAN_POINT('Ctrl Pts',(-18.8647581576385,-14.5037585011487,
115.209714066002)) ;
#183102=CARTESIAN_POINT('Ctrl Pts',(-18.9385619715001,-14.5037584650538,
115.185482934287)) ;
#183103=CARTESIAN_POINT('Ctrl Pts',(-18.9472129540579,-14.4330905333239,
115.211832429368)) ;
#183104=CARTESIAN_POINT('Ctrl Pts',(-19.0250383188823,-14.5004556458798,
115.484322413278)) ;
#183105=CARTESIAN_POINT('Ctrl Pts',(-19.0275352173107,-14.424978464963,
115.491927561146)) ;
#183106=CARTESIAN_POINT('Ctrl Pts',(-18.9537314039739,-14.4249784742085,
115.51615869446)) ;
#183107=CARTESIAN_POINT('Ctrl Pts',(-18.879927590637,-14.4249784834539,
115.540389827774)) ;
#183108=CARTESIAN_POINT('Ctrl Pts',(-18.8774306922086,-14.5004556643706,
115.532784679906)) ;
#183109=CARTESIAN_POINT('Ctrl Pts',(-18.8749337937802,-14.5759328452874,
115.525179532038)) ;
#183110=CARTESIAN_POINT('Ctrl Pts',(-18.9487376071171,-14.5759328360419,
115.500948398724)) ;
#183111=CARTESIAN_POINT('Ctrl Pts',(-19.0225414204539,-14.5759328267965,
115.47671726541)) ;
#183112=CARTESIAN_POINT('Ctrl Pts',(-19.0250383188823,-14.5004556458798,
115.484322413278)) ;
#183113=CARTESIAN_POINT('Ctrl Pts',(-19.1050415480743,-14.4906784452632,
115.763353035226)) ;
#183114=CARTESIAN_POINT('Ctrl Pts',(-19.1012249635907,-14.4157707960699,
115.751728332911)) ;
#183115=CARTESIAN_POINT('Ctrl Pts',(-19.0274211485121,-14.4157707802425,
115.77595946092)) ;
#183116=CARTESIAN_POINT('Ctrl Pts',(-18.9536173334336,-14.4157707644151,
115.80019058893)) ;
#183117=CARTESIAN_POINT('Ctrl Pts',(-18.9574339179171,-14.4906784136084,
115.811815291245)) ;
#183118=CARTESIAN_POINT('Ctrl Pts',(-18.9612505024007,-14.5655860628017,
115.82343999356)) ;
#183119=CARTESIAN_POINT('Ctrl Pts',(-19.0350543174793,-14.5655860786291,
115.79920886555)) ;
#183120=CARTESIAN_POINT('Ctrl Pts',(-19.1088581325578,-14.5655860944565,
115.774977737541)) ;
#183121=CARTESIAN_POINT('Ctrl Pts',(-19.1050415480743,-14.4906784452632,
115.763353035226)) ;
#183122=CARTESIAN_POINT('Ctrl Pts',(-19.1811866606781,-14.4044504861589,
116.030699387926)) ;
#183123=CARTESIAN_POINT('Ctrl Pts',(-19.171315094255,-14.3354504116019,
116.000632187703)) ;
#183124=CARTESIAN_POINT('Ctrl Pts',(-19.0975112751908,-14.3354503745246,
116.024863303572)) ;
#183125=CARTESIAN_POINT('Ctrl Pts',(-19.0237074561265,-14.3354503374474,
116.049094419442)) ;
#183126=CARTESIAN_POINT('Ctrl Pts',(-19.0335790225497,-14.4044504120043,
116.079161619665)) ;
#183127=CARTESIAN_POINT('Ctrl Pts',(-19.0434505889729,-14.4734504865613,
116.109228819889)) ;
#183128=CARTESIAN_POINT('Ctrl Pts',(-19.1172544080371,-14.4734505236385,
116.084997704019)) ;
#183129=CARTESIAN_POINT('Ctrl Pts',(-19.1910582271013,-14.4734505607158,
116.06076658815)) ;
#183130=CARTESIAN_POINT('Ctrl Pts',(-19.1811866606781,-14.4044504861589,
116.030699387926)) ;
#183131=CARTESIAN_POINT('Ctrl Pts',(-19.2474615033651,-14.2464177648016,
116.26820558113)) ;
#183132=CARTESIAN_POINT('Ctrl Pts',(-19.2322101937286,-14.1883465874269,
116.22175255126)) ;
#183133=CARTESIAN_POINT('Ctrl Pts',(-19.1584063686785,-14.1883465362759,
116.245983648898)) ;
#183134=CARTESIAN_POINT('Ctrl Pts',(-19.0846025436284,-14.1883464851249,
116.270214746535)) ;
#183135=CARTESIAN_POINT('Ctrl Pts',(-19.0998538532649,-14.2464176624996,
116.316667776405)) ;
#183136=CARTESIAN_POINT('Ctrl Pts',(-19.1151051629013,-14.3044888398743,
116.363120806274)) ;
#183137=CARTESIAN_POINT('Ctrl Pts',(-19.1889089879514,-14.3044888910253,
116.338889708637)) ;
#183138=CARTESIAN_POINT('Ctrl Pts',(-19.2627128130015,-14.3044889421763,
116.314658611)) ;
#183139=CARTESIAN_POINT('Ctrl Pts',(-19.2474615033651,-14.2464177648016,
116.26820558113)) ;
#183140=CARTESIAN_POINT('Ctrl Pts',(-19.2975522404832,-14.0296079395376,
116.456228657709)) ;
#183141=CARTESIAN_POINT('Ctrl Pts',(-19.2780468758366,-13.9865865421538,
116.396818462815)) ;
#183142=CARTESIAN_POINT('Ctrl Pts',(-19.2042430445828,-13.9865864836806,
116.421049541558)) ;
#183143=CARTESIAN_POINT('Ctrl Pts',(-19.1304392133291,-13.9865864252074,
116.4452806203)) ;
#183144=CARTESIAN_POINT('Ctrl Pts',(-19.1499445779758,-14.0296078225912,
116.504690815193)) ;
#183145=CARTESIAN_POINT('Ctrl Pts',(-19.1694499426224,-14.072629219975,
116.564101010086)) ;
#183146=CARTESIAN_POINT('Ctrl Pts',(-19.2432537738762,-14.0726292784482,
116.539869931344)) ;
#183147=CARTESIAN_POINT('Ctrl Pts',(-19.3170576051299,-14.0726293369214,
116.515638852602)) ;
#183148=CARTESIAN_POINT('Ctrl Pts',(-19.2975522404832,-14.0296079395376,
116.456228657709)) ;
#183149=CARTESIAN_POINT('Ctrl Pts',(-19.3275320163761,-13.7700542634679,
116.582883427607)) ;
#183150=CARTESIAN_POINT('Ctrl Pts',(-19.3051727068637,-13.7450900092007,
116.514780577272)) ;
#183151=CARTESIAN_POINT('Ctrl Pts',(-19.2313688696332,-13.7450899491233,
116.539011637809)) ;
#183152=CARTESIAN_POINT('Ctrl Pts',(-19.1575650324027,-13.7450898890458,
116.563242698347)) ;
#183153=CARTESIAN_POINT('Ctrl Pts',(-19.179924341915,-13.7700541433129,
116.631345548683)) ;
#183154=CARTESIAN_POINT('Ctrl Pts',(-19.2022836514274,-13.79501839758,116.699448399019)) ;
#183155=CARTESIAN_POINT('Ctrl Pts',(-19.2760874886579,-13.7950184576575,
116.675217338481)) ;
#183156=CARTESIAN_POINT('Ctrl Pts',(-19.3498913258885,-13.795018517735,
116.650986277943)) ;
#183157=CARTESIAN_POINT('Ctrl Pts',(-19.3275320163761,-13.7700542634679,
116.582883427607)) ;
#183158=CARTESIAN_POINT('Ctrl Pts',(-19.3346750163065,-13.4844393542531,
116.640102123225)) ;
#183159=CARTESIAN_POINT('Ctrl Pts',(-19.311049259971,-13.4793790766449,
116.56814188037)) ;
#183160=CARTESIAN_POINT('Ctrl Pts',(-19.2372454173489,-13.4793790219259,
116.592372924486)) ;
#183161=CARTESIAN_POINT('Ctrl Pts',(-19.1634415747268,-13.479378967207,
116.616603968602)) ;
#183162=CARTESIAN_POINT('Ctrl Pts',(-19.1870673310623,-13.4844392448151,
116.688564211457)) ;
#183163=CARTESIAN_POINT('Ctrl Pts',(-19.2106930873978,-13.4894995224233,
116.760524454312)) ;
#183164=CARTESIAN_POINT('Ctrl Pts',(-19.2844969300199,-13.4894995771423,
116.736293410196)) ;
#183165=CARTESIAN_POINT('Ctrl Pts',(-19.358300772642,-13.4894996318613,
116.71206236608)) ;
#183166=CARTESIAN_POINT('Ctrl Pts',(-19.3346750163065,-13.4844393542531,
116.640102123225)) ;
#183167=CARTESIAN_POINT('Ctrl Pts',(-19.3174944725961,-13.1938467066394,
116.623262581033)) ;
#183168=CARTESIAN_POINT('Ctrl Pts',(-19.2942980324291,-13.2090684129076,
116.55260996613)) ;
#183169=CARTESIAN_POINT('Ctrl Pts',(-19.2204941858365,-13.2090683682137,
116.576840998153)) ;
#183170=CARTESIAN_POINT('Ctrl Pts',(-19.1466903392439,-13.2090683235198,
116.601072030175)) ;
#183171=CARTESIAN_POINT('Ctrl Pts',(-19.1698867794109,-13.1938466172516,
116.671724645078)) ;
#183172=CARTESIAN_POINT('Ctrl Pts',(-19.1930832195779,-13.1786249109835,
116.74237725998)) ;
#183173=CARTESIAN_POINT('Ctrl Pts',(-19.2668870661705,-13.1786249556774,
116.718146227958)) ;
#183174=CARTESIAN_POINT('Ctrl Pts',(-19.3406909127631,-13.1786250003713,
116.693915195935)) ;
#183175=CARTESIAN_POINT('Ctrl Pts',(-19.3174944725961,-13.1938467066394,
116.623262581033)) ;
#183176=CARTESIAN_POINT('Ctrl Pts',(-19.2765712704978,-12.9193998282655,
116.534084192877)) ;
#183177=CARTESIAN_POINT('Ctrl Pts',(-19.2554630438177,-12.9538071121124,
116.469791939493)) ;
#183178=CARTESIAN_POINT('Ctrl Pts',(-19.1816591948598,-12.9538070795867,
116.494022964311)) ;
#183179=CARTESIAN_POINT('Ctrl Pts',(-19.107855345902,-12.9538070470611,
116.51825398913)) ;
#183180=CARTESIAN_POINT('Ctrl Pts',(-19.1289635725821,-12.9193997632142,
116.582546242514)) ;
#183181=CARTESIAN_POINT('Ctrl Pts',(-19.1500717992623,-12.8849924793673,
116.646838495899)) ;
#183182=CARTESIAN_POINT('Ctrl Pts',(-19.2238756482201,-12.884992511893,
116.62260747108)) ;
#183183=CARTESIAN_POINT('Ctrl Pts',(-19.297679497178,-12.8849925444186,
116.598376446262)) ;
#183184=CARTESIAN_POINT('Ctrl Pts',(-19.2765712704978,-12.9193998282655,
116.534084192877)) ;
#183185=CARTESIAN_POINT('Ctrl Pts',(-19.2136556163805,-12.679977460876,
116.378071311553)) ;
#183186=CARTESIAN_POINT('Ctrl Pts',(-19.1961712122001,-12.7311545599109,
116.324816636992)) ;
#183187=CARTESIAN_POINT('Ctrl Pts',(-19.1223673628755,-12.7311545403401,
116.349047660693)) ;
#183188=CARTESIAN_POINT('Ctrl Pts',(-19.0485635135508,-12.7311545207693,
116.373278684394)) ;
#183189=CARTESIAN_POINT('Ctrl Pts',(-19.0660479177312,-12.6799774217345,
116.426533358955)) ;
#183190=CARTESIAN_POINT('Ctrl Pts',(-19.0835323219115,-12.6288003226997,
116.479788033517)) ;
#183191=CARTESIAN_POINT('Ctrl Pts',(-19.1573361712362,-12.6288003422704,
116.455557009816)) ;
#183192=CARTESIAN_POINT('Ctrl Pts',(-19.2311400205609,-12.6288003618412,
116.431325986115)) ;
#183193=CARTESIAN_POINT('Ctrl Pts',(-19.2136556163805,-12.679977460876,
116.378071311553)) ;
#183194=CARTESIAN_POINT('Ctrl Pts',(-19.1338523199838,-12.4956043021029,
116.170183536347)) ;
#183195=CARTESIAN_POINT('Ctrl Pts',(-19.1211857358534,-12.5597317655866,
116.13160316441)) ;
#183196=CARTESIAN_POINT('Ctrl Pts',(-19.0473818865867,-12.5597317545878,
116.155834188288)) ;
#183197=CARTESIAN_POINT('Ctrl Pts',(-18.9735780373201,-12.5597317435889,
116.180065212166)) ;
#183198=CARTESIAN_POINT('Ctrl Pts',(-18.9862446214504,-12.4956042801052,
116.218645584102)) ;
#183199=CARTESIAN_POINT('Ctrl Pts',(-18.9989112055808,-12.4314768166214,
116.257225956039)) ;
#183200=CARTESIAN_POINT('Ctrl Pts',(-19.0727150548475,-12.4314768276203,
116.232994932161)) ;
#183201=CARTESIAN_POINT('Ctrl Pts',(-19.1465189041141,-12.4314768386191,
116.208763908283)) ;
#183202=CARTESIAN_POINT('Ctrl Pts',(-19.1338523199838,-12.4956043021029,
116.170183536347)) ;
#183203=CARTESIAN_POINT('Ctrl Pts',(-19.0401108727425,-12.3751190535725,
115.920306886088)) ;
#183204=CARTESIAN_POINT('Ctrl Pts',(-19.0332329599517,-12.4477568900421,
115.899357873225)) ;
#183205=CARTESIAN_POINT('Ctrl Pts',(-18.9594291126121,-12.4477568870231,
115.923588902972)) ;
#183206=CARTESIAN_POINT('Ctrl Pts',(-18.8856252652726,-12.4477568840041,
115.94781993272)) ;
#183207=CARTESIAN_POINT('Ctrl Pts',(-18.8925031780634,-12.3751190475345,
115.968768945583)) ;
#183208=CARTESIAN_POINT('Ctrl Pts',(-18.8993810908542,-12.3024812110649,
115.989717958446)) ;
#183209=CARTESIAN_POINT('Ctrl Pts',(-18.9731849381938,-12.3024812140839,
115.965486928699)) ;
#183210=CARTESIAN_POINT('Ctrl Pts',(-19.0469887855334,-12.3024812171029,
115.941255898952)) ;
#183211=CARTESIAN_POINT('Ctrl Pts',(-19.0401108727425,-12.3751190535725,
115.920306886088)) ;
#183212=CARTESIAN_POINT('Ctrl Pts',(-18.9401330390511,-12.3303020351126,
115.651151126256)) ;
#183213=CARTESIAN_POINT('Ctrl Pts',(-18.9394940201831,-12.4061784488461,
115.649204777747)) ;
#183214=CARTESIAN_POINT('Ctrl Pts',(-18.8656901744884,-12.4061784491626,
115.673435812505)) ;
#183215=CARTESIAN_POINT('Ctrl Pts',(-18.7918863287937,-12.4061784494791,
115.697666847262)) ;
#183216=CARTESIAN_POINT('Ctrl Pts',(-18.7925253476617,-12.3303020357456,
115.699613195771)) ;
#183217=CARTESIAN_POINT('Ctrl Pts',(-18.7931643665296,-12.2544256220122,
115.701559544279)) ;
#183218=CARTESIAN_POINT('Ctrl Pts',(-18.8669682122243,-12.2544256216956,
115.677328509522)) ;
#183219=CARTESIAN_POINT('Ctrl Pts',(-18.940772057919,-12.2544256213791,
115.653097474764)) ;
#183220=CARTESIAN_POINT('Ctrl Pts',(-18.9401330390511,-12.3303020351126,
115.651151126256)) ;
#183221=CARTESIAN_POINT('Ctrl Pts',(-18.839178326217,-12.3631774170788,
115.379196252521)) ;
#183222=CARTESIAN_POINT('Ctrl Pts',(-18.8448523121877,-12.4368724586972,
115.396478298259)) ;
#183223=CARTESIAN_POINT('Ctrl Pts',(-18.7710484682646,-12.4368724595397,
115.420709338412)) ;
#183224=CARTESIAN_POINT('Ctrl Pts',(-18.6972446243415,-12.4368724603823,
115.444940378566)) ;
#183225=CARTESIAN_POINT('Ctrl Pts',(-18.6915706383708,-12.363177418764,
115.427658332828)) ;
#183226=CARTESIAN_POINT('Ctrl Pts',(-18.6858966524001,-12.2894823771457,
115.41037628709)) ;
#183227=CARTESIAN_POINT('Ctrl Pts',(-18.7597004963232,-12.2894823763031,
115.386145246937)) ;
#183228=CARTESIAN_POINT('Ctrl Pts',(-18.8335043402463,-12.2894823754605,
115.361914206783)) ;
#183229=CARTESIAN_POINT('Ctrl Pts',(-18.839178326217,-12.3631774170788,
115.379196252521)) ;
#183230=CARTESIAN_POINT('Ctrl Pts',(-18.7446035699514,-12.4713342743348,
115.126509818248)) ;
#183231=CARTESIAN_POINT('Ctrl Pts',(-18.756157869452,-12.5375870378766,
115.161702350275)) ;
#183232=CARTESIAN_POINT('Ctrl Pts',(-18.6823540264618,-12.5375870373685,
115.18593339327)) ;
#183233=CARTESIAN_POINT('Ctrl Pts',(-18.6085501834715,-12.5375870368604,
115.210164436265)) ;
#183234=CARTESIAN_POINT('Ctrl Pts',(-18.5969958839709,-12.4713342733185,
115.174971904238)) ;
#183235=CARTESIAN_POINT('Ctrl Pts',(-18.5854415844703,-12.4050815097766,
115.139779372211)) ;
#183236=CARTESIAN_POINT('Ctrl Pts',(-18.6592454274606,-12.4050815102848,
115.115548329217)) ;
#183237=CARTESIAN_POINT('Ctrl Pts',(-18.7330492704508,-12.4050815107929,
115.091317286222)) ;
#183238=CARTESIAN_POINT('Ctrl Pts',(-18.7446035699514,-12.4713342743348,
115.126509818248)) ;
#183239=CARTESIAN_POINT('Ctrl Pts',(-18.6616637495359,-12.6476404276989,
114.909396069518)) ;
#183240=CARTESIAN_POINT('Ctrl Pts',(-18.6782920578757,-12.7016806543081,
114.960043213818)) ;
#183241=CARTESIAN_POINT('Ctrl Pts',(-18.6044882152249,-12.7016806520052,
114.984274257847)) ;
#183242=CARTESIAN_POINT('Ctrl Pts',(-18.530684372574,-12.7016806497023,
115.008505301875)) ;
#183243=CARTESIAN_POINT('Ctrl Pts',(-18.5140560642342,-12.6476404230932,
114.957858157575)) ;
#183244=CARTESIAN_POINT('Ctrl Pts',(-18.4974277558943,-12.5936001964841,
114.907211013275)) ;
#183245=CARTESIAN_POINT('Ctrl Pts',(-18.5712315985452,-12.5936001987869,
114.882979969247)) ;
#183246=CARTESIAN_POINT('Ctrl Pts',(-18.6450354411961,-12.5936002010898,
114.858748925218)) ;
#183247=CARTESIAN_POINT('Ctrl Pts',(-18.6616637495359,-12.6476404276989,
114.909396069518)) ;
#183248=CARTESIAN_POINT('Ctrl Pts',(-18.5959843317389,-12.8790215196565,
114.744812606196)) ;
#183249=CARTESIAN_POINT('Ctrl Pts',(-18.6164896477251,-12.9169844114343,
114.807268490226)) ;
#183250=CARTESIAN_POINT('Ctrl Pts',(-18.542685804714,-12.916984408831,114.831499533157)) ;
#183251=CARTESIAN_POINT('Ctrl Pts',(-18.468881961703,-12.9169844062277,
114.855730576088)) ;
#183252=CARTESIAN_POINT('Ctrl Pts',(-18.4483766457167,-12.87902151445,114.793274692059)) ;
#183253=CARTESIAN_POINT('Ctrl Pts',(-18.4278713297304,-12.8410586226723,
114.730818808029)) ;
#183254=CARTESIAN_POINT('Ctrl Pts',(-18.5016751727415,-12.8410586252756,
114.706587765098)) ;
#183255=CARTESIAN_POINT('Ctrl Pts',(-18.5754790157526,-12.8410586278788,
114.682356722167)) ;
#183256=CARTESIAN_POINT('Ctrl Pts',(-18.5959843317389,-12.8790215196565,
114.744812606196)) ;
#183257=CARTESIAN_POINT('Ctrl Pts',(-18.5513499003185,-13.1499133657009,
114.644442101082)) ;
#183258=CARTESIAN_POINT('Ctrl Pts',(-18.574265896151,-13.1690162421117,
114.714240526902)) ;
#183259=CARTESIAN_POINT('Ctrl Pts',(-18.5004620526313,-13.1690162422106,
114.738471568284)) ;
#183260=CARTESIAN_POINT('Ctrl Pts',(-18.4266582091115,-13.1690162423095,
114.762702609666)) ;
#183261=CARTESIAN_POINT('Ctrl Pts',(-18.403742213279,-13.1499133658987,
114.692904183846)) ;
#183262=CARTESIAN_POINT('Ctrl Pts',(-18.3808262174465,-13.1308104894879,
114.623105758027)) ;
#183263=CARTESIAN_POINT('Ctrl Pts',(-18.4546300609663,-13.130810489389,
114.598874716645)) ;
#183264=CARTESIAN_POINT('Ctrl Pts',(-18.528433904486,-13.1308104892901,
114.574643675262)) ;
#183265=CARTESIAN_POINT('Ctrl Pts',(-18.5513499003185,-13.1499133657009,
114.644442101082)) ;
#183266=CARTESIAN_POINT('Ctrl Pts',(-18.5304611078023,-13.4386144880716,
114.616209853643)) ;
#183267=CARTESIAN_POINT('Ctrl Pts',(-18.5541367214207,-13.437586579743,
114.688321952596)) ;
#183268=CARTESIAN_POINT('Ctrl Pts',(-18.4803328778889,-13.4375865840391,
114.712552993941)) ;
#183269=CARTESIAN_POINT('Ctrl Pts',(-18.406529034357,-13.4375865883353,
114.736784035286)) ;
#183270=CARTESIAN_POINT('Ctrl Pts',(-18.3828534207386,-13.438614496664,
114.664671936333)) ;
#183271=CARTESIAN_POINT('Ctrl Pts',(-18.3591778071202,-13.4396424049927,
114.59255983738)) ;
#183272=CARTESIAN_POINT('Ctrl Pts',(-18.4329816506521,-13.4396424006965,
114.568328796035)) ;
#183273=CARTESIAN_POINT('Ctrl Pts',(-18.5067854941839,-13.4396423964003,
114.54409775469)) ;
#183274=CARTESIAN_POINT('Ctrl Pts',(-18.5304611078023,-13.4386144880716,
114.616209853643)) ;
#183275=CARTESIAN_POINT('Ctrl Pts',(-18.5338401235194,-13.7268235527867,
114.662025079469)) ;
#183276=CARTESIAN_POINT('Ctrl Pts',(-18.556579229651,-13.7056699529127,
114.731284727602)) ;
#183277=CARTESIAN_POINT('Ctrl Pts',(-18.4827753870096,-13.7056699630902,
114.75551577166)) ;
#183278=CARTESIAN_POINT('Ctrl Pts',(-18.4089715443681,-13.7056699732676,
114.779746815717)) ;
#183279=CARTESIAN_POINT('Ctrl Pts',(-18.3862324382365,-13.7268235731417,
114.710487167584)) ;
#183280=CARTESIAN_POINT('Ctrl Pts',(-18.3634933321048,-13.7479771730157,
114.64122751945)) ;
#183281=CARTESIAN_POINT('Ctrl Pts',(-18.4372971747463,-13.7479771628382,
114.616996475393)) ;
#183282=CARTESIAN_POINT('Ctrl Pts',(-18.5111010173877,-13.7479771526607,
114.592765431336)) ;
#183283=CARTESIAN_POINT('Ctrl Pts',(-18.5338401235194,-13.7268235527867,
114.662025079469)) ;
#183284=CARTESIAN_POINT('Ctrl Pts',(-18.5603928248668,-13.9914324144424,
114.778219545102)) ;
#183285=CARTESIAN_POINT('Ctrl Pts',(-18.5805799757975,-13.9517725540924,
114.839706349339)) ;
#183286=CARTESIAN_POINT('Ctrl Pts',(-18.5067761349001,-13.9517725681727,
114.863937398709)) ;
#183287=CARTESIAN_POINT('Ctrl Pts',(-18.4329722940027,-13.9517725822531,
114.888168448078)) ;
#183288=CARTESIAN_POINT('Ctrl Pts',(-18.4127851430721,-13.9914324426031,
114.826681643841)) ;
#183289=CARTESIAN_POINT('Ctrl Pts',(-18.3925979921414,-14.0310923029532,
114.765194839604)) ;
#183290=CARTESIAN_POINT('Ctrl Pts',(-18.4664018330387,-14.0310922888728,
114.740963790235)) ;
#183291=CARTESIAN_POINT('Ctrl Pts',(-18.5402056739361,-14.0310922747924,
114.716732740866)) ;
#183292=CARTESIAN_POINT('Ctrl Pts',(-18.5603928248668,-13.9914324144424,
114.778219545102)) ;
#183293=CARTESIAN_POINT('Ctrl Pts',(-18.6076829202727,-14.2164140691066,
114.957760632545)) ;
#183294=CARTESIAN_POINT('Ctrl Pts',(-18.6238627885757,-14.1609879110475,
115.007041900317)) ;
#183295=CARTESIAN_POINT('Ctrl Pts',(-18.5500589505241,-14.1609879280051,
115.031272958354)) ;
#183296=CARTESIAN_POINT('Ctrl Pts',(-18.4762551124724,-14.1609879449628,
115.055504016391)) ;
#183297=CARTESIAN_POINT('Ctrl Pts',(-18.4600752441693,-14.2164141030218,
115.006222748618)) ;
#183298=CARTESIAN_POINT('Ctrl Pts',(-18.4438953758662,-14.2718402610809,
114.956941480846)) ;
#183299=CARTESIAN_POINT('Ctrl Pts',(-18.5176992139179,-14.2718402441232,
114.932710422809)) ;
#183300=CARTESIAN_POINT('Ctrl Pts',(-18.5915030519696,-14.2718402271656,
114.908479364772)) ;
#183301=CARTESIAN_POINT('Ctrl Pts',(-18.6076829202727,-14.2164140691066,
114.957760632545)) ;
#183302=CARTESIAN_POINT('Ctrl Pts',(-18.6716131600408,-14.384032579335,
115.188003285153)) ;
#183303=CARTESIAN_POINT('Ctrl Pts',(-18.6826177315112,-14.3168227397863,
115.221521433634)) ;
#183304=CARTESIAN_POINT('Ctrl Pts',(-18.6088138971231,-14.3168227556033,
115.24575250283)) ;
#183305=CARTESIAN_POINT('Ctrl Pts',(-18.5350100627351,-14.3168227714204,
115.269983572026)) ;
#183306=CARTESIAN_POINT('Ctrl Pts',(-18.5240054912648,-14.3840326109691,
115.236465423545)) ;
#183307=CARTESIAN_POINT('Ctrl Pts',(-18.5130009197944,-14.4512424505178,
115.202947275064)) ;
#183308=CARTESIAN_POINT('Ctrl Pts',(-18.5868047541824,-14.4512424347008,
115.178716205868)) ;
#183309=CARTESIAN_POINT('Ctrl Pts',(-18.6606085885704,-14.4512424188837,
115.154485136673)) ;
#183310=CARTESIAN_POINT('Ctrl Pts',(-18.6716131600408,-14.384032579335,
115.188003285153)) ;
#183311=CARTESIAN_POINT('Ctrl Pts',(-18.7465062676533,-14.4820529544929,
115.451530561366)) ;
#183312=CARTESIAN_POINT('Ctrl Pts',(-18.751564849774,-14.40790231883,115.466938185513)) ;
#183313=CARTESIAN_POINT('Ctrl Pts',(-18.6777610188436,-14.4079023280758,
115.49116926524)) ;
#183314=CARTESIAN_POINT('Ctrl Pts',(-18.6039571879133,-14.4079023373216,
115.515400344967)) ;
#183315=CARTESIAN_POINT('Ctrl Pts',(-18.5988986057926,-14.4820529729845,
115.499992720821)) ;
#183316=CARTESIAN_POINT('Ctrl Pts',(-18.593840023672,-14.5562036086474,
115.484585096674)) ;
#183317=CARTESIAN_POINT('Ctrl Pts',(-18.6676438546023,-14.5562035994016,
115.460354016947)) ;
#183318=CARTESIAN_POINT('Ctrl Pts',(-18.7414476855327,-14.5562035901558,
115.43612293722)) ;
#183319=CARTESIAN_POINT('Ctrl Pts',(-18.7465062676533,-14.4820529544929,
115.451530561366)) ;
#183320=CARTESIAN_POINT('Ctrl Pts',(-18.8266090365466,-14.5042250600488,
115.730991693486)) ;
#183321=CARTESIAN_POINT('Ctrl Pts',(-18.8253480296144,-14.4284191898376,
115.727150868868)) ;
#183322=CARTESIAN_POINT('Ctrl Pts',(-18.7515442017851,-14.4284191877868,
115.751381958041)) ;
#183323=CARTESIAN_POINT('Ctrl Pts',(-18.6777403739558,-14.428419185736,
115.775613047213)) ;
#183324=CARTESIAN_POINT('Ctrl Pts',(-18.679001380888,-14.5042250559472,
115.779453871831)) ;
#183325=CARTESIAN_POINT('Ctrl Pts',(-18.6802623878202,-14.5800309261584,
115.78329469645)) ;
#183326=CARTESIAN_POINT('Ctrl Pts',(-18.7540662156495,-14.5800309282092,
115.759063607277)) ;
#183327=CARTESIAN_POINT('Ctrl Pts',(-18.8278700434788,-14.58003093026,115.734832518105)) ;
#183328=CARTESIAN_POINT('Ctrl Pts',(-18.8266090365466,-14.5042250600488,
115.730991693486)) ;
#183329=CARTESIAN_POINT('Ctrl Pts',(-18.9055245763069,-14.4479097103847,
116.006958567327)) ;
#183330=CARTESIAN_POINT('Ctrl Pts',(-18.8980152465996,-14.3759257111989,
115.984086359506)) ;
#183331=CARTESIAN_POINT('Ctrl Pts',(-18.8242114209466,-14.3759256925376,
116.008317455307)) ;
#183332=CARTESIAN_POINT('Ctrl Pts',(-18.7504075952935,-14.3759256738764,
116.032548551108)) ;
#183333=CARTESIAN_POINT('Ctrl Pts',(-18.7579169250007,-14.4479096730622,
116.055420758929)) ;
#183334=CARTESIAN_POINT('Ctrl Pts',(-18.7654262547079,-14.519893672248,
116.078292966749)) ;
#183335=CARTESIAN_POINT('Ctrl Pts',(-18.839230080361,-14.5198936909092,
116.054061870948)) ;
#183336=CARTESIAN_POINT('Ctrl Pts',(-18.9130339060141,-14.5198937095705,
116.029830775147)) ;
#183337=CARTESIAN_POINT('Ctrl Pts',(-18.9055245763069,-14.4479097103847,
116.006958567327)) ;
#183338=CARTESIAN_POINT('Ctrl Pts',(-18.9759850270256,-14.3189148106109,
116.25684843315)) ;
#183339=CARTESIAN_POINT('Ctrl Pts',(-18.9628155048468,-14.2558334084202,
116.216736192202)) ;
#183340=CARTESIAN_POINT('Ctrl Pts',(-18.889011678749,-14.2558333716659,
116.240967286648)) ;
#183341=CARTESIAN_POINT('Ctrl Pts',(-18.8152078526511,-14.2558333349115,
116.265198381095)) ;
#183342=CARTESIAN_POINT('Ctrl Pts',(-18.82837737483,-14.3189147371022,116.305310622043)) ;
#183343=CARTESIAN_POINT('Ctrl Pts',(-18.8415468970088,-14.3819961392929,
116.345422862991)) ;
#183344=CARTESIAN_POINT('Ctrl Pts',(-18.9153507231067,-14.3819961760472,
116.321191768545)) ;
#183345=CARTESIAN_POINT('Ctrl Pts',(-18.9891545492045,-14.3819962128016,
116.296960674098)) ;
#183346=CARTESIAN_POINT('Ctrl Pts',(-18.9759850270256,-14.3189148106109,
116.25684843315)) ;
#183347=CARTESIAN_POINT('Ctrl Pts',(-19.0333811299086,-14.1239822238445,
116.467278862587)) ;
#183348=CARTESIAN_POINT('Ctrl Pts',(-19.0154483528946,-14.0744187665949,
116.412658515781)) ;
#183349=CARTESIAN_POINT('Ctrl Pts',(-18.9416445249628,-14.074418709394,
116.436889604641)) ;
#183350=CARTESIAN_POINT('Ctrl Pts',(-18.8678406970309,-14.0744186521931,
116.461120693501)) ;
#183351=CARTESIAN_POINT('Ctrl Pts',(-18.8857734740448,-14.1239821094427,
116.515741040307)) ;
#183352=CARTESIAN_POINT('Ctrl Pts',(-18.9037062510588,-14.1735455666924,
116.570361387112)) ;
#183353=CARTESIAN_POINT('Ctrl Pts',(-18.9775100789907,-14.1735456238933,
116.546130298252)) ;
#183354=CARTESIAN_POINT('Ctrl Pts',(-19.0513139069226,-14.1735456810942,
116.521899209392)) ;
#183355=CARTESIAN_POINT('Ctrl Pts',(-19.0333811299086,-14.1239822238445,
116.467278862587)) ;
#183356=CARTESIAN_POINT('Ctrl Pts',(-19.0719097483262,-13.8804446676162,
116.619916310961)) ;
#183357=CARTESIAN_POINT('Ctrl Pts',(-19.0505310135905,-13.8478127953866,
116.554800132824)) ;
#183358=CARTESIAN_POINT('Ctrl Pts',(-18.9767271811777,-13.8478127217154,
116.579031208036)) ;
#183359=CARTESIAN_POINT('Ctrl Pts',(-18.902923348765,-13.8478126480443,
116.603262283248)) ;
#183360=CARTESIAN_POINT('Ctrl Pts',(-18.9243020835006,-13.8804445202739,
116.668378461384)) ;
#183361=CARTESIAN_POINT('Ctrl Pts',(-18.9456808182363,-13.9130763925035,
116.733494639521)) ;
#183362=CARTESIAN_POINT('Ctrl Pts',(-19.0194846506491,-13.9130764661746,
116.709263564309)) ;
#183363=CARTESIAN_POINT('Ctrl Pts',(-19.0932884830618,-13.9130765398458,
116.685032489097)) ;
#183364=CARTESIAN_POINT('Ctrl Pts',(-19.0719097483262,-13.8804446676162,
116.619916310961)) ;
#183365=CARTESIAN_POINT('Ctrl Pts',(-19.088702598421,-13.6007259227713,
116.70677615132)) ;
#183366=CARTESIAN_POINT('Ctrl Pts',(-19.0653812357714,-13.5875751539527,
116.635743041836)) ;
#183367=CARTESIAN_POINT('Ctrl Pts',(-18.9915773972596,-13.5875750652436,
116.659974098472)) ;
#183368=CARTESIAN_POINT('Ctrl Pts',(-18.9177735587479,-13.5875749765345,
116.684205155107)) ;
#183369=CARTESIAN_POINT('Ctrl Pts',(-18.9410949213975,-13.6007257453531,
116.755238264591)) ;
#183370=CARTESIAN_POINT('Ctrl Pts',(-18.9644162840471,-13.6138765141717,
116.826271374075)) ;
#183371=CARTESIAN_POINT('Ctrl Pts',(-19.0382201225589,-13.6138766028808,
116.80204031744)) ;
#183372=CARTESIAN_POINT('Ctrl Pts',(-19.1120239610706,-13.6138766915899,
116.777809260804)) ;
#183373=CARTESIAN_POINT('Ctrl Pts',(-19.088702598421,-13.6007259227713,
116.70677615132)) ;
#183374=CARTESIAN_POINT('Ctrl Pts',(-19.0813475062609,-13.310886389785,
116.719690814776)) ;
#183375=CARTESIAN_POINT('Ctrl Pts',(-19.0577750307551,-13.3179522424612,
116.647892855958)) ;
#183376=CARTESIAN_POINT('Ctrl Pts',(-18.9839711845376,-13.3179521481175,
116.672123889123)) ;
#183377=CARTESIAN_POINT('Ctrl Pts',(-18.9101673383201,-13.3179520537738,
116.696354922288)) ;
#183378=CARTESIAN_POINT('Ctrl Pts',(-18.933739813826,-13.3108862010977,
116.768152881106)) ;
#183379=CARTESIAN_POINT('Ctrl Pts',(-18.9573122893318,-13.3038203484215,
116.839950839923)) ;
#183380=CARTESIAN_POINT('Ctrl Pts',(-19.0311161355493,-13.3038204427652,
116.815719806758)) ;
#183381=CARTESIAN_POINT('Ctrl Pts',(-19.1049199817667,-13.3038205371088,
116.791488773593)) ;
#183382=CARTESIAN_POINT('Ctrl Pts',(-19.0813475062609,-13.310886389785,
116.719690814776)) ;
#183383=CARTESIAN_POINT('Ctrl Pts',(-19.0499358228212,-13.0275729196668,
116.659478806876)) ;
#183384=CARTESIAN_POINT('Ctrl Pts',(-19.0277881847409,-13.0544289037497,
116.592020672865)) ;
#183385=CARTESIAN_POINT('Ctrl Pts',(-18.9539843302875,-13.0544288105617,
116.616251680945)) ;
#183386=CARTESIAN_POINT('Ctrl Pts',(-18.8801804758341,-13.0544287173738,
116.640482689024)) ;
#183387=CARTESIAN_POINT('Ctrl Pts',(-18.9023281139144,-13.0275727332909,
116.707940823035)) ;
#183388=CARTESIAN_POINT('Ctrl Pts',(-18.9244757519947,-13.000716749208,
116.775398957047)) ;
#183389=CARTESIAN_POINT('Ctrl Pts',(-18.9982796064481,-13.000716842396,
116.751167948967)) ;
#183390=CARTESIAN_POINT('Ctrl Pts',(-19.0720834609015,-13.000716935584,
116.726936940887)) ;
#183391=CARTESIAN_POINT('Ctrl Pts',(-19.0499358228212,-13.0275729196668,
116.659478806876)) ;
#183392=CARTESIAN_POINT('Ctrl Pts',(-18.9956010454947,-12.7715214711428,
116.529545008738)) ;
#183393=CARTESIAN_POINT('Ctrl Pts',(-18.9764784771327,-12.8162933310401,
116.471300748914)) ;
#183394=CARTESIAN_POINT('Ctrl Pts',(-18.9026746145278,-12.8162932472945,
116.495531732165)) ;
#183395=CARTESIAN_POINT('Ctrl Pts',(-18.8288707519228,-12.8162931635489,
116.519762715417)) ;
#183396=CARTESIAN_POINT('Ctrl Pts',(-18.8479933202848,-12.7715213036516,
116.578006975241)) ;
#183397=CARTESIAN_POINT('Ctrl Pts',(-18.8671158886468,-12.7267494437543,
116.636251235064)) ;
#183398=CARTESIAN_POINT('Ctrl Pts',(-18.9409197512517,-12.7267495274999,
116.612020251813)) ;
#183399=CARTESIAN_POINT('Ctrl Pts',(-19.0147236138567,-12.7267496112455,
116.587789268561)) ;
#183400=CARTESIAN_POINT('Ctrl Pts',(-18.9956010454947,-12.7715214711428,
116.529545008738)) ;
#183401=CARTESIAN_POINT('Ctrl Pts',(-18.9217241255641,-12.5625540682405,
116.340023816642)) ;
#183402=CARTESIAN_POINT('Ctrl Pts',(-18.9069967558379,-12.6219811291845,
116.295166622649)) ;
#183403=CARTESIAN_POINT('Ctrl Pts',(-18.8331928863221,-12.6219810632867,
116.319397584851)) ;
#183404=CARTESIAN_POINT('Ctrl Pts',(-18.7593890168062,-12.6219809973889,
116.343628547053)) ;
#183405=CARTESIAN_POINT('Ctrl Pts',(-18.7741163865324,-12.5625539364449,
116.388485741045)) ;
#183406=CARTESIAN_POINT('Ctrl Pts',(-18.7888437562586,-12.5031268755009,
116.433342935038)) ;
#183407=CARTESIAN_POINT('Ctrl Pts',(-18.8626476257744,-12.5031269413987,
116.409111972836)) ;
#183408=CARTESIAN_POINT('Ctrl Pts',(-18.9364514952903,-12.5031270072965,
116.384881010634)) ;
#183409=CARTESIAN_POINT('Ctrl Pts',(-18.9217241255641,-12.5625540682405,
116.340023816642)) ;
#183410=CARTESIAN_POINT('Ctrl Pts',(-18.8334781141802,-12.4155360311479,
116.106499613622)) ;
#183411=CARTESIAN_POINT('Ctrl Pts',(-18.824160647094,-12.4853145096468,
116.078120110162)) ;
#183412=CARTESIAN_POINT('Ctrl Pts',(-18.7503567727018,-12.4853144677288,
116.102351057511)) ;
#183413=CARTESIAN_POINT('Ctrl Pts',(-18.6765528983095,-12.4853144258108,
116.12658200486)) ;
#183414=CARTESIAN_POINT('Ctrl Pts',(-18.6858703653957,-12.4155359473118,
116.154961508321)) ;
#183415=CARTESIAN_POINT('Ctrl Pts',(-18.6951878324819,-12.3457574688128,
116.183341011781)) ;
#183416=CARTESIAN_POINT('Ctrl Pts',(-18.7689917068741,-12.3457575107309,
116.159110064432)) ;
#183417=CARTESIAN_POINT('Ctrl Pts',(-18.8427955812663,-12.3457575526489,
116.134879117083)) ;
#183418=CARTESIAN_POINT('Ctrl Pts',(-18.8334781141802,-12.4155360311479,
116.106499613622)) ;
#183419=CARTESIAN_POINT('Ctrl Pts',(-18.7350882955953,-12.339199302571,
115.842366036142)) ;
#183420=CARTESIAN_POINT('Ctrl Pts',(-18.7318906960185,-12.4144106897109,
115.832626661666)) ;
#183421=CARTESIAN_POINT('Ctrl Pts',(-18.6580868190615,-12.41441067568,115.856857601203)) ;
#183422=CARTESIAN_POINT('Ctrl Pts',(-18.5842829421045,-12.4144106616491,
115.881088540741)) ;
#183423=CARTESIAN_POINT('Ctrl Pts',(-18.5874805416813,-12.3391992745091,
115.890827915217)) ;
#183424=CARTESIAN_POINT('Ctrl Pts',(-18.5906781412581,-12.2639878873692,
115.900567289693)) ;
#183425=CARTESIAN_POINT('Ctrl Pts',(-18.6644820182151,-12.2639879014001,
115.876336350156)) ;
#183426=CARTESIAN_POINT('Ctrl Pts',(-18.7382858951721,-12.2639879154311,
115.852105410619)) ;
#183427=CARTESIAN_POINT('Ctrl Pts',(-18.7350882955953,-12.339199302571,
115.842366036142)) ;
#183428=CARTESIAN_POINT('Ctrl Pts',(-18.6339421925997,-12.3403409953756,
115.569683136395)) ;
#183429=CARTESIAN_POINT('Ctrl Pts',(-18.6370692220127,-12.4155840268561,
115.579207561357)) ;
#183430=CARTESIAN_POINT('Ctrl Pts',(-18.5632653452636,-12.4155840418634,
115.603438501527)) ;
#183431=CARTESIAN_POINT('Ctrl Pts',(-18.4894614685145,-12.4155840568707,
115.627669441698)) ;
#183432=CARTESIAN_POINT('Ctrl Pts',(-18.4863344391015,-12.3403410253901,
115.618145016736)) ;
#183433=CARTESIAN_POINT('Ctrl Pts',(-18.4832074096885,-12.2650979939095,
115.608620591774)) ;
#183434=CARTESIAN_POINT('Ctrl Pts',(-18.5570112864376,-12.2650979789023,
115.584389651604)) ;
#183435=CARTESIAN_POINT('Ctrl Pts',(-18.6308151631867,-12.265097963895,
115.560158711433)) ;
#183436=CARTESIAN_POINT('Ctrl Pts',(-18.6339421925997,-12.3403409953756,
115.569683136395)) ;
#183437=CARTESIAN_POINT('Ctrl Pts',(-18.5356154875398,-12.4190382667156,
115.305787998287)) ;
#183438=CARTESIAN_POINT('Ctrl Pts',(-18.5448755304968,-12.488899337021,
115.333992592985)) ;
#183439=CARTESIAN_POINT('Ctrl Pts',(-18.4710716567852,-12.488899379198,
115.358223542407)) ;
#183440=CARTESIAN_POINT('Ctrl Pts',(-18.3972677830735,-12.488899421375,
115.382454491829)) ;
#183441=CARTESIAN_POINT('Ctrl Pts',(-18.3880077401164,-12.4190383510696,
115.354249897131)) ;
#183442=CARTESIAN_POINT('Ctrl Pts',(-18.3787476971593,-12.3491772807642,
115.326045302433)) ;
#183443=CARTESIAN_POINT('Ctrl Pts',(-18.452551570871,-12.3491772385872,
115.301814353011)) ;
#183444=CARTESIAN_POINT('Ctrl Pts',(-18.5263554445827,-12.3491771964102,
115.277583403589)) ;
#183445=CARTESIAN_POINT('Ctrl Pts',(-18.5356154875398,-12.4190382667156,
115.305787998287)) ;
#183446=CARTESIAN_POINT('Ctrl Pts',(-18.4475845571782,-12.5685297170459,
115.072992627023)) ;
#183447=CARTESIAN_POINT('Ctrl Pts',(-18.4622733767878,-12.6280576016783,
115.117732399523)) ;
#183448=CARTESIAN_POINT('Ctrl Pts',(-18.3884695082534,-12.6280576665216,
115.141963364715)) ;
#183449=CARTESIAN_POINT('Ctrl Pts',(-18.314665639719,-12.6280577313649,
115.166194329906)) ;
#183450=CARTESIAN_POINT('Ctrl Pts',(-18.2999768201094,-12.5685298467324,
115.121454557406)) ;
#183451=CARTESIAN_POINT('Ctrl Pts',(-18.2852880004998,-12.5090019621,115.076714784906)) ;
#183452=CARTESIAN_POINT('Ctrl Pts',(-18.3590918690342,-12.5090018972567,
115.052483819715)) ;
#183453=CARTESIAN_POINT('Ctrl Pts',(-18.4328957375686,-12.5090018324134,
115.028252854523)) ;
#183454=CARTESIAN_POINT('Ctrl Pts',(-18.4475845571782,-12.5685297170459,
115.072992627023)) ;
#183455=CARTESIAN_POINT('Ctrl Pts',(-18.3743096061269,-12.7793086778933,
114.885300417553)) ;
#183456=CARTESIAN_POINT('Ctrl Pts',(-18.3934018856474,-12.8242097756673,
114.943452418522)) ;
#183457=CARTESIAN_POINT('Ctrl Pts',(-18.3195980241341,-12.8242098564781,
114.967683405098)) ;
#183458=CARTESIAN_POINT('Ctrl Pts',(-18.2457941626207,-12.8242099372889,
114.991914391674)) ;
#183459=CARTESIAN_POINT('Ctrl Pts',(-18.2267018831002,-12.7793088395149,
114.933762390705)) ;
#183460=CARTESIAN_POINT('Ctrl Pts',(-18.2076096035796,-12.7344077417409,
114.875610389736)) ;
#183461=CARTESIAN_POINT('Ctrl Pts',(-18.281413465093,-12.7344076609301,
114.85137940316)) ;
#183462=CARTESIAN_POINT('Ctrl Pts',(-18.3552173266063,-12.7344075801193,
114.827148416584)) ;
#183463=CARTESIAN_POINT('Ctrl Pts',(-18.3743096061269,-12.7793086778933,
114.885300417553)) ;
#183464=CARTESIAN_POINT('Ctrl Pts',(-18.3207591758651,-13.0361487300971,
114.757699953502)) ;
#183465=CARTESIAN_POINT('Ctrl Pts',(-18.3428842461716,-13.0631853690337,
114.825089345966)) ;
#183466=CARTESIAN_POINT('Ctrl Pts',(-18.2690803925913,-13.0631854575266,
114.849320356705)) ;
#183467=CARTESIAN_POINT('Ctrl Pts',(-18.195276539011,-13.0631855460195,
114.873551367444)) ;
#183468=CARTESIAN_POINT('Ctrl Pts',(-18.1731514687044,-13.0361489070829,
114.80616197498)) ;
#183469=CARTESIAN_POINT('Ctrl Pts',(-18.1510263983979,-13.0091122681464,
114.738772582515)) ;
#183470=CARTESIAN_POINT('Ctrl Pts',(-18.2248302519782,-13.0091121796535,
114.714541571777)) ;
#183471=CARTESIAN_POINT('Ctrl Pts',(-18.2986341055586,-13.0091120911606,
114.690310561038)) ;
#183472=CARTESIAN_POINT('Ctrl Pts',(-18.3207591758651,-13.0361487300971,
114.757699953502)) ;
#183473=CARTESIAN_POINT('Ctrl Pts',(-18.2900556295031,-13.3199156358865,
114.699632332883)) ;
#183474=CARTESIAN_POINT('Ctrl Pts',(-18.3136241193877,-13.3271808481679,
114.771418148599)) ;
#183475=CARTESIAN_POINT('Ctrl Pts',(-18.2398202736646,-13.3271809363831,
114.79564918327)) ;
#183476=CARTESIAN_POINT('Ctrl Pts',(-18.1660164279415,-13.3271810245983,
114.819880217941)) ;
#183477=CARTESIAN_POINT('Ctrl Pts',(-18.1424479380569,-13.3199158123169,
114.748094402225)) ;
#183478=CARTESIAN_POINT('Ctrl Pts',(-18.1188794481722,-13.3126506000355,
114.676308586509)) ;
#183479=CARTESIAN_POINT('Ctrl Pts',(-18.1926832938953,-13.3126505118203,
114.652077551838)) ;
#183480=CARTESIAN_POINT('Ctrl Pts',(-18.2664871396184,-13.312650423605,
114.627846517168)) ;
#183481=CARTESIAN_POINT('Ctrl Pts',(-18.2900556295031,-13.3199156358865,
114.699632332883)) ;
#183482=CARTESIAN_POINT('Ctrl Pts',(-18.2835244771423,-13.61053350134,114.715169773089)) ;
#183483=CARTESIAN_POINT('Ctrl Pts',(-18.3068513562178,-13.5975190949255,
114.786219681388)) ;
#183484=CARTESIAN_POINT('Ctrl Pts',(-18.2330475175386,-13.5975191756466,
114.810450737514)) ;
#183485=CARTESIAN_POINT('Ctrl Pts',(-18.1592436788595,-13.5975192563676,
114.834681793639)) ;
#183486=CARTESIAN_POINT('Ctrl Pts',(-18.1359167997839,-13.6105336627821,
114.76363188534)) ;
#183487=CARTESIAN_POINT('Ctrl Pts',(-18.1125899207084,-13.6235480691965,
114.692581977042)) ;
#183488=CARTESIAN_POINT('Ctrl Pts',(-18.1863937593876,-13.6235479884755,
114.668350920916)) ;
#183489=CARTESIAN_POINT('Ctrl Pts',(-18.2601975980667,-13.6235479077544,
114.644119864791)) ;
#183490=CARTESIAN_POINT('Ctrl Pts',(-18.2835244771423,-13.61053350134,114.715169773089)) ;
#183491=CARTESIAN_POINT('Ctrl Pts',(-18.300904682681,-13.8877845324202,
114.80358738621)) ;
#183492=CARTESIAN_POINT('Ctrl Pts',(-18.3223191972819,-13.8553930149523,
114.868812541022)) ;
#183493=CARTESIAN_POINT('Ctrl Pts',(-18.2485153641365,-13.8553930819553,
114.893043614003)) ;
#183494=CARTESIAN_POINT('Ctrl Pts',(-18.1747115309911,-13.8553931489583,
114.917274686983)) ;
#183495=CARTESIAN_POINT('Ctrl Pts',(-18.1532970163902,-13.8877846664262,
114.85204953217)) ;
#183496=CARTESIAN_POINT('Ctrl Pts',(-18.1318825017893,-13.9201761838941,
114.786824377358)) ;
#183497=CARTESIAN_POINT('Ctrl Pts',(-18.2056863349347,-13.9201761168911,
114.762593304377)) ;
#183498=CARTESIAN_POINT('Ctrl Pts',(-18.2794901680801,-13.9201760498881,
114.738362231397)) ;
#183499=CARTESIAN_POINT('Ctrl Pts',(-18.300904682681,-13.8877845324202,
114.80358738621)) ;
#183500=CARTESIAN_POINT('Ctrl Pts',(-18.3402955625269,-14.1315208949384,
114.95907694666)) ;
#183501=CARTESIAN_POINT('Ctrl Pts',(-18.3582574587125,-14.0820626171462,
115.01378598302)) ;
#183502=CARTESIAN_POINT('Ctrl Pts',(-18.2844536290332,-14.0820626666498,
115.038017066558)) ;
#183503=CARTESIAN_POINT('Ctrl Pts',(-18.210649799354,-14.0820627161535,
115.062248150096)) ;
#183504=CARTESIAN_POINT('Ctrl Pts',(-18.1926879031684,-14.1315209939457,
115.007539113736)) ;
#183505=CARTESIAN_POINT('Ctrl Pts',(-18.1747260069828,-14.1809792717379,
114.952830077376)) ;
#183506=CARTESIAN_POINT('Ctrl Pts',(-18.2485298366621,-14.1809792222342,
114.928598993838)) ;
#183507=CARTESIAN_POINT('Ctrl Pts',(-18.3223336663413,-14.1809791727306,
114.9043679103)) ;
#183508=CARTESIAN_POINT('Ctrl Pts',(-18.3402955625269,-14.1315208949384,
114.95907694666)) ;
#183509=CARTESIAN_POINT('Ctrl Pts',(-18.3979499293583,-14.3236676354294,
115.170121270634)) ;
#183510=CARTESIAN_POINT('Ctrl Pts',(-18.4111802519547,-14.2607186290668,
115.210418697435)) ;
#183511=CARTESIAN_POINT('Ctrl Pts',(-18.3373764237579,-14.260718660624,
115.234649785488)) ;
#183512=CARTESIAN_POINT('Ctrl Pts',(-18.2635725955611,-14.2607186921811,
115.258880873542)) ;
#183513=CARTESIAN_POINT('Ctrl Pts',(-18.2503422729647,-14.3236676985437,
115.21858344674)) ;
#183514=CARTESIAN_POINT('Ctrl Pts',(-18.2371119503683,-14.3866167049062,
115.178286019939)) ;
#183515=CARTESIAN_POINT('Ctrl Pts',(-18.3109157785651,-14.3866166733491,
115.154054931886)) ;
#183516=CARTESIAN_POINT('Ctrl Pts',(-18.3847196067618,-14.3866166417919,
115.129823843832)) ;
#183517=CARTESIAN_POINT('Ctrl Pts',(-18.3979499293583,-14.3236676354294,
115.170121270634)) ;
#183518=CARTESIAN_POINT('Ctrl Pts',(-18.4691141873596,-14.451213086268,
115.422348614941)) ;
#183519=CARTESIAN_POINT('Ctrl Pts',(-18.4766617833605,-14.3792631912131,
115.445337373605)) ;
#183520=CARTESIAN_POINT('Ctrl Pts',(-18.402857954655,-14.3792632058746,
115.469568460109)) ;
#183521=CARTESIAN_POINT('Ctrl Pts',(-18.3290541259495,-14.3792632205361,
115.493799546613)) ;
#183522=CARTESIAN_POINT('Ctrl Pts',(-18.3215065299486,-14.451213115591,
115.470810787948)) ;
#183523=CARTESIAN_POINT('Ctrl Pts',(-18.3139589339478,-14.5231630106458,
115.447822029284)) ;
#183524=CARTESIAN_POINT('Ctrl Pts',(-18.3877627626533,-14.5231629959843,
115.42359094278)) ;
#183525=CARTESIAN_POINT('Ctrl Pts',(-18.4615665913588,-14.5231629813228,
115.399359856276)) ;
#183526=CARTESIAN_POINT('Ctrl Pts',(-18.4691141873596,-14.451213086268,
115.422348614941)) ;
#183527=CARTESIAN_POINT('Ctrl Pts',(-18.5480547946809,-14.5046478984509,
115.698323016836)) ;
#183528=CARTESIAN_POINT('Ctrl Pts',(-18.5493667384091,-14.4288576762163,
115.702318984979)) ;
#183529=CARTESIAN_POINT('Ctrl Pts',(-18.4755629074551,-14.4288576774106,
115.726550064634)) ;
#183530=CARTESIAN_POINT('Ctrl Pts',(-18.4017590765011,-14.4288576786049,
115.750781144289)) ;
#183531=CARTESIAN_POINT('Ctrl Pts',(-18.4004471327729,-14.5046479008395,
115.746785176146)) ;
#183532=CARTESIAN_POINT('Ctrl Pts',(-18.3991351890446,-14.5804381230741,
115.742789208003)) ;
#183533=CARTESIAN_POINT('Ctrl Pts',(-18.4729390199986,-14.5804381218798,
115.718558128348)) ;
#183534=CARTESIAN_POINT('Ctrl Pts',(-18.5467428509526,-14.5804381206855,
115.694327048693)) ;
#183535=CARTESIAN_POINT('Ctrl Pts',(-18.5480547946809,-14.5046478984509,
115.698323016836)) ;
#183536=CARTESIAN_POINT('Ctrl Pts',(-18.6278722273307,-14.4801334339684,
115.976822091214)) ;
#183537=CARTESIAN_POINT('Ctrl Pts',(-18.6228807745293,-14.4059401882447,
115.961618930727)) ;
#183538=CARTESIAN_POINT('Ctrl Pts',(-18.5490769408651,-14.405940180657,
115.985850002128)) ;
#183539=CARTESIAN_POINT('Ctrl Pts',(-18.475273107201,-14.4059401730692,
116.010081073528)) ;
#183540=CARTESIAN_POINT('Ctrl Pts',(-18.4802645600025,-14.4801334187929,
116.025284234015)) ;
#183541=CARTESIAN_POINT('Ctrl Pts',(-18.4852560128039,-14.5543266645165,
116.040487394502)) ;
#183542=CARTESIAN_POINT('Ctrl Pts',(-18.5590598464681,-14.5543266721042,
116.016256323101)) ;
#183543=CARTESIAN_POINT('Ctrl Pts',(-18.6328636801322,-14.554326679692,
115.9920252517)) ;
#183544=CARTESIAN_POINT('Ctrl Pts',(-18.6278722273307,-14.4801334339684,
115.976822091214)) ;
#183545=CARTESIAN_POINT('Ctrl Pts',(-18.7025035045635,-14.3800974324411,
116.239533090197)) ;
#183546=CARTESIAN_POINT('Ctrl Pts',(-18.6915610435405,-14.3127767665056,
116.206204119007)) ;
#183547=CARTESIAN_POINT('Ctrl Pts',(-18.6177572067622,-14.3127767543614,
116.230435180923)) ;
#183548=CARTESIAN_POINT('Ctrl Pts',(-18.5439533699839,-14.3127767422172,
116.254666242838)) ;
#183549=CARTESIAN_POINT('Ctrl Pts',(-18.5548958310069,-14.3800974081526,
116.287995214028)) ;
#183550=CARTESIAN_POINT('Ctrl Pts',(-18.56583829203,-14.4474180740881,116.321324185218)) ;
#183551=CARTESIAN_POINT('Ctrl Pts',(-18.6396421288082,-14.4474180862324,
116.297093123302)) ;
#183552=CARTESIAN_POINT('Ctrl Pts',(-18.7134459655865,-14.4474180983766,
116.272862061387)) ;
#183553=CARTESIAN_POINT('Ctrl Pts',(-18.7025035045635,-14.3800974324411,
116.239533090197)) ;
#183554=CARTESIAN_POINT('Ctrl Pts',(-18.7661852178501,-14.2097836883392,
116.469145099282)) ;
#183555=CARTESIAN_POINT('Ctrl Pts',(-18.7500418045665,-14.1542529210645,
116.419974866854)) ;
#183556=CARTESIAN_POINT('Ctrl Pts',(-18.6762379644893,-14.1542529100711,
116.444205918722)) ;
#183557=CARTESIAN_POINT('Ctrl Pts',(-18.6024341244121,-14.1542528990776,
116.468436970589)) ;
#183558=CARTESIAN_POINT('Ctrl Pts',(-18.6185775376956,-14.2097836663522,
116.517607203017)) ;
#183559=CARTESIAN_POINT('Ctrl Pts',(-18.6347209509792,-14.2653144336269,
116.566777435444)) ;
#183560=CARTESIAN_POINT('Ctrl Pts',(-18.7085247910564,-14.2653144446203,
116.542546383577)) ;
#183561=CARTESIAN_POINT('Ctrl Pts',(-18.7823286311337,-14.2653144556138,
116.518315331709)) ;
#183562=CARTESIAN_POINT('Ctrl Pts',(-18.7661852178501,-14.2097836883392,
116.469145099282)) ;
#183563=CARTESIAN_POINT('Ctrl Pts',(-18.8126736298305,-13.9844447661634,
116.646062755378)) ;
#183564=CARTESIAN_POINT('Ctrl Pts',(-18.7925289620469,-13.944564790948,
116.584705347452)) ;
#183565=CARTESIAN_POINT('Ctrl Pts',(-18.7187251200822,-13.9445647824093,
116.60893639357)) ;
#183566=CARTESIAN_POINT('Ctrl Pts',(-18.6449212781175,-13.9445647738706,
116.633167439689)) ;
#183567=CARTESIAN_POINT('Ctrl Pts',(-18.6650659459011,-13.984444749086,
116.694524847615)) ;
#183568=CARTESIAN_POINT('Ctrl Pts',(-18.6852106136848,-14.0243247243014,
116.755882255542)) ;
#183569=CARTESIAN_POINT('Ctrl Pts',(-18.7590144556495,-14.0243247328401,
116.731651209424)) ;
#183570=CARTESIAN_POINT('Ctrl Pts',(-18.8328182976142,-14.0243247413788,
116.707420163305)) ;
#183571=CARTESIAN_POINT('Ctrl Pts',(-18.8126736298305,-13.9844447661634,
116.646062755378)) ;
#183572=CARTESIAN_POINT('Ctrl Pts',(-18.8387106000838,-13.7175338810347,
116.760872830317)) ;
#183573=CARTESIAN_POINT('Ctrl Pts',(-18.815982735405,-13.6962312533339,
116.691647421561)) ;
#183574=CARTESIAN_POINT('Ctrl Pts',(-18.7421788921662,-13.6962312496336,
116.715878463799)) ;
#183575=CARTESIAN_POINT('Ctrl Pts',(-18.6683750489273,-13.6962312459334,
116.740109506036)) ;
#183576=CARTESIAN_POINT('Ctrl Pts',(-18.691102913606,-13.7175338736341,
116.809334914792)) ;
#183577=CARTESIAN_POINT('Ctrl Pts',(-18.7138307782847,-13.7388365013348,
116.878560323548)) ;
#183578=CARTESIAN_POINT('Ctrl Pts',(-18.7876346215236,-13.7388365050351,
116.85432928131)) ;
#183579=CARTESIAN_POINT('Ctrl Pts',(-18.8614384647625,-13.7388365087354,
116.830098239072)) ;
#183580=CARTESIAN_POINT('Ctrl Pts',(-18.8387106000838,-13.7175338810347,
116.760872830317)) ;
#183581=CARTESIAN_POINT('Ctrl Pts',(-18.8412499966495,-13.4290941380284,
116.804105500737)) ;
#183582=CARTESIAN_POINT('Ctrl Pts',(-18.8175760945561,-13.42790072271,116.731998614741)) ;
#183583=CARTESIAN_POINT('Ctrl Pts',(-18.7437722510543,-13.4279007232461,
116.756229656177)) ;
#183584=CARTESIAN_POINT('Ctrl Pts',(-18.6699684075526,-13.4279007237822,
116.780460697614)) ;
#183585=CARTESIAN_POINT('Ctrl Pts',(-18.693642309646,-13.4290941391006,
116.852567583611)) ;
#183586=CARTESIAN_POINT('Ctrl Pts',(-18.7173162117394,-13.430287554419,
116.924674469607)) ;
#183587=CARTESIAN_POINT('Ctrl Pts',(-18.7911200552412,-13.4302875538829,
116.90044342817)) ;
#183588=CARTESIAN_POINT('Ctrl Pts',(-18.864923898743,-13.4302875533468,
116.876212386733)) ;
#183589=CARTESIAN_POINT('Ctrl Pts',(-18.8412499966495,-13.4290941380284,
116.804105500737)) ;
#183590=CARTESIAN_POINT('Ctrl Pts',(-18.8195971871137,-13.1407025280343,
116.773545460015)) ;
#183591=CARTESIAN_POINT('Ctrl Pts',(-18.7966675811409,-13.1596450179659,
116.703705579957)) ;
#183592=CARTESIAN_POINT('Ctrl Pts',(-18.7228637379266,-13.1596450208018,
116.727936622269)) ;
#183593=CARTESIAN_POINT('Ctrl Pts',(-18.6490598947122,-13.1596450236377,
116.752167664581)) ;
#183594=CARTESIAN_POINT('Ctrl Pts',(-18.671989500685,-13.1407025337061,
116.82200754464)) ;
#183595=CARTESIAN_POINT('Ctrl Pts',(-18.6949191066578,-13.1217600437745,
116.891847424699)) ;
#183596=CARTESIAN_POINT('Ctrl Pts',(-18.7687229498721,-13.1217600409386,
116.867616382386)) ;
#183597=CARTESIAN_POINT('Ctrl Pts',(-18.8425267930865,-13.1217600381026,
116.843385340074)) ;
#183598=CARTESIAN_POINT('Ctrl Pts',(-18.8195971871137,-13.1407025280343,
116.773545460015)) ;
#183599=CARTESIAN_POINT('Ctrl Pts',(-18.7741929648226,-12.8707969653127,
116.670833856634)) ;
#183600=CARTESIAN_POINT('Ctrl Pts',(-18.7536634762867,-12.9086154474282,
116.608304347037)) ;
#183601=CARTESIAN_POINT('Ctrl Pts',(-18.6798596333953,-12.9086154501767,
116.632535390332)) ;
#183602=CARTESIAN_POINT('Ctrl Pts',(-18.6060557905039,-12.9086154529253,
116.656766433628)) ;
#183603=CARTESIAN_POINT('Ctrl Pts',(-18.6265852790397,-12.8707969708098,
116.719295943226)) ;
#183604=CARTESIAN_POINT('Ctrl Pts',(-18.6471147675756,-12.8329784886943,
116.781825452824)) ;
#183605=CARTESIAN_POINT('Ctrl Pts',(-18.720918610467,-12.8329784859458,
116.757594409528)) ;
#183606=CARTESIAN_POINT('Ctrl Pts',(-18.7947224533584,-12.8329784831972,
116.733363366232)) ;
#183607=CARTESIAN_POINT('Ctrl Pts',(-18.7741929648226,-12.8707969653127,
116.670833856634)) ;
#183608=CARTESIAN_POINT('Ctrl Pts',(-18.7081893525992,-12.6417711077458,
116.505122794438)) ;
#183609=CARTESIAN_POINT('Ctrl Pts',(-18.6915075220937,-12.6956372286185,
116.454312630352)) ;
#183610=CARTESIAN_POINT('Ctrl Pts',(-18.6177036790936,-12.6956372295276,
116.478543673317)) ;
#183611=CARTESIAN_POINT('Ctrl Pts',(-18.5438998360935,-12.6956372304368,
116.502774716282)) ;
#183612=CARTESIAN_POINT('Ctrl Pts',(-18.5605816665991,-12.6417711095641,
116.553584880368)) ;
#183613=CARTESIAN_POINT('Ctrl Pts',(-18.5772634971046,-12.5879049886915,
116.604395044454)) ;
#183614=CARTESIAN_POINT('Ctrl Pts',(-18.6510673401047,-12.5879049877823,
116.580164001489)) ;
#183615=CARTESIAN_POINT('Ctrl Pts',(-18.7248711831048,-12.5879049868731,
116.555932958525)) ;
#183616=CARTESIAN_POINT('Ctrl Pts',(-18.7081893525992,-12.6417711077458,
116.505122794438)) ;
#183617=CARTESIAN_POINT('Ctrl Pts',(-18.624745958435,-12.4670674817275,
116.286513958254)) ;
#183618=CARTESIAN_POINT('Ctrl Pts',(-18.6131306242191,-12.5332118470618,
116.251135524313)) ;
#183619=CARTESIAN_POINT('Ctrl Pts',(-18.5393267802208,-12.5332118456008,
116.275366564238)) ;
#183620=CARTESIAN_POINT('Ctrl Pts',(-18.4655229362226,-12.5332118441398,
116.299597604162)) ;
#183621=CARTESIAN_POINT('Ctrl Pts',(-18.4771382704385,-12.4670674788054,
116.334976038103)) ;
#183622=CARTESIAN_POINT('Ctrl Pts',(-18.4887536046544,-12.4009231134711,
116.370354472043)) ;
#183623=CARTESIAN_POINT('Ctrl Pts',(-18.5625574486526,-12.4009231149321,
116.346123432119)) ;
#183624=CARTESIAN_POINT('Ctrl Pts',(-18.6363612926509,-12.4009231163931,
116.321892392194)) ;
#183625=CARTESIAN_POINT('Ctrl Pts',(-18.624745958435,-12.4670674817275,
116.286513958254)) ;
#183626=CARTESIAN_POINT('Ctrl Pts',(-18.5299237726579,-12.3610581795072,
116.033065517688)) ;
#183627=CARTESIAN_POINT('Ctrl Pts',(-18.5241806065629,-12.434700867629,
116.015572760285)) ;
#183628=CARTESIAN_POINT('Ctrl Pts',(-18.4503767610872,-12.4347008654183,
116.039803795709)) ;
#183629=CARTESIAN_POINT('Ctrl Pts',(-18.3765729156115,-12.4347008632077,
116.064034831134)) ;
#183630=CARTESIAN_POINT('Ctrl Pts',(-18.3823160817065,-12.3610581750859,
116.081527588537)) ;
#183631=CARTESIAN_POINT('Ctrl Pts',(-18.3880592478014,-12.2874154869641,
116.09902034594)) ;
#183632=CARTESIAN_POINT('Ctrl Pts',(-18.4618630932771,-12.2874154891748,
116.074789310515)) ;
#183633=CARTESIAN_POINT('Ctrl Pts',(-18.5356669387528,-12.2874154913854,
116.050558275091)) ;
#183634=CARTESIAN_POINT('Ctrl Pts',(-18.5299237726579,-12.3610581795072,
116.033065517688)) ;
#183635=CARTESIAN_POINT('Ctrl Pts',(-18.4285423943449,-12.3304705905987,
115.759931665259)) ;
#183636=CARTESIAN_POINT('Ctrl Pts',(-18.4291318873858,-12.4063567534876,
115.761727165661)) ;
#183637=CARTESIAN_POINT('Ctrl Pts',(-18.3553280393615,-12.4063567532817,
115.785958193323)) ;
#183638=CARTESIAN_POINT('Ctrl Pts',(-18.2815241913372,-12.4063567530759,
115.810189220985)) ;
#183639=CARTESIAN_POINT('Ctrl Pts',(-18.2809346982963,-12.330470590187,
115.808393720582)) ;
#183640=CARTESIAN_POINT('Ctrl Pts',(-18.2803452052554,-12.2545844272981,
115.80659822018)) ;
#183641=CARTESIAN_POINT('Ctrl Pts',(-18.3541490532797,-12.254584427504,
115.782367192518)) ;
#183642=CARTESIAN_POINT('Ctrl Pts',(-18.427952901304,-12.2545844277098,
115.758136164857)) ;
#183643=CARTESIAN_POINT('Ctrl Pts',(-18.4285423943449,-12.3304705905987,
115.759931665259)) ;
#183644=CARTESIAN_POINT('Ctrl Pts',(-18.3286734717406,-12.3780041179342,
115.491117750201)) ;
#183645=CARTESIAN_POINT('Ctrl Pts',(-18.3355049446952,-12.4506811357788,
115.511925314151)) ;
#183646=CARTESIAN_POINT('Ctrl Pts',(-18.2617010948026,-12.4506811414498,
115.536156336123)) ;
#183647=CARTESIAN_POINT('Ctrl Pts',(-18.1878972449099,-12.4506811471207,
115.560387358094)) ;
#183648=CARTESIAN_POINT('Ctrl Pts',(-18.1810657719553,-12.3780041292761,
115.539579794144)) ;
#183649=CARTESIAN_POINT('Ctrl Pts',(-18.1742342990006,-12.3053271114316,
115.518772230194)) ;
#183650=CARTESIAN_POINT('Ctrl Pts',(-18.2480381488933,-12.3053271057606,
115.494541208223)) ;
#183651=CARTESIAN_POINT('Ctrl Pts',(-18.321841998786,-12.3053271000897,
115.470310186251)) ;
#183652=CARTESIAN_POINT('Ctrl Pts',(-18.3286734717406,-12.3780041179342,
115.491117750201)) ;
#183653=CARTESIAN_POINT('Ctrl Pts',(-18.2355472337233,-12.5002675543906,
115.242998586149)) ;
#183654=CARTESIAN_POINT('Ctrl Pts',(-18.2481556577856,-12.5645133223993,
115.281401810897)) ;
#183655=CARTESIAN_POINT('Ctrl Pts',(-18.1743518063322,-12.5645133380227,
115.305632828115)) ;
#183656=CARTESIAN_POINT('Ctrl Pts',(-18.1005479548788,-12.5645133536461,
115.329863845332)) ;
#183657=CARTESIAN_POINT('Ctrl Pts',(-18.0879395308165,-12.5002675856374,
115.291460620583)) ;
#183658=CARTESIAN_POINT('Ctrl Pts',(-18.0753311067543,-12.4360218176287,
115.253057395835)) ;
#183659=CARTESIAN_POINT('Ctrl Pts',(-18.1491349582077,-12.4360218020053,
115.228826378617)) ;
#183660=CARTESIAN_POINT('Ctrl Pts',(-18.2229388096611,-12.4360217863819,
115.2045953614)) ;
#183661=CARTESIAN_POINT('Ctrl Pts',(-18.2355472337233,-12.5002675543906,
115.242998586149)) ;
#183662=CARTESIAN_POINT('Ctrl Pts',(-18.1559065411703,-12.6872113223539,
115.03574587489)) ;
#183663=CARTESIAN_POINT('Ctrl Pts',(-18.1733627764867,-12.7384971666027,
115.08891475039)) ;
#183664=CARTESIAN_POINT('Ctrl Pts',(-18.099558925084,-12.7384971937162,
115.113145767762)) ;
#183665=CARTESIAN_POINT('Ctrl Pts',(-18.0257550736814,-12.7384972208297,
115.137376785134)) ;
#183666=CARTESIAN_POINT('Ctrl Pts',(-18.008298838365,-12.6872113765809,
115.084207909633)) ;
#183667=CARTESIAN_POINT('Ctrl Pts',(-17.9908426030485,-12.635925532332,
115.031039034133)) ;
#183668=CARTESIAN_POINT('Ctrl Pts',(-18.0646464544512,-12.6359255052185,
115.006808016761)) ;
#183669=CARTESIAN_POINT('Ctrl Pts',(-18.1384503058539,-12.635925478105,
114.98257699939)) ;
#183670=CARTESIAN_POINT('Ctrl Pts',(-18.1559065411703,-12.6872113223539,
115.03574587489)) ;
#183671=CARTESIAN_POINT('Ctrl Pts',(-18.0936528156396,-12.928470822573,
114.881781285062)) ;
#183672=CARTESIAN_POINT('Ctrl Pts',(-18.1147432667107,-12.9629864518457,
114.946019395169)) ;
#183673=CARTESIAN_POINT('Ctrl Pts',(-18.0409394163538,-12.9629864941427,
114.970250415726)) ;
#183674=CARTESIAN_POINT('Ctrl Pts',(-17.9671355659969,-12.9629865364398,
114.994481436283)) ;
#183675=CARTESIAN_POINT('Ctrl Pts',(-17.9460451149259,-12.9284709071671,
114.930243326176)) ;
#183676=CARTESIAN_POINT('Ctrl Pts',(-17.9249546638548,-12.8939552778944,
114.866005216069)) ;
#183677=CARTESIAN_POINT('Ctrl Pts',(-17.9987585142116,-12.8939552355973,
114.841774195512)) ;
#183678=CARTESIAN_POINT('Ctrl Pts',(-18.0725623645685,-12.8939551933003,
114.817543174955)) ;
#183679=CARTESIAN_POINT('Ctrl Pts',(-18.0936528156396,-12.928470822573,
114.881781285062)) ;
#183680=CARTESIAN_POINT('Ctrl Pts',(-18.053566961881,-13.2034657060163,
114.795110966265)) ;
#183681=CARTESIAN_POINT('Ctrl Pts',(-18.0767535884705,-13.2188313176784,
114.865733688623)) ;
#183682=CARTESIAN_POINT('Ctrl Pts',(-18.0029497413991,-13.2188313725587,
114.889964719188)) ;
#183683=CARTESIAN_POINT('Ctrl Pts',(-17.9291458943278,-13.218831427439,
114.914195749752)) ;
#183684=CARTESIAN_POINT('Ctrl Pts',(-17.9059592677383,-13.2034658157769,
114.843573027393)) ;
#183685=CARTESIAN_POINT('Ctrl Pts',(-17.8827726411489,-13.1881002041148,
114.772950305034)) ;
#183686=CARTESIAN_POINT('Ctrl Pts',(-17.9565764882202,-13.1881001492345,
114.74871927447)) ;
#183687=CARTESIAN_POINT('Ctrl Pts',(-18.0303803352916,-13.1881000943542,
114.724488243906)) ;
#183688=CARTESIAN_POINT('Ctrl Pts',(-18.053566961881,-13.2034657060163,
114.795110966265)) ;
#183689=CARTESIAN_POINT('Ctrl Pts',(-18.0372153758526,-13.4939400108665,
114.780761585915)) ;
#183690=CARTESIAN_POINT('Ctrl Pts',(-18.0608435214232,-13.4890474543543,
114.852729103689)) ;
#183691=CARTESIAN_POINT('Ctrl Pts',(-17.9870396792037,-13.4890475187126,
114.876960149031)) ;
#183692=CARTESIAN_POINT('Ctrl Pts',(-17.9132358369841,-13.4890475830709,
114.901191194373)) ;
#183693=CARTESIAN_POINT('Ctrl Pts',(-17.8896076914135,-13.4939401395831,
114.829223676599)) ;
#183694=CARTESIAN_POINT('Ctrl Pts',(-17.8659795458429,-13.4988326960953,
114.757256158824)) ;
#183695=CARTESIAN_POINT('Ctrl Pts',(-17.9397833880625,-13.498832631737,
114.733025113482)) ;
#183696=CARTESIAN_POINT('Ctrl Pts',(-18.0135872302821,-13.4988325673787,
114.70879406814)) ;
#183697=CARTESIAN_POINT('Ctrl Pts',(-18.0372153758526,-13.4939400108665,
114.780761585915)) ;
#183698=CARTESIAN_POINT('Ctrl Pts',(-18.045087176113,-13.7785749983251,
114.84013824791)) ;
#183699=CARTESIAN_POINT('Ctrl Pts',(-18.0674673661548,-13.7538028114636,
114.908304694356)) ;
#183700=CARTESIAN_POINT('Ctrl Pts',(-17.9936635300079,-13.7538028795782,
114.932535758194)) ;
#183701=CARTESIAN_POINT('Ctrl Pts',(-17.9198596938609,-13.7538029476928,
114.956766822033)) ;
#183702=CARTESIAN_POINT('Ctrl Pts',(-17.8974795038191,-13.7785751345543,
114.888600375587)) ;
#183703=CARTESIAN_POINT('Ctrl Pts',(-17.8750993137773,-13.8033473214157,
114.820433929141)) ;
#183704=CARTESIAN_POINT('Ctrl Pts',(-17.9489031499242,-13.8033472533012,
114.796202865303)) ;
#183705=CARTESIAN_POINT('Ctrl Pts',(-18.0227069860712,-13.8033471851866,
114.771971801464)) ;
#183706=CARTESIAN_POINT('Ctrl Pts',(-18.045087176113,-13.7785749983251,
114.84013824791)) ;
#183707=CARTESIAN_POINT('Ctrl Pts',(-18.0758126785522,-14.0376123935157,
114.969142216543)) ;
#183708=CARTESIAN_POINT('Ctrl Pts',(-18.0953472138535,-13.9947190826741,
115.028641257654)) ;
#183709=CARTESIAN_POINT('Ctrl Pts',(-18.0215433843608,-13.9947191481114,
115.05287234176)) ;
#183710=CARTESIAN_POINT('Ctrl Pts',(-17.947739554868,-13.9947192135486,
115.077103425866)) ;
#183711=CARTESIAN_POINT('Ctrl Pts',(-17.9282050195667,-14.0376125243903,
115.017604384755)) ;
#183712=CARTESIAN_POINT('Ctrl Pts',(-17.9086704842654,-14.0805058352319,
114.958105343643)) ;
#183713=CARTESIAN_POINT('Ctrl Pts',(-17.9824743137582,-14.0805057697947,
114.933874259537)) ;
#183714=CARTESIAN_POINT('Ctrl Pts',(-18.0562781432509,-14.0805057043574,
114.909643175431)) ;
#183715=CARTESIAN_POINT('Ctrl Pts',(-18.0758126785522,-14.0376123935157,
114.969142216543)) ;
#183716=CARTESIAN_POINT('Ctrl Pts',(-18.126546298458,-14.2526152270872,
115.159131089373)) ;
#183717=CARTESIAN_POINT('Ctrl Pts',(-18.1418333641264,-14.1946488297789,
115.205693023175)) ;
#183718=CARTESIAN_POINT('Ctrl Pts',(-18.0680295412189,-14.1946488854693,
115.229924127339)) ;
#183719=CARTESIAN_POINT('Ctrl Pts',(-17.9942257183115,-14.1946489411597,
115.254155231503)) ;
#183720=CARTESIAN_POINT('Ctrl Pts',(-17.9789386526431,-14.252615338468,
115.207593297701)) ;
#183721=CARTESIAN_POINT('Ctrl Pts',(-17.9636515869747,-14.3105817357762,
115.161031363899)) ;
#183722=CARTESIAN_POINT('Ctrl Pts',(-18.0374554098822,-14.3105816800858,
115.136800259735)) ;
#183723=CARTESIAN_POINT('Ctrl Pts',(-18.1112592327896,-14.3105816243954,
115.112569155571)) ;
#183724=CARTESIAN_POINT('Ctrl Pts',(-18.126546298458,-14.2526152270872,
115.159131089373)) ;
#183725=CARTESIAN_POINT('Ctrl Pts',(-18.1929627182085,-14.4080507138092,
115.39693012817)) ;
#183726=CARTESIAN_POINT('Ctrl Pts',(-18.202900452688,-14.3391479238767,
115.427198862157)) ;
#183727=CARTESIAN_POINT('Ctrl Pts',(-18.1290966355056,-14.3391479627699,
115.451429983758)) ;
#183728=CARTESIAN_POINT('Ctrl Pts',(-18.055292818323,-14.3391480016631,
115.475661105359)) ;
#183729=CARTESIAN_POINT('Ctrl Pts',(-18.0453550838435,-14.4080507915956,
115.445392371372)) ;
#183730=CARTESIAN_POINT('Ctrl Pts',(-18.0354173493639,-14.4769535815281,
115.415123637385)) ;
#183731=CARTESIAN_POINT('Ctrl Pts',(-18.1092211665464,-14.4769535426349,
115.390892515784)) ;
#183732=CARTESIAN_POINT('Ctrl Pts',(-18.1830249837289,-14.4769535037417,
115.366661394183)) ;
#183733=CARTESIAN_POINT('Ctrl Pts',(-18.1929627182085,-14.4080507138092,
115.39693012817)) ;
#183734=CARTESIAN_POINT('Ctrl Pts',(-18.2695829032393,-14.4922598223547,
115.665846830142)) ;
#183735=CARTESIAN_POINT('Ctrl Pts',(-18.2734503895257,-14.4173770699575,
115.677626567456)) ;
#183736=CARTESIAN_POINT('Ctrl Pts',(-18.1996465763506,-14.4173770858156,
115.701857701262)) ;
#183737=CARTESIAN_POINT('Ctrl Pts',(-18.1258427631755,-14.4173771016737,
115.726088835069)) ;
#183738=CARTESIAN_POINT('Ctrl Pts',(-18.1219752768891,-14.4922598540709,
115.714309097756)) ;
#183739=CARTESIAN_POINT('Ctrl Pts',(-18.1181077906028,-14.5671426064681,
115.702529360442)) ;
#183740=CARTESIAN_POINT('Ctrl Pts',(-18.1919116037779,-14.56714259061,115.678298226636)) ;
#183741=CARTESIAN_POINT('Ctrl Pts',(-18.265715416953,-14.5671425747519,
115.654067092829)) ;
#183742=CARTESIAN_POINT('Ctrl Pts',(-18.2695829032393,-14.4922598223547,
115.665846830142)) ;
#183743=CARTESIAN_POINT('Ctrl Pts',(-18.3495327203372,-14.4995566650645,
115.94467290167)) ;
#183744=CARTESIAN_POINT('Ctrl Pts',(-18.3470933653197,-14.4240553765711,
115.937243017908)) ;
#183745=CARTESIAN_POINT('Ctrl Pts',(-18.2732895534782,-14.4240553658153,
115.961474155777)) ;
#183746=CARTESIAN_POINT('Ctrl Pts',(-18.1994857416366,-14.4240553550595,
115.985705293645)) ;
#183747=CARTESIAN_POINT('Ctrl Pts',(-18.2019250966542,-14.4995566435528,
115.993135177407)) ;
#183748=CARTESIAN_POINT('Ctrl Pts',(-18.2043644516717,-14.5750579320462,
116.000565061168)) ;
#183749=CARTESIAN_POINT('Ctrl Pts',(-18.2781682635132,-14.575057942802,
115.9763339233)) ;
#183750=CARTESIAN_POINT('Ctrl Pts',(-18.3519720753547,-14.5750579535578,
115.952102785431)) ;
#183751=CARTESIAN_POINT('Ctrl Pts',(-18.3495327203372,-14.4995566650645,
115.94467290167)) ;
#183752=CARTESIAN_POINT('Ctrl Pts',(-18.4275077803074,-14.4291954268347,
116.217786788456)) ;
#183753=CARTESIAN_POINT('Ctrl Pts',(-18.418884064598,-14.3584951723125,
116.191520339796)) ;
#183754=CARTESIAN_POINT('Ctrl Pts',(-18.3450802518238,-14.3584951335383,
116.215751474823)) ;
#183755=CARTESIAN_POINT('Ctrl Pts',(-18.2712764390496,-14.358495094764,
116.239982609851)) ;
#183756=CARTESIAN_POINT('Ctrl Pts',(-18.279900154759,-14.4291953492863,
116.266249058511)) ;
#183757=CARTESIAN_POINT('Ctrl Pts',(-18.2885238704684,-14.4998956038086,
116.292515507171)) ;
#183758=CARTESIAN_POINT('Ctrl Pts',(-18.3623276832426,-14.4998956425828,
116.268284372143)) ;
#183759=CARTESIAN_POINT('Ctrl Pts',(-18.4361314960168,-14.499895681357,
116.244053237115)) ;
#183760=CARTESIAN_POINT('Ctrl Pts',(-18.4275077803074,-14.4291954268347,
116.217786788456)) ;
#183761=CARTESIAN_POINT('Ctrl Pts',(-18.4961354751818,-14.2862746553945,
116.462278671806)) ;
#183762=CARTESIAN_POINT('Ctrl Pts',(-18.4819739418317,-14.2254484542933,
116.4191449241)) ;
#183763=CARTESIAN_POINT('Ctrl Pts',(-18.4081701251921,-14.2254483895805,
116.443376047354)) ;
#183764=CARTESIAN_POINT('Ctrl Pts',(-18.3343663085526,-14.2254483248678,
116.467607170609)) ;
#183765=CARTESIAN_POINT('Ctrl Pts',(-18.3485278419026,-14.286274525969,
116.510740918315)) ;
#183766=CARTESIAN_POINT('Ctrl Pts',(-18.3626893752527,-14.3471007270702,
116.553874666022)) ;
#183767=CARTESIAN_POINT('Ctrl Pts',(-18.4364931918923,-14.347100791783,
116.529643542767)) ;
#183768=CARTESIAN_POINT('Ctrl Pts',(-18.5102970085318,-14.3471008564957,
116.505412419513)) ;
#183769=CARTESIAN_POINT('Ctrl Pts',(-18.4961354751818,-14.2862746553945,
116.462278671806)) ;
#183770=CARTESIAN_POINT('Ctrl Pts',(-18.5499768620455,-14.0821782924177,
116.661608442272)) ;
#183771=CARTESIAN_POINT('Ctrl Pts',(-18.5313042749872,-14.0355118999346,
116.60473475281)) ;
#183772=CARTESIAN_POINT('Ctrl Pts',(-18.4575004522042,-14.0355118141507,
116.628965857352)) ;
#183773=CARTESIAN_POINT('Ctrl Pts',(-18.3836966294212,-14.0355117283667,
116.653196961895)) ;
#183774=CARTESIAN_POINT('Ctrl Pts',(-18.4023692164795,-14.0821781208498,
116.710070651357)) ;
#183775=CARTESIAN_POINT('Ctrl Pts',(-18.4210418035377,-14.1288445133328,
116.766944340819)) ;
#183776=CARTESIAN_POINT('Ctrl Pts',(-18.4948456263207,-14.1288445991168,
116.742713236277)) ;
#183777=CARTESIAN_POINT('Ctrl Pts',(-18.5686494491038,-14.1288446849008,
116.718482131734)) ;
#183778=CARTESIAN_POINT('Ctrl Pts',(-18.5499768620455,-14.0821782924177,
116.661608442272)) ;
#183779=CARTESIAN_POINT('Ctrl Pts',(-18.5848332719322,-13.8298750263426,
116.803243954575)) ;
#183780=CARTESIAN_POINT('Ctrl Pts',(-18.5629655938444,-13.8007543288235,
116.736638533363)) ;
#183781=CARTESIAN_POINT('Ctrl Pts',(-18.4891617631906,-13.8007542285384,
116.760869613933)) ;
#183782=CARTESIAN_POINT('Ctrl Pts',(-18.4153579325368,-13.8007541282534,
116.785100694502)) ;
#183783=CARTESIAN_POINT('Ctrl Pts',(-18.4372256106246,-13.8298748257726,
116.851706115714)) ;
#183784=CARTESIAN_POINT('Ctrl Pts',(-18.4590932887124,-13.8589955232917,
116.918311536925)) ;
#183785=CARTESIAN_POINT('Ctrl Pts',(-18.5328971193662,-13.8589956235767,
116.894080456356)) ;
#183786=CARTESIAN_POINT('Ctrl Pts',(-18.6067009500199,-13.8589957238618,
116.869849375786)) ;
#183787=CARTESIAN_POINT('Ctrl Pts',(-18.5848332719322,-13.8298750263426,
116.803243954575)) ;
#183788=CARTESIAN_POINT('Ctrl Pts',(-18.597136541653,-13.5470860719876,
116.876296357144)) ;
#183789=CARTESIAN_POINT('Ctrl Pts',(-18.5736411104493,-13.5376651784076,
116.804733062608)) ;
#183790=CARTESIAN_POINT('Ctrl Pts',(-18.4998372709234,-13.5376650723535,
116.828964116154)) ;
#183791=CARTESIAN_POINT('Ctrl Pts',(-18.4260334313975,-13.5376649662995,
116.8531951697)) ;
#183792=CARTESIAN_POINT('Ctrl Pts',(-18.4495288626012,-13.5470858598794,
116.924758464237)) ;
#183793=CARTESIAN_POINT('Ctrl Pts',(-18.4730242938049,-13.5565067534594,
116.996321758773)) ;
#183794=CARTESIAN_POINT('Ctrl Pts',(-18.5468281333308,-13.5565068595135,
116.972090705226)) ;
#183795=CARTESIAN_POINT('Ctrl Pts',(-18.6206319728567,-13.5565069655676,
116.94785965168)) ;
#183796=CARTESIAN_POINT('Ctrl Pts',(-18.597136541653,-13.5470860719876,
116.876296357144)) ;
#183797=CARTESIAN_POINT('Ctrl Pts',(-18.5852386802465,-13.2560613841224,
116.875504551637)) ;
#183798=CARTESIAN_POINT('Ctrl Pts',(-18.561805431591,-13.2669448864172,
116.804130655157)) ;
#183799=CARTESIAN_POINT('Ctrl Pts',(-18.4880015832393,-13.266944783336,
116.828361681822)) ;
#183800=CARTESIAN_POINT('Ctrl Pts',(-18.4141977348876,-13.2669446802549,
116.852592708486)) ;
#183801=CARTESIAN_POINT('Ctrl Pts',(-18.4376309835431,-13.2560611779601,
116.923966604966)) ;
#183802=CARTESIAN_POINT('Ctrl Pts',(-18.4610642321986,-13.2451776756653,
116.995340501446)) ;
#183803=CARTESIAN_POINT('Ctrl Pts',(-18.5348680805503,-13.2451777787465,
116.971109474781)) ;
#183804=CARTESIAN_POINT('Ctrl Pts',(-18.6086719289019,-13.2451778818276,
116.946878448116)) ;
#183805=CARTESIAN_POINT('Ctrl Pts',(-18.5852386802465,-13.2560613841224,
116.875504551637)) ;
#183806=CARTESIAN_POINT('Ctrl Pts',(-18.549259012026,-12.9762949722028,
116.801413358043)) ;
#183807=CARTESIAN_POINT('Ctrl Pts',(-18.5275681764739,-13.0067272528639,
116.735346570811)) ;
#183808=CARTESIAN_POINT('Ctrl Pts',(-18.4537643202221,-13.0067271611354,
116.759577573413)) ;
#183809=CARTESIAN_POINT('Ctrl Pts',(-18.3799604639702,-13.0067270694068,
116.783808576015)) ;
#183810=CARTESIAN_POINT('Ctrl Pts',(-18.4016512995223,-12.9762947887458,
116.849875363246)) ;
#183811=CARTESIAN_POINT('Ctrl Pts',(-18.4233421350744,-12.9458625080848,
116.915942150478)) ;
#183812=CARTESIAN_POINT('Ctrl Pts',(-18.4971459913262,-12.9458625998133,
116.891711147876)) ;
#183813=CARTESIAN_POINT('Ctrl Pts',(-18.570949847578,-12.9458626915418,
116.867480145274)) ;
#183814=CARTESIAN_POINT('Ctrl Pts',(-18.549259012026,-12.9762949722028,
116.801413358043)) ;
#183815=CARTESIAN_POINT('Ctrl Pts',(-18.4912772241492,-12.729021213087,
116.66017876415)) ;
#183816=CARTESIAN_POINT('Ctrl Pts',(-18.4728702553292,-12.7767631435002,
116.604114105214)) ;
#183817=CARTESIAN_POINT('Ctrl Pts',(-18.3990663927569,-12.7767630691524,
116.628345088564)) ;
#183818=CARTESIAN_POINT('Ctrl Pts',(-18.3252625301846,-12.7767629948046,
116.652576071915)) ;
#183819=CARTESIAN_POINT('Ctrl Pts',(-18.3436694990045,-12.7290210643915,
116.708640730851)) ;
#183820=CARTESIAN_POINT('Ctrl Pts',(-18.3620764678245,-12.6812791339783,
116.764705389787)) ;
#183821=CARTESIAN_POINT('Ctrl Pts',(-18.4358803303968,-12.6812792083261,
116.740474406437)) ;
#183822=CARTESIAN_POINT('Ctrl Pts',(-18.5096841929691,-12.6812792826738,
116.716243423086)) ;
#183823=CARTESIAN_POINT('Ctrl Pts',(-18.4912772241492,-12.729021213087,
116.66017876415)) ;
#183824=CARTESIAN_POINT('Ctrl Pts',(-18.4142572250889,-12.5300504685621,
116.461103914665)) ;
#183825=CARTESIAN_POINT('Ctrl Pts',(-18.4004650084343,-12.5917559666324,
116.419095046349)) ;
#183826=CARTESIAN_POINT('Ctrl Pts',(-18.3266611418317,-12.5917559147477,
116.443326017425)) ;
#183827=CARTESIAN_POINT('Ctrl Pts',(-18.2528572752292,-12.5917558628629,
116.4675569885)) ;
#183828=CARTESIAN_POINT('Ctrl Pts',(-18.2666494918838,-12.5300503647925,
116.509565856816)) ;
#183829=CARTESIAN_POINT('Ctrl Pts',(-18.2804417085384,-12.4683448667222,
116.551574725132)) ;
#183830=CARTESIAN_POINT('Ctrl Pts',(-18.3542455751409,-12.468344918607,
116.527343754057)) ;
#183831=CARTESIAN_POINT('Ctrl Pts',(-18.4280494417435,-12.4683449704918,
116.503112782981)) ;
#183832=CARTESIAN_POINT('Ctrl Pts',(-18.4142572250889,-12.5300504685621,
116.461103914665)) ;
#183833=CARTESIAN_POINT('Ctrl Pts',(-18.3230315098279,-12.3949013412461,
116.218789967548)) ;
#183834=CARTESIAN_POINT('Ctrl Pts',(-18.3148521863386,-12.4661360013531,
116.193877066313)) ;
#183835=CARTESIAN_POINT('Ctrl Pts',(-18.2410483183401,-12.4661359735393,
116.218108033137)) ;
#183836=CARTESIAN_POINT('Ctrl Pts',(-18.1672444503415,-12.4661359457255,
116.24233899996)) ;
#183837=CARTESIAN_POINT('Ctrl Pts',(-18.1754237738308,-12.3949012856185,
116.267251901195)) ;
#183838=CARTESIAN_POINT('Ctrl Pts',(-18.18360309732,-12.3236666255115,116.29216480243)) ;
#183839=CARTESIAN_POINT('Ctrl Pts',(-18.2574069653186,-12.3236666533253,
116.267933835606)) ;
#183840=CARTESIAN_POINT('Ctrl Pts',(-18.3312108333171,-12.3236666811392,
116.243702868783)) ;
#183841=CARTESIAN_POINT('Ctrl Pts',(-18.3230315098279,-12.3949013412461,
116.218789967548)) ;
#183842=CARTESIAN_POINT('Ctrl Pts',(-18.223852812221,-12.3334783627152,
115.952132037095)) ;
#183843=CARTESIAN_POINT('Ctrl Pts',(-18.2218527152486,-12.4091090544744,
115.946040062949)) ;
#183844=CARTESIAN_POINT('Ctrl Pts',(-18.1480488479811,-12.4091090490569,
115.970271031999)) ;
#183845=CARTESIAN_POINT('Ctrl Pts',(-18.0742449807137,-12.4091090436395,
115.99450200105)) ;
#183846=CARTESIAN_POINT('Ctrl Pts',(-18.0762450776861,-12.3334783518803,
116.000593975195)) ;
#183847=CARTESIAN_POINT('Ctrl Pts',(-18.0782451746585,-12.2578476601211,
116.006685949341)) ;
#183848=CARTESIAN_POINT('Ctrl Pts',(-18.1520490419259,-12.2578476655386,
115.98245498029)) ;
#183849=CARTESIAN_POINT('Ctrl Pts',(-18.2258529091934,-12.257847670956,
115.95822401124)) ;
#183850=CARTESIAN_POINT('Ctrl Pts',(-18.223852812221,-12.3334783627152,
115.952132037095)) ;
#183851=CARTESIAN_POINT('Ctrl Pts',(-18.1228645176016,-12.3494129205617,
115.679929191813)) ;
#183852=CARTESIAN_POINT('Ctrl Pts',(-18.1271800410317,-12.4240452801496,
115.69307357853)) ;
#183853=CARTESIAN_POINT('Ctrl Pts',(-18.0533761763498,-12.4240452938977,
115.717304555455)) ;
#183854=CARTESIAN_POINT('Ctrl Pts',(-17.9795723116678,-12.4240453076458,
115.74153553238)) ;
#183855=CARTESIAN_POINT('Ctrl Pts',(-17.9752567882376,-12.3494129480579,
115.728391145663)) ;
#183856=CARTESIAN_POINT('Ctrl Pts',(-17.9709412648075,-12.27478058847,115.715246758947)) ;
#183857=CARTESIAN_POINT('Ctrl Pts',(-18.0447451294895,-12.2747805747219,
115.691015782021)) ;
#183858=CARTESIAN_POINT('Ctrl Pts',(-18.1185489941715,-12.2747805609737,
115.666784805096)) ;
#183859=CARTESIAN_POINT('Ctrl Pts',(-18.1228645176016,-12.3494129205617,
115.679929191813)) ;
#183860=CARTESIAN_POINT('Ctrl Pts',(-18.0261149973896,-12.4418688951199,
115.420743578469)) ;
#183861=CARTESIAN_POINT('Ctrl Pts',(-18.036457582096,-12.5101591784945,
115.452245421536)) ;
#183862=CARTESIAN_POINT('Ctrl Pts',(-17.9626537217423,-12.5101592062549,
115.476476411644)) ;
#183863=CARTESIAN_POINT('Ctrl Pts',(-17.8888498613887,-12.5101592340153,
115.500707401753)) ;
#183864=CARTESIAN_POINT('Ctrl Pts',(-17.8785072766823,-12.4418689506407,
115.469205558686)) ;
#183865=CARTESIAN_POINT('Ctrl Pts',(-17.868164691976,-12.373578667266,115.43770371562)) ;
#183866=CARTESIAN_POINT('Ctrl Pts',(-17.9419685523296,-12.3735786395056,
115.413472725511)) ;
#183867=CARTESIAN_POINT('Ctrl Pts',(-18.0157724126832,-12.3735786117452,
115.389241735402)) ;
#183868=CARTESIAN_POINT('Ctrl Pts',(-18.0261149973896,-12.4418688951199,
115.420743578469)) ;
#183869=CARTESIAN_POINT('Ctrl Pts',(-17.9399661082425,-12.6051421932678,
115.193941498684)) ;
#183870=CARTESIAN_POINT('Ctrl Pts',(-17.955602936904,-12.6621364558016,
115.241568754806)) ;
#183871=CARTESIAN_POINT('Ctrl Pts',(-17.881799081728,-12.6621364903346,
115.265799760685)) ;
#183872=CARTESIAN_POINT('Ctrl Pts',(-17.807995226552,-12.6621365248676,
115.290030766564)) ;
#183873=CARTESIAN_POINT('Ctrl Pts',(-17.7923583978905,-12.6051422623338,
115.242403510442)) ;
#183874=CARTESIAN_POINT('Ctrl Pts',(-17.776721569229,-12.5481479998,115.19477625432)) ;
#183875=CARTESIAN_POINT('Ctrl Pts',(-17.850525424405,-12.548147965267,115.170545248441)) ;
#183876=CARTESIAN_POINT('Ctrl Pts',(-17.9243292795811,-12.548147930734,
115.146314242563)) ;
#183877=CARTESIAN_POINT('Ctrl Pts',(-17.9399661082425,-12.6051421932678,
115.193941498684)) ;
#183878=CARTESIAN_POINT('Ctrl Pts',(-17.8706577437902,-12.824581983231,
115.018086912983)) ;
#183879=CARTESIAN_POINT('Ctrl Pts',(-17.8904279981358,-12.866340572483,
115.078303916939)) ;
#183880=CARTESIAN_POINT('Ctrl Pts',(-17.8166241473241,-12.8663406101773,
115.102534936111)) ;
#183881=CARTESIAN_POINT('Ctrl Pts',(-17.7428202965123,-12.8663406478716,
115.126765955283)) ;
#183882=CARTESIAN_POINT('Ctrl Pts',(-17.7230500421668,-12.8245820586196,
115.066548951326)) ;
#183883=CARTESIAN_POINT('Ctrl Pts',(-17.7032797878212,-12.7828234693676,
115.00633194737)) ;
#183884=CARTESIAN_POINT('Ctrl Pts',(-17.7770836386329,-12.7828234316733,
114.982100928198)) ;
#183885=CARTESIAN_POINT('Ctrl Pts',(-17.8508874894446,-12.782823393979,
114.957869909026)) ;
#183886=CARTESIAN_POINT('Ctrl Pts',(-17.8706577437902,-12.824581983231,
115.018086912983)) ;
#183887=CARTESIAN_POINT('Ctrl Pts',(-17.8211647568461,-13.0878606072953,
114.902837359147)) ;
#183888=CARTESIAN_POINT('Ctrl Pts',(-17.843686172388,-13.1112998695193,
114.971433956383)) ;
#183889=CARTESIAN_POINT('Ctrl Pts',(-17.7698823258549,-13.1112999036755,
114.995664988587)) ;
#183890=CARTESIAN_POINT('Ctrl Pts',(-17.6960784793217,-13.1112999378317,
115.019896020791)) ;
#183891=CARTESIAN_POINT('Ctrl Pts',(-17.6735570637799,-13.0878606756077,
114.951299423555)) ;
#183892=CARTESIAN_POINT('Ctrl Pts',(-17.651035648238,-13.0644214133836,
114.882702826318)) ;
#183893=CARTESIAN_POINT('Ctrl Pts',(-17.7248394947711,-13.0644213792274,
114.858471794115)) ;
#183894=CARTESIAN_POINT('Ctrl Pts',(-17.7986433413042,-13.0644213450712,
114.834240761911)) ;
#183895=CARTESIAN_POINT('Ctrl Pts',(-17.8211647568461,-13.0878606072953,
114.902837359147)) ;
#183896=CARTESIAN_POINT('Ctrl Pts',(-17.7949112979524,-13.3747557627756,
114.858346400162)) ;
#183897=CARTESIAN_POINT('Ctrl Pts',(-17.818565917269,-13.378198596209,114.930394553419)) ;
#183898=CARTESIAN_POINT('Ctrl Pts',(-17.7447620737718,-13.3781986232595,
114.954625594869)) ;
#183899=CARTESIAN_POINT('Ctrl Pts',(-17.6709582302744,-13.37819865031,114.97885663632)) ;
#183900=CARTESIAN_POINT('Ctrl Pts',(-17.6473036109578,-13.3747558168767,
114.906808483063)) ;
#183901=CARTESIAN_POINT('Ctrl Pts',(-17.6236489916412,-13.3713129834433,
114.834760329806)) ;
#183902=CARTESIAN_POINT('Ctrl Pts',(-17.6974528351385,-13.3713129563928,
114.810529288356)) ;
#183903=CARTESIAN_POINT('Ctrl Pts',(-17.7712566786358,-13.3713129293423,
114.786298246905)) ;
#183904=CARTESIAN_POINT('Ctrl Pts',(-17.7949112979524,-13.3747557627756,
114.858346400162)) ;
#183905=CARTESIAN_POINT('Ctrl Pts',(-17.7930142307547,-13.6654070056361,
114.888132109586)) ;
#183906=CARTESIAN_POINT('Ctrl Pts',(-17.8161012539618,-13.648560400251,
114.958451456842)) ;
#183907=CARTESIAN_POINT('Ctrl Pts',(-17.7422974120605,-13.6485604179734,
114.982682503154)) ;
#183908=CARTESIAN_POINT('Ctrl Pts',(-17.6684935701592,-13.6485604356957,
115.006913549465)) ;
#183909=CARTESIAN_POINT('Ctrl Pts',(-17.6454065469521,-13.6654070410809,
114.936594202209)) ;
#183910=CARTESIAN_POINT('Ctrl Pts',(-17.6223195237451,-13.682253646466,
114.866274854952)) ;
#183911=CARTESIAN_POINT('Ctrl Pts',(-17.6961233656464,-13.6822536287436,
114.84204380864)) ;
#183912=CARTESIAN_POINT('Ctrl Pts',(-17.7699272075477,-13.6822536110213,
114.817812762329)) ;
#183913=CARTESIAN_POINT('Ctrl Pts',(-17.7930142307547,-13.6654070056361,
114.888132109586)) ;
#183914=CARTESIAN_POINT('Ctrl Pts',(-17.8147252087611,-13.9370542943595,
114.989647338605)) ;
#183915=CARTESIAN_POINT('Ctrl Pts',(-17.835598783078,-13.901214603103,115.053224877806)) ;
#183916=CARTESIAN_POINT('Ctrl Pts',(-17.7617949415956,-13.9012146131836,
115.077455925394)) ;
#183917=CARTESIAN_POINT('Ctrl Pts',(-17.6879911001133,-13.9012146232642,
115.101686972982)) ;
#183918=CARTESIAN_POINT('Ctrl Pts',(-17.6671175257964,-13.9370543145207,
115.03810943378)) ;
#183919=CARTESIAN_POINT('Ctrl Pts',(-17.6462439514795,-13.9728940057772,
114.974531894578)) ;
#183920=CARTESIAN_POINT('Ctrl Pts',(-17.7200477929618,-13.9728939956966,
114.95030084699)) ;
#183921=CARTESIAN_POINT('Ctrl Pts',(-17.7938516344442,-13.972893985616,
114.926069799403)) ;
#183922=CARTESIAN_POINT('Ctrl Pts',(-17.8147252087611,-13.9370542943595,
114.989647338605)) ;
#183923=CARTESIAN_POINT('Ctrl Pts',(-17.8580728556449,-14.1729033532404,
115.157292589129)) ;
#183924=CARTESIAN_POINT('Ctrl Pts',(-17.8752140934939,-14.1205407691761,
115.209502033795)) ;
#183925=CARTESIAN_POINT('Ctrl Pts',(-17.8014102512489,-14.1205407723559,
115.233733079059)) ;
#183926=CARTESIAN_POINT('Ctrl Pts',(-17.7276064090039,-14.1205407755357,
115.257964124324)) ;
#183927=CARTESIAN_POINT('Ctrl Pts',(-17.7104651711549,-14.1729033596,115.205754679658)) ;
#183928=CARTESIAN_POINT('Ctrl Pts',(-17.6933239333059,-14.2252659436643,
115.153545234993)) ;
#183929=CARTESIAN_POINT('Ctrl Pts',(-17.7671277755509,-14.2252659404845,
115.129314189728)) ;
#183930=CARTESIAN_POINT('Ctrl Pts',(-17.8409316177959,-14.2252659373047,
115.105083144464)) ;
#183931=CARTESIAN_POINT('Ctrl Pts',(-17.8580728556449,-14.1729033532404,
115.157292589129)) ;
#183932=CARTESIAN_POINT('Ctrl Pts',(-17.9184133421674,-14.3528610645483,
115.376351104933)) ;
#183933=CARTESIAN_POINT('Ctrl Pts',(-17.9306369507618,-14.2878546501218,
115.413582244416)) ;
#183934=CARTESIAN_POINT('Ctrl Pts',(-17.8568331077171,-14.2878546504462,
115.437813287245)) ;
#183935=CARTESIAN_POINT('Ctrl Pts',(-17.7830292646724,-14.2878546507707,
115.462044330074)) ;
#183936=CARTESIAN_POINT('Ctrl Pts',(-17.7708056560779,-14.3528610651972,
115.42481319059)) ;
#183937=CARTESIAN_POINT('Ctrl Pts',(-17.7585820474835,-14.4178674796237,
115.387582051107)) ;
#183938=CARTESIAN_POINT('Ctrl Pts',(-17.8323858905282,-14.4178674792993,
115.363351008278)) ;
#183939=CARTESIAN_POINT('Ctrl Pts',(-17.906189733573,-14.4178674789748,
115.339119965449)) ;
#183940=CARTESIAN_POINT('Ctrl Pts',(-17.9184133421674,-14.3528610645483,
115.376351104933)) ;
#183941=CARTESIAN_POINT('Ctrl Pts',(-17.991766676009,-14.4673900074207,
115.635384696762)) ;
#183942=CARTESIAN_POINT('Ctrl Pts',(-17.9981494388776,-14.3942885636895,
115.654825562653)) ;
#183943=CARTESIAN_POINT('Ctrl Pts',(-17.9243455947338,-14.39428856281,115.679056602134)) ;
#183944=CARTESIAN_POINT('Ctrl Pts',(-17.8505417505901,-14.3942885619306,
115.703287641616)) ;
#183945=CARTESIAN_POINT('Ctrl Pts',(-17.8441589877216,-14.4673900056618,
115.683846775725)) ;
#183946=CARTESIAN_POINT('Ctrl Pts',(-17.837776224853,-14.5404914493931,
115.664405909834)) ;
#183947=CARTESIAN_POINT('Ctrl Pts',(-17.9115800689967,-14.5404914502725,
115.640174870352)) ;
#183948=CARTESIAN_POINT('Ctrl Pts',(-17.9853839131405,-14.540491451152,
115.615943830871)) ;
#183949=CARTESIAN_POINT('Ctrl Pts',(-17.991766676009,-14.4673900074207,
115.635384696762)) ;
#183950=CARTESIAN_POINT('Ctrl Pts',(-18.0711284340199,-14.5059091307987,
115.912498667304)) ;
#183951=CARTESIAN_POINT('Ctrl Pts',(-18.0712464888033,-14.4300095722764,
115.91285824319)) ;
#183952=CARTESIAN_POINT('Ctrl Pts',(-17.9974426443487,-14.4300095722936,
115.937089281725)) ;
#183953=CARTESIAN_POINT('Ctrl Pts',(-17.9236387998941,-14.4300095723109,
115.96132032026)) ;
#183954=CARTESIAN_POINT('Ctrl Pts',(-17.9235207451107,-14.5059091308332,
115.960960744373)) ;
#183955=CARTESIAN_POINT('Ctrl Pts',(-17.9234026903274,-14.5818086893555,
115.960601168487)) ;
#183956=CARTESIAN_POINT('Ctrl Pts',(-17.997206534782,-14.5818086893382,
115.936370129952)) ;
#183957=CARTESIAN_POINT('Ctrl Pts',(-18.0710103792366,-14.581808689321,
115.912139091418)) ;
#183958=CARTESIAN_POINT('Ctrl Pts',(-18.0711284340199,-14.5059091307987,
115.912498667304)) ;
#183959=CARTESIAN_POINT('Ctrl Pts',(-18.1505342643703,-14.467003448986,
116.1897784186)) ;
#183960=CARTESIAN_POINT('Ctrl Pts',(-18.1443746311779,-14.3937086480908,
116.171017169796)) ;
#183961=CARTESIAN_POINT('Ctrl Pts',(-18.0705707870571,-14.3937086489183,
116.195248209347)) ;
#183962=CARTESIAN_POINT('Ctrl Pts',(-17.9967669429363,-14.3937086497458,
116.219479248898)) ;
#183963=CARTESIAN_POINT('Ctrl Pts',(-18.0029265761288,-14.4670034506409,
116.238240497703)) ;
#183964=CARTESIAN_POINT('Ctrl Pts',(-18.0090862093212,-14.5402982515361,
116.257001746507)) ;
#183965=CARTESIAN_POINT('Ctrl Pts',(-18.082890053442,-14.5402982507086,
116.232770706956)) ;
#183966=CARTESIAN_POINT('Ctrl Pts',(-18.1566938975628,-14.5402982498811,
116.208539667404)) ;
#183967=CARTESIAN_POINT('Ctrl Pts',(-18.1505342643703,-14.467003448986,
116.1897784186)) ;
#183968=CARTESIAN_POINT('Ctrl Pts',(-18.2236575677772,-14.3526296857438,
116.448006484568)) ;
#183969=CARTESIAN_POINT('Ctrl Pts',(-18.2116480597675,-14.2872135873285,
116.411427460882)) ;
#183970=CARTESIAN_POINT('Ctrl Pts',(-18.1378442166257,-14.2872135872054,
116.435658503415)) ;
#183971=CARTESIAN_POINT('Ctrl Pts',(-18.0640403734839,-14.2872135870823,
116.459889545948)) ;
#183972=CARTESIAN_POINT('Ctrl Pts',(-18.0760498814937,-14.3526296854977,
116.496468569635)) ;
#183973=CARTESIAN_POINT('Ctrl Pts',(-18.0880593895034,-14.418045783913,
116.533047593321)) ;
#183974=CARTESIAN_POINT('Ctrl Pts',(-18.1618632326452,-14.4180457840361,
116.508816550788)) ;
#183975=CARTESIAN_POINT('Ctrl Pts',(-18.2356670757869,-14.4180457841592,
116.484585508255)) ;
#183976=CARTESIAN_POINT('Ctrl Pts',(-18.2236575677772,-14.3526296857438,
116.448006484568)) ;
#183977=CARTESIAN_POINT('Ctrl Pts',(-18.2841253649015,-14.1719531187117,
116.667560097024)) ;
#183978=CARTESIAN_POINT('Ctrl Pts',(-18.2671440519089,-14.1190573784708,
116.615837757477)) ;
#183979=CARTESIAN_POINT('Ctrl Pts',(-18.1933402096846,-14.1190573751839,
116.640068802804)) ;
#183980=CARTESIAN_POINT('Ctrl Pts',(-18.1195363674603,-14.119057371897,
116.664299848132)) ;
#183981=CARTESIAN_POINT('Ctrl Pts',(-18.1365176804528,-14.1719531121379,
116.716022187679)) ;
#183982=CARTESIAN_POINT('Ctrl Pts',(-18.1534989934453,-14.2248488523788,
116.767744527226)) ;
#183983=CARTESIAN_POINT('Ctrl Pts',(-18.2273028356696,-14.2248488556657,
116.743513481899)) ;
#183984=CARTESIAN_POINT('Ctrl Pts',(-18.301106677894,-14.2248488589527,
116.719282436571)) ;
#183985=CARTESIAN_POINT('Ctrl Pts',(-18.2841253649015,-14.1719531187117,
116.667560097024)) ;
#183986=CARTESIAN_POINT('Ctrl Pts',(-18.3272925522858,-13.936583984801,
116.834555335885)) ;
#183987=CARTESIAN_POINT('Ctrl Pts',(-18.3065373884678,-13.9000456634002,
116.771338455511)) ;
#183988=CARTESIAN_POINT('Ctrl Pts',(-18.2327335469008,-13.9000456537943,
116.79556950284)) ;
#183989=CARTESIAN_POINT('Ctrl Pts',(-18.1589297053339,-13.9000456441885,
116.81980055017)) ;
#183990=CARTESIAN_POINT('Ctrl Pts',(-18.1796848691519,-13.9365839655893,
116.883017430544)) ;
#183991=CARTESIAN_POINT('Ctrl Pts',(-18.2004400329699,-13.9731222869902,
116.946234310919)) ;
#183992=CARTESIAN_POINT('Ctrl Pts',(-18.2742438745369,-13.973122296596,
116.922003263589)) ;
#183993=CARTESIAN_POINT('Ctrl Pts',(-18.3480477161039,-13.9731223062019,
116.897772216259)) ;
#183994=CARTESIAN_POINT('Ctrl Pts',(-18.3272925522858,-13.936583984801,
116.834555335885)) ;
#183995=CARTESIAN_POINT('Ctrl Pts',(-18.3489789369998,-13.6642946874373,
116.936073490923)) ;
#183996=CARTESIAN_POINT('Ctrl Pts',(-18.3259455354646,-13.6467154172206,
116.865917465918)) ;
#183997=CARTESIAN_POINT('Ctrl Pts',(-18.2521416935426,-13.646715399489,
116.890148512166)) ;
#183998=CARTESIAN_POINT('Ctrl Pts',(-18.1783378516205,-13.6467153817574,
116.914379558414)) ;
#183999=CARTESIAN_POINT('Ctrl Pts',(-18.2013712531556,-13.664294651974,
116.984535583419)) ;
#184000=CARTESIAN_POINT('Ctrl Pts',(-18.2244046546907,-13.6818739221906,
117.054691608424)) ;
#184001=CARTESIAN_POINT('Ctrl Pts',(-18.2982084966128,-13.6818739399222,
117.030460562176)) ;
#184002=CARTESIAN_POINT('Ctrl Pts',(-18.3720123385349,-13.6818739576539,
117.006229515928)) ;
#184003=CARTESIAN_POINT('Ctrl Pts',(-18.3489789369998,-13.6642946874373,
116.936073490923)) ;
#184004=CARTESIAN_POINT('Ctrl Pts',(-18.3470303613831,-13.3747428455626,
116.965562261399)) ;
#184005=CARTESIAN_POINT('Ctrl Pts',(-18.3233666532677,-13.377355159395,
116.893486424106)) ;
#184006=CARTESIAN_POINT('Ctrl Pts',(-18.2495628097586,-13.3773551335995,
116.91771746552)) ;
#184007=CARTESIAN_POINT('Ctrl Pts',(-18.1757589662495,-13.3773551078041,
116.941948506935)) ;
#184008=CARTESIAN_POINT('Ctrl Pts',(-18.199422674365,-13.3747427939718,
117.014024344228)) ;
#184009=CARTESIAN_POINT('Ctrl Pts',(-18.2230863824804,-13.3721304801394,
117.086100181521)) ;
#184010=CARTESIAN_POINT('Ctrl Pts',(-18.2968902259895,-13.3721305059348,
117.061869140106)) ;
#184011=CARTESIAN_POINT('Ctrl Pts',(-18.3706940694986,-13.3721305317302,
117.037638098692)) ;
#184012=CARTESIAN_POINT('Ctrl Pts',(-18.3470303613831,-13.3747428455626,
116.965562261399)) ;
#184013=CARTESIAN_POINT('Ctrl Pts',(-18.3207665837922,-13.0876482903165,
116.921069134503)) ;
#184014=CARTESIAN_POINT('Ctrl Pts',(-18.2981677310769,-13.1103096275797,
116.852236674777)) ;
#184015=CARTESIAN_POINT('Ctrl Pts',(-18.2243638846365,-13.1103095944857,
116.876467707263)) ;
#184016=CARTESIAN_POINT('Ctrl Pts',(-18.1505600381961,-13.1103095613917,
116.900698739749)) ;
#184017=CARTESIAN_POINT('Ctrl Pts',(-18.1731588909114,-13.0876482241285,
116.969531199475)) ;
#184018=CARTESIAN_POINT('Ctrl Pts',(-18.1957577436267,-13.0649868868653,
117.038363659201)) ;
#184019=CARTESIAN_POINT('Ctrl Pts',(-18.2695615900671,-13.0649869199593,
117.014132626715)) ;
#184020=CARTESIAN_POINT('Ctrl Pts',(-18.3433654365075,-13.0649869530533,
116.989901594229)) ;
#184021=CARTESIAN_POINT('Ctrl Pts',(-18.3207665837922,-13.0876482903165,
116.921069134503)) ;
#184022=CARTESIAN_POINT('Ctrl Pts',(-18.2712815660308,-12.8243385253649,
116.805840132971)) ;
#184023=CARTESIAN_POINT('Ctrl Pts',(-18.2513706019285,-12.8654169528501,
116.745194548098)) ;
#184024=CARTESIAN_POINT('Ctrl Pts',(-18.1775667513243,-12.8654169160371,
116.769425567902)) ;
#184025=CARTESIAN_POINT('Ctrl Pts',(-18.1037629007201,-12.8654168792241,
116.793656587706)) ;
#184026=CARTESIAN_POINT('Ctrl Pts',(-18.1236738648224,-12.824338451739,
116.854302172579)) ;
#184027=CARTESIAN_POINT('Ctrl Pts',(-18.1435848289247,-12.7832600242539,
116.914947757451)) ;
#184028=CARTESIAN_POINT('Ctrl Pts',(-18.2173886795289,-12.7832600610668,
116.890716737647)) ;
#184029=CARTESIAN_POINT('Ctrl Pts',(-18.2911925301331,-12.7832600978798,
116.866485717843)) ;
#184030=CARTESIAN_POINT('Ctrl Pts',(-18.2712815660308,-12.8243385253649,
116.805840132971)) ;
#184031=CARTESIAN_POINT('Ctrl Pts',(-18.2015034322164,-12.6038922563675,
116.628754857575)) ;
#184032=CARTESIAN_POINT('Ctrl Pts',(-18.1857020695232,-12.6604213844926,
116.580626455347)) ;
#184033=CARTESIAN_POINT('Ctrl Pts',(-18.1118982141328,-12.6604213494665,
116.604857460573)) ;
#184034=CARTESIAN_POINT('Ctrl Pts',(-18.0380943587424,-12.6604213144404,
116.629088465799)) ;
#184035=CARTESIAN_POINT('Ctrl Pts',(-18.0538957214356,-12.6038921863153,
116.677216868027)) ;
#184036=CARTESIAN_POINT('Ctrl Pts',(-18.0696970841289,-12.5473630581902,
116.725345270255)) ;
#184037=CARTESIAN_POINT('Ctrl Pts',(-18.1435009395192,-12.5473630932163,
116.701114265029)) ;
#184038=CARTESIAN_POINT('Ctrl Pts',(-18.2173047949096,-12.5473631282424,
116.676883259803)) ;
#184039=CARTESIAN_POINT('Ctrl Pts',(-18.2015034322164,-12.6038922563675,
116.628754857575)) ;
#184040=CARTESIAN_POINT('Ctrl Pts',(-18.1155659825145,-12.4415502102937,
116.402472433253)) ;
#184041=CARTESIAN_POINT('Ctrl Pts',(-18.1050078606537,-12.5094955214015,
116.370314096439)) ;
#184042=CARTESIAN_POINT('Ctrl Pts',(-18.0312040003716,-12.5094954939584,
116.394545086766)) ;
#184043=CARTESIAN_POINT('Ctrl Pts',(-17.9574001400895,-12.5094954665153,
116.418776077093)) ;
#184044=CARTESIAN_POINT('Ctrl Pts',(-17.9679582619504,-12.4415501554076,
116.450934413906)) ;
#184045=CARTESIAN_POINT('Ctrl Pts',(-17.9785163838113,-12.3736048442999,
116.483092750719)) ;
#184046=CARTESIAN_POINT('Ctrl Pts',(-18.0523202440933,-12.3736048717429,
116.458861760393)) ;
#184047=CARTESIAN_POINT('Ctrl Pts',(-18.1261241043754,-12.373604899186,
116.434630770066)) ;
#184048=CARTESIAN_POINT('Ctrl Pts',(-18.1155659825145,-12.4415502102937,
116.402472433253)) ;
#184049=CARTESIAN_POINT('Ctrl Pts',(-18.0188186140626,-12.3493107874977,
116.143292052209)) ;
#184050=CARTESIAN_POINT('Ctrl Pts',(-18.0142654159233,-12.4237944597024,
116.129423743995)) ;
#184051=CARTESIAN_POINT('Ctrl Pts',(-17.9404615513583,-12.4237944461757,
116.153654721277)) ;
#184052=CARTESIAN_POINT('Ctrl Pts',(-17.8666576867933,-12.4237944326489,
116.177885698558)) ;
#184053=CARTESIAN_POINT('Ctrl Pts',(-17.8712108849327,-12.3493107604442,
116.191754006772)) ;
#184054=CARTESIAN_POINT('Ctrl Pts',(-17.8757640830721,-12.2748270882395,
116.205622314986)) ;
#184055=CARTESIAN_POINT('Ctrl Pts',(-17.949567947637,-12.2748271017662,
116.181391337704)) ;
#184056=CARTESIAN_POINT('Ctrl Pts',(-18.023371812202,-12.274827115293,116.157160360422)) ;
#184057=CARTESIAN_POINT('Ctrl Pts',(-18.0188186140626,-12.3493107874977,
116.143292052209)) ;
#184058=CARTESIAN_POINT('Ctrl Pts',(-17.917965944462,-12.3333698024851,
115.871447888668)) ;
#184059=CARTESIAN_POINT('Ctrl Pts',(-17.9197162551571,-12.409073916813,
115.876779051166)) ;
#184060=CARTESIAN_POINT('Ctrl Pts',(-17.8459123881107,-12.409073922124,
115.901010020889)) ;
#184061=CARTESIAN_POINT('Ctrl Pts',(-17.7721085210643,-12.4090739274351,
115.925240990613)) ;
#184062=CARTESIAN_POINT('Ctrl Pts',(-17.7703582103692,-12.3333698131071,
115.919909828115)) ;
#184063=CARTESIAN_POINT('Ctrl Pts',(-17.7686078996741,-12.2576656987791,
115.914578665616)) ;
#184064=CARTESIAN_POINT('Ctrl Pts',(-17.8424117667205,-12.2576656934681,
115.890347695893)) ;
#184065=CARTESIAN_POINT('Ctrl Pts',(-17.9162156337669,-12.2576656881571,
115.86611672617)) ;
#184066=CARTESIAN_POINT('Ctrl Pts',(-17.917965944462,-12.3333698024851,
115.871447888668)) ;
#184067=CARTESIAN_POINT('Ctrl Pts',(-17.8179951285442,-12.3958418590805,
115.602676622725)) ;
#184068=CARTESIAN_POINT('Ctrl Pts',(-17.825988435529,-12.4672950791635,
115.627022944439)) ;
#184069=CARTESIAN_POINT('Ctrl Pts',(-17.7521845670926,-12.467295107772,
115.651253909928)) ;
#184070=CARTESIAN_POINT('Ctrl Pts',(-17.6783806986561,-12.4672951363806,
115.675484875418)) ;
#184071=CARTESIAN_POINT('Ctrl Pts',(-17.6703873916712,-12.3958419162977,
115.651138553704)) ;
#184072=CARTESIAN_POINT('Ctrl Pts',(-17.6623940846864,-12.3243886962147,
115.62679223199)) ;
#184073=CARTESIAN_POINT('Ctrl Pts',(-17.7361979531229,-12.3243886676062,
115.6025612665)) ;
#184074=CARTESIAN_POINT('Ctrl Pts',(-17.8100018215593,-12.3243886389976,
115.578330301011)) ;
#184075=CARTESIAN_POINT('Ctrl Pts',(-17.8179951285442,-12.3958418590805,
115.602676622725)) ;
#184076=CARTESIAN_POINT('Ctrl Pts',(-17.7275667072708,-12.5305465195612,
115.362515531508)) ;
#184077=CARTESIAN_POINT('Ctrl Pts',(-17.7411552505888,-12.5926984144573,
115.40390404021)) ;
#184078=CARTESIAN_POINT('Ctrl Pts',(-17.6673513841811,-12.592698466259,
115.428135011879)) ;
#184079=CARTESIAN_POINT('Ctrl Pts',(-17.5935475177734,-12.5926985180608,
115.452365983547)) ;
#184080=CARTESIAN_POINT('Ctrl Pts',(-17.5799589744555,-12.5305466231647,
115.410977474846)) ;
#184081=CARTESIAN_POINT('Ctrl Pts',(-17.5663704311375,-12.4683947282686,
115.369588966144)) ;
#184082=CARTESIAN_POINT('Ctrl Pts',(-17.6401742975452,-12.4683946764668,
115.345357994475)) ;
#184083=CARTESIAN_POINT('Ctrl Pts',(-17.7139781639529,-12.4683946246651,
115.321127022806)) ;
#184084=CARTESIAN_POINT('Ctrl Pts',(-17.7275667072708,-12.5305465195612,
115.362515531508)) ;
#184085=CARTESIAN_POINT('Ctrl Pts',(-17.6506148333136,-12.7291635452138,
115.163608506426)) ;
#184086=CARTESIAN_POINT('Ctrl Pts',(-17.6688616218621,-12.7775393659294,
115.219185278384)) ;
#184087=CARTESIAN_POINT('Ctrl Pts',(-17.5950577594212,-12.7775394398199,
115.243416262135)) ;
#184088=CARTESIAN_POINT('Ctrl Pts',(-17.5212538969802,-12.7775395137104,
115.267647245886)) ;
#184089=CARTESIAN_POINT('Ctrl Pts',(-17.5030071084317,-12.7291636929948,
115.212070473928)) ;
#184090=CARTESIAN_POINT('Ctrl Pts',(-17.4847603198832,-12.6807878722793,
115.15649370197)) ;
#184091=CARTESIAN_POINT('Ctrl Pts',(-17.5585641823242,-12.6807877983888,
115.132262718219)) ;
#184092=CARTESIAN_POINT('Ctrl Pts',(-17.6323680447651,-12.6807877244983,
115.108031734468)) ;
#184093=CARTESIAN_POINT('Ctrl Pts',(-17.6506148333136,-12.7291635452138,
115.163608506426)) ;
#184094=CARTESIAN_POINT('Ctrl Pts',(-17.5925315518145,-12.9771312925897,
115.022149073148)) ;
#184095=CARTESIAN_POINT('Ctrl Pts',(-17.6141265834111,-13.0082656414961,
115.087924053104)) ;
#184096=CARTESIAN_POINT('Ctrl Pts',(-17.5403227272072,-13.0082657332076,
115.112155055852)) ;
#184097=CARTESIAN_POINT('Ctrl Pts',(-17.4665188710033,-13.008265824919,
115.1363860586)) ;
#184098=CARTESIAN_POINT('Ctrl Pts',(-17.4449238394067,-12.9771314760126,
115.070611078644)) ;
#184099=CARTESIAN_POINT('Ctrl Pts',(-17.4233288078101,-12.9459971271062,
115.004836098687)) ;
#184100=CARTESIAN_POINT('Ctrl Pts',(-17.497132664014,-12.9459970353947,
114.980605095939)) ;
#184101=CARTESIAN_POINT('Ctrl Pts',(-17.5709365202179,-12.9459969436833,
114.956374093191)) ;
#184102=CARTESIAN_POINT('Ctrl Pts',(-17.5925315518145,-12.9771312925897,
115.022149073148)) ;
#184103=CARTESIAN_POINT('Ctrl Pts',(-17.5565878319294,-13.2574946761857,
114.948229481288)) ;
#184104=CARTESIAN_POINT('Ctrl Pts',(-17.5799882779951,-13.269101018714,
115.019503462338)) ;
#184105=CARTESIAN_POINT('Ctrl Pts',(-17.5061844297033,-13.2691011219862,
115.043734489184)) ;
#184106=CARTESIAN_POINT('Ctrl Pts',(-17.4323805814114,-13.2691012252584,
115.067965516031)) ;
#184107=CARTESIAN_POINT('Ctrl Pts',(-17.4089801353457,-13.2574948827302,
114.996691534982)) ;
#184108=CARTESIAN_POINT('Ctrl Pts',(-17.38557968928,-13.2458885402019,114.925417553932)) ;
#184109=CARTESIAN_POINT('Ctrl Pts',(-17.4593835375718,-13.2458884369297,
114.901186527085)) ;
#184110=CARTESIAN_POINT('Ctrl Pts',(-17.5331873858637,-13.2458883336575,
114.876955500239)) ;
#184111=CARTESIAN_POINT('Ctrl Pts',(-17.5565878319294,-13.2574946761857,
114.948229481288)) ;
#184112=CARTESIAN_POINT('Ctrl Pts',(-17.5448475110634,-13.5486172877669,
114.947929919244)) ;
#184113=CARTESIAN_POINT('Ctrl Pts',(-17.5683683296816,-13.5399156323179,
115.01957053562)) ;
#184114=CARTESIAN_POINT('Ctrl Pts',(-17.4945644902396,-13.5399157383977,
115.043801589422)) ;
#184115=CARTESIAN_POINT('Ctrl Pts',(-17.4207606507977,-13.5399158444775,
115.068032643224)) ;
#184116=CARTESIAN_POINT('Ctrl Pts',(-17.3972398321794,-13.5486174999264,
114.996392026848)) ;
#184117=CARTESIAN_POINT('Ctrl Pts',(-17.3737190135613,-13.5573191553753,
114.924751410472)) ;
#184118=CARTESIAN_POINT('Ctrl Pts',(-17.4475228530032,-13.5573190492956,
114.90052035667)) ;
#184119=CARTESIAN_POINT('Ctrl Pts',(-17.5213266924452,-13.5573189432158,
114.876289302868)) ;
#184120=CARTESIAN_POINT('Ctrl Pts',(-17.5448475110634,-13.5486172877669,
114.947929919244)) ;
#184121=CARTESIAN_POINT('Ctrl Pts',(-17.5571682124288,-13.8299622964239,
115.020863384168)) ;
#184122=CARTESIAN_POINT('Ctrl Pts',(-17.5791308719583,-13.8016053515907,
115.087758099343)) ;
#184123=CARTESIAN_POINT('Ctrl Pts',(-17.5053270413127,-13.8016054516698,
115.111989179937)) ;
#184124=CARTESIAN_POINT('Ctrl Pts',(-17.4315232106671,-13.8016055517489,
115.136220260531)) ;
#184125=CARTESIAN_POINT('Ctrl Pts',(-17.4095605511376,-13.8299624965821,
115.069325545356)) ;
#184126=CARTESIAN_POINT('Ctrl Pts',(-17.3875978916081,-13.8583194414153,
115.002430830181)) ;
#184127=CARTESIAN_POINT('Ctrl Pts',(-17.4614017222537,-13.8583193413362,
114.978199749587)) ;
#184128=CARTESIAN_POINT('Ctrl Pts',(-17.5352055528993,-13.8583192412571,
114.953968668993)) ;
#184129=CARTESIAN_POINT('Ctrl Pts',(-17.5571682124288,-13.8299622964239,
115.020863384168)) ;
#184130=CARTESIAN_POINT('Ctrl Pts',(-17.5919536420937,-14.082140489746,
115.162256577588)) ;
#184131=CARTESIAN_POINT('Ctrl Pts',(-17.6107868349062,-14.0361354675862,
115.219619442075)) ;
#184132=CARTESIAN_POINT('Ctrl Pts',(-17.5369830121559,-14.0361355534221,
115.243850546717)) ;
#184133=CARTESIAN_POINT('Ctrl Pts',(-17.4631791894057,-14.0361356392581,
115.268081651359)) ;
#184134=CARTESIAN_POINT('Ctrl Pts',(-17.4443459965932,-14.0821406614179,
115.210718786872)) ;
#184135=CARTESIAN_POINT('Ctrl Pts',(-17.4255128037808,-14.1281456835778,
115.153355922385)) ;
#184136=CARTESIAN_POINT('Ctrl Pts',(-17.499316626531,-14.1281455977418,
115.129124817743)) ;
#184137=CARTESIAN_POINT('Ctrl Pts',(-17.5731204492813,-14.1281455119059,
115.104893713101)) ;
#184138=CARTESIAN_POINT('Ctrl Pts',(-17.5919536420937,-14.082140489746,
115.162256577588)) ;
#184139=CARTESIAN_POINT('Ctrl Pts',(-17.6460547424978,-14.2871395255682,
115.362533542529)) ;
#184140=CARTESIAN_POINT('Ctrl Pts',(-17.6604043679569,-14.2267539066878,
115.406240184295)) ;
#184141=CARTESIAN_POINT('Ctrl Pts',(-17.5866005513895,-14.2267539712464,
115.430471307769)) ;
#184142=CARTESIAN_POINT('Ctrl Pts',(-17.5127967348221,-14.2267540358049,
115.454702431244)) ;
#184143=CARTESIAN_POINT('Ctrl Pts',(-17.498447109363,-14.2871396546853,
115.410995789478)) ;
#184144=CARTESIAN_POINT('Ctrl Pts',(-17.4840974839038,-14.3475252735657,
115.367289147712)) ;
#184145=CARTESIAN_POINT('Ctrl Pts',(-17.5579013004713,-14.3475252090071,
115.343058024237)) ;
#184146=CARTESIAN_POINT('Ctrl Pts',(-17.6317051170386,-14.3475251444486,
115.318826900763)) ;
#184147=CARTESIAN_POINT('Ctrl Pts',(-17.6460547424978,-14.2871395255682,
115.362533542529)) ;
#184148=CARTESIAN_POINT('Ctrl Pts',(-17.7149985645736,-14.4298488440199,
115.608097682744)) ;
#184149=CARTESIAN_POINT('Ctrl Pts',(-17.7238201732498,-14.3594095209829,
115.634966877378)) ;
#184150=CARTESIAN_POINT('Ctrl Pts',(-17.6500163603788,-14.3594095593736,
115.659198012111)) ;
#184151=CARTESIAN_POINT('Ctrl Pts',(-17.5762125475078,-14.3594095977643,
115.683429146844)) ;
#184152=CARTESIAN_POINT('Ctrl Pts',(-17.5673909388317,-14.4298489208013,
115.65655995221)) ;
#184153=CARTESIAN_POINT('Ctrl Pts',(-17.5585693301555,-14.5002882438384,
115.629690757576)) ;
#184154=CARTESIAN_POINT('Ctrl Pts',(-17.6323731430264,-14.5002882054477,
115.605459622843)) ;
#184155=CARTESIAN_POINT('Ctrl Pts',(-17.7061769558974,-14.500288167057,
115.58122848811)) ;
#184156=CARTESIAN_POINT('Ctrl Pts',(-17.7149985645736,-14.4298488440199,
115.608097682744)) ;
#184157=CARTESIAN_POINT('Ctrl Pts',(-17.7923224785126,-14.4994383097765,
115.878923588417)) ;
#184158=CARTESIAN_POINT('Ctrl Pts',(-17.7950280138778,-14.4240356160354,
115.887164210622)) ;
#184159=CARTESIAN_POINT('Ctrl Pts',(-17.7212242022659,-14.4240356268717,
115.91139534919)) ;
#184160=CARTESIAN_POINT('Ctrl Pts',(-17.6474203906539,-14.424035637708,
115.935626487757)) ;
#184161=CARTESIAN_POINT('Ctrl Pts',(-17.6447148552887,-14.4994383314491,
115.927385865553)) ;
#184162=CARTESIAN_POINT('Ctrl Pts',(-17.6420093199235,-14.5748410251902,
115.919145243348)) ;
#184163=CARTESIAN_POINT('Ctrl Pts',(-17.7158131315355,-14.5748410143539,
115.89491410478)) ;
#184164=CARTESIAN_POINT('Ctrl Pts',(-17.7896169431474,-14.5748410035177,
115.870682966212)) ;
#184165=CARTESIAN_POINT('Ctrl Pts',(-17.7923224785126,-14.4994383097765,
115.878923588417)) ;
#184166=CARTESIAN_POINT('Ctrl Pts',(-17.8726588843966,-14.4922423916848,
116.159099968041)) ;
#184167=CARTESIAN_POINT('Ctrl Pts',(-17.8690253884429,-14.4172290917828,
116.148032923727)) ;
#184168=CARTESIAN_POINT('Ctrl Pts',(-17.7952215753068,-14.4172290756449,
116.172264057653)) ;
#184169=CARTESIAN_POINT('Ctrl Pts',(-17.7214177621707,-14.417229059507,
116.196495191578)) ;
#184170=CARTESIAN_POINT('Ctrl Pts',(-17.7250512581244,-14.492242359409,
116.207562235892)) ;
#184171=CARTESIAN_POINT('Ctrl Pts',(-17.7286847540781,-14.567255659311,
116.218629280206)) ;
#184172=CARTESIAN_POINT('Ctrl Pts',(-17.8024885672142,-14.5672556754489,
116.194398146281)) ;
#184173=CARTESIAN_POINT('Ctrl Pts',(-17.8762923803503,-14.5672556915868,
116.170167012355)) ;
#184174=CARTESIAN_POINT('Ctrl Pts',(-17.8726588843966,-14.4922423916848,
116.159099968041)) ;
#184175=CARTESIAN_POINT('Ctrl Pts',(-17.9492605892441,-14.4074859363464,
116.427972082509)) ;
#184176=CARTESIAN_POINT('Ctrl Pts',(-17.9395377455059,-14.3382771247353,
116.398357867468)) ;
#184177=CARTESIAN_POINT('Ctrl Pts',(-17.8657339283016,-14.3382770857767,
116.422588989002)) ;
#184178=CARTESIAN_POINT('Ctrl Pts',(-17.7919301110973,-14.3382770468181,
116.446820110537)) ;
#184179=CARTESIAN_POINT('Ctrl Pts',(-17.8016529548354,-14.4074858584293,
116.476434325578)) ;
#184180=CARTESIAN_POINT('Ctrl Pts',(-17.8113757985735,-14.4766946700404,
116.506048540618)) ;
#184181=CARTESIAN_POINT('Ctrl Pts',(-17.8851796157779,-14.476694708999,
116.481817419084)) ;
#184182=CARTESIAN_POINT('Ctrl Pts',(-17.9589834329822,-14.4766947479576,
116.45758629755)) ;
#184183=CARTESIAN_POINT('Ctrl Pts',(-17.9492605892441,-14.4074859363464,
116.427972082509)) ;
#184184=CARTESIAN_POINT('Ctrl Pts',(-18.0153695983152,-14.2527213410347,
116.664674816876)) ;
#184185=CARTESIAN_POINT('Ctrl Pts',(-18.00028515088,-14.1942140636659,116.618730022167)) ;
#184186=CARTESIAN_POINT('Ctrl Pts',(-17.9264813282525,-14.1942140071928,
116.642961127183)) ;
#184187=CARTESIAN_POINT('Ctrl Pts',(-17.8526775056251,-14.1942139507198,
116.6671922322)) ;
#184188=CARTESIAN_POINT('Ctrl Pts',(-17.8677619530604,-14.2527212280886,
116.713137026909)) ;
#184189=CARTESIAN_POINT('Ctrl Pts',(-17.8828464004957,-14.3112285054574,
116.759081821618)) ;
#184190=CARTESIAN_POINT('Ctrl Pts',(-17.9566502231231,-14.3112285619304,
116.734850716602)) ;
#184191=CARTESIAN_POINT('Ctrl Pts',(-18.0304540457505,-14.3112286184035,
116.710619611585)) ;
#184192=CARTESIAN_POINT('Ctrl Pts',(-18.0153695983152,-14.2527213410347,
116.664674816876)) ;
#184193=CARTESIAN_POINT('Ctrl Pts',(-18.0662184898938,-14.0372448891262,
116.855097648155)) ;
#184194=CARTESIAN_POINT('Ctrl Pts',(-18.0468255144096,-13.9936933807782,
116.796029772331)) ;
#184195=CARTESIAN_POINT('Ctrl Pts',(-17.9730216850138,-13.993693314701,
116.820260856732)) ;
#184196=CARTESIAN_POINT('Ctrl Pts',(-17.8992178556179,-13.9936932486239,
116.844491941133)) ;
#184197=CARTESIAN_POINT('Ctrl Pts',(-17.9186108311021,-14.0372447569719,
116.903559816957)) ;
#184198=CARTESIAN_POINT('Ctrl Pts',(-17.9380038065863,-14.08079626532,116.96262769278)) ;
#184199=CARTESIAN_POINT('Ctrl Pts',(-18.0118076359821,-14.0807963313971,
116.938396608379)) ;
#184200=CARTESIAN_POINT('Ctrl Pts',(-18.085611465378,-14.0807963974743,
116.914165523978)) ;
#184201=CARTESIAN_POINT('Ctrl Pts',(-18.0662184898938,-14.0372448891262,
116.855097648155)) ;
#184202=CARTESIAN_POINT('Ctrl Pts',(-18.0969238178348,-13.7782273369584,
116.984027397216)) ;
#184203=CARTESIAN_POINT('Ctrl Pts',(-18.0746250853086,-13.7526945200312,
116.91610905442)) ;
#184204=CARTESIAN_POINT('Ctrl Pts',(-18.0008212491944,-13.75269445107,116.940340118358)) ;
#184205=CARTESIAN_POINT('Ctrl Pts',(-17.9270174130802,-13.7526943821088,
116.964571182296)) ;
#184206=CARTESIAN_POINT('Ctrl Pts',(-17.9493161456064,-13.778227199036,
117.032489525092)) ;
#184207=CARTESIAN_POINT('Ctrl Pts',(-17.9716148781326,-13.8037600159632,
117.100407867887)) ;
#184208=CARTESIAN_POINT('Ctrl Pts',(-18.0454187142468,-13.8037600849244,
117.076176803949)) ;
#184209=CARTESIAN_POINT('Ctrl Pts',(-18.119222550361,-13.8037601538856,
117.051945740011)) ;
#184210=CARTESIAN_POINT('Ctrl Pts',(-18.0969238178348,-13.7782273369584,
116.984027397216)) ;
#184211=CARTESIAN_POINT('Ctrl Pts',(-18.1047200617367,-13.4921296981973,
117.043351119596)) ;
#184212=CARTESIAN_POINT('Ctrl Pts',(-18.0811069226382,-13.4865334475081,
116.971429306637)) ;
#184213=CARTESIAN_POINT('Ctrl Pts',(-18.0073030803503,-13.4865333838988,
116.995660351771)) ;
#184214=CARTESIAN_POINT('Ctrl Pts',(-17.9334992380623,-13.4865333202894,
117.019891396905)) ;
#184215=CARTESIAN_POINT('Ctrl Pts',(-17.9571123771608,-13.4921295709785,
117.091813209864)) ;
#184216=CARTESIAN_POINT('Ctrl Pts',(-17.9807255162593,-13.4977258216677,
117.163735022823)) ;
#184217=CARTESIAN_POINT('Ctrl Pts',(-18.0545293585472,-13.497725885277,
117.139503977689)) ;
#184218=CARTESIAN_POINT('Ctrl Pts',(-18.1283332008352,-13.4977259488864,
117.115272932555)) ;
#184219=CARTESIAN_POINT('Ctrl Pts',(-18.1047200617367,-13.4921296981973,
117.043351119596)) ;
#184220=CARTESIAN_POINT('Ctrl Pts',(-18.0883120122329,-13.2025980491625,
117.028710821866)) ;
#184221=CARTESIAN_POINT('Ctrl Pts',(-18.0650776141143,-13.2172086619386,
116.957942592962)) ;
#184222=CARTESIAN_POINT('Ctrl Pts',(-17.9912737669891,-13.2172086067816,
116.982173623362)) ;
#184223=CARTESIAN_POINT('Ctrl Pts',(-17.9174699198639,-13.2172085516246,
117.006404653763)) ;
#184224=CARTESIAN_POINT('Ctrl Pts',(-17.9407043179825,-13.2025979388484,
117.077172882667)) ;
#184225=CARTESIAN_POINT('Ctrl Pts',(-17.9639387161011,-13.1879873260723,
117.14794111157)) ;
#184226=CARTESIAN_POINT('Ctrl Pts',(-18.0377425632263,-13.1879873812294,
117.12371008117)) ;
#184227=CARTESIAN_POINT('Ctrl Pts',(-18.1115464103515,-13.1879874363864,
117.09947905077)) ;
#184228=CARTESIAN_POINT('Ctrl Pts',(-18.0883120122329,-13.2025980491625,
117.028710821866)) ;
#184229=CARTESIAN_POINT('Ctrl Pts',(-18.0479516493469,-12.9267373644591,
116.941340583606)) ;
#184230=CARTESIAN_POINT('Ctrl Pts',(-18.0267640646557,-12.960631185249,
116.876806618336)) ;
#184231=CARTESIAN_POINT('Ctrl Pts',(-17.9529602144129,-12.9606311438607,
116.901037639241)) ;
#184232=CARTESIAN_POINT('Ctrl Pts',(-17.8791563641702,-12.9606311024724,
116.925268660146)) ;
#184233=CARTESIAN_POINT('Ctrl Pts',(-17.9003439488613,-12.9267372816824,
116.989802625416)) ;
#184234=CARTESIAN_POINT('Ctrl Pts',(-17.9215315335525,-12.8928434608925,
117.054336590686)) ;
#184235=CARTESIAN_POINT('Ctrl Pts',(-17.9953353837953,-12.8928435022808,
117.030105569781)) ;
#184236=CARTESIAN_POINT('Ctrl Pts',(-18.0691392340381,-12.8928435436691,
117.005874548876)) ;
#184237=CARTESIAN_POINT('Ctrl Pts',(-18.0479516493469,-12.9267373644591,
116.941340583606)) ;
#184238=CARTESIAN_POINT('Ctrl Pts',(-17.9859929653459,-12.6871394629104,
116.788053385825)) ;
#184239=CARTESIAN_POINT('Ctrl Pts',(-17.9683662277458,-12.7378139602179,
116.734365186415)) ;
#184240=CARTESIAN_POINT('Ctrl Pts',(-17.894562376113,-12.7378139322017,
116.758596203086)) ;
#184241=CARTESIAN_POINT('Ctrl Pts',(-17.8207585244803,-12.7378139041855,
116.782827219757)) ;
#184242=CARTESIAN_POINT('Ctrl Pts',(-17.8383852620805,-12.687139406878,
116.836515419167)) ;
#184243=CARTESIAN_POINT('Ctrl Pts',(-17.8560119996807,-12.6364649095704,
116.890203618577)) ;
#184244=CARTESIAN_POINT('Ctrl Pts',(-17.9298158513134,-12.6364649375867,
116.865972601906)) ;
#184245=CARTESIAN_POINT('Ctrl Pts',(-18.0036197029461,-12.6364649656029,
116.841741585235)) ;
#184246=CARTESIAN_POINT('Ctrl Pts',(-17.9859929653459,-12.6871394629104,
116.788053385825)) ;
#184247=CARTESIAN_POINT('Ctrl Pts',(-17.906099050151,-12.4995507390681,
116.580148460195)) ;
#184248=CARTESIAN_POINT('Ctrl Pts',(-17.8932906510401,-12.5633999915825,
116.541136142548)) ;
#184249=CARTESIAN_POINT('Ctrl Pts',(-17.8194867995482,-12.5633999761432,
116.565367159648)) ;
#184250=CARTESIAN_POINT('Ctrl Pts',(-17.7456829480562,-12.5633999607039,
116.589598176748)) ;
#184251=CARTESIAN_POINT('Ctrl Pts',(-17.7584913471671,-12.4995507081895,
116.628610494395)) ;
#184252=CARTESIAN_POINT('Ctrl Pts',(-17.7712997462779,-12.4357014556752,
116.667622812042)) ;
#184253=CARTESIAN_POINT('Ctrl Pts',(-17.8451035977699,-12.4357014711144,
116.643391794942)) ;
#184254=CARTESIAN_POINT('Ctrl Pts',(-17.9189074492618,-12.4357014865537,
116.619160777842)) ;
#184255=CARTESIAN_POINT('Ctrl Pts',(-17.906099050151,-12.4995507390681,
116.580148460195)) ;
#184256=CARTESIAN_POINT('Ctrl Pts',(-17.8126198276704,-12.3773999719713,
116.331056854077)) ;
#184257=CARTESIAN_POINT('Ctrl Pts',(-17.8055817580206,-12.4498755259628,
116.309620029115)) ;
#184258=CARTESIAN_POINT('Ctrl Pts',(-17.7317779084013,-12.4498755206207,
116.333851051918)) ;
#184259=CARTESIAN_POINT('Ctrl Pts',(-17.657974058782,-12.4498755152786,
116.358082074722)) ;
#184260=CARTESIAN_POINT('Ctrl Pts',(-17.6650121284318,-12.377399961287,
116.379518899685)) ;
#184261=CARTESIAN_POINT('Ctrl Pts',(-17.6720501980816,-12.3049244072955,
116.400955724648)) ;
#184262=CARTESIAN_POINT('Ctrl Pts',(-17.7458540477008,-12.3049244126376,
116.376724701844)) ;
#184263=CARTESIAN_POINT('Ctrl Pts',(-17.8196578973201,-12.3049244179797,
116.35249367904)) ;
#184264=CARTESIAN_POINT('Ctrl Pts',(-17.8126198276704,-12.3773999719713,
116.331056854077)) ;
#184265=CARTESIAN_POINT('Ctrl Pts',(-17.7129634648674,-12.3305982965088,
116.062809081793)) ;
#184266=CARTESIAN_POINT('Ctrl Pts',(-17.7121429577396,-12.4064507655152,
116.060309949185)) ;
#184267=CARTESIAN_POINT('Ctrl Pts',(-17.6383391097371,-12.4064507656023,
116.084540976913)) ;
#184268=CARTESIAN_POINT('Ctrl Pts',(-17.5645352617346,-12.4064507656893,
116.108772004641)) ;
#184269=CARTESIAN_POINT('Ctrl Pts',(-17.5653557688624,-12.3305982966829,
116.111271137249)) ;
#184270=CARTESIAN_POINT('Ctrl Pts',(-17.5661762759903,-12.2547458276765,
116.113770269857)) ;
#184271=CARTESIAN_POINT('Ctrl Pts',(-17.6399801239928,-12.2547458275895,
116.089539242129)) ;
#184272=CARTESIAN_POINT('Ctrl Pts',(-17.7137839719953,-12.2547458275024,
116.0653082144)) ;
#184273=CARTESIAN_POINT('Ctrl Pts',(-17.7129634648674,-12.3305982965088,
116.062809081793)) ;
#184274=CARTESIAN_POINT('Ctrl Pts',(-17.6121496035904,-12.3609522062499,
115.791201386233)) ;
#184275=CARTESIAN_POINT('Ctrl Pts',(-17.617633502554,-12.4347996190351,
115.807904457495)) ;
#184276=CARTESIAN_POINT('Ctrl Pts',(-17.5438296567185,-12.4347996215548,
115.832135491824)) ;
#184277=CARTESIAN_POINT('Ctrl Pts',(-17.4700258108831,-12.4347996240744,
115.856366526153)) ;
#184278=CARTESIAN_POINT('Ctrl Pts',(-17.4645419119195,-12.3609522112891,
115.839663454891)) ;
#184279=CARTESIAN_POINT('Ctrl Pts',(-17.4590580129559,-12.2871047985038,
115.822960383629)) ;
#184280=CARTESIAN_POINT('Ctrl Pts',(-17.5328618587913,-12.2871047959842,
115.7987293493)) ;
#184281=CARTESIAN_POINT('Ctrl Pts',(-17.6066657046268,-12.2871047934646,
115.774498314971)) ;
#184282=CARTESIAN_POINT('Ctrl Pts',(-17.6121496035904,-12.3609522062499,
115.791201386233)) ;
#184283=CARTESIAN_POINT('Ctrl Pts',(-17.5168160586638,-12.4676416333475,
115.536394386331)) ;
#184284=CARTESIAN_POINT('Ctrl Pts',(-17.5282291491706,-12.5341505224267,
115.571156818475)) ;
#184285=CARTESIAN_POINT('Ctrl Pts',(-17.4544253052102,-12.5341505238971,
115.595387858515)) ;
#184286=CARTESIAN_POINT('Ctrl Pts',(-17.3806214612499,-12.5341505253675,
115.619618898555)) ;
#184287=CARTESIAN_POINT('Ctrl Pts',(-17.3692083707431,-12.4676416362883,
115.584856466411)) ;
#184288=CARTESIAN_POINT('Ctrl Pts',(-17.3577952802364,-12.4011327472091,
115.550094034267)) ;
#184289=CARTESIAN_POINT('Ctrl Pts',(-17.4315991241967,-12.4011327457387,
115.525862994227)) ;
#184290=CARTESIAN_POINT('Ctrl Pts',(-17.5054029681571,-12.4011327442682,
115.501631954187)) ;
#184291=CARTESIAN_POINT('Ctrl Pts',(-17.5168160586638,-12.4676416333475,
115.536394386331)) ;
#184292=CARTESIAN_POINT('Ctrl Pts',(-17.4336916866709,-12.6420295507419,
115.31863885574)) ;
#184293=CARTESIAN_POINT('Ctrl Pts',(-17.450193039918,-12.6964607838734,
115.368899315271)) ;
#184294=CARTESIAN_POINT('Ctrl Pts',(-17.3763891968336,-12.6964607831673,
115.393130357979)) ;
#184295=CARTESIAN_POINT('Ctrl Pts',(-17.3025853537493,-12.6964607824612,
115.417361400687)) ;
#184296=CARTESIAN_POINT('Ctrl Pts',(-17.2860840005021,-12.6420295493297,
115.367100941156)) ;
#184297=CARTESIAN_POINT('Ctrl Pts',(-17.269582647255,-12.5875983161982,
115.316840481625)) ;
#184298=CARTESIAN_POINT('Ctrl Pts',(-17.3433864903394,-12.5875983169043,
115.292609438917)) ;
#184299=CARTESIAN_POINT('Ctrl Pts',(-17.4171903334238,-12.5875983176104,
115.268378396209)) ;
#184300=CARTESIAN_POINT('Ctrl Pts',(-17.4336916866709,-12.6420295507419,
115.31863885574)) ;
#184301=CARTESIAN_POINT('Ctrl Pts',(-17.3676172772984,-12.8715204701867,
115.152776949811)) ;
#184302=CARTESIAN_POINT('Ctrl Pts',(-17.3880246049082,-12.9100077875802,
115.21493437706)) ;
#184303=CARTESIAN_POINT('Ctrl Pts',(-17.3142207620158,-12.9100077849432,
115.239165420353)) ;
#184304=CARTESIAN_POINT('Ctrl Pts',(-17.2404169191235,-12.9100077823063,
115.263396463646)) ;
#184305=CARTESIAN_POINT('Ctrl Pts',(-17.2200095915137,-12.8715204649127,
115.201239036397)) ;
#184306=CARTESIAN_POINT('Ctrl Pts',(-17.1996022639038,-12.8330331475192,
115.139081609148)) ;
#184307=CARTESIAN_POINT('Ctrl Pts',(-17.2734061067962,-12.8330331501562,
115.114850565855)) ;
#184308=CARTESIAN_POINT('Ctrl Pts',(-17.3472099496886,-12.8330331527932,
115.090619522562)) ;
#184309=CARTESIAN_POINT('Ctrl Pts',(-17.3676172772984,-12.8715204701867,
115.152776949811)) ;
#184310=CARTESIAN_POINT('Ctrl Pts',(-17.3223473460117,-13.1406452081899,
115.050364660564)) ;
#184311=CARTESIAN_POINT('Ctrl Pts',(-17.3452119870668,-13.1603966221908,
115.120006668083)) ;
#184312=CARTESIAN_POINT('Ctrl Pts',(-17.2714081438692,-13.1603966190533,
115.144237710446)) ;
#184313=CARTESIAN_POINT('Ctrl Pts',(-17.1976043006715,-13.1603966159158,
115.168468752809)) ;
#184314=CARTESIAN_POINT('Ctrl Pts',(-17.1747396596163,-13.1406452019148,
115.09882674529)) ;
#184315=CARTESIAN_POINT('Ctrl Pts',(-17.1518750185612,-13.1208937879139,
115.02918473777)) ;
#184316=CARTESIAN_POINT('Ctrl Pts',(-17.2256788617588,-13.1208937910514,
115.004953695407)) ;
#184317=CARTESIAN_POINT('Ctrl Pts',(-17.2994827049565,-13.1208937941889,
114.980722653044)) ;
#184318=CARTESIAN_POINT('Ctrl Pts',(-17.3223473460117,-13.1406452081899,
115.050364660564)) ;
#184319=CARTESIAN_POINT('Ctrl Pts',(-17.3006206315397,-13.4310927688211,
115.019830516096)) ;
#184320=CARTESIAN_POINT('Ctrl Pts',(-17.3242986066671,-13.4305915609801,
115.091949807911)) ;
#184321=CARTESIAN_POINT('Ctrl Pts',(-17.2504947631562,-13.4305915607747,
115.11618084932)) ;
#184322=CARTESIAN_POINT('Ctrl Pts',(-17.1766909196454,-13.4305915605693,
115.140411890729)) ;
#184323=CARTESIAN_POINT('Ctrl Pts',(-17.153012944518,-13.4310927684104,
115.068292598915)) ;
#184324=CARTESIAN_POINT('Ctrl Pts',(-17.1293349693906,-13.4315939762514,
114.9961733071)) ;
#184325=CARTESIAN_POINT('Ctrl Pts',(-17.2031388129014,-13.4315939764568,
114.971942265691)) ;
#184326=CARTESIAN_POINT('Ctrl Pts',(-17.2769426564123,-13.4315939766622,
114.947711224282)) ;
#184327=CARTESIAN_POINT('Ctrl Pts',(-17.3006206315397,-13.4310927688211,
115.019830516096)) ;
#184328=CARTESIAN_POINT('Ctrl Pts',(-17.3033372707699,-13.7181744540682,
115.063445924555)) ;
#184329=CARTESIAN_POINT('Ctrl Pts',(-17.3261287288481,-13.6976269857138,
115.132865028405)) ;
#184330=CARTESIAN_POINT('Ctrl Pts',(-17.2523248856312,-13.6976269892172,
115.157096070709)) ;
#184331=CARTESIAN_POINT('Ctrl Pts',(-17.1785210424142,-13.6976269927207,
115.181327113013)) ;
#184332=CARTESIAN_POINT('Ctrl Pts',(-17.155729584336,-13.718174461075,115.111908009164)) ;
#184333=CARTESIAN_POINT('Ctrl Pts',(-17.1329381262578,-13.7387219294293,
115.042488905314)) ;
#184334=CARTESIAN_POINT('Ctrl Pts',(-17.2067419694747,-13.7387219259259,
115.01825786301)) ;
#184335=CARTESIAN_POINT('Ctrl Pts',(-17.2805458126917,-13.7387219224225,
114.994026820705)) ;
#184336=CARTESIAN_POINT('Ctrl Pts',(-17.3033372707699,-13.7181744540682,
115.063445924555)) ;
#184337=CARTESIAN_POINT('Ctrl Pts',(-17.3292593238166,-13.9844854804917,
115.177817625919)) ;
#184338=CARTESIAN_POINT('Ctrl Pts',(-17.349541065467,-13.9453130684822,
115.239592538371)) ;
#184339=CARTESIAN_POINT('Ctrl Pts',(-17.2757372233181,-13.9453130761656,
115.263823583929)) ;
#184340=CARTESIAN_POINT('Ctrl Pts',(-17.2019333811692,-13.945313083849,
115.288054629486)) ;
#184341=CARTESIAN_POINT('Ctrl Pts',(-17.1816516395188,-13.9844854958585,
115.226279717033)) ;
#184342=CARTESIAN_POINT('Ctrl Pts',(-17.1613698978684,-14.023657907868,
115.164504804581)) ;
#184343=CARTESIAN_POINT('Ctrl Pts',(-17.2351737400173,-14.0236579001846,
115.140273759023)) ;
#184344=CARTESIAN_POINT('Ctrl Pts',(-17.3089775821662,-14.0236578925012,
115.116042713466)) ;
#184345=CARTESIAN_POINT('Ctrl Pts',(-17.3292593238166,-13.9844854804917,
115.177817625919)) ;
#184346=CARTESIAN_POINT('Ctrl Pts',(-17.3760632823759,-14.2108138750807,
115.35588254334)) ;
#184347=CARTESIAN_POINT('Ctrl Pts',(-17.3923717224603,-14.1557813405772,
115.405555420177)) ;
#184348=CARTESIAN_POINT('Ctrl Pts',(-17.3185678824734,-14.1557813517834,
115.42978647232)) ;
#184349=CARTESIAN_POINT('Ctrl Pts',(-17.2447640424865,-14.1557813629896,
115.454017524462)) ;
#184350=CARTESIAN_POINT('Ctrl Pts',(-17.2284556024021,-14.2108138974931,
115.404344647625)) ;
#184351=CARTESIAN_POINT('Ctrl Pts',(-17.2121471623177,-14.2658464319965,
115.354671770788)) ;
#184352=CARTESIAN_POINT('Ctrl Pts',(-17.2859510023046,-14.2658464207903,
115.330440718646)) ;
#184353=CARTESIAN_POINT('Ctrl Pts',(-17.3597548422915,-14.2658464095841,
115.306209666503)) ;
#184354=CARTESIAN_POINT('Ctrl Pts',(-17.3760632823759,-14.2108138750807,
115.35588254334)) ;
#184355=CARTESIAN_POINT('Ctrl Pts',(-17.4394638024811,-14.3800184665147,
115.584449969473)) ;
#184356=CARTESIAN_POINT('Ctrl Pts',(-17.4506353318876,-14.313091902712,
115.618476645077)) ;
#184357=CARTESIAN_POINT('Ctrl Pts',(-17.37683149478,-14.3130919141767,115.64270770599)) ;
#184358=CARTESIAN_POINT('Ctrl Pts',(-17.3030276576725,-14.3130919256413,
115.666938766902)) ;
#184359=CARTESIAN_POINT('Ctrl Pts',(-17.291856128266,-14.3800184894439,
115.632912091298)) ;
#184360=CARTESIAN_POINT('Ctrl Pts',(-17.2806845988595,-14.4469450532465,
115.598885415694)) ;
#184361=CARTESIAN_POINT('Ctrl Pts',(-17.3544884359671,-14.4469450417819,
115.574654354782)) ;
#184362=CARTESIAN_POINT('Ctrl Pts',(-17.4282922730746,-14.4469450303173,
115.55042329387)) ;
#184363=CARTESIAN_POINT('Ctrl Pts',(-17.4394638024811,-14.3800184665147,
115.584449969473)) ;
#184364=CARTESIAN_POINT('Ctrl Pts',(-17.5142370059596,-14.4803359496639,
115.847668381267)) ;
#184365=CARTESIAN_POINT('Ctrl Pts',(-17.5194699341939,-14.4063082157353,
115.863607035731)) ;
#184366=CARTESIAN_POINT('Ctrl Pts',(-17.4456661003206,-14.4063082232175,
115.887838106494)) ;
#184367=CARTESIAN_POINT('Ctrl Pts',(-17.3718622664474,-14.4063082306997,
115.912069177258)) ;
#184368=CARTESIAN_POINT('Ctrl Pts',(-17.3666293382131,-14.4803359646283,
115.896130522795)) ;
#184369=CARTESIAN_POINT('Ctrl Pts',(-17.3613964099789,-14.554363698557,
115.880191868331)) ;
#184370=CARTESIAN_POINT('Ctrl Pts',(-17.4352002438521,-14.5543636910748,
115.855960797567)) ;
#184371=CARTESIAN_POINT('Ctrl Pts',(-17.5090040777254,-14.5543636835926,
115.831729726804)) ;
#184372=CARTESIAN_POINT('Ctrl Pts',(-17.5142370059596,-14.4803359496639,
115.847668381267)) ;
#184373=CARTESIAN_POINT('Ctrl Pts',(-17.5941239798052,-14.5045829128103,
116.126404146317)) ;
#184374=CARTESIAN_POINT('Ctrl Pts',(-17.5930539491612,-14.4287553960091,
116.123145004861)) ;
#184375=CARTESIAN_POINT('Ctrl Pts',(-17.5192501180761,-14.4287553947463,
116.147376084117)) ;
#184376=CARTESIAN_POINT('Ctrl Pts',(-17.4454462869911,-14.4287553934836,
116.171607163373)) ;
#184377=CARTESIAN_POINT('Ctrl Pts',(-17.446516317635,-14.5045829102848,
116.174866304829)) ;
#184378=CARTESIAN_POINT('Ctrl Pts',(-17.447586348279,-14.580410427086,116.178125446286)) ;
#184379=CARTESIAN_POINT('Ctrl Pts',(-17.5213901793641,-14.5804104283487,
116.15389436703)) ;
#184380=CARTESIAN_POINT('Ctrl Pts',(-17.5951940104491,-14.5804104296115,
116.129663287774)) ;
#184381=CARTESIAN_POINT('Ctrl Pts',(-17.5941239798052,-14.5045829128103,
116.126404146317)) ;
#184382=CARTESIAN_POINT('Ctrl Pts',(-17.6729871089332,-14.4510580252238,
116.402111327135)) ;
#184383=CARTESIAN_POINT('Ctrl Pts',(-17.665674706909,-14.3788579006376,
116.379838929482)) ;
#184384=CARTESIAN_POINT('Ctrl Pts',(-17.5918708779827,-14.3788578861591,
116.404070015313)) ;
#184385=CARTESIAN_POINT('Ctrl Pts',(-17.5180670490564,-14.3788578716805,
116.428301101144)) ;
#184386=CARTESIAN_POINT('Ctrl Pts',(-17.5253794510806,-14.4510579962666,
116.450573498798)) ;
#184387=CARTESIAN_POINT('Ctrl Pts',(-17.5326918531049,-14.5232581208527,
116.472845896452)) ;
#184388=CARTESIAN_POINT('Ctrl Pts',(-17.6064956820311,-14.5232581353313,
116.448614810621)) ;
#184389=CARTESIAN_POINT('Ctrl Pts',(-17.6802995109574,-14.5232581498099,
116.424383724789)) ;
#184390=CARTESIAN_POINT('Ctrl Pts',(-17.6729871089332,-14.4510580252238,
116.402111327135)) ;
#184391=CARTESIAN_POINT('Ctrl Pts',(-17.7442108074172,-14.3231627979094,
116.654564949859)) ;
#184392=CARTESIAN_POINT('Ctrl Pts',(-17.7311801239932,-14.2597876685306,
116.614875589526)) ;
#184393=CARTESIAN_POINT('Ctrl Pts',(-17.6573762957046,-14.2597876370506,
116.639106677299)) ;
#184394=CARTESIAN_POINT('Ctrl Pts',(-17.583572467416,-14.2597876055706,
116.663337765073)) ;
#184395=CARTESIAN_POINT('Ctrl Pts',(-17.59660315084,-14.3231627349493,116.703027125406)) ;
#184396=CARTESIAN_POINT('Ctrl Pts',(-17.6096338342639,-14.386537864328,
116.74271648574)) ;
#184397=CARTESIAN_POINT('Ctrl Pts',(-17.6834376625525,-14.3865378958081,
116.718485397966)) ;
#184398=CARTESIAN_POINT('Ctrl Pts',(-17.7572414908411,-14.3865379272881,
116.694254310193)) ;
#184399=CARTESIAN_POINT('Ctrl Pts',(-17.7442108074172,-14.3231627979094,
116.654564949859)) ;
#184400=CARTESIAN_POINT('Ctrl Pts',(-17.8017294897933,-14.1311846385056,
116.865136329538)) ;
#184401=CARTESIAN_POINT('Ctrl Pts',(-17.7839321083557,-14.0811216324566,
116.810928376012)) ;
#184402=CARTESIAN_POINT('Ctrl Pts',(-17.7101282784815,-14.0811215835067,
116.835159458956)) ;
#184403=CARTESIAN_POINT('Ctrl Pts',(-17.6363244486073,-14.0811215345568,
116.8593905419)) ;
#184404=CARTESIAN_POINT('Ctrl Pts',(-17.6541218300448,-14.1311845406059,
116.913598495426)) ;
#184405=CARTESIAN_POINT('Ctrl Pts',(-17.6719192114823,-14.181247546655,
116.967806448952)) ;
#184406=CARTESIAN_POINT('Ctrl Pts',(-17.7457230413565,-14.1812475956048,
116.943575366008)) ;
#184407=CARTESIAN_POINT('Ctrl Pts',(-17.8195268712308,-14.1812476445547,
116.919344283064)) ;
#184408=CARTESIAN_POINT('Ctrl Pts',(-17.8017294897933,-14.1311846385056,
116.865136329538)) ;
#184409=CARTESIAN_POINT('Ctrl Pts',(-17.841097170979,-13.8873682377616,
117.020560844287)) ;
#184410=CARTESIAN_POINT('Ctrl Pts',(-17.8197905237819,-13.8542552865156,
116.955664233311)) ;
#184411=CARTESIAN_POINT('Ctrl Pts',(-17.7459866905101,-13.8542552201397,
116.979895305907)) ;
#184412=CARTESIAN_POINT('Ctrl Pts',(-17.6721828572383,-13.8542551537638,
117.004126378502)) ;
#184413=CARTESIAN_POINT('Ctrl Pts',(-17.6934895044355,-13.8873681050098,
117.069022989479)) ;
#184414=CARTESIAN_POINT('Ctrl Pts',(-17.7147961516327,-13.9204810562558,
117.133919600455)) ;
#184415=CARTESIAN_POINT('Ctrl Pts',(-17.7885999849044,-13.9204811226317,
117.109688527859)) ;
#184416=CARTESIAN_POINT('Ctrl Pts',(-17.8624038181762,-13.9204811890076,
117.085457455263)) ;
#184417=CARTESIAN_POINT('Ctrl Pts',(-17.841097170979,-13.8873682377616,
117.020560844287)) ;
#184418=CARTESIAN_POINT('Ctrl Pts',(-17.858439925497,-13.6103444957185,
117.108831164747)) ;
#184419=CARTESIAN_POINT('Ctrl Pts',(-17.8351581118065,-13.5965245493847,
117.037918515183)) ;
#184420=CARTESIAN_POINT('Ctrl Pts',(-17.7613542730539,-13.5965244695658,
117.062149571085)) ;
#184421=CARTESIAN_POINT('Ctrl Pts',(-17.6875504343013,-13.5965243897469,
117.086380626987)) ;
#184422=CARTESIAN_POINT('Ctrl Pts',(-17.7108322479918,-13.6103443360808,
117.157293276551)) ;
#184423=CARTESIAN_POINT('Ctrl Pts',(-17.7341140616824,-13.6241642824146,
117.228205926115)) ;
#184424=CARTESIAN_POINT('Ctrl Pts',(-17.807917900435,-13.6241643622335,
117.203974870213)) ;
#184425=CARTESIAN_POINT('Ctrl Pts',(-17.8817217391876,-13.6241644420523,
117.179743814311)) ;
#184426=CARTESIAN_POINT('Ctrl Pts',(-17.858439925497,-13.6103444957185,
117.108831164747)) ;
#184427=CARTESIAN_POINT('Ctrl Pts',(-17.8518767191496,-13.3193309051749,
117.12431916614)) ;
#184428=CARTESIAN_POINT('Ctrl Pts',(-17.8282851787465,-13.3258084661624,
117.052463138851)) ;
#184429=CARTESIAN_POINT('Ctrl Pts',(-17.7544813330107,-13.3258083784264,
117.076694173483)) ;
#184430=CARTESIAN_POINT('Ctrl Pts',(-17.680677487275,-13.3258082906904,
117.100925208115)) ;
#184431=CARTESIAN_POINT('Ctrl Pts',(-17.7042690276781,-13.3193307297029,
117.172781235404)) ;
#184432=CARTESIAN_POINT('Ctrl Pts',(-17.7278605680812,-13.3128531687154,
117.244637262693)) ;
#184433=CARTESIAN_POINT('Ctrl Pts',(-17.801664413817,-13.3128532564514,
117.22040622806)) ;
#184434=CARTESIAN_POINT('Ctrl Pts',(-17.8754682595527,-13.3128533441874,
117.196175193428)) ;
#184435=CARTESIAN_POINT('Ctrl Pts',(-17.8518767191496,-13.3193309051749,
117.12431916614)) ;
#184436=CARTESIAN_POINT('Ctrl Pts',(-17.8211064298511,-13.0356124679736,
117.066047429482)) ;
#184437=CARTESIAN_POINT('Ctrl Pts',(-17.7988953105037,-13.0619076839879,
116.998395941887)) ;
#184438=CARTESIAN_POINT('Ctrl Pts',(-17.7250914569277,-13.061907595961,
117.022626952639)) ;
#184439=CARTESIAN_POINT('Ctrl Pts',(-17.6512876033518,-13.061907507934,
117.046857963391)) ;
#184440=CARTESIAN_POINT('Ctrl Pts',(-17.6734987226992,-13.0356122919197,
117.114509450987)) ;
#184441=CARTESIAN_POINT('Ctrl Pts',(-17.6957098420467,-13.0093170759053,
117.182160938582)) ;
#184442=CARTESIAN_POINT('Ctrl Pts',(-17.7695136956227,-13.0093171639322,
117.15792992783)) ;
#184443=CARTESIAN_POINT('Ctrl Pts',(-17.8433175491986,-13.0093172519592,
117.133698917078)) ;
#184444=CARTESIAN_POINT('Ctrl Pts',(-17.8211064298511,-13.0356124679736,
117.066047429482)) ;
#184445=CARTESIAN_POINT('Ctrl Pts',(-17.7676238677098,-12.7792808148317,
116.938592617512)) ;
#184446=CARTESIAN_POINT('Ctrl Pts',(-17.7483808915062,-12.8235105133311,
116.87998161493)) ;
#184447=CARTESIAN_POINT('Ctrl Pts',(-17.6745770300968,-12.8235104331366,
116.904212601823)) ;
#184448=CARTESIAN_POINT('Ctrl Pts',(-17.6007731686875,-12.8235103529421,
116.928443588715)) ;
#184449=CARTESIAN_POINT('Ctrl Pts',(-17.6200161448911,-12.7792806544427,
116.987054591298)) ;
#184450=CARTESIAN_POINT('Ctrl Pts',(-17.6392591210947,-12.7350509559433,
117.045665593881)) ;
#184451=CARTESIAN_POINT('Ctrl Pts',(-17.7130629825041,-12.7350510361378,
117.021434606988)) ;
#184452=CARTESIAN_POINT('Ctrl Pts',(-17.7868668439134,-12.7350511163323,
116.997203620095)) ;
#184453=CARTESIAN_POINT('Ctrl Pts',(-17.7676238677098,-12.7792808148317,
116.938592617512)) ;
#184454=CARTESIAN_POINT('Ctrl Pts',(-17.6943411970397,-12.568318140118,
116.750890389629)) ;
#184455=CARTESIAN_POINT('Ctrl Pts',(-17.6794516619109,-12.6273412297626,
116.705539266054)) ;
#184456=CARTESIAN_POINT('Ctrl Pts',(-17.6056477934581,-12.6273411651946,
116.729770231493)) ;
#184457=CARTESIAN_POINT('Ctrl Pts',(-17.5318439250053,-12.6273411006266,
116.754001196933)) ;
#184458=CARTESIAN_POINT('Ctrl Pts',(-17.5467334601341,-12.568318010982,
116.799352320509)) ;
#184459=CARTESIAN_POINT('Ctrl Pts',(-17.5616229952629,-12.5092949213373,
116.844703444085)) ;
#184460=CARTESIAN_POINT('Ctrl Pts',(-17.6354268637157,-12.5092949859053,
116.820472478645)) ;
#184461=CARTESIAN_POINT('Ctrl Pts',(-17.7092307321685,-12.5092950504733,
116.796241513205)) ;
#184462=CARTESIAN_POINT('Ctrl Pts',(-17.6943411970397,-12.568318140118,
116.750890389629)) ;
#184463=CARTESIAN_POINT('Ctrl Pts',(-17.6058868196778,-12.4185302079718,
116.516953818039)) ;
#184464=CARTESIAN_POINT('Ctrl Pts',(-17.5964167836325,-12.4880976547663,
116.488109614182)) ;
#184465=CARTESIAN_POINT('Ctrl Pts',(-17.5226129098786,-12.4880976127796,
116.512340563475)) ;
#184466=CARTESIAN_POINT('Ctrl Pts',(-17.4488090361247,-12.4880975707929,
116.536571512769)) ;
#184467=CARTESIAN_POINT('Ctrl Pts',(-17.45827907217,-12.4185301239984,116.565415716626)) ;
#184468=CARTESIAN_POINT('Ctrl Pts',(-17.4677491082153,-12.3489626772039,
116.594259920483)) ;
#184469=CARTESIAN_POINT('Ctrl Pts',(-17.5415529819692,-12.3489627191906,
116.57002897119)) ;
#184470=CARTESIAN_POINT('Ctrl Pts',(-17.6153568557232,-12.3489627611773,
116.545798021896)) ;
#184471=CARTESIAN_POINT('Ctrl Pts',(-17.6058868196778,-12.4185302079718,
116.516953818039)) ;
#184472=CARTESIAN_POINT('Ctrl Pts',(-17.5081423472344,-12.3404555156159,
116.254614223986)) ;
#184473=CARTESIAN_POINT('Ctrl Pts',(-17.5047506152582,-12.415576081878,
116.24428355356)) ;
#184474=CARTESIAN_POINT('Ctrl Pts',(-17.4309467386001,-12.415576066971,
116.268514494008)) ;
#184475=CARTESIAN_POINT('Ctrl Pts',(-17.3571428619421,-12.415576052064,
116.292745434456)) ;
#184476=CARTESIAN_POINT('Ctrl Pts',(-17.3605345939183,-12.3404554858018,
116.303076104882)) ;
#184477=CARTESIAN_POINT('Ctrl Pts',(-17.3639263258945,-12.2653349195397,
116.313406775308)) ;
#184478=CARTESIAN_POINT('Ctrl Pts',(-17.4377302025526,-12.2653349344467,
116.28917583486)) ;
#184479=CARTESIAN_POINT('Ctrl Pts',(-17.5115340792106,-12.2653349493537,
116.264944894412)) ;
#184480=CARTESIAN_POINT('Ctrl Pts',(-17.5081423472344,-12.3404555156159,
116.254614223986)) ;
#184481=CARTESIAN_POINT('Ctrl Pts',(-17.4066726357581,-12.3391866191646,
115.981062491338)) ;
#184482=CARTESIAN_POINT('Ctrl Pts',(-17.4096253543423,-12.414506911119,
115.990055993629)) ;
#184483=CARTESIAN_POINT('Ctrl Pts',(-17.3358214773743,-12.4145069252737,
116.014286933133)) ;
#184484=CARTESIAN_POINT('Ctrl Pts',(-17.2620176004063,-12.4145069394284,
116.038517872637)) ;
#184485=CARTESIAN_POINT('Ctrl Pts',(-17.2590648818221,-12.339186647474,
116.029524370346)) ;
#184486=CARTESIAN_POINT('Ctrl Pts',(-17.2561121632379,-12.2638663555197,
116.020530868055)) ;
#184487=CARTESIAN_POINT('Ctrl Pts',(-17.3299160402059,-12.263866341365,
115.996299928551)) ;
#184488=CARTESIAN_POINT('Ctrl Pts',(-17.4037199171738,-12.2638663272102,
115.972068989047)) ;
#184489=CARTESIAN_POINT('Ctrl Pts',(-17.4066726357581,-12.3391866191646,
115.981062491338)) ;
#184490=CARTESIAN_POINT('Ctrl Pts',(-17.3082335377069,-12.4158174303531,
115.716800039723)) ;
#184491=CARTESIAN_POINT('Ctrl Pts',(-17.3173273514836,-12.4858997019266,
115.74449832712)) ;
#184492=CARTESIAN_POINT('Ctrl Pts',(-17.2435234770911,-12.4858997440293,
115.768729274469)) ;
#184493=CARTESIAN_POINT('Ctrl Pts',(-17.1697196026986,-12.4858997861321,
115.792960221817)) ;
#184494=CARTESIAN_POINT('Ctrl Pts',(-17.160625788922,-12.4158175145586,
115.76526193442)) ;
#184495=CARTESIAN_POINT('Ctrl Pts',(-17.1515319751453,-12.3457352429851,
115.737563647023)) ;
#184496=CARTESIAN_POINT('Ctrl Pts',(-17.2253358495378,-12.3457352008824,
115.713332699674)) ;
#184497=CARTESIAN_POINT('Ctrl Pts',(-17.2991397239303,-12.3457351587796,
115.689101752326)) ;
#184498=CARTESIAN_POINT('Ctrl Pts',(-17.3082335377069,-12.4158174303531,
115.716800039723)) ;
#184499=CARTESIAN_POINT('Ctrl Pts',(-17.219815391379,-12.5633739390689,
115.482834834317)) ;
#184500=CARTESIAN_POINT('Ctrl Pts',(-17.2343644873207,-12.6232581610032,
115.527149031009)) ;
#184501=CARTESIAN_POINT('Ctrl Pts',(-17.1605606178606,-12.623258227084,
115.551379993381)) ;
#184502=CARTESIAN_POINT('Ctrl Pts',(-17.0867567484005,-12.6232582931649,
115.575610955753)) ;
#184503=CARTESIAN_POINT('Ctrl Pts',(-17.0722076524589,-12.5633740712307,
115.53129675906)) ;
#184504=CARTESIAN_POINT('Ctrl Pts',(-17.0576585565172,-12.5034898492964,
115.486982562368)) ;
#184505=CARTESIAN_POINT('Ctrl Pts',(-17.1314624259772,-12.5034897832155,
115.462751599996)) ;
#184506=CARTESIAN_POINT('Ctrl Pts',(-17.2052662954373,-12.5034897171346,
115.438520637625)) ;
#184507=CARTESIAN_POINT('Ctrl Pts',(-17.219815391379,-12.5633739390689,
115.482834834317)) ;
#184508=CARTESIAN_POINT('Ctrl Pts',(-17.1458699167164,-12.7732714821549,
115.293194413268)) ;
#184509=CARTESIAN_POINT('Ctrl Pts',(-17.1648670745331,-12.8185910964645,
115.351056688798)) ;
#184510=CARTESIAN_POINT('Ctrl Pts',(-17.0910632120963,-12.8185911800319,
115.375287672561)) ;
#184511=CARTESIAN_POINT('Ctrl Pts',(-17.0172593496596,-12.8185912635994,
115.399518656325)) ;
#184512=CARTESIAN_POINT('Ctrl Pts',(-16.9982621918429,-12.7732716492898,
115.341656380795)) ;
#184513=CARTESIAN_POINT('Ctrl Pts',(-16.9792650340262,-12.7279520349803,
115.283794105265)) ;
#184514=CARTESIAN_POINT('Ctrl Pts',(-17.053068896463,-12.7279519514128,
115.259563121501)) ;
#184515=CARTESIAN_POINT('Ctrl Pts',(-17.1268727588998,-12.7279518678453,
115.235332137738)) ;
#184516=CARTESIAN_POINT('Ctrl Pts',(-17.1458699167164,-12.7732714821549,
115.293194413268)) ;
#184517=CARTESIAN_POINT('Ctrl Pts',(-17.0918463264668,-13.0290278048664,
115.164127748858)) ;
#184518=CARTESIAN_POINT('Ctrl Pts',(-17.1139095830556,-13.0565590545988,
115.231328866614)) ;
#184519=CARTESIAN_POINT('Ctrl Pts',(-17.0401057286706,-13.0565591475459,
115.255559874902)) ;
#184520=CARTESIAN_POINT('Ctrl Pts',(-16.9663018742856,-13.056559240493,
115.27979088319)) ;
#184521=CARTESIAN_POINT('Ctrl Pts',(-16.9442386176968,-13.0290279907607,
115.212589765435)) ;
#184522=CARTESIAN_POINT('Ctrl Pts',(-16.922175361108,-13.0014967410283,
115.145388647679)) ;
#184523=CARTESIAN_POINT('Ctrl Pts',(-16.995979215493,-13.0014966480811,
115.121157639391)) ;
#184524=CARTESIAN_POINT('Ctrl Pts',(-17.0697830698779,-13.001496555134,
115.096926631103)) ;
#184525=CARTESIAN_POINT('Ctrl Pts',(-17.0918463264668,-13.0290278048664,
115.164127748858)) ;
#184526=CARTESIAN_POINT('Ctrl Pts',(-17.0605849362923,-13.311039520292,
115.10420715475)) ;
#184527=CARTESIAN_POINT('Ctrl Pts',(-17.0841334043175,-13.3189223773524,
115.175931986978)) ;
#184528=CARTESIAN_POINT('Ctrl Pts',(-17.0103295581193,-13.3189224724508,
115.200163020201)) ;
#184529=CARTESIAN_POINT('Ctrl Pts',(-16.936525711921,-13.3189225675491,
115.224394053425)) ;
#184530=CARTESIAN_POINT('Ctrl Pts',(-16.9129772438958,-13.3110397104886,
115.152669221197)) ;
#184531=CARTESIAN_POINT('Ctrl Pts',(-16.8894287758706,-13.3031568534281,
115.08094438897)) ;
#184532=CARTESIAN_POINT('Ctrl Pts',(-16.9632326220688,-13.3031567583298,
115.056713355746)) ;
#184533=CARTESIAN_POINT('Ctrl Pts',(-17.0370364682671,-13.3031566632315,
115.032482322523)) ;
#184534=CARTESIAN_POINT('Ctrl Pts',(-17.0605849362923,-13.311039520292,
115.10420715475)) ;
#184535=CARTESIAN_POINT('Ctrl Pts',(-17.0532782891826,-13.6025944687999,
115.117484856744)) ;
#184536=CARTESIAN_POINT('Ctrl Pts',(-17.0766371468441,-13.5901335291486,
115.188632166515)) ;
#184537=CARTESIAN_POINT('Ctrl Pts',(-17.0028333083748,-13.5901336172138,
115.212863223279)) ;
#184538=CARTESIAN_POINT('Ctrl Pts',(-16.9290294699055,-13.5901337052789,
115.237094280044)) ;
#184539=CARTESIAN_POINT('Ctrl Pts',(-16.905670612244,-13.6025946449302,
115.165946970274)) ;
#184540=CARTESIAN_POINT('Ctrl Pts',(-16.8823117545824,-13.6150555845815,
115.094799660503)) ;
#184541=CARTESIAN_POINT('Ctrl Pts',(-16.9561155930517,-13.6150554965163,
115.070568603739)) ;
#184542=CARTESIAN_POINT('Ctrl Pts',(-17.029919431521,-13.6150554084512,
115.046337546974)) ;
#184543=CARTESIAN_POINT('Ctrl Pts',(-17.0532782891826,-13.6025944687999,
115.117484856744)) ;
#184544=CARTESIAN_POINT('Ctrl Pts',(-17.070132390923,-13.8812809383862,
115.204405035369)) ;
#184545=CARTESIAN_POINT('Ctrl Pts',(-17.0916135474401,-13.8493436684039,
115.269833170565)) ;
#184546=CARTESIAN_POINT('Ctrl Pts',(-17.0178097151085,-13.8493437421996,
115.294064246025)) ;
#184547=CARTESIAN_POINT('Ctrl Pts',(-16.9440058827769,-13.8493438159953,
115.318295321484)) ;
#184548=CARTESIAN_POINT('Ctrl Pts',(-16.9225247262599,-13.8812810859776,
115.252867186287)) ;
#184549=CARTESIAN_POINT('Ctrl Pts',(-16.9010435697428,-13.91321835596,115.187439051091)) ;
#184550=CARTESIAN_POINT('Ctrl Pts',(-16.9748474020744,-13.9132182821642,
115.163207975632)) ;
#184551=CARTESIAN_POINT('Ctrl Pts',(-17.048651234406,-13.9132182083685,
115.138976900173)) ;
#184552=CARTESIAN_POINT('Ctrl Pts',(-17.070132390923,-13.8812809383862,
115.204405035369)) ;
#184553=CARTESIAN_POINT('Ctrl Pts',(-17.1089513768232,-14.1255805603194,
115.358085859789)) ;
#184554=CARTESIAN_POINT('Ctrl Pts',(-17.1270212361338,-14.0765381533461,
115.413123734245)) ;
#184555=CARTESIAN_POINT('Ctrl Pts',(-17.0532174080133,-14.0765382096367,
115.437354822531)) ;
#184556=CARTESIAN_POINT('Ctrl Pts',(-16.9794135798929,-14.0765382659272,
115.461585910816)) ;
#184557=CARTESIAN_POINT('Ctrl Pts',(-16.9613437205823,-14.1255806729005,
115.40654803636)) ;
#184558=CARTESIAN_POINT('Ctrl Pts',(-16.9432738612718,-14.1746230798738,
115.351510161904)) ;
#184559=CARTESIAN_POINT('Ctrl Pts',(-17.0170776893922,-14.1746230235832,
115.327279073618)) ;
#184560=CARTESIAN_POINT('Ctrl Pts',(-17.0908815175127,-14.1746229672927,
115.303047985333)) ;
#184561=CARTESIAN_POINT('Ctrl Pts',(-17.1089513768232,-14.1255805603194,
115.358085859789)) ;
#184562=CARTESIAN_POINT('Ctrl Pts',(-17.1659520639075,-14.3187775567506,
115.567024046266)) ;
#184563=CARTESIAN_POINT('Ctrl Pts',(-17.1793384581924,-14.2561721996919,
115.607796842057)) ;
#184564=CARTESIAN_POINT('Ctrl Pts',(-17.1055346324634,-14.2561722372695,
115.632027937627)) ;
#184565=CARTESIAN_POINT('Ctrl Pts',(-17.0317308067344,-14.256172274847,
115.656259033196)) ;
#184566=CARTESIAN_POINT('Ctrl Pts',(-17.0183444124495,-14.3187776319056,
115.615486237406)) ;
#184567=CARTESIAN_POINT('Ctrl Pts',(-17.0049580181646,-14.3813829889642,
115.574713441615)) ;
#184568=CARTESIAN_POINT('Ctrl Pts',(-17.0787618438936,-14.3813829513867,
115.550482346045)) ;
#184569=CARTESIAN_POINT('Ctrl Pts',(-17.1525656696226,-14.3813829138092,
115.526251250476)) ;
#184570=CARTESIAN_POINT('Ctrl Pts',(-17.1659520639075,-14.3187775567506,
115.567024046266)) ;
#184571=CARTESIAN_POINT('Ctrl Pts',(-17.2367614107398,-14.4483980300764,
115.818159542775)) ;
#184572=CARTESIAN_POINT('Ctrl Pts',(-17.2444903655536,-14.3766476693991,
115.841700690922)) ;
#184573=CARTESIAN_POINT('Ctrl Pts',(-17.1706865398769,-14.3766476878194,
115.865931786651)) ;
#184574=CARTESIAN_POINT('Ctrl Pts',(-17.0968827142002,-14.3766477062396,
115.89016288238)) ;
#184575=CARTESIAN_POINT('Ctrl Pts',(-17.0891537593863,-14.4483980669169,
115.866621734233)) ;
#184576=CARTESIAN_POINT('Ctrl Pts',(-17.0814248045724,-14.5201484275943,
115.843080586087)) ;
#184577=CARTESIAN_POINT('Ctrl Pts',(-17.1552286302491,-14.520148409174,
115.818849490358)) ;
#184578=CARTESIAN_POINT('Ctrl Pts',(-17.2290324559259,-14.5201483907537,
115.794618394629)) ;
#184579=CARTESIAN_POINT('Ctrl Pts',(-17.2367614107398,-14.4483980300764,
115.818159542775)) ;
#184580=CARTESIAN_POINT('Ctrl Pts',(-17.3155873842172,-14.5042941688686,
116.093793589286)) ;
#184581=CARTESIAN_POINT('Ctrl Pts',(-17.3170888936789,-14.4285319857966,
116.098366943866)) ;
#184582=CARTESIAN_POINT('Ctrl Pts',(-17.2432850659568,-14.4285319877587,
116.122598033365)) ;
#184583=CARTESIAN_POINT('Ctrl Pts',(-17.1694812382346,-14.4285319897207,
116.146829122864)) ;
#184584=CARTESIAN_POINT('Ctrl Pts',(-17.1679797287729,-14.5042941727927,
116.142255768284)) ;
#184585=CARTESIAN_POINT('Ctrl Pts',(-17.1664782193112,-14.5800563558646,
116.137682413704)) ;
#184586=CARTESIAN_POINT('Ctrl Pts',(-17.2402820470333,-14.5800563539026,
116.113451324205)) ;
#184587=CARTESIAN_POINT('Ctrl Pts',(-17.3140858747555,-14.5800563519406,
116.089220234706)) ;
#184588=CARTESIAN_POINT('Ctrl Pts',(-17.3155873842172,-14.5042941688686,
116.093793589286)) ;
#184589=CARTESIAN_POINT('Ctrl Pts',(-17.3959128562578,-14.4816544194473,
116.374043524353)) ;
#184590=CARTESIAN_POINT('Ctrl Pts',(-17.3910716132192,-14.4073576522614,
116.359297878409)) ;
#184591=CARTESIAN_POINT('Ctrl Pts',(-17.3172677820769,-14.4073576431116,
116.383528957491)) ;
#184592=CARTESIAN_POINT('Ctrl Pts',(-17.2434639509345,-14.4073576339619,
116.407760036573)) ;
#184593=CARTESIAN_POINT('Ctrl Pts',(-17.2483051939732,-14.4816544011478,
116.422505682517)) ;
#184594=CARTESIAN_POINT('Ctrl Pts',(-17.2531464370118,-14.5559511683337,
116.437251328461)) ;
#184595=CARTESIAN_POINT('Ctrl Pts',(-17.3269502681541,-14.5559511774834,
116.413020249379)) ;
#184596=CARTESIAN_POINT('Ctrl Pts',(-17.4007540992964,-14.5559511866331,
116.388789170297)) ;
#184597=CARTESIAN_POINT('Ctrl Pts',(-17.3959128562578,-14.4816544194473,
116.374043524353)) ;
#184598=CARTESIAN_POINT('Ctrl Pts',(-17.470339914178,-14.3839486349316,
116.635941043976)) ;
#184599=CARTESIAN_POINT('Ctrl Pts',(-17.4595662274915,-14.3163620052717,
116.603126131994)) ;
#184600=CARTESIAN_POINT('Ctrl Pts',(-17.3857623934809,-14.3163619889056,
116.627357202339)) ;
#184601=CARTESIAN_POINT('Ctrl Pts',(-17.3119585594702,-14.3163619725394,
116.651588272685)) ;
#184602=CARTESIAN_POINT('Ctrl Pts',(-17.3227322461567,-14.3839486021993,
116.684403184667)) ;
#184603=CARTESIAN_POINT('Ctrl Pts',(-17.3335059328432,-14.4515352318592,
116.717218096649)) ;
#184604=CARTESIAN_POINT('Ctrl Pts',(-17.4073097668538,-14.4515352482253,
116.692987026303)) ;
#184605=CARTESIAN_POINT('Ctrl Pts',(-17.4811136008645,-14.4515352645915,
116.668755955958)) ;
#184606=CARTESIAN_POINT('Ctrl Pts',(-17.470339914178,-14.3839486349316,
116.635941043976)) ;
#184607=CARTESIAN_POINT('Ctrl Pts',(-17.5344056730198,-14.2160711628555,
116.866668150428)) ;
#184608=CARTESIAN_POINT('Ctrl Pts',(-17.5184057446407,-14.1601035188724,
116.817934949686)) ;
#184609=CARTESIAN_POINT('Ctrl Pts',(-17.4446019067002,-14.1601035014112,
116.842166008062)) ;
#184610=CARTESIAN_POINT('Ctrl Pts',(-17.3707980687597,-14.1601034839499,
116.866397066437)) ;
#184611=CARTESIAN_POINT('Ctrl Pts',(-17.3867979971388,-14.216071127933,
116.915130267179)) ;
#184612=CARTESIAN_POINT('Ctrl Pts',(-17.4027979255179,-14.272038771916,
116.96386346792)) ;
#184613=CARTESIAN_POINT('Ctrl Pts',(-17.4766017634584,-14.2720387893772,
116.939632409545)) ;
#184614=CARTESIAN_POINT('Ctrl Pts',(-17.5504056013989,-14.2720388068385,
116.915401351169)) ;
#184615=CARTESIAN_POINT('Ctrl Pts',(-17.5344056730198,-14.2160711628555,
116.866668150428)) ;
#184616=CARTESIAN_POINT('Ctrl Pts',(-17.5816569877728,-13.9907700541576,
117.046110214416)) ;
#184617=CARTESIAN_POINT('Ctrl Pts',(-17.5615983820216,-13.9504492968838,
116.985014937421)) ;
#184618=CARTESIAN_POINT('Ctrl Pts',(-17.4877945411903,-13.950449282471,
117.009245986992)) ;
#184619=CARTESIAN_POINT('Ctrl Pts',(-17.4139907003589,-13.9504492680581,
117.033477036562)) ;
#184620=CARTESIAN_POINT('Ctrl Pts',(-17.4340493061101,-13.9907700253318,
117.094572313557)) ;
#184621=CARTESIAN_POINT('Ctrl Pts',(-17.4541079118614,-14.0310907826056,
117.155667590553)) ;
#184622=CARTESIAN_POINT('Ctrl Pts',(-17.5279117526927,-14.0310907970185,
117.131436540982)) ;
#184623=CARTESIAN_POINT('Ctrl Pts',(-17.601715593524,-14.0310908114314,
117.107205491412)) ;
#184624=CARTESIAN_POINT('Ctrl Pts',(-17.5816569877728,-13.9907700541576,
117.046110214416)) ;
#184625=CARTESIAN_POINT('Ctrl Pts',(-17.6081495369059,-13.7263636069236,
117.162089654627)) ;
#184626=CARTESIAN_POINT('Ctrl Pts',(-17.5854807397544,-13.7044442251976,
117.093044155887)) ;
#184627=CARTESIAN_POINT('Ctrl Pts',(-17.5116768971497,-13.7044442144499,
117.117275200056)) ;
#184628=CARTESIAN_POINT('Ctrl Pts',(-17.437873054545,-13.7044442037021,
117.141506244225)) ;
#184629=CARTESIAN_POINT('Ctrl Pts',(-17.4605418516965,-13.7263635854281,
117.210551742966)) ;
#184630=CARTESIAN_POINT('Ctrl Pts',(-17.4832106488481,-13.7482829671541,
117.279597241706)) ;
#184631=CARTESIAN_POINT('Ctrl Pts',(-17.5570144914527,-13.7482829779018,
117.255366197537)) ;
#184632=CARTESIAN_POINT('Ctrl Pts',(-17.6308183340574,-13.7482829886496,
117.231135153367)) ;
#184633=CARTESIAN_POINT('Ctrl Pts',(-17.6081495369059,-13.7263636069236,
117.162089654627)) ;
#184634=CARTESIAN_POINT('Ctrl Pts',(-17.6114977252136,-13.4372481920934,
117.207915677809)) ;
#184635=CARTESIAN_POINT('Ctrl Pts',(-17.5878235258813,-13.4354837655308,
117.135807886383)) ;
#184636=CARTESIAN_POINT('Ctrl Pts',(-17.5140196823244,-13.4354837614887,
117.160038927651)) ;
#184637=CARTESIAN_POINT('Ctrl Pts',(-17.4402158387675,-13.4354837574465,
117.18426996892)) ;
#184638=CARTESIAN_POINT('Ctrl Pts',(-17.4638900380998,-13.4372481840091,
117.256377760346)) ;
#184639=CARTESIAN_POINT('Ctrl Pts',(-17.4875642374321,-13.4390126105717,
117.328485551772)) ;
#184640=CARTESIAN_POINT('Ctrl Pts',(-17.561368080989,-13.4390126146139,
117.304254510503)) ;
#184641=CARTESIAN_POINT('Ctrl Pts',(-17.6351719245459,-13.4390126186561,
117.280023469235)) ;
#184642=CARTESIAN_POINT('Ctrl Pts',(-17.6114977252136,-13.4372481920934,
117.207915677809)) ;
#184643=CARTESIAN_POINT('Ctrl Pts',(-17.5903413936119,-13.1479585724495,
117.178954366257)) ;
#184644=CARTESIAN_POINT('Ctrl Pts',(-17.5673748053404,-13.1663919966203,
117.10900184403)) ;
#184645=CARTESIAN_POINT('Ctrl Pts',(-17.4935709618626,-13.1663919968395,
117.13323288554)) ;
#184646=CARTESIAN_POINT('Ctrl Pts',(-17.4197671183847,-13.1663919970587,
117.157463927049)) ;
#184647=CARTESIAN_POINT('Ctrl Pts',(-17.4427337066562,-13.1479585728878,
117.227416449276)) ;
#184648=CARTESIAN_POINT('Ctrl Pts',(-17.4657002949275,-13.1295251487169,
117.297368971502)) ;
#184649=CARTESIAN_POINT('Ctrl Pts',(-17.5395041384054,-13.1295251484978,
117.273137929993)) ;
#184650=CARTESIAN_POINT('Ctrl Pts',(-17.6133079818833,-13.1295251482786,
117.248906888483)) ;
#184651=CARTESIAN_POINT('Ctrl Pts',(-17.5903413936119,-13.1479585724495,
117.178954366257)) ;
#184652=CARTESIAN_POINT('Ctrl Pts',(-17.5459869448181,-12.8791408632362,
117.079169963688)) ;
#184653=CARTESIAN_POINT('Ctrl Pts',(-17.52535255275,-12.9163723052174,117.016320934844)) ;
#184654=CARTESIAN_POINT('Ctrl Pts',(-17.4515487096923,-12.9163723075118,
117.040551977634)) ;
#184655=CARTESIAN_POINT('Ctrl Pts',(-17.3777448666347,-12.9163723098062,
117.064783020423)) ;
#184656=CARTESIAN_POINT('Ctrl Pts',(-17.3983792587028,-12.8791408678251,
117.127632049267)) ;
#184657=CARTESIAN_POINT('Ctrl Pts',(-17.419013650771,-12.8419094258439,
117.19048107811)) ;
#184658=CARTESIAN_POINT('Ctrl Pts',(-17.4928174938286,-12.8419094235494,
117.166250035321)) ;
#184659=CARTESIAN_POINT('Ctrl Pts',(-17.5666213368863,-12.841909421255,
117.142018992531)) ;
#184660=CARTESIAN_POINT('Ctrl Pts',(-17.5459869448181,-12.8791408632362,
117.079169963688)) ;
#184661=CARTESIAN_POINT('Ctrl Pts',(-17.480026568366,-12.6468837882592,
116.913878073808)) ;
#184662=CARTESIAN_POINT('Ctrl Pts',(-17.4632304799261,-12.7003895422397,
116.862719898524)) ;
#184663=CARTESIAN_POINT('Ctrl Pts',(-17.389426637272,-12.7003895445952,
116.886950942542)) ;
#184664=CARTESIAN_POINT('Ctrl Pts',(-17.3156227946178,-12.7003895469507,
116.911181986561)) ;
#184665=CARTESIAN_POINT('Ctrl Pts',(-17.3324188830577,-12.6468837929702,
116.962340161844)) ;
#184666=CARTESIAN_POINT('Ctrl Pts',(-17.3492149714976,-12.5933780389898,
117.013498337128)) ;
#184667=CARTESIAN_POINT('Ctrl Pts',(-17.4230188141518,-12.5933780366342,
116.98926729311)) ;
#184668=CARTESIAN_POINT('Ctrl Pts',(-17.4968226568059,-12.5933780342787,
116.965036249091)) ;
#184669=CARTESIAN_POINT('Ctrl Pts',(-17.480026568366,-12.6468837882592,
116.913878073808)) ;
#184670=CARTESIAN_POINT('Ctrl Pts',(-17.3974510186948,-12.471578495706,
116.697698668639)) ;
#184671=CARTESIAN_POINT('Ctrl Pts',(-17.3856651005318,-12.5374039130151,
116.661800663601)) ;
#184672=CARTESIAN_POINT('Ctrl Pts',(-17.3118612576612,-12.5374039137778,
116.68603170696)) ;
#184673=CARTESIAN_POINT('Ctrl Pts',(-17.2380574147905,-12.5374039145406,
116.710262750319)) ;
#184674=CARTESIAN_POINT('Ctrl Pts',(-17.2498433329535,-12.4715784972316,
116.746160755357)) ;
#184675=CARTESIAN_POINT('Ctrl Pts',(-17.2616292511165,-12.4057530799226,
116.782058760395)) ;
#184676=CARTESIAN_POINT('Ctrl Pts',(-17.3354330939871,-12.4057530791598,
116.757827717036)) ;
#184677=CARTESIAN_POINT('Ctrl Pts',(-17.4092369368578,-12.405753078397,
116.733596673676)) ;
#184678=CARTESIAN_POINT('Ctrl Pts',(-17.3974510186948,-12.471578495706,
116.697698668639)) ;
#184679=CARTESIAN_POINT('Ctrl Pts',(-17.3026957115669,-12.3629963199509,
116.444542308675)) ;
#184680=CARTESIAN_POINT('Ctrl Pts',(-17.2967752602771,-12.4365002767228,
116.426509569284)) ;
#184681=CARTESIAN_POINT('Ctrl Pts',(-17.2229714165425,-12.4365002760064,
116.450740610012)) ;
#184682=CARTESIAN_POINT('Ctrl Pts',(-17.1491675728079,-12.4365002752899,
116.47497165074)) ;
#184683=CARTESIAN_POINT('Ctrl Pts',(-17.1550880240977,-12.362996318518,
116.49300439013)) ;
#184684=CARTESIAN_POINT('Ctrl Pts',(-17.1610084753875,-12.289492361746,
116.51103712952)) ;
#184685=CARTESIAN_POINT('Ctrl Pts',(-17.2348123191221,-12.2894923624625,
116.486806088793)) ;
#184686=CARTESIAN_POINT('Ctrl Pts',(-17.3086161628567,-12.289492363179,
116.462575048065)) ;
#184687=CARTESIAN_POINT('Ctrl Pts',(-17.3026957115669,-12.3629963199509,
116.444542308675)) ;
#184688=CARTESIAN_POINT('Ctrl Pts',(-17.2013092259047,-12.3302292617424,
116.171414664088)) ;
#184689=CARTESIAN_POINT('Ctrl Pts',(-17.2017212267144,-12.4061292172083,
116.172669551933)) ;
#184690=CARTESIAN_POINT('Ctrl Pts',(-17.1279173809519,-12.4061292167983,
116.196900586484)) ;
#184691=CARTESIAN_POINT('Ctrl Pts',(-17.0541135351894,-12.4061292163883,
116.221131621035)) ;
#184692=CARTESIAN_POINT('Ctrl Pts',(-17.0537015343797,-12.3302292609224,
116.21987673319)) ;
#184693=CARTESIAN_POINT('Ctrl Pts',(-17.05328953357,-12.2543293054565,116.218621845346)) ;
#184694=CARTESIAN_POINT('Ctrl Pts',(-17.1270933793325,-12.2543293058665,
116.194390810795)) ;
#184695=CARTESIAN_POINT('Ctrl Pts',(-17.200897225095,-12.2543293062765,
116.170159776244)) ;
#184696=CARTESIAN_POINT('Ctrl Pts',(-17.2013092259047,-12.3302292617424,
116.171414664088)) ;
#184697=CARTESIAN_POINT('Ctrl Pts',(-17.1012548069171,-12.3757631813199,
115.902068780532)) ;
#184698=CARTESIAN_POINT('Ctrl Pts',(-17.1079209304104,-12.4485939704729,
115.922372716854)) ;
#184699=CARTESIAN_POINT('Ctrl Pts',(-17.03411708288,-12.448593973849,115.946603746021)) ;
#184700=CARTESIAN_POINT('Ctrl Pts',(-16.9603132353497,-12.448593977225,
115.970834775187)) ;
#184701=CARTESIAN_POINT('Ctrl Pts',(-16.9536471118565,-12.3757631880721,
115.950530838865)) ;
#184702=CARTESIAN_POINT('Ctrl Pts',(-16.9469809883632,-12.3029323989191,
115.930226902543)) ;
#184703=CARTESIAN_POINT('Ctrl Pts',(-17.0207848358935,-12.302932395543,
115.905995873376)) ;
#184704=CARTESIAN_POINT('Ctrl Pts',(-17.0945886834239,-12.302932392167,
115.88176484421)) ;
#184705=CARTESIAN_POINT('Ctrl Pts',(-17.1012548069171,-12.3757631813199,
115.902068780532)) ;
#184706=CARTESIAN_POINT('Ctrl Pts',(-17.0081478668239,-12.4955339259777,
115.653885289273)) ;
#184707=CARTESIAN_POINT('Ctrl Pts',(-17.0205919444078,-12.560107521336,
115.691787941355)) ;
#184708=CARTESIAN_POINT('Ctrl Pts',(-16.946788095502,-12.5601075316302,
115.716018966332)) ;
#184709=CARTESIAN_POINT('Ctrl Pts',(-16.8729842465962,-12.5601075419243,
115.740249991309)) ;
#184710=CARTESIAN_POINT('Ctrl Pts',(-16.8605401690123,-12.495533946566,
115.702347339227)) ;
#184711=CARTESIAN_POINT('Ctrl Pts',(-16.8480960914284,-12.4309603512076,
115.664444687145)) ;
#184712=CARTESIAN_POINT('Ctrl Pts',(-16.9218999403342,-12.4309603409135,
115.640213662168)) ;
#184713=CARTESIAN_POINT('Ctrl Pts',(-16.99570378924,-12.4309603306194,115.615982637191)) ;
#184714=CARTESIAN_POINT('Ctrl Pts',(-17.0081478668239,-12.4955339259777,
115.653885289273)) ;
#184715=CARTESIAN_POINT('Ctrl Pts',(-16.927880930918,-12.6811191445398,
115.444803605489)) ;
#184716=CARTESIAN_POINT('Ctrl Pts',(-16.9452148438001,-12.7328282545194,
115.497599906775)) ;
#184717=CARTESIAN_POINT('Ctrl Pts',(-16.8714109943575,-12.7328282744618,
115.521830930117)) ;
#184718=CARTESIAN_POINT('Ctrl Pts',(-16.7976071449149,-12.7328282944042,
115.546061953459)) ;
#184719=CARTESIAN_POINT('Ctrl Pts',(-16.7802732320328,-12.6811191844247,
115.493265652173)) ;
#184720=CARTESIAN_POINT('Ctrl Pts',(-16.7629393191507,-12.6294100744451,
115.440469350888)) ;
#184721=CARTESIAN_POINT('Ctrl Pts',(-16.8367431685933,-12.6294100545027,
115.416238327546)) ;
#184722=CARTESIAN_POINT('Ctrl Pts',(-16.9105470180359,-12.6294100345603,
115.392007304204)) ;
#184723=CARTESIAN_POINT('Ctrl Pts',(-16.927880930918,-12.6811191445398,
115.444803605489)) ;
#184724=CARTESIAN_POINT('Ctrl Pts',(-16.8652589405334,-12.9201897809832,
115.289585909363)) ;
#184725=CARTESIAN_POINT('Ctrl Pts',(-16.8862552957216,-12.9552816729516,
115.353537418807)) ;
#184726=CARTESIAN_POINT('Ctrl Pts',(-16.8124514468531,-12.9552817052441,
115.377768443898)) ;
#184727=CARTESIAN_POINT('Ctrl Pts',(-16.7386475979846,-12.9552817375366,
115.401999468988)) ;
#184728=CARTESIAN_POINT('Ctrl Pts',(-16.7176512427965,-12.9201898455682,
115.338047959545)) ;
#184729=CARTESIAN_POINT('Ctrl Pts',(-16.6966548876083,-12.8850979535998,
115.274096450101)) ;
#184730=CARTESIAN_POINT('Ctrl Pts',(-16.7704587364768,-12.8850979213072,
115.24986542501)) ;
#184731=CARTESIAN_POINT('Ctrl Pts',(-16.8442625853453,-12.8850978890147,
115.225634399919)) ;
#184732=CARTESIAN_POINT('Ctrl Pts',(-16.8652589405334,-12.9201897809832,
115.289585909363)) ;
#184733=CARTESIAN_POINT('Ctrl Pts',(-16.8243940341797,-13.1945616988577,
115.200574037482)) ;
#184734=CARTESIAN_POINT('Ctrl Pts',(-16.8475402280435,-13.2105476900329,
115.271073608491)) ;
#184735=CARTESIAN_POINT('Ctrl Pts',(-16.7737363815082,-13.2105477342474,
115.295304640688)) ;
#184736=CARTESIAN_POINT('Ctrl Pts',(-16.699932534973,-13.2105477784618,
115.319535672885)) ;
#184737=CARTESIAN_POINT('Ctrl Pts',(-16.6767863411092,-13.1945617872866,
115.249036101877)) ;
#184738=CARTESIAN_POINT('Ctrl Pts',(-16.6536401472453,-13.1785757961114,
115.178536530868)) ;
#184739=CARTESIAN_POINT('Ctrl Pts',(-16.7274439937806,-13.178575751897,
115.154305498671)) ;
#184740=CARTESIAN_POINT('Ctrl Pts',(-16.8012478403159,-13.1785757076825,
115.130074466474)) ;
#184741=CARTESIAN_POINT('Ctrl Pts',(-16.8243940341797,-13.1945616988577,
115.200574037482)) ;
#184742=CARTESIAN_POINT('Ctrl Pts',(-16.8072714937354,-13.4849425718836,
115.183882623779)) ;
#184743=CARTESIAN_POINT('Ctrl Pts',(-16.8309128359796,-13.4806775745737,
115.255890336694)) ;
#184744=CARTESIAN_POINT('Ctrl Pts',(-16.7571089933573,-13.4806776285265,
115.28012138081)) ;
#184745=CARTESIAN_POINT('Ctrl Pts',(-16.683305150735,-13.4806776824793,
115.304352424926)) ;
#184746=CARTESIAN_POINT('Ctrl Pts',(-16.6596638084908,-13.4849426797892,
115.23234471201)) ;
#184747=CARTESIAN_POINT('Ctrl Pts',(-16.6360224662466,-13.4892076770991,
115.160336999094)) ;
#184748=CARTESIAN_POINT('Ctrl Pts',(-16.7098263088689,-13.4892076231463,
115.136105954979)) ;
#184749=CARTESIAN_POINT('Ctrl Pts',(-16.7836301514911,-13.4892075691935,
115.111874910863)) ;
#184750=CARTESIAN_POINT('Ctrl Pts',(-16.8072714937354,-13.4849425718836,
115.183882623779)) ;
#184751=CARTESIAN_POINT('Ctrl Pts',(-16.8144795961222,-13.7714537290315,
115.241411416659)) ;
#184752=CARTESIAN_POINT('Ctrl Pts',(-16.8369158670254,-13.7471788354609,
115.309748676522)) ;
#184753=CARTESIAN_POINT('Ctrl Pts',(-16.7631120298244,-13.7471788958938,
115.33397973715)) ;
#184754=CARTESIAN_POINT('Ctrl Pts',(-16.6893081926234,-13.7471789563267,
115.358210797778)) ;
#184755=CARTESIAN_POINT('Ctrl Pts',(-16.6668719217202,-13.7714538498972,
115.289873537915)) ;
#184756=CARTESIAN_POINT('Ctrl Pts',(-16.6444356508169,-13.7957287434678,
115.221536278052)) ;
#184757=CARTESIAN_POINT('Ctrl Pts',(-16.718239488018,-13.7957286830349,
115.197305217424)) ;
#184758=CARTESIAN_POINT('Ctrl Pts',(-16.792043325219,-13.7957286226021,
115.173074156796)) ;
#184759=CARTESIAN_POINT('Ctrl Pts',(-16.8144795961222,-13.7714537290315,
115.241411416659)) ;
#184760=CARTESIAN_POINT('Ctrl Pts',(-16.8447740676149,-14.0317199143361,
115.369164792903)) ;
#184761=CARTESIAN_POINT('Ctrl Pts',(-16.8643935570099,-13.9892386384962,
115.428922590618)) ;
#184762=CARTESIAN_POINT('Ctrl Pts',(-16.7905897260983,-13.9892386981122,
115.453153670403)) ;
#184763=CARTESIAN_POINT('Ctrl Pts',(-16.7167858951867,-13.9892387577282,
115.477384750187)) ;
#184764=CARTESIAN_POINT('Ctrl Pts',(-16.6971664057917,-14.0317200335681,
115.417626952471)) ;
#184765=CARTESIAN_POINT('Ctrl Pts',(-16.6775469163966,-14.074201309408,
115.357869154755)) ;
#184766=CARTESIAN_POINT('Ctrl Pts',(-16.7513507473083,-14.074201249792,
115.333638074971)) ;
#184767=CARTESIAN_POINT('Ctrl Pts',(-16.8251545782199,-14.074201190176,
115.309406995187)) ;
#184768=CARTESIAN_POINT('Ctrl Pts',(-16.8447740676149,-14.0317199143361,
115.369164792903)) ;
#184769=CARTESIAN_POINT('Ctrl Pts',(-16.8947662272287,-14.2471737495219,
115.556725502171)) ;
#184770=CARTESIAN_POINT('Ctrl Pts',(-16.9101934226221,-14.1895888186294,
115.603714248662)) ;
#184771=CARTESIAN_POINT('Ctrl Pts',(-16.836389597641,-14.1895888696549,
115.627945346509)) ;
#184772=CARTESIAN_POINT('Ctrl Pts',(-16.7625857726599,-14.1895889206804,
115.652176444357)) ;
#184773=CARTESIAN_POINT('Ctrl Pts',(-16.7471585772665,-14.2471738515729,
115.605187697866)) ;
#184774=CARTESIAN_POINT('Ctrl Pts',(-16.7317313818732,-14.3047587824654,
115.558198951375)) ;
#184775=CARTESIAN_POINT('Ctrl Pts',(-16.8055352068543,-14.3047587314399,
115.533967853527)) ;
#184776=CARTESIAN_POINT('Ctrl Pts',(-16.8793390318354,-14.3047586804144,
115.50973675568)) ;
#184777=CARTESIAN_POINT('Ctrl Pts',(-16.8947662272287,-14.2471737495219,
115.556725502171)) ;
#184778=CARTESIAN_POINT('Ctrl Pts',(-16.961109045615,-14.4050269028801,
115.794454092593)) ;
#184779=CARTESIAN_POINT('Ctrl Pts',(-16.9711891073453,-14.3363371537911,
115.825156332537)) ;
#184780=CARTESIAN_POINT('Ctrl Pts',(-16.8973852883592,-14.3363371907916,
115.849387448645)) ;
#184781=CARTESIAN_POINT('Ctrl Pts',(-16.8235814693732,-14.3363372277921,
115.873618564752)) ;
#184782=CARTESIAN_POINT('Ctrl Pts',(-16.813501407643,-14.4050269768811,
115.842916324808)) ;
#184783=CARTESIAN_POINT('Ctrl Pts',(-16.8034213459128,-14.47371672597,115.812214084863)) ;
#184784=CARTESIAN_POINT('Ctrl Pts',(-16.8772251648988,-14.4737166889695,
115.787982968756)) ;
#184785=CARTESIAN_POINT('Ctrl Pts',(-16.9510289838848,-14.473716651969,
115.763751852648)) ;
#184786=CARTESIAN_POINT('Ctrl Pts',(-16.961109045615,-14.4050269028801,
115.794454092593)) ;
#184787=CARTESIAN_POINT('Ctrl Pts',(-17.0371572122292,-14.4907853879862,
116.061445277914)) ;
#184788=CARTESIAN_POINT('Ctrl Pts',(-17.0412107801516,-14.4160085433366,
116.073791789988)) ;
#184789=CARTESIAN_POINT('Ctrl Pts',(-16.9674069650101,-14.4160085589544,
116.098022917805)) ;
#184790=CARTESIAN_POINT('Ctrl Pts',(-16.8936031498686,-14.4160085745722,
116.122254045622)) ;
#184791=CARTESIAN_POINT('Ctrl Pts',(-16.8895495819462,-14.4907854192218,
116.109907533549)) ;
#184792=CARTESIAN_POINT('Ctrl Pts',(-16.8854960140238,-14.5655622638714,
116.097561021475)) ;
#184793=CARTESIAN_POINT('Ctrl Pts',(-16.9592998291653,-14.5655622482536,
116.073329893658)) ;
#184794=CARTESIAN_POINT('Ctrl Pts',(-17.0331036443068,-14.5655622326357,
116.04909876584)) ;
#184795=CARTESIAN_POINT('Ctrl Pts',(-17.0371572122292,-14.4907853879862,
116.061445277914)) ;
#184796=CARTESIAN_POINT('Ctrl Pts',(-17.1172490342387,-14.5004458117326,
116.340780850017)) ;
#184797=CARTESIAN_POINT('Ctrl Pts',(-17.1149845378817,-14.4248856962509,
116.333883557615)) ;
#184798=CARTESIAN_POINT('Ctrl Pts',(-17.0411807245678,-14.4248856868723,
116.358114690999)) ;
#184799=CARTESIAN_POINT('Ctrl Pts',(-16.9673769112539,-14.4248856774938,
116.382345824383)) ;
#184800=CARTESIAN_POINT('Ctrl Pts',(-16.9696414076109,-14.5004457929755,
116.389243116785)) ;
#184801=CARTESIAN_POINT('Ctrl Pts',(-16.9719059039679,-14.5760059084573,
116.396140409187)) ;
#184802=CARTESIAN_POINT('Ctrl Pts',(-17.0457097172818,-14.5760059178358,
116.371909275803)) ;
#184803=CARTESIAN_POINT('Ctrl Pts',(-17.1195135305957,-14.5760059272144,
116.347678142419)) ;
#184804=CARTESIAN_POINT('Ctrl Pts',(-17.1172490342387,-14.5004458117326,
116.340780850017)) ;
#184805=CARTESIAN_POINT('Ctrl Pts',(-17.195241265685,-14.4322721687238,
116.613881501569)) ;
#184806=CARTESIAN_POINT('Ctrl Pts',(-17.1867927976471,-14.3613608624439,
116.588148829115)) ;
#184807=CARTESIAN_POINT('Ctrl Pts',(-17.1129889838628,-14.3613608259143,
116.612379961066)) ;
#184808=CARTESIAN_POINT('Ctrl Pts',(-17.0391851700784,-14.3613607893847,
116.636611093017)) ;
#184809=CARTESIAN_POINT('Ctrl Pts',(-17.0476336381162,-14.4322720956646,
116.662343765471)) ;
#184810=CARTESIAN_POINT('Ctrl Pts',(-17.056082106154,-14.5031834019444,
116.688076437926)) ;
#184811=CARTESIAN_POINT('Ctrl Pts',(-17.1298859199384,-14.5031834384741,
116.663845305975)) ;
#184812=CARTESIAN_POINT('Ctrl Pts',(-17.2036897337228,-14.5031834750037,
116.639614174024)) ;
#184813=CARTESIAN_POINT('Ctrl Pts',(-17.195241265685,-14.4322721687238,
116.613881501569)) ;
#184814=CARTESIAN_POINT('Ctrl Pts',(-17.2641686388444,-14.2916898608516,
116.859246556023)) ;
#184815=CARTESIAN_POINT('Ctrl Pts',(-17.2501625770948,-14.2304895577996,
116.816586349776)) ;
#184816=CARTESIAN_POINT('Ctrl Pts',(-17.1763587600007,-14.2304894954371,
116.840817471646)) ;
#184817=CARTESIAN_POINT('Ctrl Pts',(-17.1025549429065,-14.2304894330745,
116.865048593516)) ;
#184818=CARTESIAN_POINT('Ctrl Pts',(-17.1165610046561,-14.2916897361264,
116.907708799763)) ;
#184819=CARTESIAN_POINT('Ctrl Pts',(-17.1305670664057,-14.3528900391783,
116.95036900601)) ;
#184820=CARTESIAN_POINT('Ctrl Pts',(-17.2043708834998,-14.3528901015409,
116.92613788414)) ;
#184821=CARTESIAN_POINT('Ctrl Pts',(-17.278174700594,-14.3528901639035,
116.90190676227)) ;
#184822=CARTESIAN_POINT('Ctrl Pts',(-17.2641686388444,-14.2916898608516,
116.859246556023)) ;
#184823=CARTESIAN_POINT('Ctrl Pts',(-17.3187345972075,-14.0883182665925,
117.060933073971)) ;
#184824=CARTESIAN_POINT('Ctrl Pts',(-17.3001640538882,-14.0412264219864,
117.004370193295)) ;
#184825=CARTESIAN_POINT('Ctrl Pts',(-17.226360231113,-14.0412263375894,
117.028601297861)) ;
#184826=CARTESIAN_POINT('Ctrl Pts',(-17.1525564083378,-14.0412262531924,
117.052832402427)) ;
#184827=CARTESIAN_POINT('Ctrl Pts',(-17.171126951657,-14.0883180977985,
117.109395283104)) ;
#184828=CARTESIAN_POINT('Ctrl Pts',(-17.1896974949763,-14.1354099424045,
117.165958163781)) ;
#184829=CARTESIAN_POINT('Ctrl Pts',(-17.2635013177515,-14.1354100268015,
117.141727059215)) ;
#184830=CARTESIAN_POINT('Ctrl Pts',(-17.3373051405268,-14.1354101111986,
117.117495954648)) ;
#184831=CARTESIAN_POINT('Ctrl Pts',(-17.3187345972075,-14.0883182665925,
117.060933073971)) ;
#184832=CARTESIAN_POINT('Ctrl Pts',(-17.3540623162582,-13.837248063462,
117.203966576996)) ;
#184833=CARTESIAN_POINT('Ctrl Pts',(-17.3322648072597,-13.8076155637165,
117.137574879509)) ;
#184834=CARTESIAN_POINT('Ctrl Pts',(-17.2584609768669,-13.8076154638135,
117.161805960873)) ;
#184835=CARTESIAN_POINT('Ctrl Pts',(-17.184657146474,-13.8076153639105,
117.186037042237)) ;
#184836=CARTESIAN_POINT('Ctrl Pts',(-17.2064546554726,-13.837247863656,
117.252428739724)) ;
#184837=CARTESIAN_POINT('Ctrl Pts',(-17.2282521644711,-13.8668803634015,
117.318820437211)) ;
#184838=CARTESIAN_POINT('Ctrl Pts',(-17.3020559948639,-13.8668804633045,
117.294589355847)) ;
#184839=CARTESIAN_POINT('Ctrl Pts',(-17.3758598252568,-13.8668805632075,
117.270358274483)) ;
#184840=CARTESIAN_POINT('Ctrl Pts',(-17.3540623162582,-13.837248063462,
117.203966576996)) ;
#184841=CARTESIAN_POINT('Ctrl Pts',(-17.3670526898512,-13.5564419727403,
117.278940688503)) ;
#184842=CARTESIAN_POINT('Ctrl Pts',(-17.3435833841598,-13.5463705176912,
117.20745696803)) ;
#184843=CARTESIAN_POINT('Ctrl Pts',(-17.2697795450213,-13.5463704101859,
117.231688022757)) ;
#184844=CARTESIAN_POINT('Ctrl Pts',(-17.1959757058828,-13.5463703026806,
117.255919077483)) ;
#184845=CARTESIAN_POINT('Ctrl Pts',(-17.2194450115743,-13.5564417577297,
117.327402797955)) ;
#184846=CARTESIAN_POINT('Ctrl Pts',(-17.2429143172658,-13.5665132127787,
117.398886518428)) ;
#184847=CARTESIAN_POINT('Ctrl Pts',(-17.3167181564042,-13.5665133202841,
117.374655463701)) ;
#184848=CARTESIAN_POINT('Ctrl Pts',(-17.3905219955427,-13.5665134277894,
117.350424408975)) ;
#184849=CARTESIAN_POINT('Ctrl Pts',(-17.3670526898512,-13.5564419727403,
117.278940688503)) ;
#184850=CARTESIAN_POINT('Ctrl Pts',(-17.355858225208,-13.2643191465395,
117.280425433147)) ;
#184851=CARTESIAN_POINT('Ctrl Pts',(-17.3323992611542,-13.2746275458087,
117.20897321166)) ;
#184852=CARTESIAN_POINT('Ctrl Pts',(-17.2585954129658,-13.2746274398407,
117.233204238822)) ;
#184853=CARTESIAN_POINT('Ctrl Pts',(-17.1847915647773,-13.2746273338727,
117.257435265983)) ;
#184854=CARTESIAN_POINT('Ctrl Pts',(-17.2082505288311,-13.2643189346036,
117.328887487471)) ;
#184855=CARTESIAN_POINT('Ctrl Pts',(-17.2317094928849,-13.2540105353345,
117.400339708958)) ;
#184856=CARTESIAN_POINT('Ctrl Pts',(-17.3055133410734,-13.2540106413025,
117.376108681796)) ;
#184857=CARTESIAN_POINT('Ctrl Pts',(-17.3793171892618,-13.2540107472704,
117.351877654634)) ;
#184858=CARTESIAN_POINT('Ctrl Pts',(-17.355858225208,-13.2643191465395,
117.280425433147)) ;
#184859=CARTESIAN_POINT('Ctrl Pts',(-17.3206670190795,-12.984649033957,
117.208638071495)) ;
#184860=CARTESIAN_POINT('Ctrl Pts',(-17.2988976194389,-13.0144985177463,
117.142331990642)) ;
#184861=CARTESIAN_POINT('Ctrl Pts',(-17.2250937629149,-13.0144984216522,
117.166562992415)) ;
#184862=CARTESIAN_POINT('Ctrl Pts',(-17.1512899063909,-13.0144983255582,
117.190793994188)) ;
#184863=CARTESIAN_POINT('Ctrl Pts',(-17.1730593060315,-12.9846488417689,
117.257100075041)) ;
#184864=CARTESIAN_POINT('Ctrl Pts',(-17.1948287056722,-12.9547993579796,
117.323406155894)) ;
#184865=CARTESIAN_POINT('Ctrl Pts',(-17.2686325621962,-12.9547994540736,
117.299175154121)) ;
#184866=CARTESIAN_POINT('Ctrl Pts',(-17.3424364187202,-12.9547995501676,
117.274944152348)) ;
#184867=CARTESIAN_POINT('Ctrl Pts',(-17.3206670190795,-12.984649033957,
117.208638071495)) ;
#184868=CARTESIAN_POINT('Ctrl Pts',(-17.2631129943276,-12.7352694992048,
117.068833096118)) ;
#184869=CARTESIAN_POINT('Ctrl Pts',(-17.2445948108717,-12.782574545107,
117.012429695249)) ;
#184870=CARTESIAN_POINT('Ctrl Pts',(-17.1707909475106,-12.7825744663775,
117.036660676197)) ;
#184871=CARTESIAN_POINT('Ctrl Pts',(-17.0969870841495,-12.782574387648,
117.060891657145)) ;
#184872=CARTESIAN_POINT('Ctrl Pts',(-17.1155052676054,-12.7352693417458,
117.117295058015)) ;
#184873=CARTESIAN_POINT('Ctrl Pts',(-17.1340234510614,-12.6879642958436,
117.173698458884)) ;
#184874=CARTESIAN_POINT('Ctrl Pts',(-17.2078273144225,-12.6879643745731,
117.149467477936)) ;
#184875=CARTESIAN_POINT('Ctrl Pts',(-17.2816311777836,-12.6879644533026,
117.125236496987)) ;
#184876=CARTESIAN_POINT('Ctrl Pts',(-17.2631129943276,-12.7352694992048,
117.068833096118)) ;
#184877=CARTESIAN_POINT('Ctrl Pts',(-17.1866392534368,-12.5350620992742,
116.87137248245)) ;
#184878=CARTESIAN_POINT('Ctrl Pts',(-17.1726986483145,-12.5964160722861,
116.828911646682)) ;
#184879=CARTESIAN_POINT('Ctrl Pts',(-17.0988947802738,-12.5964160160119,
116.853142613377)) ;
#184880=CARTESIAN_POINT('Ctrl Pts',(-17.0250909122331,-12.5964159597377,
116.877373580072)) ;
#184881=CARTESIAN_POINT('Ctrl Pts',(-17.0390315173554,-12.5350619867258,
116.91983441584)) ;
#184882=CARTESIAN_POINT('Ctrl Pts',(-17.0529721224778,-12.4737080137138,
116.962295251609)) ;
#184883=CARTESIAN_POINT('Ctrl Pts',(-17.1267759905185,-12.4737080699881,
116.938064284914)) ;
#184884=CARTESIAN_POINT('Ctrl Pts',(-17.2005798585592,-12.4737081262623,
116.913833318219)) ;
#184885=CARTESIAN_POINT('Ctrl Pts',(-17.1866392534368,-12.5350620992742,
116.87137248245)) ;
#184886=CARTESIAN_POINT('Ctrl Pts',(-17.0960336520393,-12.3981381252086,
116.630846912972)) ;
#184887=CARTESIAN_POINT('Ctrl Pts',(-17.0876645823112,-12.4691440372206,
116.605356075152)) ;
#184888=CARTESIAN_POINT('Ctrl Pts',(-17.0138607120287,-12.4691440057978,
116.629587035019)) ;
#184889=CARTESIAN_POINT('Ctrl Pts',(-16.9400568417462,-12.4691439743751,
116.653817994886)) ;
#184890=CARTESIAN_POINT('Ctrl Pts',(-16.9484259114743,-12.3981380623631,
116.679308832706)) ;
#184891=CARTESIAN_POINT('Ctrl Pts',(-16.9567949812024,-12.3271321503511,
116.704799670525)) ;
#184892=CARTESIAN_POINT('Ctrl Pts',(-17.0305988514848,-12.3271321817739,
116.680568710658)) ;
#184893=CARTESIAN_POINT('Ctrl Pts',(-17.1044027217673,-12.3271322131966,
116.656337750791)) ;
#184894=CARTESIAN_POINT('Ctrl Pts',(-17.0960336520393,-12.3981381252086,
116.630846912972)) ;
#184895=CARTESIAN_POINT('Ctrl Pts',(-16.9968920488552,-12.3341497286325,
116.364349421587)) ;
#184896=CARTESIAN_POINT('Ctrl Pts',(-16.9946982815475,-12.4097302348877,
116.35766755868)) ;
#184897=CARTESIAN_POINT('Ctrl Pts',(-16.9208944115846,-12.4097302280834,
116.381898519521)) ;
#184898=CARTESIAN_POINT('Ctrl Pts',(-16.8470905416218,-12.409730221279,
116.406129480361)) ;
#184899=CARTESIAN_POINT('Ctrl Pts',(-16.8492843089295,-12.3341497150238,
116.412811343268)) ;
#184900=CARTESIAN_POINT('Ctrl Pts',(-16.8514780762372,-12.2585692087685,
116.419493206174)) ;
#184901=CARTESIAN_POINT('Ctrl Pts',(-16.9252819462,-12.2585692155729,116.395262245333)) ;
#184902=CARTESIAN_POINT('Ctrl Pts',(-16.9990858161628,-12.2585692223772,
116.371031284493)) ;
#184903=CARTESIAN_POINT('Ctrl Pts',(-16.9968920488552,-12.3341497286325,
116.364349421587)) ;
#184904=CARTESIAN_POINT('Ctrl Pts',(-16.8955934699839,-12.3478638226298,
116.091294655271)) ;
#184905=CARTESIAN_POINT('Ctrl Pts',(-16.89973469377,-12.4226010423524,116.103908153229)) ;
#184906=CARTESIAN_POINT('Ctrl Pts',(-16.8259308264129,-12.4226010571477,
116.128139122006)) ;
#184907=CARTESIAN_POINT('Ctrl Pts',(-16.7521269590558,-12.422601071943,
116.152370090783)) ;
#184908=CARTESIAN_POINT('Ctrl Pts',(-16.7479857352698,-12.3478638522204,
116.139756592826)) ;
#184909=CARTESIAN_POINT('Ctrl Pts',(-16.7438445114837,-12.2731266324978,
116.127143094869)) ;
#184910=CARTESIAN_POINT('Ctrl Pts',(-16.8176483788408,-12.2731266177025,
116.102912126092)) ;
#184911=CARTESIAN_POINT('Ctrl Pts',(-16.8914522461979,-12.2731266029072,
116.078681157314)) ;
#184912=CARTESIAN_POINT('Ctrl Pts',(-16.8955934699839,-12.3478638226298,
116.091294655271)) ;
#184913=CARTESIAN_POINT('Ctrl Pts',(-16.7987277286322,-12.4382992209291,
115.831728050634)) ;
#184914=CARTESIAN_POINT('Ctrl Pts',(-16.8089043705112,-12.5068353759983,
115.862724458441)) ;
#184915=CARTESIAN_POINT('Ctrl Pts',(-16.7351005074183,-12.5068354072617,
115.886955440206)) ;
#184916=CARTESIAN_POINT('Ctrl Pts',(-16.6612966443254,-12.5068354385251,
115.911186421972)) ;
#184917=CARTESIAN_POINT('Ctrl Pts',(-16.6511200024464,-12.4382992834559,
115.880190014164)) ;
#184918=CARTESIAN_POINT('Ctrl Pts',(-16.6409433605675,-12.3697631283867,
115.849193606357)) ;
#184919=CARTESIAN_POINT('Ctrl Pts',(-16.7147472236604,-12.3697630971233,
115.824962624592)) ;
#184920=CARTESIAN_POINT('Ctrl Pts',(-16.7885510867532,-12.3697630658599,
115.800731642826)) ;
#184921=CARTESIAN_POINT('Ctrl Pts',(-16.7987277286322,-12.4382992209291,
115.831728050634)) ;
#184922=CARTESIAN_POINT('Ctrl Pts',(-16.7125017303928,-12.5986984925073,
115.604533974206)) ;
#184923=CARTESIAN_POINT('Ctrl Pts',(-16.7279808214323,-12.6561393028317,
115.651680786763)) ;
#184924=CARTESIAN_POINT('Ctrl Pts',(-16.654176963508,-12.65613934453,115.675911784271)) ;
#184925=CARTESIAN_POINT('Ctrl Pts',(-16.5803731055837,-12.6561393862282,
115.700142781779)) ;
#184926=CARTESIAN_POINT('Ctrl Pts',(-16.5648940145443,-12.5986985759038,
115.652995969222)) ;
#184927=CARTESIAN_POINT('Ctrl Pts',(-16.5494149235048,-12.5412577655794,
115.605849156666)) ;
#184928=CARTESIAN_POINT('Ctrl Pts',(-16.6232187814291,-12.5412577238812,
115.581618159158)) ;
#184929=CARTESIAN_POINT('Ctrl Pts',(-16.6970226393534,-12.541257682183,
115.557387161649)) ;
#184930=CARTESIAN_POINT('Ctrl Pts',(-16.7125017303928,-12.5986984925073,
115.604533974206)) ;
#184931=CARTESIAN_POINT('Ctrl Pts',(-16.6421521442805,-12.8181589219149,
115.425759855238)) ;
#184932=CARTESIAN_POINT('Ctrl Pts',(-16.6618320255675,-12.8603639864266,
115.485701597265)) ;
#184933=CARTESIAN_POINT('Ctrl Pts',(-16.5880281731401,-12.8603640315663,
115.509932611516)) ;
#184934=CARTESIAN_POINT('Ctrl Pts',(-16.5142243207128,-12.8603640767059,
115.534163625767)) ;
#184935=CARTESIAN_POINT('Ctrl Pts',(-16.4945444394258,-12.8181590121942,
115.47422188374)) ;
#184936=CARTESIAN_POINT('Ctrl Pts',(-16.4748645581388,-12.7759539476825,
115.414280141713)) ;
#184937=CARTESIAN_POINT('Ctrl Pts',(-16.5486684105661,-12.7759539025429,
115.390049127462)) ;
#184938=CARTESIAN_POINT('Ctrl Pts',(-16.6224722629935,-12.7759538574032,
115.365818113211)) ;
#184939=CARTESIAN_POINT('Ctrl Pts',(-16.6421521442805,-12.8181589219149,
115.425759855238)) ;
#184940=CARTESIAN_POINT('Ctrl Pts',(-16.5922545474962,-13.0797516616193,
115.309162122654)) ;
#184941=CARTESIAN_POINT('Ctrl Pts',(-16.6147159819925,-13.1037557901174,
115.377576027107)) ;
#184942=CARTESIAN_POINT('Ctrl Pts',(-16.5409121343667,-13.1037558337794,
115.401807055983)) ;
#184943=CARTESIAN_POINT('Ctrl Pts',(-16.4671082867409,-13.1037558774415,
115.426038084858)) ;
#184944=CARTESIAN_POINT('Ctrl Pts',(-16.4446468522446,-13.0797517489434,
115.357624180405)) ;
#184945=CARTESIAN_POINT('Ctrl Pts',(-16.4221854177483,-13.0557476204452,
115.289210275952)) ;
#184946=CARTESIAN_POINT('Ctrl Pts',(-16.4959892653741,-13.0557475767832,
115.264979247076)) ;
#184947=CARTESIAN_POINT('Ctrl Pts',(-16.5697931129999,-13.0557475331212,
115.2407482182)) ;
#184948=CARTESIAN_POINT('Ctrl Pts',(-16.5922545474962,-13.0797516616193,
115.309162122654)) ;
#184949=CARTESIAN_POINT('Ctrl Pts',(-16.5652750102249,-13.3661182947965,
115.262452316505)) ;
#184950=CARTESIAN_POINT('Ctrl Pts',(-16.5889203991877,-13.3701640997913,
115.334472355401)) ;
#184951=CARTESIAN_POINT('Ctrl Pts',(-16.5151165554926,-13.3701641367874,
115.358703396249)) ;
#184952=CARTESIAN_POINT('Ctrl Pts',(-16.4413127117975,-13.3701641737835,
115.382934437097)) ;
#184953=CARTESIAN_POINT('Ctrl Pts',(-16.4176673228348,-13.3661183687887,
115.310914398201)) ;
#184954=CARTESIAN_POINT('Ctrl Pts',(-16.394021933872,-13.3620725637939,
115.238894359305)) ;
#184955=CARTESIAN_POINT('Ctrl Pts',(-16.4678257775671,-13.3620725267978,
115.214663318457)) ;
#184956=CARTESIAN_POINT('Ctrl Pts',(-16.5416296212622,-13.3620724898017,
115.190432277609)) ;
#184957=CARTESIAN_POINT('Ctrl Pts',(-16.5652750102249,-13.3661182947965,
115.262452316505)) ;
#184958=CARTESIAN_POINT('Ctrl Pts',(-16.5626467913676,-13.656951267572,
115.290002450311)) ;
#184959=CARTESIAN_POINT('Ctrl Pts',(-16.5857758666926,-13.6406962235438,
115.360449881353)) ;
#184960=CARTESIAN_POINT('Ctrl Pts',(-16.5119720254153,-13.6406962503813,
115.384680929566)) ;
#184961=CARTESIAN_POINT('Ctrl Pts',(-16.438168184138,-13.6406962772189,
115.408911977778)) ;
#184962=CARTESIAN_POINT('Ctrl Pts',(-16.4150391088129,-13.6569513212471,
115.338464546735)) ;
#184963=CARTESIAN_POINT('Ctrl Pts',(-16.3919100334878,-13.6732063652754,
115.268017115692)) ;
#184964=CARTESIAN_POINT('Ctrl Pts',(-16.4657138747652,-13.6732063384378,
115.24378606748)) ;
#184965=CARTESIAN_POINT('Ctrl Pts',(-16.5395177160425,-13.6732063116003,
115.219555019268)) ;
#184966=CARTESIAN_POINT('Ctrl Pts',(-16.5626467913676,-13.656951267572,
115.290002450311)) ;
#184967=CARTESIAN_POINT('Ctrl Pts',(-16.5837488475447,-13.9296721739865,
115.389708810494)) ;
#184968=CARTESIAN_POINT('Ctrl Pts',(-16.6047062406092,-13.8943500486195,
115.453541647919)) ;
#184969=CARTESIAN_POINT('Ctrl Pts',(-16.5309024003191,-13.8943500659771,
115.477772699138)) ;
#184970=CARTESIAN_POINT('Ctrl Pts',(-16.457098560029,-13.8943500833347,
115.502003750357)) ;
#184971=CARTESIAN_POINT('Ctrl Pts',(-16.4361411669645,-13.9296722087017,
115.438170912932)) ;
#184972=CARTESIAN_POINT('Ctrl Pts',(-16.4151837738999,-13.9649943340687,
115.374338075508)) ;
#184973=CARTESIAN_POINT('Ctrl Pts',(-16.48898761419,-13.9649943167111,115.350107024289)) ;
#184974=CARTESIAN_POINT('Ctrl Pts',(-16.5627914544801,-13.9649942993535,
115.32587597307)) ;
#184975=CARTESIAN_POINT('Ctrl Pts',(-16.5837488475447,-13.9296721739865,
115.389708810494)) ;
#184976=CARTESIAN_POINT('Ctrl Pts',(-16.6262908326384,-14.1660389555352,
115.554751277984)) ;
#184977=CARTESIAN_POINT('Ctrl Pts',(-16.6435754639849,-14.1141591424512,
115.607397475954)) ;
#184978=CARTESIAN_POINT('Ctrl Pts',(-16.569771623452,-14.114159151286,115.631628526433)) ;
#184979=CARTESIAN_POINT('Ctrl Pts',(-16.495967782919,-14.1141591601208,
115.655859576913)) ;
#184980=CARTESIAN_POINT('Ctrl Pts',(-16.4786831515725,-14.1660389732048,
115.603213378943)) ;
#184981=CARTESIAN_POINT('Ctrl Pts',(-16.461398520226,-14.2179187862889,
115.550567180973)) ;
#184982=CARTESIAN_POINT('Ctrl Pts',(-16.535202360759,-14.2179187774541,
115.526336130494)) ;
#184983=CARTESIAN_POINT('Ctrl Pts',(-16.609006201292,-14.2179187686193,
115.502105080014)) ;
#184984=CARTESIAN_POINT('Ctrl Pts',(-16.6262908326384,-14.1660389555352,
115.554751277984)) ;
#184985=CARTESIAN_POINT('Ctrl Pts',(-16.6865043266641,-14.3487828478669,
115.773619369682)) ;
#184986=CARTESIAN_POINT('Ctrl Pts',(-16.6988765648799,-14.2840645582721,
115.811303210909)) ;
#184987=CARTESIAN_POINT('Ctrl Pts',(-16.625072723286,-14.2840645612063,
115.835534258157)) ;
#184988=CARTESIAN_POINT('Ctrl Pts',(-16.5512688816921,-14.2840645641405,
115.859765305405)) ;
#184989=CARTESIAN_POINT('Ctrl Pts',(-16.5388966434763,-14.3487828537354,
115.822081464178)) ;
#184990=CARTESIAN_POINT('Ctrl Pts',(-16.5265244052603,-14.4135011433302,
115.784397622951)) ;
#184991=CARTESIAN_POINT('Ctrl Pts',(-16.6003282468543,-14.413501140396,
115.760166575704)) ;
#184992=CARTESIAN_POINT('Ctrl Pts',(-16.6741320884482,-14.4135011374618,
115.735935528456)) ;
#184993=CARTESIAN_POINT('Ctrl Pts',(-16.6865043266641,-14.3487828478669,
115.773619369682)) ;
#184994=CARTESIAN_POINT('Ctrl Pts',(-16.7592456254264,-14.4648357931477,
116.030618712201)) ;
#184995=CARTESIAN_POINT('Ctrl Pts',(-16.7658237132317,-14.391916747365,
116.050654506254)) ;
#184996=CARTESIAN_POINT('Ctrl Pts',(-16.6920198703368,-14.3919167474485,
116.074885549539)) ;
#184997=CARTESIAN_POINT('Ctrl Pts',(-16.6182160274419,-14.391916747532,
116.099116592824)) ;
#184998=CARTESIAN_POINT('Ctrl Pts',(-16.6116379396366,-14.4648357933146,
116.079080798771)) ;
#184999=CARTESIAN_POINT('Ctrl Pts',(-16.6050598518314,-14.5377548390973,
116.059045004718)) ;
#185000=CARTESIAN_POINT('Ctrl Pts',(-16.6788636947263,-14.5377548390138,
116.034813961433)) ;
#185001=CARTESIAN_POINT('Ctrl Pts',(-16.7526675376212,-14.5377548389303,
116.010582918148)) ;
#185002=CARTESIAN_POINT('Ctrl Pts',(-16.7592456254264,-14.4648357931477,
116.030618712201)) ;
#185003=CARTESIAN_POINT('Ctrl Pts',(-16.8386665689219,-14.5058959818021,
116.307994675603)) ;
#185004=CARTESIAN_POINT('Ctrl Pts',(-16.8389745832277,-14.4300007264442,
116.308932837514)) ;
#185005=CARTESIAN_POINT('Ctrl Pts',(-16.7651707392682,-14.4300007261889,
116.333163877557)) ;
#185006=CARTESIAN_POINT('Ctrl Pts',(-16.6913668953086,-14.4300007259336,
116.357394917599)) ;
#185007=CARTESIAN_POINT('Ctrl Pts',(-16.6910588810028,-14.5058959812914,
116.356456755687)) ;
#185008=CARTESIAN_POINT('Ctrl Pts',(-16.690750866697,-14.5817912366492,
116.355518593776)) ;
#185009=CARTESIAN_POINT('Ctrl Pts',(-16.7645547106565,-14.5817912369046,
116.331287553734)) ;
#185010=CARTESIAN_POINT('Ctrl Pts',(-16.8383585546161,-14.5817912371599,
116.307056513691)) ;
#185011=CARTESIAN_POINT('Ctrl Pts',(-16.8386665689219,-14.5058959818021,
116.307994675603)) ;
#185012=CARTESIAN_POINT('Ctrl Pts',(-16.9180971410873,-14.4694242942484,
116.585309225375)) ;
#185013=CARTESIAN_POINT('Ctrl Pts',(-16.9121269062051,-14.3959630196689,
116.567124853285)) ;
#185014=CARTESIAN_POINT('Ctrl Pts',(-16.8383230617492,-14.3959630205436,
116.591355891816)) ;
#185015=CARTESIAN_POINT('Ctrl Pts',(-16.7645192172934,-14.3959630214183,
116.615586930346)) ;
#185016=CARTESIAN_POINT('Ctrl Pts',(-16.7704894521756,-14.4694242959978,
116.633771302437)) ;
#185017=CARTESIAN_POINT('Ctrl Pts',(-16.7764596870578,-14.5428855705773,
116.651955674527)) ;
#185018=CARTESIAN_POINT('Ctrl Pts',(-16.8502635315136,-14.5428855697026,
116.627724635996)) ;
#185019=CARTESIAN_POINT('Ctrl Pts',(-16.9240673759695,-14.542885568828,
116.603493597466)) ;
#185020=CARTESIAN_POINT('Ctrl Pts',(-16.9180971410873,-14.4694242942484,
116.585309225375)) ;
#185021=CARTESIAN_POINT('Ctrl Pts',(-16.9919081234988,-14.356381751671,
116.845841056527)) ;
#185022=CARTESIAN_POINT('Ctrl Pts',(-16.980035442802,-14.2907051755566,
116.809678786819)) ;
#185023=CARTESIAN_POINT('Ctrl Pts',(-16.9062315987896,-14.2907051768879,
116.833909826701)) ;
#185024=CARTESIAN_POINT('Ctrl Pts',(-16.8324277547772,-14.2907051782191,
116.858140866582)) ;
#185025=CARTESIAN_POINT('Ctrl Pts',(-16.8443004354741,-14.3563817543336,
116.89430313629)) ;
#185026=CARTESIAN_POINT('Ctrl Pts',(-16.8561731161709,-14.422058330448,
116.930465405997)) ;
#185027=CARTESIAN_POINT('Ctrl Pts',(-16.9299769601833,-14.4220583291168,
116.906234366116)) ;
#185028=CARTESIAN_POINT('Ctrl Pts',(-17.0037808041957,-14.4220583277855,
116.882003326234)) ;
#185029=CARTESIAN_POINT('Ctrl Pts',(-16.9919081234988,-14.356381751671,
116.845841056527)) ;
#185030=CARTESIAN_POINT('Ctrl Pts',(-17.0525352838852,-14.1778422798436,
117.06575399033)) ;
#185031=CARTESIAN_POINT('Ctrl Pts',(-17.0356824497799,-14.1245364286659,
117.014422976839)) ;
#185032=CARTESIAN_POINT('Ctrl Pts',(-16.9618786064408,-14.1245364288381,
117.038654018772)) ;
#185033=CARTESIAN_POINT('Ctrl Pts',(-16.8880747631017,-14.1245364290103,
117.062885060704)) ;
#185034=CARTESIAN_POINT('Ctrl Pts',(-16.904927597207,-14.177842280188,117.114216074195)) ;
#185035=CARTESIAN_POINT('Ctrl Pts',(-16.9217804313123,-14.2311481313656,
117.165547087685)) ;
#185036=CARTESIAN_POINT('Ctrl Pts',(-16.9955842746514,-14.2311481311934,
117.141316045753)) ;
#185037=CARTESIAN_POINT('Ctrl Pts',(-17.0693881179905,-14.2311481310212,
117.117085003821)) ;
#185038=CARTESIAN_POINT('Ctrl Pts',(-17.0525352838852,-14.1778422798436,
117.06575399033)) ;
#185039=CARTESIAN_POINT('Ctrl Pts',(-17.0962610112578,-13.9441247450056,
117.234417675053)) ;
#185040=CARTESIAN_POINT('Ctrl Pts',(-17.0755960229063,-13.9070603957443,
117.171475454734)) ;
#185041=CARTESIAN_POINT('Ctrl Pts',(-17.0017921802879,-13.9070603921811,
117.195706498861)) ;
#185042=CARTESIAN_POINT('Ctrl Pts',(-16.9279883376695,-13.9070603886178,
117.219937542989)) ;
#185043=CARTESIAN_POINT('Ctrl Pts',(-16.948653326021,-13.9441247378791,
117.282879763307)) ;
#185044=CARTESIAN_POINT('Ctrl Pts',(-16.9693183143724,-13.9811890871404,
117.345821983626)) ;
#185045=CARTESIAN_POINT('Ctrl Pts',(-17.0431221569908,-13.9811890907036,
117.321590939499)) ;
#185046=CARTESIAN_POINT('Ctrl Pts',(-17.1169259996092,-13.9811890942669,
117.297359895372)) ;
#185047=CARTESIAN_POINT('Ctrl Pts',(-17.0962610112578,-13.9441247450056,
117.234417675053)) ;
#185048=CARTESIAN_POINT('Ctrl Pts',(-17.1185983352745,-13.6724643503177,
117.337941114439)) ;
#185049=CARTESIAN_POINT('Ctrl Pts',(-17.0956091461605,-13.6543146170461,
117.267919753489)) ;
#185050=CARTESIAN_POINT('Ctrl Pts',(-17.021805303656,-13.6543146070783,
117.292150797963)) ;
#185051=CARTESIAN_POINT('Ctrl Pts',(-16.9480014611515,-13.6543145971105,
117.316381842438)) ;
#185052=CARTESIAN_POINT('Ctrl Pts',(-16.9709906502654,-13.6724643303821,
117.386403203388)) ;
#185053=CARTESIAN_POINT('Ctrl Pts',(-16.9939798393793,-13.6906140636538,
117.456424564338)) ;
#185054=CARTESIAN_POINT('Ctrl Pts',(-17.0677836818839,-13.6906140736215,
117.432193519863)) ;
#185055=CARTESIAN_POINT('Ctrl Pts',(-17.1415875243884,-13.6906140835893,
117.407962475389)) ;
#185056=CARTESIAN_POINT('Ctrl Pts',(-17.1185983352745,-13.6724643503177,
117.337941114439)) ;
#185057=CARTESIAN_POINT('Ctrl Pts',(-17.117418789511,-13.3835337156027,
117.369720038339)) ;
#185058=CARTESIAN_POINT('Ctrl Pts',(-17.0937466861375,-13.3855315872837,
117.297618630625)) ;
#185059=CARTESIAN_POINT('Ctrl Pts',(-17.019942842807,-13.3855315707962,
117.321849672584)) ;
#185060=CARTESIAN_POINT('Ctrl Pts',(-16.9461389994764,-13.3855315543086,
117.346080714542)) ;
#185061=CARTESIAN_POINT('Ctrl Pts',(-16.96981110285,-13.3835336826277,117.418182122256)) ;
#185062=CARTESIAN_POINT('Ctrl Pts',(-16.9934832062235,-13.3815358109467,
117.49028352997)) ;
#185063=CARTESIAN_POINT('Ctrl Pts',(-17.067287049554,-13.3815358274342,
117.466052488011)) ;
#185064=CARTESIAN_POINT('Ctrl Pts',(-17.1410908928846,-13.3815358439218,
117.441821446053)) ;
#185065=CARTESIAN_POINT('Ctrl Pts',(-17.117418789511,-13.3835337156027,
117.369720038339)) ;
#185066=CARTESIAN_POINT('Ctrl Pts',(-17.0915909181535,-13.0942320536069,
117.326791158127)) ;
#185067=CARTESIAN_POINT('Ctrl Pts',(-17.0689480758727,-13.1164328568091,
117.257824713433)) ;
#185068=CARTESIAN_POINT('Ctrl Pts',(-16.9951442302083,-13.1164328311838,
117.282055748283)) ;
#185069=CARTESIAN_POINT('Ctrl Pts',(-16.9213403845439,-13.1164328055585,
117.306286783133)) ;
#185070=CARTESIAN_POINT('Ctrl Pts',(-16.9439832268247,-13.0942320023563,
117.375253227826)) ;
#185071=CARTESIAN_POINT('Ctrl Pts',(-16.9666260691055,-13.0720311991542,
117.444219672519)) ;
#185072=CARTESIAN_POINT('Ctrl Pts',(-17.0404299147699,-13.0720312247795,
117.419988637669)) ;
#185073=CARTESIAN_POINT('Ctrl Pts',(-17.1142337604343,-13.0720312504048,
117.39575760282)) ;
#185074=CARTESIAN_POINT('Ctrl Pts',(-17.0915909181535,-13.0942320536069,
117.326791158127)) ;
#185075=CARTESIAN_POINT('Ctrl Pts',(-17.0430263168028,-12.8318300831267,
117.214118671673)) ;
#185076=CARTESIAN_POINT('Ctrl Pts',(-17.0230123581187,-12.8723837829672,
117.153159382125)) ;
#185077=CARTESIAN_POINT('Ctrl Pts',(-16.9492085093455,-12.8723837548031,
117.177390407506)) ;
#185078=CARTESIAN_POINT('Ctrl Pts',(-16.8754046605723,-12.872383726639,
117.201621432886)) ;
#185079=CARTESIAN_POINT('Ctrl Pts',(-16.8954186192564,-12.8318300267985,
117.262580722435)) ;
#185080=CARTESIAN_POINT('Ctrl Pts',(-16.9154325779404,-12.791276326958,
117.323540011983)) ;
#185081=CARTESIAN_POINT('Ctrl Pts',(-16.9892364267137,-12.7912763551221,
117.299308986602)) ;
#185082=CARTESIAN_POINT('Ctrl Pts',(-17.0630402754869,-12.7912763832862,
117.275077961222)) ;
#185083=CARTESIAN_POINT('Ctrl Pts',(-17.0430263168028,-12.8318300831267,
117.214118671673)) ;
#185084=CARTESIAN_POINT('Ctrl Pts',(-16.9734981845306,-12.608937228869,
117.037951919378)) ;
#185085=CARTESIAN_POINT('Ctrl Pts',(-16.957572902719,-12.6651122393528,
116.989446079685)) ;
#185086=CARTESIAN_POINT('Ctrl Pts',(-16.8837690495209,-12.6651122100812,
117.013677091588)) ;
#185087=CARTESIAN_POINT('Ctrl Pts',(-16.8099651963227,-12.6651121808096,
117.037908103491)) ;
#185088=CARTESIAN_POINT('Ctrl Pts',(-16.8258904781343,-12.6089371703258,
117.086413943185)) ;
#185089=CARTESIAN_POINT('Ctrl Pts',(-16.8418157599459,-12.5527621598419,
117.134919782878)) ;
#185090=CARTESIAN_POINT('Ctrl Pts',(-16.9156196131441,-12.5527621891136,
117.110688770975)) ;
#185091=CARTESIAN_POINT('Ctrl Pts',(-16.9894234663423,-12.5527622183852,
117.086457759072)) ;
#185092=CARTESIAN_POINT('Ctrl Pts',(-16.9734981845306,-12.608937228869,
117.037951919378)) ;
#185093=CARTESIAN_POINT('Ctrl Pts',(-16.8882820075866,-12.4456165862493,
116.813713510996)) ;
#185094=CARTESIAN_POINT('Ctrl Pts',(-16.8775527597793,-12.5132753292444,
116.781033952363)) ;
#185095=CARTESIAN_POINT('Ctrl Pts',(-16.8037489024639,-12.5132753061601,
116.805264951725)) ;
#185096=CARTESIAN_POINT('Ctrl Pts',(-16.7299450451485,-12.5132752830759,
116.829495951088)) ;
#185097=CARTESIAN_POINT('Ctrl Pts',(-16.7406742929557,-12.4456165400809,
116.862175509721)) ;
#185098=CARTESIAN_POINT('Ctrl Pts',(-16.751403540763,-12.3779577970859,
116.894855068354)) ;
#185099=CARTESIAN_POINT('Ctrl Pts',(-16.8252073980784,-12.3779578201701,
116.870624068992)) ;
#185100=CARTESIAN_POINT('Ctrl Pts',(-16.8990112553938,-12.3779578432543,
116.846393069629)) ;
#185101=CARTESIAN_POINT('Ctrl Pts',(-16.8882820075866,-12.4456165862493,
116.813713510996)) ;
#185102=CARTESIAN_POINT('Ctrl Pts',(-16.7917570614056,-12.3507741827119,
116.555224982685)) ;
#185103=CARTESIAN_POINT('Ctrl Pts',(-16.7870167098958,-12.4251525805178,
116.540786635693)) ;
#185104=CARTESIAN_POINT('Ctrl Pts',(-16.713212848396,-12.425152568096,116.565017622311)) ;
#185105=CARTESIAN_POINT('Ctrl Pts',(-16.6394089868962,-12.4251525556743,
116.589248608929)) ;
#185106=CARTESIAN_POINT('Ctrl Pts',(-16.644149338406,-12.3507741578684,
116.603686955921)) ;
#185107=CARTESIAN_POINT('Ctrl Pts',(-16.6488896899159,-12.2763957600624,
116.618125302913)) ;
#185108=CARTESIAN_POINT('Ctrl Pts',(-16.7226935514157,-12.2763957724842,
116.593894316295)) ;
#185109=CARTESIAN_POINT('Ctrl Pts',(-16.7964974129154,-12.276395784906,
116.569663329677)) ;
#185110=CARTESIAN_POINT('Ctrl Pts',(-16.7917570614056,-12.3507741827119,
116.555224982685)) ;
#185111=CARTESIAN_POINT('Ctrl Pts',(-16.6902172566931,-12.3329811601702,
116.281543753901)) ;
#185112=CARTESIAN_POINT('Ctrl Pts',(-16.6918228500276,-12.4087098331506,
116.286434130807)) ;
#185113=CARTESIAN_POINT('Ctrl Pts',(-16.6180189852007,-12.4087098375423,
116.310665107291)) ;
#185114=CARTESIAN_POINT('Ctrl Pts',(-16.5442151203738,-12.408709841934,
116.334896083775)) ;
#185115=CARTESIAN_POINT('Ctrl Pts',(-16.5426095270393,-12.3329811689535,
116.330005706869)) ;
#185116=CARTESIAN_POINT('Ctrl Pts',(-16.5410039337048,-12.2572524959731,
116.325115329963)) ;
#185117=CARTESIAN_POINT('Ctrl Pts',(-16.6148077985317,-12.2572524915815,
116.30088435348)) ;
#185118=CARTESIAN_POINT('Ctrl Pts',(-16.6886116633586,-12.2572524871898,
116.276653376996)) ;
#185119=CARTESIAN_POINT('Ctrl Pts',(-16.6902172566931,-12.3329811601702,
116.281543753901)) ;
#185120=CARTESIAN_POINT('Ctrl Pts',(-16.5913515055266,-12.3924859215409,
116.015688386954)) ;
#185121=CARTESIAN_POINT('Ctrl Pts',(-16.5991321052098,-12.4641691937461,
116.039386836745)) ;
#185122=CARTESIAN_POINT('Ctrl Pts',(-16.5253282397077,-12.4641692182498,
116.063617811173)) ;
#185123=CARTESIAN_POINT('Ctrl Pts',(-16.4515243742057,-12.4641692427536,
116.0878487856)) ;
#185124=CARTESIAN_POINT('Ctrl Pts',(-16.4437437745226,-12.3924859705485,
116.064150335809)) ;
#185125=CARTESIAN_POINT('Ctrl Pts',(-16.4359631748395,-12.3208026983433,
116.040451886018)) ;
#185126=CARTESIAN_POINT('Ctrl Pts',(-16.5097670403415,-12.3208026738395,
116.01622091159)) ;
#185127=CARTESIAN_POINT('Ctrl Pts',(-16.5835709058435,-12.3208026493358,
115.991989937163)) ;
#185128=CARTESIAN_POINT('Ctrl Pts',(-16.5913515055266,-12.3924859215409,
116.015688386954)) ;
#185129=CARTESIAN_POINT('Ctrl Pts',(-16.4999410090283,-12.5254680767671,
115.772761598066)) ;
#185130=CARTESIAN_POINT('Ctrl Pts',(-16.513380438689,-12.5879710242858,
115.813695930772)) ;
#185131=CARTESIAN_POINT('Ctrl Pts',(-16.4395765740198,-12.587971070974,
115.837926907736)) ;
#185132=CARTESIAN_POINT('Ctrl Pts',(-16.3657727093505,-12.5879711176621,
115.8621578847)) ;
#185133=CARTESIAN_POINT('Ctrl Pts',(-16.3523332796897,-12.5254681701434,
115.821223551993)) ;
#185134=CARTESIAN_POINT('Ctrl Pts',(-16.338893850029,-12.4629652226247,
115.780289219287)) ;
#185135=CARTESIAN_POINT('Ctrl Pts',(-16.4126977146982,-12.4629651759366,
115.756058242323)) ;
#185136=CARTESIAN_POINT('Ctrl Pts',(-16.4865015793675,-12.4629651292484,
115.731827265359)) ;
#185137=CARTESIAN_POINT('Ctrl Pts',(-16.4999410090283,-12.5254680767671,
115.772761598066)) ;
#185138=CARTESIAN_POINT('Ctrl Pts',(-16.4223757171239,-12.7232333026618,
115.572077481631)) ;
#185139=CARTESIAN_POINT('Ctrl Pts',(-16.4405141467196,-12.7720201100749,
115.627324209818)) ;
#185140=CARTESIAN_POINT('Ctrl Pts',(-16.3667102852944,-12.7720201789256,
115.651555196663)) ;
#185141=CARTESIAN_POINT('Ctrl Pts',(-16.2929064238692,-12.7720202477763,
115.675786183508)) ;
#185142=CARTESIAN_POINT('Ctrl Pts',(-16.2747679942734,-12.7232334403633,
115.620539455321)) ;
#185143=CARTESIAN_POINT('Ctrl Pts',(-16.2566295646777,-12.6744466329502,
115.565292727134)) ;
#185144=CARTESIAN_POINT('Ctrl Pts',(-16.3304334261029,-12.6744465640995,
115.541061740289)) ;
#185145=CARTESIAN_POINT('Ctrl Pts',(-16.4042372875281,-12.6744464952487,
115.516830753444)) ;
#185146=CARTESIAN_POINT('Ctrl Pts',(-16.4223757171239,-12.7232333026618,
115.572077481631)) ;
#185147=CARTESIAN_POINT('Ctrl Pts',(-16.3639160111054,-12.9691613747719,
115.429347837265)) ;
#185148=CARTESIAN_POINT('Ctrl Pts',(-16.3854312159419,-13.0008491150667,
115.494879677901)) ;
#185149=CARTESIAN_POINT('Ctrl Pts',(-16.3116273602281,-13.0008492011903,
115.519110682142)) ;
#185150=CARTESIAN_POINT('Ctrl Pts',(-16.2378235045142,-13.0008492873139,
115.543341686382)) ;
#185151=CARTESIAN_POINT('Ctrl Pts',(-16.2163082996777,-12.9691615470191,
115.477809845746)) ;
#185152=CARTESIAN_POINT('Ctrl Pts',(-16.1947930948412,-12.9374738067243,
115.41227800511)) ;
#185153=CARTESIAN_POINT('Ctrl Pts',(-16.268596950555,-12.9374737206007,
115.38804700087)) ;
#185154=CARTESIAN_POINT('Ctrl Pts',(-16.3424008062689,-12.937473634477,
115.363815996629)) ;
#185155=CARTESIAN_POINT('Ctrl Pts',(-16.3639160111054,-12.9691613747719,
115.429347837265)) ;
#185156=CARTESIAN_POINT('Ctrl Pts',(-16.3272518685413,-13.2488218748192,
115.353233566025)) ;
#185157=CARTESIAN_POINT('Ctrl Pts',(-16.3506225649115,-13.2610313034061,
115.424416934386)) ;
#185158=CARTESIAN_POINT('Ctrl Pts',(-16.2768187165298,-13.2610314022195,
115.448647960959)) ;
#185159=CARTESIAN_POINT('Ctrl Pts',(-16.203014868148,-13.2610315010329,
115.472878987532)) ;
#185160=CARTESIAN_POINT('Ctrl Pts',(-16.1796441717778,-13.248822072446,
115.401695619171)) ;
#185161=CARTESIAN_POINT('Ctrl Pts',(-16.1562734754075,-13.2366126438591,
115.330512250809)) ;
#185162=CARTESIAN_POINT('Ctrl Pts',(-16.2300773237893,-13.2366125450457,
115.306281224236)) ;
#185163=CARTESIAN_POINT('Ctrl Pts',(-16.303881172171,-13.2366124462323,
115.282050197664)) ;
#185164=CARTESIAN_POINT('Ctrl Pts',(-16.3272518685413,-13.2488218748192,
115.353233566025)) ;
#185165=CARTESIAN_POINT('Ctrl Pts',(-16.3147673231041,-13.5399745855604,
115.350672599282)) ;
#185166=CARTESIAN_POINT('Ctrl Pts',(-16.3383100754923,-13.5318747593251,
115.422380022441)) ;
#185167=CARTESIAN_POINT('Ctrl Pts',(-16.2645062356431,-13.5318748625201,
115.446611075003)) ;
#185168=CARTESIAN_POINT('Ctrl Pts',(-16.1907023957939,-13.5318749657152,
115.470842127564)) ;
#185169=CARTESIAN_POINT('Ctrl Pts',(-16.1671596434057,-13.5399747919505,
115.399134704405)) ;
#185170=CARTESIAN_POINT('Ctrl Pts',(-16.1436168910174,-13.5480746181859,
115.327427281246)) ;
#185171=CARTESIAN_POINT('Ctrl Pts',(-16.2174207308666,-13.5480745149908,
115.303196228684)) ;
#185172=CARTESIAN_POINT('Ctrl Pts',(-16.2912245707158,-13.5480744117958,
115.278965176123)) ;
#185173=CARTESIAN_POINT('Ctrl Pts',(-16.3147673231041,-13.5399745855604,
115.350672599282)) ;
#185174=CARTESIAN_POINT('Ctrl Pts',(-16.3264516296071,-13.8224630035439,
115.42174671114)) ;
#185175=CARTESIAN_POINT('Ctrl Pts',(-16.3484790098761,-13.7946290334854,
115.488838555276)) ;
#185176=CARTESIAN_POINT('Ctrl Pts',(-16.2746751787747,-13.7946291324029,
115.513069634482)) ;
#185177=CARTESIAN_POINT('Ctrl Pts',(-16.2008713476733,-13.7946292313203,
115.537300713688)) ;
#185178=CARTESIAN_POINT('Ctrl Pts',(-16.1788439674043,-13.8224632013788,
115.470208869552)) ;
#185179=CARTESIAN_POINT('Ctrl Pts',(-16.1568165871353,-13.8502971714373,
115.403117025416)) ;
#185180=CARTESIAN_POINT('Ctrl Pts',(-16.2306204182367,-13.8502970725198,
115.378885946209)) ;
#185181=CARTESIAN_POINT('Ctrl Pts',(-16.3044242493381,-13.8502969736024,
115.354654867003)) ;
#185182=CARTESIAN_POINT('Ctrl Pts',(-16.3264516296071,-13.8224630035439,
115.42174671114)) ;
#185183=CARTESIAN_POINT('Ctrl Pts',(-16.3605782808278,-14.0755037719121,
115.561087662163)) ;
#185184=CARTESIAN_POINT('Ctrl Pts',(-16.3795230750246,-14.0299625115252,
115.618790446467)) ;
#185185=CARTESIAN_POINT('Ctrl Pts',(-16.3057192519711,-14.0299625976229,
115.643021550186)) ;
#185186=CARTESIAN_POINT('Ctrl Pts',(-16.2319154289175,-14.0299626837205,
115.667252653904)) ;
#185187=CARTESIAN_POINT('Ctrl Pts',(-16.2129706347207,-14.0755039441074,
115.6095498696)) ;
#185188=CARTESIAN_POINT('Ctrl Pts',(-16.1940258405239,-14.1210452044942,
115.551847085295)) ;
#185189=CARTESIAN_POINT('Ctrl Pts',(-16.2678296635774,-14.1210451183966,
115.527615981577)) ;
#185190=CARTESIAN_POINT('Ctrl Pts',(-16.3416334866309,-14.121045032299,
115.503384877858)) ;
#185191=CARTESIAN_POINT('Ctrl Pts',(-16.3605782808278,-14.0755037719121,
115.561087662163)) ;
#185192=CARTESIAN_POINT('Ctrl Pts',(-16.4144569396317,-14.2826234653696,
115.760827462951)) ;
#185193=CARTESIAN_POINT('Ctrl Pts',(-16.4289310027573,-14.2225542775354,
115.804913121755)) ;
#185194=CARTESIAN_POINT('Ctrl Pts',(-16.3551271862276,-14.2225543432862,
115.829144245344)) ;
#185195=CARTESIAN_POINT('Ctrl Pts',(-16.2813233696978,-14.222554409037,
115.853375368933)) ;
#185196=CARTESIAN_POINT('Ctrl Pts',(-16.2668493065721,-14.2826235968712,
115.809289710129)) ;
#185197=CARTESIAN_POINT('Ctrl Pts',(-16.2523752434465,-14.3426927847054,
115.765204051324)) ;
#185198=CARTESIAN_POINT('Ctrl Pts',(-16.3261790599763,-14.3426927189546,
115.740972927735)) ;
#185199=CARTESIAN_POINT('Ctrl Pts',(-16.399982876506,-14.3426926532038,
115.716741804146)) ;
#185200=CARTESIAN_POINT('Ctrl Pts',(-16.4144569396317,-14.2826234653696,
115.760827462951)) ;
#185201=CARTESIAN_POINT('Ctrl Pts',(-16.4823985818851,-14.4260980932151,
116.003005069228)) ;
#185202=CARTESIAN_POINT('Ctrl Pts',(-16.4914213499877,-14.3559233104312,
116.030486962966)) ;
#185203=CARTESIAN_POINT('Ctrl Pts',(-16.4176175377613,-14.3559233508218,
116.054718099662)) ;
#185204=CARTESIAN_POINT('Ctrl Pts',(-16.3438137255349,-14.3559233912124,
116.078949236359)) ;
#185205=CARTESIAN_POINT('Ctrl Pts',(-16.3347909574323,-14.4260981739963,
116.05146734262)) ;
#185206=CARTESIAN_POINT('Ctrl Pts',(-16.3257681893297,-14.4962729567803,
116.023985448882)) ;
#185207=CARTESIAN_POINT('Ctrl Pts',(-16.3995720015561,-14.4962729163896,
115.999754312186)) ;
#185208=CARTESIAN_POINT('Ctrl Pts',(-16.4733758137825,-14.496272875999,
115.975523175489)) ;
#185209=CARTESIAN_POINT('Ctrl Pts',(-16.4823985818851,-14.4260980932151,
116.003005069228)) ;
#185210=CARTESIAN_POINT('Ctrl Pts',(-16.5601782984998,-14.4987580687002,
116.275521075133)) ;
#185211=CARTESIAN_POINT('Ctrl Pts',(-16.5630474354816,-14.4234055963817,
116.284260001402)) ;
#185212=CARTESIAN_POINT('Ctrl Pts',(-16.4892436248514,-14.423405608344,
116.308491142959)) ;
#185213=CARTESIAN_POINT('Ctrl Pts',(-16.4154398142211,-14.4234056203062,
116.332722284517)) ;
#185214=CARTESIAN_POINT('Ctrl Pts',(-16.4125706772393,-14.4987580926247,
116.323983358248)) ;
#185215=CARTESIAN_POINT('Ctrl Pts',(-16.4097015402575,-14.5741105649432,
116.315244431979)) ;
#185216=CARTESIAN_POINT('Ctrl Pts',(-16.4835053508878,-14.5741105529809,
116.291013290421)) ;
#185217=CARTESIAN_POINT('Ctrl Pts',(-16.557309161518,-14.5741105410186,
116.266782148863)) ;
#185218=CARTESIAN_POINT('Ctrl Pts',(-16.5601782984998,-14.4987580687002,
116.275521075133)) ;
#185219=CARTESIAN_POINT('Ctrl Pts',(-16.6403598990909,-14.4933400096758,
116.55514982289)) ;
#185220=CARTESIAN_POINT('Ctrl Pts',(-16.636902579237,-14.4182534186233,
116.544619382463)) ;
#185221=CARTESIAN_POINT('Ctrl Pts',(-16.5630987675235,-14.4182534027344,
116.568850520722)) ;
#185222=CARTESIAN_POINT('Ctrl Pts',(-16.48929495581,-14.4182533868454,116.59308165898)) ;
#185223=CARTESIAN_POINT('Ctrl Pts',(-16.4927522756639,-14.493339977898,
116.603612099407)) ;
#185224=CARTESIAN_POINT('Ctrl Pts',(-16.4962095955177,-14.5684265689505,
116.614142539833)) ;
#185225=CARTESIAN_POINT('Ctrl Pts',(-16.5700134072313,-14.5684265848394,
116.589911401574)) ;
#185226=CARTESIAN_POINT('Ctrl Pts',(-16.6438172189447,-14.5684266007284,
116.565680263316)) ;
#185227=CARTESIAN_POINT('Ctrl Pts',(-16.6403598990909,-14.4933400096758,
116.55514982289)) ;
#185228=CARTESIAN_POINT('Ctrl Pts',(-16.716958755928,-14.4113489345642,
116.823901650034)) ;
#185229=CARTESIAN_POINT('Ctrl Pts',(-16.7074149546365,-14.3418743538158,
116.794832769273)) ;
#185230=CARTESIAN_POINT('Ctrl Pts',(-16.6336111393608,-14.3418743129385,
116.819063896682)) ;
#185231=CARTESIAN_POINT('Ctrl Pts',(-16.559807324085,-14.3418742720612,
116.84329502409)) ;
#185232=CARTESIAN_POINT('Ctrl Pts',(-16.5693511253766,-14.4113488528096,
116.872363904851)) ;
#185233=CARTESIAN_POINT('Ctrl Pts',(-16.5788949266681,-14.4808234335579,
116.901432785613)) ;
#185234=CARTESIAN_POINT('Ctrl Pts',(-16.6526987419438,-14.4808234744352,
116.877201658204)) ;
#185235=CARTESIAN_POINT('Ctrl Pts',(-16.7265025572196,-14.4808235153125,
116.852970530796)) ;
#185236=CARTESIAN_POINT('Ctrl Pts',(-16.716958755928,-14.4113489345642,
116.823901650034)) ;
#185237=CARTESIAN_POINT('Ctrl Pts',(-16.7838983833734,-14.2570982982162,
117.06340817062)) ;
#185238=CARTESIAN_POINT('Ctrl Pts',(-16.768929594028,-14.1982882942638,
117.017815651682)) ;
#185239=CARTESIAN_POINT('Ctrl Pts',(-16.6951257728925,-14.1982882346942,
117.042046761243)) ;
#185240=CARTESIAN_POINT('Ctrl Pts',(-16.6213219517571,-14.1982881751247,
117.066277870804)) ;
#185241=CARTESIAN_POINT('Ctrl Pts',(-16.6362907411025,-14.2570981790771,
117.111870389742)) ;
#185242=CARTESIAN_POINT('Ctrl Pts',(-16.651259530448,-14.3159081830295,
117.15746290868)) ;
#185243=CARTESIAN_POINT('Ctrl Pts',(-16.7250633515835,-14.3159082425991,
117.133231799119)) ;
#185244=CARTESIAN_POINT('Ctrl Pts',(-16.7988671727189,-14.3159083021687,
117.109000689558)) ;
#185245=CARTESIAN_POINT('Ctrl Pts',(-16.7838983833734,-14.2570982982162,
117.06340817062)) ;
#185246=CARTESIAN_POINT('Ctrl Pts',(-16.834856327063,-14.044633200838,117.25389164477)) ;
#185247=CARTESIAN_POINT('Ctrl Pts',(-16.8155774044462,-14.000569128791,
117.195171155415)) ;
#185248=CARTESIAN_POINT('Ctrl Pts',(-16.7417735767459,-14.0005690563028,
117.219402244981)) ;
#185249=CARTESIAN_POINT('Ctrl Pts',(-16.6679697490455,-14.0005689838146,
117.243633334546)) ;
#185250=CARTESIAN_POINT('Ctrl Pts',(-16.6872486716623,-14.0446330558616,
117.3023538239)) ;
#185251=CARTESIAN_POINT('Ctrl Pts',(-16.7065275942791,-14.0886971279086,
117.361074313255)) ;
#185252=CARTESIAN_POINT('Ctrl Pts',(-16.7803314219795,-14.0886972003968,
117.336843223689)) ;
#185253=CARTESIAN_POINT('Ctrl Pts',(-16.8541352496798,-14.088697272885,
117.312612134124)) ;
#185254=CARTESIAN_POINT('Ctrl Pts',(-16.834856327063,-14.044633200838,117.25389164477)) ;
#185255=CARTESIAN_POINT('Ctrl Pts',(-16.8663296783061,-13.785410087343,
117.385342864865)) ;
#185256=CARTESIAN_POINT('Ctrl Pts',(-16.8440877467271,-13.7593778661625,
117.31759752844)) ;
#185257=CARTESIAN_POINT('Ctrl Pts',(-16.7702839116196,-13.7593777900464,
117.341828595444)) ;
#185258=CARTESIAN_POINT('Ctrl Pts',(-16.6964800765121,-13.7593777139303,
117.366059662449)) ;
#185259=CARTESIAN_POINT('Ctrl Pts',(-16.718722008091,-13.7854099351107,
117.433804998873)) ;
#185260=CARTESIAN_POINT('Ctrl Pts',(-16.74096393967,-13.8114421562912,117.501550335298)) ;
#185261=CARTESIAN_POINT('Ctrl Pts',(-16.8147677747775,-13.8114422324073,
117.477319268294)) ;
#185262=CARTESIAN_POINT('Ctrl Pts',(-16.888571609885,-13.8114423085234,
117.45308820129)) ;
#185263=CARTESIAN_POINT('Ctrl Pts',(-16.8663296783061,-13.785410087343,
117.385342864865)) ;
#185264=CARTESIAN_POINT('Ctrl Pts',(-16.8748051062788,-13.5013707464361,
117.446525551891)) ;
#185265=CARTESIAN_POINT('Ctrl Pts',(-16.8512060293604,-13.4951307017579,
117.374646569865)) ;
#185266=CARTESIAN_POINT('Ctrl Pts',(-16.7774021874673,-13.4951306279953,
117.398877616201)) ;
#185267=CARTESIAN_POINT('Ctrl Pts',(-16.7035983455741,-13.4951305542326,
117.423108662538)) ;
#185268=CARTESIAN_POINT('Ctrl Pts',(-16.7271974224926,-13.5013705989108,
117.494987644563)) ;
#185269=CARTESIAN_POINT('Ctrl Pts',(-16.7507964994111,-13.507610643589,
117.566866626589)) ;
#185270=CARTESIAN_POINT('Ctrl Pts',(-16.8246003413042,-13.5076107173517,
117.542635580253)) ;
#185271=CARTESIAN_POINT('Ctrl Pts',(-16.8984041831973,-13.5076107911143,
117.518404533917)) ;
#185272=CARTESIAN_POINT('Ctrl Pts',(-16.8748051062788,-13.5013707464361,
117.446525551891)) ;
#185273=CARTESIAN_POINT('Ctrl Pts',(-16.8588838729658,-13.209135818783,
117.433694846988)) ;
#185274=CARTESIAN_POINT('Ctrl Pts',(-16.8356225305324,-13.2232901390273,
117.362844549901)) ;
#185275=CARTESIAN_POINT('Ctrl Pts',(-16.7618186830723,-13.2232900762476,
117.387075579282)) ;
#185276=CARTESIAN_POINT('Ctrl Pts',(-16.6880148356122,-13.2232900134679,
117.411306608662)) ;
#185277=CARTESIAN_POINT('Ctrl Pts',(-16.7112761780455,-13.2091356932237,
117.482156905748)) ;
#185278=CARTESIAN_POINT('Ctrl Pts',(-16.7345375204789,-13.1949813729794,
117.553007202835)) ;
#185279=CARTESIAN_POINT('Ctrl Pts',(-16.8083413679391,-13.1949814357591,
117.528776173455)) ;
#185280=CARTESIAN_POINT('Ctrl Pts',(-16.8821452153992,-13.1949814985388,
117.504545144075)) ;
#185281=CARTESIAN_POINT('Ctrl Pts',(-16.8588838729658,-13.209135818783,
117.433694846988)) ;
#185282=CARTESIAN_POINT('Ctrl Pts',(-16.8195694538494,-12.935507537228,
117.349125089638)) ;
#185283=CARTESIAN_POINT('Ctrl Pts',(-16.7982901950563,-12.9687880563088,
117.284311899622)) ;
#185284=CARTESIAN_POINT('Ctrl Pts',(-16.7244863433739,-12.9687880043352,
117.308542916142)) ;
#185285=CARTESIAN_POINT('Ctrl Pts',(-16.6506824916915,-12.9687879523617,
117.332773932661)) ;
#185286=CARTESIAN_POINT('Ctrl Pts',(-16.6719617504845,-12.9355074332809,
117.397587122678)) ;
#185287=CARTESIAN_POINT('Ctrl Pts',(-16.6932410092776,-12.9022269142001,
117.462400312694)) ;
#185288=CARTESIAN_POINT('Ctrl Pts',(-16.76704486096,-12.9022269661736,117.438169296175)) ;
#185289=CARTESIAN_POINT('Ctrl Pts',(-16.8408487126425,-12.9022270181472,
117.413938279655)) ;
#185290=CARTESIAN_POINT('Ctrl Pts',(-16.8195694538494,-12.935507537228,
117.349125089638)) ;
#185291=CARTESIAN_POINT('Ctrl Pts',(-16.7579313251563,-12.6930981261278,
117.197023501417)) ;
#185292=CARTESIAN_POINT('Ctrl Pts',(-16.7401858356171,-12.7433547054021,
117.142973602577)) ;
#185293=CARTESIAN_POINT('Ctrl Pts',(-16.6663819820211,-12.7433546700873,
117.167204613268)) ;
#185294=CARTESIAN_POINT('Ctrl Pts',(-16.5925781284251,-12.7433546347726,
117.191435623959)) ;
#185295=CARTESIAN_POINT('Ctrl Pts',(-16.6103236179643,-12.6930980554983,
117.2454855228)) ;
#185296=CARTESIAN_POINT('Ctrl Pts',(-16.6280691075034,-12.642841476224,
117.299535421641)) ;
#185297=CARTESIAN_POINT('Ctrl Pts',(-16.7018729610994,-12.6428415115388,
117.27530441095)) ;
#185298=CARTESIAN_POINT('Ctrl Pts',(-16.7756768146954,-12.6428415468535,
117.251073400258)) ;
#185299=CARTESIAN_POINT('Ctrl Pts',(-16.7579313251563,-12.6930981261278,
117.197023501417)) ;
#185300=CARTESIAN_POINT('Ctrl Pts',(-16.6787204475409,-12.5044954568888,
116.991078724866)) ;
#185301=CARTESIAN_POINT('Ctrl Pts',(-16.6657479281678,-12.5679966014652,
116.951566523176)) ;
#185302=CARTESIAN_POINT('Ctrl Pts',(-16.5919440739595,-12.5679965800268,
116.975797532002)) ;
#185303=CARTESIAN_POINT('Ctrl Pts',(-16.5181402197511,-12.5679965585884,
117.000028540829)) ;
#185304=CARTESIAN_POINT('Ctrl Pts',(-16.5311127391241,-12.504495414012,
117.039540742518)) ;
#185305=CARTESIAN_POINT('Ctrl Pts',(-16.5440852584971,-12.4409942694355,
117.079052944207)) ;
#185306=CARTESIAN_POINT('Ctrl Pts',(-16.6178891127055,-12.440994290874,
117.054821935381)) ;
#185307=CARTESIAN_POINT('Ctrl Pts',(-16.6916929669139,-12.4409943123124,
117.030590926555)) ;
#185308=CARTESIAN_POINT('Ctrl Pts',(-16.6787204475409,-12.5044954568888,
116.991078724866)) ;
#185309=CARTESIAN_POINT('Ctrl Pts',(-16.5854915695396,-12.3799491141259,
116.742785488435)) ;
#185310=CARTESIAN_POINT('Ctrl Pts',(-16.5782707497597,-12.4522433406483,
116.720792035876)) ;
#185311=CARTESIAN_POINT('Ctrl Pts',(-16.5044668972683,-12.4522433323691,
116.745023049931)) ;
#185312=CARTESIAN_POINT('Ctrl Pts',(-16.4306630447769,-12.4522433240898,
116.769254063987)) ;
#185313=CARTESIAN_POINT('Ctrl Pts',(-16.4378838645568,-12.3799490975675,
116.791247516546)) ;
#185314=CARTESIAN_POINT('Ctrl Pts',(-16.4451046843367,-12.3076548710451,
116.813240969105)) ;
#185315=CARTESIAN_POINT('Ctrl Pts',(-16.5189085368281,-12.3076548793244,
116.789009955049)) ;
#185316=CARTESIAN_POINT('Ctrl Pts',(-16.5927123893195,-12.3076548876036,
116.764778940994)) ;
#185317=CARTESIAN_POINT('Ctrl Pts',(-16.5854915695396,-12.3799491141259,
116.742785488435)) ;
#185318=CARTESIAN_POINT('Ctrl Pts',(-16.4858486944927,-12.3308555788642,
116.474611823742)) ;
#185319=CARTESIAN_POINT('Ctrl Pts',(-16.4848434460203,-12.4066867963508,
116.471549998639)) ;
#185320=CARTESIAN_POINT('Ctrl Pts',(-16.4110395953124,-12.4066867960904,
116.495781018126)) ;
#185321=CARTESIAN_POINT('Ctrl Pts',(-16.3372357446044,-12.4066867958299,
116.520012037614)) ;
#185322=CARTESIAN_POINT('Ctrl Pts',(-16.3382409930768,-12.3308555783432,
116.523073862718)) ;
#185323=CARTESIAN_POINT('Ctrl Pts',(-16.3392462415492,-12.2550243608565,
116.526135687821)) ;
#185324=CARTESIAN_POINT('Ctrl Pts',(-16.4130500922572,-12.255024361117,
116.501904668333)) ;
#185325=CARTESIAN_POINT('Ctrl Pts',(-16.4868539429651,-12.2550243613775,
116.477673648845)) ;
#185326=CARTESIAN_POINT('Ctrl Pts',(-16.4858486944927,-12.3308555788642,
116.474611823742)) ;
#185327=CARTESIAN_POINT('Ctrl Pts',(-16.3849423803949,-12.3590358220882,
116.202733804349)) ;
#185328=CARTESIAN_POINT('Ctrl Pts',(-16.3902473975342,-12.4330140750954,
116.218892030289)) ;
#185329=CARTESIAN_POINT('Ctrl Pts',(-16.3164435493756,-12.4330140793916,
116.243123057542)) ;
#185330=CARTESIAN_POINT('Ctrl Pts',(-16.242639701217,-12.4330140836878,
116.267354084794)) ;
#185331=CARTESIAN_POINT('Ctrl Pts',(-16.2373346840777,-12.3590358306806,
116.251195858855)) ;
#185332=CARTESIAN_POINT('Ctrl Pts',(-16.2320296669384,-12.2850575776733,
116.235037632915)) ;
#185333=CARTESIAN_POINT('Ctrl Pts',(-16.305833515097,-12.2850575733772,
116.210806605662)) ;
#185334=CARTESIAN_POINT('Ctrl Pts',(-16.3796373632556,-12.285057569081,
116.186575578409)) ;
#185335=CARTESIAN_POINT('Ctrl Pts',(-16.3849423803949,-12.3590358220882,
116.202733804349)) ;
#185336=CARTESIAN_POINT('Ctrl Pts',(-16.2895213068132,-12.4632787296656,
115.947588740383)) ;
#185337=CARTESIAN_POINT('Ctrl Pts',(-16.3007626967771,-12.5300899100408,
115.981828200251)) ;
#185338=CARTESIAN_POINT('Ctrl Pts',(-16.2269588510408,-12.5300899147854,
116.006059234882)) ;
#185339=CARTESIAN_POINT('Ctrl Pts',(-16.1531550053045,-12.5300899195299,
116.030290269513)) ;
#185340=CARTESIAN_POINT('Ctrl Pts',(-16.1419136153406,-12.4632787391547,
115.996050809645)) ;
#185341=CARTESIAN_POINT('Ctrl Pts',(-16.1306722253766,-12.3964675587795,
115.961811349777)) ;
#185342=CARTESIAN_POINT('Ctrl Pts',(-16.2044760711129,-12.396467554035,
115.937580315146)) ;
#185343=CARTESIAN_POINT('Ctrl Pts',(-16.2782799168492,-12.3964675492904,
115.913349280515)) ;
#185344=CARTESIAN_POINT('Ctrl Pts',(-16.2895213068132,-12.4632787296656,
115.947588740383)) ;
#185345=CARTESIAN_POINT('Ctrl Pts',(-16.205735751125,-12.6363587431469,
115.727927057703)) ;
#185346=CARTESIAN_POINT('Ctrl Pts',(-16.2221091925139,-12.6911848598895,
115.77779791827)) ;
#185347=CARTESIAN_POINT('Ctrl Pts',(-16.1483053485157,-12.6911848623011,
115.802028958194)) ;
#185348=CARTESIAN_POINT('Ctrl Pts',(-16.0745015045173,-12.6911848647128,
115.826259998119)) ;
#185349=CARTESIAN_POINT('Ctrl Pts',(-16.0581280631284,-12.6363587479702,
115.776389137552)) ;
#185350=CARTESIAN_POINT('Ctrl Pts',(-16.0417546217395,-12.5815326312277,
115.726518276985)) ;
#185351=CARTESIAN_POINT('Ctrl Pts',(-16.1155584657378,-12.5815326288161,
115.70228723706)) ;
#185352=CARTESIAN_POINT('Ctrl Pts',(-16.1893623097361,-12.5815326264044,
115.678056197136)) ;
#185353=CARTESIAN_POINT('Ctrl Pts',(-16.205735751125,-12.6363587431469,
115.727927057703)) ;
#185354=CARTESIAN_POINT('Ctrl Pts',(-16.139154962057,-12.864158222785,115.560475584254)) ;
#185355=CARTESIAN_POINT('Ctrl Pts',(-16.1594705534534,-12.9031598637825,
115.622353597751)) ;
#185356=CARTESIAN_POINT('Ctrl Pts',(-16.0856667102229,-12.9031598633717,
115.646584640014)) ;
#185357=CARTESIAN_POINT('Ctrl Pts',(-16.0118628669925,-12.9031598629608,
115.670815682277)) ;
#185358=CARTESIAN_POINT('Ctrl Pts',(-15.9915472755961,-12.8641582219634,
115.60893766878)) ;
#185359=CARTESIAN_POINT('Ctrl Pts',(-15.9712316841997,-12.8251565809659,
115.547059655283)) ;
#185360=CARTESIAN_POINT('Ctrl Pts',(-16.0450355274302,-12.8251565813767,
115.52282861302)) ;
#185361=CARTESIAN_POINT('Ctrl Pts',(-16.1188393706606,-12.8251565817875,
115.498597570757)) ;
#185362=CARTESIAN_POINT('Ctrl Pts',(-16.139154962057,-12.864158222785,115.560475584254)) ;
#185363=CARTESIAN_POINT('Ctrl Pts',(-16.0930899176048,-13.1343225359667,
115.455877741141)) ;
#185364=CARTESIAN_POINT('Ctrl Pts',(-16.1159137349886,-13.1545167875365,
115.525395406345)) ;
#185365=CARTESIAN_POINT('Ctrl Pts',(-16.0421098918826,-13.1545167844315,
115.549626448987)) ;
#185366=CARTESIAN_POINT('Ctrl Pts',(-15.9683060487766,-13.1545167813264,
115.57385749163)) ;
#185367=CARTESIAN_POINT('Ctrl Pts',(-15.9454822313929,-13.1343225297566,
115.504339826425)) ;
#185368=CARTESIAN_POINT('Ctrl Pts',(-15.9226584140091,-13.1141282781868,
115.434822161221)) ;
#185369=CARTESIAN_POINT('Ctrl Pts',(-15.9964622571151,-13.1141282812919,
115.410591118579)) ;
#185370=CARTESIAN_POINT('Ctrl Pts',(-16.0702661002211,-13.114128284397,
115.386360075936)) ;
#185371=CARTESIAN_POINT('Ctrl Pts',(-16.0930899176048,-13.1343225359667,
115.455877741141)) ;
#185372=CARTESIAN_POINT('Ctrl Pts',(-16.0709494733631,-13.4205967944479,
115.423599773257)) ;
#185373=CARTESIAN_POINT('Ctrl Pts',(-16.094625220264,-13.4208311388444,
115.495712278311)) ;
#185374=CARTESIAN_POINT('Ctrl Pts',(-16.0208213768168,-13.4208311356135,
115.519943319914)) ;
#185375=CARTESIAN_POINT('Ctrl Pts',(-15.9470175333695,-13.4208311323827,
115.544174361517)) ;
#185376=CARTESIAN_POINT('Ctrl Pts',(-15.9233417864687,-13.4205967879863,
115.472061856462)) ;
#185377=CARTESIAN_POINT('Ctrl Pts',(-15.8996660395678,-13.4203624435898,
115.399949351408)) ;
#185378=CARTESIAN_POINT('Ctrl Pts',(-15.9734698830151,-13.4203624468207,
115.375718309805)) ;
#185379=CARTESIAN_POINT('Ctrl Pts',(-16.0472737264623,-13.4203624500515,
115.351487268202)) ;
#185380=CARTESIAN_POINT('Ctrl Pts',(-16.0709494733631,-13.4205967944479,
115.423599773257)) ;
#185381=CARTESIAN_POINT('Ctrl Pts',(-16.0728139419201,-13.7102521447362,
115.464896490808)) ;
#185382=CARTESIAN_POINT('Ctrl Pts',(-16.0956574052163,-13.6902603542672,
115.534473994251)) ;
#185383=CARTESIAN_POINT('Ctrl Pts',(-16.021853561637,-13.6902603532413,
115.558705035452)) ;
#185384=CARTESIAN_POINT('Ctrl Pts',(-15.9480497180577,-13.6902603522153,
115.582936076653)) ;
#185385=CARTESIAN_POINT('Ctrl Pts',(-15.9252062547615,-13.7102521426842,
115.51335857321)) ;
#185386=CARTESIAN_POINT('Ctrl Pts',(-15.9023627914653,-13.7302439331532,
115.443781069767)) ;
#185387=CARTESIAN_POINT('Ctrl Pts',(-15.9761666350445,-13.7302439341791,
115.419550028566)) ;
#185388=CARTESIAN_POINT('Ctrl Pts',(-16.0499704786238,-13.7302439352051,
115.395318987366)) ;
#185389=CARTESIAN_POINT('Ctrl Pts',(-16.0728139419201,-13.7102521447362,
115.464896490808)) ;
#185390=CARTESIAN_POINT('Ctrl Pts',(-16.0981489870159,-13.9772668612757,
115.577456504473)) ;
#185391=CARTESIAN_POINT('Ctrl Pts',(-16.1185243546186,-13.9386012749513,
115.639516586589)) ;
#185392=CARTESIAN_POINT('Ctrl Pts',(-16.0447205114953,-13.9386012773307,
115.663747629179)) ;
#185393=CARTESIAN_POINT('Ctrl Pts',(-15.970916668372,-13.9386012797101,
115.687978671768)) ;
#185394=CARTESIAN_POINT('Ctrl Pts',(-15.9505413007694,-13.9772668660344,
115.625918589653)) ;
#185395=CARTESIAN_POINT('Ctrl Pts',(-15.9301659331668,-14.0159324523587,
115.563858507537)) ;
#185396=CARTESIAN_POINT('Ctrl Pts',(-16.0039697762901,-14.0159324499793,
115.539627464947)) ;
#185397=CARTESIAN_POINT('Ctrl Pts',(-16.0777736194133,-14.0159324476,115.515396422358)) ;
#185398=CARTESIAN_POINT('Ctrl Pts',(-16.0981489870159,-13.9772668612757,
115.577456504473)) ;
#185399=CARTESIAN_POINT('Ctrl Pts',(-16.1444518589437,-14.2052355202481,
115.754036564004)) ;
#185400=CARTESIAN_POINT('Ctrl Pts',(-16.1608882398116,-14.1505953290783,
115.804099127967)) ;
#185401=CARTESIAN_POINT('Ctrl Pts',(-16.0870843981636,-14.1505953352011,
115.82833017505)) ;
#185402=CARTESIAN_POINT('Ctrl Pts',(-16.0132805565157,-14.150595341324,
115.852561222133)) ;
#185403=CARTESIAN_POINT('Ctrl Pts',(-15.9968441756478,-14.2052355324938,
115.802498658171)) ;
#185404=CARTESIAN_POINT('Ctrl Pts',(-15.9804077947799,-14.2598757236637,
115.752436094208)) ;
#185405=CARTESIAN_POINT('Ctrl Pts',(-16.0542116364279,-14.2598757175408,
115.728205047125)) ;
#185406=CARTESIAN_POINT('Ctrl Pts',(-16.1280154780758,-14.259875711418,
115.703974000042)) ;
#185407=CARTESIAN_POINT('Ctrl Pts',(-16.1444518589437,-14.2052355202481,
115.754036564004)) ;
#185408=CARTESIAN_POINT('Ctrl Pts',(-16.2073387806654,-14.3759216033723,
115.980973148425)) ;
#185409=CARTESIAN_POINT('Ctrl Pts',(-16.2186756236728,-14.3092842663228,
116.015503342754)) ;
#185410=CARTESIAN_POINT('Ctrl Pts',(-16.1448717841291,-14.309284273676,
116.039734396247)) ;
#185411=CARTESIAN_POINT('Ctrl Pts',(-16.0710679445855,-14.3092842810292,
116.06396544974)) ;
#185412=CARTESIAN_POINT('Ctrl Pts',(-16.0597311015782,-14.3759216180787,
116.02943525541)) ;
#185413=CARTESIAN_POINT('Ctrl Pts',(-16.0483942585708,-14.4425589551282,
115.994905061081)) ;
#185414=CARTESIAN_POINT('Ctrl Pts',(-16.1221980981144,-14.442558947775,
115.970674007588)) ;
#185415=CARTESIAN_POINT('Ctrl Pts',(-16.196001937658,-14.4425589404218,
115.946442954095)) ;
#185416=CARTESIAN_POINT('Ctrl Pts',(-16.2073387806654,-14.3759216033723,
115.980973148425)) ;
#185417=CARTESIAN_POINT('Ctrl Pts',(-16.2818319731242,-14.478404639523,
116.243331183075)) ;
#185418=CARTESIAN_POINT('Ctrl Pts',(-16.2872500889696,-14.404515033937,
116.259833889309)) ;
#185419=CARTESIAN_POINT('Ctrl Pts',(-16.2134462521354,-14.4045150394246,
116.284064951054)) ;
#185420=CARTESIAN_POINT('Ctrl Pts',(-16.1396424153012,-14.4045150449122,
116.308296012799)) ;
#185421=CARTESIAN_POINT('Ctrl Pts',(-16.1342242994558,-14.4784046504982,
116.291793306565)) ;
#185422=CARTESIAN_POINT('Ctrl Pts',(-16.1288061836104,-14.5522942560841,
116.275290600331)) ;
#185423=CARTESIAN_POINT('Ctrl Pts',(-16.2026100204446,-14.5522942505966,
116.251059538586)) ;
#185424=CARTESIAN_POINT('Ctrl Pts',(-16.2764138572788,-14.552294245109,
116.226828476841)) ;
#185425=CARTESIAN_POINT('Ctrl Pts',(-16.2818319731242,-14.478404639523,
116.243331183075)) ;
#185426=CARTESIAN_POINT('Ctrl Pts',(-16.3616827803532,-14.505089399069,
116.521964167678)) ;
#185427=CARTESIAN_POINT('Ctrl Pts',(-16.3608004973226,-14.4292297938268,
116.519276875353)) ;
#185428=CARTESIAN_POINT('Ctrl Pts',(-16.2869966631093,-14.4292297934085,
116.543507945081)) ;
#185429=CARTESIAN_POINT('Ctrl Pts',(-16.2131928288959,-14.4292297929902,
116.567739014809)) ;
#185430=CARTESIAN_POINT('Ctrl Pts',(-16.2140751119266,-14.5050893982325,
116.570426307133)) ;
#185431=CARTESIAN_POINT('Ctrl Pts',(-16.2149573949572,-14.5809490034747,
116.573113599458)) ;
#185432=CARTESIAN_POINT('Ctrl Pts',(-16.2887612291705,-14.580949003893,
116.54888252973)) ;
#185433=CARTESIAN_POINT('Ctrl Pts',(-16.3625650633839,-14.5809490043113,
116.524651460002)) ;
#185434=CARTESIAN_POINT('Ctrl Pts',(-16.3616827803532,-14.505089399069,
116.521964167678)) ;
#185435=CARTESIAN_POINT('Ctrl Pts',(-16.4409954196579,-14.4533114988155,
116.799196663572)) ;
#185436=CARTESIAN_POINT('Ctrl Pts',(-16.4338362755014,-14.3809567964235,
116.777391064824)) ;
#185437=CARTESIAN_POINT('Ctrl Pts',(-16.3600324439956,-14.3809567849074,
116.801622142798)) ;
#185438=CARTESIAN_POINT('Ctrl Pts',(-16.2862286124899,-14.3809567733913,
116.825853220773)) ;
#185439=CARTESIAN_POINT('Ctrl Pts',(-16.2933877566465,-14.4533114757834,
116.847658819521)) ;
#185440=CARTESIAN_POINT('Ctrl Pts',(-16.300546900803,-14.5256661781754,
116.869464418269)) ;
#185441=CARTESIAN_POINT('Ctrl Pts',(-16.3743507323088,-14.5256661896915,
116.845233340294)) ;
#185442=CARTESIAN_POINT('Ctrl Pts',(-16.4481545638145,-14.5256662012075,
116.821002262319)) ;
#185443=CARTESIAN_POINT('Ctrl Pts',(-16.4409954196579,-14.4533114988155,
116.799196663572)) ;
#185444=CARTESIAN_POINT('Ctrl Pts',(-16.5121187619909,-14.3281114059052,
117.051140482076)) ;
#185445=CARTESIAN_POINT('Ctrl Pts',(-16.4992528101108,-14.2643939997168,
117.011952867652)) ;
#185446=CARTESIAN_POINT('Ctrl Pts',(-16.4254489791142,-14.26439397447,117.036183947178)) ;
#185447=CARTESIAN_POINT('Ctrl Pts',(-16.3516451481177,-14.2643939492231,
117.060415026704)) ;
#185448=CARTESIAN_POINT('Ctrl Pts',(-16.3645110999979,-14.3281113554114,
117.099602641127)) ;
#185449=CARTESIAN_POINT('Ctrl Pts',(-16.377377051878,-14.3918287615997,
117.138790255551)) ;
#185450=CARTESIAN_POINT('Ctrl Pts',(-16.4511808828745,-14.3918287868466,
117.114559176025)) ;
#185451=CARTESIAN_POINT('Ctrl Pts',(-16.524984713871,-14.3918288120935,
117.090328096499)) ;
#185452=CARTESIAN_POINT('Ctrl Pts',(-16.5121187619909,-14.3281114059052,
117.051140482076)) ;
#185453=CARTESIAN_POINT('Ctrl Pts',(-16.5703367983849,-14.1371521548342,
117.263984046408)) ;
#185454=CARTESIAN_POINT('Ctrl Pts',(-16.5526525054601,-14.0866750756418,
117.210120542421)) ;
#185455=CARTESIAN_POINT('Ctrl Pts',(-16.4788486738412,-14.0866750338847,
117.234351620051)) ;
#185456=CARTESIAN_POINT('Ctrl Pts',(-16.4050448422222,-14.0866749921275,
117.258582697681)) ;
#185457=CARTESIAN_POINT('Ctrl Pts',(-16.4227291351469,-14.1371520713199,
117.312446201668)) ;
#185458=CARTESIAN_POINT('Ctrl Pts',(-16.4404134280717,-14.1876291505123,
117.366309705655)) ;
#185459=CARTESIAN_POINT('Ctrl Pts',(-16.5142172596906,-14.1876291922694,
117.342078628026)) ;
#185460=CARTESIAN_POINT('Ctrl Pts',(-16.5880210913096,-14.1876292340265,
117.317847550396)) ;
#185461=CARTESIAN_POINT('Ctrl Pts',(-16.5703367983849,-14.1371521548342,
117.263984046408)) ;
#185462=CARTESIAN_POINT('Ctrl Pts',(-16.6101467780063,-13.8952369066383,
117.420645973384)) ;
#185463=CARTESIAN_POINT('Ctrl Pts',(-16.588924848466,-13.8615770485299,
117.356007398908)) ;
#185464=CARTESIAN_POINT('Ctrl Pts',(-16.5151210140409,-13.861576991076,
117.380238467991)) ;
#185465=CARTESIAN_POINT('Ctrl Pts',(-16.4413171796157,-13.8615769336222,
117.404469537073)) ;
#185466=CARTESIAN_POINT('Ctrl Pts',(-16.4625391091561,-13.8952367917306,
117.469108111549)) ;
#185467=CARTESIAN_POINT('Ctrl Pts',(-16.4837610386964,-13.928896649839,
117.533746686025)) ;
#185468=CARTESIAN_POINT('Ctrl Pts',(-16.5575648731215,-13.9288967072929,
117.509515616943)) ;
#185469=CARTESIAN_POINT('Ctrl Pts',(-16.6313687075466,-13.9288967647467,
117.48528454786)) ;
#185470=CARTESIAN_POINT('Ctrl Pts',(-16.6101467780063,-13.8952369066383,
117.420645973384)) ;
#185471=CARTESIAN_POINT('Ctrl Pts',(-16.6282135641197,-13.6186018565224,
117.511169862453)) ;
#185472=CARTESIAN_POINT('Ctrl Pts',(-16.6049650461497,-13.6042072181223,
117.440358626447)) ;
#185473=CARTESIAN_POINT('Ctrl Pts',(-16.5311612071269,-13.6042071468649,
117.464589681526)) ;
#185474=CARTESIAN_POINT('Ctrl Pts',(-16.4573573681042,-13.6042070756075,
117.488820736605)) ;
#185475=CARTESIAN_POINT('Ctrl Pts',(-16.4806058860742,-13.6186017140076,
117.559631972611)) ;
#185476=CARTESIAN_POINT('Ctrl Pts',(-16.5038544040443,-13.6329963524077,
117.630443208617)) ;
#185477=CARTESIAN_POINT('Ctrl Pts',(-16.577658243067,-13.6329964236651,
117.606212153538)) ;
#185478=CARTESIAN_POINT('Ctrl Pts',(-16.6514620820897,-13.6329964949225,
117.581981098459)) ;
#185479=CARTESIAN_POINT('Ctrl Pts',(-16.6282135641197,-13.6186018565224,
117.511169862453)) ;
#185480=CARTESIAN_POINT('Ctrl Pts',(-16.6223501381899,-13.3278430882069,
117.528769090005)) ;
#185481=CARTESIAN_POINT('Ctrl Pts',(-16.5987435957387,-13.3337275360589,
117.456867369051)) ;
#185482=CARTESIAN_POINT('Ctrl Pts',(-16.524939750447,-13.3337274561623,
117.481098405036)) ;
#185483=CARTESIAN_POINT('Ctrl Pts',(-16.4511359051553,-13.3337273762658,
117.505329441021)) ;
#185484=CARTESIAN_POINT('Ctrl Pts',(-16.4747424476065,-13.3278429284139,
117.577231161974)) ;
#185485=CARTESIAN_POINT('Ctrl Pts',(-16.4983489900577,-13.3219584805619,
117.649132882927)) ;
#185486=CARTESIAN_POINT('Ctrl Pts',(-16.5721528353494,-13.3219585604584,
117.624901846943)) ;
#185487=CARTESIAN_POINT('Ctrl Pts',(-16.645956680641,-13.3219586403549,
117.600670810958)) ;
#185488=CARTESIAN_POINT('Ctrl Pts',(-16.6223501381899,-13.3278430882069,
117.528769090005)) ;
#185489=CARTESIAN_POINT('Ctrl Pts',(-16.5922344703617,-13.0431633993278,
117.472546786263)) ;
#185490=CARTESIAN_POINT('Ctrl Pts',(-16.5699615140208,-13.0689317715885,
117.404706953289)) ;
#185491=CARTESIAN_POINT('Ctrl Pts',(-16.4961576613975,-13.0689316894194,
117.428937966943)) ;
#185492=CARTESIAN_POINT('Ctrl Pts',(-16.4223538087744,-13.0689316072503,
117.453168980598)) ;
#185493=CARTESIAN_POINT('Ctrl Pts',(-16.4446267651153,-13.0431632349896,
117.521008813571)) ;
#185494=CARTESIAN_POINT('Ctrl Pts',(-16.4668997214564,-13.0173948627289,
117.588848646545)) ;
#185495=CARTESIAN_POINT('Ctrl Pts',(-16.5407035740795,-13.017394944898,
117.564617632891)) ;
#185496=CARTESIAN_POINT('Ctrl Pts',(-16.6145074267027,-13.0173950270671,
117.540386619237)) ;
#185497=CARTESIAN_POINT('Ctrl Pts',(-16.5922344703617,-13.0431633993278,
117.472546786263)) ;
#185498=CARTESIAN_POINT('Ctrl Pts',(-16.5392017956511,-12.7854826732307,
117.346522184248)) ;
#185499=CARTESIAN_POINT('Ctrl Pts',(-16.5198642813153,-12.8292789756885,
117.28762323387)) ;
#185500=CARTESIAN_POINT('Ctrl Pts',(-16.4460604210477,-12.8292788993553,
117.311854224241)) ;
#185501=CARTESIAN_POINT('Ctrl Pts',(-16.3722565607802,-12.8292788230221,
117.336085214612)) ;
#185502=CARTESIAN_POINT('Ctrl Pts',(-16.3915940751159,-12.7854825205643,
117.39498416499)) ;
#185503=CARTESIAN_POINT('Ctrl Pts',(-16.4109315894516,-12.7416862181065,
117.453883115367)) ;
#185504=CARTESIAN_POINT('Ctrl Pts',(-16.4847354497192,-12.7416862944397,
117.429652124997)) ;
#185505=CARTESIAN_POINT('Ctrl Pts',(-16.5585393099868,-12.7416863707729,
117.405421134626)) ;
#185506=CARTESIAN_POINT('Ctrl Pts',(-16.5392017956511,-12.7854826732307,
117.346522184248)) ;
#185507=CARTESIAN_POINT('Ctrl Pts',(-16.4667915995857,-12.5740916835464,
117.161296219297)) ;
#185508=CARTESIAN_POINT('Ctrl Pts',(-16.451750503951,-12.6327102616695,
117.115483466974)) ;
#185509=CARTESIAN_POINT('Ctrl Pts',(-16.3779466369284,-12.6327101996491,
117.13971443677)) ;
#185510=CARTESIAN_POINT('Ctrl Pts',(-16.3041427699058,-12.6327101376288,
117.163945406566)) ;
#185511=CARTESIAN_POINT('Ctrl Pts',(-16.3191838655404,-12.5740915595058,
117.209758158888)) ;
#185512=CARTESIAN_POINT('Ctrl Pts',(-16.3342249611751,-12.5154729813828,
117.255570911211)) ;
#185513=CARTESIAN_POINT('Ctrl Pts',(-16.4080288281977,-12.5154730434031,
117.231339941415)) ;
#185514=CARTESIAN_POINT('Ctrl Pts',(-16.4818326952203,-12.5154731054234,
117.207108971619)) ;
#185515=CARTESIAN_POINT('Ctrl Pts',(-16.4667915995857,-12.5740916835464,
117.161296219297)) ;
#185516=CARTESIAN_POINT('Ctrl Pts',(-16.3787109405611,-12.4220262848849,
116.928516659474)) ;
#185517=CARTESIAN_POINT('Ctrl Pts',(-16.3690627026773,-12.4913473054171,
116.89912968164)) ;
#185518=CARTESIAN_POINT('Ctrl Pts',(-16.2952588300958,-12.49134726396,116.923360634505)) ;
#185519=CARTESIAN_POINT('Ctrl Pts',(-16.2214549575144,-12.491347222503,
116.947591587369)) ;
#185520=CARTESIAN_POINT('Ctrl Pts',(-16.2311031953983,-12.4220262019709,
116.976978565203)) ;
#185521=CARTESIAN_POINT('Ctrl Pts',(-16.2407514332821,-12.3527051814387,
117.006365543037)) ;
#185522=CARTESIAN_POINT('Ctrl Pts',(-16.3145553058636,-12.3527052228958,
116.982134590172)) ;
#185523=CARTESIAN_POINT('Ctrl Pts',(-16.388359178445,-12.3527052643528,
116.957903637308)) ;
#185524=CARTESIAN_POINT('Ctrl Pts',(-16.3787109405611,-12.4220262848849,
116.928516659474)) ;
#185525=CARTESIAN_POINT('Ctrl Pts',(-16.2808900951267,-12.3415697140928,
116.666038345692)) ;
#185526=CARTESIAN_POINT('Ctrl Pts',(-16.277323271128,-12.4166096733525,
116.655174373259)) ;
#185527=CARTESIAN_POINT('Ctrl Pts',(-16.2035193951826,-12.4166096578571,
116.679405315878)) ;
#185528=CARTESIAN_POINT('Ctrl Pts',(-16.1297155192372,-12.4166096423617,
116.703636258496)) ;
#185529=CARTESIAN_POINT('Ctrl Pts',(-16.1332823432358,-12.341569683102,
116.714500230929)) ;
#185530=CARTESIAN_POINT('Ctrl Pts',(-16.1368491672345,-12.2665297238424,
116.725364203362)) ;
#185531=CARTESIAN_POINT('Ctrl Pts',(-16.2106530431799,-12.2665297393378,
116.701133260744)) ;
#185532=CARTESIAN_POINT('Ctrl Pts',(-16.2844569191253,-12.2665297548332,
116.676902318125)) ;
#185533=CARTESIAN_POINT('Ctrl Pts',(-16.2808900951267,-12.3415697140928,
116.666038345692)) ;
#185534=CARTESIAN_POINT('Ctrl Pts',(-16.1795322882749,-12.3382226972324,
116.392792739754)) ;
#185535=CARTESIAN_POINT('Ctrl Pts',(-16.1823026066868,-12.4136068588393,
116.40123068057)) ;
#185536=CARTESIAN_POINT('Ctrl Pts',(-16.1084987299936,-12.413606871913,
116.425461620911)) ;
#185537=CARTESIAN_POINT('Ctrl Pts',(-16.0346948533003,-12.4136068849868,
116.449692561251)) ;
#185538=CARTESIAN_POINT('Ctrl Pts',(-16.0319245348884,-12.3382227233798,
116.441254620435)) ;
#185539=CARTESIAN_POINT('Ctrl Pts',(-16.0291542164764,-12.2628385617728,
116.432816679619)) ;
#185540=CARTESIAN_POINT('Ctrl Pts',(-16.1029580931697,-12.2628385486991,
116.408585739279)) ;
#185541=CARTESIAN_POINT('Ctrl Pts',(-16.1767619698629,-12.2628385356254,
116.384354798938)) ;
#185542=CARTESIAN_POINT('Ctrl Pts',(-16.1795322882749,-12.3382226972324,
116.392792739754)) ;
#185543=CARTESIAN_POINT('Ctrl Pts',(-16.081237325198,-12.4121411260321,
116.128842285068)) ;
#185544=CARTESIAN_POINT('Ctrl Pts',(-16.0901410081958,-12.4824758625955,
116.155961464781)) ;
#185545=CARTESIAN_POINT('Ctrl Pts',(-16.0163371335278,-12.4824759039206,
116.18019241129)) ;
#185546=CARTESIAN_POINT('Ctrl Pts',(-15.9425332588598,-12.4824759452457,
116.204423357799)) ;
#185547=CARTESIAN_POINT('Ctrl Pts',(-15.933629575862,-12.4121412086823,
116.177304178087)) ;
#185548=CARTESIAN_POINT('Ctrl Pts',(-15.9247258928641,-12.3418064721188,
116.150184998374)) ;
#185549=CARTESIAN_POINT('Ctrl Pts',(-15.9985297675321,-12.3418064307938,
116.125954051865)) ;
#185550=CARTESIAN_POINT('Ctrl Pts',(-16.0723336422001,-12.3418063894687,
116.101723105356)) ;
#185551=CARTESIAN_POINT('Ctrl Pts',(-16.081237325198,-12.4121411260321,
116.128842285068)) ;
#185552=CARTESIAN_POINT('Ctrl Pts',(-15.9921008262012,-12.5582147089023,
115.892828190481)) ;
#185553=CARTESIAN_POINT('Ctrl Pts',(-16.0065067244686,-12.6184554167387,
115.93670623013)) ;
#185554=CARTESIAN_POINT('Ctrl Pts',(-15.9327028544161,-12.6184554831094,
115.960937190697)) ;
#185555=CARTESIAN_POINT('Ctrl Pts',(-15.8588989843637,-12.61845554948,115.985168151265)) ;
#185556=CARTESIAN_POINT('Ctrl Pts',(-15.8444930860963,-12.5582148416436,
115.941290111616)) ;
#185557=CARTESIAN_POINT('Ctrl Pts',(-15.8300871878288,-12.4979741338071,
115.897412071967)) ;
#185558=CARTESIAN_POINT('Ctrl Pts',(-15.9038910578813,-12.4979740674365,
115.873181111399)) ;
#185559=CARTESIAN_POINT('Ctrl Pts',(-15.9776949279337,-12.4979740010659,
115.848950150832)) ;
#185560=CARTESIAN_POINT('Ctrl Pts',(-15.9921008262012,-12.5582147089023,
115.892828190481)) ;
#185561=CARTESIAN_POINT('Ctrl Pts',(-15.917928987099,-12.7657436426172,
115.702363572167)) ;
#185562=CARTESIAN_POINT('Ctrl Pts',(-15.936801184951,-12.8115849189124,
115.759845239742)) ;
#185563=CARTESIAN_POINT('Ctrl Pts',(-15.8629973216198,-12.8115850045316,
115.784076220781)) ;
#185564=CARTESIAN_POINT('Ctrl Pts',(-15.7891934582887,-12.8115850901508,
115.808307201821)) ;
#185565=CARTESIAN_POINT('Ctrl Pts',(-15.7703212604367,-12.7657438138556,
115.750825534246)) ;
#185566=CARTESIAN_POINT('Ctrl Pts',(-15.7514490625847,-12.7199025375603,
115.693343866671)) ;
#185567=CARTESIAN_POINT('Ctrl Pts',(-15.8252529259159,-12.7199024519411,
115.669112885632)) ;
#185568=CARTESIAN_POINT('Ctrl Pts',(-15.8990567892471,-12.7199023663219,
115.644881904592)) ;
#185569=CARTESIAN_POINT('Ctrl Pts',(-15.917928987099,-12.7657436426172,
115.702363572167)) ;
#185570=CARTESIAN_POINT('Ctrl Pts',(-15.8631509693549,-13.0202106019441,
115.571004295202)) ;
#185571=CARTESIAN_POINT('Ctrl Pts',(-15.8851414927432,-13.0483542398271,
115.637983879269)) ;
#185572=CARTESIAN_POINT('Ctrl Pts',(-15.8113376375345,-13.0483543369911,
115.662214885049)) ;
#185573=CARTESIAN_POINT('Ctrl Pts',(-15.7375337823258,-13.0483544341551,
115.686445890828)) ;
#185574=CARTESIAN_POINT('Ctrl Pts',(-15.7155432589375,-13.0202107962721,
115.61946630676)) ;
#185575=CARTESIAN_POINT('Ctrl Pts',(-15.6935527355492,-12.992067158389,
115.552486722692)) ;
#185576=CARTESIAN_POINT('Ctrl Pts',(-15.7673565907579,-12.9920670612251,
115.528255716913)) ;
#185577=CARTESIAN_POINT('Ctrl Pts',(-15.8411604459666,-12.9920669640611,
115.504024711134)) ;
#185578=CARTESIAN_POINT('Ctrl Pts',(-15.8631509693549,-13.0202106019441,
115.571004295202)) ;
#185579=CARTESIAN_POINT('Ctrl Pts',(-15.8310465221303,-13.3031020545658,
115.508689927351)) ;
#185580=CARTESIAN_POINT('Ctrl Pts',(-15.8545774432419,-13.3115371239571,
115.580361314412)) ;
#185581=CARTESIAN_POINT('Ctrl Pts',(-15.7807735966424,-13.3115372240585,
115.604592346413)) ;
#185582=CARTESIAN_POINT('Ctrl Pts',(-15.7069697500429,-13.3115373241599,
115.628823378414)) ;
#185583=CARTESIAN_POINT('Ctrl Pts',(-15.6834388289312,-13.3031022547687,
115.557151991353)) ;
#185584=CARTESIAN_POINT('Ctrl Pts',(-15.6599079078196,-13.2946671853774,
115.485480604292)) ;
#185585=CARTESIAN_POINT('Ctrl Pts',(-15.7337117544191,-13.2946670852759,
115.461249572291)) ;
#185586=CARTESIAN_POINT('Ctrl Pts',(-15.8075156010186,-13.2946669851745,
115.437018540289)) ;
#185587=CARTESIAN_POINT('Ctrl Pts',(-15.8310465221303,-13.3031020545658,
115.508689927351)) ;
#185588=CARTESIAN_POINT('Ctrl Pts',(-15.8231198539142,-13.593918747588,
115.519982474148)) ;
#185589=CARTESIAN_POINT('Ctrl Pts',(-15.8465062326338,-13.5820623140505,
115.591213608491)) ;
#185590=CARTESIAN_POINT('Ctrl Pts',(-15.7727023942151,-13.5820624088636,
115.61544466541)) ;
#185591=CARTESIAN_POINT('Ctrl Pts',(-15.6988985557964,-13.5820625036768,
115.639675722329)) ;
#185592=CARTESIAN_POINT('Ctrl Pts',(-15.6755121770768,-13.5939189372143,
115.568444587986)) ;
#185593=CARTESIAN_POINT('Ctrl Pts',(-15.6521257983572,-13.6057753707518,
115.497213453642)) ;
#185594=CARTESIAN_POINT('Ctrl Pts',(-15.7259296367759,-13.6057752759387,
115.472982396723)) ;
#185595=CARTESIAN_POINT('Ctrl Pts',(-15.7997334751946,-13.6057751811255,
115.448751339805)) ;
#185596=CARTESIAN_POINT('Ctrl Pts',(-15.8231198539142,-13.593918747588,
115.519982474148)) ;
#185597=CARTESIAN_POINT('Ctrl Pts',(-15.8391226607634,-13.8723058564386,
115.604173660196)) ;
#185598=CARTESIAN_POINT('Ctrl Pts',(-15.8606934004284,-13.8409951979867,
115.669874651036)) ;
#185599=CARTESIAN_POINT('Ctrl Pts',(-15.7868895690113,-13.8409952801853,
115.694105729281)) ;
#185600=CARTESIAN_POINT('Ctrl Pts',(-15.7130857375942,-13.8409953623839,
115.718336807525)) ;
#185601=CARTESIAN_POINT('Ctrl Pts',(-15.6915149979293,-13.8723060208357,
115.652635816686)) ;
#185602=CARTESIAN_POINT('Ctrl Pts',(-15.6699442582643,-13.9036166792876,
115.586934825846)) ;
#185603=CARTESIAN_POINT('Ctrl Pts',(-15.7437480896814,-13.903616597089,
115.562703747601)) ;
#185604=CARTESIAN_POINT('Ctrl Pts',(-15.8175519210985,-13.9036165148904,
115.538472669357)) ;
#185605=CARTESIAN_POINT('Ctrl Pts',(-15.8391226607634,-13.8723058564386,
115.604173660196)) ;
#185606=CARTESIAN_POINT('Ctrl Pts',(-15.8773871785258,-14.118869151071,
115.756288039499)) ;
#185607=CARTESIAN_POINT('Ctrl Pts',(-15.8955830177552,-14.070296502829,
115.81170962829)) ;
#185608=CARTESIAN_POINT('Ctrl Pts',(-15.8217791912897,-14.0702965663063,
115.835940721616)) ;
#185609=CARTESIAN_POINT('Ctrl Pts',(-15.7479753648241,-14.0702966297837,
115.860171814942)) ;
#185610=CARTESIAN_POINT('Ctrl Pts',(-15.7297795255947,-14.1188692780257,
115.804750226151)) ;
#185611=CARTESIAN_POINT('Ctrl Pts',(-15.7115836863652,-14.1674419262677,
115.749328637361)) ;
#185612=CARTESIAN_POINT('Ctrl Pts',(-15.7853875128308,-14.1674418627903,
115.725097544035)) ;
#185613=CARTESIAN_POINT('Ctrl Pts',(-15.8591913392963,-14.167441799313,
115.700866450708)) ;
#185614=CARTESIAN_POINT('Ctrl Pts',(-15.8773871785258,-14.118869151071,
115.756288039499)) ;
#185615=CARTESIAN_POINT('Ctrl Pts',(-15.9340609590514,-14.3141618691383,
115.964310153546)) ;
#185616=CARTESIAN_POINT('Ctrl Pts',(-15.9475947541449,-14.2518807456653,
116.005531908246)) ;
#185617=CARTESIAN_POINT('Ctrl Pts',(-15.8737909305843,-14.2518807886643,
116.029763010421)) ;
#185618=CARTESIAN_POINT('Ctrl Pts',(-15.7999871070237,-14.2518808316633,
116.053994112595)) ;
#185619=CARTESIAN_POINT('Ctrl Pts',(-15.7864533119302,-14.3141619551363,
116.012772357894)) ;
#185620=CARTESIAN_POINT('Ctrl Pts',(-15.7729195168366,-14.3764430786093,
115.971550603193)) ;
#185621=CARTESIAN_POINT('Ctrl Pts',(-15.8467233403972,-14.3764430356103,
115.947319501019)) ;
#185622=CARTESIAN_POINT('Ctrl Pts',(-15.9205271639579,-14.3764429926113,
115.923088398845)) ;
#185623=CARTESIAN_POINT('Ctrl Pts',(-15.9340609590514,-14.3141618691383,
115.964310153546)) ;
#185624=CARTESIAN_POINT('Ctrl Pts',(-16.0045560916089,-14.4456574881185,
116.214482017729)) ;
#185625=CARTESIAN_POINT('Ctrl Pts',(-16.0124547601936,-14.3741011608773,
116.238540086457)) ;
#185626=CARTESIAN_POINT('Ctrl Pts',(-15.9386509372217,-14.3741011828996,
116.262771190424)) ;
#185627=CARTESIAN_POINT('Ctrl Pts',(-15.8648471142499,-14.3741012049218,
116.287002294392)) ;
#185628=CARTESIAN_POINT('Ctrl Pts',(-15.8569484456653,-14.4456575321631,
116.262944225664)) ;
#185629=CARTESIAN_POINT('Ctrl Pts',(-15.8490497770806,-14.5172138594043,
116.238886156936)) ;
#185630=CARTESIAN_POINT('Ctrl Pts',(-15.9228536000524,-14.5172138373821,
116.214655052969)) ;
#185631=CARTESIAN_POINT('Ctrl Pts',(-15.9966574230242,-14.5172138153598,
116.190423949001)) ;
#185632=CARTESIAN_POINT('Ctrl Pts',(-16.0045560916089,-14.4456574881185,
116.214482017729)) ;
#185633=CARTESIAN_POINT('Ctrl Pts',(-16.0830095747665,-14.5036635199146,
116.488878900793)) ;
#185634=CARTESIAN_POINT('Ctrl Pts',(-16.0847092169098,-14.4279488253923,
116.494055735345)) ;
#185635=CARTESIAN_POINT('Ctrl Pts',(-16.0109053925219,-14.4279488285843,
116.518286835)) ;
#185636=CARTESIAN_POINT('Ctrl Pts',(-15.9371015681339,-14.4279488317762,
116.542517934654)) ;
#185637=CARTESIAN_POINT('Ctrl Pts',(-15.9354019259906,-14.5036635262985,
116.537341100102)) ;
#185638=CARTESIAN_POINT('Ctrl Pts',(-15.9337022838474,-14.5793782208208,
116.53216426555)) ;
#185639=CARTESIAN_POINT('Ctrl Pts',(-16.0075061082353,-14.5793782176288,
116.507933165896)) ;
#185640=CARTESIAN_POINT('Ctrl Pts',(-16.0813099326232,-14.5793782144369,
116.483702066242)) ;
#185641=CARTESIAN_POINT('Ctrl Pts',(-16.0830095747665,-14.5036635199146,
116.488878900793)) ;
#185642=CARTESIAN_POINT('Ctrl Pts',(-16.1633742770454,-14.4836080857303,
116.76924043046)) ;
#185643=CARTESIAN_POINT('Ctrl Pts',(-16.1587290093675,-14.409178476904,
116.755091693632)) ;
#185644=CARTESIAN_POINT('Ctrl Pts',(-16.0849251815922,-14.4091784657996,
116.779322782969)) ;
#185645=CARTESIAN_POINT('Ctrl Pts',(-16.011121353817,-14.4091784546952,
116.803553872307)) ;
#185646=CARTESIAN_POINT('Ctrl Pts',(-16.0157666214949,-14.4836080635215,
116.817702609134)) ;
#185647=CARTESIAN_POINT('Ctrl Pts',(-16.0204118891728,-14.5580376723478,
116.831851345961)) ;
#185648=CARTESIAN_POINT('Ctrl Pts',(-16.094215716948,-14.5580376834522,
116.807620256624)) ;
#185649=CARTESIAN_POINT('Ctrl Pts',(-16.1680195447233,-14.5580376945566,
116.783389167287)) ;
#185650=CARTESIAN_POINT('Ctrl Pts',(-16.1633742770454,-14.4836080857303,
116.76924043046)) ;
#185651=CARTESIAN_POINT('Ctrl Pts',(-16.2383518880624,-14.3877127605132,
117.03295492109)) ;
#185652=CARTESIAN_POINT('Ctrl Pts',(-16.2277331466029,-14.319866136678,
117.000611947086)) ;
#185653=CARTESIAN_POINT('Ctrl Pts',(-16.1539293152376,-14.3198661161146,
117.024843025489)) ;
#185654=CARTESIAN_POINT('Ctrl Pts',(-16.0801254838723,-14.3198660955512,
117.049074103891)) ;
#185655=CARTESIAN_POINT('Ctrl Pts',(-16.0907442253319,-14.3877127193864,
117.081417077895)) ;
#185656=CARTESIAN_POINT('Ctrl Pts',(-16.1013629667914,-14.4555593432216,
117.113760051899)) ;
#185657=CARTESIAN_POINT('Ctrl Pts',(-16.1751667981567,-14.455559363785,
117.089528973497)) ;
#185658=CARTESIAN_POINT('Ctrl Pts',(-16.2489706295219,-14.4555593843484,
117.065297895094)) ;
#185659=CARTESIAN_POINT('Ctrl Pts',(-16.2383518880624,-14.3877127605132,
117.03295492109)) ;
#185660=CARTESIAN_POINT('Ctrl Pts',(-16.3028078351628,-14.2212524561287,
117.264903394669)) ;
#185661=CARTESIAN_POINT('Ctrl Pts',(-16.2869351807354,-14.1649252203371,
117.216557849678)) ;
#185662=CARTESIAN_POINT('Ctrl Pts',(-16.2131313448875,-14.1649251971047,
117.240788914427)) ;
#185663=CARTESIAN_POINT('Ctrl Pts',(-16.1393275090396,-14.1649251738723,
117.265019979176)) ;
#185664=CARTESIAN_POINT('Ctrl Pts',(-16.155200163467,-14.2212524096639,
117.313365524167)) ;
#185665=CARTESIAN_POINT('Ctrl Pts',(-16.1710728178944,-14.2775796454555,
117.361711069158)) ;
#185666=CARTESIAN_POINT('Ctrl Pts',(-16.2448766537423,-14.2775796686879,
117.337480004409)) ;
#185667=CARTESIAN_POINT('Ctrl Pts',(-16.3186804895902,-14.2775796919203,
117.31324893966)) ;
#185668=CARTESIAN_POINT('Ctrl Pts',(-16.3028078351628,-14.2212524561287,
117.264903394669)) ;
#185669=CARTESIAN_POINT('Ctrl Pts',(-16.3503835879466,-13.9987538981264,
117.445133843183)) ;
#185670=CARTESIAN_POINT('Ctrl Pts',(-16.3304341319157,-13.9578771653023,
117.384371018433)) ;
#185671=CARTESIAN_POINT('Ctrl Pts',(-16.2566302927543,-13.9578771425154,
117.408602073089)) ;
#185672=CARTESIAN_POINT('Ctrl Pts',(-16.1828264535928,-13.9578771197285,
117.432833127746)) ;
#185673=CARTESIAN_POINT('Ctrl Pts',(-16.2027759096237,-13.9987538525526,
117.493595952497)) ;
#185674=CARTESIAN_POINT('Ctrl Pts',(-16.2227253656546,-14.0396305853768,
117.554358777247)) ;
#185675=CARTESIAN_POINT('Ctrl Pts',(-16.296529204816,-14.0396306081637,
117.530127722591)) ;
#185676=CARTESIAN_POINT('Ctrl Pts',(-16.3703330439775,-14.0396306309506,
117.505896667934)) ;
#185677=CARTESIAN_POINT('Ctrl Pts',(-16.3503835879466,-13.9987538981264,
117.445133843183)) ;
#185678=CARTESIAN_POINT('Ctrl Pts',(-16.3776742277473,-13.7338214529053,
117.563745231452)) ;
#185679=CARTESIAN_POINT('Ctrl Pts',(-16.3550546145414,-13.7113815142411,
117.494849538931)) ;
#185680=CARTESIAN_POINT('Ctrl Pts',(-16.2812507726019,-13.7113814963311,
117.519080585126)) ;
#185681=CARTESIAN_POINT('Ctrl Pts',(-16.2074469306623,-13.7113814784212,
117.543311631321)) ;
#185682=CARTESIAN_POINT('Ctrl Pts',(-16.2300665438682,-13.7338214170854,
117.612207323843)) ;
#185683=CARTESIAN_POINT('Ctrl Pts',(-16.2526861570741,-13.7562613557496,
117.681103016364)) ;
#185684=CARTESIAN_POINT('Ctrl Pts',(-16.3264899990136,-13.7562613736596,
117.656871970169)) ;
#185685=CARTESIAN_POINT('Ctrl Pts',(-16.4002938409532,-13.7562613915695,
117.632640923974)) ;
#185686=CARTESIAN_POINT('Ctrl Pts',(-16.3776742277473,-13.7338214529053,
117.563745231452)) ;
#185687=CARTESIAN_POINT('Ctrl Pts',(-16.3816715029604,-13.4466916236415,
117.611342756202)) ;
#185688=CARTESIAN_POINT('Ctrl Pts',(-16.3580056108764,-13.4442666484752,
117.539260267165)) ;
#185689=CARTESIAN_POINT('Ctrl Pts',(-16.2842017673765,-13.4442666367421,
117.563491308608)) ;
#185690=CARTESIAN_POINT('Ctrl Pts',(-16.2103979238767,-13.4442666250089,
117.58772235005)) ;
#185691=CARTESIAN_POINT('Ctrl Pts',(-16.2340638159607,-13.4466916001752,
117.659804839087)) ;
#185692=CARTESIAN_POINT('Ctrl Pts',(-16.2577297080446,-13.4491165753415,
117.731887328124)) ;
#185693=CARTESIAN_POINT('Ctrl Pts',(-16.3315335515445,-13.4491165870746,
117.707656286682)) ;
#185694=CARTESIAN_POINT('Ctrl Pts',(-16.4053373950444,-13.4491165988078,
117.683425245239)) ;
#185695=CARTESIAN_POINT('Ctrl Pts',(-16.3816715029604,-13.4466916236415,
117.611342756202)) ;
#185696=CARTESIAN_POINT('Ctrl Pts',(-16.3613250579378,-13.1565169960044,
117.584919941758)) ;
#185697=CARTESIAN_POINT('Ctrl Pts',(-16.3383084793065,-13.1743502694123,
117.51481515686)) ;
#185698=CARTESIAN_POINT('Ctrl Pts',(-16.2645046353523,-13.1743502645941,
117.539046196918)) ;
#185699=CARTESIAN_POINT('Ctrl Pts',(-16.1907007913981,-13.174350259776,
117.563277236977)) ;
#185700=CARTESIAN_POINT('Ctrl Pts',(-16.2137173700294,-13.156516986368,
117.633382021875)) ;
#185701=CARTESIAN_POINT('Ctrl Pts',(-16.2367339486607,-13.1386837129601,
117.703486806774)) ;
#185702=CARTESIAN_POINT('Ctrl Pts',(-16.3105377926149,-13.1386837177783,
117.679255766715)) ;
#185703=CARTESIAN_POINT('Ctrl Pts',(-16.3843416365691,-13.1386837225965,
117.655024726656)) ;
#185704=CARTESIAN_POINT('Ctrl Pts',(-16.3613250579378,-13.1565169960044,
117.584919941758)) ;
#185705=CARTESIAN_POINT('Ctrl Pts',(-16.3173032833634,-12.8855146893556,
117.486337024747)) ;
#185706=CARTESIAN_POINT('Ctrl Pts',(-16.2965914011344,-12.9222982070888,
117.423251973321)) ;
#185707=CARTESIAN_POINT('Ctrl Pts',(-16.2227875575851,-12.9222982069282,
117.447483014612)) ;
#185708=CARTESIAN_POINT('Ctrl Pts',(-16.1489837140357,-12.9222982067677,
117.471714055904)) ;
#185709=CARTESIAN_POINT('Ctrl Pts',(-16.1696955962647,-12.8855146890345,
117.534799107331)) ;
#185710=CARTESIAN_POINT('Ctrl Pts',(-16.1904074784936,-12.8487311713013,
117.597884158757)) ;
#185711=CARTESIAN_POINT('Ctrl Pts',(-16.2642113220429,-12.8487311714619,
117.573653117466)) ;
#185712=CARTESIAN_POINT('Ctrl Pts',(-16.3380151655923,-12.8487311716225,
117.549422076174)) ;
#185713=CARTESIAN_POINT('Ctrl Pts',(-16.3173032833634,-12.8855146893556,
117.486337024747)) ;
#185714=CARTESIAN_POINT('Ctrl Pts',(-16.2522540404142,-12.6534167842388,
117.323607876768)) ;
#185715=CARTESIAN_POINT('Ctrl Pts',(-16.2353209157865,-12.7064619703102,
117.272032311344)) ;
#185716=CARTESIAN_POINT('Ctrl Pts',(-16.1615170728299,-12.706461972049,
117.296263354442)) ;
#185717=CARTESIAN_POINT('Ctrl Pts',(-16.0877132298733,-12.7064619737879,
117.320494397539)) ;
#185718=CARTESIAN_POINT('Ctrl Pts',(-16.104646354501,-12.6534167877166,
117.372069962962)) ;
#185719=CARTESIAN_POINT('Ctrl Pts',(-16.1215794791288,-12.6003716016452,
117.423645528385)) ;
#185720=CARTESIAN_POINT('Ctrl Pts',(-16.1953833220854,-12.6003715999064,
117.399414485288)) ;
#185721=CARTESIAN_POINT('Ctrl Pts',(-16.269187165042,-12.6003715981675,
117.375183442191)) ;
#185722=CARTESIAN_POINT('Ctrl Pts',(-16.2522540404142,-12.6534167842388,
117.323607876768)) ;
#185723=CARTESIAN_POINT('Ctrl Pts',(-16.1701161398685,-12.475742126735,
117.108794315217)) ;
#185724=CARTESIAN_POINT('Ctrl Pts',(-16.158161556272,-12.5412726842435,
117.072382582516)) ;
#185725=CARTESIAN_POINT('Ctrl Pts',(-16.0843577138288,-12.5412726859999,
117.096613627177)) ;
#185726=CARTESIAN_POINT('Ctrl Pts',(-16.0105538713855,-12.5412726877563,
117.120844671838)) ;
#185727=CARTESIAN_POINT('Ctrl Pts',(-16.0225084549819,-12.4757421302478,
117.157256404539)) ;
#185728=CARTESIAN_POINT('Ctrl Pts',(-16.0344630385783,-12.4102115727394,
117.19366813724)) ;
#185729=CARTESIAN_POINT('Ctrl Pts',(-16.1082668810216,-12.410211570983,
117.169437092579)) ;
#185730=CARTESIAN_POINT('Ctrl Pts',(-16.1820707234649,-12.4102115692266,
117.145206047918)) ;
#185731=CARTESIAN_POINT('Ctrl Pts',(-16.1701161398685,-12.475742126735,
117.108794315217)) ;
#185732=CARTESIAN_POINT('Ctrl Pts',(-16.0748178977869,-12.3646792210001,
116.854266992389)) ;
#185733=CARTESIAN_POINT('Ctrl Pts',(-16.0687608064458,-12.438062944576,
116.835818069506)) ;
#185734=CARTESIAN_POINT('Ctrl Pts',(-15.994956963594,-12.4380629448186,
116.860049112923)) ;
#185735=CARTESIAN_POINT('Ctrl Pts',(-15.9211531207422,-12.4380629450611,
116.884280156339)) ;
#185736=CARTESIAN_POINT('Ctrl Pts',(-15.9272102120833,-12.3646792214852,
116.902729079222)) ;
#185737=CARTESIAN_POINT('Ctrl Pts',(-15.9332673034244,-12.2912954979092,
116.921178002105)) ;
#185738=CARTESIAN_POINT('Ctrl Pts',(-16.0070711462762,-12.2912954976667,
116.896946958688)) ;
#185739=CARTESIAN_POINT('Ctrl Pts',(-16.080874989128,-12.2912954974242,
116.872715915272)) ;
#185740=CARTESIAN_POINT('Ctrl Pts',(-16.0748178977869,-12.3646792210001,
116.854266992389)) ;
#185741=CARTESIAN_POINT('Ctrl Pts',(-15.974621026397,-12.33019827638,116.584367210853)) ;
#185742=CARTESIAN_POINT('Ctrl Pts',(-15.9748212050105,-12.4060967099992,
116.584976922591)) ;
#185743=CARTESIAN_POINT('Ctrl Pts',(-15.9010173612801,-12.4060967096592,
116.609207963332)) ;
#185744=CARTESIAN_POINT('Ctrl Pts',(-15.8272135175496,-12.4060967093193,
116.633439004072)) ;
#185745=CARTESIAN_POINT('Ctrl Pts',(-15.8270133389361,-12.3301982757,116.632829292334)) ;
#185746=CARTESIAN_POINT('Ctrl Pts',(-15.8268131603226,-12.2542998420808,
116.632219580595)) ;
#185747=CARTESIAN_POINT('Ctrl Pts',(-15.900617004053,-12.2542998424208,
116.607988539855)) ;
#185748=CARTESIAN_POINT('Ctrl Pts',(-15.9744208477835,-12.2542998427607,
116.583757499115)) ;
#185749=CARTESIAN_POINT('Ctrl Pts',(-15.974621026397,-12.33019827638,116.584367210853)) ;
#185750=CARTESIAN_POINT('Ctrl Pts',(-15.8740611512203,-12.3732244526573,
116.313621656584)) ;
#185751=CARTESIAN_POINT('Ctrl Pts',(-15.8805477737599,-12.4462297114867,
116.333378862108)) ;
#185752=CARTESIAN_POINT('Ctrl Pts',(-15.8067439284556,-12.4462297127272,
116.357609898054)) ;
#185753=CARTESIAN_POINT('Ctrl Pts',(-15.7329400831513,-12.4462297139677,
116.381840934001)) ;
#185754=CARTESIAN_POINT('Ctrl Pts',(-15.7264534606117,-12.3732244551383,
116.362083728477)) ;
#185755=CARTESIAN_POINT('Ctrl Pts',(-15.7199668380721,-12.300219196309,
116.342326522954)) ;
#185756=CARTESIAN_POINT('Ctrl Pts',(-15.7937706833764,-12.3002191950685,
116.318095487007)) ;
#185757=CARTESIAN_POINT('Ctrl Pts',(-15.8675745286806,-12.300219193828,
116.293864451061)) ;
#185758=CARTESIAN_POINT('Ctrl Pts',(-15.8740611512203,-12.3732244526573,
116.313621656584)) ;
#185759=CARTESIAN_POINT('Ctrl Pts',(-15.7806896879086,-12.4909980427198,
116.064622149398)) ;
#185760=CARTESIAN_POINT('Ctrl Pts',(-15.7929728305085,-12.5558859351168,
116.102034619648)) ;
#185761=CARTESIAN_POINT('Ctrl Pts',(-15.7191689838426,-12.555885940904,
116.126265651448)) ;
#185762=CARTESIAN_POINT('Ctrl Pts',(-15.6453651371768,-12.5558859466913,
116.150496683248)) ;
#185763=CARTESIAN_POINT('Ctrl Pts',(-15.6330819945769,-12.4909980542943,
116.113084212997)) ;
#185764=CARTESIAN_POINT('Ctrl Pts',(-15.6207988519771,-12.4261101618973,
116.075671742746)) ;
#185765=CARTESIAN_POINT('Ctrl Pts',(-15.6946026986429,-12.4261101561101,
116.051440710946)) ;
#185766=CARTESIAN_POINT('Ctrl Pts',(-15.7684065453087,-12.4261101503228,
116.027209679147)) ;
#185767=CARTESIAN_POINT('Ctrl Pts',(-15.7806896879086,-12.4909980427198,
116.064622149398)) ;
#185768=CARTESIAN_POINT('Ctrl Pts',(-15.6998735281005,-12.67497986033,115.853907441211)) ;
#185769=CARTESIAN_POINT('Ctrl Pts',(-15.7170839596561,-12.7271157689749,
115.906327638474)) ;
#185770=CARTESIAN_POINT('Ctrl Pts',(-15.6432801120866,-12.727115782205,
115.930558667521)) ;
#185771=CARTESIAN_POINT('Ctrl Pts',(-15.569476264517,-12.7271157954351,
115.954789696568)) ;
#185772=CARTESIAN_POINT('Ctrl Pts',(-15.5522658329614,-12.6749798867901,
115.902369499305)) ;
#185773=CARTESIAN_POINT('Ctrl Pts',(-15.5350554014057,-12.6228439781452,
115.849949302042)) ;
#185774=CARTESIAN_POINT('Ctrl Pts',(-15.6088592489752,-12.6228439649152,
115.825718272995)) ;
#185775=CARTESIAN_POINT('Ctrl Pts',(-15.6826630965448,-12.6228439516851,
115.801487243948)) ;
#185776=CARTESIAN_POINT('Ctrl Pts',(-15.6998735281005,-12.67497986033,115.853907441211)) ;
#185777=CARTESIAN_POINT('Ctrl Pts',(-15.6366680399121,-12.9129719673497,
115.696933930181)) ;
#185778=CARTESIAN_POINT('Ctrl Pts',(-15.6575811570006,-12.9485664184321,
115.760631909985)) ;
#185779=CARTESIAN_POINT('Ctrl Pts',(-15.5837773094315,-12.9485664423294,
115.784862939033)) ;
#185780=CARTESIAN_POINT('Ctrl Pts',(-15.5099734618623,-12.9485664662267,
115.809093968081)) ;
#185781=CARTESIAN_POINT('Ctrl Pts',(-15.4890603447738,-12.9129720151443,
115.745395988277)) ;
#185782=CARTESIAN_POINT('Ctrl Pts',(-15.4681472276853,-12.8773775640619,
115.681698008474)) ;
#185783=CARTESIAN_POINT('Ctrl Pts',(-15.5419510752545,-12.8773775401646,
115.657466979426)) ;
#185784=CARTESIAN_POINT('Ctrl Pts',(-15.6157549228236,-12.8773775162673,
115.633235950377)) ;
#185785=CARTESIAN_POINT('Ctrl Pts',(-15.6366680399121,-12.9129719673497,
115.696933930181)) ;
#185786=CARTESIAN_POINT('Ctrl Pts',(-15.5952249708799,-13.1860117694584,
115.606088574179)) ;
#185787=CARTESIAN_POINT('Ctrl Pts',(-15.6183296594594,-13.2025937727261,
115.676461726988)) ;
#185788=CARTESIAN_POINT('Ctrl Pts',(-15.5445258135152,-13.2025938067603,
115.700692760986)) ;
#185789=CARTESIAN_POINT('Ctrl Pts',(-15.4707219675711,-13.2025938407946,
115.724923794983)) ;
#185790=CARTESIAN_POINT('Ctrl Pts',(-15.4476172789917,-13.1860118375269,
115.654550642175)) ;
#185791=CARTESIAN_POINT('Ctrl Pts',(-15.4245125904123,-13.1694298342593,
115.584177489366)) ;
#185792=CARTESIAN_POINT('Ctrl Pts',(-15.4983164363564,-13.169429800225,
115.559946455368)) ;
#185793=CARTESIAN_POINT('Ctrl Pts',(-15.5721202823005,-13.1694297661908,
115.53571542137)) ;
#185794=CARTESIAN_POINT('Ctrl Pts',(-15.5952249708799,-13.1860117694584,
115.606088574179)) ;
#185795=CARTESIAN_POINT('Ctrl Pts',(-15.5773486535781,-13.4763914936473,
115.587122093888)) ;
#185796=CARTESIAN_POINT('Ctrl Pts',(-15.6010006622766,-13.4727232020181,
115.659162295299)) ;
#185797=CARTESIAN_POINT('Ctrl Pts',(-15.5271968193326,-13.4727232458184,
115.683393338435)) ;
#185798=CARTESIAN_POINT('Ctrl Pts',(-15.4533929763885,-13.4727232896187,
115.70762438157)) ;
#185799=CARTESIAN_POINT('Ctrl Pts',(-15.42974096769,-13.4763915812479,115.635584180159)) ;
#185800=CARTESIAN_POINT('Ctrl Pts',(-15.4060889589915,-13.4800598728771,
115.563543978747)) ;
#185801=CARTESIAN_POINT('Ctrl Pts',(-15.4798928019355,-13.4800598290768,
115.539312935612)) ;
#185802=CARTESIAN_POINT('Ctrl Pts',(-15.5536966448795,-13.4800597852765,
115.515081892476)) ;
#185803=CARTESIAN_POINT('Ctrl Pts',(-15.5773486535781,-13.4763914936473,
115.587122093888)) ;
#185804=CARTESIAN_POINT('Ctrl Pts',(-15.5838924485424,-13.7633156829476,
115.642631367891)) ;
#185805=CARTESIAN_POINT('Ctrl Pts',(-15.6063856690625,-13.7396092222064,
115.711142087291)) ;
#185806=CARTESIAN_POINT('Ctrl Pts',(-15.5325818307443,-13.7396092733025,
115.735373144516)) ;
#185807=CARTESIAN_POINT('Ctrl Pts',(-15.4587779924262,-13.7396093243987,
115.759604201741)) ;
#185808=CARTESIAN_POINT('Ctrl Pts',(-15.4362847719061,-13.7633157851398,
115.691093482342)) ;
#185809=CARTESIAN_POINT('Ctrl Pts',(-15.4137915513859,-13.787022245881,
115.622582762942)) ;
#185810=CARTESIAN_POINT('Ctrl Pts',(-15.4875953897041,-13.7870221947849,
115.598351705717)) ;
#185811=CARTESIAN_POINT('Ctrl Pts',(-15.5613992280222,-13.7870221436888,
115.574120648491)) ;
#185812=CARTESIAN_POINT('Ctrl Pts',(-15.5838924485424,-13.7633156829476,
115.642631367891)) ;
#185813=CARTESIAN_POINT('Ctrl Pts',(-15.6133732890566,-14.0239605605361,
115.767794362967)) ;
#185814=CARTESIAN_POINT('Ctrl Pts',(-15.6331087715713,-13.9820221332016,
115.827905457214)) ;
#185815=CARTESIAN_POINT('Ctrl Pts',(-15.5593049386299,-13.9820221845115,
115.852136530816)) ;
#185816=CARTESIAN_POINT('Ctrl Pts',(-15.4855011056886,-13.9820222358214,
115.876367604418)) ;
#185817=CARTESIAN_POINT('Ctrl Pts',(-15.4657656231739,-14.023960663156,
115.816256510171)) ;
#185818=CARTESIAN_POINT('Ctrl Pts',(-15.4460301406592,-14.0658990904905,
115.756145415925)) ;
#185819=CARTESIAN_POINT('Ctrl Pts',(-15.5198339736006,-14.0658990391806,
115.731914342323)) ;
#185820=CARTESIAN_POINT('Ctrl Pts',(-15.5936378065419,-14.0658989878706,
115.707683268721)) ;
#185821=CARTESIAN_POINT('Ctrl Pts',(-15.6133732890566,-14.0239605605361,
115.767794362967)) ;
#185822=CARTESIAN_POINT('Ctrl Pts',(-15.6631890060082,-14.2421936446632,
115.955049772158)) ;
#185823=CARTESIAN_POINT('Ctrl Pts',(-15.678739990713,-14.1849578741807,
116.002415561072)) ;
#185824=CARTESIAN_POINT('Ctrl Pts',(-15.604936163726,-14.1849579203882,
116.026646652811)) ;
#185825=CARTESIAN_POINT('Ctrl Pts',(-15.5311323367391,-14.1849579665956,
116.050877744549)) ;
#185826=CARTESIAN_POINT('Ctrl Pts',(-15.5155813520343,-14.2421937370781,
116.003511955634)) ;
#185827=CARTESIAN_POINT('Ctrl Pts',(-15.5000303673295,-14.2994295075606,
115.95614616672)) ;
#185828=CARTESIAN_POINT('Ctrl Pts',(-15.5738341943165,-14.2994294613532,
115.931915074982)) ;
#185829=CARTESIAN_POINT('Ctrl Pts',(-15.6476380213034,-14.2994294151457,
115.907683983244)) ;
#185830=CARTESIAN_POINT('Ctrl Pts',(-15.6631890060082,-14.2421936446632,
115.955049772158)) ;
#185831=CARTESIAN_POINT('Ctrl Pts',(-15.728520728614,-14.4005934040497,
116.189363403692)) ;
#185832=CARTESIAN_POINT('Ctrl Pts',(-15.7388019491786,-14.3322159891563,
116.220678341182)) ;
#185833=CARTESIAN_POINT('Ctrl Pts',(-15.664998127278,-14.3322160226317,
116.244909448412)) ;
#185834=CARTESIAN_POINT('Ctrl Pts',(-15.5911943053774,-14.332216056107,
116.269140555643)) ;
#185835=CARTESIAN_POINT('Ctrl Pts',(-15.5809130848128,-14.4005934710005,
116.237825618152)) ;
#185836=CARTESIAN_POINT('Ctrl Pts',(-15.5706318642482,-14.4689708858939,
116.206510680662)) ;
#185837=CARTESIAN_POINT('Ctrl Pts',(-15.6444356861487,-14.4689708524185,
116.182279573432)) ;
#185838=CARTESIAN_POINT('Ctrl Pts',(-15.7182395080493,-14.4689708189432,
116.158048466201)) ;
#185839=CARTESIAN_POINT('Ctrl Pts',(-15.728520728614,-14.4005934040497,
116.189363403692)) ;
#185840=CARTESIAN_POINT('Ctrl Pts',(-15.80481754392,-14.4895021228897,116.457354192915)) ;
#185841=CARTESIAN_POINT('Ctrl Pts',(-15.8090502714838,-14.4148177682025,
116.470246396486)) ;
#185842=CARTESIAN_POINT('Ctrl Pts',(-15.7352464541145,-14.4148177835068,
116.494477517518)) ;
#185843=CARTESIAN_POINT('Ctrl Pts',(-15.6614426367453,-14.4148177988111,
116.51870863855)) ;
#185844=CARTESIAN_POINT('Ctrl Pts',(-15.6572099091815,-14.4895021534983,
116.505816434979)) ;
#185845=CARTESIAN_POINT('Ctrl Pts',(-15.6529771816177,-14.5641865081855,
116.492924231409)) ;
#185846=CARTESIAN_POINT('Ctrl Pts',(-15.7267809989869,-14.5641864928812,
116.468693110377)) ;
#185847=CARTESIAN_POINT('Ctrl Pts',(-15.8005848163562,-14.5641864775769,
116.444461989345)) ;
#185848=CARTESIAN_POINT('Ctrl Pts',(-15.80481754392,-14.4895021228897,116.457354192915)) ;
#185849=CARTESIAN_POINT('Ctrl Pts',(-15.8848712831143,-14.5012817728617,
116.736556722847)) ;
#185850=CARTESIAN_POINT('Ctrl Pts',(-15.8827891653978,-14.425666653241,
116.73021492648)) ;
#185851=CARTESIAN_POINT('Ctrl Pts',(-15.8089853501543,-14.4256666452889,
116.754446053986)) ;
#185852=CARTESIAN_POINT('Ctrl Pts',(-15.7351815349108,-14.4256666373369,
116.778677181493)) ;
#185853=CARTESIAN_POINT('Ctrl Pts',(-15.7372636526273,-14.5012817569575,
116.78501897786)) ;
#185854=CARTESIAN_POINT('Ctrl Pts',(-15.7393457703438,-14.5768968765781,
116.791360774228)) ;
#185855=CARTESIAN_POINT('Ctrl Pts',(-15.8131495855873,-14.5768968845302,
116.767129646721)) ;
#185856=CARTESIAN_POINT('Ctrl Pts',(-15.8869534008308,-14.5768968924823,
116.742898519214)) ;
#185857=CARTESIAN_POINT('Ctrl Pts',(-15.8848712831143,-14.5012817728617,
116.736556722847)) ;
#185858=CARTESIAN_POINT('Ctrl Pts',(-15.9632161467547,-14.43501211062,117.010828764806)) ;
#185859=CARTESIAN_POINT('Ctrl Pts',(-15.9549236920078,-14.363912820796,
116.985571283752)) ;
#185860=CARTESIAN_POINT('Ctrl Pts',(-15.8811198769776,-14.3639127866614,
117.009802411908)) ;
#185861=CARTESIAN_POINT('Ctrl Pts',(-15.8073160619473,-14.3639127525269,
117.034033540064)) ;
#185862=CARTESIAN_POINT('Ctrl Pts',(-15.8156085166942,-14.4350120423509,
117.059291021119)) ;
#185863=CARTESIAN_POINT('Ctrl Pts',(-15.823900971441,-14.506111332175,117.084548502173)) ;
#185864=CARTESIAN_POINT('Ctrl Pts',(-15.8977047864712,-14.5061113663095,
117.060317374017)) ;
#185865=CARTESIAN_POINT('Ctrl Pts',(-15.9715086015015,-14.5061114004441,
117.036086245861)) ;
#185866=CARTESIAN_POINT('Ctrl Pts',(-15.9632161467547,-14.43501211062,117.010828764806)) ;
#185867=CARTESIAN_POINT('Ctrl Pts',(-16.0321824010801,-14.2968843843662,
117.256163976492)) ;
#185868=CARTESIAN_POINT('Ctrl Pts',(-16.0183329772586,-14.2353253070851,
117.213980864183)) ;
#185869=CARTESIAN_POINT('Ctrl Pts',(-15.9445291592642,-14.2353252479564,
117.238211983311)) ;
#185870=CARTESIAN_POINT('Ctrl Pts',(-15.8707253412697,-14.2353251888277,
117.262443102438)) ;
#185871=CARTESIAN_POINT('Ctrl Pts',(-15.8845747650913,-14.2968842661087,
117.304626214748)) ;
#185872=CARTESIAN_POINT('Ctrl Pts',(-15.8984241889128,-14.3584433433898,
117.346809327058)) ;
#185873=CARTESIAN_POINT('Ctrl Pts',(-15.9722280069073,-14.3584434025185,
117.32257820793)) ;
#185874=CARTESIAN_POINT('Ctrl Pts',(-16.0460318249017,-14.3584434616473,
117.298347088802)) ;
#185875=CARTESIAN_POINT('Ctrl Pts',(-16.0321824010801,-14.2968843843662,
117.256163976492)) ;
#185876=CARTESIAN_POINT('Ctrl Pts',(-16.0872824733374,-14.0952651274861,
117.459484020203)) ;
#185877=CARTESIAN_POINT('Ctrl Pts',(-16.0688314524017,-14.0476919571474,
117.403285185476)) ;
#185878=CARTESIAN_POINT('Ctrl Pts',(-15.9950276293236,-14.0476918755957,
117.42751628912)) ;
#185879=CARTESIAN_POINT('Ctrl Pts',(-15.9212238062455,-14.047691794044,
117.451747392764)) ;
#185880=CARTESIAN_POINT('Ctrl Pts',(-15.9396748271812,-14.0952649643827,
117.507946227491)) ;
#185881=CARTESIAN_POINT('Ctrl Pts',(-15.9581258481169,-14.1428381347214,
117.564145062217)) ;
#185882=CARTESIAN_POINT('Ctrl Pts',(-16.031929671195,-14.1428382162731,
117.539913958574)) ;
#185883=CARTESIAN_POINT('Ctrl Pts',(-16.1057334942731,-14.1428382978248,
117.51568285493)) ;
#185884=CARTESIAN_POINT('Ctrl Pts',(-16.0872824733374,-14.0952651274861,
117.459484020203)) ;
#185885=CARTESIAN_POINT('Ctrl Pts',(-16.1232711688005,-13.8453444760412,
117.604537921654)) ;
#185886=CARTESIAN_POINT('Ctrl Pts',(-16.101547172297,-13.8151498849244,
117.538370131394)) ;
#185887=CARTESIAN_POINT('Ctrl Pts',(-16.0277433420106,-13.8151497867456,
117.562601213082)) ;
#185888=CARTESIAN_POINT('Ctrl Pts',(-15.9539395117242,-13.8151496885667,
117.586832294771)) ;
#185889=CARTESIAN_POINT('Ctrl Pts',(-15.9756635082278,-13.8453442796835,
117.653000085031)) ;
#185890=CARTESIAN_POINT('Ctrl Pts',(-15.9973875047314,-13.8755388708002,
117.719167875291)) ;
#185891=CARTESIAN_POINT('Ctrl Pts',(-16.0711913350178,-13.8755389689791,
117.694936793603)) ;
#185892=CARTESIAN_POINT('Ctrl Pts',(-16.1449951653041,-13.8755390671579,
117.670705711914)) ;
#185893=CARTESIAN_POINT('Ctrl Pts',(-16.1232711688005,-13.8453444760412,
117.604537921654)) ;
#185894=CARTESIAN_POINT('Ctrl Pts',(-16.1369703680654,-13.5639203016943,
117.681820810949)) ;
#185895=CARTESIAN_POINT('Ctrl Pts',(-16.1135220904896,-13.5533288537195,
117.610401138726)) ;
#185896=CARTESIAN_POINT('Ctrl Pts',(-16.0397182516176,-13.5533287463832,
117.634632194264)) ;
#185897=CARTESIAN_POINT('Ctrl Pts',(-15.9659144127456,-13.5533286390469,
117.658863249802)) ;
#185898=CARTESIAN_POINT('Ctrl Pts',(-15.9893626903214,-13.5639200870216,
117.730282922026)) ;
#185899=CARTESIAN_POINT('Ctrl Pts',(-16.0128109678972,-13.5745115349964,
117.801702594249)) ;
#185900=CARTESIAN_POINT('Ctrl Pts',(-16.0866148067692,-13.5745116423327,
117.777471538711)) ;
#185901=CARTESIAN_POINT('Ctrl Pts',(-16.1604186456412,-13.574511749669,
117.753240483173)) ;
#185902=CARTESIAN_POINT('Ctrl Pts',(-16.1369703680654,-13.5639203016943,
117.681820810949)) ;
#185903=CARTESIAN_POINT('Ctrl Pts',(-16.1263949656492,-13.2722319962961,
117.685137077864)) ;
#185904=CARTESIAN_POINT('Ctrl Pts',(-16.102915121327,-13.2819894198182,
117.613621258424)) ;
#185905=CARTESIAN_POINT('Ctrl Pts',(-16.0291112733662,-13.2819893125246,
117.637852286279)) ;
#185906=CARTESIAN_POINT('Ctrl Pts',(-15.9553074254054,-13.281989205231,
117.662083314134)) ;
#185907=CARTESIAN_POINT('Ctrl Pts',(-15.9787872697277,-13.2722317817088,
117.733599133574)) ;
#185908=CARTESIAN_POINT('Ctrl Pts',(-16.0022671140499,-13.2624743581867,
117.805114953013)) ;
#185909=CARTESIAN_POINT('Ctrl Pts',(-16.0760709620107,-13.2624744654803,
117.780883925158)) ;
#185910=CARTESIAN_POINT('Ctrl Pts',(-16.1498748099715,-13.262474572774,
117.756652897303)) ;
#185911=CARTESIAN_POINT('Ctrl Pts',(-16.1263949656492,-13.2722319962961,
117.685137077864)) ;
#185912=CARTESIAN_POINT('Ctrl Pts',(-16.0919950705927,-12.9927108288244,
117.6156635482)) ;
#185913=CARTESIAN_POINT('Ctrl Pts',(-16.070151731594,-13.0219980101555,
117.549132259942)) ;
#185914=CARTESIAN_POINT('Ctrl Pts',(-15.9963478750301,-13.0219979113137,
117.573363261593)) ;
#185915=CARTESIAN_POINT('Ctrl Pts',(-15.9225440184661,-13.0219978124719,
117.597594263245)) ;
#185916=CARTESIAN_POINT('Ctrl Pts',(-15.9443873574648,-12.9927106311408,
117.664125551502)) ;
#185917=CARTESIAN_POINT('Ctrl Pts',(-15.9662306964635,-12.9634234498097,
117.730656839759)) ;
#185918=CARTESIAN_POINT('Ctrl Pts',(-16.0400345530275,-12.9634235486515,
117.706425838108)) ;
#185919=CARTESIAN_POINT('Ctrl Pts',(-16.1138384095914,-12.9634236474933,
117.682194836457)) ;
#185920=CARTESIAN_POINT('Ctrl Pts',(-16.0919950705927,-12.9927108288244,
117.6156635482)) ;
#185921=CARTESIAN_POINT('Ctrl Pts',(-16.0350077383484,-12.7419081122581,
117.477619455827)) ;
#185922=CARTESIAN_POINT('Ctrl Pts',(-16.016375282967,-12.7887491311702,
117.420868001036)) ;
#185923=CARTESIAN_POINT('Ctrl Pts',(-15.942571419085,-12.78874904886,117.445098980398)) ;
#185924=CARTESIAN_POINT('Ctrl Pts',(-15.8687675552031,-12.7887489665498,
117.46932995976)) ;
#185925=CARTESIAN_POINT('Ctrl Pts',(-15.8874000105845,-12.7419079476376,
117.52608141455)) ;
#185926=CARTESIAN_POINT('Ctrl Pts',(-15.9060324659659,-12.6950669287254,
117.582832869341)) ;
#185927=CARTESIAN_POINT('Ctrl Pts',(-15.9798363298478,-12.6950670110357,
117.558601889979)) ;
#185928=CARTESIAN_POINT('Ctrl Pts',(-16.0536401937297,-12.6950670933459,
117.534370910617)) ;
#185929=CARTESIAN_POINT('Ctrl Pts',(-16.0350077383484,-12.7419081122581,
117.477619455827)) ;
#185930=CARTESIAN_POINT('Ctrl Pts',(-15.9591220993108,-12.5402274188012,
117.281908126571)) ;
#185931=CARTESIAN_POINT('Ctrl Pts',(-15.9450269627281,-12.6012191381552,
117.238976612807)) ;
#185932=CARTESIAN_POINT('Ctrl Pts',(-15.8712230935302,-12.6012190780927,
117.263207575978)) ;
#185933=CARTESIAN_POINT('Ctrl Pts',(-15.7974192243324,-12.6012190180302,
117.287438539148)) ;
#185934=CARTESIAN_POINT('Ctrl Pts',(-15.8115143609151,-12.5402272986761,
117.330370052912)) ;
#185935=CARTESIAN_POINT('Ctrl Pts',(-15.8256094974978,-12.479235579322,
117.373301566676)) ;
#185936=CARTESIAN_POINT('Ctrl Pts',(-15.8994133666956,-12.4792356393845,
117.349070603506)) ;
#185937=CARTESIAN_POINT('Ctrl Pts',(-15.9732172358935,-12.4792356994471,
117.324839640335)) ;
#185938=CARTESIAN_POINT('Ctrl Pts',(-15.9591220993108,-12.5402274188012,
117.281908126571)) ;
#185939=CARTESIAN_POINT('Ctrl Pts',(-15.8687073550715,-12.4011175779625,
117.042022844154)) ;
#185940=CARTESIAN_POINT('Ctrl Pts',(-15.8601689623456,-12.4719130809355,
117.016016275687)) ;
#185941=CARTESIAN_POINT('Ctrl Pts',(-15.7863650903915,-12.4719130465785,
117.040247230462)) ;
#185942=CARTESIAN_POINT('Ctrl Pts',(-15.7125612184373,-12.4719130122216,
117.064478185237)) ;
#185943=CARTESIAN_POINT('Ctrl Pts',(-15.7210996111632,-12.4011175092485,
117.090484753705)) ;
#185944=CARTESIAN_POINT('Ctrl Pts',(-15.729638003889,-12.3303220062755,
117.116491322172)) ;
#185945=CARTESIAN_POINT('Ctrl Pts',(-15.8034418758432,-12.3303220406325,
117.092260367396)) ;
#185946=CARTESIAN_POINT('Ctrl Pts',(-15.8772457477973,-12.3303220749894,
117.068029412621)) ;
#185947=CARTESIAN_POINT('Ctrl Pts',(-15.8687073550715,-12.4011175779625,
117.042022844154)) ;
#185948=CARTESIAN_POINT('Ctrl Pts',(-15.7700176989328,-12.3349520470046,
116.776796250554)) ;
#185949=CARTESIAN_POINT('Ctrl Pts',(-15.767625022208,-12.4104731774987,
116.769508541507)) ;
#185950=CARTESIAN_POINT('Ctrl Pts',(-15.6938211498566,-12.4104731691892,
116.793739495072)) ;
#185951=CARTESIAN_POINT('Ctrl Pts',(-15.6200172775051,-12.4104731608796,
116.817970448637)) ;
#185952=CARTESIAN_POINT('Ctrl Pts',(-15.6224099542299,-12.3349520303855,
116.825258157684)) ;
#185953=CARTESIAN_POINT('Ctrl Pts',(-15.6248026309546,-12.2594308998913,
116.832545866731)) ;
#185954=CARTESIAN_POINT('Ctrl Pts',(-15.6986065033061,-12.2594309082008,
116.808314913166)) ;
#185955=CARTESIAN_POINT('Ctrl Pts',(-15.7724103756575,-12.2594309165104,
116.784083959601)) ;
#185956=CARTESIAN_POINT('Ctrl Pts',(-15.7700176989328,-12.3349520470046,
116.776796250554)) ;
#185957=CARTESIAN_POINT('Ctrl Pts',(-15.6682261809247,-12.346456548631,
116.502406394127)) ;
#185958=CARTESIAN_POINT('Ctrl Pts',(-15.6721990720837,-12.4212888141347,
116.514507177916)) ;
#185959=CARTESIAN_POINT('Ctrl Pts',(-15.5983952023686,-12.4212888296186,
116.538738139512)) ;
#185960=CARTESIAN_POINT('Ctrl Pts',(-15.5245913326536,-12.4212888451025,
116.562969101107)) ;
#185961=CARTESIAN_POINT('Ctrl Pts',(-15.5206184414946,-12.3464565795988,
116.550868317317)) ;
#185962=CARTESIAN_POINT('Ctrl Pts',(-15.5166455503357,-12.2716243140951,
116.538767533527)) ;
#185963=CARTESIAN_POINT('Ctrl Pts',(-15.5904494200508,-12.2716242986112,
116.514536571932)) ;
#185964=CARTESIAN_POINT('Ctrl Pts',(-15.6642532897658,-12.2716242831273,
116.490305610337)) ;
#185965=CARTESIAN_POINT('Ctrl Pts',(-15.6682261809247,-12.346456548631,
116.502406394127)) ;
#185966=CARTESIAN_POINT('Ctrl Pts',(-15.5714939849773,-12.4344867986536,
116.243115588663)) ;
#185967=CARTESIAN_POINT('Ctrl Pts',(-15.5814953588048,-12.5032854856229,
116.273578158085)) ;
#185968=CARTESIAN_POINT('Ctrl Pts',(-15.5076914930099,-12.5032855202655,
116.297809131621)) ;
#185969=CARTESIAN_POINT('Ctrl Pts',(-15.4338876272149,-12.503285554908,
116.322040105156)) ;
#185970=CARTESIAN_POINT('Ctrl Pts',(-15.4238862533874,-12.4344868679388,
116.291577535733)) ;
#185971=CARTESIAN_POINT('Ctrl Pts',(-15.4138848795598,-12.3656881809695,
116.261114966311)) ;
#185972=CARTESIAN_POINT('Ctrl Pts',(-15.4876887453548,-12.365688146327,
116.236883992776)) ;
#185973=CARTESIAN_POINT('Ctrl Pts',(-15.5614926111498,-12.3656881116844,
116.21265301924)) ;
#185974=CARTESIAN_POINT('Ctrl Pts',(-15.5714939849773,-12.4344867986536,
116.243115588663)) ;
#185975=CARTESIAN_POINT('Ctrl Pts',(-15.4847018094329,-12.5932721982848,
116.014273618595)) ;
#185976=CARTESIAN_POINT('Ctrl Pts',(-15.5000432541393,-12.6510887725529,
116.061001182452)) ;
#185977=CARTESIAN_POINT('Ctrl Pts',(-15.4262393939096,-12.6510888198682,
116.085232172938)) ;
#185978=CARTESIAN_POINT('Ctrl Pts',(-15.3524355336799,-12.6510888671835,
116.109463163424)) ;
#185979=CARTESIAN_POINT('Ctrl Pts',(-15.3370940889735,-12.5932722929155,
116.062735599568)) ;
#185980=CARTESIAN_POINT('Ctrl Pts',(-15.3217526442671,-12.5354557186474,
116.016008035711)) ;
#185981=CARTESIAN_POINT('Ctrl Pts',(-15.3955565044968,-12.5354556713321,
115.991777045225)) ;
#185982=CARTESIAN_POINT('Ctrl Pts',(-15.4693603647265,-12.5354556240167,
115.967546054739)) ;
#185983=CARTESIAN_POINT('Ctrl Pts',(-15.4847018094329,-12.5932721982848,
116.014273618595)) ;
#185984=CARTESIAN_POINT('Ctrl Pts',(-15.4140311873583,-12.8103924299054,
115.834395867115)) ;
#185985=CARTESIAN_POINT('Ctrl Pts',(-15.4335980718028,-12.8531370145114,
115.893993438782)) ;
#185986=CARTESIAN_POINT('Ctrl Pts',(-15.3597942173693,-12.8531370683972,
115.918224446923)) ;
#185987=CARTESIAN_POINT('Ctrl Pts',(-15.2859903629358,-12.8531371222829,
115.942455455063)) ;
#185988=CARTESIAN_POINT('Ctrl Pts',(-15.2664234784913,-12.810392537677,
115.882857883396)) ;
#185989=CARTESIAN_POINT('Ctrl Pts',(-15.2468565940469,-12.767647953071,
115.823260311728)) ;
#185990=CARTESIAN_POINT('Ctrl Pts',(-15.3206604484804,-12.7676478991852,
115.799029303588)) ;
#185991=CARTESIAN_POINT('Ctrl Pts',(-15.3944643029138,-12.7676478452995,
115.774798295448)) ;
#185992=CARTESIAN_POINT('Ctrl Pts',(-15.4140311873583,-12.8103924299054,
115.834395867115)) ;
#185993=CARTESIAN_POINT('Ctrl Pts',(-15.3631390797612,-13.0726323412443,
115.714998308832)) ;
#185994=CARTESIAN_POINT('Ctrl Pts',(-15.3855521726195,-13.0971322435792,
115.783264972285)) ;
#185995=CARTESIAN_POINT('Ctrl Pts',(-15.3117483240823,-13.0971322955942,
115.807495998385)) ;
#185996=CARTESIAN_POINT('Ctrl Pts',(-15.2379444755452,-13.0971323476091,
115.831727024485)) ;
#185997=CARTESIAN_POINT('Ctrl Pts',(-15.2155313826869,-13.0726324452743,
115.763460361032)) ;
#185998=CARTESIAN_POINT('Ctrl Pts',(-15.1931182898287,-13.0481325429394,
115.695193697579)) ;
#185999=CARTESIAN_POINT('Ctrl Pts',(-15.2669221383658,-13.0481324909245,
115.670962671479)) ;
#186000=CARTESIAN_POINT('Ctrl Pts',(-15.3407259869029,-13.0481324389095,
115.646731645379)) ;
#186001=CARTESIAN_POINT('Ctrl Pts',(-15.3631390797612,-13.0726323412443,
115.714998308832)) ;
#186002=CARTESIAN_POINT('Ctrl Pts',(-15.335631959363,-13.3588849654739,
115.66670490255)) ;
#186003=CARTESIAN_POINT('Ctrl Pts',(-15.359265307546,-13.3634353466295,
115.738688267008)) ;
#186004=CARTESIAN_POINT('Ctrl Pts',(-15.2854614635794,-13.3634353921752,
115.762919307028)) ;
#186005=CARTESIAN_POINT('Ctrl Pts',(-15.2116576196127,-13.3634354377208,
115.787150347049)) ;
#186006=CARTESIAN_POINT('Ctrl Pts',(-15.1880242714297,-13.3588850565651,
115.715166982591)) ;
#186007=CARTESIAN_POINT('Ctrl Pts',(-15.1643909232466,-13.3543346754094,
115.643183618133)) ;
#186008=CARTESIAN_POINT('Ctrl Pts',(-15.2381947672133,-13.3543346298638,
115.618952578112)) ;
#186009=CARTESIAN_POINT('Ctrl Pts',(-15.3119986111799,-13.3543345843182,
115.594721538092)) ;
#186010=CARTESIAN_POINT('Ctrl Pts',(-15.335631959363,-13.3588849654739,
115.66670490255)) ;
#186011=CARTESIAN_POINT('Ctrl Pts',(-15.3323120932461,-13.6479812710763,
115.691913999484)) ;
#186012=CARTESIAN_POINT('Ctrl Pts',(-15.3554820543391,-13.6323532637261,
115.762485961773)) ;
#186013=CARTESIAN_POINT('Ctrl Pts',(-15.2816782136833,-13.6323533009956,
115.786717011878)) ;
#186014=CARTESIAN_POINT('Ctrl Pts',(-15.2078743730274,-13.632353338265,
115.810948061983)) ;
#186015=CARTESIAN_POINT('Ctrl Pts',(-15.1847044119345,-13.6479813456151,
115.740376099694)) ;
#186016=CARTESIAN_POINT('Ctrl Pts',(-15.1615344508415,-13.6636093529653,
115.669804137404)) ;
#186017=CARTESIAN_POINT('Ctrl Pts',(-15.2353382914973,-13.6636093156958,
115.645573087299)) ;
#186018=CARTESIAN_POINT('Ctrl Pts',(-15.3091421321531,-13.6636092784264,
115.621342037194)) ;
#186019=CARTESIAN_POINT('Ctrl Pts',(-15.3323120932461,-13.6479812710763,
115.691913999484)) ;
#186020=CARTESIAN_POINT('Ctrl Pts',(-15.3527558752554,-13.9223253071587,
115.789719726039)) ;
#186021=CARTESIAN_POINT('Ctrl Pts',(-15.3737981985428,-13.8875179705717,
115.853811247044)) ;
#186022=CARTESIAN_POINT('Ctrl Pts',(-15.2999943595609,-13.8875179960034,
115.878042302247)) ;
#186023=CARTESIAN_POINT('Ctrl Pts',(-15.2261905205791,-13.8875180214352,
115.902273357451)) ;
#186024=CARTESIAN_POINT('Ctrl Pts',(-15.2051481972916,-13.9223253580222,
115.838181836446)) ;
#186025=CARTESIAN_POINT('Ctrl Pts',(-15.1841058740042,-13.9571326946092,
115.774090315441)) ;
#186026=CARTESIAN_POINT('Ctrl Pts',(-15.2579097129861,-13.9571326691774,
115.749859260238)) ;
#186027=CARTESIAN_POINT('Ctrl Pts',(-15.3317135519679,-13.9571326437457,
115.725628205034)) ;
#186028=CARTESIAN_POINT('Ctrl Pts',(-15.3527558752554,-13.9223253071587,
115.789719726039)) ;
#186029=CARTESIAN_POINT('Ctrl Pts',(-15.3947103578552,-14.1598247969233,
115.952946574138)) ;
#186030=CARTESIAN_POINT('Ctrl Pts',(-15.4121217162786,-14.1083816279705,
116.005978762172)) ;
#186031=CARTESIAN_POINT('Ctrl Pts',(-15.3383178775536,-14.1083816430256,
116.030209818158)) ;
#186032=CARTESIAN_POINT('Ctrl Pts',(-15.2645140388287,-14.1083816580807,
116.054440874144)) ;
#186033=CARTESIAN_POINT('Ctrl Pts',(-15.2471026804054,-14.1598248270335,
116.00140868611)) ;
#186034=CARTESIAN_POINT('Ctrl Pts',(-15.229691321982,-14.2112679959863,
115.948376498076)) ;
#186035=CARTESIAN_POINT('Ctrl Pts',(-15.303495160707,-14.2112679809312,
115.92414544209)) ;
#186036=CARTESIAN_POINT('Ctrl Pts',(-15.3772989994319,-14.2112679658761,
115.899914386104)) ;
#186037=CARTESIAN_POINT('Ctrl Pts',(-15.3947103578552,-14.1598247969233,
115.952946574138)) ;
#186038=CARTESIAN_POINT('Ctrl Pts',(-15.4546404114478,-14.3448019435796,
116.171044680752)) ;
#186039=CARTESIAN_POINT('Ctrl Pts',(-15.4671576233587,-14.2803646984367,
116.209170088335)) ;
#186040=CARTESIAN_POINT('Ctrl Pts',(-15.3933537835408,-14.2803647047343,
116.233401140992)) ;
#186041=CARTESIAN_POINT('Ctrl Pts',(-15.3195499437229,-14.2803647110319,
116.257632193649)) ;
#186042=CARTESIAN_POINT('Ctrl Pts',(-15.307032731812,-14.3448019561748,
116.219506786067)) ;
#186043=CARTESIAN_POINT('Ctrl Pts',(-15.2945155199011,-14.4092392013176,
116.181381378484)) ;
#186044=CARTESIAN_POINT('Ctrl Pts',(-15.368319359719,-14.40923919502,116.157150325827)) ;
#186045=CARTESIAN_POINT('Ctrl Pts',(-15.4421231995369,-14.4092391887224,
116.13291927317)) ;
#186046=CARTESIAN_POINT('Ctrl Pts',(-15.4546404114478,-14.3448019435796,
116.171044680752)) ;
#186047=CARTESIAN_POINT('Ctrl Pts',(-15.527126191388,-14.4625579261475,
116.427260546478)) ;
#186048=CARTESIAN_POINT('Ctrl Pts',(-15.5338675385338,-14.3898012184393,
116.447793602035)) ;
#186049=CARTESIAN_POINT('Ctrl Pts',(-15.4600636972832,-14.3898012199962,
116.472024650328)) ;
#186050=CARTESIAN_POINT('Ctrl Pts',(-15.3862598560326,-14.3898012215531,
116.496255698622)) ;
#186051=CARTESIAN_POINT('Ctrl Pts',(-15.3795185088869,-14.4625579292612,
116.475722643065)) ;
#186052=CARTESIAN_POINT('Ctrl Pts',(-15.3727771617411,-14.5353146369693,
116.455189587508)) ;
#186053=CARTESIAN_POINT('Ctrl Pts',(-15.4465810029917,-14.5353146354125,
116.430958539215)) ;
#186054=CARTESIAN_POINT('Ctrl Pts',(-15.5203848442423,-14.5353146338556,
116.406727490921)) ;
#186055=CARTESIAN_POINT('Ctrl Pts',(-15.527126191388,-14.4625579261475,
116.427260546478)) ;
#186056=CARTESIAN_POINT('Ctrl Pts',(-15.6061068479536,-14.5058691718866,
116.703142474044)) ;
#186057=CARTESIAN_POINT('Ctrl Pts',(-15.6066125191928,-14.4299792998369,
116.704682666998)) ;
#186058=CARTESIAN_POINT('Ctrl Pts',(-15.5328086766044,-14.429979299475,
116.728913711217)) ;
#186059=CARTESIAN_POINT('Ctrl Pts',(-15.4590048340161,-14.4299792991131,
116.753144755436)) ;
#186060=CARTESIAN_POINT('Ctrl Pts',(-15.4584991627769,-14.5058691711628,
116.751604562482)) ;
#186061=CARTESIAN_POINT('Ctrl Pts',(-15.4579934915378,-14.5817590432124,
116.750064369528)) ;
#186062=CARTESIAN_POINT('Ctrl Pts',(-15.5317973341261,-14.5817590435743,
116.725833325309)) ;
#186063=CARTESIAN_POINT('Ctrl Pts',(-15.6056011767145,-14.5817590439362,
116.70160228109)) ;
#186064=CARTESIAN_POINT('Ctrl Pts',(-15.6061068479536,-14.5058691718866,
116.703142474044)) ;
#186065=CARTESIAN_POINT('Ctrl Pts',(-15.6860762715054,-14.471221053196,
116.98231319858)) ;
#186066=CARTESIAN_POINT('Ctrl Pts',(-15.6802618468492,-14.3976366078093,
116.964603399263)) ;
#186067=CARTESIAN_POINT('Ctrl Pts',(-15.6064580029253,-14.397636607939,
116.988834439414)) ;
#186068=CARTESIAN_POINT('Ctrl Pts',(-15.5326541590014,-14.3976366080687,
117.013065479565)) ;
#186069=CARTESIAN_POINT('Ctrl Pts',(-15.5384685836576,-14.4712210534553,
117.030775278883)) ;
#186070=CARTESIAN_POINT('Ctrl Pts',(-15.5442830083138,-14.5448054988419,
117.0484850782)) ;
#186071=CARTESIAN_POINT('Ctrl Pts',(-15.6180868522377,-14.5448054987123,
117.024254038049)) ;
#186072=CARTESIAN_POINT('Ctrl Pts',(-15.6918906961616,-14.5448054985826,
117.000022997898)) ;
#186073=CARTESIAN_POINT('Ctrl Pts',(-15.6860762715054,-14.471221053196,
116.98231319858)) ;
#186074=CARTESIAN_POINT('Ctrl Pts',(-15.7595355968029,-14.3613267795073,
117.241458486077)) ;
#186075=CARTESIAN_POINT('Ctrl Pts',(-15.7478503794398,-14.2953066789367,
117.205867199456)) ;
#186076=CARTESIAN_POINT('Ctrl Pts',(-15.6740465351294,-14.2953066805575,
117.23009823843)) ;
#186077=CARTESIAN_POINT('Ctrl Pts',(-15.6002426908189,-14.2953066821784,
117.254329277403)) ;
#186078=CARTESIAN_POINT('Ctrl Pts',(-15.611927908182,-14.361326782749,117.289920564025)) ;
#186079=CARTESIAN_POINT('Ctrl Pts',(-15.6236131255451,-14.4273468833197,
117.325511850646)) ;
#186080=CARTESIAN_POINT('Ctrl Pts',(-15.6974169698556,-14.4273468816988,
117.301280811672)) ;
#186081=CARTESIAN_POINT('Ctrl Pts',(-15.771220814166,-14.4273468800779,
117.277049772699)) ;
#186082=CARTESIAN_POINT('Ctrl Pts',(-15.7595355968029,-14.3613267795073,
117.241458486077)) ;
#186083=CARTESIAN_POINT('Ctrl Pts',(-15.8211678092068,-14.1831445066676,
117.464752006046)) ;
#186084=CARTESIAN_POINT('Ctrl Pts',(-15.8044252431337,-14.1294690686809,
117.413756851243)) ;
#186085=CARTESIAN_POINT('Ctrl Pts',(-15.7306213991478,-14.1294690707301,
117.437987891205)) ;
#186086=CARTESIAN_POINT('Ctrl Pts',(-15.6568175551618,-14.1294690727794,
117.462218931167)) ;
#186087=CARTESIAN_POINT('Ctrl Pts',(-15.6735601212348,-14.1831445107661,
117.513214085969)) ;
#186088=CARTESIAN_POINT('Ctrl Pts',(-15.6903026873078,-14.2368199487529,
117.564209240772)) ;
#186089=CARTESIAN_POINT('Ctrl Pts',(-15.7641065312938,-14.2368199467036,
117.53997820081)) ;
#186090=CARTESIAN_POINT('Ctrl Pts',(-15.8379103752798,-14.2368199446543,
117.515747160848)) ;
#186091=CARTESIAN_POINT('Ctrl Pts',(-15.8211678092068,-14.1831445066676,
117.464752006046)) ;
#186092=CARTESIAN_POINT('Ctrl Pts',(-15.8652118608313,-13.9512771233317,
117.634264239109)) ;
#186093=CARTESIAN_POINT('Ctrl Pts',(-15.8446375283888,-13.9137135164908,
117.571598142153)) ;
#186094=CARTESIAN_POINT('Ctrl Pts',(-15.7708336850023,-13.9137135169973,
117.59582918394)) ;
#186095=CARTESIAN_POINT('Ctrl Pts',(-15.6970298416157,-13.9137135175038,
117.620060225728)) ;
#186096=CARTESIAN_POINT('Ctrl Pts',(-15.7176041740582,-13.9512771243447,
117.682726322684)) ;
#186097=CARTESIAN_POINT('Ctrl Pts',(-15.7381785065007,-13.9888407311855,
117.74539241964)) ;
#186098=CARTESIAN_POINT('Ctrl Pts',(-15.8119823498873,-13.988840730679,
117.721161377852)) ;
#186099=CARTESIAN_POINT('Ctrl Pts',(-15.8857861932738,-13.9888407301726,
117.696930336064)) ;
#186100=CARTESIAN_POINT('Ctrl Pts',(-15.8652118608313,-13.9512771233317,
117.634264239109)) ;
#186101=CARTESIAN_POINT('Ctrl Pts',(-15.8882370524503,-13.6804917592119,
117.739885224289)) ;
#186102=CARTESIAN_POINT('Ctrl Pts',(-15.8652903721225,-13.6617810820817,
117.669993338368)) ;
#186103=CARTESIAN_POINT('Ctrl Pts',(-15.7914865291288,-13.6617810784038,
117.694224381352)) ;
#186104=CARTESIAN_POINT('Ctrl Pts',(-15.717682686135,-13.6617810747259,
117.718455424336)) ;
#186105=CARTESIAN_POINT('Ctrl Pts',(-15.7406293664628,-13.6804917518562,
117.788347310257)) ;
#186106=CARTESIAN_POINT('Ctrl Pts',(-15.7635760467906,-13.6992024289864,
117.858239196178)) ;
#186107=CARTESIAN_POINT('Ctrl Pts',(-15.8373798897843,-13.6992024326643,
117.834008153193)) ;
#186108=CARTESIAN_POINT('Ctrl Pts',(-15.9111837327781,-13.6992024363421,
117.809777110209)) ;
#186109=CARTESIAN_POINT('Ctrl Pts',(-15.8882370524503,-13.6804917592119,
117.739885224289)) ;
#186110=CARTESIAN_POINT('Ctrl Pts',(-15.8876883146916,-13.3916820675785,
117.773598447878)) ;
#186111=CARTESIAN_POINT('Ctrl Pts',(-15.8640143289905,-13.3931100750182,
117.701491307042)) ;
#186112=CARTESIAN_POINT('Ctrl Pts',(-15.7902104856931,-13.3931100660094,
117.725722349101)) ;
#186113=CARTESIAN_POINT('Ctrl Pts',(-15.7164066423956,-13.3931100570005,
117.74995339116)) ;
#186114=CARTESIAN_POINT('Ctrl Pts',(-15.7400806280968,-13.3916820495608,
117.822060531996)) ;
#186115=CARTESIAN_POINT('Ctrl Pts',(-15.7637546137979,-13.390254042121,
117.894167672832)) ;
#186116=CARTESIAN_POINT('Ctrl Pts',(-15.8375584570953,-13.3902540511299,
117.869936630773)) ;
#186117=CARTESIAN_POINT('Ctrl Pts',(-15.9113623003928,-13.3902540601387,
117.845705588714)) ;
#186118=CARTESIAN_POINT('Ctrl Pts',(-15.8876883146916,-13.3916820675785,
117.773598447878)) ;
#186119=CARTESIAN_POINT('Ctrl Pts',(-15.8627383173475,-13.10326146677,117.733182994211)) ;
#186120=CARTESIAN_POINT('Ctrl Pts',(-15.8400356809096,-13.1248302660667,
117.664034426357)) ;
#186121=CARTESIAN_POINT('Ctrl Pts',(-15.7662318362027,-13.12483024999,117.688265464123)) ;
#186122=CARTESIAN_POINT('Ctrl Pts',(-15.6924279914958,-13.1248302339134,
117.712496501889)) ;
#186123=CARTESIAN_POINT('Ctrl Pts',(-15.7151306279336,-13.1032614346168,
117.781645069743)) ;
#186124=CARTESIAN_POINT('Ctrl Pts',(-15.7378332643715,-13.0816926353201,
117.850793637597)) ;
#186125=CARTESIAN_POINT('Ctrl Pts',(-15.8116371090784,-13.0816926513967,
117.82656259983)) ;
#186126=CARTESIAN_POINT('Ctrl Pts',(-15.8854409537853,-13.0816926674734,
117.802331562064)) ;
#186127=CARTESIAN_POINT('Ctrl Pts',(-15.8627383173475,-13.10326146677,117.733182994211)) ;
#186128=CARTESIAN_POINT('Ctrl Pts',(-15.8145961245661,-12.8385043736975,
117.621981799066)) ;
#186129=CARTESIAN_POINT('Ctrl Pts',(-15.794488798957,-12.8785902983801,
117.560738129102)) ;
#186130=CARTESIAN_POINT('Ctrl Pts',(-15.7206849517495,-12.8785902776547,
117.584969159251)) ;
#186131=CARTESIAN_POINT('Ctrl Pts',(-15.6468811045419,-12.8785902569293,
117.609200189401)) ;
#186132=CARTESIAN_POINT('Ctrl Pts',(-15.6669884301511,-12.8385043322466,
117.670443859365)) ;
#186133=CARTESIAN_POINT('Ctrl Pts',(-15.6870957557602,-12.7984184075639,
117.73168752933)) ;
#186134=CARTESIAN_POINT('Ctrl Pts',(-15.7608996029678,-12.7984184282893,
117.70745649918)) ;
#186135=CARTESIAN_POINT('Ctrl Pts',(-15.8347034501753,-12.7984184490148,
117.683225469031)) ;
#186136=CARTESIAN_POINT('Ctrl Pts',(-15.8145961245661,-12.8385043736975,
117.621981799066)) ;
#186137=CARTESIAN_POINT('Ctrl Pts',(-15.7456754097843,-12.6146172171064,
117.447606611484)) ;
#186138=CARTESIAN_POINT('Ctrl Pts',(-15.7296155103452,-12.6703934014124,
117.398690748409)) ;
#186139=CARTESIAN_POINT('Ctrl Pts',(-15.655811659486,-12.6703933786195,
117.422921767436)) ;
#186140=CARTESIAN_POINT('Ctrl Pts',(-15.5820078086268,-12.6703933558266,
117.447152786463)) ;
#186141=CARTESIAN_POINT('Ctrl Pts',(-15.598067708066,-12.6146171715207,
117.496068649538)) ;
#186142=CARTESIAN_POINT('Ctrl Pts',(-15.6141276075051,-12.5588409872148,
117.544984512613)) ;
#186143=CARTESIAN_POINT('Ctrl Pts',(-15.6879314583643,-12.5588410100077,
117.520753493586)) ;
#186144=CARTESIAN_POINT('Ctrl Pts',(-15.7617353092235,-12.5588410328005,
117.496522474558)) ;
#186145=CARTESIAN_POINT('Ctrl Pts',(-15.7456754097843,-12.6146172171064,
117.447606611484)) ;
#186146=CARTESIAN_POINT('Ctrl Pts',(-15.6606952599714,-12.4490452703409,
117.224157743888)) ;
#186147=CARTESIAN_POINT('Ctrl Pts',(-15.6498132626341,-12.5164621248353,
117.191012935012)) ;
#186148=CARTESIAN_POINT('Ctrl Pts',(-15.5760094079726,-12.5164621055273,
117.215243942458)) ;
#186149=CARTESIAN_POINT('Ctrl Pts',(-15.5022055533111,-12.5164620862193,
117.239474949904)) ;
#186150=CARTESIAN_POINT('Ctrl Pts',(-15.5130875506483,-12.449045231725,
117.27261975878)) ;
#186151=CARTESIAN_POINT('Ctrl Pts',(-15.5239695479856,-12.3816283772306,
117.305764567655)) ;
#186152=CARTESIAN_POINT('Ctrl Pts',(-15.5977734026471,-12.3816283965386,
117.28153356021)) ;
#186153=CARTESIAN_POINT('Ctrl Pts',(-15.6715772573086,-12.3816284158465,
117.257302552764)) ;
#186154=CARTESIAN_POINT('Ctrl Pts',(-15.6606952599714,-12.4490452703409,
117.224157743888)) ;
#186155=CARTESIAN_POINT('Ctrl Pts',(-15.5642062371029,-12.3524023594542,
116.965836028037)) ;
#186156=CARTESIAN_POINT('Ctrl Pts',(-15.5593092972053,-12.4266644816829,
116.950920738249)) ;
#186157=CARTESIAN_POINT('Ctrl Pts',(-15.4855054383831,-12.4266644707959,
116.975151733023)) ;
#186158=CARTESIAN_POINT('Ctrl Pts',(-15.4117015795609,-12.4266644599088,
116.999382727796)) ;
#186159=CARTESIAN_POINT('Ctrl Pts',(-15.4165985194586,-12.3524023376801,
117.014298017584)) ;
#186160=CARTESIAN_POINT('Ctrl Pts',(-15.4214954593561,-12.2781402154514,
117.029213307372)) ;
#186161=CARTESIAN_POINT('Ctrl Pts',(-15.4952993181783,-12.2781402263384,
117.004982312599)) ;
#186162=CARTESIAN_POINT('Ctrl Pts',(-15.5691031770005,-12.2781402372254,
116.980751317825)) ;
#186163=CARTESIAN_POINT('Ctrl Pts',(-15.5642062371029,-12.3524023594542,
116.965836028037)) ;
#186164=CARTESIAN_POINT('Ctrl Pts',(-15.4635911617765,-12.3322917866331,
116.694660585488)) ;
#186165=CARTESIAN_POINT('Ctrl Pts',(-15.4649819187286,-12.4080647606153,
116.698896605655)) ;
#186166=CARTESIAN_POINT('Ctrl Pts',(-15.3911780574036,-12.4080647636104,
116.723127592805)) ;
#186167=CARTESIAN_POINT('Ctrl Pts',(-15.3173741960785,-12.4080647666054,
116.747358579955)) ;
#186168=CARTESIAN_POINT('Ctrl Pts',(-15.3159834391265,-12.3322917926232,
116.743122559788)) ;
#186169=CARTESIAN_POINT('Ctrl Pts',(-15.3145926821743,-12.256518818641,
116.73888653962)) ;
#186170=CARTESIAN_POINT('Ctrl Pts',(-15.3883965434994,-12.256518815646,
116.71465555247)) ;
#186171=CARTESIAN_POINT('Ctrl Pts',(-15.4622004048243,-12.2565188126509,
116.69042456532)) ;
#186172=CARTESIAN_POINT('Ctrl Pts',(-15.4635911617765,-12.3322917866331,
116.694660585488)) ;
#186173=CARTESIAN_POINT('Ctrl Pts',(-15.363777095621,-12.3899082998251,
116.426207229955)) ;
#186174=CARTESIAN_POINT('Ctrl Pts',(-15.3714027978846,-12.4617684939858,
116.449433887356)) ;
#186175=CARTESIAN_POINT('Ctrl Pts',(-15.2975989347207,-12.4617685151837,
116.473664868905)) ;
#186176=CARTESIAN_POINT('Ctrl Pts',(-15.2237950715568,-12.4617685363815,
116.497895850454)) ;
#186177=CARTESIAN_POINT('Ctrl Pts',(-15.2161693692933,-12.3899083422208,
116.474669193054)) ;
#186178=CARTESIAN_POINT('Ctrl Pts',(-15.2085436670297,-12.3180481480601,
116.451442535653)) ;
#186179=CARTESIAN_POINT('Ctrl Pts',(-15.2823475301936,-12.3180481268623,
116.427211554104)) ;
#186180=CARTESIAN_POINT('Ctrl Pts',(-15.3561513933575,-12.3180481056645,
116.402980572555)) ;
#186181=CARTESIAN_POINT('Ctrl Pts',(-15.363777095621,-12.3899082998251,
116.426207229955)) ;
#186182=CARTESIAN_POINT('Ctrl Pts',(-15.2724808702363,-12.5204817202917,
116.18346404372)) ;
#186183=CARTESIAN_POINT('Ctrl Pts',(-15.2857605963654,-12.5833292491025,
116.223911945411)) ;
#186184=CARTESIAN_POINT('Ctrl Pts',(-15.211956733883,-12.5833292901703,
116.248142929035)) ;
#186185=CARTESIAN_POINT('Ctrl Pts',(-15.1381528714006,-12.5833293312382,
116.27237391266)) ;
#186186=CARTESIAN_POINT('Ctrl Pts',(-15.1248731452714,-12.5204818024274,
116.231926010969)) ;
#186187=CARTESIAN_POINT('Ctrl Pts',(-15.1115934191423,-12.4576342736166,
116.191478109279)) ;
#186188=CARTESIAN_POINT('Ctrl Pts',(-15.1853972816247,-12.4576342325488,
116.167247125654)) ;
#186189=CARTESIAN_POINT('Ctrl Pts',(-15.2592011441071,-12.457634191481,
116.143016142029)) ;
#186190=CARTESIAN_POINT('Ctrl Pts',(-15.2724808702363,-12.5204817202917,
116.18346404372)) ;
#186191=CARTESIAN_POINT('Ctrl Pts',(-15.1942105603966,-12.7170079033734,
115.980733336847)) ;
#186192=CARTESIAN_POINT('Ctrl Pts',(-15.2122362128416,-12.7662262828423,
116.035636564168)) ;
#186193=CARTESIAN_POINT('Ctrl Pts',(-15.1384323526754,-12.7662263456653,
116.059867554848)) ;
#186194=CARTESIAN_POINT('Ctrl Pts',(-15.0646284925093,-12.7662264084883,
116.084098545527)) ;
#186195=CARTESIAN_POINT('Ctrl Pts',(-15.0466028400643,-12.7170080290195,
116.029195318206)) ;
#186196=CARTESIAN_POINT('Ctrl Pts',(-15.0285771876193,-12.6677896495507,
115.974292090885)) ;
#186197=CARTESIAN_POINT('Ctrl Pts',(-15.1023810477854,-12.6677895867277,
115.950061100206)) ;
#186198=CARTESIAN_POINT('Ctrl Pts',(-15.1761849079516,-12.6677895239046,
115.925830109526)) ;
#186199=CARTESIAN_POINT('Ctrl Pts',(-15.1942105603966,-12.7170079033734,
115.980733336847)) ;
#186200=CARTESIAN_POINT('Ctrl Pts',(-15.1352265619382,-12.9615280720901,
115.836366093429)) ;
#186201=CARTESIAN_POINT('Ctrl Pts',(-15.1566661866156,-12.9937459693296,
115.901667729225)) ;
#186202=CARTESIAN_POINT('Ctrl Pts',(-15.0828623315335,-12.9937460490588,
115.92589873539)) ;
#186203=CARTESIAN_POINT('Ctrl Pts',(-15.0090584764514,-12.9937461287879,
115.950129741554)) ;
#186204=CARTESIAN_POINT('Ctrl Pts',(-14.987618851774,-12.9615282315483,
115.884828105759)) ;
#186205=CARTESIAN_POINT('Ctrl Pts',(-14.9661792270966,-12.9293103343088,
115.819526469964)) ;
#186206=CARTESIAN_POINT('Ctrl Pts',(-15.0399830821787,-12.9293102545796,
115.795295463799)) ;
#186207=CARTESIAN_POINT('Ctrl Pts',(-15.1137869372607,-12.9293101748505,
115.771064457634)) ;
#186208=CARTESIAN_POINT('Ctrl Pts',(-15.1352265619382,-12.9615280720901,
115.836366093429)) ;
#186209=CARTESIAN_POINT('Ctrl Pts',(-15.0978086326599,-13.241668548695,
115.758096626062)) ;
#186210=CARTESIAN_POINT('Ctrl Pts',(-15.1211533914122,-13.2543754677215,
115.829200992715)) ;
#186211=CARTESIAN_POINT('Ctrl Pts',(-15.0473495430318,-13.2543755617733,
115.853432019292)) ;
#186212=CARTESIAN_POINT('Ctrl Pts',(-14.9735456946513,-13.2543756558251,
115.877663045869)) ;
#186213=CARTESIAN_POINT('Ctrl Pts',(-14.9502009358991,-13.2416687367986,
115.806558679216)) ;
#186214=CARTESIAN_POINT('Ctrl Pts',(-14.9268561771469,-13.228961817772,
115.735454312564)) ;
#186215=CARTESIAN_POINT('Ctrl Pts',(-15.0006600255273,-13.2289617237202,
115.711223285987)) ;
#186216=CARTESIAN_POINT('Ctrl Pts',(-15.0744638739077,-13.2289616296684,
115.68699225941)) ;
#186217=CARTESIAN_POINT('Ctrl Pts',(-15.0978086326599,-13.241668548695,
115.758096626062)) ;
#186218=CARTESIAN_POINT('Ctrl Pts',(-15.084760361114,-13.5312927388049,
115.753637119194)) ;
#186219=CARTESIAN_POINT('Ctrl Pts',(-15.1083199747751,-13.5237974675911,
115.825395899159)) ;
#186220=CARTESIAN_POINT('Ctrl Pts',(-15.0345161345071,-13.5237975662632,
115.849626950445)) ;
#186221=CARTESIAN_POINT('Ctrl Pts',(-14.9607122942391,-13.5237976649353,
115.873858001731)) ;
#186222=CARTESIAN_POINT('Ctrl Pts',(-14.9371526805781,-13.5312929361492,
115.802099221766)) ;
#186223=CARTESIAN_POINT('Ctrl Pts',(-14.913593066917,-13.538788207363,115.730340441801)) ;
#186224=CARTESIAN_POINT('Ctrl Pts',(-14.987396907185,-13.5387881086909,
115.706109390515)) ;
#186225=CARTESIAN_POINT('Ctrl Pts',(-15.061200747453,-13.5387880100187,
115.681878339228)) ;
#186226=CARTESIAN_POINT('Ctrl Pts',(-15.084760361114,-13.5312927388049,
115.753637119194)) ;
#186227=CARTESIAN_POINT('Ctrl Pts',(-15.0956720661844,-13.8141856043051,
115.822335205277)) ;
#186228=CARTESIAN_POINT('Ctrl Pts',(-15.1177705883915,-13.7869289146623,
115.889643736342)) ;
#186229=CARTESIAN_POINT('Ctrl Pts',(-15.0439667566183,-13.7869290108332,
115.913874813502)) ;
#186230=CARTESIAN_POINT('Ctrl Pts',(-14.9701629248451,-13.7869291070041,
115.938105890662)) ;
#186231=CARTESIAN_POINT('Ctrl Pts',(-14.9480644026381,-13.8141857966469,
115.870797359597)) ;
#186232=CARTESIAN_POINT('Ctrl Pts',(-14.925965880431,-13.8414424862897,
115.803488828531)) ;
#186233=CARTESIAN_POINT('Ctrl Pts',(-14.9997697122042,-13.8414423901188,
115.779257751371)) ;
#186234=CARTESIAN_POINT('Ctrl Pts',(-15.0735735439773,-13.8414422939479,
115.755026674211)) ;
#186235=CARTESIAN_POINT('Ctrl Pts',(-15.0956720661844,-13.8141856043051,
115.822335205277)) ;
#186236=CARTESIAN_POINT('Ctrl Pts',(-15.1292184993136,-14.0686273114668,
115.959949911345)) ;
#186237=CARTESIAN_POINT('Ctrl Pts',(-15.1482741234775,-14.0235664995227,
116.017990265886)) ;
#186238=CARTESIAN_POINT('Ctrl Pts',(-15.0744702998026,-14.0235665846011,
116.042221367712)) ;
#186239=CARTESIAN_POINT('Ctrl Pts',(-15.0006664761278,-14.0235666696795,
116.066452469538)) ;
#186240=CARTESIAN_POINT('Ctrl Pts',(-14.9816108519638,-14.0686274816236,
116.008412114997)) ;
#186241=CARTESIAN_POINT('Ctrl Pts',(-14.9625552277998,-14.1136882935678,
115.950371760456)) ;
#186242=CARTESIAN_POINT('Ctrl Pts',(-15.0363590514747,-14.1136882084894,
115.92614065863)) ;
#186243=CARTESIAN_POINT('Ctrl Pts',(-15.1101628751496,-14.113688123411,
115.901909556804)) ;
#186244=CARTESIAN_POINT('Ctrl Pts',(-15.1292184993136,-14.0686273114668,
115.959949911345)) ;
#186245=CARTESIAN_POINT('Ctrl Pts',(-15.1825001129318,-14.2772225776637,
116.157827602682)) ;
#186246=CARTESIAN_POINT('Ctrl Pts',(-15.1971276181691,-14.2175318931739,
116.202380621409)) ;
#186247=CARTESIAN_POINT('Ctrl Pts',(-15.1233238013441,-14.2175319594466,
116.226611744099)) ;
#186248=CARTESIAN_POINT('Ctrl Pts',(-15.0495199845191,-14.2175320257193,
116.250842866789)) ;
#186249=CARTESIAN_POINT('Ctrl Pts',(-15.0348924792818,-14.2772227102091,
116.206289848062)) ;
#186250=CARTESIAN_POINT('Ctrl Pts',(-15.0202649740445,-14.3369133946989,
116.161736829335)) ;
#186251=CARTESIAN_POINT('Ctrl Pts',(-15.0940687908695,-14.3369133284262,
116.137505706645)) ;
#186252=CARTESIAN_POINT('Ctrl Pts',(-15.1678726076945,-14.3369132621536,
116.113274583955)) ;
#186253=CARTESIAN_POINT('Ctrl Pts',(-15.1825001129318,-14.2772225776637,
116.157827602682)) ;
#186254=CARTESIAN_POINT('Ctrl Pts',(-15.2502956526181,-14.4229662306659,
116.399664973007)) ;
#186255=CARTESIAN_POINT('Ctrl Pts',(-15.2594801383945,-14.3530122150386,
116.427639432676)) ;
#186256=CARTESIAN_POINT('Ctrl Pts',(-15.1856763262186,-14.3530122565041,
116.451870569526)) ;
#186257=CARTESIAN_POINT('Ctrl Pts',(-15.1118725140427,-14.3530122979697,
116.476101706376)) ;
#186258=CARTESIAN_POINT('Ctrl Pts',(-15.1026880282663,-14.4229663135971,
116.448127246707)) ;
#186259=CARTESIAN_POINT('Ctrl Pts',(-15.0935035424898,-14.4929203292244,
116.420152787038)) ;
#186260=CARTESIAN_POINT('Ctrl Pts',(-15.1673073546657,-14.4929202877588,
116.395921650188)) ;
#186261=CARTESIAN_POINT('Ctrl Pts',(-15.2411111668416,-14.4929202462933,
116.371690513338)) ;
#186262=CARTESIAN_POINT('Ctrl Pts',(-15.2502956526181,-14.4229662306659,
116.399664973007)) ;
#186263=CARTESIAN_POINT('Ctrl Pts',(-15.3275171004924,-14.4976749709137,
116.670306720102)) ;
#186264=CARTESIAN_POINT('Ctrl Pts',(-15.3305906375755,-14.4224014624097,
116.679668216054)) ;
#186265=CARTESIAN_POINT('Ctrl Pts',(-15.2567868276272,-14.4224014756821,
116.70389935969)) ;
#186266=CARTESIAN_POINT('Ctrl Pts',(-15.182983017679,-14.4224014889544,
116.728130503325)) ;
#186267=CARTESIAN_POINT('Ctrl Pts',(-15.179909480596,-14.4976749974584,
116.718769007372)) ;
#186268=CARTESIAN_POINT('Ctrl Pts',(-15.176835943513,-14.5729485059623,
116.70940751142)) ;
#186269=CARTESIAN_POINT('Ctrl Pts',(-15.2506397534612,-14.57294849269,116.685176367784)) ;
#186270=CARTESIAN_POINT('Ctrl Pts',(-15.3244435634094,-14.5729484794176,
116.660945224149)) ;
#186271=CARTESIAN_POINT('Ctrl Pts',(-15.3275171004924,-14.4976749709137,
116.670306720102)) ;
#186272=CARTESIAN_POINT('Ctrl Pts',(-15.4083349615168,-14.4944851703305,
116.952154625279)) ;
#186273=CARTESIAN_POINT('Ctrl Pts',(-15.4050322512228,-14.4193216059584,
116.942095100569)) ;
#186274=CARTESIAN_POINT('Ctrl Pts',(-15.3312284404642,-14.4193215903829,
116.966326241736)) ;
#186275=CARTESIAN_POINT('Ctrl Pts',(-15.2574246297056,-14.4193215748074,
116.990557382903)) ;
#186276=CARTESIAN_POINT('Ctrl Pts',(-15.2607273399995,-14.4944851391795,
117.000616907613)) ;
#186277=CARTESIAN_POINT('Ctrl Pts',(-15.2640300502934,-14.5696487035515,
117.010676432323)) ;
#186278=CARTESIAN_POINT('Ctrl Pts',(-15.3378338610521,-14.5696487191271,
116.986445291156)) ;
#186279=CARTESIAN_POINT('Ctrl Pts',(-15.4116376718107,-14.5696487347026,
116.962214149989)) ;
#186280=CARTESIAN_POINT('Ctrl Pts',(-15.4083349615168,-14.4944851703305,
116.952154625279)) ;
#186281=CARTESIAN_POINT('Ctrl Pts',(-15.4846889044359,-14.4147277655596,
117.219968470872)) ;
#186282=CARTESIAN_POINT('Ctrl Pts',(-15.4753209992311,-14.3450211180556,
117.191435341122)) ;
#186283=CARTESIAN_POINT('Ctrl Pts',(-15.4015171853854,-14.3450210762549,
117.215666472886)) ;
#186284=CARTESIAN_POINT('Ctrl Pts',(-15.3277133715397,-14.3450210344541,
117.23989760465)) ;
#186285=CARTESIAN_POINT('Ctrl Pts',(-15.3370812767445,-14.4147276819581,
117.2684307344)) ;
#186286=CARTESIAN_POINT('Ctrl Pts',(-15.3464491819492,-14.4844343294621,
117.29696386415)) ;
#186287=CARTESIAN_POINT('Ctrl Pts',(-15.4202529957949,-14.4844343712628,
117.272732732386)) ;
#186288=CARTESIAN_POINT('Ctrl Pts',(-15.4940568096406,-14.4844344130636,
117.248501600622)) ;
#186289=CARTESIAN_POINT('Ctrl Pts',(-15.4846889044359,-14.4147277655596,
117.219968470872)) ;
#186290=CARTESIAN_POINT('Ctrl Pts',(-15.5519059399888,-14.2631098096402,
117.460240523406)) ;
#186291=CARTESIAN_POINT('Ctrl Pts',(-15.5370957241803,-14.2038841179929,
117.41513099375)) ;
#186292=CARTESIAN_POINT('Ctrl Pts',(-15.4632919047968,-14.2038840550099,
117.439362108647)) ;
#186293=CARTESIAN_POINT('Ctrl Pts',(-15.3894880854134,-14.203883992027,
117.463593223544)) ;
#186294=CARTESIAN_POINT('Ctrl Pts',(-15.4042983012219,-14.2631096836743,
117.5087027532)) ;
#186295=CARTESIAN_POINT('Ctrl Pts',(-15.4191085170304,-14.3223353753216,
117.553812282856)) ;
#186296=CARTESIAN_POINT('Ctrl Pts',(-15.4929123364138,-14.3223354383045,
117.529581167959)) ;
#186297=CARTESIAN_POINT('Ctrl Pts',(-15.5667161557973,-14.3223355012875,
117.505350053062)) ;
#186298=CARTESIAN_POINT('Ctrl Pts',(-15.5519059399888,-14.2631098096402,
117.460240523406)) ;
#186299=CARTESIAN_POINT('Ctrl Pts',(-15.6035818704614,-14.0515534840703,
117.653029803228)) ;
#186300=CARTESIAN_POINT('Ctrl Pts',(-15.5844092168002,-14.0070094522688,
117.594632991836)) ;
#186301=CARTESIAN_POINT('Ctrl Pts',(-15.5106053905118,-14.0070093747174,
117.618864085702)) ;
#186302=CARTESIAN_POINT('Ctrl Pts',(-15.4368015642234,-14.007009297166,
117.643095179568)) ;
#186303=CARTESIAN_POINT('Ctrl Pts',(-15.4559742178847,-14.0515533289676,
117.70149199096)) ;
#186304=CARTESIAN_POINT('Ctrl Pts',(-15.4751468715459,-14.0960973607691,
117.759888802352)) ;
#186305=CARTESIAN_POINT('Ctrl Pts',(-15.5489506978343,-14.0960974383204,
117.735657708486)) ;
#186306=CARTESIAN_POINT('Ctrl Pts',(-15.6227545241227,-14.0960975158718,
117.711426614621)) ;
#186307=CARTESIAN_POINT('Ctrl Pts',(-15.6035818704614,-14.0515534840703,
117.653029803228)) ;
#186308=CARTESIAN_POINT('Ctrl Pts',(-15.6356848695643,-13.793288943793,
117.786406026282)) ;
#186309=CARTESIAN_POINT('Ctrl Pts',(-15.6135053515169,-13.7667090894671,
117.718850791254)) ;
#186310=CARTESIAN_POINT('Ctrl Pts',(-15.539701517435,-13.7667090063188,
117.743081861382)) ;
#186311=CARTESIAN_POINT('Ctrl Pts',(-15.465897683353,-13.7667089231704,
117.76731293151)) ;
#186312=CARTESIAN_POINT('Ctrl Pts',(-15.4880772014003,-13.7932887774963,
117.834868166537)) ;
#186313=CARTESIAN_POINT('Ctrl Pts',(-15.5102567194477,-13.8198686318222,
117.902423401565)) ;
#186314=CARTESIAN_POINT('Ctrl Pts',(-15.5840605535297,-13.8198687149705,
117.878192331437)) ;
#186315=CARTESIAN_POINT('Ctrl Pts',(-15.6578643876116,-13.8198687981189,
117.853961261309)) ;
#186316=CARTESIAN_POINT('Ctrl Pts',(-15.6356848695643,-13.793288943793,
117.786406026282)) ;
#186317=CARTESIAN_POINT('Ctrl Pts',(-15.6447985101952,-13.5095097704303,
117.849560702245)) ;
#186318=CARTESIAN_POINT('Ctrl Pts',(-15.6212168570663,-13.5027030390007,
117.777734790113)) ;
#186319=CARTESIAN_POINT('Ctrl Pts',(-15.5474130156155,-13.5027029571053,
117.801965837796)) ;
#186320=CARTESIAN_POINT('Ctrl Pts',(-15.4736091741646,-13.50270287521,117.826196885479)) ;
#186321=CARTESIAN_POINT('Ctrl Pts',(-15.4971908272935,-13.5095096066396,
117.898022797612)) ;
#186322=CARTESIAN_POINT('Ctrl Pts',(-15.5207724804223,-13.5163163380692,
117.969848709744)) ;
#186323=CARTESIAN_POINT('Ctrl Pts',(-15.5945763218732,-13.5163164199646,
117.945617662061)) ;
#186324=CARTESIAN_POINT('Ctrl Pts',(-15.668380163324,-13.5163165018599,
117.921386614378)) ;
#186325=CARTESIAN_POINT('Ctrl Pts',(-15.6447985101952,-13.5095097704303,
117.849560702245)) ;
#186326=CARTESIAN_POINT('Ctrl Pts',(-15.6297417008337,-13.218674427129,
117.839172279436)) ;
#186327=CARTESIAN_POINT('Ctrl Pts',(-15.6064416512002,-13.2321633115492,
117.768204086257)) ;
#186328=CARTESIAN_POINT('Ctrl Pts',(-15.5326378033173,-13.2321632381837,
117.79243511435)) ;
#186329=CARTESIAN_POINT('Ctrl Pts',(-15.4588339554343,-13.2321631648182,
117.816666142442)) ;
#186330=CARTESIAN_POINT('Ctrl Pts',(-15.4821340050678,-13.2186742803981,
117.887634335621)) ;
#186331=CARTESIAN_POINT('Ctrl Pts',(-15.5054340547013,-13.2051853959779,
117.9586025288)) ;
#186332=CARTESIAN_POINT('Ctrl Pts',(-15.5792379025843,-13.2051854693434,
117.934371500708)) ;
#186333=CARTESIAN_POINT('Ctrl Pts',(-15.6530417504672,-13.2051855427089,
117.910140472615)) ;
#186334=CARTESIAN_POINT('Ctrl Pts',(-15.6297417008337,-13.218674427129,
117.839172279436)) ;
#186335=CARTESIAN_POINT('Ctrl Pts',(-15.5909058637976,-12.9425272619773,
117.756286254308)) ;
#186336=CARTESIAN_POINT('Ctrl Pts',(-15.5695495533161,-12.9753170489684,
117.691238377106)) ;
#186337=CARTESIAN_POINT('Ctrl Pts',(-15.4957457004882,-12.9753169887403,
117.715469390137)) ;
#186338=CARTESIAN_POINT('Ctrl Pts',(-15.4219418476603,-12.9753169285121,
117.739700403168)) ;
#186339=CARTESIAN_POINT('Ctrl Pts',(-15.4432981581418,-12.942527141521,
117.804748280369)) ;
#186340=CARTESIAN_POINT('Ctrl Pts',(-15.4646544686234,-12.9097373545299,
117.86979615757)) ;
#186341=CARTESIAN_POINT('Ctrl Pts',(-15.5384583214513,-12.9097374147581,
117.84556514454)) ;
#186342=CARTESIAN_POINT('Ctrl Pts',(-15.6122621742792,-12.9097374749862,
117.821334131509)) ;
#186343=CARTESIAN_POINT('Ctrl Pts',(-15.5909058637976,-12.9425272619773,
117.756286254308)) ;
#186344=CARTESIAN_POINT('Ctrl Pts',(-15.5297839260892,-12.6990701230285,
117.605746240807)) ;
#186345=CARTESIAN_POINT('Ctrl Pts',(-15.511925441269,-12.7489081846955,
117.55135217639)) ;
#186346=CARTESIAN_POINT('Ctrl Pts',(-15.438121585841,-12.748908142065,117.575583181502)) ;
#186347=CARTESIAN_POINT('Ctrl Pts',(-15.364317730413,-12.7489080994345,
117.599814186613)) ;
#186348=CARTESIAN_POINT('Ctrl Pts',(-15.3821762152333,-12.6990700377675,
117.65420825103)) ;
#186349=CARTESIAN_POINT('Ctrl Pts',(-15.4000347000535,-12.6492319761005,
117.708602315447)) ;
#186350=CARTESIAN_POINT('Ctrl Pts',(-15.4738385554815,-12.649232018731,
117.684371310335)) ;
#186351=CARTESIAN_POINT('Ctrl Pts',(-15.5476424109095,-12.6492320613615,
117.660140305224)) ;
#186352=CARTESIAN_POINT('Ctrl Pts',(-15.5297839260892,-12.6990701230285,
117.605746240807)) ;
#186353=CARTESIAN_POINT('Ctrl Pts',(-15.4511561549076,-12.5091750901202,
117.40151828196)) ;
#186354=CARTESIAN_POINT('Ctrl Pts',(-15.438030988428,-12.5723470280859,
117.361541141619)) ;
#186355=CARTESIAN_POINT('Ctrl Pts',(-15.3642271316641,-12.5723470007831,
117.385772142662)) ;
#186356=CARTESIAN_POINT('Ctrl Pts',(-15.2904232749002,-12.5723469734802,
117.410003143704)) ;
#186357=CARTESIAN_POINT('Ctrl Pts',(-15.3035484413797,-12.5091750355146,
117.449980284045)) ;
#186358=CARTESIAN_POINT('Ctrl Pts',(-15.3166736078593,-12.4460030975489,
117.489957424385)) ;
#186359=CARTESIAN_POINT('Ctrl Pts',(-15.3904774646233,-12.4460031248517,
117.465726423343)) ;
#186360=CARTESIAN_POINT('Ctrl Pts',(-15.4642813213872,-12.4460031521546,
117.441495422301)) ;
#186361=CARTESIAN_POINT('Ctrl Pts',(-15.4511561549076,-12.5091750901202,
117.40151828196)) ;
#186362=CARTESIAN_POINT('Ctrl Pts',(-15.3584459875218,-12.3826566850404,
117.154731104865)) ;
#186363=CARTESIAN_POINT('Ctrl Pts',(-15.3510375064598,-12.4547585599534,
117.132166066116)) ;
#186364=CARTESIAN_POINT('Ctrl Pts',(-15.2772336508438,-12.4547585482587,
117.156397070654)) ;
#186365=CARTESIAN_POINT('Ctrl Pts',(-15.2034297952278,-12.4547585365639,
117.180628075193)) ;
#186366=CARTESIAN_POINT('Ctrl Pts',(-15.2108382762898,-12.3826566616509,
117.203193113943)) ;
#186367=CARTESIAN_POINT('Ctrl Pts',(-15.2182467573518,-12.3105547867379,
117.225758152692)) ;
#186368=CARTESIAN_POINT('Ctrl Pts',(-15.2920506129678,-12.3105547984326,
117.201527148153)) ;
#186369=CARTESIAN_POINT('Ctrl Pts',(-15.3658544685838,-12.3105548101274,
117.177296143615)) ;
#186370=CARTESIAN_POINT('Ctrl Pts',(-15.3584459875218,-12.3826566850404,
117.154731104865)) ;
#186371=CARTESIAN_POINT('Ctrl Pts',(-15.2584754294207,-12.3310754563828,
116.885718823753)) ;
#186372=CARTESIAN_POINT('Ctrl Pts',(-15.2573017097217,-12.4068883304643,
116.882143862309)) ;
#186373=CARTESIAN_POINT('Ctrl Pts',(-15.1834978563234,-12.406888329813,
116.906374873603)) ;
#186374=CARTESIAN_POINT('Ctrl Pts',(-15.1096940029252,-12.4068883291616,
116.930605884896)) ;
#186375=CARTESIAN_POINT('Ctrl Pts',(-15.1108677226242,-12.3310754550801,
116.93418084634)) ;
#186376=CARTESIAN_POINT('Ctrl Pts',(-15.1120414423232,-12.2552625809986,
116.937755807783)) ;
#186377=CARTESIAN_POINT('Ctrl Pts',(-15.1858452957214,-12.25526258165,116.91352479649)) ;
#186378=CARTESIAN_POINT('Ctrl Pts',(-15.2596491491197,-12.2552625823013,
116.889293785196)) ;
#186379=CARTESIAN_POINT('Ctrl Pts',(-15.2584754294207,-12.3310754563828,
116.885718823753)) ;
#186380=CARTESIAN_POINT('Ctrl Pts',(-15.1575649005721,-12.357364074466,
116.613810250569)) ;
#186381=CARTESIAN_POINT('Ctrl Pts',(-15.1627017931781,-12.4314561765023,
116.629456396148)) ;
#186382=CARTESIAN_POINT('Ctrl Pts',(-15.0888979425083,-12.4314561824614,
116.653687415753)) ;
#186383=CARTESIAN_POINT('Ctrl Pts',(-15.0150940918386,-12.4314561884204,
116.677918435357)) ;
#186384=CARTESIAN_POINT('Ctrl Pts',(-15.0099571992326,-12.3573640863842,
116.662272289777)) ;
#186385=CARTESIAN_POINT('Ctrl Pts',(-15.0048203066266,-12.2832719843479,
116.646626144198)) ;
#186386=CARTESIAN_POINT('Ctrl Pts',(-15.0786241572964,-12.2832719783889,
116.622395124594)) ;
#186387=CARTESIAN_POINT('Ctrl Pts',(-15.1524280079661,-12.2832719724298,
116.59816410499)) ;
#186388=CARTESIAN_POINT('Ctrl Pts',(-15.1575649005721,-12.357364074466,
116.613810250569)) ;
#186389=CARTESIAN_POINT('Ctrl Pts',(-15.0622843285041,-12.4589530543375,
116.358945148846)) ;
#186390=CARTESIAN_POINT('Ctrl Pts',(-15.0733504108087,-12.5260636075349,
116.392650649706)) ;
#186391=CARTESIAN_POINT('Ctrl Pts',(-14.9995465627523,-12.5260636163209,
116.41688167727)) ;
#186392=CARTESIAN_POINT('Ctrl Pts',(-14.9257427146959,-12.5260636251069,
116.441112704835)) ;
#186393=CARTESIAN_POINT('Ctrl Pts',(-14.9146766323914,-12.4589530719095,
116.407407203975)) ;
#186394=CARTESIAN_POINT('Ctrl Pts',(-14.9036105500868,-12.3918425187121,
116.373701703115)) ;
#186395=CARTESIAN_POINT('Ctrl Pts',(-14.9774143981431,-12.3918425099261,
116.349470675551)) ;
#186396=CARTESIAN_POINT('Ctrl Pts',(-15.0512182461995,-12.3918425011401,
116.325239647987)) ;
#186397=CARTESIAN_POINT('Ctrl Pts',(-15.0622843285041,-12.4589530543375,
116.358945148846)) ;
#186398=CARTESIAN_POINT('Ctrl Pts',(-14.9777630331864,-12.6306888766498,
116.137164147509)) ;
#186399=CARTESIAN_POINT('Ctrl Pts',(-14.9940098346291,-12.6859095379068,
116.186649283117)) ;
#186400=CARTESIAN_POINT('Ctrl Pts',(-14.9202059893101,-12.6859095445597,
116.210880319019)) ;
#186401=CARTESIAN_POINT('Ctrl Pts',(-14.8464021439911,-12.6859095512127,
116.235111354921)) ;
#186402=CARTESIAN_POINT('Ctrl Pts',(-14.8301553425484,-12.6306888899557,
116.185626219312)) ;
#186403=CARTESIAN_POINT('Ctrl Pts',(-14.8139085411057,-12.5754682286988,
116.136141083704)) ;
#186404=CARTESIAN_POINT('Ctrl Pts',(-14.8877123864247,-12.5754682220458,
116.111910047802)) ;
#186405=CARTESIAN_POINT('Ctrl Pts',(-14.9615162317436,-12.5754682153929,
116.0876790119)) ;
#186406=CARTESIAN_POINT('Ctrl Pts',(-14.9777630331864,-12.6306888766498,
116.137164147509)) ;
#186407=CARTESIAN_POINT('Ctrl Pts',(-14.9108196105475,-12.8569331102211,
115.968557829525)) ;
#186408=CARTESIAN_POINT('Ctrl Pts',(-14.9310347417438,-12.8964388496988,
116.030129857362)) ;
#186409=CARTESIAN_POINT('Ctrl Pts',(-14.8572308977073,-12.8964388537721,
116.05436089717)) ;
#186410=CARTESIAN_POINT('Ctrl Pts',(-14.7834270536708,-12.8964388578454,
116.078591936978)) ;
#186411=CARTESIAN_POINT('Ctrl Pts',(-14.7632119224746,-12.8569331183677,
116.017019909141)) ;
#186412=CARTESIAN_POINT('Ctrl Pts',(-14.7429967912783,-12.81742737889,115.955447881304)) ;
#186413=CARTESIAN_POINT('Ctrl Pts',(-14.8168006353148,-12.8174273748167,
115.931216841496)) ;
#186414=CARTESIAN_POINT('Ctrl Pts',(-14.8906044793512,-12.8174273707434,
115.906985801688)) ;
#186415=CARTESIAN_POINT('Ctrl Pts',(-14.9108196105475,-12.8569331102211,
115.968557829525)) ;
#186416=CARTESIAN_POINT('Ctrl Pts',(-14.8642028462685,-13.124308622433,
115.862054279518)) ;
#186417=CARTESIAN_POINT('Ctrl Pts',(-14.8869691156441,-13.1452036324507,
115.931396662715)) ;
#186418=CARTESIAN_POINT('Ctrl Pts',(-14.8131652723611,-13.1452036323883,
115.955627704818)) ;
#186419=CARTESIAN_POINT('Ctrl Pts',(-14.739361429078,-13.1452036323259,
115.979858746921)) ;
#186420=CARTESIAN_POINT('Ctrl Pts',(-14.7165951597023,-13.1243086223082,
115.910516363724)) ;
#186421=CARTESIAN_POINT('Ctrl Pts',(-14.6938288903267,-13.1034136122904,
115.841173980526)) ;
#186422=CARTESIAN_POINT('Ctrl Pts',(-14.7676327336098,-13.1034136123528,
115.816942938423)) ;
#186423=CARTESIAN_POINT('Ctrl Pts',(-14.8414365768928,-13.1034136124152,
115.79271189632)) ;
#186424=CARTESIAN_POINT('Ctrl Pts',(-14.8642028462685,-13.124308622433,
115.862054279518)) ;
#186425=CARTESIAN_POINT('Ctrl Pts',(-14.8411123635601,-13.4140118065031,
115.82734739657)) ;
#186426=CARTESIAN_POINT('Ctrl Pts',(-14.8647879122609,-13.4147080729357,
115.899459297934)) ;
#186427=CARTESIAN_POINT('Ctrl Pts',(-14.7909840688978,-13.414708069978,
115.923690339793)) ;
#186428=CARTESIAN_POINT('Ctrl Pts',(-14.7171802255347,-13.4147080670203,
115.947921381652)) ;
#186429=CARTESIAN_POINT('Ctrl Pts',(-14.693504676834,-13.4140118005876,
115.875809480288)) ;
#186430=CARTESIAN_POINT('Ctrl Pts',(-14.6698291281333,-13.413315534155,
115.803697578925)) ;
#186431=CARTESIAN_POINT('Ctrl Pts',(-14.7436329714963,-13.4133155371127,
115.779466537066)) ;
#186432=CARTESIAN_POINT('Ctrl Pts',(-14.8174368148594,-13.4133155400704,
115.755235495206)) ;
#186433=CARTESIAN_POINT('Ctrl Pts',(-14.8411123635601,-13.4140118065031,
115.82734739657)) ;
#186434=CARTESIAN_POINT('Ctrl Pts',(-14.8423364229059,-13.700942777731,
115.866314358884)) ;
#186435=CARTESIAN_POINT('Ctrl Pts',(-14.8652321436292,-13.6816044417709,
115.936051030061)) ;
#186436=CARTESIAN_POINT('Ctrl Pts',(-14.791428299926,-13.6816044385339,
115.960282070884)) ;
#186437=CARTESIAN_POINT('Ctrl Pts',(-14.7176244562229,-13.6816044352969,
115.984513111707)) ;
#186438=CARTESIAN_POINT('Ctrl Pts',(-14.6947287354995,-13.700942771257,
115.91477644053)) ;
#186439=CARTESIAN_POINT('Ctrl Pts',(-14.6718330147762,-13.7202811072171,
115.845039769353)) ;
#186440=CARTESIAN_POINT('Ctrl Pts',(-14.7456368584794,-13.7202811104541,
115.82080872853)) ;
#186441=CARTESIAN_POINT('Ctrl Pts',(-14.8194407021826,-13.7202811136911,
115.796577687706)) ;
#186442=CARTESIAN_POINT('Ctrl Pts',(-14.8423364229059,-13.700942777731,
115.866314358884)) ;
#186443=CARTESIAN_POINT('Ctrl Pts',(-14.8671060908768,-13.9707477592159,
115.9774009813)) ;
#186444=CARTESIAN_POINT('Ctrl Pts',(-14.8875684376904,-13.9325402407103,
116.039725988136)) ;
#186445=CARTESIAN_POINT('Ctrl Pts',(-14.81376459397,-13.9325402395383,116.063957028906)) ;
#186446=CARTESIAN_POINT('Ctrl Pts',(-14.7399607502495,-13.9325402383663,
116.088188069677)) ;
#186447=CARTESIAN_POINT('Ctrl Pts',(-14.7194984034359,-13.9707477568719,
116.025863062841)) ;
#186448=CARTESIAN_POINT('Ctrl Pts',(-14.6990360566222,-14.0089552753775,
115.963538056005)) ;
#186449=CARTESIAN_POINT('Ctrl Pts',(-14.7728399003427,-14.0089552765495,
115.939307015234)) ;
#186450=CARTESIAN_POINT('Ctrl Pts',(-14.8466437440631,-14.0089552777215,
115.915075974463)) ;
#186451=CARTESIAN_POINT('Ctrl Pts',(-14.8671060908768,-13.9707477592159,
115.9774009813)) ;
#186452=CARTESIAN_POINT('Ctrl Pts',(-14.9128113608891,-14.199353333197,
116.152059746698)) ;
#186453=CARTESIAN_POINT('Ctrl Pts',(-14.9293786536738,-14.1451271098491,
116.202521047353)) ;
#186454=CARTESIAN_POINT('Ctrl Pts',(-14.8555748106877,-14.1451271117169,
116.226752090361)) ;
#186455=CARTESIAN_POINT('Ctrl Pts',(-14.7817709677015,-14.1451271135848,
116.250983133368)) ;
#186456=CARTESIAN_POINT('Ctrl Pts',(-14.7652036749168,-14.1993533369326,
116.200521832713)) ;
#186457=CARTESIAN_POINT('Ctrl Pts',(-14.7486363821321,-14.2535795602805,
116.150060532057)) ;
#186458=CARTESIAN_POINT('Ctrl Pts',(-14.8224402251183,-14.2535795584127,
116.12582948905)) ;
#186459=CARTESIAN_POINT('Ctrl Pts',(-14.8962440681044,-14.2535795565448,
116.101598446043)) ;
#186460=CARTESIAN_POINT('Ctrl Pts',(-14.9128113608891,-14.199353333197,
116.152059746698)) ;
#186461=CARTESIAN_POINT('Ctrl Pts',(-14.9753472996786,-14.3720888987135,
116.377975410379)) ;
#186462=CARTESIAN_POINT('Ctrl Pts',(-14.986838764229,-14.3057223139106,
116.412976557117)) ;
#186463=CARTESIAN_POINT('Ctrl Pts',(-14.9130349227356,-14.3057223178457,
116.437207604671)) ;
#186464=CARTESIAN_POINT('Ctrl Pts',(-14.8392310812422,-14.3057223217808,
116.461438652225)) ;
#186465=CARTESIAN_POINT('Ctrl Pts',(-14.8277396166918,-14.3720889065837,
116.426437505486)) ;
#186466=CARTESIAN_POINT('Ctrl Pts',(-14.8162481521414,-14.4384554913866,
116.391436358748)) ;
#186467=CARTESIAN_POINT('Ctrl Pts',(-14.8900519936348,-14.4384554874515,
116.367205311194)) ;
#186468=CARTESIAN_POINT('Ctrl Pts',(-14.9638558351282,-14.4384554835164,
116.34297426364)) ;
#186469=CARTESIAN_POINT('Ctrl Pts',(-14.9753472996786,-14.3720888987135,
116.377975410379)) ;
#186470=CARTESIAN_POINT('Ctrl Pts',(-15.0495832763769,-14.4765884160959,
116.639535491124)) ;
#186471=CARTESIAN_POINT('Ctrl Pts',(-15.0551744341217,-14.4028287794428,
116.656565255222)) ;
#186472=CARTESIAN_POINT('Ctrl Pts',(-14.9813705947848,-14.4028287831727,
116.680796309345)) ;
#186473=CARTESIAN_POINT('Ctrl Pts',(-14.907566755448,-14.4028287869026,
116.705027363467)) ;
#186474=CARTESIAN_POINT('Ctrl Pts',(-14.9019755977032,-14.4765884235558,
116.687997599369)) ;
#186475=CARTESIAN_POINT('Ctrl Pts',(-14.8963844399584,-14.5503480602089,
116.67096783527)) ;
#186476=CARTESIAN_POINT('Ctrl Pts',(-14.9701882792953,-14.550348056479,
116.646736781148)) ;
#186477=CARTESIAN_POINT('Ctrl Pts',(-15.0439921186321,-14.550348052749,
116.622505727025)) ;
#186478=CARTESIAN_POINT('Ctrl Pts',(-15.0495832763769,-14.4765884160959,
116.639535491124)) ;
#186479=CARTESIAN_POINT('Ctrl Pts',(-15.1294503292581,-14.5052820126098,
116.918258658341)) ;
#186480=CARTESIAN_POINT('Ctrl Pts',(-15.1287392558924,-14.4294119228674,
116.916092843196)) ;
#186481=CARTESIAN_POINT('Ctrl Pts',(-15.054935418997,-14.4294119227756,
116.940323904755)) ;
#186482=CARTESIAN_POINT('Ctrl Pts',(-14.9811315821015,-14.4294119226838,
116.964554966313)) ;
#186483=CARTESIAN_POINT('Ctrl Pts',(-14.9818426554672,-14.5052820124263,
116.966720781458)) ;
#186484=CARTESIAN_POINT('Ctrl Pts',(-14.9825537288328,-14.5811521021687,
116.968886596602)) ;
#186485=CARTESIAN_POINT('Ctrl Pts',(-15.0563575657283,-14.5811521022605,
116.944655535043)) ;
#186486=CARTESIAN_POINT('Ctrl Pts',(-15.1301614026238,-14.5811521023523,
116.920424473485)) ;
#186487=CARTESIAN_POINT('Ctrl Pts',(-15.1294503292581,-14.5052820126098,
116.918258658341)) ;
#186488=CARTESIAN_POINT('Ctrl Pts',(-15.2083554184061,-14.4562719682351,
117.194003127052)) ;
#186489=CARTESIAN_POINT('Ctrl Pts',(-15.2014012663886,-14.3837141408082,
117.172821901506)) ;
#186490=CARTESIAN_POINT('Ctrl Pts',(-15.1275974315029,-14.383714132999,
117.197052969186)) ;
#186491=CARTESIAN_POINT('Ctrl Pts',(-15.0537935966172,-14.3837141251898,
117.221284036866)) ;
#186492=CARTESIAN_POINT('Ctrl Pts',(-15.0607477486347,-14.4562719526167,
117.242465262412)) ;
#186493=CARTESIAN_POINT('Ctrl Pts',(-15.0677019006523,-14.5288297800436,
117.263646487958)) ;
#186494=CARTESIAN_POINT('Ctrl Pts',(-15.141505735538,-14.5288297878528,
117.239415420278)) ;
#186495=CARTESIAN_POINT('Ctrl Pts',(-15.2153095704236,-14.528829795662,
117.215184352598)) ;
#186496=CARTESIAN_POINT('Ctrl Pts',(-15.2083554184061,-14.4562719682351,
117.194003127052)) ;
#186497=CARTESIAN_POINT('Ctrl Pts',(-15.2801775082366,-14.3327513043896,
117.448257959663)) ;
#186498=CARTESIAN_POINT('Ctrl Pts',(-15.2674641035531,-14.2687127593662,
117.409534979579)) ;
#186499=CARTESIAN_POINT('Ctrl Pts',(-15.1936602700235,-14.2687127399002,
117.433766051389)) ;
#186500=CARTESIAN_POINT('Ctrl Pts',(-15.1198564364938,-14.2687127204341,
117.4579971232)) ;
#186501=CARTESIAN_POINT('Ctrl Pts',(-15.1325698411772,-14.3327512654575,
117.496720103284)) ;
#186502=CARTESIAN_POINT('Ctrl Pts',(-15.1452832458607,-14.3967898104809,
117.535443083367)) ;
#186503=CARTESIAN_POINT('Ctrl Pts',(-15.2190870793904,-14.3967898299469,
117.511212011557)) ;
#186504=CARTESIAN_POINT('Ctrl Pts',(-15.29289091292,-14.396789849413,117.486980939747)) ;
#186505=CARTESIAN_POINT('Ctrl Pts',(-15.2801775082366,-14.3327513043896,
117.448257959663)) ;
#186506=CARTESIAN_POINT('Ctrl Pts',(-15.3387805415736,-14.1436492001557,
117.662231074929)) ;
#186507=CARTESIAN_POINT('Ctrl Pts',(-15.321222983922,-14.0927211498799,
117.608753586334)) ;
#186508=CARTESIAN_POINT('Ctrl Pts',(-15.2474191502595,-14.0927211161122,
117.63298465774)) ;
#186509=CARTESIAN_POINT('Ctrl Pts',(-15.173615316597,-14.0927210823444,
117.657215729146)) ;
#186510=CARTESIAN_POINT('Ctrl Pts',(-15.1911728742487,-14.1436491326202,
117.71069321774)) ;
#186511=CARTESIAN_POINT('Ctrl Pts',(-15.2087304319003,-14.194577182896,
117.764170706335)) ;
#186512=CARTESIAN_POINT('Ctrl Pts',(-15.2825342655628,-14.1945772166637,
117.739939634929)) ;
#186513=CARTESIAN_POINT('Ctrl Pts',(-15.3563380992252,-14.1945772504315,
117.715708563523)) ;
#186514=CARTESIAN_POINT('Ctrl Pts',(-15.3387805415736,-14.1436492001557,
117.662231074929)) ;
#186515=CARTESIAN_POINT('Ctrl Pts',(-15.3792583067542,-13.9025966993027,
117.820992658252)) ;
#186516=CARTESIAN_POINT('Ctrl Pts',(-15.3581152443244,-13.8684250728151,
117.756594300452)) ;
#186517=CARTESIAN_POINT('Ctrl Pts',(-15.2843114087381,-13.8684250241037,
117.780825365998)) ;
#186518=CARTESIAN_POINT('Ctrl Pts',(-15.2105075731519,-13.8684249753923,
117.805056431544)) ;
#186519=CARTESIAN_POINT('Ctrl Pts',(-15.2316506355817,-13.9025966018799,
117.869454789344)) ;
#186520=CARTESIAN_POINT('Ctrl Pts',(-15.2527936980115,-13.9367682283676,
117.933853147143)) ;
#186521=CARTESIAN_POINT('Ctrl Pts',(-15.3265975335978,-13.936768277079,
117.909622081597)) ;
#186522=CARTESIAN_POINT('Ctrl Pts',(-15.400401369184,-13.9367683257904,
117.885391016051)) ;
#186523=CARTESIAN_POINT('Ctrl Pts',(-15.3792583067542,-13.9025966993027,
117.820992658252)) ;
#186524=CARTESIAN_POINT('Ctrl Pts',(-15.3979595900405,-13.6267191611602,
117.91343726374)) ;
#186525=CARTESIAN_POINT('Ctrl Pts',(-15.3747460243894,-13.6117593942212,
117.842732487035)) ;
#186526=CARTESIAN_POINT('Ctrl Pts',(-15.3009421849996,-13.6117593320571,
117.866963540996)) ;
#186527=CARTESIAN_POINT('Ctrl Pts',(-15.2271383456097,-13.6117592698929,
117.891194594957)) ;
#186528=CARTESIAN_POINT('Ctrl Pts',(-15.2503519112607,-13.6267190368318,
117.961899371662)) ;
#186529=CARTESIAN_POINT('Ctrl Pts',(-15.2735654769117,-13.6416788037708,
118.032604148367)) ;
#186530=CARTESIAN_POINT('Ctrl Pts',(-15.3473693163016,-13.641678865935,
118.008373094406)) ;
#186531=CARTESIAN_POINT('Ctrl Pts',(-15.4211731556915,-13.6416789280991,
117.984142040445)) ;
#186532=CARTESIAN_POINT('Ctrl Pts',(-15.3979595900405,-13.6267191611602,
117.91343726374)) ;
#186533=CARTESIAN_POINT('Ctrl Pts',(-15.3927825723995,-13.3360804435672,
117.933129443873)) ;
#186534=CARTESIAN_POINT('Ctrl Pts',(-15.3691631161479,-13.3413907563864,
117.861188389733)) ;
#186535=CARTESIAN_POINT('Ctrl Pts',(-15.2953592712623,-13.3413906849688,
117.885419426954)) ;
#186536=CARTESIAN_POINT('Ctrl Pts',(-15.2215554263766,-13.3413906135511,
117.909650464176)) ;
#186537=CARTESIAN_POINT('Ctrl Pts',(-15.2451748826282,-13.3360803007319,
117.981591518316)) ;
#186538=CARTESIAN_POINT('Ctrl Pts',(-15.2687943388797,-13.3307699879127,
118.053532572457)) ;
#186539=CARTESIAN_POINT('Ctrl Pts',(-15.3425981837654,-13.3307700593304,
118.029301535235)) ;
#186540=CARTESIAN_POINT('Ctrl Pts',(-15.416402028651,-13.330770130748,118.005070498014)) ;
#186541=CARTESIAN_POINT('Ctrl Pts',(-15.3927825723995,-13.3360804435672,
117.933129443873)) ;
#186542=CARTESIAN_POINT('Ctrl Pts',(-15.3633873922544,-13.0512189530207,
117.879062741303)) ;
#186543=CARTESIAN_POINT('Ctrl Pts',(-15.3410521280606,-13.076425168365,
117.811033128819)) ;
#186544=CARTESIAN_POINT('Ctrl Pts',(-15.2672482765079,-13.0764250935319,
117.835264145734)) ;
#186545=CARTESIAN_POINT('Ctrl Pts',(-15.1934444249552,-13.0764250186989,
117.859495162648)) ;
#186546=CARTESIAN_POINT('Ctrl Pts',(-15.215779689149,-13.0512188033546,
117.927524775132)) ;
#186547=CARTESIAN_POINT('Ctrl Pts',(-15.2381149533427,-13.0260125880103,
117.995554387616)) ;
#186548=CARTESIAN_POINT('Ctrl Pts',(-15.3119188048954,-13.0260126628434,
117.971323370702)) ;
#186549=CARTESIAN_POINT('Ctrl Pts',(-15.3857226564481,-13.0260127376764,
117.947092353787)) ;
#186550=CARTESIAN_POINT('Ctrl Pts',(-15.3633873922544,-13.0512189530207,
117.879062741303)) ;
#186551=CARTESIAN_POINT('Ctrl Pts',(-15.3109908652404,-12.7925464774136,
117.754972225267)) ;
#186552=CARTESIAN_POINT('Ctrl Pts',(-15.291546720893,-12.835849054134,117.695748497217)) ;
#186553=CARTESIAN_POINT('Ctrl Pts',(-15.2177428621128,-12.8358489831972,
117.719979492118)) ;
#186554=CARTESIAN_POINT('Ctrl Pts',(-15.1439390033326,-12.8358489122603,
117.744210487019)) ;
#186555=CARTESIAN_POINT('Ctrl Pts',(-15.16338314768,-12.7925463355399,117.803434215069)) ;
#186556=CARTESIAN_POINT('Ctrl Pts',(-15.1828272920273,-12.7492437588195,
117.86265794312)) ;
#186557=CARTESIAN_POINT('Ctrl Pts',(-15.2566311508075,-12.7492438297564,
117.838426948219)) ;
#186558=CARTESIAN_POINT('Ctrl Pts',(-15.3304350095877,-12.7492439006932,
117.814195953318)) ;
#186559=CARTESIAN_POINT('Ctrl Pts',(-15.3109908652404,-12.7925464774136,
117.754972225267)) ;
#186560=CARTESIAN_POINT('Ctrl Pts',(-15.2391823230942,-12.5795095572681,
117.571559510383)) ;
#186561=CARTESIAN_POINT('Ctrl Pts',(-15.2239929392201,-12.6377483614764,
117.525295096131)) ;
#186562=CARTESIAN_POINT('Ctrl Pts',(-15.1501890738939,-12.6377483026741,
117.549526071094)) ;
#186563=CARTESIAN_POINT('Ctrl Pts',(-15.0763852085677,-12.6377482438719,
117.573757046056)) ;
#186564=CARTESIAN_POINT('Ctrl Pts',(-15.0915745924417,-12.5795094396635,
117.620021460309)) ;
#186565=CARTESIAN_POINT('Ctrl Pts',(-15.1067639763158,-12.5212706354552,
117.666285874561)) ;
#186566=CARTESIAN_POINT('Ctrl Pts',(-15.180567841642,-12.5212706942575,
117.642054899598)) ;
#186567=CARTESIAN_POINT('Ctrl Pts',(-15.2543717069682,-12.5212707530598,
117.617823924636)) ;
#186568=CARTESIAN_POINT('Ctrl Pts',(-15.2391823230942,-12.5795095572681,
117.571559510383)) ;
#186569=CARTESIAN_POINT('Ctrl Pts',(-15.1507434986883,-12.4247175389401,
117.337961032472)) ;
#186570=CARTESIAN_POINT('Ctrl Pts',(-15.140965995546,-12.4938489762306,
117.308180333589)) ;
#186571=CARTESIAN_POINT('Ctrl Pts',(-15.067162124109,-12.4938489356481,
117.332411289939)) ;
#186572=CARTESIAN_POINT('Ctrl Pts',(-14.993358252672,-12.4938488950656,
117.356642246289)) ;
#186573=CARTESIAN_POINT('Ctrl Pts',(-15.0031357558144,-12.4247174577751,
117.386422945172)) ;
#186574=CARTESIAN_POINT('Ctrl Pts',(-15.0129132589567,-12.3555860204846,
117.416203644056)) ;
#186575=CARTESIAN_POINT('Ctrl Pts',(-15.0867171303937,-12.3555860610671,
117.391972687705)) ;
#186576=CARTESIAN_POINT('Ctrl Pts',(-15.1605210018307,-12.3555861016496,
117.367741731355)) ;
#186577=CARTESIAN_POINT('Ctrl Pts',(-15.1507434986883,-12.4247175389401,
117.337961032472)) ;
#186578=CARTESIAN_POINT('Ctrl Pts',(-15.0539963052002,-12.3430591277612,
117.078422578942)) ;
#186579=CARTESIAN_POINT('Ctrl Pts',(-15.050232182881,-12.417991968948,117.06695766774)) ;
#186580=CARTESIAN_POINT('Ctrl Pts',(-14.976428308272,-12.4179919531806,
117.091188614429)) ;
#186581=CARTESIAN_POINT('Ctrl Pts',(-14.902624433663,-12.4179919374132,
117.115419561118)) ;
#186582=CARTESIAN_POINT('Ctrl Pts',(-14.9063885559822,-12.3430590962263,
117.12688447232)) ;
#186583=CARTESIAN_POINT('Ctrl Pts',(-14.9101526783013,-12.2681262550395,
117.138349383522)) ;
#186584=CARTESIAN_POINT('Ctrl Pts',(-14.9839565529103,-12.2681262708069,
117.114118436833)) ;
#186585=CARTESIAN_POINT('Ctrl Pts',(-15.0577604275193,-12.2681262865743,
117.089887490144)) ;
#186586=CARTESIAN_POINT('Ctrl Pts',(-15.0539963052002,-12.3430591277612,
117.078422578942)) ;
#186587=CARTESIAN_POINT('Ctrl Pts',(-14.9522545120357,-12.3371678726539,
116.804152632931)) ;
#186588=CARTESIAN_POINT('Ctrl Pts',(-14.9548509777493,-12.4126223874774,
116.812061046522)) ;
#186589=CARTESIAN_POINT('Ctrl Pts',(-14.8810471017157,-12.4126223993309,
116.836291988872)) ;
#186590=CARTESIAN_POINT('Ctrl Pts',(-14.8072432256821,-12.4126224111843,
116.860522931222)) ;
#186591=CARTESIAN_POINT('Ctrl Pts',(-14.8046467599684,-12.3371678963608,
116.852614517631)) ;
#186592=CARTESIAN_POINT('Ctrl Pts',(-14.8020502942548,-12.2617133815373,
116.84470610404)) ;
#186593=CARTESIAN_POINT('Ctrl Pts',(-14.8758541702884,-12.2617133696838,
116.82047516169)) ;
#186594=CARTESIAN_POINT('Ctrl Pts',(-14.949658046322,-12.2617133578303,
116.79624421934)) ;
#186595=CARTESIAN_POINT('Ctrl Pts',(-14.9522545120357,-12.3371678726539,
116.804152632931)) ;
#186596=CARTESIAN_POINT('Ctrl Pts',(-14.8538527368102,-12.4090465693171,
116.539851551766)) ;
#186597=CARTESIAN_POINT('Ctrl Pts',(-14.8625902865125,-12.4795937186109,
116.566464716288)) ;
#186598=CARTESIAN_POINT('Ctrl Pts',(-14.7887864120648,-12.4795937586664,
116.590695663468)) ;
#186599=CARTESIAN_POINT('Ctrl Pts',(-14.7149825376171,-12.4795937987218,
116.614926610649)) ;
#186600=CARTESIAN_POINT('Ctrl Pts',(-14.7062449879148,-12.409046649428,
116.588313446127)) ;
#186601=CARTESIAN_POINT('Ctrl Pts',(-14.6975074382125,-12.3384995001342,
116.561700281605)) ;
#186602=CARTESIAN_POINT('Ctrl Pts',(-14.7713113126602,-12.3384994600787,
116.537469334425)) ;
#186603=CARTESIAN_POINT('Ctrl Pts',(-14.8451151871079,-12.3384994200233,
116.513238387244)) ;
#186604=CARTESIAN_POINT('Ctrl Pts',(-14.8538527368102,-12.4090465693171,
116.539851551766)) ;
#186605=CARTESIAN_POINT('Ctrl Pts',(-14.7642677691781,-12.5533759332391,
116.302515678383)) ;
#186606=CARTESIAN_POINT('Ctrl Pts',(-14.778537622709,-12.6139509456652,
116.345979347711)) ;
#186607=CARTESIAN_POINT('Ctrl Pts',(-14.7047337524295,-12.6139510114575,
116.370210307587)) ;
#186608=CARTESIAN_POINT('Ctrl Pts',(-14.63092988215,-12.6139510772497,116.394441267463)) ;
#186609=CARTESIAN_POINT('Ctrl Pts',(-14.616660028619,-12.5533760648236,
116.350977598135)) ;
#186610=CARTESIAN_POINT('Ctrl Pts',(-14.6023901750881,-12.4928010523974,
116.307513928807)) ;
#186611=CARTESIAN_POINT('Ctrl Pts',(-14.6761940453676,-12.4928009866052,
116.283282968931)) ;
#186612=CARTESIAN_POINT('Ctrl Pts',(-14.7499979156471,-12.4928009208129,
116.259052009055)) ;
#186613=CARTESIAN_POINT('Ctrl Pts',(-14.7642677691781,-12.5533759332391,
116.302515678383)) ;
#186614=CARTESIAN_POINT('Ctrl Pts',(-14.6896786909459,-12.75934674632,116.110760879403)) ;
#186615=CARTESIAN_POINT('Ctrl Pts',(-14.7084440858535,-12.8056312692346,
116.167917242415)) ;
#186616=CARTESIAN_POINT('Ctrl Pts',(-14.6346402220319,-12.8056313554312,
116.19214822196)) ;
#186617=CARTESIAN_POINT('Ctrl Pts',(-14.5608363582103,-12.8056314416279,
116.216379201506)) ;
#186618=CARTESIAN_POINT('Ctrl Pts',(-14.5420709633026,-12.7593469187134,
116.159222838494)) ;
#186619=CARTESIAN_POINT('Ctrl Pts',(-14.523305568395,-12.7130623957988,
116.102066475482)) ;
#186620=CARTESIAN_POINT('Ctrl Pts',(-14.5971094322166,-12.7130623096021,
116.077835495937)) ;
#186621=CARTESIAN_POINT('Ctrl Pts',(-14.6709132960383,-12.7130622234055,
116.053604516391)) ;
#186622=CARTESIAN_POINT('Ctrl Pts',(-14.6896786909459,-12.75934674632,116.110760879403)) ;
#186623=CARTESIAN_POINT('Ctrl Pts',(-14.6343789414248,-13.0122957598429,
115.977755201021)) ;
#186624=CARTESIAN_POINT('Ctrl Pts',(-14.6562999607946,-13.0409889610471,
116.044523087009)) ;
#186625=CARTESIAN_POINT('Ctrl Pts',(-14.5824961049884,-13.0409890604734,
116.068754090968)) ;
#186626=CARTESIAN_POINT('Ctrl Pts',(-14.5086922491823,-13.0409891598997,
116.092985094927)) ;
#186627=CARTESIAN_POINT('Ctrl Pts',(-14.4867712298125,-13.0122959586955,
116.02621720894)) ;
#186628=CARTESIAN_POINT('Ctrl Pts',(-14.4648502104427,-12.9836027574913,
115.959449322952)) ;
#186629=CARTESIAN_POINT('Ctrl Pts',(-14.5386540662488,-12.983602658065,
115.935218318993)) ;
#186630=CARTESIAN_POINT('Ctrl Pts',(-14.612457922055,-12.9836025586387,
115.910987315034)) ;
#186631=CARTESIAN_POINT('Ctrl Pts',(-14.6343789414248,-13.0122957598429,
115.977755201021)) ;
#186632=CARTESIAN_POINT('Ctrl Pts',(-14.6015670654935,-13.2947806869138,
115.913305234625)) ;
#186633=CARTESIAN_POINT('Ctrl Pts',(-14.6250772645124,-13.3037945330256,
115.984913505458)) ;
#186634=CARTESIAN_POINT('Ctrl Pts',(-14.5512734174972,-13.303794637043,
116.009144536193)) ;
#186635=CARTESIAN_POINT('Ctrl Pts',(-14.4774695704819,-13.3037947410603,
116.033375566928)) ;
#186636=CARTESIAN_POINT('Ctrl Pts',(-14.4539593714631,-13.2947808949484,
115.961767296095)) ;
#186637=CARTESIAN_POINT('Ctrl Pts',(-14.4304491724442,-13.2857670488366,
115.890159025263)) ;
#186638=CARTESIAN_POINT('Ctrl Pts',(-14.5042530194594,-13.2857669448193,
115.865927994528)) ;
#186639=CARTESIAN_POINT('Ctrl Pts',(-14.5780568664746,-13.2857668408019,
115.841696963793)) ;
#186640=CARTESIAN_POINT('Ctrl Pts',(-14.6015670654935,-13.2947806869138,
115.913305234625)) ;
#186641=CARTESIAN_POINT('Ctrl Pts',(-14.5929308331265,-13.5857642149866,
115.922448315919)) ;
#186642=CARTESIAN_POINT('Ctrl Pts',(-14.6163456531128,-13.5744758994453,
115.993766077673)) ;
#186643=CARTESIAN_POINT('Ctrl Pts',(-14.542541814698,-13.574475999467,116.017997134604)) ;
#186644=CARTESIAN_POINT('Ctrl Pts',(-14.4687379762832,-13.5744760994887,
116.042228191534)) ;
#186645=CARTESIAN_POINT('Ctrl Pts',(-14.4453231562969,-13.58576441503,115.970910429781)) ;
#186646=CARTESIAN_POINT('Ctrl Pts',(-14.4219083363105,-13.5970527305713,
115.899592668027)) ;
#186647=CARTESIAN_POINT('Ctrl Pts',(-14.4957121747253,-13.5970526305496,
115.875361611096)) ;
#186648=CARTESIAN_POINT('Ctrl Pts',(-14.5695160131401,-13.5970525305279,
115.851130554166)) ;
#186649=CARTESIAN_POINT('Ctrl Pts',(-14.5929308331265,-13.5857642149866,
115.922448315919)) ;
#186650=CARTESIAN_POINT('Ctrl Pts',(-14.6083539544559,-13.8655802602202,
116.00497775363)) ;
#186651=CARTESIAN_POINT('Ctrl Pts',(-14.6299915248511,-13.8347390280632,
116.070882299983)) ;
#186652=CARTESIAN_POINT('Ctrl Pts',(-14.5561876939648,-13.8347391156571,
116.095113379844)) ;
#186653=CARTESIAN_POINT('Ctrl Pts',(-14.4823838630785,-13.834739203251,
116.119344459705)) ;
#186654=CARTESIAN_POINT('Ctrl Pts',(-14.4607462926832,-13.865580435408,
116.053439913352)) ;
#186655=CARTESIAN_POINT('Ctrl Pts',(-14.439108722288,-13.8964216675651,
115.987535367)) ;
#186656=CARTESIAN_POINT('Ctrl Pts',(-14.5129125531743,-13.8964215799712,
115.963304287139)) ;
#186657=CARTESIAN_POINT('Ctrl Pts',(-14.5867163840606,-13.8964214923772,
115.939073207277)) ;
#186658=CARTESIAN_POINT('Ctrl Pts',(-14.6083539544559,-13.8655802602202,
116.00497775363)) ;
#186659=CARTESIAN_POINT('Ctrl Pts',(-14.6460817889764,-14.1129045177148,
116.155423205873)) ;
#186660=CARTESIAN_POINT('Ctrl Pts',(-14.6643826463311,-14.0647490921529,
116.211164662798)) ;
#186661=CARTESIAN_POINT('Ctrl Pts',(-14.5905788210321,-14.0647491613001,
116.235395759677)) ;
#186662=CARTESIAN_POINT('Ctrl Pts',(-14.516774995733,-14.0647492304473,
116.259626856556)) ;
#186663=CARTESIAN_POINT('Ctrl Pts',(-14.4984741383783,-14.1129046560093,
116.203885399631)) ;
#186664=CARTESIAN_POINT('Ctrl Pts',(-14.4801732810236,-14.1610600815713,
116.148143942706)) ;
#186665=CARTESIAN_POINT('Ctrl Pts',(-14.5539771063227,-14.161060012424,
116.123912845827)) ;
#186666=CARTESIAN_POINT('Ctrl Pts',(-14.6277809316217,-14.1610599432768,
116.099681748948)) ;
#186667=CARTESIAN_POINT('Ctrl Pts',(-14.6460817889764,-14.1129045177148,
116.155423205873)) ;
#186668=CARTESIAN_POINT('Ctrl Pts',(-14.7021022989247,-14.3092608415155,
116.361345320201)) ;
#186669=CARTESIAN_POINT('Ctrl Pts',(-14.7157890443858,-14.2473238052157,
116.403032936882)) ;
#186670=CARTESIAN_POINT('Ctrl Pts',(-14.6419852228446,-14.2473238535572,
116.427264045207)) ;
#186671=CARTESIAN_POINT('Ctrl Pts',(-14.5681814013034,-14.2473239018987,
116.451495153532)) ;
#186672=CARTESIAN_POINT('Ctrl Pts',(-14.5544946558422,-14.3092609381985,
116.409807536851)) ;
#186673=CARTESIAN_POINT('Ctrl Pts',(-14.5408079103811,-14.3711979744983,
116.368119920171)) ;
#186674=CARTESIAN_POINT('Ctrl Pts',(-14.6146117319223,-14.3711979261568,
116.343888811846)) ;
#186675=CARTESIAN_POINT('Ctrl Pts',(-14.6884155534635,-14.3711978778153,
116.319657703521)) ;
#186676=CARTESIAN_POINT('Ctrl Pts',(-14.7021022989247,-14.3092608415155,
116.361345320201)) ;
#186677=CARTESIAN_POINT('Ctrl Pts',(-14.7724489534844,-14.4430503329775,
116.611150402582)) ;
#186678=CARTESIAN_POINT('Ctrl Pts',(-14.7805094778502,-14.3716785302195,
116.635701457742)) ;
#186679=CARTESIAN_POINT('Ctrl Pts',(-14.7067056572874,-14.371678555561,
116.659932569047)) ;
#186680=CARTESIAN_POINT('Ctrl Pts',(-14.6329018367247,-14.3716785809024,
116.684163680352)) ;
#186681=CARTESIAN_POINT('Ctrl Pts',(-14.6248413123589,-14.4430503836605,
116.659612625192)) ;
#186682=CARTESIAN_POINT('Ctrl Pts',(-14.6167807879931,-14.5144221864185,
116.635061570032)) ;
#186683=CARTESIAN_POINT('Ctrl Pts',(-14.6905846085559,-14.5144221610771,
116.610830458727)) ;
#186684=CARTESIAN_POINT('Ctrl Pts',(-14.7643884291186,-14.5144221357356,
116.586599347422)) ;
#186685=CARTESIAN_POINT('Ctrl Pts',(-14.7724489534844,-14.4430503329775,
116.611150402582)) ;
#186686=CARTESIAN_POINT('Ctrl Pts',(-14.8505663309753,-14.5029681127336,
116.88443223403)) ;
#186687=CARTESIAN_POINT('Ctrl Pts',(-14.852453421253,-14.4273052047568,
116.890180005168)) ;
#186688=CARTESIAN_POINT('Ctrl Pts',(-14.778649599869,-14.427305209291,116.914411113971)) ;
#186689=CARTESIAN_POINT('Ctrl Pts',(-14.704845778485,-14.4273052138253,
116.938642222775)) ;
#186690=CARTESIAN_POINT('Ctrl Pts',(-14.7029586882074,-14.5029681218021,
116.932894451638)) ;
#186691=CARTESIAN_POINT('Ctrl Pts',(-14.7010715979297,-14.5786310297789,
116.927146680501)) ;
#186692=CARTESIAN_POINT('Ctrl Pts',(-14.7748754193137,-14.5786310252447,
116.902915571697)) ;
#186693=CARTESIAN_POINT('Ctrl Pts',(-14.8486792406976,-14.5786310207104,
116.878684462893)) ;
#186694=CARTESIAN_POINT('Ctrl Pts',(-14.8505663309753,-14.5029681127336,
116.88443223403)) ;
#186695=CARTESIAN_POINT('Ctrl Pts',(-14.9309079279403,-14.4854361051768,
117.164690654725)) ;
#186696=CARTESIAN_POINT('Ctrl Pts',(-14.9264527867039,-14.4108823854582,
117.151121012159)) ;
#186697=CARTESIAN_POINT('Ctrl Pts',(-14.8526489621555,-14.4108823726848,
117.175352111325)) ;
#186698=CARTESIAN_POINT('Ctrl Pts',(-14.7788451376072,-14.4108823599115,
117.199583210491)) ;
#186699=CARTESIAN_POINT('Ctrl Pts',(-14.7833002788435,-14.4854360796301,
117.213152853056)) ;
#186700=CARTESIAN_POINT('Ctrl Pts',(-14.7877554200799,-14.5599897993486,
117.226722495622)) ;
#186701=CARTESIAN_POINT('Ctrl Pts',(-14.8615592446283,-14.559989812122,
117.202491396456)) ;
#186702=CARTESIAN_POINT('Ctrl Pts',(-14.9353630691767,-14.5599898248954,
117.17826029729)) ;
#186703=CARTESIAN_POINT('Ctrl Pts',(-14.9309079279403,-14.4854361051768,
117.164690654725)) ;
#186704=CARTESIAN_POINT('Ctrl Pts',(-15.0063578899015,-14.3912934817558,
117.429961830675)) ;
#186705=CARTESIAN_POINT('Ctrl Pts',(-14.9958941718393,-14.3231998086573,
117.398091032744)) ;
#186706=CARTESIAN_POINT('Ctrl Pts',(-14.9220903431598,-14.323199784148,
117.422322119327)) ;
#186707=CARTESIAN_POINT('Ctrl Pts',(-14.8482865144804,-14.3231997596387,
117.44655320591)) ;
#186708=CARTESIAN_POINT('Ctrl Pts',(-14.8587502325426,-14.3912934327372,
117.478424003842)) ;
#186709=CARTESIAN_POINT('Ctrl Pts',(-14.8692139506049,-14.4593871058357,
117.510294801773)) ;
#186710=CARTESIAN_POINT('Ctrl Pts',(-14.9430177792843,-14.459387130345,
117.48606371519)) ;
#186711=CARTESIAN_POINT('Ctrl Pts',(-15.0168216079637,-14.4593871548543,
117.461832628607)) ;
#186712=CARTESIAN_POINT('Ctrl Pts',(-15.0063578899015,-14.3912934817558,
117.429961830675)) ;
#186713=CARTESIAN_POINT('Ctrl Pts',(-15.0709894180942,-14.2271892392871,
117.662327292392)) ;
#186714=CARTESIAN_POINT('Ctrl Pts',(-15.0552623334199,-14.1704502048887,
117.614425129178)) ;
#186715=CARTESIAN_POINT('Ctrl Pts',(-14.9814585000848,-14.1704501748707,
117.638656201581)) ;
#186716=CARTESIAN_POINT('Ctrl Pts',(-14.9076546667496,-14.1704501448526,
117.662887273983)) ;
#186717=CARTESIAN_POINT('Ctrl Pts',(-14.923381751424,-14.227189179251,117.710789437197)) ;
#186718=CARTESIAN_POINT('Ctrl Pts',(-14.9391088360983,-14.2839282136493,
117.758691600411)) ;
#186719=CARTESIAN_POINT('Ctrl Pts',(-15.0129126694335,-14.2839282436673,
117.734460528009)) ;
#186720=CARTESIAN_POINT('Ctrl Pts',(-15.0867165027686,-14.2839282736854,
117.710229455606)) ;
#186721=CARTESIAN_POINT('Ctrl Pts',(-15.0709894180942,-14.2271892392871,
117.662327292392)) ;
#186722=CARTESIAN_POINT('Ctrl Pts',(-15.1191773884386,-14.0061849375035,
117.844439920784)) ;
#186723=CARTESIAN_POINT('Ctrl Pts',(-15.0993306388851,-13.9647911087946,
117.783989923197)) ;
#186724=CARTESIAN_POINT('Ctrl Pts',(-15.0255268014512,-13.9647910776001,
117.808220983116)) ;
#186725=CARTESIAN_POINT('Ctrl Pts',(-14.9517229640173,-13.9647910464057,
117.832452043034)) ;
#186726=CARTESIAN_POINT('Ctrl Pts',(-14.9715697135709,-14.0061848751146,
117.892902040621)) ;
#186727=CARTESIAN_POINT('Ctrl Pts',(-14.9914164631244,-14.0475787038235,
117.953352038208)) ;
#186728=CARTESIAN_POINT('Ctrl Pts',(-15.0652203005583,-14.047578735018,
117.929120978289)) ;
#186729=CARTESIAN_POINT('Ctrl Pts',(-15.1390241379922,-14.0475787662124,
117.904889918371)) ;
#186730=CARTESIAN_POINT('Ctrl Pts',(-15.1191773884386,-14.0061849375035,
117.844439920784)) ;
#186731=CARTESIAN_POINT('Ctrl Pts',(-15.147137619444,-13.7418695803109,
117.965135185314)) ;
#186732=CARTESIAN_POINT('Ctrl Pts',(-15.1245731450587,-13.7188682914606,
117.896407436568)) ;
#186733=CARTESIAN_POINT('Ctrl Pts',(-15.0507693039846,-13.7188682649132,
117.920638485399)) ;
#186734=CARTESIAN_POINT('Ctrl Pts',(-14.9769654629104,-13.7188682383657,
117.94486953423)) ;
#186735=CARTESIAN_POINT('Ctrl Pts',(-14.9995299372958,-13.741869527216,
118.013597282976)) ;
#186736=CARTESIAN_POINT('Ctrl Pts',(-15.022094411681,-13.7648708160662,
118.082325031721)) ;
#186737=CARTESIAN_POINT('Ctrl Pts',(-15.0958982527552,-13.7648708426137,
118.05809398289)) ;
#186738=CARTESIAN_POINT('Ctrl Pts',(-15.1697020938293,-13.7648708691611,
118.033862934059)) ;
#186739=CARTESIAN_POINT('Ctrl Pts',(-15.147137619444,-13.7418695803109,
117.965135185314)) ;
#186740=CARTESIAN_POINT('Ctrl Pts',(-15.1518624783003,-13.4550293844737,
118.014955235042)) ;
#186741=CARTESIAN_POINT('Ctrl Pts',(-15.1282007920477,-13.4520215652615,
117.942885556132)) ;
#186742=CARTESIAN_POINT('Ctrl Pts',(-15.0543969486045,-13.4520215454244,
117.967116597747)) ;
#186743=CARTESIAN_POINT('Ctrl Pts',(-14.9805931051612,-13.4520215255873,
117.991347639362)) ;
#186744=CARTESIAN_POINT('Ctrl Pts',(-15.0042547914137,-13.4550293447994,
118.063417318272)) ;
#186745=CARTESIAN_POINT('Ctrl Pts',(-15.0279164776663,-13.4580371640116,
118.135486997181)) ;
#186746=CARTESIAN_POINT('Ctrl Pts',(-15.1017203211096,-13.4580371838487,
118.111255955567)) ;
#186747=CARTESIAN_POINT('Ctrl Pts',(-15.1755241645529,-13.4580372036859,
118.087024913952)) ;
#186748=CARTESIAN_POINT('Ctrl Pts',(-15.1518624783003,-13.4550293844737,
118.014955235042)) ;
#186749=CARTESIAN_POINT('Ctrl Pts',(-15.1320243079306,-13.1635845721582,
117.990218757168)) ;
#186750=CARTESIAN_POINT('Ctrl Pts',(-15.1089733666003,-13.180922781359,
117.920009308918)) ;
#186751=CARTESIAN_POINT('Ctrl Pts',(-15.0351695222069,-13.1809227707576,
117.944240347639)) ;
#186752=CARTESIAN_POINT('Ctrl Pts',(-14.9613656778135,-13.1809227601562,
117.96847138636)) ;
#186753=CARTESIAN_POINT('Ctrl Pts',(-14.9844166191439,-13.1635845509553,
118.03868083461)) ;
#186754=CARTESIAN_POINT('Ctrl Pts',(-15.0074675604742,-13.1462463417545,
118.10889028286)) ;
#186755=CARTESIAN_POINT('Ctrl Pts',(-15.0812714048676,-13.1462463523559,
118.084659244139)) ;
#186756=CARTESIAN_POINT('Ctrl Pts',(-15.155075249261,-13.1462463629573,
118.060428205418)) ;
#186757=CARTESIAN_POINT('Ctrl Pts',(-15.1320243079306,-13.1635845721582,
117.990218757168)) ;
#186758=CARTESIAN_POINT('Ctrl Pts',(-15.0890308858548,-12.8938493439813,
117.894483238794)) ;
#186759=CARTESIAN_POINT('Ctrl Pts',(-15.0682186826188,-12.9300476003649,
117.831092625647)) ;
#186760=CARTESIAN_POINT('Ctrl Pts',(-14.9944148381014,-12.9300475948517,
117.85532366399)) ;
#186761=CARTESIAN_POINT('Ctrl Pts',(-14.9206109935841,-12.9300475893384,
117.879554702334)) ;
#186762=CARTESIAN_POINT('Ctrl Pts',(-14.9414231968201,-12.8938493329547,
117.942945315481)) ;
#186763=CARTESIAN_POINT('Ctrl Pts',(-14.962235400056,-12.857651076571,118.006335928628)) ;
#186764=CARTESIAN_POINT('Ctrl Pts',(-15.0360392445734,-12.8576510820843,
117.982104890284)) ;
#186765=CARTESIAN_POINT('Ctrl Pts',(-15.1098430890907,-12.8576510875976,
117.957873851941)) ;
#186766=CARTESIAN_POINT('Ctrl Pts',(-15.0890308858548,-12.8938493439813,
117.894483238794)) ;
#186767=CARTESIAN_POINT('Ctrl Pts',(-15.0240348200628,-12.658475902558,
117.732210088055)) ;
#186768=CARTESIAN_POINT('Ctrl Pts',(-15.006991084424,-12.7111646806542,
117.680297619284)) ;
#186769=CARTESIAN_POINT('Ctrl Pts',(-14.9331872407942,-12.7111646805121,
117.704528660331)) ;
#186770=CARTESIAN_POINT('Ctrl Pts',(-14.8593833971644,-12.7111646803699,
117.728759701378)) ;
#186771=CARTESIAN_POINT('Ctrl Pts',(-14.8764271328032,-12.6584759022737,
117.780672170148)) ;
#186772=CARTESIAN_POINT('Ctrl Pts',(-14.8934708684419,-12.6057871241775,
117.832584638919)) ;
#186773=CARTESIAN_POINT('Ctrl Pts',(-14.9672747120717,-12.6057871243196,
117.808353597872)) ;
#186774=CARTESIAN_POINT('Ctrl Pts',(-15.0410785557015,-12.6057871244618,
117.784122556825)) ;
#186775=CARTESIAN_POINT('Ctrl Pts',(-15.0240348200628,-12.658475902558,
117.732210088055)) ;
#186776=CARTESIAN_POINT('Ctrl Pts',(-14.9426437722386,-12.480124052921,
117.519499741541)) ;
#186777=CARTESIAN_POINT('Ctrl Pts',(-14.930529597909,-12.545344547809,117.482601921182)) ;
#186778=CARTESIAN_POINT('Ctrl Pts',(-14.8567257549558,-12.5453445488469,
117.506832964289)) ;
#186779=CARTESIAN_POINT('Ctrl Pts',(-14.7829219120025,-12.5453445498848,
117.531064007397)) ;
#186780=CARTESIAN_POINT('Ctrl Pts',(-14.7950360863321,-12.4801240549968,
117.567961827756)) ;
#186781=CARTESIAN_POINT('Ctrl Pts',(-14.8071502606617,-12.4149035601088,
117.604859648115)) ;
#186782=CARTESIAN_POINT('Ctrl Pts',(-14.8809541036149,-12.414903559071,
117.580628605007)) ;
#186783=CARTESIAN_POINT('Ctrl Pts',(-14.9547579465681,-12.4149035580331,
117.556397561899)) ;
#186784=CARTESIAN_POINT('Ctrl Pts',(-14.9426437722386,-12.480124052921,
117.519499741541)) ;
#186785=CARTESIAN_POINT('Ctrl Pts',(-14.8475793344936,-12.366810202119,
117.265710821588)) ;
#186786=CARTESIAN_POINT('Ctrl Pts',(-14.8413454317599,-12.4400414291151,
117.246723359765)) ;
#186787=CARTESIAN_POINT('Ctrl Pts',(-14.7675415893947,-12.4400414300861,
117.270954404664)) ;
#186788=CARTESIAN_POINT('Ctrl Pts',(-14.6937377470295,-12.4400414310572,
117.295185449562)) ;
#186789=CARTESIAN_POINT('Ctrl Pts',(-14.6999716497632,-12.3668102040611,
117.314172911385)) ;
#186790=CARTESIAN_POINT('Ctrl Pts',(-14.7062055524968,-12.2935789770651,
117.333160373209)) ;
#186791=CARTESIAN_POINT('Ctrl Pts',(-14.780009394862,-12.293578976094,117.30892932831)) ;
#186792=CARTESIAN_POINT('Ctrl Pts',(-14.8538132372272,-12.293578975123,
117.284698283411)) ;
#186793=CARTESIAN_POINT('Ctrl Pts',(-14.8475793344936,-12.366810202119,
117.265710821588)) ;
#186794=CARTESIAN_POINT('Ctrl Pts',(-14.7476028807063,-12.3300613553443,
116.996429637178)) ;
#186795=CARTESIAN_POINT('Ctrl Pts',(-14.7476117897904,-12.4059660659724,
116.99645677286)) ;
#186796=CARTESIAN_POINT('Ctrl Pts',(-14.6738079471839,-12.4059660657075,
117.020687817024)) ;
#186797=CARTESIAN_POINT('Ctrl Pts',(-14.6000041045774,-12.4059660654426,
117.044918861187)) ;
#186798=CARTESIAN_POINT('Ctrl Pts',(-14.5999951954933,-12.3300613548144,
117.044891725505)) ;
#186799=CARTESIAN_POINT('Ctrl Pts',(-14.5999862864092,-12.2541566441862,
117.044864589822)) ;
#186800=CARTESIAN_POINT('Ctrl Pts',(-14.6737901290157,-12.2541566444512,
117.020633545659)) ;
#186801=CARTESIAN_POINT('Ctrl Pts',(-14.7475939716222,-12.2541566447161,
116.996402501495)) ;
#186802=CARTESIAN_POINT('Ctrl Pts',(-14.7476028807063,-12.3300613553443,
116.996429637178)) ;
#186803=CARTESIAN_POINT('Ctrl Pts',(-14.6466367120282,-12.3711193571588,
116.724562625234)) ;
#186804=CARTESIAN_POINT('Ctrl Pts',(-14.6529580061683,-12.4442691147832,
116.743816267228)) ;
#186805=CARTESIAN_POINT('Ctrl Pts',(-14.5791541624313,-12.4442691147866,
116.768047307948)) ;
#186806=CARTESIAN_POINT('Ctrl Pts',(-14.5053503186943,-12.44426911479,116.792278348668)) ;
#186807=CARTESIAN_POINT('Ctrl Pts',(-14.4990290245542,-12.3711193571657,
116.773024706675)) ;
#186808=CARTESIAN_POINT('Ctrl Pts',(-14.4927077304141,-12.2979695995413,
116.753771064681)) ;
#186809=CARTESIAN_POINT('Ctrl Pts',(-14.5665115741511,-12.2979695995379,
116.72954002396)) ;
#186810=CARTESIAN_POINT('Ctrl Pts',(-14.6403154178881,-12.2979695995345,
116.70530898324)) ;
#186811=CARTESIAN_POINT('Ctrl Pts',(-14.6466367120282,-12.3711193571588,
116.724562625234)) ;
#186812=CARTESIAN_POINT('Ctrl Pts',(-14.5534726344851,-12.4860834955726,
116.475997560767)) ;
#186813=CARTESIAN_POINT('Ctrl Pts',(-14.5655797908285,-12.5513121633835,
116.512874005424)) ;
#186814=CARTESIAN_POINT('Ctrl Pts',(-14.4917759461966,-12.5513121652031,
116.537105043419)) ;
#186815=CARTESIAN_POINT('Ctrl Pts',(-14.4179721015648,-12.5513121670227,
116.561336081413)) ;
#186816=CARTESIAN_POINT('Ctrl Pts',(-14.4058649452214,-12.4860834992117,
116.524459636757)) ;
#186817=CARTESIAN_POINT('Ctrl Pts',(-14.393757788878,-12.4208548314008,
116.4875831921)) ;
#186818=CARTESIAN_POINT('Ctrl Pts',(-14.4675616335099,-12.4208548295812,
116.463352154105)) ;
#186819=CARTESIAN_POINT('Ctrl Pts',(-14.5413654781417,-12.4208548277616,
116.439121116111)) ;
#186820=CARTESIAN_POINT('Ctrl Pts',(-14.5534726344851,-12.4860834955726,
116.475997560767)) ;
#186821=CARTESIAN_POINT('Ctrl Pts',(-14.4716712825806,-12.6694591781323,
116.26251906764)) ;
#186822=CARTESIAN_POINT('Ctrl Pts',(-14.488769754576,-12.7219791159764,
116.314598254288)) ;
#186823=CARTESIAN_POINT('Ctrl Pts',(-14.4149659085601,-12.7219791238396,
116.338829288067)) ;
#186824=CARTESIAN_POINT('Ctrl Pts',(-14.3411620625442,-12.7219791317028,
116.363060321847)) ;
#186825=CARTESIAN_POINT('Ctrl Pts',(-14.3240635905488,-12.6694591938587,
116.310981135199)) ;
#186826=CARTESIAN_POINT('Ctrl Pts',(-14.3069651185534,-12.6169392560146,
116.258901948551)) ;
#186827=CARTESIAN_POINT('Ctrl Pts',(-14.3807689645693,-12.6169392481514,
116.234670914771)) ;
#186828=CARTESIAN_POINT('Ctrl Pts',(-14.4545728105852,-12.6169392402883,
116.210439880992)) ;
#186829=CARTESIAN_POINT('Ctrl Pts',(-14.4716712825806,-12.6694591781323,
116.26251906764)) ;
#186830=CARTESIAN_POINT('Ctrl Pts',(-14.4081656716587,-12.9054683696908,
116.104505284909)) ;
#186831=CARTESIAN_POINT('Ctrl Pts',(-14.4289902353886,-12.9415855764778,
116.167933545647)) ;
#186832=CARTESIAN_POINT('Ctrl Pts',(-14.3551863891245,-12.9415855922766,
116.19216457867)) ;
#186833=CARTESIAN_POINT('Ctrl Pts',(-14.2813825428604,-12.9415856080754,
116.216395611693)) ;
#186834=CARTESIAN_POINT('Ctrl Pts',(-14.2605579791305,-12.9054684012884,
116.152967350955)) ;
#186835=CARTESIAN_POINT('Ctrl Pts',(-14.2397334154006,-12.8693511945013,
116.089539090218)) ;
#186836=CARTESIAN_POINT('Ctrl Pts',(-14.3135372616647,-12.8693511787026,
116.065308057194)) ;
#186837=CARTESIAN_POINT('Ctrl Pts',(-14.3873411079288,-12.8693511629038,
116.041077024171)) ;
#186838=CARTESIAN_POINT('Ctrl Pts',(-14.4081656716587,-12.9054683696908,
116.104505284909)) ;
#186839=CARTESIAN_POINT('Ctrl Pts',(-14.3659620806529,-13.1783417993353,
116.011426957597)) ;
#186840=CARTESIAN_POINT('Ctrl Pts',(-14.389029628698,-13.1954587831432,
116.081686986504)) ;
#186841=CARTESIAN_POINT('Ctrl Pts',(-14.3152257832912,-13.1954588083928,
116.105918022139)) ;
#186842=CARTESIAN_POINT('Ctrl Pts',(-14.2414219378845,-13.1954588336424,
116.130149057773)) ;
#186843=CARTESIAN_POINT('Ctrl Pts',(-14.2183543898394,-13.1783418498345,
116.059889028866)) ;
#186844=CARTESIAN_POINT('Ctrl Pts',(-14.1952868417943,-13.1612248660266,
115.98962899996)) ;
#186845=CARTESIAN_POINT('Ctrl Pts',(-14.269090687201,-13.161224840777,115.965397964325)) ;
#186846=CARTESIAN_POINT('Ctrl Pts',(-14.3428945326078,-13.1612248155274,
115.941166928691)) ;
#186847=CARTESIAN_POINT('Ctrl Pts',(-14.3659620806529,-13.1783417993353,
116.011426957597)) ;
#186848=CARTESIAN_POINT('Ctrl Pts',(-14.3475114543578,-13.4677014527882,
115.990609557701)) ;
#186849=CARTESIAN_POINT('Ctrl Pts',(-14.3711684091168,-13.4646398279822,
116.062664824212)) ;
#186850=CARTESIAN_POINT('Ctrl Pts',(-14.2973645659806,-13.4646398615466,
116.086895866763)) ;
#186851=CARTESIAN_POINT('Ctrl Pts',(-14.2235607228445,-13.464639895111,
116.111126909313)) ;
#186852=CARTESIAN_POINT('Ctrl Pts',(-14.1999037680856,-13.4677015199171,
116.039071642802)) ;
#186853=CARTESIAN_POINT('Ctrl Pts',(-14.1762468133266,-13.4707631447231,
115.967016376291)) ;
#186854=CARTESIAN_POINT('Ctrl Pts',(-14.2500506564628,-13.4707631111587,
115.94278533374)) ;
#186855=CARTESIAN_POINT('Ctrl Pts',(-14.3238544995989,-13.4707630775943,
115.91855429119)) ;
#186856=CARTESIAN_POINT('Ctrl Pts',(-14.3475114543578,-13.4677014527882,
115.990609557701)) ;
#186857=CARTESIAN_POINT('Ctrl Pts',(-14.3531957687261,-13.7542094632266,
116.043383175808)) ;
#186858=CARTESIAN_POINT('Ctrl Pts',(-14.3757562745192,-13.7311394476093,
116.112098835515)) ;
#186859=CARTESIAN_POINT('Ctrl Pts',(-14.3019524349061,-13.7311394879972,
116.136329888796)) ;
#186860=CARTESIAN_POINT('Ctrl Pts',(-14.2281485952931,-13.7311395283851,
116.160560942077)) ;
#186861=CARTESIAN_POINT('Ctrl Pts',(-14.2055880895,-13.7542095440024,116.09184528237)) ;
#186862=CARTESIAN_POINT('Ctrl Pts',(-14.1830275837069,-13.7772795596197,
116.023129622664)) ;
#186863=CARTESIAN_POINT('Ctrl Pts',(-14.25683142332,-13.7772795192318,115.998898569382)) ;
#186864=CARTESIAN_POINT('Ctrl Pts',(-14.330635262933,-13.7772794788439,
115.974667516101)) ;
#186865=CARTESIAN_POINT('Ctrl Pts',(-14.3531957687261,-13.7542094632266,
116.043383175808)) ;
#186866=CARTESIAN_POINT('Ctrl Pts',(-14.3823024085504,-14.0177953901298,
116.167684414506)) ;
#186867=CARTESIAN_POINT('Ctrl Pts',(-14.4021258436985,-13.976288401055,
116.228063398449)) ;
#186868=CARTESIAN_POINT('Ctrl Pts',(-14.32832200916,-13.9762884453848,116.252294467187)) ;
#186869=CARTESIAN_POINT('Ctrl Pts',(-14.2545181746215,-13.9762884897146,
116.276525535924)) ;
#186870=CARTESIAN_POINT('Ctrl Pts',(-14.2346947394735,-14.0177954787893,
116.216146551981)) ;
#186871=CARTESIAN_POINT('Ctrl Pts',(-14.2148713043254,-14.0593024678641,
116.155767568038)) ;
#186872=CARTESIAN_POINT('Ctrl Pts',(-14.2886751388639,-14.0593024235343,
116.1315364993)) ;
#186873=CARTESIAN_POINT('Ctrl Pts',(-14.3624789734024,-14.0593023792045,
116.107305430563)) ;
#186874=CARTESIAN_POINT('Ctrl Pts',(-14.3823024085504,-14.0177953901298,
116.167684414506)) ;
#186875=CARTESIAN_POINT('Ctrl Pts',(-14.4312100219503,-14.2358411050757,
116.351892811391)) ;
#186876=CARTESIAN_POINT('Ctrl Pts',(-14.4469180075591,-14.1790508956255,
116.399736799939)) ;
#186877=CARTESIAN_POINT('Ctrl Pts',(-14.3731141778863,-14.1790509350975,
116.423967883496)) ;
#186878=CARTESIAN_POINT('Ctrl Pts',(-14.2993103482134,-14.1790509745695,
116.448198967053)) ;
#186879=CARTESIAN_POINT('Ctrl Pts',(-14.2836023626046,-14.2358411840197,
116.400354978505)) ;
#186880=CARTESIAN_POINT('Ctrl Pts',(-14.2678943769957,-14.2926313934699,
116.352510989957)) ;
#186881=CARTESIAN_POINT('Ctrl Pts',(-14.3416982066686,-14.2926313539979,
116.3282799064)) ;
#186882=CARTESIAN_POINT('Ctrl Pts',(-14.4155020363414,-14.2926313145259,
116.304048822843)) ;
#186883=CARTESIAN_POINT('Ctrl Pts',(-14.4312100219503,-14.2358411050757,
116.351892811391)) ;
#186884=CARTESIAN_POINT('Ctrl Pts',(-14.496559976539,-14.3973545116793,
116.586508356455)) ;
#186885=CARTESIAN_POINT('Ctrl Pts',(-14.5069921514621,-14.3292054144305,
116.618283076722)) ;
#186886=CARTESIAN_POINT('Ctrl Pts',(-14.4331883271676,-14.3292054449857,
116.642514176661)) ;
#186887=CARTESIAN_POINT('Ctrl Pts',(-14.3593845028732,-14.3292054755409,
116.6667452766)) ;
#186888=CARTESIAN_POINT('Ctrl Pts',(-14.3489523279501,-14.3973545727897,
116.634970556333)) ;
#186889=CARTESIAN_POINT('Ctrl Pts',(-14.3385201530271,-14.4655036700385,
116.603195836066)) ;
#186890=CARTESIAN_POINT('Ctrl Pts',(-14.4123239773215,-14.4655036394833,
116.578964736127)) ;
#186891=CARTESIAN_POINT('Ctrl Pts',(-14.4861278016159,-14.4655036089281,
116.554733636188)) ;
#186892=CARTESIAN_POINT('Ctrl Pts',(-14.496559976539,-14.3973545116793,
116.586508356455)) ;
#186893=CARTESIAN_POINT('Ctrl Pts',(-14.5724186742539,-14.487909543941,
116.85304175223)) ;
#186894=CARTESIAN_POINT('Ctrl Pts',(-14.5768355566869,-14.4133393487521,
116.866494861983)) ;
#186895=CARTESIAN_POINT('Ctrl Pts',(-14.5030317366878,-14.4133393631785,
116.890725975005)) ;
#186896=CARTESIAN_POINT('Ctrl Pts',(-14.4292279166886,-14.413339377605,
116.914957088027)) ;
#186897=CARTESIAN_POINT('Ctrl Pts',(-14.4248110342556,-14.4879095727939,
116.901503978274)) ;
#186898=CARTESIAN_POINT('Ctrl Pts',(-14.4203941518226,-14.5624797679828,
116.888050868521)) ;
#186899=CARTESIAN_POINT('Ctrl Pts',(-14.4941979718218,-14.5624797535563,
116.863819755499)) ;
#186900=CARTESIAN_POINT('Ctrl Pts',(-14.5680017918209,-14.5624797391299,
116.839588642478)) ;
#186901=CARTESIAN_POINT('Ctrl Pts',(-14.5724186742539,-14.487909543941,
116.85304175223)) ;
#186902=CARTESIAN_POINT('Ctrl Pts',(-14.6524842329724,-14.501998059837,
117.132307744548)) ;
#186903=CARTESIAN_POINT('Ctrl Pts',(-14.6505851061445,-14.4263362561648,
117.126523309047)) ;
#186904=CARTESIAN_POINT('Ctrl Pts',(-14.576781288592,-14.4263362496198,
117.15075442952)) ;
#186905=CARTESIAN_POINT('Ctrl Pts',(-14.5029774710394,-14.4263362430748,
117.174985549994)) ;
#186906=CARTESIAN_POINT('Ctrl Pts',(-14.5048765978673,-14.501998046747,
117.180769985496)) ;
#186907=CARTESIAN_POINT('Ctrl Pts',(-14.5067757246951,-14.5776598504192,
117.186554420997)) ;
#186908=CARTESIAN_POINT('Ctrl Pts',(-14.5805795422476,-14.5776598569642,
117.162323300523)) ;
#186909=CARTESIAN_POINT('Ctrl Pts',(-14.6543833598002,-14.5776598635092,
117.13809218005)) ;
#186910=CARTESIAN_POINT('Ctrl Pts',(-14.6524842329724,-14.501998059837,
117.132307744548)) ;
#186911=CARTESIAN_POINT('Ctrl Pts',(-14.7306703976459,-14.4383564825309,
117.405946024149)) ;
#186912=CARTESIAN_POINT('Ctrl Pts',(-14.7225753482943,-14.3670278101873,
117.381289808219)) ;
#186913=CARTESIAN_POINT('Ctrl Pts',(-14.6487715312239,-14.3670277794582,
117.405520930161)) ;
#186914=CARTESIAN_POINT('Ctrl Pts',(-14.5749677141534,-14.3670277487292,
117.429752052103)) ;
#186915=CARTESIAN_POINT('Ctrl Pts',(-14.583062763505,-14.4383564210728,
117.454408268033)) ;
#186916=CARTESIAN_POINT('Ctrl Pts',(-14.5911578128565,-14.5096850934165,
117.479064483963)) ;
#186917=CARTESIAN_POINT('Ctrl Pts',(-14.6649616299269,-14.5096851241455,
117.454833362021)) ;
#186918=CARTESIAN_POINT('Ctrl Pts',(-14.7387654469974,-14.5096851548746,
117.430602240079)) ;
#186919=CARTESIAN_POINT('Ctrl Pts',(-14.7306703976459,-14.4383564825309,
117.405946024149)) ;
#186920=CARTESIAN_POINT('Ctrl Pts',(-14.8002394306533,-14.3021834028963,
117.653221965588)) ;
#186921=CARTESIAN_POINT('Ctrl Pts',(-14.7865434900334,-14.2402581580985,
117.611506338454)) ;
#186922=CARTESIAN_POINT('Ctrl Pts',(-14.7127396708168,-14.2402581030473,
117.635737453859)) ;
#186923=CARTESIAN_POINT('Ctrl Pts',(-14.6389358516002,-14.2402580479961,
117.659968569264)) ;
#186924=CARTESIAN_POINT('Ctrl Pts',(-14.6526317922202,-14.3021832927938,
117.701684196398)) ;
#186925=CARTESIAN_POINT('Ctrl Pts',(-14.6663277328401,-14.3641085375916,
117.743399823533)) ;
#186926=CARTESIAN_POINT('Ctrl Pts',(-14.7401315520567,-14.3641085926428,
117.719168708127)) ;
#186927=CARTESIAN_POINT('Ctrl Pts',(-14.8139353712733,-14.364108647694,
117.694937592722)) ;
#186928=CARTESIAN_POINT('Ctrl Pts',(-14.8002394306533,-14.3021834028963,
117.653221965588)) ;
#186929=CARTESIAN_POINT('Ctrl Pts',(-14.8560459100839,-14.1010124276425,
117.858868514753)) ;
#186930=CARTESIAN_POINT('Ctrl Pts',(-14.8376956312076,-14.0530410261757,
117.802976524153)) ;
#186931=CARTESIAN_POINT('Ctrl Pts',(-14.7638918076274,-14.0530409478965,
117.827207626268)) ;
#186932=CARTESIAN_POINT('Ctrl Pts',(-14.6900879840472,-14.0530408696173,
117.851438728382)) ;
#186933=CARTESIAN_POINT('Ctrl Pts',(-14.7084382629236,-14.101012271084,
117.907330718982)) ;
#186934=CARTESIAN_POINT('Ctrl Pts',(-14.7267885417999,-14.1489836725507,
117.963222709582)) ;
#186935=CARTESIAN_POINT('Ctrl Pts',(-14.8005923653801,-14.14898375083,117.938991607467)) ;
#186936=CARTESIAN_POINT('Ctrl Pts',(-14.8743961889603,-14.1489838291092,
117.914760505353)) ;
#186937=CARTESIAN_POINT('Ctrl Pts',(-14.8560459100839,-14.1010124276425,
117.858868514753)) ;
#186938=CARTESIAN_POINT('Ctrl Pts',(-14.8924029143783,-13.8533300885713,
118.004875316646)) ;
#186939=CARTESIAN_POINT('Ctrl Pts',(-14.8707577701644,-13.822581157602,
117.938947697799)) ;
#186940=CARTESIAN_POINT('Ctrl Pts',(-14.7969539397415,-13.8225810627118,
117.963178779072)) ;
#186941=CARTESIAN_POINT('Ctrl Pts',(-14.7231501093185,-13.8225809678216,
117.987409860344)) ;
#186942=CARTESIAN_POINT('Ctrl Pts',(-14.7447952535323,-13.8533298987908,
118.053337479191)) ;
#186943=CARTESIAN_POINT('Ctrl Pts',(-14.7664403977462,-13.8840788297601,
118.119265098038)) ;
#186944=CARTESIAN_POINT('Ctrl Pts',(-14.8402442281691,-13.8840789246503,
118.095034016765)) ;
#186945=CARTESIAN_POINT('Ctrl Pts',(-14.9140480585921,-13.8840790195405,
118.070802935493)) ;
#186946=CARTESIAN_POINT('Ctrl Pts',(-14.8924029143783,-13.8533300885713,
118.004875316646)) ;
#186947=CARTESIAN_POINT('Ctrl Pts',(-14.9068420422244,-13.5731370136184,
118.084346390465)) ;
#186948=CARTESIAN_POINT('Ctrl Pts',(-14.8834226218003,-13.5619047330003,
118.013014612504)) ;
#186949=CARTESIAN_POINT('Ctrl Pts',(-14.8096187831826,-13.5619046275825,
118.037245668817)) ;
#186950=CARTESIAN_POINT('Ctrl Pts',(-14.735814944565,-13.5619045221647,
118.061476725129)) ;
#186951=CARTESIAN_POINT('Ctrl Pts',(-14.7592343649891,-13.5731368027828,
118.132808503091)) ;
#186952=CARTESIAN_POINT('Ctrl Pts',(-14.7826537854132,-13.5843690834008,
118.204140281052)) ;
#186953=CARTESIAN_POINT('Ctrl Pts',(-14.8564576240309,-13.5843691888186,
118.179909224739)) ;
#186954=CARTESIAN_POINT('Ctrl Pts',(-14.9302614626486,-13.5843692942365,
118.155678168426)) ;
#186955=CARTESIAN_POINT('Ctrl Pts',(-14.9068420422244,-13.5731370136184,
118.084346390465)) ;
#186956=CARTESIAN_POINT('Ctrl Pts',(-14.8970281712621,-13.2811248351023,
118.09002242941)) ;
#186957=CARTESIAN_POINT('Ctrl Pts',(-14.873523327877,-13.2902630338005,
118.018430466862)) ;
#186958=CARTESIAN_POINT('Ctrl Pts',(-14.7997194802372,-13.2902629265376,
118.042661495695)) ;
#186959=CARTESIAN_POINT('Ctrl Pts',(-14.7259156325975,-13.2902628192747,
118.066892524528)) ;
#186960=CARTESIAN_POINT('Ctrl Pts',(-14.7494204759826,-13.2811246205765,
118.138484487076)) ;
#186961=CARTESIAN_POINT('Ctrl Pts',(-14.7729253193677,-13.2719864218783,
118.210076449624)) ;
#186962=CARTESIAN_POINT('Ctrl Pts',(-14.8467291670075,-13.2719865291412,
118.185845420791)) ;
#186963=CARTESIAN_POINT('Ctrl Pts',(-14.9205330146472,-13.2719866364041,
118.161614391958)) ;
#186964=CARTESIAN_POINT('Ctrl Pts',(-14.8970281712621,-13.2811248351023,
118.09002242941)) ;
#186965=CARTESIAN_POINT('Ctrl Pts',(-14.8632710167406,-13.0003515927813,
118.022582055255)) ;
#186966=CARTESIAN_POINT('Ctrl Pts',(-14.8413562508323,-13.0291058472193,
117.955833212136)) ;
#186967=CARTESIAN_POINT('Ctrl Pts',(-14.7675523944075,-13.029105747077,
117.980064214212)) ;
#186968=CARTESIAN_POINT('Ctrl Pts',(-14.6937485379827,-13.0291056469348,
118.004295216287)) ;
#186969=CARTESIAN_POINT('Ctrl Pts',(-14.715663303891,-13.0003513924967,
118.071044059405)) ;
#186970=CARTESIAN_POINT('Ctrl Pts',(-14.7375780697992,-12.9715971380587,
118.137792902524)) ;
#186971=CARTESIAN_POINT('Ctrl Pts',(-14.811381926224,-12.971597238201,118.113561900449)) ;
#186972=CARTESIAN_POINT('Ctrl Pts',(-14.8851857826488,-12.9715973383433,
118.089330898374)) ;
#186973=CARTESIAN_POINT('Ctrl Pts',(-14.8632710167406,-13.0003515927813,
118.022582055255)) ;
#186974=CARTESIAN_POINT('Ctrl Pts',(-14.8066072910896,-12.7476820967297,
117.885649589391)) ;
#186975=CARTESIAN_POINT('Ctrl Pts',(-14.7878780661755,-12.7941196142379,
117.828603390177)) ;
#186976=CARTESIAN_POINT('Ctrl Pts',(-14.7140742020926,-12.794119529764,
117.852834368926)) ;
#186977=CARTESIAN_POINT('Ctrl Pts',(-14.6402703380096,-12.7941194452901,
117.877065347676)) ;
#186978=CARTESIAN_POINT('Ctrl Pts',(-14.6589995629237,-12.7476819277819,
117.93411154689)) ;
#186979=CARTESIAN_POINT('Ctrl Pts',(-14.6777287878378,-12.7012444102737,
117.991157746104)) ;
#186980=CARTESIAN_POINT('Ctrl Pts',(-14.7515326519207,-12.7012444947476,
117.966926767354)) ;
#186981=CARTESIAN_POINT('Ctrl Pts',(-14.8253365160036,-12.7012445792215,
117.942695788605)) ;
#186982=CARTESIAN_POINT('Ctrl Pts',(-14.8066072910896,-12.7476820967297,
117.885649589391)) ;
#186983=CARTESIAN_POINT('Ctrl Pts',(-14.731619858714,-12.5456564605608,
117.692468627956)) ;
#186984=CARTESIAN_POINT('Ctrl Pts',(-14.7173696349214,-12.6062676271749,
117.649064743502)) ;
#186985=CARTESIAN_POINT('Ctrl Pts',(-14.6435657649829,-12.6062675641062,
117.673295704416)) ;
#186986=CARTESIAN_POINT('Ctrl Pts',(-14.5697618950443,-12.6062675010375,
117.697526665331)) ;
#186987=CARTESIAN_POINT('Ctrl Pts',(-14.584012118837,-12.5456563344234,
117.740930549785)) ;
#186988=CARTESIAN_POINT('Ctrl Pts',(-14.5982623426296,-12.4850451678094,
117.784334434238)) ;
#186989=CARTESIAN_POINT('Ctrl Pts',(-14.6720662125682,-12.4850452308781,
117.760103473324)) ;
#186990=CARTESIAN_POINT('Ctrl Pts',(-14.7458700825067,-12.4850452939468,
117.735872512409)) ;
#186991=CARTESIAN_POINT('Ctrl Pts',(-14.731619858714,-12.5456564605608,
117.692468627956)) ;
#186992=CARTESIAN_POINT('Ctrl Pts',(-14.6415003508754,-12.4041536111177,
117.453518839536)) ;
#186993=CARTESIAN_POINT('Ctrl Pts',(-14.6327852655242,-12.4747346832578,
117.426974093744)) ;
#186994=CARTESIAN_POINT('Ctrl Pts',(-14.5589813922061,-12.474734646304,
117.451205044365)) ;
#186995=CARTESIAN_POINT('Ctrl Pts',(-14.485177518888,-12.4747346093502,
117.475435994985)) ;
#186996=CARTESIAN_POINT('Ctrl Pts',(-14.4938926042392,-12.4041535372102,
117.501980740777)) ;
#186997=CARTESIAN_POINT('Ctrl Pts',(-14.5026076895904,-12.3335724650701,
117.528525486569)) ;
#186998=CARTESIAN_POINT('Ctrl Pts',(-14.5764115629085,-12.3335725020239,
117.504294535948)) ;
#186999=CARTESIAN_POINT('Ctrl Pts',(-14.6502154362266,-12.3335725389777,
117.480063585327)) ;
#187000=CARTESIAN_POINT('Ctrl Pts',(-14.6415003508754,-12.4041536111177,
117.453518839536)) ;
#187001=CARTESIAN_POINT('Ctrl Pts',(-14.5427756645505,-12.3358248594298,
117.188253387746)) ;
#187002=CARTESIAN_POINT('Ctrl Pts',(-14.540207049171,-12.4112821257934,
117.180429797836)) ;
#187003=CARTESIAN_POINT('Ctrl Pts',(-14.4664031750961,-12.4112821160611,
117.204660746152)) ;
#187004=CARTESIAN_POINT('Ctrl Pts',(-14.3925993010213,-12.4112821063287,
117.228891694468)) ;
#187005=CARTESIAN_POINT('Ctrl Pts',(-14.3951679164008,-12.3358248399652,
117.236715284378)) ;
#187006=CARTESIAN_POINT('Ctrl Pts',(-14.3977365317803,-12.2603675736016,
117.244538874289)) ;
#187007=CARTESIAN_POINT('Ctrl Pts',(-14.4715404058551,-12.2603675833339,
117.220307925973)) ;
#187008=CARTESIAN_POINT('Ctrl Pts',(-14.54534427993,-12.2603675930662,117.196076977657)) ;
#187009=CARTESIAN_POINT('Ctrl Pts',(-14.5427756645505,-12.3358248594298,
117.188253387746)) ;
#187010=CARTESIAN_POINT('Ctrl Pts',(-14.4412974521352,-12.3448661715,116.914695399422)) ;
#187011=CARTESIAN_POINT('Ctrl Pts',(-14.445074775662,-12.4198057290159,
116.926200515611)) ;
#187012=CARTESIAN_POINT('Ctrl Pts',(-14.3712709035495,-12.41980574501,116.950431469904)) ;
#187013=CARTESIAN_POINT('Ctrl Pts',(-14.2974670314371,-12.4198057610042,
116.974662424197)) ;
#187014=CARTESIAN_POINT('Ctrl Pts',(-14.2936897079104,-12.3448662034884,
116.963157308008)) ;
#187015=CARTESIAN_POINT('Ctrl Pts',(-14.2899123843836,-12.2699266459725,
116.95165219182)) ;
#187016=CARTESIAN_POINT('Ctrl Pts',(-14.363716256496,-12.2699266299783,
116.927421237527)) ;
#187017=CARTESIAN_POINT('Ctrl Pts',(-14.4375201286084,-12.2699266139842,
116.903190283233)) ;
#187018=CARTESIAN_POINT('Ctrl Pts',(-14.4412974521352,-12.3448661715,116.914695399422)) ;
#187019=CARTESIAN_POINT('Ctrl Pts',(-14.343860133739,-12.4312374679016,
116.653442961443)) ;
#187020=CARTESIAN_POINT('Ctrl Pts',(-14.3537109607349,-12.5002598101882,
116.683446989369)) ;
#187021=CARTESIAN_POINT('Ctrl Pts',(-14.2799070928255,-12.5002598472916,
116.707677956464)) ;
#187022=CARTESIAN_POINT('Ctrl Pts',(-14.206103224916,-12.5002598843951,
116.731908923559)) ;
#187023=CARTESIAN_POINT('Ctrl Pts',(-14.1962523979201,-12.4312375421085,
116.701904895633)) ;
#187024=CARTESIAN_POINT('Ctrl Pts',(-14.1864015709241,-12.3622151998219,
116.671900867707)) ;
#187025=CARTESIAN_POINT('Ctrl Pts',(-14.2602054388336,-12.3622151627184,
116.647669900612)) ;
#187026=CARTESIAN_POINT('Ctrl Pts',(-14.334009306743,-12.362215125615,116.623438933518)) ;
#187027=CARTESIAN_POINT('Ctrl Pts',(-14.343860133739,-12.4312374679016,
116.653442961443)) ;
#187028=CARTESIAN_POINT('Ctrl Pts',(-14.2571254625577,-12.5874506151636,
116.424600508651)) ;
#187029=CARTESIAN_POINT('Ctrl Pts',(-14.2723156315512,-12.6456701044934,
116.470867310915)) ;
#187030=CARTESIAN_POINT('Ctrl Pts',(-14.1985117689653,-12.6456701572597,
116.495098294225)) ;
#187031=CARTESIAN_POINT('Ctrl Pts',(-14.1247079063794,-12.6456702100259,
116.519329277534)) ;
#187032=CARTESIAN_POINT('Ctrl Pts',(-14.1095177373858,-12.5874507206961,
116.47306247527)) ;
#187033=CARTESIAN_POINT('Ctrl Pts',(-14.0943275683923,-12.5292312313663,
116.426795673006)) ;
#187034=CARTESIAN_POINT('Ctrl Pts',(-14.1681314309782,-12.5292311786001,
116.402564689697)) ;
#187035=CARTESIAN_POINT('Ctrl Pts',(-14.2419352935641,-12.5292311258338,
116.378333706388)) ;
#187036=CARTESIAN_POINT('Ctrl Pts',(-14.2571254625577,-12.5874506151636,
116.424600508651)) ;
#187037=CARTESIAN_POINT('Ctrl Pts',(-14.1857294690377,-12.8034012905554,
116.242593659253)) ;
#187038=CARTESIAN_POINT('Ctrl Pts',(-14.2051937787915,-12.8466312900345,
116.301878804784)) ;
#187039=CARTESIAN_POINT('Ctrl Pts',(-14.1313899225984,-12.8466313512928,
116.326109807565)) ;
#187040=CARTESIAN_POINT('Ctrl Pts',(-14.0575860664052,-12.8466314125512,
116.350340810346)) ;
#187041=CARTESIAN_POINT('Ctrl Pts',(-14.0381217566514,-12.8034014130721,
116.291055664815)) ;
#187042=CARTESIAN_POINT('Ctrl Pts',(-14.0186574468976,-12.760171413593,
116.231770519284)) ;
#187043=CARTESIAN_POINT('Ctrl Pts',(-14.0924613030908,-12.7601713523347,
116.207539516503)) ;
#187044=CARTESIAN_POINT('Ctrl Pts',(-14.1662651592839,-12.7601712910763,
116.183308513722)) ;
#187045=CARTESIAN_POINT('Ctrl Pts',(-14.1857294690377,-12.8034012905554,
116.242593659253)) ;
#187046=CARTESIAN_POINT('Ctrl Pts',(-14.1342915112544,-13.0643708673509,
116.121492146728)) ;
#187047=CARTESIAN_POINT('Ctrl Pts',(-14.1566407442375,-13.0894456413712,
116.18956430311)) ;
#187048=CARTESIAN_POINT('Ctrl Pts',(-14.0828368945042,-13.0894457028003,
116.213795325566)) ;
#187049=CARTESIAN_POINT('Ctrl Pts',(-14.009033044771,-13.0894457642295,
116.238026348023)) ;
#187050=CARTESIAN_POINT('Ctrl Pts',(-13.9866838117879,-13.0643709902092,
116.169954191642)) ;
#187051=CARTESIAN_POINT('Ctrl Pts',(-13.9643345788048,-13.0392962161889,
116.10188203526)) ;
#187052=CARTESIAN_POINT('Ctrl Pts',(-14.0381384285381,-13.0392961547597,
116.077651012804)) ;
#187053=CARTESIAN_POINT('Ctrl Pts',(-14.1119422782713,-13.0392960933306,
116.053419990347)) ;
#187054=CARTESIAN_POINT('Ctrl Pts',(-14.1342915112544,-13.0643708673509,
116.121492146728)) ;
#187055=CARTESIAN_POINT('Ctrl Pts',(-14.1060138274789,-13.3499213722247,
116.070822960069)) ;
#187056=CARTESIAN_POINT('Ctrl Pts',(-14.1296375462713,-13.355096833582,
116.142776994751)) ;
#187057=CARTESIAN_POINT('Ctrl Pts',(-14.0558337020276,-13.3550968897529,
116.167008033928)) ;
#187058=CARTESIAN_POINT('Ctrl Pts',(-13.982029857784,-13.3550969459238,
116.191239073105)) ;
#187059=CARTESIAN_POINT('Ctrl Pts',(-13.9584061389915,-13.3499214845666,
116.119285038423)) ;
#187060=CARTESIAN_POINT('Ctrl Pts',(-13.9347824201991,-13.3447460232093,
116.047331003741)) ;
#187061=CARTESIAN_POINT('Ctrl Pts',(-14.0085862644428,-13.3447459670383,
116.023099964565)) ;
#187062=CARTESIAN_POINT('Ctrl Pts',(-14.0823901086865,-13.3447459108674,
115.998868925388)) ;
#187063=CARTESIAN_POINT('Ctrl Pts',(-14.1060138274789,-13.3499213722247,
116.070822960069)) ;
#187064=CARTESIAN_POINT('Ctrl Pts',(-14.1020431169035,-13.6410985525755,
116.094287590877)) ;
#187065=CARTESIAN_POINT('Ctrl Pts',(-14.1252441893859,-13.6259514029626,
116.164954313278)) ;
#187066=CARTESIAN_POINT('Ctrl Pts',(-14.0514403491928,-13.625951448446,
116.189185364793)) ;
#187067=CARTESIAN_POINT('Ctrl Pts',(-13.9776365089998,-13.6259514939294,
116.213416416307)) ;
#187068=CARTESIAN_POINT('Ctrl Pts',(-13.9544354365173,-13.6410986435423,
116.142749693906)) ;
#187069=CARTESIAN_POINT('Ctrl Pts',(-13.9312343640349,-13.6562457931553,
116.072082971505)) ;
#187070=CARTESIAN_POINT('Ctrl Pts',(-14.0050382042279,-13.6562457476719,
116.04785191999)) ;
#187071=CARTESIAN_POINT('Ctrl Pts',(-14.078842044421,-13.6562457021885,
116.023620868476)) ;
#187072=CARTESIAN_POINT('Ctrl Pts',(-14.1020431169035,-13.6410985525755,
116.094287590877)) ;
#187073=CARTESIAN_POINT('Ctrl Pts',(-14.1217724434522,-13.9144130152127,
116.189693352615)) ;
#187074=CARTESIAN_POINT('Ctrl Pts',(-14.142900281541,-13.8801596021724,
116.254045337708)) ;
#187075=CARTESIAN_POINT('Ctrl Pts',(-14.06909644393,-13.8801596369213,116.278276397087)) ;
#187076=CARTESIAN_POINT('Ctrl Pts',(-13.995292606319,-13.8801596716703,
116.302507456466)) ;
#187077=CARTESIAN_POINT('Ctrl Pts',(-13.9741647682302,-13.9144130847105,
116.238155471373)) ;
#187078=CARTESIAN_POINT('Ctrl Pts',(-13.9530369301413,-13.9486664977508,
116.173803486281)) ;
#187079=CARTESIAN_POINT('Ctrl Pts',(-14.0268407677523,-13.9486664630018,
116.149572426902)) ;
#187080=CARTESIAN_POINT('Ctrl Pts',(-14.1006446053633,-13.9486664282529,
116.125341367522)) ;
#187081=CARTESIAN_POINT('Ctrl Pts',(-14.1217724434522,-13.9144130152127,
116.189693352615)) ;
#187082=CARTESIAN_POINT('Ctrl Pts',(-14.1631227784727,-14.1534993419982,
116.351109244316)) ;
#187083=CARTESIAN_POINT('Ctrl Pts',(-14.1806614860516,-14.1025003039047,
116.404529317146)) ;
#187084=CARTESIAN_POINT('Ctrl Pts',(-14.1068576493241,-14.1025003260636,
116.428760379216)) ;
#187085=CARTESIAN_POINT('Ctrl Pts',(-14.0330538125967,-14.1025003482225,
116.452991441286)) ;
#187086=CARTESIAN_POINT('Ctrl Pts',(-14.0155151050178,-14.153499386316,
116.399571368456)) ;
#187087=CARTESIAN_POINT('Ctrl Pts',(-13.9979763974389,-14.2044984244094,
116.346151295626)) ;
#187088=CARTESIAN_POINT('Ctrl Pts',(-14.0717802341664,-14.2044984022505,
116.321920233556)) ;
#187089=CARTESIAN_POINT('Ctrl Pts',(-14.1455840708938,-14.2044983800916,
116.297689171486)) ;
#187090=CARTESIAN_POINT('Ctrl Pts',(-14.1631227784727,-14.1534993419982,
116.351109244316)) ;
#187091=CARTESIAN_POINT('Ctrl Pts',(-14.2224761505657,-14.3398532357648,
116.567378763877)) ;
#187092=CARTESIAN_POINT('Ctrl Pts',(-14.2351627561795,-14.2757649069183,
116.606020117166)) ;
#187093=CARTESIAN_POINT('Ctrl Pts',(-14.1613589188212,-14.275764918267,
116.630251177315)) ;
#187094=CARTESIAN_POINT('Ctrl Pts',(-14.0875550814629,-14.2757649296157,
116.654482237464)) ;
#187095=CARTESIAN_POINT('Ctrl Pts',(-14.074868475849,-14.3398532584622,
116.615840884175)) ;
#187096=CARTESIAN_POINT('Ctrl Pts',(-14.0621818702352,-14.4039415873087,
116.577199530885)) ;
#187097=CARTESIAN_POINT('Ctrl Pts',(-14.1359857075935,-14.4039415759601,
116.552968470736)) ;
#187098=CARTESIAN_POINT('Ctrl Pts',(-14.2097895449518,-14.4039415646114,
116.528737410587)) ;
#187099=CARTESIAN_POINT('Ctrl Pts',(-14.2224761505657,-14.3398532357648,
116.567378763877)) ;
#187100=CARTESIAN_POINT('Ctrl Pts',(-14.2946184727388,-14.4601239905911,
116.822545240019)) ;
#187101=CARTESIAN_POINT('Ctrl Pts',(-14.3015537228685,-14.3875409587586,
116.843668892623)) ;
#187102=CARTESIAN_POINT('Ctrl Pts',(-14.2277498840453,-14.3875409624437,
116.86789994831)) ;
#187103=CARTESIAN_POINT('Ctrl Pts',(-14.153946045222,-14.3875409661288,
116.892131003996)) ;
#187104=CARTESIAN_POINT('Ctrl Pts',(-14.1470107950923,-14.4601239979614,
116.871007351393)) ;
#187105=CARTESIAN_POINT('Ctrl Pts',(-14.1400755449626,-14.532707029794,
116.849883698789)) ;
#187106=CARTESIAN_POINT('Ctrl Pts',(-14.2138793837858,-14.5327070261088,
116.825652643102)) ;
#187107=CARTESIAN_POINT('Ctrl Pts',(-14.2876832226091,-14.5327070224237,
116.801421587416)) ;
#187108=CARTESIAN_POINT('Ctrl Pts',(-14.2946184727388,-14.4601239905911,
116.822545240019)) ;
#187109=CARTESIAN_POINT('Ctrl Pts',(-14.3741114267092,-14.5056532387337,
117.100264991934)) ;
#187110=CARTESIAN_POINT('Ctrl Pts',(-14.3747697725925,-14.4297812015044,
117.102270207122)) ;
#187111=CARTESIAN_POINT('Ctrl Pts',(-14.3009659315983,-14.4297812011716,
117.126501256196)) ;
#187112=CARTESIAN_POINT('Ctrl Pts',(-14.227162090604,-14.4297812008388,
117.150732305271)) ;
#187113=CARTESIAN_POINT('Ctrl Pts',(-14.2265037447207,-14.5056532380682,
117.148727090083)) ;
#187114=CARTESIAN_POINT('Ctrl Pts',(-14.2258453988374,-14.5815252752975,
117.146721874895)) ;
#187115=CARTESIAN_POINT('Ctrl Pts',(-14.2996492398317,-14.5815252756303,
117.122490825821)) ;
#187116=CARTESIAN_POINT('Ctrl Pts',(-14.3734530808259,-14.5815252759631,
117.098259776747)) ;
#187117=CARTESIAN_POINT('Ctrl Pts',(-14.3741114267092,-14.5056532387337,
117.100264991934)) ;
#187118=CARTESIAN_POINT('Ctrl Pts',(-14.4533987795497,-14.4736304498916,
117.377007393314)) ;
#187119=CARTESIAN_POINT('Ctrl Pts',(-14.4477925032055,-14.3998809483868,
117.35993158007)) ;
#187120=CARTESIAN_POINT('Ctrl Pts',(-14.3739886608311,-14.3998809471274,
117.384162624941)) ;
#187121=CARTESIAN_POINT('Ctrl Pts',(-14.3001848184568,-14.399880945868,
117.408393669812)) ;
#187122=CARTESIAN_POINT('Ctrl Pts',(-14.305791094801,-14.4736304473727,
117.425469483055)) ;
#187123=CARTESIAN_POINT('Ctrl Pts',(-14.3113973711451,-14.5473799488775,
117.442545296299)) ;
#187124=CARTESIAN_POINT('Ctrl Pts',(-14.3852012135195,-14.5473799501369,
117.418314251428)) ;
#187125=CARTESIAN_POINT('Ctrl Pts',(-14.4590050558939,-14.5473799513963,
117.394083206557)) ;
#187126=CARTESIAN_POINT('Ctrl Pts',(-14.4533987795497,-14.4736304498916,
117.377007393314)) ;
#187127=CARTESIAN_POINT('Ctrl Pts',(-14.5277960537178,-14.3649486844788,
117.639339779354)) ;
#187128=CARTESIAN_POINT('Ctrl Pts',(-14.5162467148877,-14.2986771390851,
117.604162356787)) ;
#187129=CARTESIAN_POINT('Ctrl Pts',(-14.4424428710041,-14.2986771395707,
117.628393397061)) ;
#187130=CARTESIAN_POINT('Ctrl Pts',(-14.3686390271205,-14.2986771400562,
117.652624437334)) ;
#187131=CARTESIAN_POINT('Ctrl Pts',(-14.3801883659506,-14.36494868545,117.687801859902)) ;
#187132=CARTESIAN_POINT('Ctrl Pts',(-14.3917377047807,-14.4312202308437,
117.722979282469)) ;
#187133=CARTESIAN_POINT('Ctrl Pts',(-14.4655415486643,-14.4312202303581,
117.698748242195)) ;
#187134=CARTESIAN_POINT('Ctrl Pts',(-14.5393453925479,-14.4312202298725,
117.674517201921)) ;
#187135=CARTESIAN_POINT('Ctrl Pts',(-14.5277960537178,-14.3649486844788,
117.639339779354)) ;
#187136=CARTESIAN_POINT('Ctrl Pts',(-14.5893935819376,-14.1895250687342,
117.862280414285)) ;
#187137=CARTESIAN_POINT('Ctrl Pts',(-14.5727948609667,-14.1354046364552,
117.81172338846)) ;
#187138=CARTESIAN_POINT('Ctrl Pts',(-14.4989910168738,-14.1354046385753,
117.835954428096)) ;
#187139=CARTESIAN_POINT('Ctrl Pts',(-14.4251871727808,-14.1354046406955,
117.860185467732)) ;
#187140=CARTESIAN_POINT('Ctrl Pts',(-14.4417858937517,-14.1895250729745,
117.910742493557)) ;
#187141=CARTESIAN_POINT('Ctrl Pts',(-14.4583846147226,-14.2436455052536,
117.961299519382)) ;
#187142=CARTESIAN_POINT('Ctrl Pts',(-14.5321884588155,-14.2436455031334,
117.937068479746)) ;
#187143=CARTESIAN_POINT('Ctrl Pts',(-14.6059923029085,-14.2436455010133,
117.91283744011)) ;
#187144=CARTESIAN_POINT('Ctrl Pts',(-14.5893935819376,-14.1895250687342,
117.862280414285)) ;
#187145=CARTESIAN_POINT('Ctrl Pts',(-14.6341408629526,-13.9587919846541,
118.03400595603)) ;
#187146=CARTESIAN_POINT('Ctrl Pts',(-14.6136596183547,-13.9207033555361,
117.971623389682)) ;
#187147=CARTESIAN_POINT('Ctrl Pts',(-14.5398557744747,-13.9207033583064,
117.995854429967)) ;
#187148=CARTESIAN_POINT('Ctrl Pts',(-14.4660519305947,-13.9207033610767,
118.020085470252)) ;
#187149=CARTESIAN_POINT('Ctrl Pts',(-14.4865331751926,-13.9587919901947,
118.0824680366)) ;
#187150=CARTESIAN_POINT('Ctrl Pts',(-14.5070144197905,-13.9968806193127,
118.144850602948)) ;
#187151=CARTESIAN_POINT('Ctrl Pts',(-14.5808182636705,-13.9968806165424,
118.120619562663)) ;
#187152=CARTESIAN_POINT('Ctrl Pts',(-14.6546221075505,-13.9968806137721,
118.096388522378)) ;
#187153=CARTESIAN_POINT('Ctrl Pts',(-14.6341408629526,-13.9587919846541,
118.03400595603)) ;
#187154=CARTESIAN_POINT('Ctrl Pts',(-14.6578474674141,-13.6889251841896,
118.141687163371)) ;
#187155=CARTESIAN_POINT('Ctrl Pts',(-14.6349465238755,-13.6696247434328,
118.071934584426)) ;
#187156=CARTESIAN_POINT('Ctrl Pts',(-14.5611426804866,-13.6696247444935,
118.096165626206)) ;
#187157=CARTESIAN_POINT('Ctrl Pts',(-14.4873388370977,-13.6696247455542,
118.120396667987)) ;
#187158=CARTESIAN_POINT('Ctrl Pts',(-14.5102397806364,-13.688925186311,
118.190149246933)) ;
#187159=CARTESIAN_POINT('Ctrl Pts',(-14.533140724175,-13.7082256270677,
118.259901825878)) ;
#187160=CARTESIAN_POINT('Ctrl Pts',(-14.6069445675639,-13.708225626007,
118.235670784098)) ;
#187161=CARTESIAN_POINT('Ctrl Pts',(-14.6807484109528,-13.7082256249463,
118.211439742317)) ;
#187162=CARTESIAN_POINT('Ctrl Pts',(-14.6578474674141,-13.6889251841896,
118.141687163371)) ;
#187163=CARTESIAN_POINT('Ctrl Pts',(-14.6579187734562,-13.3992086458092,
118.177435917564)) ;
#187164=CARTESIAN_POINT('Ctrl Pts',(-14.6342439439393,-13.4001099249718,
118.10532620671)) ;
#187165=CARTESIAN_POINT('Ctrl Pts',(-14.5604401006268,-13.4001099216027,
118.129557248723)) ;
#187166=CARTESIAN_POINT('Ctrl Pts',(-14.4866362573143,-13.4001099182335,
118.153788290736)) ;
#187167=CARTESIAN_POINT('Ctrl Pts',(-14.5103110868312,-13.3992086390708,
118.225898001591)) ;
#187168=CARTESIAN_POINT('Ctrl Pts',(-14.5339859163481,-13.3983073599082,
118.298007712445)) ;
#187169=CARTESIAN_POINT('Ctrl Pts',(-14.6077897596606,-13.3983073632774,
118.273776670431)) ;
#187170=CARTESIAN_POINT('Ctrl Pts',(-14.6815936029731,-13.3983073666465,
118.249545628418)) ;
#187171=CARTESIAN_POINT('Ctrl Pts',(-14.6579187734562,-13.3992086458092,
118.177435917564)) ;
#187172=CARTESIAN_POINT('Ctrl Pts',(-14.6338690635927,-13.1124266878776,
118.139508403159)) ;
#187173=CARTESIAN_POINT('Ctrl Pts',(-14.6111080927267,-13.13335350732,118.070182158217)) ;
#187174=CARTESIAN_POINT('Ctrl Pts',(-14.5373042487991,-13.1333534995856,
118.094413198357)) ;
#187175=CARTESIAN_POINT('Ctrl Pts',(-14.4635004048714,-13.1333534918511,
118.118644238497)) ;
#187176=CARTESIAN_POINT('Ctrl Pts',(-14.4862613757375,-13.1124266724087,
118.187970483438)) ;
#187177=CARTESIAN_POINT('Ctrl Pts',(-14.5090223466035,-13.0914998529662,
118.257296728379)) ;
#187178=CARTESIAN_POINT('Ctrl Pts',(-14.5828261905311,-13.0914998607007,
118.233065688239)) ;
#187179=CARTESIAN_POINT('Ctrl Pts',(-14.6566300344588,-13.0914998684351,
118.2088346481)) ;
#187180=CARTESIAN_POINT('Ctrl Pts',(-14.6338690635927,-13.1124266878776,
118.139508403159)) ;
#187181=CARTESIAN_POINT('Ctrl Pts',(-14.5860912781424,-12.8450096600115,
118.029650693302)) ;
#187182=CARTESIAN_POINT('Ctrl Pts',(-14.5658950360717,-12.8846394195873,
117.968136198297)) ;
#187183=CARTESIAN_POINT('Ctrl Pts',(-14.492091190218,-12.8846394056337,
117.99236723257)) ;
#187184=CARTESIAN_POINT('Ctrl Pts',(-14.4182873443643,-12.8846393916802,
118.016598266843)) ;
#187185=CARTESIAN_POINT('Ctrl Pts',(-14.4384835864349,-12.8450096321044,
118.078112761848)) ;
#187186=CARTESIAN_POINT('Ctrl Pts',(-14.4586798285056,-12.8053798725287,
118.139627256853)) ;
#187187=CARTESIAN_POINT('Ctrl Pts',(-14.5324836743593,-12.8053798864822,
118.11539622258)) ;
#187188=CARTESIAN_POINT('Ctrl Pts',(-14.606287520213,-12.8053799004358,
118.091165188307)) ;
#187189=CARTESIAN_POINT('Ctrl Pts',(-14.5860912781424,-12.8450096600115,
118.029650693302)) ;
#187190=CARTESIAN_POINT('Ctrl Pts',(-14.5180421746605,-12.6209217910559,
117.857738555032)) ;
#187191=CARTESIAN_POINT('Ctrl Pts',(-14.5018364773262,-12.6762550632743,
117.808378615293)) ;
#187192=CARTESIAN_POINT('Ctrl Pts',(-14.4280326288564,-12.6762550473825,
117.832609641598)) ;
#187193=CARTESIAN_POINT('Ctrl Pts',(-14.3542287803866,-12.6762550314906,
117.856840667903)) ;
#187194=CARTESIAN_POINT('Ctrl Pts',(-14.370434477721,-12.6209217592723,
117.906200607642)) ;
#187195=CARTESIAN_POINT('Ctrl Pts',(-14.3866401750554,-12.5655884870539,
117.955560547382)) ;
#187196=CARTESIAN_POINT('Ctrl Pts',(-14.4604440235251,-12.5655885029457,
117.931329521077)) ;
#187197=CARTESIAN_POINT('Ctrl Pts',(-14.5342478719949,-12.5655885188375,
117.907098494772)) ;
#187198=CARTESIAN_POINT('Ctrl Pts',(-14.5180421746605,-12.6209217910559,
117.857738555032)) ;
#187199=CARTESIAN_POINT('Ctrl Pts',(-14.4333682313744,-12.453038777336,
117.635286933608)) ;
#187200=CARTESIAN_POINT('Ctrl Pts',(-14.4223175253448,-12.520173907181,
117.601628265473)) ;
#187201=CARTESIAN_POINT('Ctrl Pts',(-14.3485136735579,-12.5201738923226,
117.625859281675)) ;
#187202=CARTESIAN_POINT('Ctrl Pts',(-14.2747098217711,-12.5201738774643,
117.650090297877)) ;
#187203=CARTESIAN_POINT('Ctrl Pts',(-14.2857605278008,-12.4530387476193,
117.683748966012)) ;
#187204=CARTESIAN_POINT('Ctrl Pts',(-14.2968112338305,-12.3859036177743,
117.717407634146)) ;
#187205=CARTESIAN_POINT('Ctrl Pts',(-14.3706150856173,-12.3859036326327,
117.693176617944)) ;
#187206=CARTESIAN_POINT('Ctrl Pts',(-14.4444189374041,-12.385903647491,
117.668945601743)) ;
#187207=CARTESIAN_POINT('Ctrl Pts',(-14.4333682313744,-12.453038777336,
117.635286933608)) ;
#187208=CARTESIAN_POINT('Ctrl Pts',(-14.337341154014,-12.3543368017594,
117.378290551669)) ;
#187209=CARTESIAN_POINT('Ctrl Pts',(-14.3322448096572,-12.4284604690025,
117.362767908288)) ;
#187210=CARTESIAN_POINT('Ctrl Pts',(-14.2584409542665,-12.4284604600379,
117.386998913513)) ;
#187211=CARTESIAN_POINT('Ctrl Pts',(-14.1846370988758,-12.4284604510733,
117.411229918738)) ;
#187212=CARTESIAN_POINT('Ctrl Pts',(-14.1897334432325,-12.3543367838302,
117.426752562119)) ;
#187213=CARTESIAN_POINT('Ctrl Pts',(-14.1948297875893,-12.2802131165871,
117.4422752055)) ;
#187214=CARTESIAN_POINT('Ctrl Pts',(-14.26863364298,-12.2802131255517,117.418044200275)) ;
#187215=CARTESIAN_POINT('Ctrl Pts',(-14.3424374983707,-12.2802131345163,
117.39381319505)) ;
#187216=CARTESIAN_POINT('Ctrl Pts',(-14.337341154014,-12.3543368017594,
117.378290551669)) ;
#187217=CARTESIAN_POINT('Ctrl Pts',(-14.2364443666952,-12.3316786589988,
117.10637745565)) ;
#187218=CARTESIAN_POINT('Ctrl Pts',(-14.2376526605417,-12.4074912166658,
117.11005772283)) ;
#187219=CARTESIAN_POINT('Ctrl Pts',(-14.1638488023011,-12.4074912185027,
117.134288719375)) ;
#187220=CARTESIAN_POINT('Ctrl Pts',(-14.0900449440605,-12.4074912203397,
117.15851971592)) ;
#187221=CARTESIAN_POINT('Ctrl Pts',(-14.0888366502139,-12.3316786626727,
117.15483944874)) ;
#187222=CARTESIAN_POINT('Ctrl Pts',(-14.0876283563674,-12.2558661050058,
117.15115918156)) ;
#187223=CARTESIAN_POINT('Ctrl Pts',(-14.161432214608,-12.2558661031688,
117.126928185015)) ;
#187224=CARTESIAN_POINT('Ctrl Pts',(-14.2352360728486,-12.2558661013318,
117.10269718847)) ;
#187225=CARTESIAN_POINT('Ctrl Pts',(-14.2364443666952,-12.3316786589988,
117.10637745565)) ;
#187226=CARTESIAN_POINT('Ctrl Pts',(-14.1362341376129,-12.3873927929882,
116.836808898935)) ;
#187227=CARTESIAN_POINT('Ctrl Pts',(-14.1437029646929,-12.4594256106333,
116.859557740007)) ;
#187228=CARTESIAN_POINT('Ctrl Pts',(-14.0698991040459,-12.4594256285176,
116.883788729222)) ;
#187229=CARTESIAN_POINT('Ctrl Pts',(-13.9960952433988,-12.4594256464019,
116.908019718436)) ;
#187230=CARTESIAN_POINT('Ctrl Pts',(-13.9886264163189,-12.3873928287568,
116.885270877365)) ;
#187231=CARTESIAN_POINT('Ctrl Pts',(-13.9811575892389,-12.3153600111117,
116.862522036293)) ;
#187232=CARTESIAN_POINT('Ctrl Pts',(-14.0549614498859,-12.3153599932274,
116.838291047078)) ;
#187233=CARTESIAN_POINT('Ctrl Pts',(-14.128765310533,-12.3153599753431,
116.814060057863)) ;
#187234=CARTESIAN_POINT('Ctrl Pts',(-14.1362341376129,-12.3873927929882,
116.836808898935)) ;
#187235=CARTESIAN_POINT('Ctrl Pts',(-14.0446632556128,-12.5162741275779,
116.593235944571)) ;
#187236=CARTESIAN_POINT('Ctrl Pts',(-14.0578049538713,-12.5794124829248,
116.633263435799)) ;
#187237=CARTESIAN_POINT('Ctrl Pts',(-13.9840010934612,-12.5794125189228,
116.657494425736)) ;
#187238=CARTESIAN_POINT('Ctrl Pts',(-13.9101972330512,-12.5794125549208,
116.681725415673)) ;
#187239=CARTESIAN_POINT('Ctrl Pts',(-13.8970555347928,-12.5162741995739,
116.641697924445)) ;
#187240=CARTESIAN_POINT('Ctrl Pts',(-13.8839138365343,-12.453135844227,
116.601670433216)) ;
#187241=CARTESIAN_POINT('Ctrl Pts',(-13.9577176969443,-12.453135808229,
116.57743944328)) ;
#187242=CARTESIAN_POINT('Ctrl Pts',(-14.0315215573543,-12.453135772231,
116.553208453343)) ;
#187243=CARTESIAN_POINT('Ctrl Pts',(-14.0446632556128,-12.5162741275779,
116.593235944571)) ;
#187244=CARTESIAN_POINT('Ctrl Pts',(-13.9661822867413,-12.7104566542012,
116.389740888653)) ;
#187245=CARTESIAN_POINT('Ctrl Pts',(-13.9840868963541,-12.7601293026598,
116.444275439204)) ;
#187246=CARTESIAN_POINT('Ctrl Pts',(-13.9102830377639,-12.7601293584612,
116.468506434684)) ;
#187247=CARTESIAN_POINT('Ctrl Pts',(-13.8364791791737,-12.7601294142626,
116.492737430164)) ;
#187248=CARTESIAN_POINT('Ctrl Pts',(-13.8185745695609,-12.7104567658041,
116.438202879613)) ;
#187249=CARTESIAN_POINT('Ctrl Pts',(-13.8006699599481,-12.6607841173455,
116.383668329061)) ;
#187250=CARTESIAN_POINT('Ctrl Pts',(-13.8744738185383,-12.6607840615441,
116.359437333582)) ;
#187251=CARTESIAN_POINT('Ctrl Pts',(-13.9482776771285,-12.6607840057427,
116.335206338102)) ;
#187252=CARTESIAN_POINT('Ctrl Pts',(-13.9661822867413,-12.7104566542012,
116.389740888653)) ;
#187253=CARTESIAN_POINT('Ctrl Pts',(-13.9065147105429,-12.9544063196606,
116.243378133493)) ;
#187254=CARTESIAN_POINT('Ctrl Pts',(-13.9278790755324,-12.9871189134417,
116.308450540564)) ;
#187255=CARTESIAN_POINT('Ctrl Pts',(-13.8540752212451,-12.9871189862544,
116.332681549149)) ;
#187256=CARTESIAN_POINT('Ctrl Pts',(-13.7802713669579,-12.987119059067,
116.356912557735)) ;
#187257=CARTESIAN_POINT('Ctrl Pts',(-13.7589070019684,-12.9544064652859,
116.291840150665)) ;
#187258=CARTESIAN_POINT('Ctrl Pts',(-13.737542636979,-12.9216938715048,
116.226767743595)) ;
#187259=CARTESIAN_POINT('Ctrl Pts',(-13.8113464912662,-12.9216937986921,
116.202536735009)) ;
#187260=CARTESIAN_POINT('Ctrl Pts',(-13.8851503455534,-12.9216937258795,
116.178305726423)) ;
#187261=CARTESIAN_POINT('Ctrl Pts',(-13.9065147105429,-12.9544063196606,
116.243378133493)) ;
#187262=CARTESIAN_POINT('Ctrl Pts',(-13.8686602732645,-13.2316631461472,
116.163500825195)) ;
#187263=CARTESIAN_POINT('Ctrl Pts',(-13.8919655852634,-13.2450660236381,
116.23448504356)) ;
#187264=CARTESIAN_POINT('Ctrl Pts',(-13.8181617370342,-13.2450661094682,
116.258716070597)) ;
#187265=CARTESIAN_POINT('Ctrl Pts',(-13.744357888805,-13.2450661952983,
116.282947097635)) ;
#187266=CARTESIAN_POINT('Ctrl Pts',(-13.7210525768062,-13.2316633178074,
116.21196287927)) ;
#187267=CARTESIAN_POINT('Ctrl Pts',(-13.6977472648073,-13.2182604403165,
116.140978660905)) ;
#187268=CARTESIAN_POINT('Ctrl Pts',(-13.7715511130365,-13.2182603544864,
116.116747633868)) ;
#187269=CARTESIAN_POINT('Ctrl Pts',(-13.8453549612656,-13.2182602686563,
116.09251660683)) ;
#187270=CARTESIAN_POINT('Ctrl Pts',(-13.8686602732645,-13.2316631461472,
116.163500825195)) ;
#187271=CARTESIAN_POINT('Ctrl Pts',(-13.854686359136,-13.5226486146427,
116.156402551173)) ;
#187272=CARTESIAN_POINT('Ctrl Pts',(-13.8782674046233,-13.5157554602217,
116.228226609137)) ;
#187273=CARTESIAN_POINT('Ctrl Pts',(-13.8044635638606,-13.5157555531286,
116.252457658916)) ;
#187274=CARTESIAN_POINT('Ctrl Pts',(-13.7306597230979,-13.5157556460354,
116.276688708695)) ;
#187275=CARTESIAN_POINT('Ctrl Pts',(-13.7070786776106,-13.5226488004565,
116.204864650732)) ;
#187276=CARTESIAN_POINT('Ctrl Pts',(-13.6834976321233,-13.5295419548775,
116.133040592768)) ;
#187277=CARTESIAN_POINT('Ctrl Pts',(-13.757301472886,-13.5295418619706,
116.108809542988)) ;
#187278=CARTESIAN_POINT('Ctrl Pts',(-13.8311053136488,-13.5295417690637,
116.084578493209)) ;
#187279=CARTESIAN_POINT('Ctrl Pts',(-13.854686359136,-13.5226486146427,
116.156402551173)) ;
#187280=CARTESIAN_POINT('Ctrl Pts',(-13.8649983319088,-13.8069296281822,
116.223380345266)) ;
#187281=CARTESIAN_POINT('Ctrl Pts',(-13.887157991961,-13.7801790343967,
116.290875092425)) ;
#187282=CARTESIAN_POINT('Ctrl Pts',(-13.8133541594712,-13.7801791269532,
116.315106167402)) ;
#187283=CARTESIAN_POINT('Ctrl Pts',(-13.7395503269813,-13.7801792195097,
116.339337242379)) ;
#187284=CARTESIAN_POINT('Ctrl Pts',(-13.717390666929,-13.8069298132952,
116.27184249522)) ;
#187285=CARTESIAN_POINT('Ctrl Pts',(-13.6952310068767,-13.8336804070807,
116.204347748061)) ;
#187286=CARTESIAN_POINT('Ctrl Pts',(-13.7690348393666,-13.8336803145242,
116.180116673084)) ;
#187287=CARTESIAN_POINT('Ctrl Pts',(-13.8428386718565,-13.8336802219677,
116.155885598107)) ;
#187288=CARTESIAN_POINT('Ctrl Pts',(-13.8649983319088,-13.8069296281822,
116.223380345266)) ;
#187289=CARTESIAN_POINT('Ctrl Pts',(-13.8980327908744,-14.0625497260425,
116.35946810785)) ;
#187290=CARTESIAN_POINT('Ctrl Pts',(-13.917184644522,-14.0179135569207,
116.41780156193)) ;
#187291=CARTESIAN_POINT('Ctrl Pts',(-13.8433808200787,-14.017913640046,
116.442032661416)) ;
#187292=CARTESIAN_POINT('Ctrl Pts',(-13.7695769956354,-14.0179137231712,
116.466263760901)) ;
#187293=CARTESIAN_POINT('Ctrl Pts',(-13.7504251419878,-14.062549892293,
116.407930306821)) ;
#187294=CARTESIAN_POINT('Ctrl Pts',(-13.7312732883402,-14.1071860614148,
116.349596852741)) ;
#187295=CARTESIAN_POINT('Ctrl Pts',(-13.8050771127835,-14.1071859782896,
116.325365753256)) ;
#187296=CARTESIAN_POINT('Ctrl Pts',(-13.8788809372268,-14.1071858951643,
116.30113465377)) ;
#187297=CARTESIAN_POINT('Ctrl Pts',(-13.8980327908744,-14.0625497260425,
116.35946810785)) ;
#187298=CARTESIAN_POINT('Ctrl Pts',(-13.9507026046682,-14.2720262448878,
116.555387635034)) ;
#187299=CARTESIAN_POINT('Ctrl Pts',(-13.9654709590495,-14.2126996245835,
116.600369657567)) ;
#187300=CARTESIAN_POINT('Ctrl Pts',(-13.8916671415546,-14.2126996903488,
116.624600778216)) ;
#187301=CARTESIAN_POINT('Ctrl Pts',(-13.8178633240598,-14.2126997561141,
116.648831898866)) ;
#187302=CARTESIAN_POINT('Ctrl Pts',(-13.8030949696785,-14.2720263764183,
116.603849876333)) ;
#187303=CARTESIAN_POINT('Ctrl Pts',(-13.7883266152972,-14.3313529967226,
116.558867853801)) ;
#187304=CARTESIAN_POINT('Ctrl Pts',(-13.8621304327921,-14.3313529309573,
116.534636733152)) ;
#187305=CARTESIAN_POINT('Ctrl Pts',(-13.9359342502869,-14.331352865192,
116.510405612502)) ;
#187306=CARTESIAN_POINT('Ctrl Pts',(-13.9507026046682,-14.2720262448878,
116.555387635034)) ;
#187307=CARTESIAN_POINT('Ctrl Pts',(-14.0181419135474,-14.4199161330371,
116.796147687548)) ;
#187308=CARTESIAN_POINT('Ctrl Pts',(-14.027492125809,-14.3501772641186,
116.824626923365)) ;
#187309=CARTESIAN_POINT('Ctrl Pts',(-13.9536883133137,-14.3501773061419,
116.848858059242)) ;
#187310=CARTESIAN_POINT('Ctrl Pts',(-13.8798845008185,-14.3501773481651,
116.87308919512)) ;
#187311=CARTESIAN_POINT('Ctrl Pts',(-13.8705342885569,-14.4199162170836,
116.844609959303)) ;
#187312=CARTESIAN_POINT('Ctrl Pts',(-13.8611840762953,-14.489655086002,
116.816130723485)) ;
#187313=CARTESIAN_POINT('Ctrl Pts',(-13.9349878887906,-14.4896550439788,
116.791899587608)) ;
#187314=CARTESIAN_POINT('Ctrl Pts',(-14.0087917012858,-14.4896550019555,
116.767668451731)) ;
#187315=CARTESIAN_POINT('Ctrl Pts',(-14.0181419135474,-14.4199161330371,
116.796147687548)) ;
#187316=CARTESIAN_POINT('Ctrl Pts',(-14.0955313329315,-14.496610258064,
117.067451422001)) ;
#187317=CARTESIAN_POINT('Ctrl Pts',(-14.098756043099,-14.4214134928077,
117.077273366771)) ;
#187318=CARTESIAN_POINT('Ctrl Pts',(-14.0249522332246,-14.4214135069691,
117.101504510631)) ;
#187319=CARTESIAN_POINT('Ctrl Pts',(-13.9511484233502,-14.4214135211306,
117.125735654491)) ;
#187320=CARTESIAN_POINT('Ctrl Pts',(-13.9479237131826,-14.496610286387,
117.115913709721)) ;
#187321=CARTESIAN_POINT('Ctrl Pts',(-13.9446990030151,-14.5718070516433,
117.106091764952)) ;
#187322=CARTESIAN_POINT('Ctrl Pts',(-14.0185028128895,-14.5718070374819,
117.081860621092)) ;
#187323=CARTESIAN_POINT('Ctrl Pts',(-14.0923066227639,-14.5718070233204,
117.057629477232)) ;
#187324=CARTESIAN_POINT('Ctrl Pts',(-14.0955313329315,-14.496610258064,
117.067451422001)) ;
#187325=CARTESIAN_POINT('Ctrl Pts',(-14.1754259823427,-14.4958941579837,
117.3460706369)) ;
#187326=CARTESIAN_POINT('Ctrl Pts',(-14.1723475785296,-14.4206364931476,
117.336694313495)) ;
#187327=CARTESIAN_POINT('Ctrl Pts',(-14.0985437685299,-14.4206364783751,
117.360925456973)) ;
#187328=CARTESIAN_POINT('Ctrl Pts',(-14.0247399585301,-14.4206364636026,
117.385156600451)) ;
#187329=CARTESIAN_POINT('Ctrl Pts',(-14.0278183623432,-14.4958941284387,
117.394532923857)) ;
#187330=CARTESIAN_POINT('Ctrl Pts',(-14.0308967661563,-14.5711517932748,
117.403909247263)) ;
#187331=CARTESIAN_POINT('Ctrl Pts',(-14.104700576156,-14.5711518080473,
117.379678103784)) ;
#187332=CARTESIAN_POINT('Ctrl Pts',(-14.1785043861558,-14.5711518228198,
117.355446960306)) ;
#187333=CARTESIAN_POINT('Ctrl Pts',(-14.1754259823427,-14.4958941579837,
117.3460706369)) ;
#187334=CARTESIAN_POINT('Ctrl Pts',(-14.2526586700799,-14.4180076226564,
117.616872676187)) ;
#187335=CARTESIAN_POINT('Ctrl Pts',(-14.2434477347778,-14.3480754910907,
117.588817651376)) ;
#187336=CARTESIAN_POINT('Ctrl Pts',(-14.1696439218951,-14.3480754488814,
117.613048786073)) ;
#187337=CARTESIAN_POINT('Ctrl Pts',(-14.0958401090124,-14.3480754066721,
117.63727992077)) ;
#187338=CARTESIAN_POINT('Ctrl Pts',(-14.1050510443145,-14.4180075382377,
117.665334945581)) ;
#187339=CARTESIAN_POINT('Ctrl Pts',(-14.1142619796166,-14.4879396698034,
117.693389970392)) ;
#187340=CARTESIAN_POINT('Ctrl Pts',(-14.1880657924993,-14.4879397120127,
117.669158835695)) ;
#187341=CARTESIAN_POINT('Ctrl Pts',(-14.261869605382,-14.4879397542221,
117.644927700998)) ;
#187342=CARTESIAN_POINT('Ctrl Pts',(-14.2526586700799,-14.4180076226564,
117.616872676187)) ;
#187343=CARTESIAN_POINT('Ctrl Pts',(-14.3200614063859,-14.2684543242656,
117.857623246459)) ;
#187344=CARTESIAN_POINT('Ctrl Pts',(-14.3053972971681,-14.2088592298977,
117.812958733819)) ;
#187345=CARTESIAN_POINT('Ctrl Pts',(-14.2315934790337,-14.2088591648377,
117.83718985252)) ;
#187346=CARTESIAN_POINT('Ctrl Pts',(-14.1577896608992,-14.2088590997777,
117.861420971222)) ;
#187347=CARTESIAN_POINT('Ctrl Pts',(-14.172453770117,-14.2684541941456,
117.906085483862)) ;
#187348=CARTESIAN_POINT('Ctrl Pts',(-14.1871178793347,-14.3280492885136,
117.950749996502)) ;
#187349=CARTESIAN_POINT('Ctrl Pts',(-14.2609216974692,-14.3280493535736,
117.926518877801)) ;
#187350=CARTESIAN_POINT('Ctrl Pts',(-14.3347255156036,-14.3280494186336,
117.902287759099)) ;
#187351=CARTESIAN_POINT('Ctrl Pts',(-14.3200614063859,-14.2684543242656,
117.857623246459)) ;
#187352=CARTESIAN_POINT('Ctrl Pts',(-14.3723441508749,-14.0580103363769,
118.052339972716)) ;
#187353=CARTESIAN_POINT('Ctrl Pts',(-14.3532738878019,-14.0130186488343,
117.994255026436)) ;
#187354=CARTESIAN_POINT('Ctrl Pts',(-14.2794700626734,-14.0130185675702,
118.018486123834)) ;
#187355=CARTESIAN_POINT('Ctrl Pts',(-14.2056662375449,-14.013018486306,
118.042717221233)) ;
#187356=CARTESIAN_POINT('Ctrl Pts',(-14.2247365006178,-14.0580101738486,
118.100802167514)) ;
#187357=CARTESIAN_POINT('Ctrl Pts',(-14.2438067636907,-14.1030018613912,
118.158887113794)) ;
#187358=CARTESIAN_POINT('Ctrl Pts',(-14.3176105888193,-14.1030019426553,
118.134656016396)) ;
#187359=CARTESIAN_POINT('Ctrl Pts',(-14.3914144139478,-14.1030020239195,
118.110424918997)) ;
#187360=CARTESIAN_POINT('Ctrl Pts',(-14.3723441508749,-14.0580103363769,
118.052339972716)) ;
#187361=CARTESIAN_POINT('Ctrl Pts',(-14.4049559952129,-13.8017355758307,
118.187134007754)) ;
#187362=CARTESIAN_POINT('Ctrl Pts',(-14.3828464247468,-13.7745688567898,
118.119791821635)) ;
#187363=CARTESIAN_POINT('Ctrl Pts',(-14.3090425916919,-13.7745687672832,
118.144022894892)) ;
#187364=CARTESIAN_POINT('Ctrl Pts',(-14.2352387586371,-13.7745686777767,
118.168253968148)) ;
#187365=CARTESIAN_POINT('Ctrl Pts',(-14.2573483291032,-13.8017353968177,
118.235596154267)) ;
#187366=CARTESIAN_POINT('Ctrl Pts',(-14.2794578995694,-13.8289021158586,
118.302938340385)) ;
#187367=CARTESIAN_POINT('Ctrl Pts',(-14.3532617326242,-13.8289022053652,
118.278707267129)) ;
#187368=CARTESIAN_POINT('Ctrl Pts',(-14.4270655656791,-13.8289022948717,
118.254476193873)) ;
#187369=CARTESIAN_POINT('Ctrl Pts',(-14.4049559952129,-13.8017355758307,
118.187134007754)) ;
#187370=CARTESIAN_POINT('Ctrl Pts',(-14.4148166276004,-13.5177911289146,
118.252654045157)) ;
#187371=CARTESIAN_POINT('Ctrl Pts',(-14.3912510399415,-13.5104079472705,
118.180877065709)) ;
#187372=CARTESIAN_POINT('Ctrl Pts',(-14.3174471989152,-13.5104078579673,
118.205108114686)) ;
#187373=CARTESIAN_POINT('Ctrl Pts',(-14.2436433578889,-13.5104077686641,
118.229339163662)) ;
#187374=CARTESIAN_POINT('Ctrl Pts',(-14.2672089455478,-13.5177909503083,
118.30111614311)) ;
#187375=CARTESIAN_POINT('Ctrl Pts',(-14.2907745332067,-13.5251741319524,
118.372893122558)) ;
#187376=CARTESIAN_POINT('Ctrl Pts',(-14.364578374233,-13.5251742212556,
118.348662073581)) ;
#187377=CARTESIAN_POINT('Ctrl Pts',(-14.4383822152593,-13.5251743105588,
118.324431024605)) ;
#187378=CARTESIAN_POINT('Ctrl Pts',(-14.4148166276004,-13.5177911289146,
118.252654045157)) ;
#187379=CARTESIAN_POINT('Ctrl Pts',(-14.4004650952962,-13.2272027816916,
118.244367863608)) ;
#187380=CARTESIAN_POINT('Ctrl Pts',(-14.3771329630221,-13.2400970018567,
118.173301951716)) ;
#187381=CARTESIAN_POINT('Ctrl Pts',(-14.3033291148763,-13.2400969198801,
118.197532979008)) ;
#187382=CARTESIAN_POINT('Ctrl Pts',(-14.2295252667306,-13.2400968379035,
118.2217640063)) ;
#187383=CARTESIAN_POINT('Ctrl Pts',(-14.2528573990047,-13.2272026177384,
118.292829918192)) ;
#187384=CARTESIAN_POINT('Ctrl Pts',(-14.2761895312788,-13.2143083975732,
118.363895830085)) ;
#187385=CARTESIAN_POINT('Ctrl Pts',(-14.3499933794246,-13.2143084795498,
118.339664802793)) ;
#187386=CARTESIAN_POINT('Ctrl Pts',(-14.4237972275703,-13.2143085615265,
118.315433775501)) ;
#187387=CARTESIAN_POINT('Ctrl Pts',(-14.4004650952962,-13.2272027816916,
118.244367863608)) ;
#187388=CARTESIAN_POINT('Ctrl Pts',(-14.3623212862769,-12.9503466746931,
118.163591806745)) ;
#187389=CARTESIAN_POINT('Ctrl Pts',(-14.3408845358734,-12.9825901613467,
118.098298922341)) ;
#187390=CARTESIAN_POINT('Ctrl Pts',(-14.267080681969,-12.9825900924411,
118.122529932092)) ;
#187391=CARTESIAN_POINT('Ctrl Pts',(-14.1932768280645,-12.9825900235354,
118.146760941844)) ;
#187392=CARTESIAN_POINT('Ctrl Pts',(-14.214713578468,-12.9503465368818,
118.212053826248)) ;
#187393=CARTESIAN_POINT('Ctrl Pts',(-14.2361503288715,-12.9181030502282,
118.277346710652)) ;
#187394=CARTESIAN_POINT('Ctrl Pts',(-14.3099541827759,-12.9181031191338,
118.253115700901)) ;
#187395=CARTESIAN_POINT('Ctrl Pts',(-14.3837580366804,-12.9181031880395,
118.228884691149)) ;
#187396=CARTESIAN_POINT('Ctrl Pts',(-14.3623212862769,-12.9503466746931,
118.163591806745)) ;
#187397=CARTESIAN_POINT('Ctrl Pts',(-14.3018636593907,-12.7057179827167,
118.015049850158)) ;
#187398=CARTESIAN_POINT('Ctrl Pts',(-14.283878771003,-12.7550903667589,
117.960270780674)) ;
#187399=CARTESIAN_POINT('Ctrl Pts',(-14.2100749136123,-12.7550903161595,
117.984501779807)) ;
#187400=CARTESIAN_POINT('Ctrl Pts',(-14.1362710562215,-12.7550902655601,
118.00873277894)) ;
#187401=CARTESIAN_POINT('Ctrl Pts',(-14.1542559446093,-12.7057178815179,
118.063511848424)) ;
#187402=CARTESIAN_POINT('Ctrl Pts',(-14.172240832997,-12.6563454974757,
118.118290917909)) ;
#187403=CARTESIAN_POINT('Ctrl Pts',(-14.2460446903878,-12.6563455480751,
118.094059918775)) ;
#187404=CARTESIAN_POINT('Ctrl Pts',(-14.3198485477785,-12.6563455986745,
118.069828919642)) ;
#187405=CARTESIAN_POINT('Ctrl Pts',(-14.3018636593907,-12.7057179827167,
118.015049850158)) ;
#187406=CARTESIAN_POINT('Ctrl Pts',(-14.223542409614,-12.5137879422887,
117.811825999988)) ;
#187407=CARTESIAN_POINT('Ctrl Pts',(-14.2102677240736,-12.5766355535095,
117.771393448525)) ;
#187408=CARTESIAN_POINT('Ctrl Pts',(-14.1364638648589,-12.5766355204259,
117.795624442103)) ;
#187409=CARTESIAN_POINT('Ctrl Pts',(-14.0626600056441,-12.5766354873422,
117.81985543568)) ;
#187410=CARTESIAN_POINT('Ctrl Pts',(-14.0759346911844,-12.5137878761215,
117.860287987143)) ;
#187411=CARTESIAN_POINT('Ctrl Pts',(-14.0892093767248,-12.4509402649008,
117.900720538606)) ;
#187412=CARTESIAN_POINT('Ctrl Pts',(-14.1630132359396,-12.4509402979844,
117.876489545029)) ;
#187413=CARTESIAN_POINT('Ctrl Pts',(-14.2368170951544,-12.450940331068,
117.852258551451)) ;
#187414=CARTESIAN_POINT('Ctrl Pts',(-14.223542409614,-12.5137879422887,
117.811825999988)) ;
#187415=CARTESIAN_POINT('Ctrl Pts',(-14.1314433751478,-12.3855428728414,
117.56678537301)) ;
#187416=CARTESIAN_POINT('Ctrl Pts',(-14.1238448332789,-12.4574400165938,
117.543641439496)) ;
#187417=CARTESIAN_POINT('Ctrl Pts',(-14.0500409744482,-12.4574400010847,
117.567872434243)) ;
#187418=CARTESIAN_POINT('Ctrl Pts',(-13.9762371156176,-12.4574399855756,
117.592103428991)) ;
#187419=CARTESIAN_POINT('Ctrl Pts',(-13.9838356574865,-12.3855428418231,
117.615247362505)) ;
#187420=CARTESIAN_POINT('Ctrl Pts',(-13.9914341993555,-12.3136456980707,
117.638391296019)) ;
#187421=CARTESIAN_POINT('Ctrl Pts',(-14.0652380581861,-12.3136457135799,
117.614160301271)) ;
#187422=CARTESIAN_POINT('Ctrl Pts',(-14.1390419170168,-12.313645729089,
117.589929306524)) ;
#187423=CARTESIAN_POINT('Ctrl Pts',(-14.1314433751478,-12.3855428728414,
117.56678537301)) ;
#187424=CARTESIAN_POINT('Ctrl Pts',(-14.031461000016,-12.3315373856839,
117.297796004923)) ;
#187425=CARTESIAN_POINT('Ctrl Pts',(-14.0300964367554,-12.4073146251765,
117.293639764585)) ;
#187426=CARTESIAN_POINT('Ctrl Pts',(-13.9562925801431,-12.4073146237206,
117.317870766089)) ;
#187427=CARTESIAN_POINT('Ctrl Pts',(-13.8824887235308,-12.4073146222647,
117.342101767593)) ;
#187428=CARTESIAN_POINT('Ctrl Pts',(-13.8838532867914,-12.331537382772,
117.346258007932)) ;
#187429=CARTESIAN_POINT('Ctrl Pts',(-13.885217850052,-12.2557601432794,
117.35041424827)) ;
#187430=CARTESIAN_POINT('Ctrl Pts',(-13.9590217066643,-12.2557601447353,
117.326183246766)) ;
#187431=CARTESIAN_POINT('Ctrl Pts',(-14.0328255632766,-12.2557601461912,
117.301952245262)) ;
#187432=CARTESIAN_POINT('Ctrl Pts',(-14.031461000016,-12.3315373856839,
117.297796004923)) ;
#187433=CARTESIAN_POINT('Ctrl Pts',(-13.930645096914,-12.3551820249381,
117.026108320911)) ;
#187434=CARTESIAN_POINT('Ctrl Pts',(-13.9355855082574,-12.4294230563163,
117.041156016064)) ;
#187435=CARTESIAN_POINT('Ctrl Pts',(-13.8617816544059,-12.4294230645316,
117.065387025977)) ;
#187436=CARTESIAN_POINT('Ctrl Pts',(-13.7879778005545,-12.4294230727469,
117.08961803589)) ;
#187437=CARTESIAN_POINT('Ctrl Pts',(-13.7830373892111,-12.3551820413687,
117.074570340737)) ;
#187438=CARTESIAN_POINT('Ctrl Pts',(-13.7780969778677,-12.2809410099905,
117.059522645584)) ;
#187439=CARTESIAN_POINT('Ctrl Pts',(-13.8519008317191,-12.2809410017752,
117.035291635671)) ;
#187440=CARTESIAN_POINT('Ctrl Pts',(-13.9257046855706,-12.2809409935599,
117.011060625758)) ;
#187441=CARTESIAN_POINT('Ctrl Pts',(-13.930645096914,-12.3551820249381,
117.026108320911)) ;
#187442=CARTESIAN_POINT('Ctrl Pts',(-13.8342954331795,-12.4558831035982,
116.768314309388)) ;
#187443=CARTESIAN_POINT('Ctrl Pts',(-13.8452327466786,-12.5232058909048,
116.801627601108)) ;
#187444=CARTESIAN_POINT('Ctrl Pts',(-13.7714288966798,-12.52320590289,116.825858622756)) ;
#187445=CARTESIAN_POINT('Ctrl Pts',(-13.6976250466809,-12.5232059148753,
116.850089644404)) ;
#187446=CARTESIAN_POINT('Ctrl Pts',(-13.6866877331818,-12.4558831275687,
116.816776352684)) ;
#187447=CARTESIAN_POINT('Ctrl Pts',(-13.6757504196827,-12.3885603402622,
116.783463060963)) ;
#187448=CARTESIAN_POINT('Ctrl Pts',(-13.7495542696815,-12.3885603282769,
116.759232039315)) ;
#187449=CARTESIAN_POINT('Ctrl Pts',(-13.8233581196804,-12.3885603162917,
116.735001017668)) ;
#187450=CARTESIAN_POINT('Ctrl Pts',(-13.8342954331795,-12.4558831035982,
116.768314309388)) ;
#187451=CARTESIAN_POINT('Ctrl Pts',(-13.7502969996175,-12.6240117159259,
116.547732522456)) ;
#187452=CARTESIAN_POINT('Ctrl Pts',(-13.7663861121361,-12.6796964809936,
116.596737362866)) ;
#187453=CARTESIAN_POINT('Ctrl Pts',(-13.6925822646977,-12.6796964939069,
116.620968392312)) ;
#187454=CARTESIAN_POINT('Ctrl Pts',(-13.6187784172594,-12.6796965068202,
116.645199421759)) ;
#187455=CARTESIAN_POINT('Ctrl Pts',(-13.6026893047407,-12.6240117417526,
116.596194581349)) ;
#187456=CARTESIAN_POINT('Ctrl Pts',(-13.5866001922221,-12.568326976685,
116.547189740939)) ;
#187457=CARTESIAN_POINT('Ctrl Pts',(-13.6604040396604,-12.5683269637716,
116.522958711493)) ;
#187458=CARTESIAN_POINT('Ctrl Pts',(-13.7342078870988,-12.5683269508583,
116.498727682046)) ;
#187459=CARTESIAN_POINT('Ctrl Pts',(-13.7502969996175,-12.6240117159259,
116.547732522456)) ;
#187460=CARTESIAN_POINT('Ctrl Pts',(-13.6822000856196,-12.8504012275685,
116.375896123701)) ;
#187461=CARTESIAN_POINT('Ctrl Pts',(-13.7023322685498,-12.8903625364955,
116.43721550439)) ;
#187462=CARTESIAN_POINT('Ctrl Pts',(-13.6285284236176,-12.8903625457094,
116.46144654147)) ;
#187463=CARTESIAN_POINT('Ctrl Pts',(-13.5547245786854,-12.8903625549234,
116.48567757855)) ;
#187464=CARTESIAN_POINT('Ctrl Pts',(-13.5345923957552,-12.8504012459964,
116.424358197861)) ;
#187465=CARTESIAN_POINT('Ctrl Pts',(-13.5144602128251,-12.8104399370694,
116.363038817172)) ;
#187466=CARTESIAN_POINT('Ctrl Pts',(-13.5882640577573,-12.8104399278554,
116.338807780093)) ;
#187467=CARTESIAN_POINT('Ctrl Pts',(-13.6620679026895,-12.8104399186415,
116.314576743013)) ;
#187468=CARTESIAN_POINT('Ctrl Pts',(-13.6822000856196,-12.8504012275685,
116.375896123701)) ;
#187469=CARTESIAN_POINT('Ctrl Pts',(-13.6351866805831,-13.116472804272,
116.268099937279)) ;
#187470=CARTESIAN_POINT('Ctrl Pts',(-13.6578993214573,-13.1379154690077,
116.337278976615)) ;
#187471=CARTESIAN_POINT('Ctrl Pts',(-13.5840954777456,-13.1379154738939,
116.361510017412)) ;
#187472=CARTESIAN_POINT('Ctrl Pts',(-13.5102916340338,-13.13791547878,116.385741058209)) ;
#187473=CARTESIAN_POINT('Ctrl Pts',(-13.4875789931596,-13.1164728140443,
116.316562018874)) ;
#187474=CARTESIAN_POINT('Ctrl Pts',(-13.4648663522853,-13.0950301493086,
116.247382979538)) ;
#187475=CARTESIAN_POINT('Ctrl Pts',(-13.5386701959971,-13.0950301444224,
116.223151938741)) ;
#187476=CARTESIAN_POINT('Ctrl Pts',(-13.6124740397088,-13.0950301395363,
116.198920897944)) ;
#187477=CARTESIAN_POINT('Ctrl Pts',(-13.6351866805831,-13.116472804272,
116.268099937279)) ;
#187478=CARTESIAN_POINT('Ctrl Pts',(-13.6114099106661,-13.4044926459014,
116.231144735483)) ;
#187479=CARTESIAN_POINT('Ctrl Pts',(-13.635082944032,-13.4058558527326,
116.303248975477)) ;
#187480=CARTESIAN_POINT('Ctrl Pts',(-13.5612791007297,-13.4058558531923,
116.327480017521)) ;
#187481=CARTESIAN_POINT('Ctrl Pts',(-13.4874752574274,-13.405855853652,
116.351711059566)) ;
#187482=CARTESIAN_POINT('Ctrl Pts',(-13.4638022240615,-13.4044926468209,
116.279606819572)) ;
#187483=CARTESIAN_POINT('Ctrl Pts',(-13.4401291906957,-13.4031294399897,
116.207502579578)) ;
#187484=CARTESIAN_POINT('Ctrl Pts',(-13.513933033998,-13.40312943953,116.183271537533)) ;
#187485=CARTESIAN_POINT('Ctrl Pts',(-13.5877368773003,-13.4031294390702,
116.159040495489)) ;
#187486=CARTESIAN_POINT('Ctrl Pts',(-13.6114099106661,-13.4044926459014,
116.231144735483)) ;
#187487=CARTESIAN_POINT('Ctrl Pts',(-13.6118756694188,-13.6930971947521,
116.26796761554)) ;
#187488=CARTESIAN_POINT('Ctrl Pts',(-13.6348188255478,-13.6743099521877,
116.337848767292)) ;
#187489=CARTESIAN_POINT('Ctrl Pts',(-13.5610149819962,-13.6743099497306,
116.362079808577)) ;
#187490=CARTESIAN_POINT('Ctrl Pts',(-13.4872111384447,-13.6743099472734,
116.386310849862)) ;
#187491=CARTESIAN_POINT('Ctrl Pts',(-13.4642679823157,-13.6930971898379,
116.31642969811)) ;
#187492=CARTESIAN_POINT('Ctrl Pts',(-13.4413248261868,-13.7118844324023,
116.246548546358)) ;
#187493=CARTESIAN_POINT('Ctrl Pts',(-13.5151286697383,-13.7118844348594,
116.222317505073)) ;
#187494=CARTESIAN_POINT('Ctrl Pts',(-13.5889325132899,-13.7118844373166,
116.198086463788)) ;
#187495=CARTESIAN_POINT('Ctrl Pts',(-13.6118756694188,-13.6930971947521,
116.26796761554)) ;
#187496=CARTESIAN_POINT('Ctrl Pts',(-13.63611364525,-13.9640294815732,116.37748207908)) ;
#187497=CARTESIAN_POINT('Ctrl Pts',(-13.6566598449573,-13.9262943650166,
116.440062488337)) ;
#187498=CARTESIAN_POINT('Ctrl Pts',(-13.5828560010043,-13.9262943620916,
116.464293528399)) ;
#187499=CARTESIAN_POINT('Ctrl Pts',(-13.5090521570513,-13.9262943591665,
116.488524568462)) ;
#187500=CARTESIAN_POINT('Ctrl Pts',(-13.4885059573441,-13.9640294757231,
116.425944159205)) ;
#187501=CARTESIAN_POINT('Ctrl Pts',(-13.4679597576368,-14.0017645922797,
116.363363749948)) ;
#187502=CARTESIAN_POINT('Ctrl Pts',(-13.5417636015898,-14.0017645952047,
116.339132709885)) ;
#187503=CARTESIAN_POINT('Ctrl Pts',(-13.6155674455427,-14.0017645981297,
116.314901669823)) ;
#187504=CARTESIAN_POINT('Ctrl Pts',(-13.63611364525,-13.9640294815732,116.37748207908)) ;
#187505=CARTESIAN_POINT('Ctrl Pts',(-13.6811255061301,-14.1931760928296,
116.549907692602)) ;
#187506=CARTESIAN_POINT('Ctrl Pts',(-13.6978277312129,-14.1393849019779,
116.600779975346)) ;
#187507=CARTESIAN_POINT('Ctrl Pts',(-13.6240238873508,-14.1393849008332,
116.625011015685)) ;
#187508=CARTESIAN_POINT('Ctrl Pts',(-13.5502200434887,-14.1393848996885,
116.649242056024)) ;
#187509=CARTESIAN_POINT('Ctrl Pts',(-13.533517818406,-14.1931760905402,
116.598369773281)) ;
#187510=CARTESIAN_POINT('Ctrl Pts',(-13.5168155933232,-14.2469672813919,
116.547497490537)) ;
#187511=CARTESIAN_POINT('Ctrl Pts',(-13.5906194371853,-14.2469672825366,
116.523266450198)) ;
#187512=CARTESIAN_POINT('Ctrl Pts',(-13.6644232810473,-14.2469672836813,
116.499035409859)) ;
#187513=CARTESIAN_POINT('Ctrl Pts',(-13.6811255061301,-14.1931760928296,
116.549907692602)) ;
#187514=CARTESIAN_POINT('Ctrl Pts',(-13.7431234444794,-14.3676938142289,
116.774142291284)) ;
#187515=CARTESIAN_POINT('Ctrl Pts',(-13.7547884992663,-14.3016378950291,
116.809672165995)) ;
#187516=CARTESIAN_POINT('Ctrl Pts',(-13.6809846560937,-14.3016378958559,
116.833903208434)) ;
#187517=CARTESIAN_POINT('Ctrl Pts',(-13.6071808129211,-14.3016378966827,
116.858134250874)) ;
#187518=CARTESIAN_POINT('Ctrl Pts',(-13.5955157581342,-14.3676938158825,
116.822604376163)) ;
#187519=CARTESIAN_POINT('Ctrl Pts',(-13.5838507033473,-14.4337497350823,
116.787074501452)) ;
#187520=CARTESIAN_POINT('Ctrl Pts',(-13.6576545465199,-14.4337497342555,
116.762843459013)) ;
#187521=CARTESIAN_POINT('Ctrl Pts',(-13.7314583896924,-14.4337497334287,
116.738612416573)) ;
#187522=CARTESIAN_POINT('Ctrl Pts',(-13.7431234444794,-14.3676938142289,
116.774142291284)) ;
#187523=CARTESIAN_POINT('Ctrl Pts',(-13.8171763031359,-14.4745465378171,
117.0351873098)) ;
#187524=CARTESIAN_POINT('Ctrl Pts',(-13.8229531340849,-14.4009329542059,
117.052782604666)) ;
#187525=CARTESIAN_POINT('Ctrl Pts',(-13.7491492924703,-14.4009329561401,
117.077013651851)) ;
#187526=CARTESIAN_POINT('Ctrl Pts',(-13.6753454508558,-14.4009329580743,
117.101244699035)) ;
#187527=CARTESIAN_POINT('Ctrl Pts',(-13.6695686199067,-14.4745465416855,
117.08364940417)) ;
#187528=CARTESIAN_POINT('Ctrl Pts',(-13.6637917889576,-14.5481601252968,
117.066054109305)) ;
#187529=CARTESIAN_POINT('Ctrl Pts',(-13.7375956305722,-14.5481601233625,
117.04182306212)) ;
#187530=CARTESIAN_POINT('Ctrl Pts',(-13.8113994721868,-14.5481601214283,
117.017592014935)) ;
#187531=CARTESIAN_POINT('Ctrl Pts',(-13.8171763031359,-14.4745465378171,
117.0351873098)) ;
#187532=CARTESIAN_POINT('Ctrl Pts',(-13.8970345888385,-14.5056303399819,
117.313909070973)) ;
#187533=CARTESIAN_POINT('Ctrl Pts',(-13.8965094386652,-14.4297391365026,
117.312309548038)) ;
#187534=CARTESIAN_POINT('Ctrl Pts',(-13.8227055991251,-14.4297391368143,
117.336540601542)) ;
#187535=CARTESIAN_POINT('Ctrl Pts',(-13.748901759585,-14.429739137126,117.360771655045)) ;
#187536=CARTESIAN_POINT('Ctrl Pts',(-13.7494269097583,-14.5056303406052,
117.36237117798)) ;
#187537=CARTESIAN_POINT('Ctrl Pts',(-13.7499520599316,-14.5815215440845,
117.363970700914)) ;
#187538=CARTESIAN_POINT('Ctrl Pts',(-13.8237558994717,-14.5815215437728,
117.339739647411)) ;
#187539=CARTESIAN_POINT('Ctrl Pts',(-13.8975597390118,-14.5815215434611,
117.315508593907)) ;
#187540=CARTESIAN_POINT('Ctrl Pts',(-13.8970345888385,-14.5056303399819,
117.313909070973)) ;
#187541=CARTESIAN_POINT('Ctrl Pts',(-13.9762710886277,-14.4584990503317,
117.590768049018)) ;
#187542=CARTESIAN_POINT('Ctrl Pts',(-13.9694776476947,-14.3857884203973,
117.570076323666)) ;
#187543=CARTESIAN_POINT('Ctrl Pts',(-13.8956738103242,-14.3857884151158,
117.594307383777)) ;
#187544=CARTESIAN_POINT('Ctrl Pts',(-13.8218699729536,-14.3857884098344,
117.618538443888)) ;
#187545=CARTESIAN_POINT('Ctrl Pts',(-13.8286634138866,-14.4584990397688,
117.639230169241)) ;
#187546=CARTESIAN_POINT('Ctrl Pts',(-13.8354568548196,-14.5312096697032,
117.659921894593)) ;
#187547=CARTESIAN_POINT('Ctrl Pts',(-13.9092606921902,-14.5312096749846,
117.635690834482)) ;
#187548=CARTESIAN_POINT('Ctrl Pts',(-13.9830645295607,-14.5312096802661,
117.61145977437)) ;
#187549=CARTESIAN_POINT('Ctrl Pts',(-13.9762710886277,-14.4584990503317,
117.590768049018)) ;
#187550=CARTESIAN_POINT('Ctrl Pts',(-14.0480660570399,-14.3375927241235,
117.844776644025)) ;
#187551=CARTESIAN_POINT('Ctrl Pts',(-14.0355188680038,-14.2732190066455,
117.806559930184)) ;
#187552=CARTESIAN_POINT('Ctrl Pts',(-13.961715031784,-14.2732189929484,
117.830790993801)) ;
#187553=CARTESIAN_POINT('Ctrl Pts',(-13.8879111955643,-14.2732189792513,
117.855022057418)) ;
#187554=CARTESIAN_POINT('Ctrl Pts',(-13.9004583846004,-14.3375926967294,
117.893238771258)) ;
#187555=CARTESIAN_POINT('Ctrl Pts',(-13.9130055736365,-14.4019664142074,
117.931455485098)) ;
#187556=CARTESIAN_POINT('Ctrl Pts',(-13.9868094098562,-14.4019664279045,
117.907224421482)) ;
#187557=CARTESIAN_POINT('Ctrl Pts',(-14.060613246076,-14.4019664416016,
117.882993357865)) ;
#187558=CARTESIAN_POINT('Ctrl Pts',(-14.0480660570399,-14.3375927241235,
117.844776644025)) ;
#187559=CARTESIAN_POINT('Ctrl Pts',(-14.1074172507216,-14.1494056626898,
118.061195966656)) ;
#187560=CARTESIAN_POINT('Ctrl Pts',(-14.0899702434343,-14.0980778114582,
118.008055196809)) ;
#187561=CARTESIAN_POINT('Ctrl Pts',(-14.0161664079691,-14.0980777847103,
118.032286262724)) ;
#187562=CARTESIAN_POINT('Ctrl Pts',(-13.942362572504,-14.0980777579623,
118.056517328639)) ;
#187563=CARTESIAN_POINT('Ctrl Pts',(-13.9598095797914,-14.1494056091939,
118.109658098486)) ;
#187564=CARTESIAN_POINT('Ctrl Pts',(-13.9772565870787,-14.2007334604254,
118.162798868333)) ;
#187565=CARTESIAN_POINT('Ctrl Pts',(-14.0510604225438,-14.2007334871734,
118.138567802417)) ;
#187566=CARTESIAN_POINT('Ctrl Pts',(-14.1248642580089,-14.2007335139213,
118.114336736502)) ;
#187567=CARTESIAN_POINT('Ctrl Pts',(-14.1074172507216,-14.1494056626898,
118.061195966656)) ;
#187568=CARTESIAN_POINT('Ctrl Pts',(-14.1483544481985,-13.9095500364901,
118.221334237361)) ;
#187569=CARTESIAN_POINT('Ctrl Pts',(-14.1272904544691,-13.8748947454948,
118.157176710245)) ;
#187570=CARTESIAN_POINT('Ctrl Pts',(-14.0534866176551,-13.874894705204,
118.181407772051)) ;
#187571=CARTESIAN_POINT('Ctrl Pts',(-13.9796827808411,-13.8748946649131,
118.205638833858)) ;
#187572=CARTESIAN_POINT('Ctrl Pts',(-14.0007467745705,-13.9095499559084,
118.269796360974)) ;
#187573=CARTESIAN_POINT('Ctrl Pts',(-14.0218107682998,-13.9442052469036,
118.33395388809)) ;
#187574=CARTESIAN_POINT('Ctrl Pts',(-14.0956146051138,-13.9442052871945,
118.309722826283)) ;
#187575=CARTESIAN_POINT('Ctrl Pts',(-14.1694184419278,-13.9442053274854,
118.285491764477)) ;
#187576=CARTESIAN_POINT('Ctrl Pts',(-14.1483544481985,-13.9095500364901,
118.221334237361)) ;
#187577=CARTESIAN_POINT('Ctrl Pts',(-14.1676613767387,-13.6354015229083,
118.315498195854)) ;
#187578=CARTESIAN_POINT('Ctrl Pts',(-14.1444874123487,-13.6198370471349,
118.2449140384)) ;
#187579=CARTESIAN_POINT('Ctrl Pts',(-14.0706835724671,-13.6198369951942,
118.269145090864)) ;
#187580=CARTESIAN_POINT('Ctrl Pts',(-13.9968797325854,-13.6198369432535,
118.293376143327)) ;
#187581=CARTESIAN_POINT('Ctrl Pts',(-14.0200536969754,-13.6354014190268,
118.36396030078)) ;
#187582=CARTESIAN_POINT('Ctrl Pts',(-14.0432276613653,-13.6509658948002,
118.434544458234)) ;
#187583=CARTESIAN_POINT('Ctrl Pts',(-14.117031501247,-13.6509659467409,
118.410313405771)) ;
#187584=CARTESIAN_POINT('Ctrl Pts',(-14.1908353411286,-13.6509659986816,
118.386082353308)) ;
#187585=CARTESIAN_POINT('Ctrl Pts',(-14.1676613767387,-13.6354015229083,
118.315498195854)) ;
#187586=CARTESIAN_POINT('Ctrl Pts',(-14.1632252950628,-13.3449945339553,
118.337440153608)) ;
#187587=CARTESIAN_POINT('Ctrl Pts',(-14.1395939545181,-13.3496833242157,
118.265462902021)) ;
#187588=CARTESIAN_POINT('Ctrl Pts',(-14.0657901100262,-13.3496832627429,
118.289693940442)) ;
#187589=CARTESIAN_POINT('Ctrl Pts',(-13.9919862655343,-13.3496832012701,
118.313924978863)) ;
#187590=CARTESIAN_POINT('Ctrl Pts',(-14.015617606079,-13.3449944110097,
118.38590223045)) ;
#187591=CARTESIAN_POINT('Ctrl Pts',(-14.0392489466237,-13.3403056207493,
118.457879482037)) ;
#187592=CARTESIAN_POINT('Ctrl Pts',(-14.1130527911156,-13.3403056822221,
118.433648443616)) ;
#187593=CARTESIAN_POINT('Ctrl Pts',(-14.1868566356075,-13.3403057436949,
118.409417405195)) ;
#187594=CARTESIAN_POINT('Ctrl Pts',(-14.1632252950628,-13.3449945339553,
118.337440153608)) ;
#187595=CARTESIAN_POINT('Ctrl Pts',(-14.1346590237781,-13.0600685836045,
118.285838693899)) ;
#187596=CARTESIAN_POINT('Ctrl Pts',(-14.1122553485649,-13.0846570049903,
118.217600712678)) ;
#187597=CARTESIAN_POINT('Ctrl Pts',(-14.0384514982716,-13.0846569392068,
118.241831733429)) ;
#187598=CARTESIAN_POINT('Ctrl Pts',(-13.9646476479783,-13.0846568734233,
118.26606275418)) ;
#187599=CARTESIAN_POINT('Ctrl Pts',(-13.9870513231916,-13.0600684520375,
118.3343007354)) ;
#187600=CARTESIAN_POINT('Ctrl Pts',(-14.0094549984048,-13.0354800306517,
118.402538716621)) ;
#187601=CARTESIAN_POINT('Ctrl Pts',(-14.0832588486981,-13.0354800964351,
118.37830769587)) ;
#187602=CARTESIAN_POINT('Ctrl Pts',(-14.1570626989914,-13.0354801622186,
118.354076675119)) ;
#187603=CARTESIAN_POINT('Ctrl Pts',(-14.1346590237781,-13.0600685836045,
118.285838693899)) ;
#187604=CARTESIAN_POINT('Ctrl Pts',(-14.0826035780406,-12.7987719757991,
118.162997434216)) ;
#187605=CARTESIAN_POINT('Ctrl Pts',(-14.0630626393208,-12.8416392533606,
118.103478886264)) ;
#187606=CARTESIAN_POINT('Ctrl Pts',(-13.9892587820211,-12.8416391878999,
118.127709885675)) ;
#187607=CARTESIAN_POINT('Ctrl Pts',(-13.9154549247215,-12.8416391224392,
118.151940885086)) ;
#187608=CARTESIAN_POINT('Ctrl Pts',(-13.9349958634413,-12.7987718448777,
118.211459433038)) ;
#187609=CARTESIAN_POINT('Ctrl Pts',(-13.9545368021612,-12.7559045673161,
118.27097798099)) ;
#187610=CARTESIAN_POINT('Ctrl Pts',(-14.0283406594608,-12.7559046327768,
118.246746981579)) ;
#187611=CARTESIAN_POINT('Ctrl Pts',(-14.1021445167604,-12.7559046982375,
118.222515982169)) ;
#187612=CARTESIAN_POINT('Ctrl Pts',(-14.0826035780406,-12.7987719757991,
118.162997434216)) ;
#187613=CARTESIAN_POINT('Ctrl Pts',(-14.0113057802947,-12.5848307790968,
117.981092726393)) ;
#187614=CARTESIAN_POINT('Ctrl Pts',(-13.9959849291863,-12.6426967262578,
117.934427884294)) ;
#187615=CARTESIAN_POINT('Ctrl Pts',(-13.9221810656705,-12.6426966715405,
117.958658864771)) ;
#187616=CARTESIAN_POINT('Ctrl Pts',(-13.8483772021547,-12.6426966168232,
117.982889845248)) ;
#187617=CARTESIAN_POINT('Ctrl Pts',(-13.863698053263,-12.5848306696622,
118.029554687347)) ;
#187618=CARTESIAN_POINT('Ctrl Pts',(-13.8790189043714,-12.5269647225012,
118.076219529447)) ;
#187619=CARTESIAN_POINT('Ctrl Pts',(-13.9528227678873,-12.5269647772185,
118.05198854897)) ;
#187620=CARTESIAN_POINT('Ctrl Pts',(-14.0266266314031,-12.5269648319358,
118.027757568493)) ;
#187621=CARTESIAN_POINT('Ctrl Pts',(-14.0113057802947,-12.5848307790968,
117.981092726393)) ;
#187622=CARTESIAN_POINT('Ctrl Pts',(-13.923908857957,-12.428840573078,117.750424143547)) ;
#187623=CARTESIAN_POINT('Ctrl Pts',(-13.9139322792742,-12.4976814923142,
117.720037092829)) ;
#187624=CARTESIAN_POINT('Ctrl Pts',(-13.8401284100277,-12.4976814537986,
117.744268055851)) ;
#187625=CARTESIAN_POINT('Ctrl Pts',(-13.7663245407813,-12.497681415283,
117.768499018874)) ;
#187626=CARTESIAN_POINT('Ctrl Pts',(-13.776301119464,-12.4288404960468,
117.798886069592)) ;
#187627=CARTESIAN_POINT('Ctrl Pts',(-13.7862776981468,-12.3599995768106,
117.829273120311)) ;
#187628=CARTESIAN_POINT('Ctrl Pts',(-13.8600815673933,-12.3599996153262,
117.805042157288)) ;
#187629=CARTESIAN_POINT('Ctrl Pts',(-13.9338854366397,-12.3599996538418,
117.780811194266)) ;
#187630=CARTESIAN_POINT('Ctrl Pts',(-13.923908857957,-12.428840573078,117.750424143547)) ;
#187631=CARTESIAN_POINT('Ctrl Pts',(-13.8265622817162,-12.3440689509793,
117.489359771701)) ;
#187632=CARTESIAN_POINT('Ctrl Pts',(-13.822634283057,-12.4189286311326,
117.477395719697)) ;
#187633=CARTESIAN_POINT('Ctrl Pts',(-13.7488304098932,-12.4189286151795,
117.501626670787)) ;
#187634=CARTESIAN_POINT('Ctrl Pts',(-13.6750265367294,-12.4189285992263,
117.525857621878)) ;
#187635=CARTESIAN_POINT('Ctrl Pts',(-13.6789545353885,-12.3440689190729,
117.537821673882)) ;
#187636=CARTESIAN_POINT('Ctrl Pts',(-13.6828825340477,-12.2692092389195,
117.549785725887)) ;
#187637=CARTESIAN_POINT('Ctrl Pts',(-13.7566864072115,-12.2692092548727,
117.525554774796)) ;
#187638=CARTESIAN_POINT('Ctrl Pts',(-13.8304902803753,-12.2692092708259,
117.501323823705)) ;
#187639=CARTESIAN_POINT('Ctrl Pts',(-13.8265622817162,-12.3440689509793,
117.489359771701)) ;
#187640=CARTESIAN_POINT('Ctrl Pts',(-13.724775039694,-12.3364316802486,
117.214968341071)) ;
#187641=CARTESIAN_POINT('Ctrl Pts',(-13.727210259981,-12.4119346033566,
117.222385627174)) ;
#187642=CARTESIAN_POINT('Ctrl Pts',(-13.6534063849637,-12.4119346140826,
117.24661657262)) ;
#187643=CARTESIAN_POINT('Ctrl Pts',(-13.5796025099464,-12.4119346248087,
117.270847518065)) ;
#187644=CARTESIAN_POINT('Ctrl Pts',(-13.5771672896594,-12.3364317017007,
117.263430231962)) ;
#187645=CARTESIAN_POINT('Ctrl Pts',(-13.5747320693725,-12.2609287785927,
117.256012945858)) ;
#187646=CARTESIAN_POINT('Ctrl Pts',(-13.6485359443898,-12.2609287678666,
117.231782000413)) ;
#187647=CARTESIAN_POINT('Ctrl Pts',(-13.722339819407,-12.2609287571406,
117.207551054968)) ;
#187648=CARTESIAN_POINT('Ctrl Pts',(-13.724775039694,-12.3364316802486,
117.214968341071)) ;
#187649=CARTESIAN_POINT('Ctrl Pts',(-13.6265849302069,-12.4059134721985,
116.95117861997)) ;
#187650=CARTESIAN_POINT('Ctrl Pts',(-13.6351489860303,-12.4766756049436,
116.977263350182)) ;
#187651=CARTESIAN_POINT('Ctrl Pts',(-13.5613451122622,-12.4766756431297,
117.001494299432)) ;
#187652=CARTESIAN_POINT('Ctrl Pts',(-13.4875412384941,-12.4766756813157,
117.025725248682)) ;
#187653=CARTESIAN_POINT('Ctrl Pts',(-13.4789771826708,-12.4059135485707,
116.99964051847)) ;
#187654=CARTESIAN_POINT('Ctrl Pts',(-13.4704131268474,-12.3351514158256,
116.973555788258)) ;
#187655=CARTESIAN_POINT('Ctrl Pts',(-13.5442170006155,-12.3351513776395,
116.949324839008)) ;
#187656=CARTESIAN_POINT('Ctrl Pts',(-13.6180208743836,-12.3351513394535,
116.925093889758)) ;
#187657=CARTESIAN_POINT('Ctrl Pts',(-13.6265849302069,-12.4059134721985,
116.95117861997)) ;
#187658=CARTESIAN_POINT('Ctrl Pts',(-13.5366237570857,-12.5482447968648,
116.712705270971)) ;
#187659=CARTESIAN_POINT('Ctrl Pts',(-13.5507458951502,-12.609174259838,
116.755719022846)) ;
#187660=CARTESIAN_POINT('Ctrl Pts',(-13.4769420250043,-12.6091743240943,
116.779949983129)) ;
#187661=CARTESIAN_POINT('Ctrl Pts',(-13.4031381548583,-12.6091743883507,
116.804180943411)) ;
#187662=CARTESIAN_POINT('Ctrl Pts',(-13.3890160167938,-12.5482449253774,
116.761167191536)) ;
#187663=CARTESIAN_POINT('Ctrl Pts',(-13.3748938787293,-12.4873154624041,
116.71815343966)) ;
#187664=CARTESIAN_POINT('Ctrl Pts',(-13.4486977488753,-12.4873153981478,
116.693922479378)) ;
#187665=CARTESIAN_POINT('Ctrl Pts',(-13.5225016190212,-12.4873153338915,
116.669691519095)) ;
#187666=CARTESIAN_POINT('Ctrl Pts',(-13.5366237570857,-12.5482447968648,
116.712705270971)) ;
#187667=CARTESIAN_POINT('Ctrl Pts',(-13.4616241401097,-12.7523234032848,
116.519655572722)) ;
#187668=CARTESIAN_POINT('Ctrl Pts',(-13.4802710790298,-12.7990945462317,
116.576451137909)) ;
#187669=CARTESIAN_POINT('Ctrl Pts',(-13.406467214966,-12.7990946317952,
116.600682116717)) ;
#187670=CARTESIAN_POINT('Ctrl Pts',(-13.3326633509022,-12.7990947173587,
116.624913095525)) ;
#187671=CARTESIAN_POINT('Ctrl Pts',(-13.314016411982,-12.7523235744117,
116.568117530338)) ;
#187672=CARTESIAN_POINT('Ctrl Pts',(-13.2953694730618,-12.7055524314648,
116.51132196515)) ;
#187673=CARTESIAN_POINT('Ctrl Pts',(-13.3691733371256,-12.7055523459013,
116.487090986342)) ;
#187674=CARTESIAN_POINT('Ctrl Pts',(-13.4429772011895,-12.7055522603379,
116.462860007534)) ;
#187675=CARTESIAN_POINT('Ctrl Pts',(-13.4616241401097,-12.7523234032848,
116.519655572722)) ;
#187676=CARTESIAN_POINT('Ctrl Pts',(-13.4055646043146,-13.0044659647124,
116.384391147857)) ;
#187677=CARTESIAN_POINT('Ctrl Pts',(-13.4274187926225,-13.0337028196908,
116.450955477187)) ;
#187678=CARTESIAN_POINT('Ctrl Pts',(-13.3536149363877,-13.0337029200477,
116.47518647984)) ;
#187679=CARTESIAN_POINT('Ctrl Pts',(-13.2798110801529,-13.0337030204046,
116.499417482494)) ;
#187680=CARTESIAN_POINT('Ctrl Pts',(-13.2579568918449,-13.0044661654261,
116.432853153164)) ;
#187681=CARTESIAN_POINT('Ctrl Pts',(-13.236102703537,-12.9752293104477,
116.366288823835)) ;
#187682=CARTESIAN_POINT('Ctrl Pts',(-13.3099065597718,-12.9752292100908,
116.342057821181)) ;
#187683=CARTESIAN_POINT('Ctrl Pts',(-13.3837104160066,-12.9752291097339,
116.317826818527)) ;
#187684=CARTESIAN_POINT('Ctrl Pts',(-13.4055646043146,-13.0044659647124,
116.384391147857)) ;
#187685=CARTESIAN_POINT('Ctrl Pts',(-13.3720356013224,-13.2877069321833,
116.317913961057)) ;
#187686=CARTESIAN_POINT('Ctrl Pts',(-13.3955257178423,-13.2972126814731,
116.389461063794)) ;
#187687=CARTESIAN_POINT('Ctrl Pts',(-13.3217218704914,-13.2972127876648,
116.413692093507)) ;
#187688=CARTESIAN_POINT('Ctrl Pts',(-13.2479180231405,-13.2972128938564,
116.437923123219)) ;
#187689=CARTESIAN_POINT('Ctrl Pts',(-13.2244279066205,-13.2877071445666,
116.366376020483)) ;
#187690=CARTESIAN_POINT('Ctrl Pts',(-13.2009377901005,-13.2782013952768,
116.294828917746)) ;
#187691=CARTESIAN_POINT('Ctrl Pts',(-13.2747416374515,-13.2782012890852,
116.270597888033)) ;
#187692=CARTESIAN_POINT('Ctrl Pts',(-13.3485454848024,-13.2782011828935,
116.24636685832)) ;
#187693=CARTESIAN_POINT('Ctrl Pts',(-13.3720356013224,-13.2877069321833,
116.317913961057)) ;
#187694=CARTESIAN_POINT('Ctrl Pts',(-13.362788115581,-13.5768962487208,
116.324968700109)) ;
#187695=CARTESIAN_POINT('Ctrl Pts',(-13.3862298492881,-13.5662255723237,
116.396368436635)) ;
#187696=CARTESIAN_POINT('Ctrl Pts',(-13.312426010763,-13.5662256764684,
116.42059949323)) ;
#187697=CARTESIAN_POINT('Ctrl Pts',(-13.2386221722379,-13.5662257806131,
116.444830549825)) ;
#187698=CARTESIAN_POINT('Ctrl Pts',(-13.2151804385309,-13.5768964570101,
116.373430813298)) ;
#187699=CARTESIAN_POINT('Ctrl Pts',(-13.1917387048238,-13.5875671334072,
116.302031076772)) ;
#187700=CARTESIAN_POINT('Ctrl Pts',(-13.2655425433489,-13.5875670292625,
116.277800020177)) ;
#187701=CARTESIAN_POINT('Ctrl Pts',(-13.339346381874,-13.5875669251178,
116.253568963582)) ;
#187702=CARTESIAN_POINT('Ctrl Pts',(-13.362788115581,-13.5768962487208,
116.324968700109)) ;
#187703=CARTESIAN_POINT('Ctrl Pts',(-13.3775423934189,-13.8582071770573,
116.405572255842)) ;
#187704=CARTESIAN_POINT('Ctrl Pts',(-13.3992513169307,-13.8278804219563,
116.471694132178)) ;
#187705=CARTESIAN_POINT('Ctrl Pts',(-13.3254474864398,-13.8278805144787,
116.495925213244)) ;
#187706=CARTESIAN_POINT('Ctrl Pts',(-13.2516436559489,-13.8278806070012,
116.520156294309)) ;
#187707=CARTESIAN_POINT('Ctrl Pts',(-13.229934732437,-13.8582073621022,
116.454034417973)) ;
#187708=CARTESIAN_POINT('Ctrl Pts',(-13.2082258089251,-13.8885341172032,
116.387912541636)) ;
#187709=CARTESIAN_POINT('Ctrl Pts',(-13.2820296394161,-13.8885340246808,
116.363681460571)) ;
#187710=CARTESIAN_POINT('Ctrl Pts',(-13.355833469907,-13.8885339321583,
116.339450379505)) ;
#187711=CARTESIAN_POINT('Ctrl Pts',(-13.3775423934189,-13.8582071770573,
116.405572255842)) ;
#187712=CARTESIAN_POINT('Ctrl Pts',(-13.4146012475886,-14.1061445299723,
116.553894025949)) ;
#187713=CARTESIAN_POINT('Ctrl Pts',(-13.4330218964066,-14.0584618505827,
116.610000348217)) ;
#187714=CARTESIAN_POINT('Ctrl Pts',(-13.3592180722115,-14.0584619253186,
116.634231448458)) ;
#187715=CARTESIAN_POINT('Ctrl Pts',(-13.2854142480164,-14.0584620000544,
116.6584625487)) ;
#187716=CARTESIAN_POINT('Ctrl Pts',(-13.2669935991984,-14.106144679444,
116.602356226433)) ;
#187717=CARTESIAN_POINT('Ctrl Pts',(-13.2485729503803,-14.1538273588336,
116.546249904166)) ;
#187718=CARTESIAN_POINT('Ctrl Pts',(-13.3223767745754,-14.1538272840978,
116.522018803924)) ;
#187719=CARTESIAN_POINT('Ctrl Pts',(-13.3961805987705,-14.1538272093619,
116.497787703682)) ;
#187720=CARTESIAN_POINT('Ctrl Pts',(-13.4146012475886,-14.1061445299723,
116.553894025949)) ;
#187721=CARTESIAN_POINT('Ctrl Pts',(-13.4702307809164,-14.3044364274605,
116.758686302977)) ;
#187722=CARTESIAN_POINT('Ctrl Pts',(-13.4840635351767,-14.2428379118998,
116.800818638766)) ;
#187723=CARTESIAN_POINT('Ctrl Pts',(-13.4102597152836,-14.2428379649648,
116.82504975211)) ;
#187724=CARTESIAN_POINT('Ctrl Pts',(-13.3364558953904,-14.2428380180299,
116.849280865455)) ;
#187725=CARTESIAN_POINT('Ctrl Pts',(-13.3226231411301,-14.3044365335905,
116.807148529667)) ;
#187726=CARTESIAN_POINT('Ctrl Pts',(-13.3087903868698,-14.3660350491512,
116.765016193878)) ;
#187727=CARTESIAN_POINT('Ctrl Pts',(-13.382594206763,-14.3660349960862,
116.740785080533)) ;
#187728=CARTESIAN_POINT('Ctrl Pts',(-13.4563980266561,-14.3660349430211,
116.716553967189)) ;
#187729=CARTESIAN_POINT('Ctrl Pts',(-13.4702307809164,-14.3044364274605,
116.758686302977)) ;
#187730=CARTESIAN_POINT('Ctrl Pts',(-13.5399984230881,-14.4399899755949,
117.006607909742)) ;
#187731=CARTESIAN_POINT('Ctrl Pts',(-13.5482480139637,-14.3688346755136,
117.031734830812)) ;
#187732=CARTESIAN_POINT('Ctrl Pts',(-13.474444195943,-14.3688347045207,
117.05596594986)) ;
#187733=CARTESIAN_POINT('Ctrl Pts',(-13.4006403779222,-14.3688347335278,
117.080197068908)) ;
#187734=CARTESIAN_POINT('Ctrl Pts',(-13.3923907870465,-14.4399900336091,
117.055070147837)) ;
#187735=CARTESIAN_POINT('Ctrl Pts',(-13.3841411961708,-14.5111453336905,
117.029943226766)) ;
#187736=CARTESIAN_POINT('Ctrl Pts',(-13.4579450141916,-14.5111453046834,
117.005712107718)) ;
#187737=CARTESIAN_POINT('Ctrl Pts',(-13.5317488322124,-14.5111452756763,
116.981480988671)) ;
#187738=CARTESIAN_POINT('Ctrl Pts',(-13.5399984230881,-14.4399899755949,
117.006607909742)) ;
#187739=CARTESIAN_POINT('Ctrl Pts',(-13.6186161086514,-14.5025588290042,
117.281708410836)) ;
#187740=CARTESIAN_POINT('Ctrl Pts',(-13.6206516993991,-14.4269270667857,
117.287908490306)) ;
#187741=CARTESIAN_POINT('Ctrl Pts',(-13.5468478802534,-14.4269270722705,
117.312139605927)) ;
#187742=CARTESIAN_POINT('Ctrl Pts',(-13.4730440611076,-14.4269270777552,
117.336370721548)) ;
#187743=CARTESIAN_POINT('Ctrl Pts',(-13.4710084703599,-14.5025588399736,
117.330170642078)) ;
#187744=CARTESIAN_POINT('Ctrl Pts',(-13.4689728796121,-14.5781906021921,
117.323970562609)) ;
#187745=CARTESIAN_POINT('Ctrl Pts',(-13.5427766987579,-14.5781905967074,
117.299739446988)) ;
#187746=CARTESIAN_POINT('Ctrl Pts',(-13.6165805179036,-14.5781905912227,
117.275508331367)) ;
#187747=CARTESIAN_POINT('Ctrl Pts',(-13.6186161086514,-14.5025588290042,
117.281708410836)) ;
#187748=CARTESIAN_POINT('Ctrl Pts',(-13.6987823075738,-14.4867545034676,
117.561336491413)) ;
#187749=CARTESIAN_POINT('Ctrl Pts',(-13.6944901322377,-14.4121117686934,
117.548263216521)) ;
#187750=CARTESIAN_POINT('Ctrl Pts',(-13.6206863103232,-14.4121117549338,
117.572494323709)) ;
#187751=CARTESIAN_POINT('Ctrl Pts',(-13.5468824884086,-14.4121117411741,
117.596725430897)) ;
#187752=CARTESIAN_POINT('Ctrl Pts',(-13.5511746637448,-14.4867544759483,
117.609798705789)) ;
#187753=CARTESIAN_POINT('Ctrl Pts',(-13.5554668390809,-14.5613972107224,
117.622871980681)) ;
#187754=CARTESIAN_POINT('Ctrl Pts',(-13.6292706609955,-14.5613972244821,
117.598640873493)) ;
#187755=CARTESIAN_POINT('Ctrl Pts',(-13.70307448291,-14.5613972382417,117.574409766305)) ;
#187756=CARTESIAN_POINT('Ctrl Pts',(-13.6987823075738,-14.4867545034676,
117.561336491413)) ;
#187757=CARTESIAN_POINT('Ctrl Pts',(-13.7741769319229,-14.395053842158,
117.826317562051)) ;
#187758=CARTESIAN_POINT('Ctrl Pts',(-13.7638829047759,-14.3267009786415,
117.794963615073)) ;
#187759=CARTESIAN_POINT('Ctrl Pts',(-13.6900790789911,-14.3267009501932,
117.819194710473)) ;
#187760=CARTESIAN_POINT('Ctrl Pts',(-13.6162752532064,-14.3267009217449,
117.843425805873)) ;
#187761=CARTESIAN_POINT('Ctrl Pts',(-13.6265692803534,-14.3950537852614,
117.874779752851)) ;
#187762=CARTESIAN_POINT('Ctrl Pts',(-13.6368633075005,-14.463406648778,
117.906133699828)) ;
#187763=CARTESIAN_POINT('Ctrl Pts',(-13.7106671332852,-14.4634066772262,
117.881902604428)) ;
#187764=CARTESIAN_POINT('Ctrl Pts',(-13.78447095907,-14.4634067056745,117.857671509028)) ;
#187765=CARTESIAN_POINT('Ctrl Pts',(-13.7741769319229,-14.395053842158,
117.826317562051)) ;
#187766=CARTESIAN_POINT('Ctrl Pts',(-13.8391716224737,-14.2332235226471,
118.059743172962)) ;
#187767=CARTESIAN_POINT('Ctrl Pts',(-13.8235901984031,-14.1760661182545,
118.012284668238)) ;
#187768=CARTESIAN_POINT('Ctrl Pts',(-13.7497863676252,-14.1760660813659,
118.03651574843)) ;
#187769=CARTESIAN_POINT('Ctrl Pts',(-13.6759825368474,-14.1760660444773,
118.060746828621)) ;
#187770=CARTESIAN_POINT('Ctrl Pts',(-13.691563960918,-14.2332234488699,
118.108205333346)) ;
#187771=CARTESIAN_POINT('Ctrl Pts',(-13.7071453849885,-14.2903808532625,
118.15566383807)) ;
#187772=CARTESIAN_POINT('Ctrl Pts',(-13.7809492157664,-14.2903808901511,
118.131432757878)) ;
#187773=CARTESIAN_POINT('Ctrl Pts',(-13.8547530465442,-14.2903809270397,
118.107201677686)) ;
#187774=CARTESIAN_POINT('Ctrl Pts',(-13.8391716224737,-14.2332235226471,
118.059743172962)) ;
#187775=CARTESIAN_POINT('Ctrl Pts',(-13.8880711188325,-14.0127300062097,
118.244172770846)) ;
#187776=CARTESIAN_POINT('Ctrl Pts',(-13.8683174044897,-13.9708810531426,
118.184006143322)) ;
#187777=CARTESIAN_POINT('Ctrl Pts',(-13.7945135686933,-13.9708810143348,
118.208237208228)) ;
#187778=CARTESIAN_POINT('Ctrl Pts',(-13.7207097328969,-13.9708809755269,
118.232468273134)) ;
#187779=CARTESIAN_POINT('Ctrl Pts',(-13.7404634472397,-14.0127299285939,
118.292634900658)) ;
#187780=CARTESIAN_POINT('Ctrl Pts',(-13.7602171615824,-14.054578881661,
118.352801528181)) ;
#187781=CARTESIAN_POINT('Ctrl Pts',(-13.8340209973788,-14.0545789204688,
118.328570463275)) ;
#187782=CARTESIAN_POINT('Ctrl Pts',(-13.9078248331752,-14.0545789592767,
118.304339398369)) ;
#187783=CARTESIAN_POINT('Ctrl Pts',(-13.8880711188325,-14.0127300062097,
118.244172770846)) ;
#187784=CARTESIAN_POINT('Ctrl Pts',(-13.9166288887075,-13.7497867225439,
118.366622212608)) ;
#187785=CARTESIAN_POINT('Ctrl Pts',(-13.8941173007303,-13.7262335262759,
118.298055547143)) ;
#187786=CARTESIAN_POINT('Ctrl Pts',(-13.8203134605769,-13.7262334907042,
118.322286598779)) ;
#187787=CARTESIAN_POINT('Ctrl Pts',(-13.7465096204236,-13.7262334551324,
118.346517650415)) ;
#187788=CARTESIAN_POINT('Ctrl Pts',(-13.7690212084009,-13.7497866514004,
118.415084315879)) ;
#187789=CARTESIAN_POINT('Ctrl Pts',(-13.7915327963782,-13.7733398476684,
118.483650981343)) ;
#187790=CARTESIAN_POINT('Ctrl Pts',(-13.8653366365315,-13.7733398832402,
118.459419929707)) ;
#187791=CARTESIAN_POINT('Ctrl Pts',(-13.9391404766848,-13.7733399188119,
118.435188878072)) ;
#187792=CARTESIAN_POINT('Ctrl Pts',(-13.9166288887075,-13.7497867225439,
118.366622212608)) ;
#187793=CARTESIAN_POINT('Ctrl Pts',(-13.9219007960497,-13.4618226176213,
118.418297641467)) ;
#187794=CARTESIAN_POINT('Ctrl Pts',(-13.8982497624361,-13.4583403895165,
118.346260408634)) ;
#187795=CARTESIAN_POINT('Ctrl Pts',(-13.8244459191647,-13.458340362269,
118.370491450772)) ;
#187796=CARTESIAN_POINT('Ctrl Pts',(-13.7506420758933,-13.4583403350215,
118.394722492911)) ;
#187797=CARTESIAN_POINT('Ctrl Pts',(-13.7742931095069,-13.4618225631264,
118.466759725744)) ;
#187798=CARTESIAN_POINT('Ctrl Pts',(-13.7979441431205,-13.4653047912312,
118.538796958577)) ;
#187799=CARTESIAN_POINT('Ctrl Pts',(-13.8717479863919,-13.4653048184787,
118.514565916438)) ;
#187800=CARTESIAN_POINT('Ctrl Pts',(-13.9455518296633,-13.4653048457262,
118.4903348743)) ;
#187801=CARTESIAN_POINT('Ctrl Pts',(-13.9219007960497,-13.4618226176213,
118.418297641467)) ;
#187802=CARTESIAN_POINT('Ctrl Pts',(-13.903127021165,-13.1741720910159,
118.396295941709)) ;
#187803=CARTESIAN_POINT('Ctrl Pts',(-13.8800232858796,-13.1907692085376,
118.325925691383)) ;
#187804=CARTESIAN_POINT('Ctrl Pts',(-13.8062194407577,-13.1907691874801,
118.350156727884)) ;
#187805=CARTESIAN_POINT('Ctrl Pts',(-13.7324155956357,-13.1907691664227,
118.374387764386)) ;
#187806=CARTESIAN_POINT('Ctrl Pts',(-13.755519330921,-13.1741720489011,
118.444758014713)) ;
#187807=CARTESIAN_POINT('Ctrl Pts',(-13.7786230662063,-13.1575749313794,
118.515128265039)) ;
#187808=CARTESIAN_POINT('Ctrl Pts',(-13.8524269113283,-13.1575749524368,
118.490897228537)) ;
#187809=CARTESIAN_POINT('Ctrl Pts',(-13.9262307564503,-13.1575749734943,
118.466666192035)) ;
#187810=CARTESIAN_POINT('Ctrl Pts',(-13.903127021165,-13.1741720910159,
118.396295941709)) ;
#187811=CARTESIAN_POINT('Ctrl Pts',(-13.8603632973549,-12.9003777795887,
118.301689211796)) ;
#187812=CARTESIAN_POINT('Ctrl Pts',(-13.8394728277255,-12.9361179634059,
118.23806021172)) ;
#187813=CARTESIAN_POINT('Ctrl Pts',(-13.7656689822045,-12.9361179523589,
118.262291247007)) ;
#187814=CARTESIAN_POINT('Ctrl Pts',(-13.6918651366836,-12.9361179413118,
118.286522282294)) ;
#187815=CARTESIAN_POINT('Ctrl Pts',(-13.712755606313,-12.9003777574947,
118.35015128237)) ;
#187816=CARTESIAN_POINT('Ctrl Pts',(-13.7336460759424,-12.8646375736775,
118.413780282446)) ;
#187817=CARTESIAN_POINT('Ctrl Pts',(-13.8074499214633,-12.8646375847245,
118.389549247159)) ;
#187818=CARTESIAN_POINT('Ctrl Pts',(-13.8812537669843,-12.8646375957715,
118.365318211872)) ;
#187819=CARTESIAN_POINT('Ctrl Pts',(-13.8603632973549,-12.9003777795887,
118.301689211796)) ;
#187820=CARTESIAN_POINT('Ctrl Pts',(-13.7965184753655,-12.6657294356323,
118.142588775569)) ;
#187821=CARTESIAN_POINT('Ctrl Pts',(-13.7793228293971,-12.7179077722526,
118.090213612314)) ;
#187822=CARTESIAN_POINT('Ctrl Pts',(-13.7055189843026,-12.7179077672934,
118.1144446489)) ;
#187823=CARTESIAN_POINT('Ctrl Pts',(-13.6317151392082,-12.7179077623343,
118.138675685485)) ;
#187824=CARTESIAN_POINT('Ctrl Pts',(-13.6489107851767,-12.665729425714,
118.19105084874)) ;
#187825=CARTESIAN_POINT('Ctrl Pts',(-13.6661064311451,-12.6135510890938,
118.243426011995)) ;
#187826=CARTESIAN_POINT('Ctrl Pts',(-13.7399102762396,-12.6135510940529,
118.219194975409)) ;
#187827=CARTESIAN_POINT('Ctrl Pts',(-13.813714121334,-12.6135510990121,
118.194963938823)) ;
#187828=CARTESIAN_POINT('Ctrl Pts',(-13.7965184753655,-12.6657294356323,
118.142588775569)) ;
#187829=CARTESIAN_POINT('Ctrl Pts',(-13.7148231526105,-12.4838951882172,
117.929294896523)) ;
#187830=CARTESIAN_POINT('Ctrl Pts',(-13.7025707556539,-12.5488490680583,
117.891976072276)) ;
#187831=CARTESIAN_POINT('Ctrl Pts',(-13.6287669116955,-12.5488490674887,
117.916207112322)) ;
#187832=CARTESIAN_POINT('Ctrl Pts',(-13.5549630677371,-12.5488490669192,
117.940438152368)) ;
#187833=CARTESIAN_POINT('Ctrl Pts',(-13.5672154646937,-12.4838951870781,
117.977756976615)) ;
#187834=CARTESIAN_POINT('Ctrl Pts',(-13.5794678616503,-12.418941307237,
118.015075800863)) ;
#187835=CARTESIAN_POINT('Ctrl Pts',(-13.6532717056087,-12.4189413078066,
117.990844760817)) ;
#187836=CARTESIAN_POINT('Ctrl Pts',(-13.727075549567,-12.4189413083761,
117.966613720771)) ;
#187837=CARTESIAN_POINT('Ctrl Pts',(-13.7148231526105,-12.4838951882172,
117.929294896523)) ;
#187838=CARTESIAN_POINT('Ctrl Pts',(-13.6210385512733,-12.3696269961183,
117.679015146672)) ;
#187839=CARTESIAN_POINT('Ctrl Pts',(-13.614584536571,-12.4426568392055,
117.659357259267)) ;
#187840=CARTESIAN_POINT('Ctrl Pts',(-13.54078069357,-12.4426568397969,117.683588302229)) ;
#187841=CARTESIAN_POINT('Ctrl Pts',(-13.466976850569,-12.4426568403884,
117.707819345191)) ;
#187842=CARTESIAN_POINT('Ctrl Pts',(-13.4734308652713,-12.3696269973012,
117.727477232596)) ;
#187843=CARTESIAN_POINT('Ctrl Pts',(-13.4798848799736,-12.2965971542141,
117.74713512)) ;
#187844=CARTESIAN_POINT('Ctrl Pts',(-13.5536887229746,-12.2965971536226,
117.722904077038)) ;
#187845=CARTESIAN_POINT('Ctrl Pts',(-13.6274925659757,-12.2965971530311,
117.698673034076)) ;
#187846=CARTESIAN_POINT('Ctrl Pts',(-13.6210385512733,-12.3696269961183,
117.679015146672)) ;
#187847=CARTESIAN_POINT('Ctrl Pts',(-13.5204267176276,-12.3300023799241,
117.408075297011)) ;
#187848=CARTESIAN_POINT('Ctrl Pts',(-13.5202538843444,-12.4059080645877,
117.407548874782)) ;
#187849=CARTESIAN_POINT('Ctrl Pts',(-13.4464500419793,-12.4059080646803,
117.431779919681)) ;
#187850=CARTESIAN_POINT('Ctrl Pts',(-13.3726461996142,-12.4059080647729,
117.456010964579)) ;
#187851=CARTESIAN_POINT('Ctrl Pts',(-13.3728190328973,-12.3300023801093,
117.456537386809)) ;
#187852=CARTESIAN_POINT('Ctrl Pts',(-13.3729918661804,-12.2540966954457,
117.457063809038)) ;
#187853=CARTESIAN_POINT('Ctrl Pts',(-13.4467957085455,-12.2540966953531,
117.432832764139)) ;
#187854=CARTESIAN_POINT('Ctrl Pts',(-13.5205995509106,-12.2540966952605,
117.40860171924)) ;
#187855=CARTESIAN_POINT('Ctrl Pts',(-13.5204267176276,-12.3300023799241,
117.408075297011)) ;
#187856=CARTESIAN_POINT('Ctrl Pts',(-13.4198641245608,-12.3684199778557,
117.137243310197)) ;
#187857=CARTESIAN_POINT('Ctrl Pts',(-13.4259793249483,-12.4417552779972,
117.155869223949)) ;
#187858=CARTESIAN_POINT('Ctrl Pts',(-13.3521754823948,-12.4417552770606,
117.180100268274)) ;
#187859=CARTESIAN_POINT('Ctrl Pts',(-13.2783716398414,-12.441755276124,
117.2043313126)) ;
#187860=CARTESIAN_POINT('Ctrl Pts',(-13.272256439454,-12.3684199759825,
117.185705398848)) ;
#187861=CARTESIAN_POINT('Ctrl Pts',(-13.2661412390666,-12.2950846758409,
117.167079485096)) ;
#187862=CARTESIAN_POINT('Ctrl Pts',(-13.33994508162,-12.2950846767775,117.14284844077)) ;
#187863=CARTESIAN_POINT('Ctrl Pts',(-13.4137489241733,-12.2950846777141,
117.118617396445)) ;
#187864=CARTESIAN_POINT('Ctrl Pts',(-13.4198641245608,-12.3684199778557,
117.137243310197)) ;
#187865=CARTESIAN_POINT('Ctrl Pts',(-13.3254467352035,-12.4825669571575,
116.885241947658)) ;
#187866=CARTESIAN_POINT('Ctrl Pts',(-13.3374276722368,-12.5480396537864,
116.92173394874)) ;
#187867=CARTESIAN_POINT('Ctrl Pts',(-13.2636238287276,-12.5480396536061,
116.945964990155)) ;
#187868=CARTESIAN_POINT('Ctrl Pts',(-13.1898199852184,-12.5480396534258,
116.970196031569)) ;
#187869=CARTESIAN_POINT('Ctrl Pts',(-13.1778390481851,-12.4825669567968,
116.933704030486)) ;
#187870=CARTESIAN_POINT('Ctrl Pts',(-13.1658581111518,-12.4170942601679,
116.897212029403)) ;
#187871=CARTESIAN_POINT('Ctrl Pts',(-13.239661954661,-12.4170942603482,
116.872980987989)) ;
#187872=CARTESIAN_POINT('Ctrl Pts',(-13.3134657981702,-12.4170942605285,
116.848749946575)) ;
#187873=CARTESIAN_POINT('Ctrl Pts',(-13.3254467352035,-12.4825669571575,
116.885241947658)) ;
#187874=CARTESIAN_POINT('Ctrl Pts',(-13.2438983807686,-12.6630281231511,
116.672250461998)) ;
#187875=CARTESIAN_POINT('Ctrl Pts',(-13.2608585513106,-12.7159956192618,
116.723908404873)) ;
#187876=CARTESIAN_POINT('Ctrl Pts',(-13.1870547068666,-12.7159956220205,
116.74813944344)) ;
#187877=CARTESIAN_POINT('Ctrl Pts',(-13.1132508624226,-12.7159956247792,
116.772370482007)) ;
#187878=CARTESIAN_POINT('Ctrl Pts',(-13.0962906918806,-12.6630281286685,
116.720712539132)) ;
#187879=CARTESIAN_POINT('Ctrl Pts',(-13.0793305213386,-12.6100606325577,
116.669054596257)) ;
#187880=CARTESIAN_POINT('Ctrl Pts',(-13.1531343657826,-12.610060629799,
116.64482355769)) ;
#187881=CARTESIAN_POINT('Ctrl Pts',(-13.2269382102266,-12.6100606270403,
116.620592519123)) ;
#187882=CARTESIAN_POINT('Ctrl Pts',(-13.2438983807686,-12.6630281231511,
116.672250461998)) ;
#187883=CARTESIAN_POINT('Ctrl Pts',(-13.1795990563112,-12.898267035054,
116.511928383513)) ;
#187884=CARTESIAN_POINT('Ctrl Pts',(-13.2003385571015,-12.9348862826856,
116.575097556412)) ;
#187885=CARTESIAN_POINT('Ctrl Pts',(-13.126534711989,-12.9348862916205,
116.599328592942)) ;
#187886=CARTESIAN_POINT('Ctrl Pts',(-13.0527308668765,-12.9348863005553,
116.623559629473)) ;
#187887=CARTESIAN_POINT('Ctrl Pts',(-13.0319913660862,-12.8982670529237,
116.560390456574)) ;
#187888=CARTESIAN_POINT('Ctrl Pts',(-13.0112518652958,-12.8616478052921,
116.497221283675)) ;
#187889=CARTESIAN_POINT('Ctrl Pts',(-13.0850557104084,-12.8616477963572,
116.472990247145)) ;
#187890=CARTESIAN_POINT('Ctrl Pts',(-13.1588595555209,-12.8616477874224,
116.448759210614)) ;
#187891=CARTESIAN_POINT('Ctrl Pts',(-13.1795990563112,-12.898267035054,
116.511928383513)) ;
#187892=CARTESIAN_POINT('Ctrl Pts',(-13.1369040201403,-13.1692444185093,
116.417205413747)) ;
#187893=CARTESIAN_POINT('Ctrl Pts',(-13.1599237253209,-13.1869963126333,
116.487319721198)) ;
#187894=CARTESIAN_POINT('Ctrl Pts',(-13.0861198805798,-13.186996328282,
116.511550758859)) ;
#187895=CARTESIAN_POINT('Ctrl Pts',(-13.0123160358387,-13.1869963439306,
116.535781796521)) ;
#187896=CARTESIAN_POINT('Ctrl Pts',(-12.9892963306581,-13.1692444498067,
116.46566748907)) ;
#187897=CARTESIAN_POINT('Ctrl Pts',(-12.9662766254774,-13.1514925556827,
116.395553181619)) ;
#187898=CARTESIAN_POINT('Ctrl Pts',(-13.0400804702186,-13.1514925400341,
116.371322143957)) ;
#187899=CARTESIAN_POINT('Ctrl Pts',(-13.1138843149597,-13.1514925243854,
116.347091106295)) ;
#187900=CARTESIAN_POINT('Ctrl Pts',(-13.1369040201403,-13.1692444185093,
116.417205413747)) ;
#187901=CARTESIAN_POINT('Ctrl Pts',(-13.1175944030743,-13.4593682561925,
116.393894522823)) ;
#187902=CARTESIAN_POINT('Ctrl Pts',(-13.141261082871,-13.4568887930797,
116.465979410413)) ;
#187903=CARTESIAN_POINT('Ctrl Pts',(-13.0674572395062,-13.4568888172156,
116.490210452267)) ;
#187904=CARTESIAN_POINT('Ctrl Pts',(-12.9936533961414,-13.4568888413516,
116.514441494121)) ;
#187905=CARTESIAN_POINT('Ctrl Pts',(-12.9699867163446,-13.4593683044645,
116.442356606531)) ;
#187906=CARTESIAN_POINT('Ctrl Pts',(-12.9463200365478,-13.4618477675773,
116.370271718941)) ;
#187907=CARTESIAN_POINT('Ctrl Pts',(-13.0201238799127,-13.4618477434414,
116.346040677087)) ;
#187908=CARTESIAN_POINT('Ctrl Pts',(-13.0939277232775,-13.4618477193054,
116.321809635233)) ;
#187909=CARTESIAN_POINT('Ctrl Pts',(-13.1175944030743,-13.4593682561925,
116.393894522823)) ;
#187910=CARTESIAN_POINT('Ctrl Pts',(-13.1227026248899,-13.7466998259824,
116.444974799646)) ;
#187911=CARTESIAN_POINT('Ctrl Pts',(-13.1453118932417,-13.7241548771273,
116.513838982417)) ;
#187912=CARTESIAN_POINT('Ctrl Pts',(-13.071508052718,-13.7241549087659,
116.538070032924)) ;
#187913=CARTESIAN_POINT('Ctrl Pts',(-12.9977042121942,-13.7241549404046,
116.562301083432)) ;
#187914=CARTESIAN_POINT('Ctrl Pts',(-12.9750949438424,-13.7466998892598,
116.493436900661)) ;
#187915=CARTESIAN_POINT('Ctrl Pts',(-12.9524856754905,-13.7692448381149,
116.42457271789)) ;
#187916=CARTESIAN_POINT('Ctrl Pts',(-13.0262895160143,-13.7692448064763,
116.400341667382)) ;
#187917=CARTESIAN_POINT('Ctrl Pts',(-13.100093356538,-13.7692447748376,
116.376110616875)) ;
#187918=CARTESIAN_POINT('Ctrl Pts',(-13.1227026248899,-13.7466998259824,
116.444974799646)) ;
#187919=CARTESIAN_POINT('Ctrl Pts',(-13.150926931708,-14.0096322945866,
116.566356438622)) ;
#187920=CARTESIAN_POINT('Ctrl Pts',(-13.1708653800573,-13.9686968355008,
116.627085734444)) ;
#187921=CARTESIAN_POINT('Ctrl Pts',(-13.0970615434274,-13.9686968703367,
116.651316796811)) ;
#187922=CARTESIAN_POINT('Ctrl Pts',(-13.0232577067976,-13.9686969051726,
116.675547859179)) ;
#187923=CARTESIAN_POINT('Ctrl Pts',(-13.0033192584483,-14.0096323642584,
116.614818563357)) ;
#187924=CARTESIAN_POINT('Ctrl Pts',(-12.983380810099,-14.0505678233442,
116.554089267536)) ;
#187925=CARTESIAN_POINT('Ctrl Pts',(-13.0571846467288,-14.0505677885083,
116.529858205168)) ;
#187926=CARTESIAN_POINT('Ctrl Pts',(-13.1309884833587,-14.0505677536723,
116.505627142801)) ;
#187927=CARTESIAN_POINT('Ctrl Pts',(-13.150926931708,-14.0096322945866,
116.566356438622)) ;
#187928=CARTESIAN_POINT('Ctrl Pts',(-13.1995653491021,-14.2308164989726,
116.74998223283)) ;
#187929=CARTESIAN_POINT('Ctrl Pts',(-13.2154025368311,-14.1743789457168,
116.798219750367)) ;
#187930=CARTESIAN_POINT('Ctrl Pts',(-13.1415987048859,-14.1743789796015,
116.822450827003)) ;
#187931=CARTESIAN_POINT('Ctrl Pts',(-13.0677948729407,-14.1743790134861,
116.846681903639)) ;
#187932=CARTESIAN_POINT('Ctrl Pts',(-13.0519576852117,-14.2308165667419,
116.798444386103)) ;
#187933=CARTESIAN_POINT('Ctrl Pts',(-13.0361204974827,-14.2872541199976,
116.750206868567)) ;
#187934=CARTESIAN_POINT('Ctrl Pts',(-13.1099243294279,-14.287254086113,
116.72597579193)) ;
#187935=CARTESIAN_POINT('Ctrl Pts',(-13.1837281613731,-14.2872540522283,
116.701744715294)) ;
#187936=CARTESIAN_POINT('Ctrl Pts',(-13.1995653491021,-14.2308164989726,
116.74998223283)) ;
#187937=CARTESIAN_POINT('Ctrl Pts',(-13.2646742672153,-14.3939170940553,
116.983896364824)) ;
#187938=CARTESIAN_POINT('Ctrl Pts',(-13.2752519050489,-14.3260101541607,
117.016114141811)) ;
#187939=CARTESIAN_POINT('Ctrl Pts',(-13.2014480783073,-14.3260101812409,
117.040345234297)) ;
#187940=CARTESIAN_POINT('Ctrl Pts',(-13.1276442515657,-14.3260102083211,
117.064576326782)) ;
#187941=CARTESIAN_POINT('Ctrl Pts',(-13.1170666137321,-14.3939171482158,
117.032358549795)) ;
#187942=CARTESIAN_POINT('Ctrl Pts',(-13.1064889758985,-14.4618240881105,
117.000140772807)) ;
#187943=CARTESIAN_POINT('Ctrl Pts',(-13.1802928026401,-14.4618240610302,
116.975909680322)) ;
#187944=CARTESIAN_POINT('Ctrl Pts',(-13.2540966293817,-14.46182403395,116.951678587836)) ;
#187945=CARTESIAN_POINT('Ctrl Pts',(-13.2646742672153,-14.3939170940553,
116.983896364824)) ;
#187946=CARTESIAN_POINT('Ctrl Pts',(-13.3398740457565,-14.4862563732453,
117.248221458507)) ;
#187947=CARTESIAN_POINT('Ctrl Pts',(-13.3444866220433,-14.411804800515,
117.262270620354)) ;
#187948=CARTESIAN_POINT('Ctrl Pts',(-13.2706827989801,-14.4118048137988,
117.286501724043)) ;
#187949=CARTESIAN_POINT('Ctrl Pts',(-13.1968789759169,-14.4118048270827,
117.310732827733)) ;
#187950=CARTESIAN_POINT('Ctrl Pts',(-13.19226639963,-14.486256399813,117.296683665885)) ;
#187951=CARTESIAN_POINT('Ctrl Pts',(-13.1876538233431,-14.5607079725433,
117.282634504038)) ;
#187952=CARTESIAN_POINT('Ctrl Pts',(-13.2614576464064,-14.5607079592595,
117.258403400348)) ;
#187953=CARTESIAN_POINT('Ctrl Pts',(-13.3352614694696,-14.5607079459756,
117.234172296659)) ;
#187954=CARTESIAN_POINT('Ctrl Pts',(-13.3398740457565,-14.4862563732453,
117.248221458507)) ;
#187955=CARTESIAN_POINT('Ctrl Pts',(-13.4203621530711,-14.5025873133897,
117.528986407561)) ;
#187956=CARTESIAN_POINT('Ctrl Pts',(-13.4186251106891,-14.4268872889833,
117.523695655272)) ;
#187957=CARTESIAN_POINT('Ctrl Pts',(-13.3448212908417,-14.4268872836565,
117.547926768756)) ;
#187958=CARTESIAN_POINT('Ctrl Pts',(-13.2710174709942,-14.4268872783298,
117.57215788224)) ;
#187959=CARTESIAN_POINT('Ctrl Pts',(-13.2727545133762,-14.5025873027362,
117.577448634529)) ;
#187960=CARTESIAN_POINT('Ctrl Pts',(-13.2744915557582,-14.5782873271426,
117.582739386817)) ;
#187961=CARTESIAN_POINT('Ctrl Pts',(-13.3482953756057,-14.5782873324694,
117.558508273334)) ;
#187962=CARTESIAN_POINT('Ctrl Pts',(-13.4220991954531,-14.5782873377961,
117.53427715985)) ;
#187963=CARTESIAN_POINT('Ctrl Pts',(-13.4203621530711,-14.5025873133897,
117.528986407561)) ;
#187964=CARTESIAN_POINT('Ctrl Pts',(-13.4982693773669,-14.4415569455837,
117.801564735725)) ;
#187965=CARTESIAN_POINT('Ctrl Pts',(-13.490360445347,-14.3700086479268,
117.777475403316)) ;
#187966=CARTESIAN_POINT('Ctrl Pts',(-13.4165566259671,-14.370008620797,
117.801706518224)) ;
#187967=CARTESIAN_POINT('Ctrl Pts',(-13.3427528065872,-14.3700085936673,
117.825937633132)) ;
#187968=CARTESIAN_POINT('Ctrl Pts',(-13.3506617386071,-14.4415568913242,
117.850026965541)) ;
#187969=CARTESIAN_POINT('Ctrl Pts',(-13.358570670627,-14.5131051889812,
117.87411629795)) ;
#187970=CARTESIAN_POINT('Ctrl Pts',(-13.4323744900069,-14.5131052161109,
117.849885183042)) ;
#187971=CARTESIAN_POINT('Ctrl Pts',(-13.5061783093868,-14.5131052432407,
117.825654068134)) ;
#187972=CARTESIAN_POINT('Ctrl Pts',(-13.4982693773669,-14.4415569455837,
117.801564735725)) ;
#187973=CARTESIAN_POINT('Ctrl Pts',(-13.5687615474577,-14.3059463498269,
118.051984040439)) ;
#187974=CARTESIAN_POINT('Ctrl Pts',(-13.555180627917,-14.2437611215803,
118.01061874905)) ;
#187975=CARTESIAN_POINT('Ctrl Pts',(-13.481376807545,-14.2437610699902,
118.034849860937)) ;
#187976=CARTESIAN_POINT('Ctrl Pts',(-13.4075729871731,-14.2437610184,118.059080972823)) ;
#187977=CARTESIAN_POINT('Ctrl Pts',(-13.4211539067137,-14.3059462466466,
118.100446264212)) ;
#187978=CARTESIAN_POINT('Ctrl Pts',(-13.4347348262544,-14.3681314748932,
118.141811555601)) ;
#187979=CARTESIAN_POINT('Ctrl Pts',(-13.5085386466263,-14.3681315264833,
118.117580443714)) ;
#187980=CARTESIAN_POINT('Ctrl Pts',(-13.5823424669983,-14.3681315780735,
118.093349331828)) ;
#187981=CARTESIAN_POINT('Ctrl Pts',(-13.5687615474577,-14.3059463498269,
118.051984040439)) ;
#187982=CARTESIAN_POINT('Ctrl Pts',(-13.6244542300278,-14.1081523204692,
118.256932053002)) ;
#187983=CARTESIAN_POINT('Ctrl Pts',(-13.6062345336819,-14.0596861997997,
118.201437795838)) ;
#187984=CARTESIAN_POINT('Ctrl Pts',(-13.5324307091071,-14.0596861267513,
118.225668894923)) ;
#187985=CARTESIAN_POINT('Ctrl Pts',(-13.4586268845323,-14.059686053703,
118.249899994008)) ;
#187986=CARTESIAN_POINT('Ctrl Pts',(-13.4768465808782,-14.1081521743725,
118.305394251172)) ;
#187987=CARTESIAN_POINT('Ctrl Pts',(-13.495066277224,-14.1566182950421,
118.360888508336)) ;
#187988=CARTESIAN_POINT('Ctrl Pts',(-13.5688701017988,-14.1566183680904,
118.336657409251)) ;
#187989=CARTESIAN_POINT('Ctrl Pts',(-13.6426739263736,-14.1566184411388,
118.312426310166)) ;
#187990=CARTESIAN_POINT('Ctrl Pts',(-13.6244542300278,-14.1081523204692,
118.256932053002)) ;
#187991=CARTESIAN_POINT('Ctrl Pts',(-13.6616915004186,-13.8605107481474,
118.405813682003)) ;
#187992=CARTESIAN_POINT('Ctrl Pts',(-13.6401116629726,-13.8292631951763,
118.340084977109)) ;
#187993=CARTESIAN_POINT('Ctrl Pts',(-13.5663078323218,-13.8292631042665,
118.364316057688)) ;
#187994=CARTESIAN_POINT('Ctrl Pts',(-13.492504001671,-13.8292630133566,
118.388547138266)) ;
#187995=CARTESIAN_POINT('Ctrl Pts',(-13.5140838391171,-13.8605105663277,
118.45427584316)) ;
#187996=CARTESIAN_POINT('Ctrl Pts',(-13.5356636765632,-13.8917581192987,
118.520004548053)) ;
#187997=CARTESIAN_POINT('Ctrl Pts',(-13.6094675072139,-13.8917582102086,
118.495773467475)) ;
#187998=CARTESIAN_POINT('Ctrl Pts',(-13.6832713378647,-13.8917583011184,
118.471542386896)) ;
#187999=CARTESIAN_POINT('Ctrl Pts',(-13.6616915004186,-13.8605107481474,
118.405813682003)) ;
#188000=CARTESIAN_POINT('Ctrl Pts',(-13.6767027193647,-13.5802159839548,
118.487096599575)) ;
#188001=CARTESIAN_POINT('Ctrl Pts',(-13.6533073461115,-13.5684914929652,
118.415838065467)) ;
#188002=CARTESIAN_POINT('Ctrl Pts',(-13.5795035076158,-13.5684913902422,
118.440069122151)) ;
#188003=CARTESIAN_POINT('Ctrl Pts',(-13.50569966912,-13.5684912875191,118.464300178835)) ;
#188004=CARTESIAN_POINT('Ctrl Pts',(-13.5290950423732,-13.5802157785087,
118.535558712943)) ;
#188005=CARTESIAN_POINT('Ctrl Pts',(-13.5524904156264,-13.5919402694983,
118.606817247052)) ;
#188006=CARTESIAN_POINT('Ctrl Pts',(-13.6262942541222,-13.5919403722214,
118.582586190367)) ;
#188007=CARTESIAN_POINT('Ctrl Pts',(-13.700098092618,-13.5919404749444,
118.558355133683)) ;
#188008=CARTESIAN_POINT('Ctrl Pts',(-13.6767027193647,-13.5802159839548,
118.487096599575)) ;
#188009=CARTESIAN_POINT('Ctrl Pts',(-13.6675174437681,-13.2888355614903,
118.494615718162)) ;
#188010=CARTESIAN_POINT('Ctrl Pts',(-13.643994456241,-13.2974368879024,
118.422968491516)) ;
#188011=CARTESIAN_POINT('Ctrl Pts',(-13.5701906089222,-13.2974367821204,
118.447199521326)) ;
#188012=CARTESIAN_POINT('Ctrl Pts',(-13.4963867616034,-13.2974366763383,
118.471430551137)) ;
#188013=CARTESIAN_POINT('Ctrl Pts',(-13.5199097491305,-13.2888353499262,
118.543077777783)) ;
#188014=CARTESIAN_POINT('Ctrl Pts',(-13.5434327366576,-13.2802340235141,
118.61472500443)) ;
#188015=CARTESIAN_POINT('Ctrl Pts',(-13.6172365839764,-13.2802341292962,
118.590493974619)) ;
#188016=CARTESIAN_POINT('Ctrl Pts',(-13.6910404312952,-13.2802342350782,
118.566262944809)) ;
#188017=CARTESIAN_POINT('Ctrl Pts',(-13.6675174437681,-13.2888355614903,
118.494615718162)) ;
#188018=CARTESIAN_POINT('Ctrl Pts',(-13.6345263965788,-13.0084923611293,
118.429389220724)) ;
#188019=CARTESIAN_POINT('Ctrl Pts',(-13.6125426984709,-13.0366789477102,
118.362430421261)) ;
#188020=CARTESIAN_POINT('Ctrl Pts',(-13.5387388424139,-13.0366788478173,
118.386661424456)) ;
#188021=CARTESIAN_POINT('Ctrl Pts',(-13.4649349863569,-13.0366787479245,
118.410892427651)) ;
#188022=CARTESIAN_POINT('Ctrl Pts',(-13.4869186844647,-13.0084921613435,
118.477851227115)) ;
#188023=CARTESIAN_POINT('Ctrl Pts',(-13.5089023825726,-12.9803055747626,
118.544810026578)) ;
#188024=CARTESIAN_POINT('Ctrl Pts',(-13.5827062386296,-12.9803056746555,
118.520579023383)) ;
#188025=CARTESIAN_POINT('Ctrl Pts',(-13.6565100946866,-12.9803057745484,
118.496348020188)) ;
#188026=CARTESIAN_POINT('Ctrl Pts',(-13.6345263965788,-13.0084923611293,
118.429389220724)) ;
#188027=CARTESIAN_POINT('Ctrl Pts',(-13.578743439224,-12.7552927085919,
118.295029267959)) ;
#188028=CARTESIAN_POINT('Ctrl Pts',(-13.5598862064938,-12.8011984065865,
118.237593177571)) ;
#188029=CARTESIAN_POINT('Ctrl Pts',(-13.4860823424701,-12.8011983205869,
118.261824156501)) ;
#188030=CARTESIAN_POINT('Ctrl Pts',(-13.4122784784464,-12.8011982345872,
118.286055135431)) ;
#188031=CARTESIAN_POINT('Ctrl Pts',(-13.4311357111765,-12.7552925365926,
118.343491225819)) ;
#188032=CARTESIAN_POINT('Ctrl Pts',(-13.4499929439066,-12.709386838598,
118.400927316208)) ;
#188033=CARTESIAN_POINT('Ctrl Pts',(-13.5237968079303,-12.7093869245976,
118.376696337278)) ;
#188034=CARTESIAN_POINT('Ctrl Pts',(-13.5976006719541,-12.7093870105973,
118.352465358348)) ;
#188035=CARTESIAN_POINT('Ctrl Pts',(-13.578743439224,-12.7552927085919,
118.295029267959)) ;
#188036=CARTESIAN_POINT('Ctrl Pts',(-13.5039282764506,-12.5504983058309,
118.102546163647)) ;
#188037=CARTESIAN_POINT('Ctrl Pts',(-13.489534151706,-12.6107700146374,
118.058703980073)) ;
#188038=CARTESIAN_POINT('Ctrl Pts',(-13.4157302814213,-12.6107699496328,
118.082934939933)) ;
#188039=CARTESIAN_POINT('Ctrl Pts',(-13.3419264111365,-12.6107698846282,
118.107165899793)) ;
#188040=CARTESIAN_POINT('Ctrl Pts',(-13.3563205358811,-12.5504981758217,
118.151008083367)) ;
#188041=CARTESIAN_POINT('Ctrl Pts',(-13.3707146606257,-12.4902264670152,
118.194850266941)) ;
#188042=CARTESIAN_POINT('Ctrl Pts',(-13.4445185309104,-12.4902265320198,
118.170619307082)) ;
#188043=CARTESIAN_POINT('Ctrl Pts',(-13.5183224011952,-12.4902265970244,
118.146388347222)) ;
#188044=CARTESIAN_POINT('Ctrl Pts',(-13.5039282764506,-12.5504983058309,
118.102546163647)) ;
#188045=CARTESIAN_POINT('Ctrl Pts',(-13.4139738325163,-12.4070470358761,
117.864151582069)) ;
#188046=CARTESIAN_POINT('Ctrl Pts',(-13.4051020323662,-12.477423987992,
117.837129508225)) ;
#188047=CARTESIAN_POINT('Ctrl Pts',(-13.3312981582326,-12.4774239490789,
117.861360456362)) ;
#188048=CARTESIAN_POINT('Ctrl Pts',(-13.2574942840989,-12.4774239101657,
117.885591404498)) ;
#188049=CARTESIAN_POINT('Ctrl Pts',(-13.266366084249,-12.4070469580498,
117.912613478343)) ;
#188050=CARTESIAN_POINT('Ctrl Pts',(-13.2752378843991,-12.336670005934,
117.939635552187)) ;
#188051=CARTESIAN_POINT('Ctrl Pts',(-13.3490417585328,-12.3366700448471,
117.91540460405)) ;
#188052=CARTESIAN_POINT('Ctrl Pts',(-13.4228456326664,-12.3366700837602,
117.891173655913)) ;
#188053=CARTESIAN_POINT('Ctrl Pts',(-13.4139738325163,-12.4070470358761,
117.864151582069)) ;
#188054=CARTESIAN_POINT('Ctrl Pts',(-13.3156962558462,-12.336806735375,
117.60014657944)) ;
#188055=CARTESIAN_POINT('Ctrl Pts',(-13.3129416529795,-12.4121923869935,
117.591756501563)) ;
#188056=CARTESIAN_POINT('Ctrl Pts',(-13.2391377775031,-12.4121923758419,
117.61598744561)) ;
#188057=CARTESIAN_POINT('Ctrl Pts',(-13.1653339020268,-12.4121923646903,
117.640218389657)) ;
#188058=CARTESIAN_POINT('Ctrl Pts',(-13.1680885048935,-12.3368067130718,
117.648608467534)) ;
#188059=CARTESIAN_POINT('Ctrl Pts',(-13.1708431077602,-12.2614210614532,
117.656998545411)) ;
#188060=CARTESIAN_POINT('Ctrl Pts',(-13.2446469832366,-12.2614210726048,
117.632767601364)) ;
#188061=CARTESIAN_POINT('Ctrl Pts',(-13.3184508587129,-12.2614210837564,
117.608536657317)) ;
#188062=CARTESIAN_POINT('Ctrl Pts',(-13.3156962558462,-12.336806735375,
117.60014657944)) ;
#188063=CARTESIAN_POINT('Ctrl Pts',(-13.2143094352689,-12.343454815208,
117.326830151226)) ;
#188064=CARTESIAN_POINT('Ctrl Pts',(-13.2178948502753,-12.4184892364302,
117.337750744908)) ;
#188065=CARTESIAN_POINT('Ctrl Pts',(-13.1440909762376,-12.4184892524871,
117.361981693338)) ;
#188066=CARTESIAN_POINT('Ctrl Pts',(-13.0702871022,-12.418489268544,117.386212641767)) ;
#188067=CARTESIAN_POINT('Ctrl Pts',(-13.0667016871936,-12.3434548473218,
117.375292048084)) ;
#188068=CARTESIAN_POINT('Ctrl Pts',(-13.0631162721871,-12.2684204260996,
117.364371454402)) ;
#188069=CARTESIAN_POINT('Ctrl Pts',(-13.1369201462248,-12.2684204100427,
117.340140505973)) ;
#188070=CARTESIAN_POINT('Ctrl Pts',(-13.2107240202625,-12.2684203939858,
117.315909557544)) ;
#188071=CARTESIAN_POINT('Ctrl Pts',(-13.2143094352689,-12.343454815208,
117.326830151226)) ;
#188072=CARTESIAN_POINT('Ctrl Pts',(-13.1166976808709,-12.4274004694333,
117.065026003125)) ;
#188073=CARTESIAN_POINT('Ctrl Pts',(-13.1263688309921,-12.4966868092395,
117.094482764137)) ;
#188074=CARTESIAN_POINT('Ctrl Pts',(-13.052564960866,-12.4966868487172,
117.11871372448)) ;
#188075=CARTESIAN_POINT('Ctrl Pts',(-12.9787610907399,-12.496686888195,
117.142944684823)) ;
#188076=CARTESIAN_POINT('Ctrl Pts',(-12.9690899406187,-12.4274005483888,
117.113487923811)) ;
#188077=CARTESIAN_POINT('Ctrl Pts',(-12.9594187904974,-12.3581142085826,
117.084031162799)) ;
#188078=CARTESIAN_POINT('Ctrl Pts',(-13.0332226606235,-12.3581141691049,
117.059800202456)) ;
#188079=CARTESIAN_POINT('Ctrl Pts',(-13.1070265307496,-12.3581141296271,
117.035569242112)) ;
#188080=CARTESIAN_POINT('Ctrl Pts',(-13.1166976808709,-12.4274004694333,
117.065026003125)) ;
#188081=CARTESIAN_POINT('Ctrl Pts',(-13.029296249753,-12.5821548538746,
116.83426577371)) ;
#188082=CARTESIAN_POINT('Ctrl Pts',(-13.0443506263033,-12.6407407748519,
116.880118973957)) ;
#188083=CARTESIAN_POINT('Ctrl Pts',(-12.9705467617918,-12.6407408319528,
116.904349951401)) ;
#188084=CARTESIAN_POINT('Ctrl Pts',(-12.8967428972803,-12.6407408890538,
116.928580928845)) ;
#188085=CARTESIAN_POINT('Ctrl Pts',(-12.88168852073,-12.5821549680765,116.882727728599)) ;
#188086=CARTESIAN_POINT('Ctrl Pts',(-12.8666341441797,-12.5235690470992,
116.836874528352)) ;
#188087=CARTESIAN_POINT('Ctrl Pts',(-12.9404380086912,-12.5235689899983,
116.812643550908)) ;
#188088=CARTESIAN_POINT('Ctrl Pts',(-13.0142418732027,-12.5235689328973,
116.788412573463)) ;
#188089=CARTESIAN_POINT('Ctrl Pts',(-13.029296249753,-12.5821548538746,
116.83426577371)) ;
#188090=CARTESIAN_POINT('Ctrl Pts',(-12.957469185764,-12.7965584285917,
116.650922402553)) ;
#188091=CARTESIAN_POINT('Ctrl Pts',(-12.9768279961232,-12.8402632676504,
116.709886213787)) ;
#188092=CARTESIAN_POINT('Ctrl Pts',(-12.903024138244,-12.8402633354297,
116.734117211432)) ;
#188093=CARTESIAN_POINT('Ctrl Pts',(-12.8292202803647,-12.8402634032089,
116.758348209077)) ;
#188094=CARTESIAN_POINT('Ctrl Pts',(-12.8098614700054,-12.7965585641502,
116.699384397843)) ;
#188095=CARTESIAN_POINT('Ctrl Pts',(-12.7905026596461,-12.7528537250914,
116.640420586608)) ;
#188096=CARTESIAN_POINT('Ctrl Pts',(-12.8643065175254,-12.7528536573122,
116.616189588963)) ;
#188097=CARTESIAN_POINT('Ctrl Pts',(-12.9381103754047,-12.752853589533,
116.591958591318)) ;
#188098=CARTESIAN_POINT('Ctrl Pts',(-12.957469185764,-12.7965584285917,
116.650922402553)) ;
#188099=CARTESIAN_POINT('Ctrl Pts',(-12.9054874508914,-13.0557769277784,
116.528074736688)) ;
#188100=CARTESIAN_POINT('Ctrl Pts',(-12.9277706871717,-13.0814494476449,
116.595945877568)) ;
#188101=CARTESIAN_POINT('Ctrl Pts',(-12.8539668362307,-13.0814495182785,
116.620176896346)) ;
#188102=CARTESIAN_POINT('Ctrl Pts',(-12.7801629852898,-13.0814495889122,
116.644407915124)) ;
#188103=CARTESIAN_POINT('Ctrl Pts',(-12.7578797490096,-13.0557770690457,
116.576536774244)) ;
#188104=CARTESIAN_POINT('Ctrl Pts',(-12.7355965127293,-13.0301045491793,
116.508665633364)) ;
#188105=CARTESIAN_POINT('Ctrl Pts',(-12.8094003636702,-13.0301044785456,
116.484434614586)) ;
#188106=CARTESIAN_POINT('Ctrl Pts',(-12.8832042146112,-13.030104407912,
116.460203595808)) ;
#188107=CARTESIAN_POINT('Ctrl Pts',(-12.9054874508914,-13.0557769277784,
116.528074736688)) ;
#188108=CARTESIAN_POINT('Ctrl Pts',(-12.8764554614161,-13.3412469909538,
116.475159277175)) ;
#188109=CARTESIAN_POINT('Ctrl Pts',(-12.9000646743804,-13.3470269436932,
116.547069129252)) ;
#188110=CARTESIAN_POINT('Ctrl Pts',(-12.826260829751,-13.3470270098198,
116.571300167254)) ;
#188111=CARTESIAN_POINT('Ctrl Pts',(-12.7524569851216,-13.3470270759464,
116.595531205256)) ;
#188112=CARTESIAN_POINT('Ctrl Pts',(-12.7288477721572,-13.341247123207,
116.523621353179)) ;
#188113=CARTESIAN_POINT('Ctrl Pts',(-12.7052385591928,-13.3354671704675,
116.451711501102)) ;
#188114=CARTESIAN_POINT('Ctrl Pts',(-12.7790424038223,-13.335467104341,
116.4274804631)) ;
#188115=CARTESIAN_POINT('Ctrl Pts',(-12.8528462484517,-13.3354670382144,
116.403249425098)) ;
#188116=CARTESIAN_POINT('Ctrl Pts',(-12.8764554614161,-13.3412469909538,
116.475159277175)) ;
#188117=CARTESIAN_POINT('Ctrl Pts',(-12.8717225081288,-13.6316256256215,
116.496181890224)) ;
#188118=CARTESIAN_POINT('Ctrl Pts',(-12.8949646242832,-13.6171399155478,
116.566973624807)) ;
#188119=CARTESIAN_POINT('Ctrl Pts',(-12.8211607846619,-13.6171399723523,
116.591204678062)) ;
#188120=CARTESIAN_POINT('Ctrl Pts',(-12.7473569450405,-13.6171400291567,
116.615435731318)) ;
#188121=CARTESIAN_POINT('Ctrl Pts',(-12.7241148288861,-13.6316257392305,
116.544643996736)) ;
#188122=CARTESIAN_POINT('Ctrl Pts',(-12.7008727127316,-13.6461114493042,
116.473852262154)) ;
#188123=CARTESIAN_POINT('Ctrl Pts',(-12.7746765523529,-13.6461113924997,
116.449621208898)) ;
#188124=CARTESIAN_POINT('Ctrl Pts',(-12.8484803919743,-13.6461113356952,
116.425390155642)) ;
#188125=CARTESIAN_POINT('Ctrl Pts',(-12.8717225081288,-13.6316256256215,
116.496181890224)) ;
#188126=CARTESIAN_POINT('Ctrl Pts',(-12.8907909191923,-13.9070076933881,
116.589733690393)) ;
#188127=CARTESIAN_POINT('Ctrl Pts',(-12.9120028931781,-13.8732725053054,
116.65434193966)) ;
#188128=CARTESIAN_POINT('Ctrl Pts',(-12.8381990569256,-13.8732725490148,
116.678573003177)) ;
#188129=CARTESIAN_POINT('Ctrl Pts',(-12.7643952206731,-13.8732725927241,
116.702804066694)) ;
#188130=CARTESIAN_POINT('Ctrl Pts',(-12.7431832466874,-13.9070077808067,
116.638195817426)) ;
#188131=CARTESIAN_POINT('Ctrl Pts',(-12.7219712727016,-13.9407429688894,
116.573587568159)) ;
#188132=CARTESIAN_POINT('Ctrl Pts',(-12.7957751089541,-13.9407429251801,
116.549356504642)) ;
#188133=CARTESIAN_POINT('Ctrl Pts',(-12.8695789452066,-13.9407428814708,
116.525125441125)) ;
#188134=CARTESIAN_POINT('Ctrl Pts',(-12.8907909191923,-13.9070076933881,
116.589733690393)) ;
#188135=CARTESIAN_POINT('Ctrl Pts',(-12.9317044536525,-14.1476875757229,
116.749883763998)) ;
#188136=CARTESIAN_POINT('Ctrl Pts',(-12.94935668604,-14.0970962848469,116.803649614901)) ;
#188137=CARTESIAN_POINT('Ctrl Pts',(-12.8755528511703,-14.0970963139386,
116.82788068263)) ;
#188138=CARTESIAN_POINT('Ctrl Pts',(-12.8017490163005,-14.0970963430303,
116.852111750358)) ;
#188139=CARTESIAN_POINT('Ctrl Pts',(-12.7840967839129,-14.1476876339063,
116.798345899455)) ;
#188140=CARTESIAN_POINT('Ctrl Pts',(-12.7664445515254,-14.1982789247823,
116.744580048552)) ;
#188141=CARTESIAN_POINT('Ctrl Pts',(-12.8402483863952,-14.1982788956906,
116.720348980823)) ;
#188142=CARTESIAN_POINT('Ctrl Pts',(-12.9140522212649,-14.1982788665989,
116.696117913095)) ;
#188143=CARTESIAN_POINT('Ctrl Pts',(-12.9317044536525,-14.1476875757229,
116.749883763998)) ;
#188144=CARTESIAN_POINT('Ctrl Pts',(-12.9904518256849,-14.3351652655006,
116.964206833377)) ;
#188145=CARTESIAN_POINT('Ctrl Pts',(-13.0032965612653,-14.2714071859544,
117.003329824843)) ;
#188146=CARTESIAN_POINT('Ctrl Pts',(-12.9294927264181,-14.2714072026928,
117.02756089264)) ;
#188147=CARTESIAN_POINT('Ctrl Pts',(-12.8556888915708,-14.2714072194312,
117.051791960437)) ;
#188148=CARTESIAN_POINT('Ctrl Pts',(-12.8428441559903,-14.3351652989775,
117.012668968971)) ;
#188149=CARTESIAN_POINT('Ctrl Pts',(-12.8299994204098,-14.3989233785238,
116.973545977504)) ;
#188150=CARTESIAN_POINT('Ctrl Pts',(-12.9038032552571,-14.3989233617854,
116.949314909707)) ;
#188151=CARTESIAN_POINT('Ctrl Pts',(-12.9776070901044,-14.3989233450469,
116.92508384191)) ;
#188152=CARTESIAN_POINT('Ctrl Pts',(-12.9904518256849,-14.3351652655006,
116.964206833377)) ;
#188153=CARTESIAN_POINT('Ctrl Pts',(-13.0621987371074,-14.4575099619995,
117.218132519493)) ;
#188154=CARTESIAN_POINT('Ctrl Pts',(-13.0693208431459,-14.3851129420045,
117.239825304866)) ;
#188155=CARTESIAN_POINT('Ctrl Pts',(-12.9955170071031,-14.38511294846,117.264056369021)) ;
#188156=CARTESIAN_POINT('Ctrl Pts',(-12.9217131710604,-14.3851129549154,
117.288287433177)) ;
#188157=CARTESIAN_POINT('Ctrl Pts',(-12.9145910650219,-14.4575099749105,
117.266594647805)) ;
#188158=CARTESIAN_POINT('Ctrl Pts',(-12.9074689589835,-14.5299069949055,
117.244901862432)) ;
#188159=CARTESIAN_POINT('Ctrl Pts',(-12.9812727950263,-14.52990698845,117.220670798277)) ;
#188160=CARTESIAN_POINT('Ctrl Pts',(-13.055076631069,-14.5299069819946,
117.196439734121)) ;
#188161=CARTESIAN_POINT('Ctrl Pts',(-13.0621987371074,-14.4575099619995,
117.218132519493)) ;
#188162=CARTESIAN_POINT('Ctrl Pts',(-13.1416934201426,-14.5055206620573,
117.495908283019)) ;
#188163=CARTESIAN_POINT('Ctrl Pts',(-13.1425378898428,-14.4296611949973,
117.498480401175)) ;
#188164=CARTESIAN_POINT('Ctrl Pts',(-13.0687340512145,-14.4296611947843,
117.522711457456)) ;
#188165=CARTESIAN_POINT('Ctrl Pts',(-12.9949302125861,-14.4296611945714,
117.546942513736)) ;
#188166=CARTESIAN_POINT('Ctrl Pts',(-12.9940857428859,-14.5055206616315,
117.54437039558)) ;
#188167=CARTESIAN_POINT('Ctrl Pts',(-12.9932412731857,-14.5813801286916,
117.541798277423)) ;
#188168=CARTESIAN_POINT('Ctrl Pts',(-13.067045111814,-14.5813801289045,
117.517567221143)) ;
#188169=CARTESIAN_POINT('Ctrl Pts',(-13.1408489504423,-14.5813801291174,
117.493336164862)) ;
#188170=CARTESIAN_POINT('Ctrl Pts',(-13.1416934201426,-14.5055206620573,
117.495908283019)) ;
#188171=CARTESIAN_POINT('Ctrl Pts',(-13.2212073264965,-14.4754288487564,
117.773416266333)) ;
#188172=CARTESIAN_POINT('Ctrl Pts',(-13.2157700751089,-14.4015565166022,
117.756855275716)) ;
#188173=CARTESIAN_POINT('Ctrl Pts',(-13.1419662346049,-14.4015565138437,
117.781086326283)) ;
#188174=CARTESIAN_POINT('Ctrl Pts',(-13.0681623941008,-14.4015565110851,
117.805317376851)) ;
#188175=CARTESIAN_POINT('Ctrl Pts',(-13.0735996454884,-14.4754288432393,
117.821878367468)) ;
#188176=CARTESIAN_POINT('Ctrl Pts',(-13.0790368968761,-14.5493011753935,
117.838439358085)) ;
#188177=CARTESIAN_POINT('Ctrl Pts',(-13.1528407373801,-14.5493011781521,
117.814208307518)) ;
#188178=CARTESIAN_POINT('Ctrl Pts',(-13.2266445778842,-14.5493011809106,
117.78997725695)) ;
#188179=CARTESIAN_POINT('Ctrl Pts',(-13.2212073264965,-14.4754288487564,
117.773416266333)) ;
#188180=CARTESIAN_POINT('Ctrl Pts',(-13.2954245315983,-14.3696969300058,
118.034975562768)) ;
#188181=CARTESIAN_POINT('Ctrl Pts',(-13.2840619904211,-14.3030961668257,
118.00036709561)) ;
#188182=CARTESIAN_POINT('Ctrl Pts',(-13.2102581479488,-14.3030961645972,
118.024598140183)) ;
#188183=CARTESIAN_POINT('Ctrl Pts',(-13.1364543054765,-14.3030961623686,
118.048829184755)) ;
#188184=CARTESIAN_POINT('Ctrl Pts',(-13.1478168466536,-14.3696969255486,
118.083437651913)) ;
#188185=CARTESIAN_POINT('Ctrl Pts',(-13.1591793878308,-14.4362976887287,
118.118046119071)) ;
#188186=CARTESIAN_POINT('Ctrl Pts',(-13.2329832303031,-14.4362976909572,
118.093815074498)) ;
#188187=CARTESIAN_POINT('Ctrl Pts',(-13.3067870727754,-14.4362976931858,
118.069584029926)) ;
#188188=CARTESIAN_POINT('Ctrl Pts',(-13.2954245315983,-14.3696969300058,
118.034975562768)) ;
#188189=CARTESIAN_POINT('Ctrl Pts',(-13.3577857668099,-14.1954536297215,
118.260415901486)) ;
#188190=CARTESIAN_POINT('Ctrl Pts',(-13.3413169958214,-14.1409200386093,
118.210254682291)) ;
#188191=CARTESIAN_POINT('Ctrl Pts',(-13.2675131522284,-14.1409200387787,
118.23448572345)) ;
#188192=CARTESIAN_POINT('Ctrl Pts',(-13.1937093086354,-14.1409200389481,
118.258716764609)) ;
#188193=CARTESIAN_POINT('Ctrl Pts',(-13.2101780796239,-14.1954536300603,
118.308877983803)) ;
#188194=CARTESIAN_POINT('Ctrl Pts',(-13.2266468506125,-14.2499872211724,
118.359039202998)) ;
#188195=CARTESIAN_POINT('Ctrl Pts',(-13.3004506942055,-14.249987221003,
118.334808161839)) ;
#188196=CARTESIAN_POINT('Ctrl Pts',(-13.3742545377985,-14.2499872208336,
118.31057712068)) ;
#188197=CARTESIAN_POINT('Ctrl Pts',(-13.3577857668099,-14.1954536297215,
118.260415901486)) ;
#188198=CARTESIAN_POINT('Ctrl Pts',(-13.4030472404078,-13.9663067477415,
118.433665970609)) ;
#188199=CARTESIAN_POINT('Ctrl Pts',(-13.3826610350393,-13.9276927071092,
118.371572878415)) ;
#188200=CARTESIAN_POINT('Ctrl Pts',(-13.308857191142,-13.9276927095559,
118.395803918647)) ;
#188201=CARTESIAN_POINT('Ctrl Pts',(-13.2350533472446,-13.9276927120025,
118.420034958879)) ;
#188202=CARTESIAN_POINT('Ctrl Pts',(-13.255439552613,-13.9663067526349,
118.482128051073)) ;
#188203=CARTESIAN_POINT('Ctrl Pts',(-13.2758257579814,-14.0049207932672,
118.544221143267)) ;
#188204=CARTESIAN_POINT('Ctrl Pts',(-13.3496296018788,-14.0049207908205,
118.519990103035)) ;
#188205=CARTESIAN_POINT('Ctrl Pts',(-13.4234334457761,-14.0049207883739,
118.495759062804)) ;
#188206=CARTESIAN_POINT('Ctrl Pts',(-13.4030472404078,-13.9663067477415,
118.433665970609)) ;
#188207=CARTESIAN_POINT('Ctrl Pts',(-13.4274257673163,-13.6964880977043,
118.543501361886)) ;
#188208=CARTESIAN_POINT('Ctrl Pts',(-13.4045704519705,-13.6766583743927,
118.473887759096)) ;
#188209=CARTESIAN_POINT('Ctrl Pts',(-13.3307666083207,-13.6766583775101,
118.498118800081)) ;
#188210=CARTESIAN_POINT('Ctrl Pts',(-13.2569627646708,-13.6766583806274,
118.522349841067)) ;
#188211=CARTESIAN_POINT('Ctrl Pts',(-13.2798180800167,-13.696488103939,
118.591963443857)) ;
#188212=CARTESIAN_POINT('Ctrl Pts',(-13.3026733953625,-13.7163178272505,
118.661577046648)) ;
#188213=CARTESIAN_POINT('Ctrl Pts',(-13.3764772390123,-13.7163178241332,
118.637346005662)) ;
#188214=CARTESIAN_POINT('Ctrl Pts',(-13.4502810826622,-13.7163178210159,
118.613114964676)) ;
#188215=CARTESIAN_POINT('Ctrl Pts',(-13.4274257673163,-13.6964880977043,
118.543501361886)) ;
#188216=CARTESIAN_POINT('Ctrl Pts',(-13.4282463775527,-13.4086720240795,
118.581326099254)) ;
#188217=CARTESIAN_POINT('Ctrl Pts',(-13.4045691840501,-13.4089104896533,
118.509209188176)) ;
#188218=CARTESIAN_POINT('Ctrl Pts',(-13.3307653407294,-13.4089104912241,
118.533440230164)) ;
#188219=CARTESIAN_POINT('Ctrl Pts',(-13.2569614974086,-13.408910492795,
118.557671272153)) ;
#188220=CARTESIAN_POINT('Ctrl Pts',(-13.2806386909112,-13.4086720272212,
118.62978818323)) ;
#188221=CARTESIAN_POINT('Ctrl Pts',(-13.3043158844138,-13.4084335616475,
118.701905094307)) ;
#188222=CARTESIAN_POINT('Ctrl Pts',(-13.3781197277346,-13.4084335600766,
118.677674052319)) ;
#188223=CARTESIAN_POINT('Ctrl Pts',(-13.4519235710553,-13.4084335585058,
118.653443010331)) ;
#188224=CARTESIAN_POINT('Ctrl Pts',(-13.4282463775527,-13.4086720240795,
118.581326099254)) ;
#188225=CARTESIAN_POINT('Ctrl Pts',(-13.4047342363666,-13.1198463580562,
118.545258189768)) ;
#188226=CARTESIAN_POINT('Ctrl Pts',(-13.3819284192765,-13.1402531049797,
118.475795350571)) ;
#188227=CARTESIAN_POINT('Ctrl Pts',(-13.3081245757733,-13.1402531026116,
118.500026392003)) ;
#188228=CARTESIAN_POINT('Ctrl Pts',(-13.2343207322702,-13.1402531002435,
118.524257433436)) ;
#188229=CARTESIAN_POINT('Ctrl Pts',(-13.2571265493602,-13.1198463533199,
118.593720272633)) ;
#188230=CARTESIAN_POINT('Ctrl Pts',(-13.2799323664503,-13.0994396063964,
118.663183111831)) ;
#188231=CARTESIAN_POINT('Ctrl Pts',(-13.3537362099535,-13.0994396087645,
118.638952070398)) ;
#188232=CARTESIAN_POINT('Ctrl Pts',(-13.4275400534566,-13.0994396111326,
118.614721028966)) ;
#188233=CARTESIAN_POINT('Ctrl Pts',(-13.4047342363666,-13.1198463580562,
118.545258189768)) ;
#188234=CARTESIAN_POINT('Ctrl Pts',(-13.3580365344568,-12.8536440540051,
118.438389162205)) ;
#188235=CARTESIAN_POINT('Ctrl Pts',(-13.3377263303549,-12.8926679376459,
118.376527557416)) ;
#188236=CARTESIAN_POINT('Ctrl Pts',(-13.2639224859729,-12.8926679313973,
118.400758596172)) ;
#188237=CARTESIAN_POINT('Ctrl Pts',(-13.1901186415909,-12.8926679251486,
118.424989634928)) ;
#188238=CARTESIAN_POINT('Ctrl Pts',(-13.2104288456928,-12.8536440415079,
118.486851239717)) ;
#188239=CARTESIAN_POINT('Ctrl Pts',(-13.2307390497946,-12.8146201578671,
118.548712844506)) ;
#188240=CARTESIAN_POINT('Ctrl Pts',(-13.3045428941766,-12.8146201641158,
118.52448180575)) ;
#188241=CARTESIAN_POINT('Ctrl Pts',(-13.3783467385586,-12.8146201703644,
118.500250766995)) ;
#188242=CARTESIAN_POINT('Ctrl Pts',(-13.3580365344568,-12.8536440540051,
118.438389162205)) ;
#188243=CARTESIAN_POINT('Ctrl Pts',(-13.2900338474699,-12.6260691585523,
118.266921417924)) ;
#188244=CARTESIAN_POINT('Ctrl Pts',(-13.2737043319057,-12.6810405314409,
118.217184347987)) ;
#188245=CARTESIAN_POINT('Ctrl Pts',(-13.19990048528,-12.6810405208292,118.241415379908)) ;
#188246=CARTESIAN_POINT('Ctrl Pts',(-13.1260966386543,-12.6810405102175,
118.26564641183)) ;
#188247=CARTESIAN_POINT('Ctrl Pts',(-13.1424261542185,-12.6260691373289,
118.315383481767)) ;
#188248=CARTESIAN_POINT('Ctrl Pts',(-13.1587556697827,-12.5710977644403,
118.365120551704)) ;
#188249=CARTESIAN_POINT('Ctrl Pts',(-13.2325595164084,-12.571097775052,
118.340889519783)) ;
#188250=CARTESIAN_POINT('Ctrl Pts',(-13.3063633630341,-12.5710977856637,
118.316658487861)) ;
#188251=CARTESIAN_POINT('Ctrl Pts',(-13.2900338474699,-12.6260691585523,
118.266921417924)) ;
#188252=CARTESIAN_POINT('Ctrl Pts',(-13.2058856946641,-12.4569456938658,
118.045990431136)) ;
#188253=CARTESIAN_POINT('Ctrl Pts',(-13.1946760329366,-12.5238051277268,
118.01184760977)) ;
#188254=CARTESIAN_POINT('Ctrl Pts',(-13.1208721836935,-12.5238051170314,
118.03607863372)) ;
#188255=CARTESIAN_POINT('Ctrl Pts',(-13.0470683344505,-12.523805106336,
118.06030965767)) ;
#188256=CARTESIAN_POINT('Ctrl Pts',(-13.058277996178,-12.4569456724751,
118.094452479035)) ;
#188257=CARTESIAN_POINT('Ctrl Pts',(-13.0694876579055,-12.3900862386142,
118.128595300401)) ;
#188258=CARTESIAN_POINT('Ctrl Pts',(-13.1432915071485,-12.3900862493095,
118.104364276451)) ;
#188259=CARTESIAN_POINT('Ctrl Pts',(-13.2170953563916,-12.3900862600049,
118.080133252501)) ;
#188260=CARTESIAN_POINT('Ctrl Pts',(-13.2058856946641,-12.4569456938658,
118.045990431136)) ;
#188261=CARTESIAN_POINT('Ctrl Pts',(-13.1099984077294,-12.3560371763605,
117.789461557574)) ;
#188262=CARTESIAN_POINT('Ctrl Pts',(-13.1047323153025,-12.4300391766208,
117.773421889139)) ;
#188263=CARTESIAN_POINT('Ctrl Pts',(-13.0309284627601,-12.43003916942,117.79765290304)) ;
#188264=CARTESIAN_POINT('Ctrl Pts',(-12.9571246102177,-12.4300391622191,
117.82188391694)) ;
#188265=CARTESIAN_POINT('Ctrl Pts',(-12.9623907026446,-12.3560371619588,
117.837923585375)) ;
#188266=CARTESIAN_POINT('Ctrl Pts',(-12.9676567950715,-12.2820351616984,
117.853963253809)) ;
#188267=CARTESIAN_POINT('Ctrl Pts',(-13.0414606476139,-12.2820351688993,
117.829732239909)) ;
#188268=CARTESIAN_POINT('Ctrl Pts',(-13.1152645001563,-12.2820351761001,
117.805501226008)) ;
#188269=CARTESIAN_POINT('Ctrl Pts',(-13.1099984077294,-12.3560371763605,
117.789461557574)) ;
#188270=CARTESIAN_POINT('Ctrl Pts',(-13.0093871644828,-12.3312869891021,
117.518335932488)) ;
#188271=CARTESIAN_POINT('Ctrl Pts',(-13.0104073119892,-12.407123602134,
117.521443136472)) ;
#188272=CARTESIAN_POINT('Ctrl Pts',(-12.9366034569471,-12.4071236031691,
117.545674142759)) ;
#188273=CARTESIAN_POINT('Ctrl Pts',(-12.862799601905,-12.4071236042042,
117.569905149046)) ;
#188274=CARTESIAN_POINT('Ctrl Pts',(-12.8617794543986,-12.3312869911723,
117.566797945062)) ;
#188275=CARTESIAN_POINT('Ctrl Pts',(-12.8607593068922,-12.2554503781403,
117.563690741078)) ;
#188276=CARTESIAN_POINT('Ctrl Pts',(-12.9345631619343,-12.2554503771052,
117.539459734791)) ;
#188277=CARTESIAN_POINT('Ctrl Pts',(-13.0083670169764,-12.2554503760701,
117.515228728505)) ;
#188278=CARTESIAN_POINT('Ctrl Pts',(-13.0093871644828,-12.3312869891021,
117.518335932488)) ;
#188279=CARTESIAN_POINT('Ctrl Pts',(-12.9090497943827,-12.384579728798,
117.248374706076)) ;
#188280=CARTESIAN_POINT('Ctrl Pts',(-12.916339277386,-12.4568056181836,
117.270577294226)) ;
#188281=CARTESIAN_POINT('Ctrl Pts',(-12.8425354197324,-12.4568056323219,
117.294808292558)) ;
#188282=CARTESIAN_POINT('Ctrl Pts',(-12.7687315620788,-12.4568056464601,
117.319039290891)) ;
#188283=CARTESIAN_POINT('Ctrl Pts',(-12.7614420790756,-12.3845797570745,
117.296836702741)) ;
#188284=CARTESIAN_POINT('Ctrl Pts',(-12.7541525960724,-12.3123538676888,
117.274634114591)) ;
#188285=CARTESIAN_POINT('Ctrl Pts',(-12.8279564537259,-12.3123538535506,
117.250403116258)) ;
#188286=CARTESIAN_POINT('Ctrl Pts',(-12.9017603113795,-12.3123538394123,
117.226172117926)) ;
#188287=CARTESIAN_POINT('Ctrl Pts',(-12.9090497943827,-12.384579728798,
117.248374706076)) ;
#188288=CARTESIAN_POINT('Ctrl Pts',(-12.8169551777731,-12.5118388251457,
117.003294087217)) ;
#188289=CARTESIAN_POINT('Ctrl Pts',(-12.8299521097154,-12.5752838792253,
117.042880643781)) ;
#188290=CARTESIAN_POINT('Ctrl Pts',(-12.7561482516071,-12.5752839097083,
117.067111640729)) ;
#188291=CARTESIAN_POINT('Ctrl Pts',(-12.6823443934988,-12.5752839401913,
117.091342637677)) ;
#188292=CARTESIAN_POINT('Ctrl Pts',(-12.6693474615566,-12.5118388861117,
117.051756081112)) ;
#188293=CARTESIAN_POINT('Ctrl Pts',(-12.6563505296143,-12.448393832032,
117.012169524548)) ;
#188294=CARTESIAN_POINT('Ctrl Pts',(-12.7301543877226,-12.4483938015491,
116.9879385276)) ;
#188295=CARTESIAN_POINT('Ctrl Pts',(-12.8039582458309,-12.4483937710661,
116.963707530652)) ;
#188296=CARTESIAN_POINT('Ctrl Pts',(-12.8169551777731,-12.5118388251457,
117.003294087217)) ;
#188297=CARTESIAN_POINT('Ctrl Pts',(-12.7382168138023,-12.7038857020727,
116.798924647324)) ;
#188298=CARTESIAN_POINT('Ctrl Pts',(-12.755996265204,-12.7540141068732,
116.853077986343)) ;
#188299=CARTESIAN_POINT('Ctrl Pts',(-12.6821924084334,-12.7540141550584,
116.877308987365)) ;
#188300=CARTESIAN_POINT('Ctrl Pts',(-12.6083885516627,-12.7540142032436,
116.901539988387)) ;
#188301=CARTESIAN_POINT('Ctrl Pts',(-12.5906091002609,-12.7038857984431,
116.847386649367)) ;
#188302=CARTESIAN_POINT('Ctrl Pts',(-12.5728296488592,-12.6537573936426,
116.793233310347)) ;
#188303=CARTESIAN_POINT('Ctrl Pts',(-12.6466335056298,-12.6537573454574,
116.769002309326)) ;
#188304=CARTESIAN_POINT('Ctrl Pts',(-12.7204373624006,-12.6537572972722,
116.744771308304)) ;
#188305=CARTESIAN_POINT('Ctrl Pts',(-12.7382168138023,-12.7038857020727,
116.798924647324)) ;
#188306=CARTESIAN_POINT('Ctrl Pts',(-12.6778922634921,-12.9467051649881,
116.650586228922)) ;
#188307=CARTESIAN_POINT('Ctrl Pts',(-12.6991766219081,-12.9799528972862,
116.715414949048)) ;
#188308=CARTESIAN_POINT('Ctrl Pts',(-12.6253727686005,-12.9799529618983,
116.739645960617)) ;
#188309=CARTESIAN_POINT('Ctrl Pts',(-12.5515689152929,-12.9799530265103,
116.763876972187)) ;
#188310=CARTESIAN_POINT('Ctrl Pts',(-12.5302845568768,-12.9467052942123,
116.699048252061)) ;
#188311=CARTESIAN_POINT('Ctrl Pts',(-12.5090001984607,-12.9134575619143,
116.634219531935)) ;
#188312=CARTESIAN_POINT('Ctrl Pts',(-12.5828040517684,-12.9134574973022,
116.609988520366)) ;
#188313=CARTESIAN_POINT('Ctrl Pts',(-12.656607905076,-12.9134574326901,
116.585757508796)) ;
#188314=CARTESIAN_POINT('Ctrl Pts',(-12.6778922634921,-12.9467051649881,
116.650586228922)) ;
#188315=CARTESIAN_POINT('Ctrl Pts',(-12.6393672663025,-13.2232753780377,
116.568664349212)) ;
#188316=CARTESIAN_POINT('Ctrl Pts',(-12.6626392596797,-13.237261879662,
116.639547084586)) ;
#188317=CARTESIAN_POINT('Ctrl Pts',(-12.588835411666,-13.237261957473,116.66377811228)) ;
#188318=CARTESIAN_POINT('Ctrl Pts',(-12.5150315636522,-13.237262035284,
116.688009139974)) ;
#188319=CARTESIAN_POINT('Ctrl Pts',(-12.4917595702749,-13.2232755336597,
116.617126404599)) ;
#188320=CARTESIAN_POINT('Ctrl Pts',(-12.4684875768976,-13.2092890320355,
116.546243669225)) ;
#188321=CARTESIAN_POINT('Ctrl Pts',(-12.5422914249114,-13.2092889542245,
116.522012641531)) ;
#188322=CARTESIAN_POINT('Ctrl Pts',(-12.6160952729252,-13.2092888764135,
116.497781613838)) ;
#188323=CARTESIAN_POINT('Ctrl Pts',(-12.6393672663025,-13.2232753780377,
116.568664349212)) ;
#188324=CARTESIAN_POINT('Ctrl Pts',(-12.6246970514702,-13.5141286997517,
116.5594436943)) ;
#188325=CARTESIAN_POINT('Ctrl Pts',(-12.6482932870681,-13.5078290678433,
116.631314019028)) ;
#188326=CARTESIAN_POINT('Ctrl Pts',(-12.5744894458595,-13.5078291537003,
116.655545067449)) ;
#188327=CARTESIAN_POINT('Ctrl Pts',(-12.500685604651,-13.5078292395572,
116.679776115871)) ;
#188328=CARTESIAN_POINT('Ctrl Pts',(-12.4770893690531,-13.5141288714655,
116.607905791143)) ;
#188329=CARTESIAN_POINT('Ctrl Pts',(-12.4534931334552,-13.5204285033738,
116.536035466415)) ;
#188330=CARTESIAN_POINT('Ctrl Pts',(-12.5272969746638,-13.5204284175169,
116.511804417994)) ;
#188331=CARTESIAN_POINT('Ctrl Pts',(-12.6011008158723,-13.52042833166,116.487573369573)) ;
#188332=CARTESIAN_POINT('Ctrl Pts',(-12.6246970514702,-13.5141286997517,
116.5594436943)) ;
#188333=CARTESIAN_POINT('Ctrl Pts',(-12.6342523291232,-13.7984771926956,
116.624052868779)) ;
#188334=CARTESIAN_POINT('Ctrl Pts',(-12.6564811749019,-13.7723162248091,
116.69175834462)) ;
#188335=CARTESIAN_POINT('Ctrl Pts',(-12.5826773414463,-13.7723163117777,
116.715989416656)) ;
#188336=CARTESIAN_POINT('Ctrl Pts',(-12.5088735079907,-13.7723163987464,
116.740220488691)) ;
#188337=CARTESIAN_POINT('Ctrl Pts',(-12.486644662212,-13.7984773666329,
116.672515012851)) ;
#188338=CARTESIAN_POINT('Ctrl Pts',(-12.4644158164333,-13.8246383345194,
116.60480953701)) ;
#188339=CARTESIAN_POINT('Ctrl Pts',(-12.5382196498889,-13.8246382475507,
116.580578464974)) ;
#188340=CARTESIAN_POINT('Ctrl Pts',(-12.6120234833445,-13.8246381605821,
116.556347392938)) ;
#188341=CARTESIAN_POINT('Ctrl Pts',(-12.6342523291232,-13.7984771926956,
116.624052868779)) ;
#188342=CARTESIAN_POINT('Ctrl Pts',(-12.6667338754881,-14.0556517682192,
116.758530399118)) ;
#188343=CARTESIAN_POINT('Ctrl Pts',(-12.6859920465302,-14.0114975765456,
116.817187678919)) ;
#188344=CARTESIAN_POINT('Ctrl Pts',(-12.6121882209902,-14.011497656322,
116.841418775065)) ;
#188345=CARTESIAN_POINT('Ctrl Pts',(-12.5383843954502,-14.0114977360984,
116.86564987121)) ;
#188346=CARTESIAN_POINT('Ctrl Pts',(-12.5191262244081,-14.055651927772,
116.806992591408)) ;
#188347=CARTESIAN_POINT('Ctrl Pts',(-12.4998680533661,-14.0998061194455,
116.748335311607)) ;
#188348=CARTESIAN_POINT('Ctrl Pts',(-12.5736718789061,-14.0998060396691,
116.724104215462)) ;
#188349=CARTESIAN_POINT('Ctrl Pts',(-12.6474757044461,-14.0998059598928,
116.699873119317)) ;
#188350=CARTESIAN_POINT('Ctrl Pts',(-12.6667338754881,-14.0556517682192,
116.758530399118)) ;
#188351=CARTESIAN_POINT('Ctrl Pts',(-12.7185614877042,-14.2658619034502,
116.951700772076)) ;
#188352=CARTESIAN_POINT('Ctrl Pts',(-12.7334986348115,-14.206967241119,
116.997196910099)) ;
#188353=CARTESIAN_POINT('Ctrl Pts',(-12.6596948160871,-14.2069673051098,
117.021428027003)) ;
#188354=CARTESIAN_POINT('Ctrl Pts',(-12.5858909973627,-14.2069673691006,
117.045659143907)) ;
#188355=CARTESIAN_POINT('Ctrl Pts',(-12.5709538502553,-14.2658620314317,
117.000163005885)) ;
#188356=CARTESIAN_POINT('Ctrl Pts',(-12.5560167031479,-14.3247566937629,
116.954666867862)) ;
#188357=CARTESIAN_POINT('Ctrl Pts',(-12.6298205218724,-14.3247566297721,
116.930435750958)) ;
#188358=CARTESIAN_POINT('Ctrl Pts',(-12.7036243405968,-14.3247565657813,
116.906204634054)) ;
#188359=CARTESIAN_POINT('Ctrl Pts',(-12.7185614877042,-14.2658619034502,
116.951700772076)) ;
#188360=CARTESIAN_POINT('Ctrl Pts',(-12.7861042651264,-14.4169100671748,
117.193039609464)) ;
#188361=CARTESIAN_POINT('Ctrl Pts',(-12.7956109926747,-14.3473831262014,
117.221995565631)) ;
#188362=CARTESIAN_POINT('Ctrl Pts',(-12.721807179474,-14.3473831682741,
117.246226699359)) ;
#188363=CARTESIAN_POINT('Ctrl Pts',(-12.6480033662733,-14.3473832103469,
117.270457833088)) ;
#188364=CARTESIAN_POINT('Ctrl Pts',(-12.638496638725,-14.4169101513204,
117.241501876921)) ;
#188365=CARTESIAN_POINT('Ctrl Pts',(-12.6289899111766,-14.4864370922939,
117.212545920754)) ;
#188366=CARTESIAN_POINT('Ctrl Pts',(-12.7027937243773,-14.4864370502211,
117.188314787025)) ;
#188367=CARTESIAN_POINT('Ctrl Pts',(-12.776597537578,-14.4864370081483,
117.164083653297)) ;
#188368=CARTESIAN_POINT('Ctrl Pts',(-12.7861042651264,-14.4169100671748,
117.193039609464)) ;
#188369=CARTESIAN_POINT('Ctrl Pts',(-12.8630657685899,-14.4953742453793,
117.462914929122)) ;
#188370=CARTESIAN_POINT('Ctrl Pts',(-12.8664795502472,-14.4202668072197,
117.473312755161)) ;
#188371=CARTESIAN_POINT('Ctrl Pts',(-12.7926757400385,-14.4202668221935,
117.497543898003)) ;
#188372=CARTESIAN_POINT('Ctrl Pts',(-12.7188719298299,-14.4202668371673,
117.521775040845)) ;
#188373=CARTESIAN_POINT('Ctrl Pts',(-12.7154581481725,-14.495374275327,
117.511377214806)) ;
#188374=CARTESIAN_POINT('Ctrl Pts',(-12.7120443665152,-14.5704817134867,
117.500979388766)) ;
#188375=CARTESIAN_POINT('Ctrl Pts',(-12.7858481767239,-14.5704816985128,
117.476748245924)) ;
#188376=CARTESIAN_POINT('Ctrl Pts',(-12.8596519869325,-14.570481683539,
117.452517103082)) ;
#188377=CARTESIAN_POINT('Ctrl Pts',(-12.8630657685899,-14.4953742453793,
117.462914929122)) ;
#188378=CARTESIAN_POINT('Ctrl Pts',(-12.9430874779425,-14.4969828286805,
117.741985737709)) ;
#188379=CARTESIAN_POINT('Ctrl Pts',(-12.9401882473644,-14.4216525600046,
117.733155147064)) ;
#188380=CARTESIAN_POINT('Ctrl Pts',(-12.8663844374637,-14.4216525461531,
117.757386290844)) ;
#188381=CARTESIAN_POINT('Ctrl Pts',(-12.7925806275628,-14.4216525323015,
117.781617434623)) ;
#188382=CARTESIAN_POINT('Ctrl Pts',(-12.7954798581409,-14.4969828009775,
117.790448025268)) ;
#188383=CARTESIAN_POINT('Ctrl Pts',(-12.7983790887189,-14.5723130696534,
117.799278615913)) ;
#188384=CARTESIAN_POINT('Ctrl Pts',(-12.8721828986197,-14.5723130835049,
117.775047472134)) ;
#188385=CARTESIAN_POINT('Ctrl Pts',(-12.9459867085205,-14.5723130973564,
117.750816328354)) ;
#188386=CARTESIAN_POINT('Ctrl Pts',(-12.9430874779425,-14.4969828286805,
117.741985737709)) ;
#188387=CARTESIAN_POINT('Ctrl Pts',(-13.0203177415346,-14.421551875411,
118.012685171403)) ;
#188388=CARTESIAN_POINT('Ctrl Pts',(-13.0112884091571,-14.3513763125925,
117.985183279766)) ;
#188389=CARTESIAN_POINT('Ctrl Pts',(-12.9374845968934,-14.3513762706419,
118.009414416348)) ;
#188390=CARTESIAN_POINT('Ctrl Pts',(-12.8636807846298,-14.3513762286912,
118.033645552931)) ;
#188391=CARTESIAN_POINT('Ctrl Pts',(-12.8727101170073,-14.4215517915098,
118.061147444569)) ;
#188392=CARTESIAN_POINT('Ctrl Pts',(-12.8817394493848,-14.4917273543283,
118.088649336206)) ;
#188393=CARTESIAN_POINT('Ctrl Pts',(-12.9555432616484,-14.491727396279,
118.064418199623)) ;
#188394=CARTESIAN_POINT('Ctrl Pts',(-13.029347073912,-14.4917274382296,
118.04018706304)) ;
#188395=CARTESIAN_POINT('Ctrl Pts',(-13.0203177415346,-14.421551875411,
118.012685171403)) ;
#188396=CARTESIAN_POINT('Ctrl Pts',(-13.0883258543975,-14.2735000710325,
118.255405538239)) ;
#188397=CARTESIAN_POINT('Ctrl Pts',(-13.0737988185205,-14.213556255384,
118.211158528823)) ;
#188398=CARTESIAN_POINT('Ctrl Pts',(-12.9999950012594,-14.2135561892348,
118.235389650184)) ;
#188399=CARTESIAN_POINT('Ctrl Pts',(-12.9261911839982,-14.2135561230857,
118.259620771545)) ;
#188400=CARTESIAN_POINT('Ctrl Pts',(-12.9407182198752,-14.2734999387342,
118.303867780962)) ;
#188401=CARTESIAN_POINT('Ctrl Pts',(-12.9552452557522,-14.3334437543827,
118.348114790378)) ;
#188402=CARTESIAN_POINT('Ctrl Pts',(-13.0290490730134,-14.3334438205319,
118.323883669017)) ;
#188403=CARTESIAN_POINT('Ctrl Pts',(-13.1028528902745,-14.3334438866811,
118.299652547656)) ;
#188404=CARTESIAN_POINT('Ctrl Pts',(-13.0883258543975,-14.2735000710325,
118.255405538239)) ;
#188405=CARTESIAN_POINT('Ctrl Pts',(-13.141058050103,-14.0646532706665,
118.451466458674)) ;
#188406=CARTESIAN_POINT('Ctrl Pts',(-13.1220942972562,-14.019201123048,
118.393705925278)) ;
#188407=CARTESIAN_POINT('Ctrl Pts',(-13.0482904731012,-14.0192010389841,
118.417937025641)) ;
#188408=CARTESIAN_POINT('Ctrl Pts',(-12.9744866489462,-14.0192009549201,
118.442168126005)) ;
#188409=CARTESIAN_POINT('Ctrl Pts',(-12.9934504017929,-14.0646531025386,
118.499928659402)) ;
#188410=CARTESIAN_POINT('Ctrl Pts',(-13.0124141546397,-14.110105250157,
118.557689192798)) ;
#188411=CARTESIAN_POINT('Ctrl Pts',(-13.0862179787947,-14.110105334221,
118.533458092435)) ;
#188412=CARTESIAN_POINT('Ctrl Pts',(-13.1600218029498,-14.1101054182849,
118.509226992071)) ;
#188413=CARTESIAN_POINT('Ctrl Pts',(-13.141058050103,-14.0646532706665,
118.451466458674)) ;
#188414=CARTESIAN_POINT('Ctrl Pts',(-13.174281067565,-13.8091818841456,
118.588155479857)) ;
#188415=CARTESIAN_POINT('Ctrl Pts',(-13.1522348887302,-13.7814979528365,
118.521006374321)) ;
#188416=CARTESIAN_POINT('Ctrl Pts',(-13.0784310564862,-13.7814978588796,
118.545237450047)) ;
#188417=CARTESIAN_POINT('Ctrl Pts',(-13.0046272242423,-13.7814977649226,
118.569468525773)) ;
#188418=CARTESIAN_POINT('Ctrl Pts',(-13.0266734030771,-13.8091816962316,
118.636617631309)) ;
#188419=CARTESIAN_POINT('Ctrl Pts',(-13.048719581912,-13.8368656275406,
118.703766736846)) ;
#188420=CARTESIAN_POINT('Ctrl Pts',(-13.1225234141559,-13.8368657214976,
118.679535661119)) ;
#188421=CARTESIAN_POINT('Ctrl Pts',(-13.1963272463998,-13.8368658154546,
118.655304585393)) ;
#188422=CARTESIAN_POINT('Ctrl Pts',(-13.174281067565,-13.8091818841456,
118.588155479857)) ;
#188423=CARTESIAN_POINT('Ctrl Pts',(-13.1847943926898,-13.5266904596517,
118.655545948521)) ;
#188424=CARTESIAN_POINT('Ctrl Pts',(-13.1612493680941,-13.5186880514058,
118.583831600714)) ;
#188425=CARTESIAN_POINT('Ctrl Pts',(-13.0874455275475,-13.5186879553988,
118.608062651152)) ;
#188426=CARTESIAN_POINT('Ctrl Pts',(-13.0136416870009,-13.5186878593918,
118.632293701589)) ;
#188427=CARTESIAN_POINT('Ctrl Pts',(-13.0371867115966,-13.5266902676377,
118.704008049396)) ;
#188428=CARTESIAN_POINT('Ctrl Pts',(-13.0607317361924,-13.5346926758837,
118.775722397203)) ;
#188429=CARTESIAN_POINT('Ctrl Pts',(-13.134535576739,-13.5346927718906,
118.751491346766)) ;
#188430=CARTESIAN_POINT('Ctrl Pts',(-13.2083394172856,-13.5346928678976,
118.727260296328)) ;
#188431=CARTESIAN_POINT('Ctrl Pts',(-13.1847943926898,-13.5266904596517,
118.655545948521)) ;
#188432=CARTESIAN_POINT('Ctrl Pts',(-13.1711799492058,-13.2352604395114,
118.649594190874)) ;
#188433=CARTESIAN_POINT('Ctrl Pts',(-13.1478151112943,-13.2475929455495,
118.578428662746)) ;
#188434=CARTESIAN_POINT('Ctrl Pts',(-13.0740112629422,-13.2475928562787,
118.602659689409)) ;
#188435=CARTESIAN_POINT('Ctrl Pts',(-13.0002074145902,-13.2475927670079,
118.626890716073)) ;
#188436=CARTESIAN_POINT('Ctrl Pts',(-13.0235722525017,-13.2352602609698,
118.698056244201)) ;
#188437=CARTESIAN_POINT('Ctrl Pts',(-13.0469370904133,-13.2229277549316,
118.769221772329)) ;
#188438=CARTESIAN_POINT('Ctrl Pts',(-13.1207409387653,-13.2229278442025,
118.744990745665)) ;
#188439=CARTESIAN_POINT('Ctrl Pts',(-13.1945447871174,-13.2229279334733,
118.720759719002)) ;
#188440=CARTESIAN_POINT('Ctrl Pts',(-13.1711799492058,-13.2352604395114,
118.649594190874)) ;
#188441=CARTESIAN_POINT('Ctrl Pts',(-13.1334389030405,-12.9567404114365,
118.570185916102)) ;
#188442=CARTESIAN_POINT('Ctrl Pts',(-13.1119382741817,-12.9885373907524,
118.504698468097)) ;
#188443=CARTESIAN_POINT('Ctrl Pts',(-13.0381344195311,-12.9885373153284,
118.528929475576)) ;
#188444=CARTESIAN_POINT('Ctrl Pts',(-12.9643305648806,-12.9885372399044,
118.553160483055)) ;
#188445=CARTESIAN_POINT('Ctrl Pts',(-12.9858311937394,-12.9567402605885,
118.618647931061)) ;
#188446=CARTESIAN_POINT('Ctrl Pts',(-13.0073318225981,-12.9249432812726,
118.684135379066)) ;
#188447=CARTESIAN_POINT('Ctrl Pts',(-13.0811356772487,-12.9249433566966,
118.659904371587)) ;
#188448=CARTESIAN_POINT('Ctrl Pts',(-13.1549395318993,-12.9249434321206,
118.635673364108)) ;
#188449=CARTESIAN_POINT('Ctrl Pts',(-13.1334389030405,-12.9567404114365,
118.570185916102)) ;
#188450=CARTESIAN_POINT('Ctrl Pts',(-13.0738178620181,-12.7122106250869,
118.424014225001)) ;
#188451=CARTESIAN_POINT('Ctrl Pts',(-13.0557144644975,-12.7611284974195,
118.368874195644)) ;
#188452=CARTESIAN_POINT('Ctrl Pts',(-12.9819106054213,-12.7611284394827,
118.393105189643)) ;
#188453=CARTESIAN_POINT('Ctrl Pts',(-12.9081067463451,-12.7611283815459,
118.417336183643)) ;
#188454=CARTESIAN_POINT('Ctrl Pts',(-12.9262101438657,-12.7122105092134,
118.472476213)) ;
#188455=CARTESIAN_POINT('Ctrl Pts',(-12.9443135413864,-12.6632926368809,
118.527616242358)) ;
#188456=CARTESIAN_POINT('Ctrl Pts',(-13.0181174004625,-12.6632926948177,
118.503385248358)) ;
#188457=CARTESIAN_POINT('Ctrl Pts',(-13.0919212595387,-12.6632927527544,
118.479154254359)) ;
#188458=CARTESIAN_POINT('Ctrl Pts',(-13.0738178620181,-12.7122106250869,
118.424014225001)) ;
#188459=CARTESIAN_POINT('Ctrl Pts',(-12.9958498760682,-12.5182289407429,
118.221927525614)) ;
#188460=CARTESIAN_POINT('Ctrl Pts',(-12.9824305092123,-12.5807644314872,
118.181054298033)) ;
#188461=CARTESIAN_POINT('Ctrl Pts',(-12.9086266477341,-12.5807643929597,
118.205285284716)) ;
#188462=CARTESIAN_POINT('Ctrl Pts',(-12.8348227862559,-12.5807643544323,
118.2295162714)) ;
#188463=CARTESIAN_POINT('Ctrl Pts',(-12.8482421531118,-12.518228863688,
118.27038949898)) ;
#188464=CARTESIAN_POINT('Ctrl Pts',(-12.8616615199678,-12.4556933729437,
118.311262726561)) ;
#188465=CARTESIAN_POINT('Ctrl Pts',(-12.9354653814459,-12.4556934114712,
118.287031739878)) ;
#188466=CARTESIAN_POINT('Ctrl Pts',(-13.0092692429241,-12.4556934499986,
118.262800753194)) ;
#188467=CARTESIAN_POINT('Ctrl Pts',(-12.9958498760682,-12.5182289407429,
118.221927525614)) ;
#188468=CARTESIAN_POINT('Ctrl Pts',(-12.903982147102,-12.3880154836096,
117.97761106073)) ;
#188469=CARTESIAN_POINT('Ctrl Pts',(-12.8962220934696,-12.4597373427525,
117.953975188267)) ;
#188470=CARTESIAN_POINT('Ctrl Pts',(-12.8224182319584,-12.4597373239449,
117.97820617485)) ;
#188471=CARTESIAN_POINT('Ctrl Pts',(-12.7486143704472,-12.4597373051373,
118.002437161433)) ;
#188472=CARTESIAN_POINT('Ctrl Pts',(-12.7563744240796,-12.3880154459944,
118.026073033896)) ;
#188473=CARTESIAN_POINT('Ctrl Pts',(-12.764134477712,-12.3162935868514,
118.049708906359)) ;
#188474=CARTESIAN_POINT('Ctrl Pts',(-12.8379383392232,-12.316293605659,
118.025477919776)) ;
#188475=CARTESIAN_POINT('Ctrl Pts',(-12.9117422007343,-12.3162936244666,
118.001246933193)) ;
#188476=CARTESIAN_POINT('Ctrl Pts',(-12.903982147102,-12.3880154836096,
117.97761106073)) ;
#188477=CARTESIAN_POINT('Ctrl Pts',(-12.8039707728634,-12.3319594983171,
117.708586088061)) ;
#188478=CARTESIAN_POINT('Ctrl Pts',(-12.8024453054662,-12.4077044418995,
117.703939759514)) ;
#188479=CARTESIAN_POINT('Ctrl Pts',(-12.7286414461199,-12.407704439621,
117.728170752691)) ;
#188480=CARTESIAN_POINT('Ctrl Pts',(-12.6548375867736,-12.4077044373425,
117.752401745868)) ;
#188481=CARTESIAN_POINT('Ctrl Pts',(-12.6563630541708,-12.33195949376,117.757048074414)) ;
#188482=CARTESIAN_POINT('Ctrl Pts',(-12.6578885215679,-12.2562145501775,
117.761694402961)) ;
#188483=CARTESIAN_POINT('Ctrl Pts',(-12.7316923809142,-12.2562145524561,
117.737463409784)) ;
#188484=CARTESIAN_POINT('Ctrl Pts',(-12.8054962402605,-12.2562145547346,
117.713232416607)) ;
#188485=CARTESIAN_POINT('Ctrl Pts',(-12.8039707728634,-12.3319594983171,
117.708586088061)) ;
#188486=CARTESIAN_POINT('Ctrl Pts',(-12.7034974125508,-12.3535606969818,
117.437807953422)) ;
#188487=CARTESIAN_POINT('Ctrl Pts',(-12.7082554753366,-12.4279116529158,
117.452300244096)) ;
#188488=CARTESIAN_POINT('Ctrl Pts',(-12.6344516183772,-12.4279116627694,
117.476531244543)) ;
#188489=CARTESIAN_POINT('Ctrl Pts',(-12.5606477614179,-12.427911672623,
117.50076224499)) ;
#188490=CARTESIAN_POINT('Ctrl Pts',(-12.5558896986321,-12.3535607166891,
117.486269954316)) ;
#188491=CARTESIAN_POINT('Ctrl Pts',(-12.5511316358463,-12.2792097607552,
117.471777663643)) ;
#188492=CARTESIAN_POINT('Ctrl Pts',(-12.6249354928057,-12.2792097509015,
117.447546663196)) ;
#188493=CARTESIAN_POINT('Ctrl Pts',(-12.698739349765,-12.2792097410479,
117.423315662748)) ;
#188494=CARTESIAN_POINT('Ctrl Pts',(-12.7034974125508,-12.3535606969818,
117.437807953422)) ;
#188495=CARTESIAN_POINT('Ctrl Pts',(-12.6073331725263,-12.451253883518,
117.180405293082)) ;
#188496=CARTESIAN_POINT('Ctrl Pts',(-12.6180782994954,-12.5188965599117,
117.213133215423)) ;
#188497=CARTESIAN_POINT('Ctrl Pts',(-12.5442744463408,-12.5188965769681,
117.237364227459)) ;
#188498=CARTESIAN_POINT('Ctrl Pts',(-12.4704705931862,-12.5188965940245,
117.261595239495)) ;
#188499=CARTESIAN_POINT('Ctrl Pts',(-12.4597254662172,-12.4512539176309,
117.228867317154)) ;
#188500=CARTESIAN_POINT('Ctrl Pts',(-12.4489803392481,-12.3836112412372,
117.196139394813)) ;
#188501=CARTESIAN_POINT('Ctrl Pts',(-12.5227841924027,-12.3836112241808,
117.171908382778)) ;
#188502=CARTESIAN_POINT('Ctrl Pts',(-12.5965880455573,-12.3836112071243,
117.147677370742)) ;
#188503=CARTESIAN_POINT('Ctrl Pts',(-12.6073331725263,-12.451253883518,
117.180405293082)) ;
#188504=CARTESIAN_POINT('Ctrl Pts',(-12.5223846797122,-12.618326669095,
116.957138731185)) ;
#188505=CARTESIAN_POINT('Ctrl Pts',(-12.538343432535,-12.6744063613934,
117.005746516825)) ;
#188506=CARTESIAN_POINT('Ctrl Pts',(-12.4645395830942,-12.6744063803127,
117.029977540172)) ;
#188507=CARTESIAN_POINT('Ctrl Pts',(-12.3907357336533,-12.6744063992319,
117.054208563519)) ;
#188508=CARTESIAN_POINT('Ctrl Pts',(-12.3747769808305,-12.6183267069335,
117.005600777879)) ;
#188509=CARTESIAN_POINT('Ctrl Pts',(-12.3588182280077,-12.5622470146351,
116.956992992239)) ;
#188510=CARTESIAN_POINT('Ctrl Pts',(-12.4326220774486,-12.5622469957158,
116.932761968892)) ;
#188511=CARTESIAN_POINT('Ctrl Pts',(-12.5064259268894,-12.5622469767965,
116.908530945545)) ;
#188512=CARTESIAN_POINT('Ctrl Pts',(-12.5223846797122,-12.618326669095,
116.957138731185)) ;
#188513=CARTESIAN_POINT('Ctrl Pts',(-12.4538138970697,-12.8433532834822,
116.783847061127)) ;
#188514=CARTESIAN_POINT('Ctrl Pts',(-12.4738488524153,-12.883805650216,
116.844870302127)) ;
#188515=CARTESIAN_POINT('Ctrl Pts',(-12.4000450061609,-12.8838056661619,
116.86910133518)) ;
#188516=CARTESIAN_POINT('Ctrl Pts',(-12.3262411599065,-12.8838056821078,
116.893332368233)) ;
#188517=CARTESIAN_POINT('Ctrl Pts',(-12.306206204561,-12.843353315374,116.832309127233)) ;
#188518=CARTESIAN_POINT('Ctrl Pts',(-12.2861712492154,-12.8029009486403,
116.771285886233)) ;
#188519=CARTESIAN_POINT('Ctrl Pts',(-12.3599750954699,-12.8029009326944,
116.74705485318)) ;
#188520=CARTESIAN_POINT('Ctrl Pts',(-12.4337789417243,-12.8029009167485,
116.722823820128)) ;
#188521=CARTESIAN_POINT('Ctrl Pts',(-12.4538138970697,-12.8433532834822,
116.783847061127)) ;
#188522=CARTESIAN_POINT('Ctrl Pts',(-12.4061377499022,-13.1083703127966,
116.674020302438)) ;
#188523=CARTESIAN_POINT('Ctrl Pts',(-12.4287995875301,-13.1303789495469,
116.74304460315)) ;
#188524=CARTESIAN_POINT('Ctrl Pts',(-12.3549957432582,-13.1303789610419,
116.767275642241)) ;
#188525=CARTESIAN_POINT('Ctrl Pts',(-12.2811918989863,-13.130378972537,
116.791506681332)) ;
#188526=CARTESIAN_POINT('Ctrl Pts',(-12.2585300613583,-13.1083703357867,
116.72248238062)) ;
#188527=CARTESIAN_POINT('Ctrl Pts',(-12.2358682237303,-13.0863616990364,
116.653458079908)) ;
#188528=CARTESIAN_POINT('Ctrl Pts',(-12.3096720680023,-13.0863616875414,
116.629227040817)) ;
#188529=CARTESIAN_POINT('Ctrl Pts',(-12.3834759122742,-13.0863616760463,
116.604996001726)) ;
#188530=CARTESIAN_POINT('Ctrl Pts',(-12.4061377499022,-13.1083703127966,
116.674020302438)) ;
#188531=CARTESIAN_POINT('Ctrl Pts',(-12.3816337942229,-13.3973093025061,
116.635000519371)) ;
#188532=CARTESIAN_POINT('Ctrl Pts',(-12.4053038929574,-13.3991753907739,
116.707095820866)) ;
#188533=CARTESIAN_POINT('Ctrl Pts',(-12.3315000496693,-13.399175395662,
116.731326862953)) ;
#188534=CARTESIAN_POINT('Ctrl Pts',(-12.2576962063811,-13.39917540055,116.755557905041)) ;
#188535=CARTESIAN_POINT('Ctrl Pts',(-12.2340261076466,-13.3973093122823,
116.683462603546)) ;
#188536=CARTESIAN_POINT('Ctrl Pts',(-12.2103560089121,-13.3954432240146,
116.611367302051)) ;
#188537=CARTESIAN_POINT('Ctrl Pts',(-12.2841598522002,-13.3954432191265,
116.587136259963)) ;
#188538=CARTESIAN_POINT('Ctrl Pts',(-12.3579636954884,-13.3954432142384,
116.562905217876)) ;
#188539=CARTESIAN_POINT('Ctrl Pts',(-12.3816337942229,-13.3973093025061,
116.635000519371)) ;
#188540=CARTESIAN_POINT('Ctrl Pts',(-12.381503672392,-13.685052446536,116.669875319027)) ;
#188541=CARTESIAN_POINT('Ctrl Pts',(-12.4044882857984,-13.666829482395,
116.739882742886)) ;
#188542=CARTESIAN_POINT('Ctrl Pts',(-12.3306844425751,-13.6668294834514,
116.764113785171)) ;
#188543=CARTESIAN_POINT('Ctrl Pts',(-12.2568805993519,-13.6668294845077,
116.788344827456)) ;
#188544=CARTESIAN_POINT('Ctrl Pts',(-12.2338959859455,-13.6850524486487,
116.718337403597)) ;
#188545=CARTESIAN_POINT('Ctrl Pts',(-12.2109113725392,-13.7032754127896,
116.648329979738)) ;
#188546=CARTESIAN_POINT('Ctrl Pts',(-12.2847152157624,-13.7032754117333,
116.624098937453)) ;
#188547=CARTESIAN_POINT('Ctrl Pts',(-12.3585190589856,-13.7032754106769,
116.599867895168)) ;
#188548=CARTESIAN_POINT('Ctrl Pts',(-12.381503672392,-13.685052446536,116.669875319027)) ;
#188549=CARTESIAN_POINT('Ctrl Pts',(-12.4049796303941,-13.9562925901238,
116.776990471733)) ;
#188550=CARTESIAN_POINT('Ctrl Pts',(-12.425622446726,-13.9191017880253,
116.839865159623)) ;
#188551=CARTESIAN_POINT('Ctrl Pts',(-12.3518186029917,-13.9191017857383,
116.864096200351)) ;
#188552=CARTESIAN_POINT('Ctrl Pts',(-12.2780147592573,-13.9191017834513,
116.88832724108)) ;
#188553=CARTESIAN_POINT('Ctrl Pts',(-12.2573719429255,-13.9562925855498,
116.82545255319)) ;
#188554=CARTESIAN_POINT('Ctrl Pts',(-12.2367291265936,-13.9934833876483,
116.762577865301)) ;
#188555=CARTESIAN_POINT('Ctrl Pts',(-12.3105329703279,-13.9934833899353,
116.738346824573)) ;
#188556=CARTESIAN_POINT('Ctrl Pts',(-12.3843368140622,-13.9934833922223,
116.714115783844)) ;
#188557=CARTESIAN_POINT('Ctrl Pts',(-12.4049796303941,-13.9562925901238,
116.776990471733)) ;
#188558=CARTESIAN_POINT('Ctrl Pts',(-12.4494947820984,-14.1872893194723,
116.947967301945)) ;
#188559=CARTESIAN_POINT('Ctrl Pts',(-12.4663273310332,-14.1339131286007,
116.999236530143)) ;
#188560=CARTESIAN_POINT('Ctrl Pts',(-12.3925234868813,-14.1339131262424,
117.023467569599)) ;
#188561=CARTESIAN_POINT('Ctrl Pts',(-12.3187196427294,-14.1339131238842,
117.047698609056)) ;
#188562=CARTESIAN_POINT('Ctrl Pts',(-12.3018870937946,-14.1872893147558,
116.996429380858)) ;
#188563=CARTESIAN_POINT('Ctrl Pts',(-12.2850545448598,-14.2406655056274,
116.94516015266)) ;
#188564=CARTESIAN_POINT('Ctrl Pts',(-12.3588583890117,-14.2406655079856,
116.920929113203)) ;
#188565=CARTESIAN_POINT('Ctrl Pts',(-12.4326622331636,-14.2406655103439,
116.896698073747)) ;
#188566=CARTESIAN_POINT('Ctrl Pts',(-12.4494947820984,-14.1872893194723,
116.947967301945)) ;
#188567=CARTESIAN_POINT('Ctrl Pts',(-12.5111240358726,-14.3636852679792,
117.17110246923)) ;
#188568=CARTESIAN_POINT('Ctrl Pts',(-12.5229448664094,-14.2979128675593,
117.207106811808)) ;
#188569=CARTESIAN_POINT('Ctrl Pts',(-12.4491410223146,-14.2979128665308,
117.231337851438)) ;
#188570=CARTESIAN_POINT('Ctrl Pts',(-12.3753371782198,-14.2979128655022,
117.255568891069)) ;
#188571=CARTESIAN_POINT('Ctrl Pts',(-12.3635163476831,-14.3636852659222,
117.219564548491)) ;
#188572=CARTESIAN_POINT('Ctrl Pts',(-12.3516955171463,-14.4294576663421,
117.183560205913)) ;
#188573=CARTESIAN_POINT('Ctrl Pts',(-12.4254993612411,-14.4294576673706,
117.159329166283)) ;
#188574=CARTESIAN_POINT('Ctrl Pts',(-12.4993032053359,-14.4294576683991,
117.135098126652)) ;
#188575=CARTESIAN_POINT('Ctrl Pts',(-12.5111240358726,-14.3636852679792,
117.17110246923)) ;
#188576=CARTESIAN_POINT('Ctrl Pts',(-12.5849595606455,-14.4725504618335,
117.431499846562)) ;
#188577=CARTESIAN_POINT('Ctrl Pts',(-12.5909072144408,-14.3990795841732,
117.449615440357)) ;
#188578=CARTESIAN_POINT('Ctrl Pts',(-12.5171033712477,-14.3990795846932,
117.473846482734)) ;
#188579=CARTESIAN_POINT('Ctrl Pts',(-12.4432995280546,-14.3990795852131,
117.498077525111)) ;
#188580=CARTESIAN_POINT('Ctrl Pts',(-12.4373518742593,-14.4725504628734,
117.479961931316)) ;
#188581=CARTESIAN_POINT('Ctrl Pts',(-12.431404220464,-14.5460213405337,
117.461846337522)) ;
#188582=CARTESIAN_POINT('Ctrl Pts',(-12.5052080636571,-14.5460213400138,
117.437615295145)) ;
#188583=CARTESIAN_POINT('Ctrl Pts',(-12.5790119068502,-14.5460213394938,
117.413384252768)) ;
#188584=CARTESIAN_POINT('Ctrl Pts',(-12.5849595606455,-14.4725504618335,
117.431499846562)) ;
#188585=CARTESIAN_POINT('Ctrl Pts',(-12.6644929453121,-14.505767100085,
117.709124162451)) ;
#188586=CARTESIAN_POINT('Ctrl Pts',(-12.664163724492,-14.4298697296846,
117.708121408856)) ;
#188587=CARTESIAN_POINT('Ctrl Pts',(-12.5903598826455,-14.429869730049,
117.732352455334)) ;
#188588=CARTESIAN_POINT('Ctrl Pts',(-12.516556040799,-14.4298697304134,
117.756583501813)) ;
#188589=CARTESIAN_POINT('Ctrl Pts',(-12.5168852616191,-14.5057671008138,
117.757586255408)) ;
#188590=CARTESIAN_POINT('Ctrl Pts',(-12.5172144824392,-14.5816644712143,
117.758589009003)) ;
#188591=CARTESIAN_POINT('Ctrl Pts',(-12.5910183242857,-14.5816644708498,
117.734357962524)) ;
#188592=CARTESIAN_POINT('Ctrl Pts',(-12.6648221661322,-14.5816644704854,
117.710126916046)) ;
#188593=CARTESIAN_POINT('Ctrl Pts',(-12.6644929453121,-14.505767100085,
117.709124162451)) ;
#188594=CARTESIAN_POINT('Ctrl Pts',(-12.7438560906552,-14.461184023194,
117.986366449058)) ;
#188595=CARTESIAN_POINT('Ctrl Pts',(-12.7372499374125,-14.388288943336,
117.966245171962)) ;
#188596=CARTESIAN_POINT('Ctrl Pts',(-12.6634460974251,-14.3882889407252,
117.990476224103)) ;
#188597=CARTESIAN_POINT('Ctrl Pts',(-12.5896422574376,-14.3882889381144,
118.014707276243)) ;
#188598=CARTESIAN_POINT('Ctrl Pts',(-12.5962484106803,-14.4611840179724,
118.034828553339)) ;
#188599=CARTESIAN_POINT('Ctrl Pts',(-12.6028545639229,-14.5340790978304,
118.054949830435)) ;
#188600=CARTESIAN_POINT('Ctrl Pts',(-12.6766584039103,-14.5340791004412,
118.030718778294)) ;
#188601=CARTESIAN_POINT('Ctrl Pts',(-12.7504622438978,-14.534079103052,
118.006487726153)) ;
#188602=CARTESIAN_POINT('Ctrl Pts',(-12.7438560906552,-14.461184023194,
117.986366449058)) ;
#188603=CARTESIAN_POINT('Ctrl Pts',(-12.8161888293578,-14.3417566878776,
118.242145226587)) ;
#188604=CARTESIAN_POINT('Ctrl Pts',(-12.8037886916051,-14.2770945733709,
118.204376407392)) ;
#188605=CARTESIAN_POINT('Ctrl Pts',(-12.7299848531598,-14.2770945642116,
118.22860746423)) ;
#188606=CARTESIAN_POINT('Ctrl Pts',(-12.6561810147145,-14.2770945550524,
118.252838521068)) ;
#188607=CARTESIAN_POINT('Ctrl Pts',(-12.6685811524673,-14.3417566695591,
118.290607340263)) ;
#188608=CARTESIAN_POINT('Ctrl Pts',(-12.68098129022,-14.4064187840659,118.328376159457)) ;
#188609=CARTESIAN_POINT('Ctrl Pts',(-12.7547851286653,-14.4064187932251,
118.304145102619)) ;
#188610=CARTESIAN_POINT('Ctrl Pts',(-12.8285889671106,-14.4064188023844,
118.279914045781)) ;
#188611=CARTESIAN_POINT('Ctrl Pts',(-12.8161888293578,-14.3417566878776,
118.242145226587)) ;
#188612=CARTESIAN_POINT('Ctrl Pts',(-12.8756299425708,-14.1564991842471,
118.458617084048)) ;
#188613=CARTESIAN_POINT('Ctrl Pts',(-12.8583285484173,-14.104678506832,
118.405919828527)) ;
#188614=CARTESIAN_POINT('Ctrl Pts',(-12.7845247106298,-14.1046784883743,
118.430150887369)) ;
#188615=CARTESIAN_POINT('Ctrl Pts',(-12.7107208728424,-14.1046784699167,
118.454381946211)) ;
#188616=CARTESIAN_POINT('Ctrl Pts',(-12.7280222669959,-14.1564991473318,
118.507079201731)) ;
#188617=CARTESIAN_POINT('Ctrl Pts',(-12.7453236611495,-14.208319824747,
118.559776457252)) ;
#188618=CARTESIAN_POINT('Ctrl Pts',(-12.8191274989369,-14.2083198432046,
118.53554539841)) ;
#188619=CARTESIAN_POINT('Ctrl Pts',(-12.8929313367243,-14.2083198616622,
118.511314339568)) ;
#188620=CARTESIAN_POINT('Ctrl Pts',(-12.8756299425708,-14.1564991842471,
118.458617084048)) ;
#188621=CARTESIAN_POINT('Ctrl Pts',(-12.9173366092664,-13.9178865274089,
118.621150963458)) ;
#188622=CARTESIAN_POINT('Ctrl Pts',(-12.8963635167268,-13.8826509917796,
118.557270306911)) ;
#188623=CARTESIAN_POINT('Ctrl Pts',(-12.8225596784781,-13.8826509615156,
118.581501364348)) ;
#188624=CARTESIAN_POINT('Ctrl Pts',(-12.7487558402295,-13.8826509312515,
118.605732421785)) ;
#188625=CARTESIAN_POINT('Ctrl Pts',(-12.7697289327691,-13.9178864668808,
118.669613078332)) ;
#188626=CARTESIAN_POINT('Ctrl Pts',(-12.7907020253087,-13.9531220025101,
118.733493734878)) ;
#188627=CARTESIAN_POINT('Ctrl Pts',(-12.8645058635573,-13.9531220327742,
118.709262677441)) ;
#188628=CARTESIAN_POINT('Ctrl Pts',(-12.9383097018059,-13.9531220630382,
118.685031620004)) ;
#188629=CARTESIAN_POINT('Ctrl Pts',(-12.9173366092664,-13.9178865274089,
118.621150963458)) ;
#188630=CARTESIAN_POINT('Ctrl Pts',(-12.9373830489153,-13.643415658276,
118.717703562338)) ;
#188631=CARTESIAN_POINT('Ctrl Pts',(-12.9142455039955,-13.6272927364366,
118.647230332902)) ;
#188632=CARTESIAN_POINT('Ctrl Pts',(-12.8404416636247,-13.627292694101,
118.671461383875)) ;
#188633=CARTESIAN_POINT('Ctrl Pts',(-12.7666378232539,-13.6272926517654,
118.695692434849)) ;
#188634=CARTESIAN_POINT('Ctrl Pts',(-12.7897753681737,-13.6434155736048,
118.766165664285)) ;
#188635=CARTESIAN_POINT('Ctrl Pts',(-12.8129129130935,-13.6595384954442,
118.836638893721)) ;
#188636=CARTESIAN_POINT('Ctrl Pts',(-12.8867167534643,-13.6595385377798,
118.812407842748)) ;
#188637=CARTESIAN_POINT('Ctrl Pts',(-12.9605205938351,-13.6595385801154,
118.788176791774)) ;
#188638=CARTESIAN_POINT('Ctrl Pts',(-12.9373830489153,-13.643415658276,
118.717703562338)) ;
#188639=CARTESIAN_POINT('Ctrl Pts',(-12.933631988452,-13.3531854263633,
118.741726098941)) ;
#188640=CARTESIAN_POINT('Ctrl Pts',(-12.9099894296058,-13.3573028544331,
118.669714678404)) ;
#188641=CARTESIAN_POINT('Ctrl Pts',(-12.8361855854579,-13.3573028025058,
118.693945717873)) ;
#188642=CARTESIAN_POINT('Ctrl Pts',(-12.76238174131,-13.3573027505784,118.718176757342)) ;
#188643=CARTESIAN_POINT('Ctrl Pts',(-12.7860243001563,-13.3531853225086,
118.790188177879)) ;
#188644=CARTESIAN_POINT('Ctrl Pts',(-12.8096668590025,-13.3490678944388,
118.862199598417)) ;
#188645=CARTESIAN_POINT('Ctrl Pts',(-12.8834707031504,-13.3490679463661,
118.837968558948)) ;
#188646=CARTESIAN_POINT('Ctrl Pts',(-12.9572745472983,-13.3490679982935,
118.813737519479)) ;
#188647=CARTESIAN_POINT('Ctrl Pts',(-12.933631988452,-13.3531854263633,
118.741726098941)) ;
#188648=CARTESIAN_POINT('Ctrl Pts',(-12.9056359229119,-13.0673885224611,
118.691923781968)) ;
#188649=CARTESIAN_POINT('Ctrl Pts',(-12.8831798942909,-13.0914657876093,
118.623526340883)) ;
#188650=CARTESIAN_POINT('Ctrl Pts',(-12.8093760450123,-13.0914657299476,
118.647757364725)) ;
#188651=CARTESIAN_POINT('Ctrl Pts',(-12.7355721957337,-13.0914656722859,
118.671988388566)) ;
#188652=CARTESIAN_POINT('Ctrl Pts',(-12.7580282243547,-13.0673884071377,
118.740385829651)) ;
#188653=CARTESIAN_POINT('Ctrl Pts',(-12.7804842529757,-13.0433111419895,
118.808783270735)) ;
#188654=CARTESIAN_POINT('Ctrl Pts',(-12.8542881022543,-13.0433111996512,
118.784552246894)) ;
#188655=CARTESIAN_POINT('Ctrl Pts',(-12.9280919515329,-13.0433112573129,
118.760321223052)) ;
#188656=CARTESIAN_POINT('Ctrl Pts',(-12.9056359229119,-13.0673885224611,
118.691923781968)) ;
#188657=CARTESIAN_POINT('Ctrl Pts',(-12.854527427208,-12.8066409255768,
118.571752043509)) ;
#188658=CARTESIAN_POINT('Ctrl Pts',(-12.8348726791899,-12.8489579270799,
118.511886850991)) ;
#188659=CARTESIAN_POINT('Ctrl Pts',(-12.7610688238133,-12.8489578695406,
118.536117856259)) ;
#188660=CARTESIAN_POINT('Ctrl Pts',(-12.6872649684367,-12.8489578120014,
118.560348861527)) ;
#188661=CARTESIAN_POINT('Ctrl Pts',(-12.7069197164548,-12.8066408104982,
118.620214054045)) ;
#188662=CARTESIAN_POINT('Ctrl Pts',(-12.7265744644729,-12.7643238089951,
118.680079246563)) ;
#188663=CARTESIAN_POINT('Ctrl Pts',(-12.8003783198495,-12.7643238665344,
118.655848241295)) ;
#188664=CARTESIAN_POINT('Ctrl Pts',(-12.8741821752261,-12.7643239240736,
118.631617236027)) ;
#188665=CARTESIAN_POINT('Ctrl Pts',(-12.854527427208,-12.8066409255768,
118.571752043509)) ;
#188666=CARTESIAN_POINT('Ctrl Pts',(-12.7836941512798,-12.5904014103484,
118.391342109483)) ;
#188667=CARTESIAN_POINT('Ctrl Pts',(-12.7682252464874,-12.6478767369269,
118.344226319916)) ;
#188668=CARTESIAN_POINT('Ctrl Pts',(-12.6944213851999,-12.6478766870741,
118.368457307181)) ;
#188669=CARTESIAN_POINT('Ctrl Pts',(-12.6206175239125,-12.6478766372212,
118.392688294445)) ;
#188670=CARTESIAN_POINT('Ctrl Pts',(-12.6360864287049,-12.5904013106426,
118.439804084012)) ;
#188671=CARTESIAN_POINT('Ctrl Pts',(-12.6515553334974,-12.5329259840641,
118.486919873579)) ;
#188672=CARTESIAN_POINT('Ctrl Pts',(-12.7253591947849,-12.5329260339169,
118.462688886314)) ;
#188673=CARTESIAN_POINT('Ctrl Pts',(-12.7991630560723,-12.5329260837698,
118.43845789905)) ;
#188674=CARTESIAN_POINT('Ctrl Pts',(-12.7836941512798,-12.5904014103484,
118.391342109483)) ;
#188675=CARTESIAN_POINT('Ctrl Pts',(-12.6961467508586,-12.4318423089519,
118.160410562632)) ;
#188676=CARTESIAN_POINT('Ctrl Pts',(-12.6860283059274,-12.500471718984,
118.12959141033)) ;
#188677=CARTESIAN_POINT('Ctrl Pts',(-12.6122244385164,-12.5004716824447,
118.153822378943)) ;
#188678=CARTESIAN_POINT('Ctrl Pts',(-12.5384205711053,-12.5004716459054,
118.178053347556)) ;
#188679=CARTESIAN_POINT('Ctrl Pts',(-12.5485390160365,-12.4318422358733,
118.208872499858)) ;
#188680=CARTESIAN_POINT('Ctrl Pts',(-12.5586574609676,-12.3632128258413,
118.239691652159)) ;
#188681=CARTESIAN_POINT('Ctrl Pts',(-12.6324613283787,-12.3632128623805,
118.215460683547)) ;
#188682=CARTESIAN_POINT('Ctrl Pts',(-12.7062651957898,-12.3632128989198,
118.191229714934)) ;
#188683=CARTESIAN_POINT('Ctrl Pts',(-12.6961467508586,-12.4318423089519,
118.160410562632)) ;
#188684=CARTESIAN_POINT('Ctrl Pts',(-12.5994432623834,-12.3456712150683,
117.901136629197)) ;
#188685=CARTESIAN_POINT('Ctrl Pts',(-12.5953319588446,-12.4204161323536,
117.888614260233)) ;
#188686=CARTESIAN_POINT('Ctrl Pts',(-12.5215280877492,-12.4204161168077,
117.912845217624)) ;
#188687=CARTESIAN_POINT('Ctrl Pts',(-12.4477242166539,-12.4204161012619,
117.937076175015)) ;
#188688=CARTESIAN_POINT('Ctrl Pts',(-12.4518355201927,-12.3456711839767,
117.949598543979)) ;
#188689=CARTESIAN_POINT('Ctrl Pts',(-12.4559468237315,-12.2709262666914,
117.962120912943)) ;
#188690=CARTESIAN_POINT('Ctrl Pts',(-12.5297506948269,-12.2709262822373,
117.937889955552)) ;
#188691=CARTESIAN_POINT('Ctrl Pts',(-12.6035545659222,-12.2709262977831,
117.913658998161)) ;
#188692=CARTESIAN_POINT('Ctrl Pts',(-12.5994432623834,-12.3456712150683,
117.901136629197)) ;
#188693=CARTESIAN_POINT('Ctrl Pts',(-12.4981428620814,-12.3353742164119,
117.628067921489)) ;
#188694=CARTESIAN_POINT('Ctrl Pts',(-12.5003639216367,-12.4109469942247,
117.634832908676)) ;
#188695=CARTESIAN_POINT('Ctrl Pts',(-12.4265600484705,-12.4109470032869,
117.659063859759)) ;
#188696=CARTESIAN_POINT('Ctrl Pts',(-12.3527561753044,-12.410947012349,
117.683294810843)) ;
#188697=CARTESIAN_POINT('Ctrl Pts',(-12.3505351157491,-12.3353742345363,
117.676529823657)) ;
#188698=CARTESIAN_POINT('Ctrl Pts',(-12.3483140561938,-12.2598014567236,
117.66976483647)) ;
#188699=CARTESIAN_POINT('Ctrl Pts',(-12.42211792936,-12.2598014476614,117.645533885386)) ;
#188700=CARTESIAN_POINT('Ctrl Pts',(-12.4959218025261,-12.2598014385992,
117.621302934303)) ;
#188701=CARTESIAN_POINT('Ctrl Pts',(-12.4981428620814,-12.3353742164119,
117.628067921489)) ;
#188702=CARTESIAN_POINT('Ctrl Pts',(-12.3992898679553,-12.402733699683,
117.362430521718)) ;
#188703=CARTESIAN_POINT('Ctrl Pts',(-12.4076821390233,-12.473714122898,
117.387992023362)) ;
#188704=CARTESIAN_POINT('Ctrl Pts',(-12.3338782663327,-12.4737141587005,
117.412222975894)) ;
#188705=CARTESIAN_POINT('Ctrl Pts',(-12.2600743936421,-12.473714194503,
117.436453928426)) ;
#188706=CARTESIAN_POINT('Ctrl Pts',(-12.2516821225741,-12.402733771288,
117.410892426782)) ;
#188707=CARTESIAN_POINT('Ctrl Pts',(-12.243289851506,-12.331753348073,117.385330925138)) ;
#188708=CARTESIAN_POINT('Ctrl Pts',(-12.3170937241966,-12.3317533122705,
117.361099972606)) ;
#188709=CARTESIAN_POINT('Ctrl Pts',(-12.3908975968872,-12.331753276468,
117.336869020074)) ;
#188710=CARTESIAN_POINT('Ctrl Pts',(-12.3992898679553,-12.402733699683,
117.362430521718)) ;
#188711=CARTESIAN_POINT('Ctrl Pts',(-12.3089264322979,-12.5432714498278,
117.122757256205)) ;
#188712=CARTESIAN_POINT('Ctrl Pts',(-12.3229040621412,-12.6045444668254,
117.165330859406)) ;
#188713=CARTESIAN_POINT('Ctrl Pts',(-12.2491001924915,-12.6045445287426,
117.1895618212)) ;
#188714=CARTESIAN_POINT('Ctrl Pts',(-12.1752963228417,-12.6045445906598,
117.213792782994)) ;
#188715=CARTESIAN_POINT('Ctrl Pts',(-12.1613186929985,-12.5432715736621,
117.171219179793)) ;
#188716=CARTESIAN_POINT('Ctrl Pts',(-12.1473410631552,-12.4819985566645,
117.128645576591)) ;
#188717=CARTESIAN_POINT('Ctrl Pts',(-12.2211449328049,-12.4819984947474,
117.104414614797)) ;
#188718=CARTESIAN_POINT('Ctrl Pts',(-12.2949488024546,-12.4819984328302,
117.080183653003)) ;
#188719=CARTESIAN_POINT('Ctrl Pts',(-12.3089264322979,-12.5432714498278,
117.122757256205)) ;
#188720=CARTESIAN_POINT('Ctrl Pts',(-12.2333037274479,-12.7462375607508,
116.92788225993)) ;
#188721=CARTESIAN_POINT('Ctrl Pts',(-12.2518478945764,-12.7934303811122,
116.984364798848)) ;
#188722=CARTESIAN_POINT('Ctrl Pts',(-12.1780440305619,-12.7934304650843,
117.008595777806)) ;
#188723=CARTESIAN_POINT('Ctrl Pts',(-12.1042401665475,-12.7934305490564,
117.032826756764)) ;
#188724=CARTESIAN_POINT('Ctrl Pts',(-12.0856959994191,-12.746237728695,
116.976344217846)) ;
#188725=CARTESIAN_POINT('Ctrl Pts',(-12.0671518322907,-12.6990449083337,
116.919861678928)) ;
#188726=CARTESIAN_POINT('Ctrl Pts',(-12.1409556963051,-12.6990448243616,
116.89563069997)) ;
#188727=CARTESIAN_POINT('Ctrl Pts',(-12.2147595603195,-12.6990447403895,
116.871399721012)) ;
#188728=CARTESIAN_POINT('Ctrl Pts',(-12.2333037274479,-12.7462375607508,
116.92788225993)) ;
#188729=CARTESIAN_POINT('Ctrl Pts',(-12.1768490292264,-12.9968255702811,
116.791336954581)) ;
#188730=CARTESIAN_POINT('Ctrl Pts',(-12.1986293527966,-13.0265927652578,
116.857676303844)) ;
#188731=CARTESIAN_POINT('Ctrl Pts',(-12.1248254963235,-13.0265928649381,
116.881907305772)) ;
#188732=CARTESIAN_POINT('Ctrl Pts',(-12.0510216398503,-13.0265929646183,
116.9061383077)) ;
#188733=CARTESIAN_POINT('Ctrl Pts',(-12.0292413162801,-12.9968257696416,
116.839798958437)) ;
#188734=CARTESIAN_POINT('Ctrl Pts',(-12.0074609927098,-12.9670585746648,
116.773459609174)) ;
#188735=CARTESIAN_POINT('Ctrl Pts',(-12.081264849183,-12.9670584749846,
116.749228607246)) ;
#188736=CARTESIAN_POINT('Ctrl Pts',(-12.1550687056562,-12.9670583753043,
116.724997605318)) ;
#188737=CARTESIAN_POINT('Ctrl Pts',(-12.1768490292264,-12.9968255702811,
116.791336954581)) ;
#188738=CARTESIAN_POINT('Ctrl Pts',(-12.1427051117451,-13.2777710794654,
116.722782478303)) ;
#188739=CARTESIAN_POINT('Ctrl Pts',(-12.1661680895721,-13.2879677234676,
116.794246920931)) ;
#188740=CARTESIAN_POINT('Ctrl Pts',(-12.0923642418223,-13.2879678309871,
116.818477949429)) ;
#188741=CARTESIAN_POINT('Ctrl Pts',(-12.0185603940725,-13.2879679385065,
116.842708977927)) ;
#188742=CARTESIAN_POINT('Ctrl Pts',(-11.9950974162455,-13.2777712945044,
116.771244535298)) ;
#188743=CARTESIAN_POINT('Ctrl Pts',(-11.9716344384184,-13.2675746505022,
116.69978009267)) ;
#188744=CARTESIAN_POINT('Ctrl Pts',(-12.0454382861683,-13.2675745429828,
116.675549064172)) ;
#188745=CARTESIAN_POINT('Ctrl Pts',(-12.1192421339181,-13.2675744354633,
116.651318035675)) ;
#188746=CARTESIAN_POINT('Ctrl Pts',(-12.1427051117451,-13.2777710794654,
116.722782478303)) ;
#188747=CARTESIAN_POINT('Ctrl Pts',(-12.132619814381,-13.5692121151867,
116.72755803208)) ;
#188748=CARTESIAN_POINT('Ctrl Pts',(-12.1560873514429,-13.5590766136152,
116.799036361418)) ;
#188749=CARTESIAN_POINT('Ctrl Pts',(-12.0822835127583,-13.5590767201184,
116.823267417527)) ;
#188750=CARTESIAN_POINT('Ctrl Pts',(-12.0084796740738,-13.5590768266217,
116.847498473636)) ;
#188751=CARTESIAN_POINT('Ctrl Pts',(-11.9850121370119,-13.5692123281932,
116.776020144298)) ;
#188752=CARTESIAN_POINT('Ctrl Pts',(-11.9615445999501,-13.5793478297647,
116.70454181496)) ;
#188753=CARTESIAN_POINT('Ctrl Pts',(-12.0353484386346,-13.5793477232615,
116.680310758851)) ;
#188754=CARTESIAN_POINT('Ctrl Pts',(-12.1091522773192,-13.5793476167582,
116.656079702742)) ;
#188755=CARTESIAN_POINT('Ctrl Pts',(-12.132619814381,-13.5692121151867,
116.72755803208)) ;
#188756=CARTESIAN_POINT('Ctrl Pts',(-12.1467639143516,-13.8503430324929,
116.806211060665)) ;
#188757=CARTESIAN_POINT('Ctrl Pts',(-12.1685429840334,-13.8205648157971,
116.872546590843)) ;
#188758=CARTESIAN_POINT('Ctrl Pts',(-12.094739153736,-13.8205649121888,
116.896777672498)) ;
#188759=CARTESIAN_POINT('Ctrl Pts',(-12.0209353234386,-13.8205650085804,
116.921008754153)) ;
#188760=CARTESIAN_POINT('Ctrl Pts',(-11.9991562537568,-13.8503432252762,
116.854673223975)) ;
#188761=CARTESIAN_POINT('Ctrl Pts',(-11.977377184075,-13.880121441972,116.788337693796)) ;
#188762=CARTESIAN_POINT('Ctrl Pts',(-12.0511810143725,-13.8801213455804,
116.764106612141)) ;
#188763=CARTESIAN_POINT('Ctrl Pts',(-12.1249848446699,-13.8801212491888,
116.739875530486)) ;
#188764=CARTESIAN_POINT('Ctrl Pts',(-12.1467639143516,-13.8503430324929,
116.806211060665)) ;
#188765=CARTESIAN_POINT('Ctrl Pts',(-12.1829893801448,-14.0986233529731,
116.951857724496)) ;
#188766=CARTESIAN_POINT('Ctrl Pts',(-12.2015410509572,-14.0514664875456,
117.008363118508)) ;
#188767=CARTESIAN_POINT('Ctrl Pts',(-12.1277372276301,-14.0514665673178,
117.032594221393)) ;
#188768=CARTESIAN_POINT('Ctrl Pts',(-12.0539334043031,-14.05146664709,117.056825324279)) ;
#188769=CARTESIAN_POINT('Ctrl Pts',(-12.0353817334907,-14.0986235125175,
117.000319930267)) ;
#188770=CARTESIAN_POINT('Ctrl Pts',(-12.0168300626784,-14.145780377945,
116.943814536255)) ;
#188771=CARTESIAN_POINT('Ctrl Pts',(-12.0906338860054,-14.1457802981728,
116.919583433369)) ;
#188772=CARTESIAN_POINT('Ctrl Pts',(-12.1644377093324,-14.1457802184006,
116.895352330483)) ;
#188773=CARTESIAN_POINT('Ctrl Pts',(-12.1829893801448,-14.0986233529731,
116.951857724496)) ;
#188774=CARTESIAN_POINT('Ctrl Pts',(-12.2382733903879,-14.2995832696182,
117.155728549187)) ;
#188775=CARTESIAN_POINT('Ctrl Pts',(-12.2522588615321,-14.2383253097085,
117.198326035843)) ;
#188776=CARTESIAN_POINT('Ctrl Pts',(-12.1784550430804,-14.2383253669594,
117.222557153578)) ;
#188777=CARTESIAN_POINT('Ctrl Pts',(-12.1046512246287,-14.2383254242103,
117.246788271313)) ;
#188778=CARTESIAN_POINT('Ctrl Pts',(-12.0906657534845,-14.29958338412,117.204190784657)) ;
#188779=CARTESIAN_POINT('Ctrl Pts',(-12.0766802823402,-14.3608413440297,
117.161593298)) ;
#188780=CARTESIAN_POINT('Ctrl Pts',(-12.1504841007919,-14.3608412867788,
117.137362180265)) ;
#188781=CARTESIAN_POINT('Ctrl Pts',(-12.2242879192436,-14.3608412295279,
117.11313106253)) ;
#188782=CARTESIAN_POINT('Ctrl Pts',(-12.2382733903879,-14.2995832696182,
117.155728549187)) ;
#188783=CARTESIAN_POINT('Ctrl Pts',(-12.3080272802778,-14.4373031232107,
117.403743324184)) ;
#188784=CARTESIAN_POINT('Ctrl Pts',(-12.3164280476558,-14.3663375815008,
117.42933070437)) ;
#188785=CARTESIAN_POINT('Ctrl Pts',(-12.2426242313647,-14.3663376133963,
117.453561828685)) ;
#188786=CARTESIAN_POINT('Ctrl Pts',(-12.1688204150736,-14.3663376452917,
117.477792953001)) ;
#188787=CARTESIAN_POINT('Ctrl Pts',(-12.1604196476955,-14.4373031870016,
117.452205572816)) ;
#188788=CARTESIAN_POINT('Ctrl Pts',(-12.1520188803175,-14.5082687287115,
117.426618192631)) ;
#188789=CARTESIAN_POINT('Ctrl Pts',(-12.2258226966086,-14.5082686968161,
117.402387068315)) ;
#188790=CARTESIAN_POINT('Ctrl Pts',(-12.2996265128997,-14.5082686649206,
117.378155943999)) ;
#188791=CARTESIAN_POINT('Ctrl Pts',(-12.3080272802778,-14.4373031232107,
117.403743324184)) ;
#188792=CARTESIAN_POINT('Ctrl Pts',(-12.3858324941963,-14.5016051754735,
117.676070811341)) ;
#188793=CARTESIAN_POINT('Ctrl Pts',(-12.3880822552564,-14.4260436157556,
117.682923218844)) ;
#188794=CARTESIAN_POINT('Ctrl Pts',(-12.3142784389973,-14.4260436229732,
117.707154343258)) ;
#188795=CARTESIAN_POINT('Ctrl Pts',(-12.2404746227383,-14.4260436301907,
117.731385467671)) ;
#188796=CARTESIAN_POINT('Ctrl Pts',(-12.2382248616783,-14.5016051899087,
117.724533060168)) ;
#188797=CARTESIAN_POINT('Ctrl Pts',(-12.2359751006182,-14.5771667496267,
117.717680652665)) ;
#188798=CARTESIAN_POINT('Ctrl Pts',(-12.3097789168773,-14.5771667424091,
117.693449528252)) ;
#188799=CARTESIAN_POINT('Ctrl Pts',(-12.3835827331363,-14.5771667351915,
117.669218403838)) ;
#188800=CARTESIAN_POINT('Ctrl Pts',(-12.3858324941963,-14.5016051754735,
117.676070811341)) ;
#188801=CARTESIAN_POINT('Ctrl Pts',(-12.4662324280866,-14.4885235205326,
117.956501349458)) ;
#188802=CARTESIAN_POINT('Ctrl Pts',(-12.4621366687095,-14.4137610040608,
117.9440263257)) ;
#188803=CARTESIAN_POINT('Ctrl Pts',(-12.3883328497861,-14.4137609891403,
117.968257441998)) ;
#188804=CARTESIAN_POINT('Ctrl Pts',(-12.3145290308627,-14.4137609742198,
117.992488558297)) ;
#188805=CARTESIAN_POINT('Ctrl Pts',(-12.3186247902397,-14.4885234906916,
118.004963582055)) ;
#188806=CARTESIAN_POINT('Ctrl Pts',(-12.3227205496168,-14.5632860071634,
118.017438605813)) ;
#188807=CARTESIAN_POINT('Ctrl Pts',(-12.3965243685402,-14.5632860220839,
117.993207489514)) ;
#188808=CARTESIAN_POINT('Ctrl Pts',(-12.4703281874636,-14.5632860370044,
117.968976373216)) ;
#188809=CARTESIAN_POINT('Ctrl Pts',(-12.4662324280866,-14.4885235205326,
117.956501349458)) ;
#188810=CARTESIAN_POINT('Ctrl Pts',(-12.542015891352,-14.3988909925641,
118.222731825387)) ;
#188811=CARTESIAN_POINT('Ctrl Pts',(-12.5318901459169,-14.3302736656516,
118.191890437167)) ;
#188812=CARTESIAN_POINT('Ctrl Pts',(-12.4580863228816,-14.3302736334562,
118.216121540941)) ;
#188813=CARTESIAN_POINT('Ctrl Pts',(-12.3842824998462,-14.3302736012609,
118.240352644715)) ;
#188814=CARTESIAN_POINT('Ctrl Pts',(-12.3944082452813,-14.3988909281734,
118.271194032935)) ;
#188815=CARTESIAN_POINT('Ctrl Pts',(-12.4045339907163,-14.4675082550859,
118.302035421155)) ;
#188816=CARTESIAN_POINT('Ctrl Pts',(-12.4783378137517,-14.4675082872812,
118.277804317381)) ;
#188817=CARTESIAN_POINT('Ctrl Pts',(-12.552141636787,-14.4675083194766,
118.253573213606)) ;
#188818=CARTESIAN_POINT('Ctrl Pts',(-12.542015891352,-14.3988909925641,
118.222731825387)) ;
#188819=CARTESIAN_POINT('Ctrl Pts',(-12.6075687803781,-14.2382785177405,
118.457972969816)) ;
#188820=CARTESIAN_POINT('Ctrl Pts',(-12.5921145495609,-14.1807709154062,
118.410901875046)) ;
#188821=CARTESIAN_POINT('Ctrl Pts',(-12.5183107209811,-14.180770872992,
118.435132961933)) ;
#188822=CARTESIAN_POINT('Ctrl Pts',(-12.4445068924013,-14.1807708305777,
118.459364048819)) ;
#188823=CARTESIAN_POINT('Ctrl Pts',(-12.4599611232185,-14.2382784329119,
118.506435143589)) ;
#188824=CARTESIAN_POINT('Ctrl Pts',(-12.4754153540358,-14.2957860352462,
118.553506238358)) ;
#188825=CARTESIAN_POINT('Ctrl Pts',(-12.5492191826155,-14.2957860776604,
118.529275151471)) ;
#188826=CARTESIAN_POINT('Ctrl Pts',(-12.6230230111953,-14.2957861200747,
118.505044064585)) ;
#188827=CARTESIAN_POINT('Ctrl Pts',(-12.6075687803781,-14.2382785177405,
118.457972969816)) ;
#188828=CARTESIAN_POINT('Ctrl Pts',(-12.6567934735026,-14.0201835577284,
118.643239416327)) ;
#188829=CARTESIAN_POINT('Ctrl Pts',(-12.6371477842982,-13.9778166138277,
118.58340181574)) ;
#188830=CARTESIAN_POINT('Ctrl Pts',(-12.5633439504344,-13.9778165664169,
118.607632886532)) ;
#188831=CARTESIAN_POINT('Ctrl Pts',(-12.4895401165705,-13.9778165190061,
118.631863957324)) ;
#188832=CARTESIAN_POINT('Ctrl Pts',(-12.5091858057748,-14.0201834629068,
118.691701557911)) ;
#188833=CARTESIAN_POINT('Ctrl Pts',(-12.5288314949792,-14.0625504068075,
118.751539158498)) ;
#188834=CARTESIAN_POINT('Ctrl Pts',(-12.6026353288431,-14.0625504542183,
118.727308087706)) ;
#188835=CARTESIAN_POINT('Ctrl Pts',(-12.6764391627069,-14.0625505016291,
118.703077016914)) ;
#188836=CARTESIAN_POINT('Ctrl Pts',(-12.6567934735026,-14.0201835577284,
118.643239416327)) ;
#188837=CARTESIAN_POINT('Ctrl Pts',(-12.6860528811102,-13.7575805640437,
118.767919765883)) ;
#188838=CARTESIAN_POINT('Ctrl Pts',(-12.6635985131685,-13.7334844884055,
118.699527383226)) ;
#188839=CARTESIAN_POINT('Ctrl Pts',(-12.5897946740628,-13.7334844436557,
118.723758438053)) ;
#188840=CARTESIAN_POINT('Ctrl Pts',(-12.515990834957,-13.7334843989059,
118.747989492879)) ;
#188841=CARTESIAN_POINT('Ctrl Pts',(-12.5384452028988,-13.7575804745442,
118.816381875535)) ;
#188842=CARTESIAN_POINT('Ctrl Pts',(-12.5608995708405,-13.7816765501825,
118.884774258192)) ;
#188843=CARTESIAN_POINT('Ctrl Pts',(-12.6347034099462,-13.7816765949322,
118.860543203365)) ;
#188844=CARTESIAN_POINT('Ctrl Pts',(-12.7085072490519,-13.781676639682,
118.836312148539)) ;
#188845=CARTESIAN_POINT('Ctrl Pts',(-12.6860528811102,-13.7575805640437,
118.767919765883)) ;
#188846=CARTESIAN_POINT('Ctrl Pts',(-12.6920563199496,-13.4715356144856,
118.821634228625)) ;
#188847=CARTESIAN_POINT('Ctrl Pts',(-12.6684156000948,-13.467375361388,
118.74962840962)) ;
#188848=CARTESIAN_POINT('Ctrl Pts',(-12.5946117570558,-13.4673753229371,
118.773859452466)) ;
#188849=CARTESIAN_POINT('Ctrl Pts',(-12.5208079140168,-13.4673752844861,
118.798090495312)) ;
#188850=CARTESIAN_POINT('Ctrl Pts',(-12.5444486338716,-13.4715355375837,
118.870096314318)) ;
#188851=CARTESIAN_POINT('Ctrl Pts',(-12.5680893537264,-13.4756957906813,
118.942102133323)) ;
#188852=CARTESIAN_POINT('Ctrl Pts',(-12.6418931967654,-13.4756958291323,
118.917871090476)) ;
#188853=CARTESIAN_POINT('Ctrl Pts',(-12.7156970398044,-13.4756958675833,
118.89364004763)) ;
#188854=CARTESIAN_POINT('Ctrl Pts',(-12.6920563199496,-13.4715356144856,
118.821634228625)) ;
#188855=CARTESIAN_POINT('Ctrl Pts',(-12.6739055959979,-13.1815808813972,
118.801789101295)) ;
#188856=CARTESIAN_POINT('Ctrl Pts',(-12.650763023528,-13.1976597435624,
118.731300559009)) ;
#188857=CARTESIAN_POINT('Ctrl Pts',(-12.5769591778132,-13.1976597143198,
118.755531593705)) ;
#188858=CARTESIAN_POINT('Ctrl Pts',(-12.5031553320983,-13.1976596850772,
118.779762628401)) ;
#188859=CARTESIAN_POINT('Ctrl Pts',(-12.5262979045681,-13.1815808229121,
118.850251170687)) ;
#188860=CARTESIAN_POINT('Ctrl Pts',(-12.549440477038,-13.1655019607469,
118.920739712973)) ;
#188861=CARTESIAN_POINT('Ctrl Pts',(-12.6232443227529,-13.1655019899895,
118.896508678276)) ;
#188862=CARTESIAN_POINT('Ctrl Pts',(-12.6970481684677,-13.1655020192321,
118.872277643581)) ;
#188863=CARTESIAN_POINT('Ctrl Pts',(-12.6739055959979,-13.1815808813972,
118.801789101295)) ;
#188864=CARTESIAN_POINT('Ctrl Pts',(-12.6316959301711,-12.9071949482228,
118.708856292433)) ;
#188865=CARTESIAN_POINT('Ctrl Pts',(-12.6107280772881,-12.9424572144763,
118.644991595303)) ;
#188866=CARTESIAN_POINT('Ctrl Pts',(-12.5369242306686,-12.9424571966172,
118.669222627244)) ;
#188867=CARTESIAN_POINT('Ctrl Pts',(-12.4631203840491,-12.9424571787581,
118.693453659185)) ;
#188868=CARTESIAN_POINT('Ctrl Pts',(-12.4840882369321,-12.9071949125046,
118.757318356314)) ;
#188869=CARTESIAN_POINT('Ctrl Pts',(-12.5050560898151,-12.8719326462511,
118.821183053443)) ;
#188870=CARTESIAN_POINT('Ctrl Pts',(-12.5788599364347,-12.8719326641102,
118.796952021502)) ;
#188871=CARTESIAN_POINT('Ctrl Pts',(-12.6526637830542,-12.8719326819694,
118.772720989562)) ;
#188872=CARTESIAN_POINT('Ctrl Pts',(-12.6316959301711,-12.9071949482228,
118.708856292433)) ;
#188873=CARTESIAN_POINT('Ctrl Pts',(-12.5685224634978,-12.6718251326146,
118.551729535265)) ;
#188874=CARTESIAN_POINT('Ctrl Pts',(-12.5512038301306,-12.723574947821,
118.498979772095)) ;
#188875=CARTESIAN_POINT('Ctrl Pts',(-12.4773999834557,-12.7235749374657,
118.523210803867)) ;
#188876=CARTESIAN_POINT('Ctrl Pts',(-12.4035961367808,-12.7235749271105,
118.547441835638)) ;
#188877=CARTESIAN_POINT('Ctrl Pts',(-12.420914770148,-12.6718251119041,
118.600191598809)) ;
#188878=CARTESIAN_POINT('Ctrl Pts',(-12.4382334035152,-12.6200752966978,
118.652941361979)) ;
#188879=CARTESIAN_POINT('Ctrl Pts',(-12.5120372501901,-12.620075307053,
118.628710330207)) ;
#188880=CARTESIAN_POINT('Ctrl Pts',(-12.585841096865,-12.6200753174082,
118.604479298435)) ;
#188881=CARTESIAN_POINT('Ctrl Pts',(-12.5685224634978,-12.6718251326146,
118.551729535265)) ;
#188882=CARTESIAN_POINT('Ctrl Pts',(-12.4874902277502,-12.4884732056212,
118.340373479315)) ;
#188883=CARTESIAN_POINT('Ctrl Pts',(-12.4750698575582,-12.553103678643,
118.302543035572)) ;
#188884=CARTESIAN_POINT('Ctrl Pts',(-12.4012660118782,-12.5531036749217,
118.326774070374)) ;
#188885=CARTESIAN_POINT('Ctrl Pts',(-12.3274621661981,-12.5531036712005,
118.351005105176)) ;
#188886=CARTESIAN_POINT('Ctrl Pts',(-12.33988253639,-12.4884731981787,118.388835548919)) ;
#188887=CARTESIAN_POINT('Ctrl Pts',(-12.3523029065819,-12.4238427251569,
118.426665992661)) ;
#188888=CARTESIAN_POINT('Ctrl Pts',(-12.426106752262,-12.4238427288782,
118.402434957859)) ;
#188889=CARTESIAN_POINT('Ctrl Pts',(-12.4999105979421,-12.4238427325995,
118.378203923057)) ;
#188890=CARTESIAN_POINT('Ctrl Pts',(-12.4874902277502,-12.4884732056212,
118.340373479315)) ;
#188891=CARTESIAN_POINT('Ctrl Pts',(-12.3934765958688,-12.3715751089405,
118.089586721581)) ;
#188892=CARTESIAN_POINT('Ctrl Pts',(-12.3868662577331,-12.4444657268571,
118.06945269815)) ;
#188893=CARTESIAN_POINT('Ctrl Pts',(-12.3130624136099,-12.4444657266469,
118.093683737694)) ;
#188894=CARTESIAN_POINT('Ctrl Pts',(-12.2392585694866,-12.4444657264366,
118.117914777237)) ;
#188895=CARTESIAN_POINT('Ctrl Pts',(-12.2458689076223,-12.3715751085199,
118.138048800668)) ;
#188896=CARTESIAN_POINT('Ctrl Pts',(-12.2524792457579,-12.2986844906033,
118.158182824099)) ;
#188897=CARTESIAN_POINT('Ctrl Pts',(-12.3262830898812,-12.2986844908136,
118.133951784556)) ;
#188898=CARTESIAN_POINT('Ctrl Pts',(-12.4000869340045,-12.2986844910239,
118.109720745012)) ;
#188899=CARTESIAN_POINT('Ctrl Pts',(-12.3934765958688,-12.3715751089405,
118.089586721581)) ;
#188900=CARTESIAN_POINT('Ctrl Pts',(-12.293164555208,-12.3301226383043,
117.819480325447)) ;
#188901=CARTESIAN_POINT('Ctrl Pts',(-12.292815707975,-12.4060167548224,
117.818417793086)) ;
#188902=CARTESIAN_POINT('Ctrl Pts',(-12.2190118649512,-12.4060167550604,
117.842648835978)) ;
#188903=CARTESIAN_POINT('Ctrl Pts',(-12.1452080219273,-12.4060167552985,
117.866879878871)) ;
#188904=CARTESIAN_POINT('Ctrl Pts',(-12.1455568691603,-12.3301226387804,
117.867942411232)) ;
#188905=CARTESIAN_POINT('Ctrl Pts',(-12.1459057163933,-12.2542285222622,
117.869004943594)) ;
#188906=CARTESIAN_POINT('Ctrl Pts',(-12.2197095594172,-12.2542285220242,
117.844773900702)) ;
#188907=CARTESIAN_POINT('Ctrl Pts',(-12.293513402441,-12.2542285217862,
117.820542857809)) ;
#188908=CARTESIAN_POINT('Ctrl Pts',(-12.293164555208,-12.3301226383043,
117.819480325447)) ;
#188909=CARTESIAN_POINT('Ctrl Pts',(-12.19274645429,-12.3662578527564,117.549013076406)) ;
#188910=CARTESIAN_POINT('Ctrl Pts',(-12.1986766714654,-12.4397415757967,
117.567075561145)) ;
#188911=CARTESIAN_POINT('Ctrl Pts',(-12.1248728290033,-12.4397415751055,
117.591306605748)) ;
#188912=CARTESIAN_POINT('Ctrl Pts',(-12.0510689865413,-12.4397415744144,
117.615537650352)) ;
#188913=CARTESIAN_POINT('Ctrl Pts',(-12.0451387693659,-12.366257851374,
117.597475165613)) ;
#188914=CARTESIAN_POINT('Ctrl Pts',(-12.0392085521905,-12.2927741283337,
117.579412680873)) ;
#188915=CARTESIAN_POINT('Ctrl Pts',(-12.1130123946526,-12.2927741290249,
117.55518163627)) ;
#188916=CARTESIAN_POINT('Ctrl Pts',(-12.1868162371146,-12.2927741297161,
117.530950591666)) ;
#188917=CARTESIAN_POINT('Ctrl Pts',(-12.19274645429,-12.3662578527564,117.549013076406)) ;
#188918=CARTESIAN_POINT('Ctrl Pts',(-12.0982790904957,-12.4776432814408,
117.296753345716)) ;
#188919=CARTESIAN_POINT('Ctrl Pts',(-12.1100806154141,-12.5434578807603,
117.33269888651)) ;
#188920=CARTESIAN_POINT('Ctrl Pts',(-12.0362767728468,-12.5434578790229,
117.356929930793)) ;
#188921=CARTESIAN_POINT('Ctrl Pts',(-11.9624729302794,-12.5434578772856,
117.381160975076)) ;
#188922=CARTESIAN_POINT('Ctrl Pts',(-11.950671405361,-12.477643277966,117.345215434282)) ;
#188923=CARTESIAN_POINT('Ctrl Pts',(-11.9388698804425,-12.4118286786465,
117.309269893487)) ;
#188924=CARTESIAN_POINT('Ctrl Pts',(-12.0126737230099,-12.4118286803839,
117.285038849205)) ;
#188925=CARTESIAN_POINT('Ctrl Pts',(-12.0864775655773,-12.4118286821212,
117.260807804922)) ;
#188926=CARTESIAN_POINT('Ctrl Pts',(-12.0982790904957,-12.4776432814408,
117.296753345716)) ;
#188927=CARTESIAN_POINT('Ctrl Pts',(-12.0157313689232,-12.6576066827307,
117.080968227054)) ;
#188928=CARTESIAN_POINT('Ctrl Pts',(-12.0325769790524,-12.71095179343,117.132277237482)) ;
#188929=CARTESIAN_POINT('Ctrl Pts',(-11.9587731356166,-12.7109517930547,
117.15650827912)) ;
#188930=CARTESIAN_POINT('Ctrl Pts',(-11.8849692921809,-12.7109517926794,
117.180739320758)) ;
#188931=CARTESIAN_POINT('Ctrl Pts',(-11.8681236820516,-12.6576066819802,
117.12943031033)) ;
#188932=CARTESIAN_POINT('Ctrl Pts',(-11.8512780719223,-12.604261571281,
117.078121299901)) ;
#188933=CARTESIAN_POINT('Ctrl Pts',(-11.9250819153581,-12.6042615716562,
117.053890258263)) ;
#188934=CARTESIAN_POINT('Ctrl Pts',(-11.9988857587939,-12.6042615720315,
117.029659216626)) ;
#188935=CARTESIAN_POINT('Ctrl Pts',(-12.0157313689232,-12.6576066827307,
117.080968227054)) ;
#188936=CARTESIAN_POINT('Ctrl Pts',(-11.9512285219355,-12.8904240369604,
116.919843926317)) ;
#188937=CARTESIAN_POINT('Ctrl Pts',(-11.9718712658943,-12.9275904125638,
116.982718393653)) ;
#188938=CARTESIAN_POINT('Ctrl Pts',(-11.8980674218478,-12.9275904154763,
117.00694943343)) ;
#188939=CARTESIAN_POINT('Ctrl Pts',(-11.8242635778013,-12.9275904183888,
117.031180473208)) ;
#188940=CARTESIAN_POINT('Ctrl Pts',(-11.8036208338425,-12.8904240427854,
116.968306005872)) ;
#188941=CARTESIAN_POINT('Ctrl Pts',(-11.7829780898837,-12.853257667182,
116.905431538537)) ;
#188942=CARTESIAN_POINT('Ctrl Pts',(-11.8567819339302,-12.8532576642695,
116.881200498759)) ;
#188943=CARTESIAN_POINT('Ctrl Pts',(-11.9305857779767,-12.853257661357,
116.856969458981)) ;
#188944=CARTESIAN_POINT('Ctrl Pts',(-11.9512285219355,-12.8904240369604,
116.919843926317)) ;
#188945=CARTESIAN_POINT('Ctrl Pts',(-11.9077036102862,-13.1612401483887,
116.822691378443)) ;
#188946=CARTESIAN_POINT('Ctrl Pts',(-11.9306826023252,-13.1795510816038,
116.892681680379)) ;
#188947=CARTESIAN_POINT('Ctrl Pts',(-11.8568787581112,-13.1795510898929,
116.916912719647)) ;
#188948=CARTESIAN_POINT('Ctrl Pts',(-11.7830749138971,-13.1795510981819,
116.941143758914)) ;
#188949=CARTESIAN_POINT('Ctrl Pts',(-11.7600959218581,-13.1612401649668,
116.871153456977)) ;
#188950=CARTESIAN_POINT('Ctrl Pts',(-11.737116929819,-13.1429292317516,
116.80116315504)) ;
#188951=CARTESIAN_POINT('Ctrl Pts',(-11.8109207740331,-13.1429292234626,
116.776932115773)) ;
#188952=CARTESIAN_POINT('Ctrl Pts',(-11.8847246182471,-13.1429292151735,
116.752701076506)) ;
#188953=CARTESIAN_POINT('Ctrl Pts',(-11.9077036102862,-13.1612401483887,
116.822691378443)) ;
#188954=CARTESIAN_POINT('Ctrl Pts',(-11.8877528191562,-13.4512163582634,
116.79743209915)) ;
#188955=CARTESIAN_POINT('Ctrl Pts',(-11.9114235075367,-13.4493066869731,
116.869529196403)) ;
#188956=CARTESIAN_POINT('Ctrl Pts',(-11.8376196640733,-13.4493067026551,
116.893760237956)) ;
#188957=CARTESIAN_POINT('Ctrl Pts',(-11.76381582061,-13.4493067183372,116.91799127951)) ;
#188958=CARTESIAN_POINT('Ctrl Pts',(-11.7401451322294,-13.4512163896275,
116.845894182257)) ;
#188959=CARTESIAN_POINT('Ctrl Pts',(-11.7164744438488,-13.4531260609178,
116.773797085004)) ;
#188960=CARTESIAN_POINT('Ctrl Pts',(-11.7902782873122,-13.4531260452357,
116.74956604345)) ;
#188961=CARTESIAN_POINT('Ctrl Pts',(-11.8640821307756,-13.4531260295536,
116.725335001897)) ;
#188962=CARTESIAN_POINT('Ctrl Pts',(-11.8877528191562,-13.4512163582634,
116.79743209915)) ;
#188963=CARTESIAN_POINT('Ctrl Pts',(-11.8921420096609,-13.7384260494091,
116.846260536763)) ;
#188964=CARTESIAN_POINT('Ctrl Pts',(-11.9148067679452,-13.7164599573725,
116.915293733103)) ;
#188965=CARTESIAN_POINT('Ctrl Pts',(-11.8410029264598,-13.7164599797673,
116.939524780681)) ;
#188966=CARTESIAN_POINT('Ctrl Pts',(-11.7671990849745,-13.7164600021621,
116.963755828259)) ;
#188967=CARTESIAN_POINT('Ctrl Pts',(-11.7445343266902,-13.7384260941987,
116.89472263192)) ;
#188968=CARTESIAN_POINT('Ctrl Pts',(-11.721869568406,-13.7603921862353,
116.82568943558)) ;
#188969=CARTESIAN_POINT('Ctrl Pts',(-11.7956734098913,-13.7603921638405,
116.801458388001)) ;
#188970=CARTESIAN_POINT('Ctrl Pts',(-11.8694772513767,-13.7603921414456,
116.777227340423)) ;
#188971=CARTESIAN_POINT('Ctrl Pts',(-11.8921420096609,-13.7384260494091,
116.846260536763)) ;
#188972=CARTESIAN_POINT('Ctrl Pts',(-11.9197697611465,-14.0027479972631,
116.965881508677)) ;
#188973=CARTESIAN_POINT('Ctrl Pts',(-11.939804311693,-13.9622948022858,
117.02690351647)) ;
#188974=CARTESIAN_POINT('Ctrl Pts',(-11.8660004733724,-13.962294829201,
117.051134573688)) ;
#188975=CARTESIAN_POINT('Ctrl Pts',(-11.7921966350518,-13.9622948561163,
117.075365630906)) ;
#188976=CARTESIAN_POINT('Ctrl Pts',(-11.7721620845053,-14.0027480510937,
117.014343623112)) ;
#188977=CARTESIAN_POINT('Ctrl Pts',(-11.7521275339589,-14.0432012460711,
116.953321615319)) ;
#188978=CARTESIAN_POINT('Ctrl Pts',(-11.8259313722795,-14.0432012191558,
116.929090558101)) ;
#188979=CARTESIAN_POINT('Ctrl Pts',(-11.8997352106001,-14.0432011922405,
116.904859500883)) ;
#188980=CARTESIAN_POINT('Ctrl Pts',(-11.9197697611465,-14.0027479972631,
116.965881508677)) ;
#188981=CARTESIAN_POINT('Ctrl Pts',(-11.9678037086644,-14.2248634912547,
117.147598095)) ;
#188982=CARTESIAN_POINT('Ctrl Pts',(-11.9837806505396,-14.1688437545673,
117.196261281318)) ;
#188983=CARTESIAN_POINT('Ctrl Pts',(-11.9099768161194,-14.1688437816251,
117.220492350416)) ;
#188984=CARTESIAN_POINT('Ctrl Pts',(-11.8361729816992,-14.168843808683,
117.244723419513)) ;
#188985=CARTESIAN_POINT('Ctrl Pts',(-11.820196039824,-14.2248635453705,
117.196060233195)) ;
#188986=CARTESIAN_POINT('Ctrl Pts',(-11.8042190979487,-14.2808832820579,
117.147397046877)) ;
#188987=CARTESIAN_POINT('Ctrl Pts',(-11.8780229323689,-14.2808832550001,
117.123165977779)) ;
#188988=CARTESIAN_POINT('Ctrl Pts',(-11.9518267667891,-14.2808832279422,
117.098934908682)) ;
#188989=CARTESIAN_POINT('Ctrl Pts',(-11.9678037086644,-14.2248634912547,
117.147598095)) ;
#188990=CARTESIAN_POINT('Ctrl Pts',(-12.0322684953334,-14.3897502001773,
117.379450247852)) ;
#188991=CARTESIAN_POINT('Ctrl Pts',(-12.0430330101594,-14.3221371212432,
117.412237222224)) ;
#188992=CARTESIAN_POINT('Ctrl Pts',(-11.9692291801814,-14.3221371438564,
117.436468304852)) ;
#188993=CARTESIAN_POINT('Ctrl Pts',(-11.8954253502033,-14.3221371664696,
117.460699387479)) ;
#188994=CARTESIAN_POINT('Ctrl Pts',(-11.8846608353774,-14.3897502454037,
117.427912413107)) ;
#188995=CARTESIAN_POINT('Ctrl Pts',(-11.8738963205514,-14.4573633243378,
117.395125438735)) ;
#188996=CARTESIAN_POINT('Ctrl Pts',(-11.9477001505294,-14.4573633017246,
117.370894356107)) ;
#188997=CARTESIAN_POINT('Ctrl Pts',(-12.0215039805075,-14.4573632791114,
117.34666327348)) ;
#188998=CARTESIAN_POINT('Ctrl Pts',(-12.0322684953334,-14.3897502001773,
117.379450247852)) ;
#188999=CARTESIAN_POINT('Ctrl Pts',(-12.107744276387,-14.4847583322739,
117.644855028012)) ;
#189000=CARTESIAN_POINT('Ctrl Pts',(-12.1125197986048,-14.4104140333925,
117.659400497042)) ;
#189001=CARTESIAN_POINT('Ctrl Pts',(-12.0387159728293,-14.4104140454356,
117.68363159247)) ;
#189002=CARTESIAN_POINT('Ctrl Pts',(-11.9649121470538,-14.4104140574787,
117.707862687898)) ;
#189003=CARTESIAN_POINT('Ctrl Pts',(-11.960136624836,-14.4847583563601,
117.693317218868)) ;
#189004=CARTESIAN_POINT('Ctrl Pts',(-11.9553611026181,-14.5591026552415,
117.678771749837)) ;
#189005=CARTESIAN_POINT('Ctrl Pts',(-12.0291649283937,-14.5591026431984,
117.654540654409)) ;
#189006=CARTESIAN_POINT('Ctrl Pts',(-12.1029687541692,-14.5591026311553,
117.630309558981)) ;
#189007=CARTESIAN_POINT('Ctrl Pts',(-12.107744276387,-14.4847583322739,
117.644855028012)) ;
#189008=CARTESIAN_POINT('Ctrl Pts',(-12.1876872494525,-14.5032991769,117.923727178985)) ;
#189009=CARTESIAN_POINT('Ctrl Pts',(-12.1861561390636,-14.4275531479525,
117.91906366252)) ;
#189010=CARTESIAN_POINT('Ctrl Pts',(-12.1123523160226,-14.4275531440522,
117.943294766276)) ;
#189011=CARTESIAN_POINT('Ctrl Pts',(-12.0385484929815,-14.427553140152,
117.967525870033)) ;
#189012=CARTESIAN_POINT('Ctrl Pts',(-12.0400796033704,-14.5032991690996,
117.972189386498)) ;
#189013=CARTESIAN_POINT('Ctrl Pts',(-12.0416107137593,-14.5790451980471,
117.976852902963)) ;
#189014=CARTESIAN_POINT('Ctrl Pts',(-12.1154145368004,-14.5790452019473,
117.952621799206)) ;
#189015=CARTESIAN_POINT('Ctrl Pts',(-12.1892183598415,-14.5790452058476,
117.928390695449)) ;
#189016=CARTESIAN_POINT('Ctrl Pts',(-12.1876872494525,-14.5032991769,117.923727178985)) ;
#189017=CARTESIAN_POINT('Ctrl Pts',(-12.26622892562,-14.4441301859155,118.198469361747)) ;
#189018=CARTESIAN_POINT('Ctrl Pts',(-12.2584771052313,-14.3724053611762,
118.174858566166)) ;
#189019=CARTESIAN_POINT('Ctrl Pts',(-12.1846732836344,-14.3724053372545,
118.199089674322)) ;
#189020=CARTESIAN_POINT('Ctrl Pts',(-12.1108694620375,-14.3724053133327,
118.223320782477)) ;
#189021=CARTESIAN_POINT('Ctrl Pts',(-12.1186212824263,-14.444130138072,
118.246931578058)) ;
#189022=CARTESIAN_POINT('Ctrl Pts',(-12.1263731028151,-14.5158549628113,
118.270542373639)) ;
#189023=CARTESIAN_POINT('Ctrl Pts',(-12.2001769244119,-14.5158549867331,
118.246311265484)) ;
#189024=CARTESIAN_POINT('Ctrl Pts',(-12.2739807460088,-14.5158550106548,
118.222080157328)) ;
#189025=CARTESIAN_POINT('Ctrl Pts',(-12.26622892562,-14.4441301859155,118.198469361747)) ;
#189026=CARTESIAN_POINT('Ctrl Pts',(-12.3365380163311,-14.3114937407021,
118.448066596164)) ;
#189027=CARTESIAN_POINT('Ctrl Pts',(-12.3231327195336,-14.2489252476856,
118.407236223487)) ;
#189028=CARTESIAN_POINT('Ctrl Pts',(-12.2493288970295,-14.2489252018326,
118.431467328879)) ;
#189029=CARTESIAN_POINT('Ctrl Pts',(-12.1755250745255,-14.2489251559797,
118.455698434271)) ;
#189030=CARTESIAN_POINT('Ctrl Pts',(-12.1889303713229,-14.3114936489961,
118.496528806949)) ;
#189031=CARTESIAN_POINT('Ctrl Pts',(-12.2023356681204,-14.3740621420126,
118.537359179626)) ;
#189032=CARTESIAN_POINT('Ctrl Pts',(-12.2761394906244,-14.3740621878656,
118.513128074234)) ;
#189033=CARTESIAN_POINT('Ctrl Pts',(-12.3499433131285,-14.3740622337185,
118.488896968842)) ;
#189034=CARTESIAN_POINT('Ctrl Pts',(-12.3365380163311,-14.3114937407021,
118.448066596164)) ;
#189035=CARTESIAN_POINT('Ctrl Pts',(-12.3930354443869,-14.114774307687,
118.655627115153)) ;
#189036=CARTESIAN_POINT('Ctrl Pts',(-12.3749320945125,-14.0658491597741,
118.600487230699)) ;
#189037=CARTESIAN_POINT('Ctrl Pts',(-12.30112826882,-14.0658490924885,118.624718326379)) ;
#189038=CARTESIAN_POINT('Ctrl Pts',(-12.2273244431275,-14.0658490252028,
118.64894942206)) ;
#189039=CARTESIAN_POINT('Ctrl Pts',(-12.245427793002,-14.1147741731156,
118.704089306515)) ;
#189040=CARTESIAN_POINT('Ctrl Pts',(-12.2635311428765,-14.1636993210285,
118.75922919097)) ;
#189041=CARTESIAN_POINT('Ctrl Pts',(-12.3373349685689,-14.1636993883142,
118.734998095289)) ;
#189042=CARTESIAN_POINT('Ctrl Pts',(-12.4111387942614,-14.1636994555999,
118.710766999608)) ;
#189043=CARTESIAN_POINT('Ctrl Pts',(-12.3930354443869,-14.114774307687,
118.655627115153)) ;
#189044=CARTESIAN_POINT('Ctrl Pts',(-12.4308165590885,-13.8682921869894,
118.806151894352)) ;
#189045=CARTESIAN_POINT('Ctrl Pts',(-12.4093156019594,-13.8365043277557,
118.740663446289)) ;
#189046=CARTESIAN_POINT('Ctrl Pts',(-12.3355117707898,-13.8365042424835,
118.764894525288)) ;
#189047=CARTESIAN_POINT('Ctrl Pts',(-12.2617079396203,-13.8365041572113,
118.789125604286)) ;
#189048=CARTESIAN_POINT('Ctrl Pts',(-12.2832088967495,-13.868292016445,
118.854614052349)) ;
#189049=CARTESIAN_POINT('Ctrl Pts',(-12.3047098538786,-13.9000798756787,
118.920102500412)) ;
#189050=CARTESIAN_POINT('Ctrl Pts',(-12.3785136850481,-13.9000799609509,
118.895871421414)) ;
#189051=CARTESIAN_POINT('Ctrl Pts',(-12.4523175162177,-13.9000800462231,
118.871640342415)) ;
#189052=CARTESIAN_POINT('Ctrl Pts',(-12.4308165590885,-13.8682921869894,
118.806151894352)) ;
#189053=CARTESIAN_POINT('Ctrl Pts',(-12.4465020803455,-13.5896536678714,
118.889371904184)) ;
#189054=CARTESIAN_POINT('Ctrl Pts',(-12.4231412470967,-13.5772729173919,
118.818218573456)) ;
#189055=CARTESIAN_POINT('Ctrl Pts',(-12.3493374086623,-13.5772728198901,
118.842449630327)) ;
#189056=CARTESIAN_POINT('Ctrl Pts',(-12.2755335702279,-13.5772727223883,
118.866680687197)) ;
#189057=CARTESIAN_POINT('Ctrl Pts',(-12.2988944034766,-13.5896534728677,
118.937834017926)) ;
#189058=CARTESIAN_POINT('Ctrl Pts',(-12.3222552367254,-13.6020342233472,
119.008987348655)) ;
#189059=CARTESIAN_POINT('Ctrl Pts',(-12.3960590751598,-13.6020343208491,
118.984756291784)) ;
#189060=CARTESIAN_POINT('Ctrl Pts',(-12.4698629135942,-13.6020344183509,
118.960525234913)) ;
#189061=CARTESIAN_POINT('Ctrl Pts',(-12.4465020803455,-13.5896536678714,
118.889371904184)) ;
#189062=CARTESIAN_POINT('Ctrl Pts',(-12.4381763312558,-13.2982167701219,
118.899517978675)) ;
#189063=CARTESIAN_POINT('Ctrl Pts',(-12.4146278754705,-13.3061648042617,
118.827793179891)) ;
#189064=CARTESIAN_POINT('Ctrl Pts',(-12.3408240286096,-13.3061647018305,
118.852024211096)) ;
#189065=CARTESIAN_POINT('Ctrl Pts',(-12.2670201817487,-13.3061645993992,
118.876255242301)) ;
#189066=CARTESIAN_POINT('Ctrl Pts',(-12.290568637534,-13.2982165652594,
118.947980041085)) ;
#189067=CARTESIAN_POINT('Ctrl Pts',(-12.3141170933193,-13.2902685311196,
119.019704839869)) ;
#189068=CARTESIAN_POINT('Ctrl Pts',(-12.3879209401802,-13.2902686335509,
118.995473808664)) ;
#189069=CARTESIAN_POINT('Ctrl Pts',(-12.4617247870411,-13.2902687359821,
118.971242777458)) ;
#189070=CARTESIAN_POINT('Ctrl Pts',(-12.4381763312558,-13.2982167701219,
118.899517978675)) ;
#189071=CARTESIAN_POINT('Ctrl Pts',(-12.4056299449732,-13.0155927262678,
118.835868127191)) ;
#189072=CARTESIAN_POINT('Ctrl Pts',(-12.3835849842552,-13.0432841492844,
118.768722731737)) ;
#189073=CARTESIAN_POINT('Ctrl Pts',(-12.3097811286645,-13.0432840507906,
118.792953736353)) ;
#189074=CARTESIAN_POINT('Ctrl Pts',(-12.2359772730738,-13.0432839522968,
118.817184740968)) ;
#189075=CARTESIAN_POINT('Ctrl Pts',(-12.2580222337918,-13.0155925292803,
118.884330136422)) ;
#189076=CARTESIAN_POINT('Ctrl Pts',(-12.2800671945098,-12.9879011062637,
118.951475531876)) ;
#189077=CARTESIAN_POINT('Ctrl Pts',(-12.3538710501005,-12.9879012047575,
118.92724452726)) ;
#189078=CARTESIAN_POINT('Ctrl Pts',(-12.4276749056913,-12.9879013032513,
118.903013522645)) ;
#189079=CARTESIAN_POINT('Ctrl Pts',(-12.4056299449732,-13.0155927262678,
118.835868127191)) ;
#189080=CARTESIAN_POINT('Ctrl Pts',(-12.3507015426636,-12.7625129426041,
118.703939374418)) ;
#189081=CARTESIAN_POINT('Ctrl Pts',(-12.3317271438295,-12.8079141772025,
118.646146414998)) ;
#189082=CARTESIAN_POINT('Ctrl Pts',(-12.2579232802105,-12.8079140912617,
118.67037739516)) ;
#189083=CARTESIAN_POINT('Ctrl Pts',(-12.1841194165914,-12.8079140053209,
118.694608375323)) ;
#189084=CARTESIAN_POINT('Ctrl Pts',(-12.2030938154255,-12.7625127707225,
118.752401334743)) ;
#189085=CARTESIAN_POINT('Ctrl Pts',(-12.2220682142596,-12.7171115361241,
118.810194294164)) ;
#189086=CARTESIAN_POINT('Ctrl Pts',(-12.2958720778787,-12.7171116220649,
118.785963314002)) ;
#189087=CARTESIAN_POINT('Ctrl Pts',(-12.3696759414977,-12.7171117080057,
118.761732333839)) ;
#189088=CARTESIAN_POINT('Ctrl Pts',(-12.3507015426636,-12.7625129426041,
118.703939374418)) ;
#189089=CARTESIAN_POINT('Ctrl Pts',(-12.276179464868,-12.5553594059935,
118.512465785977)) ;
#189090=CARTESIAN_POINT('Ctrl Pts',(-12.2616450921185,-12.6152904005215,
118.468196429597)) ;
#189091=CARTESIAN_POINT('Ctrl Pts',(-12.1878412218671,-12.6152903344179,
118.492427389559)) ;
#189092=CARTESIAN_POINT('Ctrl Pts',(-12.1140373516158,-12.6152902683143,
118.516658349521)) ;
#189093=CARTESIAN_POINT('Ctrl Pts',(-12.1285717243653,-12.5553592737864,
118.5609277059)) ;
#189094=CARTESIAN_POINT('Ctrl Pts',(-12.1431060971148,-12.4954282792585,
118.60519706228)) ;
#189095=CARTESIAN_POINT('Ctrl Pts',(-12.2169099673661,-12.4954283453621,
118.580966102318)) ;
#189096=CARTESIAN_POINT('Ctrl Pts',(-12.2907138376175,-12.4954284114656,
118.556735142357)) ;
#189097=CARTESIAN_POINT('Ctrl Pts',(-12.276179464868,-12.5553594059935,
118.512465785977)) ;
#189098=CARTESIAN_POINT('Ctrl Pts',(-12.1866037708491,-12.4101759250027,
118.275199832939)) ;
#189099=CARTESIAN_POINT('Ctrl Pts',(-12.1775656705167,-12.4803322250042,
118.247671235534)) ;
#189100=CARTESIAN_POINT('Ctrl Pts',(-12.1037617959182,-12.4803321844946,
118.271902182255)) ;
#189101=CARTESIAN_POINT('Ctrl Pts',(-12.0299579213197,-12.4803321439849,
118.296133128976)) ;
#189102=CARTESIAN_POINT('Ctrl Pts',(-12.0389960216522,-12.4101758439834,
118.323661726381)) ;
#189103=CARTESIAN_POINT('Ctrl Pts',(-12.0480341219847,-12.3400195439819,
118.351190323787)) ;
#189104=CARTESIAN_POINT('Ctrl Pts',(-12.1218379965832,-12.3400195844916,
118.326959377066)) ;
#189105=CARTESIAN_POINT('Ctrl Pts',(-12.1956418711816,-12.3400196250012,
118.302728430345)) ;
#189106=CARTESIAN_POINT('Ctrl Pts',(-12.1866037708491,-12.4101759250027,
118.275199832939)) ;
#189107=CARTESIAN_POINT('Ctrl Pts',(-12.0884786810735,-12.3376963152453,
118.011668844001)) ;
#189108=CARTESIAN_POINT('Ctrl Pts',(-12.085546690365,-12.4130169374688,
118.002738471319)) ;
#189109=CARTESIAN_POINT('Ctrl Pts',(-12.0117428139613,-12.4130169250925,
118.026969412542)) ;
#189110=CARTESIAN_POINT('Ctrl Pts',(-11.9379389375575,-12.4130169127163,
118.051200353765)) ;
#189111=CARTESIAN_POINT('Ctrl Pts',(-11.940870928266,-12.3376962904928,
118.060130726446)) ;
#189112=CARTESIAN_POINT('Ctrl Pts',(-11.9438029189746,-12.2623756682694,
118.069061099127)) ;
#189113=CARTESIAN_POINT('Ctrl Pts',(-12.0176067953783,-12.2623756806456,
118.044830157905)) ;
#189114=CARTESIAN_POINT('Ctrl Pts',(-12.091410671782,-12.2623756930219,
118.020599216682)) ;
#189115=CARTESIAN_POINT('Ctrl Pts',(-12.0884786810735,-12.3376963152453,
118.011668844001)) ;
#189116=CARTESIAN_POINT('Ctrl Pts',(-11.9868042804343,-12.3422639933637,
117.737570588473)) ;
#189117=CARTESIAN_POINT('Ctrl Pts',(-11.9902301097811,-12.4173784848516,
117.748005109908)) ;
#189118=CARTESIAN_POINT('Ctrl Pts',(-11.9164262344824,-12.4173785007626,
117.772236054496)) ;
#189119=CARTESIAN_POINT('Ctrl Pts',(-11.8426223591838,-12.4173785166736,
117.796466999085)) ;
#189120=CARTESIAN_POINT('Ctrl Pts',(-11.8391965298369,-12.3422640251856,
117.786032477649)) ;
#189121=CARTESIAN_POINT('Ctrl Pts',(-11.83577070049,-12.2671495336977,117.775597956213)) ;
#189122=CARTESIAN_POINT('Ctrl Pts',(-11.9095745757887,-12.2671495177867,
117.751367011625)) ;
#189123=CARTESIAN_POINT('Ctrl Pts',(-11.9833784510874,-12.2671495018757,
117.727136067037)) ;
#189124=CARTESIAN_POINT('Ctrl Pts',(-11.9868042804343,-12.3422639933637,
117.737570588473)) ;
#189125=CARTESIAN_POINT('Ctrl Pts',(-11.8890994352425,-12.4243537888734,
117.475457869454)) ;
#189126=CARTESIAN_POINT('Ctrl Pts',(-11.8986177488891,-12.4938495197523,
117.504449115127)) ;
#189127=CARTESIAN_POINT('Ctrl Pts',(-11.8248138772114,-12.4938495605533,
117.528680070744)) ;
#189128=CARTESIAN_POINT('Ctrl Pts',(-11.7510100055337,-12.4938496013543,
117.552911026361)) ;
#189129=CARTESIAN_POINT('Ctrl Pts',(-11.7414916918871,-12.4243538704754,
117.523919780688)) ;
#189130=CARTESIAN_POINT('Ctrl Pts',(-11.7319733782405,-12.3548581395965,
117.494928535016)) ;
#189131=CARTESIAN_POINT('Ctrl Pts',(-11.8057772499182,-12.3548580987955,
117.470697579399)) ;
#189132=CARTESIAN_POINT('Ctrl Pts',(-11.879581121596,-12.3548580579945,
117.446466623782)) ;
#189133=CARTESIAN_POINT('Ctrl Pts',(-11.8890994352425,-12.4243537888734,
117.475457869454)) ;
#189134=CARTESIAN_POINT('Ctrl Pts',(-11.8017044319056,-12.5764990896273,
117.244563346778)) ;
#189135=CARTESIAN_POINT('Ctrl Pts',(-11.8166083589498,-12.6354761389067,
117.289958301969)) ;
#189136=CARTESIAN_POINT('Ctrl Pts',(-11.7428044925836,-12.6354761997948,
117.314189273764)) ;
#189137=CARTESIAN_POINT('Ctrl Pts',(-11.6690006262173,-12.6354762606829,
117.338420245559)) ;
#189138=CARTESIAN_POINT('Ctrl Pts',(-11.6540966991731,-12.5764992114035,
117.293025290368)) ;
#189139=CARTESIAN_POINT('Ctrl Pts',(-11.6391927721289,-12.5175221621241,
117.247630335178)) ;
#189140=CARTESIAN_POINT('Ctrl Pts',(-11.7129966384952,-12.517522101236,
117.223399363383)) ;
#189141=CARTESIAN_POINT('Ctrl Pts',(-11.7868005048614,-12.5175220403479,
117.199168391588)) ;
#189142=CARTESIAN_POINT('Ctrl Pts',(-11.8017044319056,-12.5764990896273,
117.244563346778)) ;
#189143=CARTESIAN_POINT('Ctrl Pts',(-11.7291135872937,-12.7898749801387,
117.058995916747)) ;
#189144=CARTESIAN_POINT('Ctrl Pts',(-11.7483728632372,-12.8340435200322,
117.117656562069)) ;
#189145=CARTESIAN_POINT('Ctrl Pts',(-11.6745690038856,-12.834043593478,
117.14188755523)) ;
#189146=CARTESIAN_POINT('Ctrl Pts',(-11.600765144534,-12.8340436669238,
117.16611854839)) ;
#189147=CARTESIAN_POINT('Ctrl Pts',(-11.5815058685905,-12.7898751270303,
117.107457903068)) ;
#189148=CARTESIAN_POINT('Ctrl Pts',(-11.5622465926471,-12.7457065871368,
117.048797257746)) ;
#189149=CARTESIAN_POINT('Ctrl Pts',(-11.6360504519986,-12.745706513691,
117.024566264585)) ;
#189150=CARTESIAN_POINT('Ctrl Pts',(-11.7098543113502,-12.7457064402452,
117.000335271425)) ;
#189151=CARTESIAN_POINT('Ctrl Pts',(-11.7291135872937,-12.7898749801387,
117.058995916747)) ;
#189152=CARTESIAN_POINT('Ctrl Pts',(-11.6764341261523,-13.0489854290901,
116.934128082032)) ;
#189153=CARTESIAN_POINT('Ctrl Pts',(-11.6986642223819,-13.0751301371368,
117.001837366752)) ;
#189154=CARTESIAN_POINT('Ctrl Pts',(-11.6248603705172,-13.0751302144171,
117.026068382717)) ;
#189155=CARTESIAN_POINT('Ctrl Pts',(-11.5510565186525,-13.0751302916973,
117.050299398681)) ;
#189156=CARTESIAN_POINT('Ctrl Pts',(-11.5288264224229,-13.0489855836505,
116.982590113961)) ;
#189157=CARTESIAN_POINT('Ctrl Pts',(-11.5065963261933,-13.0228408756037,
116.914880829242)) ;
#189158=CARTESIAN_POINT('Ctrl Pts',(-11.580400178058,-13.0228407983235,
116.890649813277)) ;
#189159=CARTESIAN_POINT('Ctrl Pts',(-11.6542040299227,-13.0228407210433,
116.866418797313)) ;
#189160=CARTESIAN_POINT('Ctrl Pts',(-11.6764341261523,-13.0489854290901,
116.934128082032)) ;
#189161=CARTESIAN_POINT('Ctrl Pts',(-11.6468794476633,-13.3335116646803,
116.879553756773)) ;
#189162=CARTESIAN_POINT('Ctrl Pts',(-11.6704731941443,-13.3398303944034,
116.951416500274)) ;
#189163=CARTESIAN_POINT('Ctrl Pts',(-11.5966693491189,-13.3398304688619,
116.97564753707)) ;
#189164=CARTESIAN_POINT('Ctrl Pts',(-11.5228655040934,-13.3398305433204,
116.999878573866)) ;
#189165=CARTESIAN_POINT('Ctrl Pts',(-11.4992717576124,-13.3335118135973,
116.928015830364)) ;
#189166=CARTESIAN_POINT('Ctrl Pts',(-11.4756780111314,-13.3271930838743,
116.856153086863)) ;
#189167=CARTESIAN_POINT('Ctrl Pts',(-11.5494818561569,-13.3271930094158,
116.831922050067)) ;
#189168=CARTESIAN_POINT('Ctrl Pts',(-11.6232857011823,-13.3271929349573,
116.807691013271)) ;
#189169=CARTESIAN_POINT('Ctrl Pts',(-11.6468794476633,-13.3335116646803,
116.879553756773)) ;
#189170=CARTESIAN_POINT('Ctrl Pts',(-11.6414627303795,-13.6230727255243,
116.898378600556)) ;
#189171=CARTESIAN_POINT('Ctrl Pts',(-11.6647393194538,-13.6091838535946,
116.969275333898)) ;
#189172=CARTESIAN_POINT('Ctrl Pts',(-11.5909354802481,-13.6091839202508,
116.99350638842)) ;
#189173=CARTESIAN_POINT('Ctrl Pts',(-11.5171316410424,-13.6091839869071,
117.017737442942)) ;
#189174=CARTESIAN_POINT('Ctrl Pts',(-11.4938550519681,-13.6230728588367,
116.9468407096)) ;
#189175=CARTESIAN_POINT('Ctrl Pts',(-11.4705784628939,-13.6369617307664,
116.875943976258)) ;
#189176=CARTESIAN_POINT('Ctrl Pts',(-11.5443823020996,-13.6369616641102,
116.851712921736)) ;
#189177=CARTESIAN_POINT('Ctrl Pts',(-11.6181861413053,-13.6369615974539,
116.827481867214)) ;
#189178=CARTESIAN_POINT('Ctrl Pts',(-11.6414627303795,-13.6230727255243,
116.898378600556)) ;
#189179=CARTESIAN_POINT('Ctrl Pts',(-11.6598233366193,-13.8991091738745,
116.989763695794)) ;
#189180=CARTESIAN_POINT('Ctrl Pts',(-11.681119458354,-13.8659263158171,
117.054628245326)) ;
#189181=CARTESIAN_POINT('Ctrl Pts',(-11.6073156234127,-13.8659263690519,
117.078859312837)) ;
#189182=CARTESIAN_POINT('Ctrl Pts',(-11.5335117884714,-13.8659264222868,
117.103090380348)) ;
#189183=CARTESIAN_POINT('Ctrl Pts',(-11.5122156667368,-13.8991092803442,
117.038225830815)) ;
#189184=CARTESIAN_POINT('Ctrl Pts',(-11.4909195450021,-13.9322921384017,
116.973361281282)) ;
#189185=CARTESIAN_POINT('Ctrl Pts',(-11.5647233799434,-13.9322920851668,
116.949130213771)) ;
#189186=CARTESIAN_POINT('Ctrl Pts',(-11.6385272148846,-13.9322920319319,
116.924899146261)) ;
#189187=CARTESIAN_POINT('Ctrl Pts',(-11.6598233366193,-13.8991091738745,
116.989763695794)) ;
#189188=CARTESIAN_POINT('Ctrl Pts',(-11.70011193344,-14.1412745978093,117.148019110991)) ;
#189189=CARTESIAN_POINT('Ctrl Pts',(-11.7178919586761,-14.0911330408888,
117.202174198091)) ;
#189190=CARTESIAN_POINT('Ctrl Pts',(-11.6440881259211,-14.0911330778526,
117.22640527226)) ;
#189191=CARTESIAN_POINT('Ctrl Pts',(-11.5702842931661,-14.0911331148164,
117.25063634643)) ;
#189192=CARTESIAN_POINT('Ctrl Pts',(-11.55250426793,-14.141274671737,117.19648125933)) ;
#189193=CARTESIAN_POINT('Ctrl Pts',(-11.5347242426939,-14.1914162286575,
117.14232617223)) ;
#189194=CARTESIAN_POINT('Ctrl Pts',(-11.6085280754489,-14.1914161916937,
117.118095098061)) ;
#189195=CARTESIAN_POINT('Ctrl Pts',(-11.6823319082039,-14.1914161547299,
117.093864023891)) ;
#189196=CARTESIAN_POINT('Ctrl Pts',(-11.70011193344,-14.1412745978093,117.148019110991)) ;
#189197=CARTESIAN_POINT('Ctrl Pts',(-11.7587869921287,-14.3313662237517,
117.362325380269)) ;
#189198=CARTESIAN_POINT('Ctrl Pts',(-11.7717607368277,-14.2678756388728,
117.401841312536)) ;
#189199=CARTESIAN_POINT('Ctrl Pts',(-11.6979569041075,-14.2678756602265,
117.426072386812)) ;
#189200=CARTESIAN_POINT('Ctrl Pts',(-11.6241530713873,-14.2678756815801,
117.450303461088)) ;
#189201=CARTESIAN_POINT('Ctrl Pts',(-11.6111793266882,-14.331366266459,
117.41078752882)) ;
#189202=CARTESIAN_POINT('Ctrl Pts',(-11.5982055819891,-14.3948568513378,
117.371271596553)) ;
#189203=CARTESIAN_POINT('Ctrl Pts',(-11.6720094147093,-14.3948568299842,
117.347040522277)) ;
#189204=CARTESIAN_POINT('Ctrl Pts',(-11.7458132474296,-14.3948568086305,
117.322809448002)) ;
#189205=CARTESIAN_POINT('Ctrl Pts',(-11.7587869921287,-14.3313662237517,
117.362325380269)) ;
#189206=CARTESIAN_POINT('Ctrl Pts',(-11.8298919850122,-14.4547660222928,
117.614104425803)) ;
#189207=CARTESIAN_POINT('Ctrl Pts',(-11.8371920680467,-14.3825637894308,
117.6363393002)) ;
#189208=CARTESIAN_POINT('Ctrl Pts',(-11.7633882348918,-14.3825637991791,
117.660570373151)) ;
#189209=CARTESIAN_POINT('Ctrl Pts',(-11.6895844017367,-14.3825638089273,
117.684801446103)) ;
#189210=CARTESIAN_POINT('Ctrl Pts',(-11.6822843187022,-14.4547660417892,
117.662566571706)) ;
#189211=CARTESIAN_POINT('Ctrl Pts',(-11.6749842356676,-14.5269682746512,
117.64033169731)) ;
#189212=CARTESIAN_POINT('Ctrl Pts',(-11.7487880688226,-14.526968264903,
117.616100624358)) ;
#189213=CARTESIAN_POINT('Ctrl Pts',(-11.8225919019776,-14.5269682551548,
117.591869551407)) ;
#189214=CARTESIAN_POINT('Ctrl Pts',(-11.8298919850122,-14.4547660222928,
117.614104425803)) ;
#189215=CARTESIAN_POINT('Ctrl Pts',(-11.9091252270702,-14.5053328691454,
117.891029238867)) ;
#189216=CARTESIAN_POINT('Ctrl Pts',(-11.9101675159898,-14.4294900381805,
117.894203882266)) ;
#189217=CARTESIAN_POINT('Ctrl Pts',(-11.8363636802989,-14.4294900382422,
117.918434947493)) ;
#189218=CARTESIAN_POINT('Ctrl Pts',(-11.762559844608,-14.4294900383039,
117.942666012721)) ;
#189219=CARTESIAN_POINT('Ctrl Pts',(-11.7615175556885,-14.5053328692688,
117.939491369322)) ;
#189220=CARTESIAN_POINT('Ctrl Pts',(-11.7604752667689,-14.5811757002337,
117.936316725924)) ;
#189221=CARTESIAN_POINT('Ctrl Pts',(-11.8342791024598,-14.581175700172,
117.912085660696)) ;
#189222=CARTESIAN_POINT('Ctrl Pts',(-11.9080829381506,-14.5811757001103,
117.887854595469)) ;
#189223=CARTESIAN_POINT('Ctrl Pts',(-11.9091252270702,-14.5053328691454,
117.891029238867)) ;
#189224=CARTESIAN_POINT('Ctrl Pts',(-11.9891525457306,-14.4771328889757,
118.170301722369)) ;
#189225=CARTESIAN_POINT('Ctrl Pts',(-11.9838733903065,-14.4031442032382,
118.154222266415)) ;
#189226=CARTESIAN_POINT('Ctrl Pts',(-11.9100695518998,-14.4031441988983,
118.17845332337)) ;
#189227=CARTESIAN_POINT('Ctrl Pts',(-11.8362657134931,-14.4031441945584,
118.202684380326)) ;
#189228=CARTESIAN_POINT('Ctrl Pts',(-11.8415448689172,-14.4771328802959,
118.21876383628)) ;
#189229=CARTESIAN_POINT('Ctrl Pts',(-11.8468240243413,-14.5511215660333,
118.234843292234)) ;
#189230=CARTESIAN_POINT('Ctrl Pts',(-11.920627862748,-14.5511215703732,
118.210612235279)) ;
#189231=CARTESIAN_POINT('Ctrl Pts',(-11.9944317011547,-14.5511215747131,
118.186381178323)) ;
#189232=CARTESIAN_POINT('Ctrl Pts',(-11.9891525457306,-14.4771328889757,
118.170301722369)) ;
#189233=CARTESIAN_POINT('Ctrl Pts',(-12.0631580436741,-14.3740575561619,
118.430997938471)) ;
#189234=CARTESIAN_POINT('Ctrl Pts',(-12.0519733519711,-14.3071548458452,
118.396931171973)) ;
#189235=CARTESIAN_POINT('Ctrl Pts',(-11.9781695115022,-14.307154840074,
118.421162222647)) ;
#189236=CARTESIAN_POINT('Ctrl Pts',(-11.9043656710333,-14.3071548343027,
118.445393273322)) ;
#189237=CARTESIAN_POINT('Ctrl Pts',(-11.9155503627364,-14.3740575446194,
118.479460039819)) ;
#189238=CARTESIAN_POINT('Ctrl Pts',(-11.9267350544394,-14.4409602549361,
118.513526806317)) ;
#189239=CARTESIAN_POINT('Ctrl Pts',(-12.0005388949083,-14.4409602607073,
118.489295755643)) ;
#189240=CARTESIAN_POINT('Ctrl Pts',(-12.0743427353772,-14.4409602664786,
118.465064704968)) ;
#189241=CARTESIAN_POINT('Ctrl Pts',(-12.0631580436741,-14.3740575561619,
118.430997938471)) ;
#189242=CARTESIAN_POINT('Ctrl Pts',(-12.1262287274815,-14.2012582823737,
118.658729046755)) ;
#189243=CARTESIAN_POINT('Ctrl Pts',(-12.1098857541428,-14.1463204404916,
118.608950986816)) ;
#189244=CARTESIAN_POINT('Ctrl Pts',(-12.0360819115211,-14.1463204373001,
118.633182030934)) ;
#189245=CARTESIAN_POINT('Ctrl Pts',(-11.9622780688994,-14.1463204341086,
118.657413075051)) ;
#189246=CARTESIAN_POINT('Ctrl Pts',(-11.9786210422382,-14.2012582759907,
118.70719113499)) ;
#189247=CARTESIAN_POINT('Ctrl Pts',(-11.9949640155769,-14.2561961178728,
118.756969194928)) ;
#189248=CARTESIAN_POINT('Ctrl Pts',(-12.0687678581985,-14.2561961210643,
118.732738150811)) ;
#189249=CARTESIAN_POINT('Ctrl Pts',(-12.1425717008202,-14.2561961242558,
118.708507106693)) ;
#189250=CARTESIAN_POINT('Ctrl Pts',(-12.1262287274815,-14.2012582823737,
118.658729046755)) ;
#189251=CARTESIAN_POINT('Ctrl Pts',(-12.1720317469942,-13.9726608385018,
118.833715114846)) ;
#189252=CARTESIAN_POINT('Ctrl Pts',(-12.1517317413815,-13.9336031304971,
118.771884573146)) ;
#189253=CARTESIAN_POINT('Ctrl Pts',(-12.0779278978753,-13.9336031304968,
118.79611561457)) ;
#189254=CARTESIAN_POINT('Ctrl Pts',(-12.0041240543692,-13.9336031304964,
118.820346655993)) ;
#189255=CARTESIAN_POINT('Ctrl Pts',(-12.0244240599819,-13.9726608385011,
118.882177197693)) ;
#189256=CARTESIAN_POINT('Ctrl Pts',(-12.0447240655947,-14.0117185465058,
118.944007739393)) ;
#189257=CARTESIAN_POINT('Ctrl Pts',(-12.1185279091008,-14.0117185465062,
118.919776697969)) ;
#189258=CARTESIAN_POINT('Ctrl Pts',(-12.192331752607,-14.0117185465065,
118.895545656546)) ;
#189259=CARTESIAN_POINT('Ctrl Pts',(-12.1720317469942,-13.9726608385018,
118.833715114846)) ;
#189260=CARTESIAN_POINT('Ctrl Pts',(-12.1969356507805,-13.7058102020006,
118.944880479442)) ;
#189261=CARTESIAN_POINT('Ctrl Pts',(-12.1741357371113,-13.6853276622156,
118.875435621207)) ;
#189262=CARTESIAN_POINT('Ctrl Pts',(-12.1003318934442,-13.685327664635,
118.899666662141)) ;
#189263=CARTESIAN_POINT('Ctrl Pts',(-12.0265280497771,-13.6853276670543,
118.923897703074)) ;
#189264=CARTESIAN_POINT('Ctrl Pts',(-12.0493279634463,-13.7058102068394,
118.993342561308)) ;
#189265=CARTESIAN_POINT('Ctrl Pts',(-12.0721278771155,-13.7262927466244,
119.062787419543)) ;
#189266=CARTESIAN_POINT('Ctrl Pts',(-12.1459317207826,-13.726292744205,
119.03855637861)) ;
#189267=CARTESIAN_POINT('Ctrl Pts',(-12.2197355644497,-13.7262927417856,
119.014325337677)) ;
#189268=CARTESIAN_POINT('Ctrl Pts',(-12.1969356507805,-13.7058102020006,
118.944880479442)) ;
#189269=CARTESIAN_POINT('Ctrl Pts',(-12.1984748836622,-13.4160016672544,
118.985181508571)) ;
#189270=CARTESIAN_POINT('Ctrl Pts',(-12.1747964593274,-13.4157263085417,
118.913060848612)) ;
#189271=CARTESIAN_POINT('Ctrl Pts',(-12.100992615932,-13.4157263119192,
118.937291890373)) ;
#189272=CARTESIAN_POINT('Ctrl Pts',(-12.0271887725366,-13.4157263152968,
118.961522932133)) ;
#189273=CARTESIAN_POINT('Ctrl Pts',(-12.0508671968713,-13.4160016740095,
119.033643592092)) ;
#189274=CARTESIAN_POINT('Ctrl Pts',(-12.074545621206,-13.4162770327222,
119.105764252051)) ;
#189275=CARTESIAN_POINT('Ctrl Pts',(-12.1483494646015,-13.4162770293446,
119.08153321029)) ;
#189276=CARTESIAN_POINT('Ctrl Pts',(-12.2221533079969,-13.4162770259671,
119.057302168529)) ;
#189277=CARTESIAN_POINT('Ctrl Pts',(-12.1984748836622,-13.4160016672544,
118.985181508571)) ;
#189278=CARTESIAN_POINT('Ctrl Pts',(-12.1757274731677,-13.1285751860039,
118.9512289621)) ;
#189279=CARTESIAN_POINT('Ctrl Pts',(-12.1528714753158,-13.1483696405658,
118.881613280481)) ;
#189280=CARTESIAN_POINT('Ctrl Pts',(-12.0790676321189,-13.1483696423267,
118.905844322846)) ;
#189281=CARTESIAN_POINT('Ctrl Pts',(-12.0052637889219,-13.1483696440876,
118.930075365211)) ;
#189282=CARTESIAN_POINT('Ctrl Pts',(-12.0281197867738,-13.1285751895257,
118.99969104683)) ;
#189283=CARTESIAN_POINT('Ctrl Pts',(-12.0509757846257,-13.1087807349637,
119.06930672845)) ;
#189284=CARTESIAN_POINT('Ctrl Pts',(-12.1247796278227,-13.1087807332029,
119.045075686085)) ;
#189285=CARTESIAN_POINT('Ctrl Pts',(-12.1985834710196,-13.108780731442,
119.020844643719)) ;
#189286=CARTESIAN_POINT('Ctrl Pts',(-12.1757274731677,-13.1285751860039,
118.9512289621)) ;
#189287=CARTESIAN_POINT('Ctrl Pts',(-12.1296371270561,-12.8607655160009,
118.846298221329)) ;
#189288=CARTESIAN_POINT('Ctrl Pts',(-12.1092322366569,-12.8992892822013,
118.784148217467)) ;
#189289=CARTESIAN_POINT('Ctrl Pts',(-12.0354283931757,-12.8992892809573,
118.808379258966)) ;
#189290=CARTESIAN_POINT('Ctrl Pts',(-11.9616245496946,-12.8992892797133,
118.832610300466)) ;
#189291=CARTESIAN_POINT('Ctrl Pts',(-11.9820294400938,-12.8607655135129,
118.894760304328)) ;
#189292=CARTESIAN_POINT('Ctrl Pts',(-12.0024343304931,-12.8222417473126,
118.95691030819)) ;
#189293=CARTESIAN_POINT('Ctrl Pts',(-12.0762381739742,-12.8222417485565,
118.932679266691)) ;
#189294=CARTESIAN_POINT('Ctrl Pts',(-12.1500420174553,-12.8222417498005,
118.908448225191)) ;
#189295=CARTESIAN_POINT('Ctrl Pts',(-12.1296371270561,-12.8607655160009,
118.846298221329)) ;
#189296=CARTESIAN_POINT('Ctrl Pts',(-12.0621098926496,-12.6316532711116,
118.676300392897)) ;
#189297=CARTESIAN_POINT('Ctrl Pts',(-12.0456518862887,-12.686231857174,
118.626171960866)) ;
#189298=CARTESIAN_POINT('Ctrl Pts',(-11.9718480413066,-12.6862318515475,
118.650402997794)) ;
#189299=CARTESIAN_POINT('Ctrl Pts',(-11.8980441963246,-12.6862318459211,
118.674634034722)) ;
#189300=CARTESIAN_POINT('Ctrl Pts',(-11.9145022026855,-12.6316532598588,
118.724762466754)) ;
#189301=CARTESIAN_POINT('Ctrl Pts',(-11.9309602090465,-12.5770746737964,
118.774890898785)) ;
#189302=CARTESIAN_POINT('Ctrl Pts',(-12.0047640540285,-12.5770746794228,
118.750659861857)) ;
#189303=CARTESIAN_POINT('Ctrl Pts',(-12.0785678990105,-12.5770746850493,
118.726428824929)) ;
#189304=CARTESIAN_POINT('Ctrl Pts',(-12.0621098926496,-12.6316532711116,
118.676300392897)) ;
#189305=CARTESIAN_POINT('Ctrl Pts',(-11.978269028545,-12.460718041819,118.456338381467)) ;
#189306=CARTESIAN_POINT('Ctrl Pts',(-11.9669085684669,-12.5273111609863,
118.42173625281)) ;
#189307=CARTESIAN_POINT('Ctrl Pts',(-11.8931047213999,-12.5273111540266,
118.445967283387)) ;
#189308=CARTESIAN_POINT('Ctrl Pts',(-11.8193008743329,-12.5273111470668,
118.470198313965)) ;
#189309=CARTESIAN_POINT('Ctrl Pts',(-11.830661334411,-12.4607180278995,
118.504800442623)) ;
#189310=CARTESIAN_POINT('Ctrl Pts',(-11.8420217944891,-12.3941249087322,
118.53940257128)) ;
#189311=CARTESIAN_POINT('Ctrl Pts',(-11.915825641556,-12.394124915692,118.515171540702)) ;
#189312=CARTESIAN_POINT('Ctrl Pts',(-11.989629488623,-12.3941249226517,
118.490940510125)) ;
#189313=CARTESIAN_POINT('Ctrl Pts',(-11.978269028545,-12.460718041819,118.456338381467)) ;
#189314=CARTESIAN_POINT('Ctrl Pts',(-11.8829561531315,-12.3580087732105,
118.201435967149)) ;
#189315=CARTESIAN_POINT('Ctrl Pts',(-11.8775015614734,-12.4318697519678,
118.184822160659)) ;
#189316=CARTESIAN_POINT('Ctrl Pts',(-11.8036977119076,-12.4318697467782,
118.209053183626)) ;
#189317=CARTESIAN_POINT('Ctrl Pts',(-11.7298938623419,-12.4318697415885,
118.233284206593)) ;
#189318=CARTESIAN_POINT('Ctrl Pts',(-11.735348454,-12.3580087628311,118.249898013083)) ;
#189319=CARTESIAN_POINT('Ctrl Pts',(-11.7408030456581,-12.2841477840738,
118.266511819573)) ;
#189320=CARTESIAN_POINT('Ctrl Pts',(-11.8146068952239,-12.2841477892635,
118.242280796606)) ;
#189321=CARTESIAN_POINT('Ctrl Pts',(-11.8884107447897,-12.2841477944531,
118.218049773639)) ;
#189322=CARTESIAN_POINT('Ctrl Pts',(-11.8829561531315,-12.3580087732105,
118.201435967149)) ;
#189323=CARTESIAN_POINT('Ctrl Pts',(-11.7821952753084,-12.3309308762199,
117.929933042971)) ;
#189324=CARTESIAN_POINT('Ctrl Pts',(-11.7830355643032,-12.4067892276866,
117.932492427132)) ;
#189325=CARTESIAN_POINT('Ctrl Pts',(-11.7092317122289,-12.4067892280987,
117.956723442458)) ;
#189326=CARTESIAN_POINT('Ctrl Pts',(-11.6354278601546,-12.4067892285108,
117.980954457785)) ;
#189327=CARTESIAN_POINT('Ctrl Pts',(-11.6345875711599,-12.330930877044,
117.978395073623)) ;
#189328=CARTESIAN_POINT('Ctrl Pts',(-11.6337472821651,-12.2550725255773,
117.975835689462)) ;
#189329=CARTESIAN_POINT('Ctrl Pts',(-11.7075511342394,-12.2550725251652,
117.951604674136)) ;
#189330=CARTESIAN_POINT('Ctrl Pts',(-11.7813549863137,-12.2550725247531,
117.92737365881)) ;
#189331=CARTESIAN_POINT('Ctrl Pts',(-11.7821952753084,-12.3309308762199,
117.929933042971)) ;
#189332=CARTESIAN_POINT('Ctrl Pts',(-11.6820920733114,-12.3817530522947,
117.660553623845)) ;
#189333=CARTESIAN_POINT('Ctrl Pts',(-11.6891878850714,-12.4541728296822,
117.682166320851)) ;
#189334=CARTESIAN_POINT('Ctrl Pts',(-11.6153840306775,-12.454172840125,
117.706397329112)) ;
#189335=CARTESIAN_POINT('Ctrl Pts',(-11.5415801762836,-12.4541728505679,
117.730628337373)) ;
#189336=CARTESIAN_POINT('Ctrl Pts',(-11.5344843645237,-12.3817530731804,
117.709015640367)) ;
#189337=CARTESIAN_POINT('Ctrl Pts',(-11.5273885527638,-12.3093332957928,
117.687402943361)) ;
#189338=CARTESIAN_POINT('Ctrl Pts',(-11.6011924071576,-12.30933328535,117.6631719351)) ;
#189339=CARTESIAN_POINT('Ctrl Pts',(-11.6749962615515,-12.3093332749072,
117.638940926839)) ;
#189340=CARTESIAN_POINT('Ctrl Pts',(-11.6820920733114,-12.3817530522947,
117.660553623845)) ;
#189341=CARTESIAN_POINT('Ctrl Pts',(-11.5895815929449,-12.506826084586,
117.414237666503)) ;
#189342=CARTESIAN_POINT('Ctrl Pts',(-11.6024130459701,-12.5706179101752,
117.453320201195)) ;
#189343=CARTESIAN_POINT('Ctrl Pts',(-11.5286091905944,-12.5706179343356,
117.477551206465)) ;
#189344=CARTESIAN_POINT('Ctrl Pts',(-11.4548053352187,-12.5706179584961,
117.501782211736)) ;
#189345=CARTESIAN_POINT('Ctrl Pts',(-11.4419738821936,-12.5068261329069,
117.462699677045)) ;
#189346=CARTESIAN_POINT('Ctrl Pts',(-11.4291424291684,-12.4430343073178,
117.423617142354)) ;
#189347=CARTESIAN_POINT('Ctrl Pts',(-11.5029462845441,-12.4430342831573,
117.399386137083)) ;
#189348=CARTESIAN_POINT('Ctrl Pts',(-11.5767501399198,-12.4430342589969,
117.375155131812)) ;
#189349=CARTESIAN_POINT('Ctrl Pts',(-11.5895815929449,-12.506826084586,
117.414237666503)) ;
#189350=CARTESIAN_POINT('Ctrl Pts',(-11.5103184193888,-12.6970626230436,
117.208275910696)) ;
#189351=CARTESIAN_POINT('Ctrl Pts',(-11.5279687114292,-12.7476645000542,
117.262035851343)) ;
#189352=CARTESIAN_POINT('Ctrl Pts',(-11.4541648566701,-12.7476645399719,
117.286266858491)) ;
#189353=CARTESIAN_POINT('Ctrl Pts',(-11.380361001911,-12.7476645798895,
117.31049786564)) ;
#189354=CARTESIAN_POINT('Ctrl Pts',(-11.3627107098707,-12.6970627028788,
117.256737924993)) ;
#189355=CARTESIAN_POINT('Ctrl Pts',(-11.3450604178303,-12.6464608258682,
117.202977984346)) ;
#189356=CARTESIAN_POINT('Ctrl Pts',(-11.4188642725894,-12.6464607859506,
117.178746977197)) ;
#189357=CARTESIAN_POINT('Ctrl Pts',(-11.4926681273484,-12.646460746033,
117.154515970049)) ;
#189358=CARTESIAN_POINT('Ctrl Pts',(-11.5103184193888,-12.6970626230436,
117.208275910696)) ;
#189359=CARTESIAN_POINT('Ctrl Pts',(-11.4490956702002,-12.9398196291384,
117.057375370954)) ;
#189360=CARTESIAN_POINT('Ctrl Pts',(-11.4703099251282,-12.9735460220805,
117.121990567328)) ;
#189361=CARTESIAN_POINT('Ctrl Pts',(-11.3965060727708,-12.9735460788729,
117.146221581792)) ;
#189362=CARTESIAN_POINT('Ctrl Pts',(-11.3227022204133,-12.9735461356652,
117.170452596256)) ;
#189363=CARTESIAN_POINT('Ctrl Pts',(-11.3014879654853,-12.9398197427232,
117.105837399882)) ;
#189364=CARTESIAN_POINT('Ctrl Pts',(-11.2802737105573,-12.9060933497811,
117.041222203508)) ;
#189365=CARTESIAN_POINT('Ctrl Pts',(-11.3540775629148,-12.9060932929888,
117.016991189044)) ;
#189366=CARTESIAN_POINT('Ctrl Pts',(-11.4278814152722,-12.9060932361964,
116.99276017458)) ;
#189367=CARTESIAN_POINT('Ctrl Pts',(-11.4490956702002,-12.9398196291384,
117.057375370954)) ;
#189368=CARTESIAN_POINT('Ctrl Pts',(-11.4099894577055,-13.2163226304817,
116.973745461531)) ;
#189369=CARTESIAN_POINT('Ctrl Pts',(-11.4332305688274,-13.2307930159817,
117.04453413468)) ;
#189370=CARTESIAN_POINT('Ctrl Pts',(-11.3594267210954,-13.2307930864604,
117.068765163233)) ;
#189371=CARTESIAN_POINT('Ctrl Pts',(-11.2856228733634,-13.2307931569392,
117.092996191785)) ;
#189372=CARTESIAN_POINT('Ctrl Pts',(-11.2623817622415,-13.2163227714392,
117.022207518635)) ;
#189373=CARTESIAN_POINT('Ctrl Pts',(-11.2391406511197,-13.2018523859393,
116.951418845486)) ;
#189374=CARTESIAN_POINT('Ctrl Pts',(-11.3129444988516,-13.2018523154605,
116.927187816934)) ;
#189375=CARTESIAN_POINT('Ctrl Pts',(-11.3867483465836,-13.2018522449817,
116.902956788382)) ;
#189376=CARTESIAN_POINT('Ctrl Pts',(-11.4099894577055,-13.2163226304817,
116.973745461531)) ;
#189377=CARTESIAN_POINT('Ctrl Pts',(-11.3947104282053,-13.5056990228868,
116.962500660225)) ;
#189378=CARTESIAN_POINT('Ctrl Pts',(-11.4183215240288,-13.4999868027269,
117.034416246959)) ;
#189379=CARTESIAN_POINT('Ctrl Pts',(-11.344517682384,-13.4999868805839,
117.058647294052)) ;
#189380=CARTESIAN_POINT('Ctrl Pts',(-11.2707138407393,-13.499986958441,
117.082878341144)) ;
#189381=CARTESIAN_POINT('Ctrl Pts',(-11.2471027449158,-13.5056991786008,
117.010962754411)) ;
#189382=CARTESIAN_POINT('Ctrl Pts',(-11.2234916490923,-13.5114113987607,
116.939047167677)) ;
#189383=CARTESIAN_POINT('Ctrl Pts',(-11.2972954907371,-13.5114113209037,
116.914816120584)) ;
#189384=CARTESIAN_POINT('Ctrl Pts',(-11.3710993323818,-13.5114112430466,
116.890585073491)) ;
#189385=CARTESIAN_POINT('Ctrl Pts',(-11.3947104282053,-13.5056990228868,
116.962500660225)) ;
#189386=CARTESIAN_POINT('Ctrl Pts',(-11.4036668088478,-13.7916926696265,
117.025439420547)) ;
#189387=CARTESIAN_POINT('Ctrl Pts',(-11.4259492352715,-13.7660050582146,
117.093308094503)) ;
#189388=CARTESIAN_POINT('Ctrl Pts',(-11.3521454009588,-13.7660051397553,
117.117539163929)) ;
#189389=CARTESIAN_POINT('Ctrl Pts',(-11.2783415666462,-13.766005221296,
117.141770233354)) ;
#189390=CARTESIAN_POINT('Ctrl Pts',(-11.2560591402225,-13.791692832708,
117.073901559397)) ;
#189391=CARTESIAN_POINT('Ctrl Pts',(-11.2337767137989,-13.81738044412,117.006032885441)) ;
#189392=CARTESIAN_POINT('Ctrl Pts',(-11.3075805481115,-13.8173803625793,
116.981801816016)) ;
#189393=CARTESIAN_POINT('Ctrl Pts',(-11.3813843824241,-13.8173802810385,
116.95757074659)) ;
#189394=CARTESIAN_POINT('Ctrl Pts',(-11.4036668088478,-13.7916926696265,
117.025439420547)) ;
#189395=CARTESIAN_POINT('Ctrl Pts',(-11.4354180827992,-14.0485418604028,
117.157509418095)) ;
#189396=CARTESIAN_POINT('Ctrl Pts',(-11.4547844005631,-14.0048845368929,
117.216496095483)) ;
#189397=CARTESIAN_POINT('Ctrl Pts',(-11.3809805736863,-14.0048846120398,
117.240727187556)) ;
#189398=CARTESIAN_POINT('Ctrl Pts',(-11.3071767468095,-14.0048846871867,
117.26495827963)) ;
#189399=CARTESIAN_POINT('Ctrl Pts',(-11.2878104290456,-14.0485420106967,
117.205971602242)) ;
#189400=CARTESIAN_POINT('Ctrl Pts',(-11.2684441112818,-14.0921993342066,
117.146984924854)) ;
#189401=CARTESIAN_POINT('Ctrl Pts',(-11.3422479381586,-14.0921992590597,
117.122753832781)) ;
#189402=CARTESIAN_POINT('Ctrl Pts',(-11.4160517650354,-14.0921991839128,
117.098522740707)) ;
#189403=CARTESIAN_POINT('Ctrl Pts',(-11.4354180827992,-14.0485418604028,
117.157509418095)) ;
#189404=CARTESIAN_POINT('Ctrl Pts',(-11.4868177885781,-14.2607963084926,
117.349453433615)) ;
#189405=CARTESIAN_POINT('Ctrl Pts',(-11.5018915030736,-14.2022566312554,
117.39536553396)) ;
#189406=CARTESIAN_POINT('Ctrl Pts',(-11.4280876830046,-14.2022566928803,
117.419596646769)) ;
#189407=CARTESIAN_POINT('Ctrl Pts',(-11.3542838629355,-14.2022567545052,
117.443827759578)) ;
#189408=CARTESIAN_POINT('Ctrl Pts',(-11.33921014844,-14.2607964317425,117.397915659233)) ;
#189409=CARTESIAN_POINT('Ctrl Pts',(-11.3241364339445,-14.3193361089797,
117.352003558888)) ;
#189410=CARTESIAN_POINT('Ctrl Pts',(-11.3979402540135,-14.3193360473548,
117.327772446079)) ;
#189411=CARTESIAN_POINT('Ctrl Pts',(-11.4717440740825,-14.3193359857299,
117.30354133327)) ;
#189412=CARTESIAN_POINT('Ctrl Pts',(-11.4868177885781,-14.2607963084926,
117.349453433615)) ;
#189413=CARTESIAN_POINT('Ctrl Pts',(-11.5538956508532,-14.4133855037132,
117.589310677699)) ;
#189414=CARTESIAN_POINT('Ctrl Pts',(-11.563572812887,-14.3441068413642,
117.618785749883)) ;
#189415=CARTESIAN_POINT('Ctrl Pts',(-11.489768998477,-14.3441068827324,
117.643016879929)) ;
#189416=CARTESIAN_POINT('Ctrl Pts',(-11.415965184067,-14.3441069241007,
117.667248009974)) ;
#189417=CARTESIAN_POINT('Ctrl Pts',(-11.4062880220333,-14.4133855864497,
117.63777293779)) ;
#189418=CARTESIAN_POINT('Ctrl Pts',(-11.3966108599995,-14.4826642487988,
117.608297865606)) ;
#189419=CARTESIAN_POINT('Ctrl Pts',(-11.4704146744095,-14.4826642074306,
117.584066735561)) ;
#189420=CARTESIAN_POINT('Ctrl Pts',(-11.5442184888195,-14.4826641660623,
117.559835605515)) ;
#189421=CARTESIAN_POINT('Ctrl Pts',(-11.5538956508532,-14.4133855037132,
117.589310677699)) ;
#189422=CARTESIAN_POINT('Ctrl Pts',(-11.6305563612239,-14.4941554742073,
117.858230229529)) ;
#189423=CARTESIAN_POINT('Ctrl Pts',(-11.6341625811807,-14.4191362246067,
117.869214191629)) ;
#189424=CARTESIAN_POINT('Ctrl Pts',(-11.5603587701322,-14.4191362402107,
117.893445331912)) ;
#189425=CARTESIAN_POINT('Ctrl Pts',(-11.4865549590836,-14.4191362558146,
117.917676472196)) ;
#189426=CARTESIAN_POINT('Ctrl Pts',(-11.4829487391268,-14.4941555054153,
117.906692510097)) ;
#189427=CARTESIAN_POINT('Ctrl Pts',(-11.4793425191701,-14.5691747550159,
117.895708547997)) ;
#189428=CARTESIAN_POINT('Ctrl Pts',(-11.5531463302186,-14.5691747394119,
117.871477407714)) ;
#189429=CARTESIAN_POINT('Ctrl Pts',(-11.6269501412672,-14.5691747238079,
117.84724626743)) ;
#189430=CARTESIAN_POINT('Ctrl Pts',(-11.6305563612239,-14.4941554742073,
117.858230229529)) ;
#189431=CARTESIAN_POINT('Ctrl Pts',(-11.7109172218611,-14.4980202636657,
118.138483857812)) ;
#189432=CARTESIAN_POINT('Ctrl Pts',(-11.7081839997789,-14.4226207212898,
118.130158902281)) ;
#189433=CARTESIAN_POINT('Ctrl Pts',(-11.6343801895775,-14.4226207084362,
118.154390045145)) ;
#189434=CARTESIAN_POINT('Ctrl Pts',(-11.5605763793761,-14.4226206955826,
118.178621188009)) ;
#189435=CARTESIAN_POINT('Ctrl Pts',(-11.5633096014583,-14.4980202379585,
118.186946143541)) ;
#189436=CARTESIAN_POINT('Ctrl Pts',(-11.5660428235405,-14.5734197803344,
118.195271099072)) ;
#189437=CARTESIAN_POINT('Ctrl Pts',(-11.6398466337419,-14.573419793188,
118.171039956207)) ;
#189438=CARTESIAN_POINT('Ctrl Pts',(-11.7136504439433,-14.5734198060416,
118.146808813343)) ;
#189439=CARTESIAN_POINT('Ctrl Pts',(-11.7109172218611,-14.4980202636657,
118.138483857812)) ;
#189440=CARTESIAN_POINT('Ctrl Pts',(-11.7882117517516,-14.4245044594768,
118.409341495335)) ;
#189441=CARTESIAN_POINT('Ctrl Pts',(-11.7793449549404,-14.3541263042152,
118.382334660807)) ;
#189442=CARTESIAN_POINT('Ctrl Pts',(-11.7055411427768,-14.3541262631264,
118.406565797695)) ;
#189443=CARTESIAN_POINT('Ctrl Pts',(-11.6317373306133,-14.3541262220375,
118.430796934583)) ;
#189444=CARTESIAN_POINT('Ctrl Pts',(-11.6406041274246,-14.4245043772991,
118.45780376911)) ;
#189445=CARTESIAN_POINT('Ctrl Pts',(-11.6494709242359,-14.4948825325607,
118.484810603637)) ;
#189446=CARTESIAN_POINT('Ctrl Pts',(-11.7232747363994,-14.4948825736496,
118.46057946675)) ;
#189447=CARTESIAN_POINT('Ctrl Pts',(-11.797078548563,-14.4948826147384,
118.436348329862)) ;
#189448=CARTESIAN_POINT('Ctrl Pts',(-11.7882117517516,-14.4245044594768,
118.409341495335)) ;
#189449=CARTESIAN_POINT('Ctrl Pts',(-11.8562827938217,-14.279297376843,
118.65208243579)) ;
#189450=CARTESIAN_POINT('Ctrl Pts',(-11.8419177852559,-14.2189530105724,
118.608328935389)) ;
#189451=CARTESIAN_POINT('Ctrl Pts',(-11.7681139685888,-14.2189529442762,
118.63256005856)) ;
#189452=CARTESIAN_POINT('Ctrl Pts',(-11.6943101519217,-14.2189528779799,
118.65679118173)) ;
#189453=CARTESIAN_POINT('Ctrl Pts',(-11.7086751604876,-14.2792972442505,
118.700544682131)) ;
#189454=CARTESIAN_POINT('Ctrl Pts',(-11.7230401690534,-14.3396416105211,
118.744298182531)) ;
#189455=CARTESIAN_POINT('Ctrl Pts',(-11.7968439857205,-14.3396416768173,
118.720067059361)) ;
#189456=CARTESIAN_POINT('Ctrl Pts',(-11.8706478023876,-14.3396417431136,
118.69583593619)) ;
#189457=CARTESIAN_POINT('Ctrl Pts',(-11.8562827938217,-14.279297376843,
118.65208243579)) ;
#189458=CARTESIAN_POINT('Ctrl Pts',(-11.9097428090595,-14.0713598205673,
118.85049429419)) ;
#189459=CARTESIAN_POINT('Ctrl Pts',(-11.8908877918867,-14.0254428843111,
118.793064952058)) ;
#189460=CARTESIAN_POINT('Ctrl Pts',(-11.8170839684841,-14.0254427985769,
118.817296054714)) ;
#189461=CARTESIAN_POINT('Ctrl Pts',(-11.7432801450815,-14.0254427128428,
118.841527157369)) ;
#189462=CARTESIAN_POINT('Ctrl Pts',(-11.7621351622542,-14.0713596490991,
118.898956499501)) ;
#189463=CARTESIAN_POINT('Ctrl Pts',(-11.780990179427,-14.1172765853553,
118.956385841632)) ;
#189464=CARTESIAN_POINT('Ctrl Pts',(-11.8547940028297,-14.1172766710895,
118.932154738977)) ;
#189465=CARTESIAN_POINT('Ctrl Pts',(-11.9285978262323,-14.1172767568236,
118.907923636322)) ;
#189466=CARTESIAN_POINT('Ctrl Pts',(-11.9097428090595,-14.0713598205673,
118.85049429419)) ;
#189467=CARTESIAN_POINT('Ctrl Pts',(-11.9435103312939,-13.8176789860274,
118.988744092681)) ;
#189468=CARTESIAN_POINT('Ctrl Pts',(-11.9215372338277,-13.7894049725344,
118.921817581118)) ;
#189469=CARTESIAN_POINT('Ctrl Pts',(-11.8477334023547,-13.7894048748747,
118.946048659193)) ;
#189470=CARTESIAN_POINT('Ctrl Pts',(-11.7739295708818,-13.789404777215,
118.970279737267)) ;
#189471=CARTESIAN_POINT('Ctrl Pts',(-11.795902668348,-13.8176787907079,
119.03720624883)) ;
#189472=CARTESIAN_POINT('Ctrl Pts',(-11.8178757658143,-13.8459528042009,
119.104132760393)) ;
#189473=CARTESIAN_POINT('Ctrl Pts',(-11.8916795972872,-13.8459529018606,
119.079901682319)) ;
#189474=CARTESIAN_POINT('Ctrl Pts',(-11.9654834287601,-13.8459529995203,
119.055670604245)) ;
#189475=CARTESIAN_POINT('Ctrl Pts',(-11.9435103312939,-13.8176789860274,
118.988744092681)) ;
#189476=CARTESIAN_POINT('Ctrl Pts',(-11.9547796677016,-13.5347545509982,
119.058563970788)) ;
#189477=CARTESIAN_POINT('Ctrl Pts',(-11.931252448714,-13.526191139526,118.986903855894)) ;
#189478=CARTESIAN_POINT('Ctrl Pts',(-11.8574486085768,-13.5261910386332,
119.011134907579)) ;
#189479=CARTESIAN_POINT('Ctrl Pts',(-11.7836447684397,-13.5261909377405,
119.035365959264)) ;
#189480=CARTESIAN_POINT('Ctrl Pts',(-11.8071719874273,-13.5347543492127,
119.107026074158)) ;
#189481=CARTESIAN_POINT('Ctrl Pts',(-11.8306992064149,-13.5433177606849,
119.178686189051)) ;
#189482=CARTESIAN_POINT('Ctrl Pts',(-11.9045030465521,-13.5433178615776,
119.154455137367)) ;
#189483=CARTESIAN_POINT('Ctrl Pts',(-11.9783068866892,-13.5433179624704,
119.130224085682)) ;
#189484=CARTESIAN_POINT('Ctrl Pts',(-11.9547796677016,-13.5347545509982,
119.058563970788)) ;
#189485=CARTESIAN_POINT('Ctrl Pts',(-11.9418285130168,-13.2436560304018,
119.054582905373)) ;
#189486=CARTESIAN_POINT('Ctrl Pts',(-11.9184363705024,-13.2554035564965,
118.983334211708)) ;
#189487=CARTESIAN_POINT('Ctrl Pts',(-11.8446325221026,-13.2554034608617,
119.007565238226)) ;
#189488=CARTESIAN_POINT('Ctrl Pts',(-11.7708286737027,-13.2554033652269,
119.031796264744)) ;
#189489=CARTESIAN_POINT('Ctrl Pts',(-11.7942208162171,-13.2436558391322,
119.103044958408)) ;
#189490=CARTESIAN_POINT('Ctrl Pts',(-11.8176129587315,-13.2319083130375,
119.174293652073)) ;
#189491=CARTESIAN_POINT('Ctrl Pts',(-11.8914168071314,-13.2319084086723,
119.150062625555)) ;
#189492=CARTESIAN_POINT('Ctrl Pts',(-11.9652206555312,-13.2319085043071,
119.125831599037)) ;
#189493=CARTESIAN_POINT('Ctrl Pts',(-11.9418285130168,-13.2436560304018,
119.054582905373)) ;
#189494=CARTESIAN_POINT('Ctrl Pts',(-11.9049261358387,-12.9652204672347,
118.977628691884)) ;
#189495=CARTESIAN_POINT('Ctrl Pts',(-11.8833418779651,-12.9964254468849,
118.911886523235)) ;
#189496=CARTESIAN_POINT('Ctrl Pts',(-11.8095380224967,-12.9964253637305,
118.936117528223)) ;
#189497=CARTESIAN_POINT('Ctrl Pts',(-11.7357341670283,-12.996425280576,
118.960348533212)) ;
#189498=CARTESIAN_POINT('Ctrl Pts',(-11.7573184249019,-12.9652203009257,
119.02609070186)) ;
#189499=CARTESIAN_POINT('Ctrl Pts',(-11.7789026827756,-12.9340153212755,
119.091832870508)) ;
#189500=CARTESIAN_POINT('Ctrl Pts',(-11.852706538244,-12.93401540443,119.06760186552)) ;
#189501=CARTESIAN_POINT('Ctrl Pts',(-11.9265103937124,-12.9340154875845,
119.043370860532)) ;
#189502=CARTESIAN_POINT('Ctrl Pts',(-11.9049261358387,-12.9652204672347,
118.977628691884)) ;
#189503=CARTESIAN_POINT('Ctrl Pts',(-11.8458933110122,-12.7189935301929,
118.833296067848)) ;
#189504=CARTESIAN_POINT('Ctrl Pts',(-11.827664106781,-12.7674367069974,
118.777772851381)) ;
#189505=CARTESIAN_POINT('Ctrl Pts',(-11.7538602461059,-12.7674366419676,
118.80200384051)) ;
#189506=CARTESIAN_POINT('Ctrl Pts',(-11.6800563854307,-12.7674365769377,
118.826234829639)) ;
#189507=CARTESIAN_POINT('Ctrl Pts',(-11.698285589662,-12.7189934001331,
118.881758046107)) ;
#189508=CARTESIAN_POINT('Ctrl Pts',(-11.7165147938932,-12.6705502233285,
118.937281262574)) ;
#189509=CARTESIAN_POINT('Ctrl Pts',(-11.7903186545683,-12.6705502883584,
118.913050273445)) ;
#189510=CARTESIAN_POINT('Ctrl Pts',(-11.8641225152435,-12.6705503533883,
118.888819284315)) ;
#189511=CARTESIAN_POINT('Ctrl Pts',(-11.8458933110122,-12.7189935301929,
118.833296067848)) ;
#189512=CARTESIAN_POINT('Ctrl Pts',(-11.768187928547,-12.5228013953796,
118.632102371038)) ;
#189513=CARTESIAN_POINT('Ctrl Pts',(-11.7546222310584,-12.585015703863,
118.590783443794)) ;
#189514=CARTESIAN_POINT('Ctrl Pts',(-11.6808183674585,-12.5850156600089,
118.615014424014)) ;
#189515=CARTESIAN_POINT('Ctrl Pts',(-11.6070145038585,-12.5850156161548,
118.639245404235)) ;
#189516=CARTESIAN_POINT('Ctrl Pts',(-11.6205802013471,-12.5228013076713,
118.680564331479)) ;
#189517=CARTESIAN_POINT('Ctrl Pts',(-11.6341458988357,-12.4605869991879,
118.721883258723)) ;
#189518=CARTESIAN_POINT('Ctrl Pts',(-11.7079497624357,-12.460587043042,
118.697652278502)) ;
#189519=CARTESIAN_POINT('Ctrl Pts',(-11.7817536260356,-12.4605870868961,
118.673421298282)) ;
#189520=CARTESIAN_POINT('Ctrl Pts',(-11.768187928547,-12.5228013953796,
118.632102371038)) ;
#189521=CARTESIAN_POINT('Ctrl Pts',(-11.6766862938013,-12.3908781186536,
118.388873969626)) ;
#189522=CARTESIAN_POINT('Ctrl Pts',(-11.6687546982478,-12.462397411453,
118.364715607968)) ;
#189523=CARTESIAN_POINT('Ctrl Pts',(-11.5949508340276,-12.4623973889088,
118.388946586299)) ;
#189524=CARTESIAN_POINT('Ctrl Pts',(-11.5211469698073,-12.4623973663647,
118.413177564631)) ;
#189525=CARTESIAN_POINT('Ctrl Pts',(-11.5290785653608,-12.3908780735653,
118.437335926289)) ;
#189526=CARTESIAN_POINT('Ctrl Pts',(-11.5370101609142,-12.3193587807659,
118.461494287948)) ;
#189527=CARTESIAN_POINT('Ctrl Pts',(-11.6108140251345,-12.3193588033101,
118.437263309616)) ;
#189528=CARTESIAN_POINT('Ctrl Pts',(-11.6846178893547,-12.3193588258542,
118.413032331285)) ;
#189529=CARTESIAN_POINT('Ctrl Pts',(-11.6766862938013,-12.3908781186536,
118.388873969626)) ;
#189530=CARTESIAN_POINT('Ctrl Pts',(-11.5772683011683,-12.3325103501403,
118.121499206796)) ;
#189531=CARTESIAN_POINT('Ctrl Pts',(-11.5755328069561,-12.4082131688575,
118.116213170239)) ;
#189532=CARTESIAN_POINT('Ctrl Pts',(-11.5017289440862,-12.4082131654103,
118.140444152683)) ;
#189533=CARTESIAN_POINT('Ctrl Pts',(-11.4279250812163,-12.4082131619632,
118.164675135128)) ;
#189534=CARTESIAN_POINT('Ctrl Pts',(-11.4296605754286,-12.332510343246,
118.169961171685)) ;
#189535=CARTESIAN_POINT('Ctrl Pts',(-11.4313960696408,-12.2568075245288,
118.175247208242)) ;
#189536=CARTESIAN_POINT('Ctrl Pts',(-11.5051999325107,-12.2568075279759,
118.151016225798)) ;
#189537=CARTESIAN_POINT('Ctrl Pts',(-11.5790037953806,-12.2568075314231,
118.126785243353)) ;
#189538=CARTESIAN_POINT('Ctrl Pts',(-11.5772683011683,-12.3325103501403,
118.121499206796)) ;
#189539=CARTESIAN_POINT('Ctrl Pts',(-11.4760325891554,-12.3519340314614,
117.848650931793)) ;
#189540=CARTESIAN_POINT('Ctrl Pts',(-11.4806282527326,-12.4263955875959,
117.862648580506)) ;
#189541=CARTESIAN_POINT('Ctrl Pts',(-11.4068243929883,-12.4263955990476,
117.886879572471)) ;
#189542=CARTESIAN_POINT('Ctrl Pts',(-11.3330205332441,-12.4263956104993,
117.911110564435)) ;
#189543=CARTESIAN_POINT('Ctrl Pts',(-11.3284248696669,-12.3519340543648,
117.897112915723)) ;
#189544=CARTESIAN_POINT('Ctrl Pts',(-11.3238292060898,-12.2774724982303,
117.88311526701)) ;
#189545=CARTESIAN_POINT('Ctrl Pts',(-11.397633065834,-12.2774724867786,
117.858884275046)) ;
#189546=CARTESIAN_POINT('Ctrl Pts',(-11.4714369255783,-12.2774724753269,
117.834653283081)) ;
#189547=CARTESIAN_POINT('Ctrl Pts',(-11.4760325891554,-12.3519340314614,
117.848650931793)) ;
#189548=CARTESIAN_POINT('Ctrl Pts',(-11.3799644765095,-12.4474402254027,
117.591425257479)) ;
#189549=CARTESIAN_POINT('Ctrl Pts',(-11.3905425586945,-12.5153461039576,
117.623644388164)) ;
#189550=CARTESIAN_POINT('Ctrl Pts',(-11.31673870267,-12.5153461252544,117.647875391459)) ;
#189551=CARTESIAN_POINT('Ctrl Pts',(-11.2429348466455,-12.5153461465513,
117.672106394753)) ;
#189552=CARTESIAN_POINT('Ctrl Pts',(-11.2323567644604,-12.4474402679963,
117.639887264068)) ;
#189553=CARTESIAN_POINT('Ctrl Pts',(-11.2217786822754,-12.3795343894413,
117.607668133383)) ;
#189554=CARTESIAN_POINT('Ctrl Pts',(-11.2955825382999,-12.3795343681445,
117.583437130089)) ;
#189555=CARTESIAN_POINT('Ctrl Pts',(-11.3693863943245,-12.3795343468477,
117.559206126794)) ;
#189556=CARTESIAN_POINT('Ctrl Pts',(-11.3799644765095,-12.4474402254027,
117.591425257479)) ;
#189557=CARTESIAN_POINT('Ctrl Pts',(-11.2946200779385,-12.6124878626438,
117.366945500947)) ;
#189558=CARTESIAN_POINT('Ctrl Pts',(-11.3104392464365,-12.6689727866278,
117.415128135064)) ;
#189559=CARTESIAN_POINT('Ctrl Pts',(-11.2366353946611,-12.6689728121277,
117.4393591513)) ;
#189560=CARTESIAN_POINT('Ctrl Pts',(-11.1628315428857,-12.6689728376277,
117.463590167537)) ;
#189561=CARTESIAN_POINT('Ctrl Pts',(-11.1470123743877,-12.6124879136438,
117.41540753342)) ;
#189562=CARTESIAN_POINT('Ctrl Pts',(-11.1311932058897,-12.5560029896598,
117.367224899304)) ;
#189563=CARTESIAN_POINT('Ctrl Pts',(-11.2049970576651,-12.5560029641598,
117.342993883067)) ;
#189564=CARTESIAN_POINT('Ctrl Pts',(-11.2788009094405,-12.5560029386599,
117.318762866831)) ;
#189565=CARTESIAN_POINT('Ctrl Pts',(-11.2946200779385,-12.6124878626438,
117.366945500947)) ;
#189566=CARTESIAN_POINT('Ctrl Pts',(-11.2254931800816,-12.8359789539693,
117.191951388043)) ;
#189567=CARTESIAN_POINT('Ctrl Pts',(-11.2454273142253,-12.8769447916209,
117.252667543749)) ;
#189568=CARTESIAN_POINT('Ctrl Pts',(-11.1716234664004,-12.8769448154243,
117.276898572018)) ;
#189569=CARTESIAN_POINT('Ctrl Pts',(-11.0978196185755,-12.8769448392277,
117.301129600287)) ;
#189570=CARTESIAN_POINT('Ctrl Pts',(-11.0778854844318,-12.8359790015761,
117.240413444581)) ;
#189571=CARTESIAN_POINT('Ctrl Pts',(-11.0579513502882,-12.7950131639245,
117.179697288875)) ;
#189572=CARTESIAN_POINT('Ctrl Pts',(-11.131755198113,-12.7950131401211,
117.155466260606)) ;
#189573=CARTESIAN_POINT('Ctrl Pts',(-11.2055590459379,-12.7950131163177,
117.131235232337)) ;
#189574=CARTESIAN_POINT('Ctrl Pts',(-11.2254931800816,-12.8359789539693,
117.191951388043)) ;
#189575=CARTESIAN_POINT('Ctrl Pts',(-11.1771457608799,-13.1004046039055,
117.080125851854)) ;
#189576=CARTESIAN_POINT('Ctrl Pts',(-11.1997526258493,-13.1229691360916,
117.148982714559)) ;
#189577=CARTESIAN_POINT('Ctrl Pts',(-11.1259487808142,-13.1229691554338,
117.173213751326)) ;
#189578=CARTESIAN_POINT('Ctrl Pts',(-11.052144935779,-13.1229691747759,
117.197444788092)) ;
#189579=CARTESIAN_POINT('Ctrl Pts',(-11.0295380708096,-13.1004046425898,
117.128587925387)) ;
#189580=CARTESIAN_POINT('Ctrl Pts',(-11.0069312058402,-13.0778401104037,
117.059731062681)) ;
#189581=CARTESIAN_POINT('Ctrl Pts',(-11.0807350508753,-13.0778400910615,
117.035500025915)) ;
#189582=CARTESIAN_POINT('Ctrl Pts',(-11.1545388959105,-13.0778400717194,
117.011268989148)) ;
#189583=CARTESIAN_POINT('Ctrl Pts',(-11.1771457608799,-13.1004046039055,
117.080125851854)) ;
#189584=CARTESIAN_POINT('Ctrl Pts',(-11.1519710721537,-13.3877822848103,
117.038914256933)) ;
#189585=CARTESIAN_POINT('Ctrl Pts',(-11.1756359825419,-13.3903147860949,
117.11099375541)) ;
#189586=CARTESIAN_POINT('Ctrl Pts',(-11.1018321392159,-13.3903147988625,
117.135224797382)) ;
#189587=CARTESIAN_POINT('Ctrl Pts',(-11.0280282958898,-13.3903148116302,
117.159455839354)) ;
#189588=CARTESIAN_POINT('Ctrl Pts',(-11.0043633855016,-13.3877823103455,
117.087376340877)) ;
#189589=CARTESIAN_POINT('Ctrl Pts',(-10.9806984751134,-13.3852498090609,
117.0152968424)) ;
#189590=CARTESIAN_POINT('Ctrl Pts',(-11.0545023184394,-13.3852497962932,
116.991065800428)) ;
#189591=CARTESIAN_POINT('Ctrl Pts',(-11.1283061617654,-13.3852497835256,
116.966834758456)) ;
#189592=CARTESIAN_POINT('Ctrl Pts',(-11.1519710721537,-13.3877822848103,
117.038914256933)) ;
#189593=CARTESIAN_POINT('Ctrl Pts',(-11.1511192899988,-13.6773386169807,
117.071787370231)) ;
#189594=CARTESIAN_POINT('Ctrl Pts',(-11.1741453692937,-13.6596563698358,
117.141921092393)) ;
#189595=CARTESIAN_POINT('Ctrl Pts',(-11.1003415265199,-13.659656376027,
117.166152136048)) ;
#189596=CARTESIAN_POINT('Ctrl Pts',(-11.0265376837462,-13.6596563822181,
117.190383179702)) ;
#189597=CARTESIAN_POINT('Ctrl Pts',(-11.0035116044512,-13.6773386293631,
117.120249457539)) ;
#189598=CARTESIAN_POINT('Ctrl Pts',(-10.9804855251563,-13.695020876508,
117.050115735377)) ;
#189599=CARTESIAN_POINT('Ctrl Pts',(-11.0542893679301,-13.6950208703168,
117.025884691723)) ;
#189600=CARTESIAN_POINT('Ctrl Pts',(-11.1280932107038,-13.6950208641256,
117.001653648069)) ;
#189601=CARTESIAN_POINT('Ctrl Pts',(-11.1511192899988,-13.6773386169807,
117.071787370231)) ;
#189602=CARTESIAN_POINT('Ctrl Pts',(-11.1738411493158,-13.9481535278235,
117.176435570806)) ;
#189603=CARTESIAN_POINT('Ctrl Pts',(-11.1945817658723,-13.9115346180425,
117.23960814232)) ;
#189604=CARTESIAN_POINT('Ctrl Pts',(-11.1207779228081,-13.9115346192683,
117.263839185089)) ;
#189605=CARTESIAN_POINT('Ctrl Pts',(-11.0469740797439,-13.9115346204941,
117.288070227859)) ;
#189606=CARTESIAN_POINT('Ctrl Pts',(-11.0262334631874,-13.948153530275,
117.224897656345)) ;
#189607=CARTESIAN_POINT('Ctrl Pts',(-11.0054928466309,-13.984772440056,
117.161725084831)) ;
#189608=CARTESIAN_POINT('Ctrl Pts',(-11.0792966896951,-13.9847724388302,
117.137494042062)) ;
#189609=CARTESIAN_POINT('Ctrl Pts',(-11.1531005327593,-13.9847724376044,
117.113262999292)) ;
#189610=CARTESIAN_POINT('Ctrl Pts',(-11.1738411493158,-13.9481535278235,
117.176435570806)) ;
#189611=CARTESIAN_POINT('Ctrl Pts',(-11.2178302810653,-14.1811353756388,
117.345891952531)) ;
#189612=CARTESIAN_POINT('Ctrl Pts',(-11.234796139088,-14.1281930358969,
117.397567218671)) ;
#189613=CARTESIAN_POINT('Ctrl Pts',(-11.1609922953461,-14.1281930344687,
117.421798259377)) ;
#189614=CARTESIAN_POINT('Ctrl Pts',(-11.0871884516043,-14.1281930330404,
117.446029300082)) ;
#189615=CARTESIAN_POINT('Ctrl Pts',(-11.0702225935816,-14.1811353727823,
117.394354033942)) ;
#189616=CARTESIAN_POINT('Ctrl Pts',(-11.0532567355589,-14.2340777125242,
117.342678767802)) ;
#189617=CARTESIAN_POINT('Ctrl Pts',(-11.1270605793008,-14.2340777139524,
117.318447727097)) ;
#189618=CARTESIAN_POINT('Ctrl Pts',(-11.2008644230427,-14.2340777153806,
117.294216686391)) ;
#189619=CARTESIAN_POINT('Ctrl Pts',(-11.2178302810653,-14.1811353756388,
117.345891952531)) ;
#189620=CARTESIAN_POINT('Ctrl Pts',(-11.2789434257265,-14.3592804603128,
117.567414573632)) ;
#189621=CARTESIAN_POINT('Ctrl Pts',(-11.2909348548221,-14.2938199374356,
117.603938531914)) ;
#189622=CARTESIAN_POINT('Ctrl Pts',(-11.2171310104801,-14.2938199356805,
117.628169570792)) ;
#189623=CARTESIAN_POINT('Ctrl Pts',(-11.1433271661381,-14.2938199339254,
117.652400609669)) ;
#189624=CARTESIAN_POINT('Ctrl Pts',(-11.1313357370424,-14.3592804568026,
117.615876651387)) ;
#189625=CARTESIAN_POINT('Ctrl Pts',(-11.1193443079467,-14.4247409796798,
117.579352693104)) ;
#189626=CARTESIAN_POINT('Ctrl Pts',(-11.1931481522888,-14.4247409814349,
117.555121654227)) ;
#189627=CARTESIAN_POINT('Ctrl Pts',(-11.2669519966308,-14.4247409831899,
117.530890615349)) ;
#189628=CARTESIAN_POINT('Ctrl Pts',(-11.2789434257265,-14.3592804603128,
117.567414573632)) ;
#189629=CARTESIAN_POINT('Ctrl Pts',(-11.3529530376374,-14.4707867328028,
117.82855139819)) ;
#189630=CARTESIAN_POINT('Ctrl Pts',(-11.3590548784153,-14.3974420670784,
117.847136620716)) ;
#189631=CARTESIAN_POINT('Ctrl Pts',(-11.285251034286,-14.3974420666518,
117.871367660241)) ;
#189632=CARTESIAN_POINT('Ctrl Pts',(-11.2114471901566,-14.3974420662252,
117.895598699767)) ;
#189633=CARTESIAN_POINT('Ctrl Pts',(-11.2053453493787,-14.4707867319496,
117.87701347724)) ;
#189634=CARTESIAN_POINT('Ctrl Pts',(-11.1992435086008,-14.5441313976739,
117.858428254714)) ;
#189635=CARTESIAN_POINT('Ctrl Pts',(-11.2730473527302,-14.5441313981005,
117.834197215189)) ;
#189636=CARTESIAN_POINT('Ctrl Pts',(-11.3468511968595,-14.5441313985271,
117.809966175664)) ;
#189637=CARTESIAN_POINT('Ctrl Pts',(-11.3529530376374,-14.4707867328028,
117.82855139819)) ;
#189638=CARTESIAN_POINT('Ctrl Pts',(-11.4321384096907,-14.5057904984994,
118.104989650374)) ;
#189639=CARTESIAN_POINT('Ctrl Pts',(-11.4319904956564,-14.429894649573,
118.104539128091)) ;
#189640=CARTESIAN_POINT('Ctrl Pts',(-11.3581866522587,-14.4298946498541,
118.128770169845)) ;
#189641=CARTESIAN_POINT('Ctrl Pts',(-11.284382808861,-14.4298946501351,
118.153001211598)) ;
#189642=CARTESIAN_POINT('Ctrl Pts',(-11.2845307228953,-14.5057904990616,
118.153451733882)) ;
#189643=CARTESIAN_POINT('Ctrl Pts',(-11.2846786369295,-14.581686347988,
118.153902256165)) ;
#189644=CARTESIAN_POINT('Ctrl Pts',(-11.3584824803272,-14.5816863477069,
118.129671214411)) ;
#189645=CARTESIAN_POINT('Ctrl Pts',(-11.4322863237249,-14.5816863474258,
118.105440172657)) ;
#189646=CARTESIAN_POINT('Ctrl Pts',(-11.4321384096907,-14.5057904984994,
118.104989650374)) ;
#189647=CARTESIAN_POINT('Ctrl Pts',(-11.5115346995745,-14.4636194148643,
118.382300113082)) ;
#189648=CARTESIAN_POINT('Ctrl Pts',(-11.5051083611355,-14.3905570608512,
118.362726522999)) ;
#189649=CARTESIAN_POINT('Ctrl Pts',(-11.4313045190715,-14.3905570601267,
118.386957568815)) ;
#189650=CARTESIAN_POINT('Ctrl Pts',(-11.3575006770075,-14.3905570594022,
118.411188614631)) ;
#189651=CARTESIAN_POINT('Ctrl Pts',(-11.3639270154464,-14.4636194134152,
118.430762204714)) ;
#189652=CARTESIAN_POINT('Ctrl Pts',(-11.3703533538854,-14.5366817674283,
118.450335794797)) ;
#189653=CARTESIAN_POINT('Ctrl Pts',(-11.4441571959494,-14.5366817681528,
118.426104748981)) ;
#189654=CARTESIAN_POINT('Ctrl Pts',(-11.5179610380134,-14.5366817688773,
118.401873703165)) ;
#189655=CARTESIAN_POINT('Ctrl Pts',(-11.5115346995745,-14.4636194148643,
118.382300113082)) ;
#189656=CARTESIAN_POINT('Ctrl Pts',(-11.5841867566869,-14.3461280489561,
118.639074111226)) ;
#189657=CARTESIAN_POINT('Ctrl Pts',(-11.5719437539166,-14.2811630148822,
118.601783899988)) ;
#189658=CARTESIAN_POINT('Ctrl Pts',(-11.4981399133463,-14.2811630098894,
118.626014950353)) ;
#189659=CARTESIAN_POINT('Ctrl Pts',(-11.4243360727761,-14.2811630048965,
118.650246000719)) ;
#189660=CARTESIAN_POINT('Ctrl Pts',(-11.4365790755464,-14.3461280389704,
118.687536211957)) ;
#189661=CARTESIAN_POINT('Ctrl Pts',(-11.4488220783168,-14.4110930730442,
118.724826423195)) ;
#189662=CARTESIAN_POINT('Ctrl Pts',(-11.522625918887,-14.4110930780371,
118.70059537283)) ;
#189663=CARTESIAN_POINT('Ctrl Pts',(-11.5964297594572,-14.41109308303,118.676364322464)) ;
#189664=CARTESIAN_POINT('Ctrl Pts',(-11.5841867566869,-14.3461280489561,
118.639074111226)) ;
#189665=CARTESIAN_POINT('Ctrl Pts',(-11.6440388517106,-14.1630186070769,
118.856745565544)) ;
#189666=CARTESIAN_POINT('Ctrl Pts',(-11.6268671158057,-14.1107446176607,
118.80444322831)) ;
#189667=CARTESIAN_POINT('Ctrl Pts',(-11.5530632760904,-14.1107446061865,
118.828674281279)) ;
#189668=CARTESIAN_POINT('Ctrl Pts',(-11.4792594363752,-14.1107445947124,
118.852905334249)) ;
#189669=CARTESIAN_POINT('Ctrl Pts',(-11.49643117228,-14.1630185841287,118.905207671484)) ;
#189670=CARTESIAN_POINT('Ctrl Pts',(-11.5136029081849,-14.215292573545,
118.957510008719)) ;
#189671=CARTESIAN_POINT('Ctrl Pts',(-11.5874067479002,-14.2152925850191,
118.933278955749)) ;
#189672=CARTESIAN_POINT('Ctrl Pts',(-11.6612105876154,-14.2152925964932,
118.909047902779)) ;
#189673=CARTESIAN_POINT('Ctrl Pts',(-11.6440388517106,-14.1630186070769,
118.856745565544)) ;
#189674=CARTESIAN_POINT('Ctrl Pts',(-11.6865201020579,-13.9239936072657,
119.021875248409)) ;
#189675=CARTESIAN_POINT('Ctrl Pts',(-11.6656175469763,-13.8883328136029,
118.95820943773)) ;
#189676=CARTESIAN_POINT('Ctrl Pts',(-11.591813707628,-13.8883327903774,
118.982440491818)) ;
#189677=CARTESIAN_POINT('Ctrl Pts',(-11.5180098682797,-13.8883327671519,
119.006671545905)) ;
#189678=CARTESIAN_POINT('Ctrl Pts',(-11.5389124233613,-13.9239935608147,
119.070337356584)) ;
#189679=CARTESIAN_POINT('Ctrl Pts',(-11.5598149784429,-13.9596543544774,
119.134003167263)) ;
#189680=CARTESIAN_POINT('Ctrl Pts',(-11.6336188177912,-13.9596543777029,
119.109772113175)) ;
#189681=CARTESIAN_POINT('Ctrl Pts',(-11.7074226571395,-13.9596544009284,
119.085541059088)) ;
#189682=CARTESIAN_POINT('Ctrl Pts',(-11.6865201020579,-13.9239936072657,
119.021875248409)) ;
#189683=CARTESIAN_POINT('Ctrl Pts',(-11.7070382005163,-13.6520857920573,
119.119617519121)) ;
#189684=CARTESIAN_POINT('Ctrl Pts',(-11.6839436556647,-13.6353584241277,
119.049275261158)) ;
#189685=CARTESIAN_POINT('Ctrl Pts',(-11.6101398146794,-13.6353583920573,
119.073506310259)) ;
#189686=CARTESIAN_POINT('Ctrl Pts',(-11.5363359736941,-13.635358359987,
119.09773735936)) ;
#189687=CARTESIAN_POINT('Ctrl Pts',(-11.5594305185456,-13.6520857279166,
119.168079617324)) ;
#189688=CARTESIAN_POINT('Ctrl Pts',(-11.5825250633972,-13.6688130958462,
119.238421875288)) ;
#189689=CARTESIAN_POINT('Ctrl Pts',(-11.6563289043825,-13.6688131279166,
119.214190826187)) ;
#189690=CARTESIAN_POINT('Ctrl Pts',(-11.7301327453678,-13.668813159987,
119.189959777085)) ;
#189691=CARTESIAN_POINT('Ctrl Pts',(-11.7070382005163,-13.6520857920573,
119.119617519121)) ;
#189692=CARTESIAN_POINT('Ctrl Pts',(-11.7039900854668,-13.3607989189298,
119.145938172776)) ;
#189693=CARTESIAN_POINT('Ctrl Pts',(-11.6803380884392,-13.3643850289944,
119.073898005236)) ;
#189694=CARTESIAN_POINT('Ctrl Pts',(-11.6065342445709,-13.3643849861059,
119.098129045556)) ;
#189695=CARTESIAN_POINT('Ctrl Pts',(-11.5327304007025,-13.3643849432174,
119.122360085876)) ;
#189696=CARTESIAN_POINT('Ctrl Pts',(-11.5563823977301,-13.3607988331528,
119.194400253416)) ;
#189697=CARTESIAN_POINT('Ctrl Pts',(-11.5800343947576,-13.3572127230881,
119.266440420956)) ;
#189698=CARTESIAN_POINT('Ctrl Pts',(-11.653838238626,-13.3572127659766,
119.242209380636)) ;
#189699=CARTESIAN_POINT('Ctrl Pts',(-11.7276420824943,-13.3572128088652,
119.217978340316)) ;
#189700=CARTESIAN_POINT('Ctrl Pts',(-11.7039900854668,-13.3607989189298,
119.145938172776)) ;
#189701=CARTESIAN_POINT('Ctrl Pts',(-11.6767330335314,-13.0758433976518,
119.098233907499)) ;
#189702=CARTESIAN_POINT('Ctrl Pts',(-11.6542192956397,-13.0993300266372,
119.029660693489)) ;
#189703=CARTESIAN_POINT('Ctrl Pts',(-11.5804154474959,-13.0993299787843,
119.053891720787)) ;
#189704=CARTESIAN_POINT('Ctrl Pts',(-11.5066115993522,-13.0993299309314,
119.078122748085)) ;
#189705=CARTESIAN_POINT('Ctrl Pts',(-11.529125337244,-13.075843301946,119.146695962096)) ;
#189706=CARTESIAN_POINT('Ctrl Pts',(-11.5516390751357,-13.0523566729605,
119.215269176106)) ;
#189707=CARTESIAN_POINT('Ctrl Pts',(-11.6254429232794,-13.0523567208134,
119.191038148808)) ;
#189708=CARTESIAN_POINT('Ctrl Pts',(-11.6992467714231,-13.0523567686663,
119.166807121509)) ;
#189709=CARTESIAN_POINT('Ctrl Pts',(-11.6767330335314,-13.0758433976518,
119.098233907499)) ;
#189710=CARTESIAN_POINT('Ctrl Pts',(-11.6263549017493,-12.8137701829539,
118.980301130087)) ;
#189711=CARTESIAN_POINT('Ctrl Pts',(-11.606591109743,-12.8555883335488,
118.920103807366)) ;
#189712=CARTESIAN_POINT('Ctrl Pts',(-11.5327872562889,-12.8555882837421,
118.944334818489)) ;
#189713=CARTESIAN_POINT('Ctrl Pts',(-11.4589834028348,-12.8555882339354,
118.968565829613)) ;
#189714=CARTESIAN_POINT('Ctrl Pts',(-11.4787471948412,-12.8137700833405,
119.028763152334)) ;
#189715=CARTESIAN_POINT('Ctrl Pts',(-11.4985109868476,-12.7719519327456,
119.088960475056)) ;
#189716=CARTESIAN_POINT('Ctrl Pts',(-11.5723148403017,-12.7719519825523,
119.064729463932)) ;
#189717=CARTESIAN_POINT('Ctrl Pts',(-11.6461186937557,-12.771952032359,
119.040498452808)) ;
#189718=CARTESIAN_POINT('Ctrl Pts',(-11.6263549017493,-12.8137701829539,
118.980301130087)) ;
#189719=CARTESIAN_POINT('Ctrl Pts',(-11.5554224404524,-12.5948352961054,
118.79984493087)) ;
#189720=CARTESIAN_POINT('Ctrl Pts',(-11.5398458335298,-12.6519997752805,
118.75240109813)) ;
#189721=CARTESIAN_POINT('Ctrl Pts',(-11.4660419740139,-12.6519997298115,
118.776632090791)) ;
#189722=CARTESIAN_POINT('Ctrl Pts',(-11.392238114498,-12.6519996843424,
118.800863083451)) ;
#189723=CARTESIAN_POINT('Ctrl Pts',(-11.4078147214206,-12.5948352051674,
118.848306916191)) ;
#189724=CARTESIAN_POINT('Ctrl Pts',(-11.4233913283432,-12.5376707259923,
118.89575074893)) ;
#189725=CARTESIAN_POINT('Ctrl Pts',(-11.4971951878591,-12.5376707714613,
118.87151975627)) ;
#189726=CARTESIAN_POINT('Ctrl Pts',(-11.570999047375,-12.5376708169303,
118.84728876361)) ;
#189727=CARTESIAN_POINT('Ctrl Pts',(-11.5554224404524,-12.5948352961054,
118.79984493087)) ;
#189728=CARTESIAN_POINT('Ctrl Pts',(-11.4693499814157,-12.4363827345609,
118.57295586756)) ;
#189729=CARTESIAN_POINT('Ctrl Pts',(-11.4590304335375,-12.5046923403289,
118.541524188328)) ;
#189730=CARTESIAN_POINT('Ctrl Pts',(-11.3852265691063,-12.5046923075435,
118.565755166016)) ;
#189731=CARTESIAN_POINT('Ctrl Pts',(-11.311422704675,-12.5046922747581,
118.589986143705)) ;
#189732=CARTESIAN_POINT('Ctrl Pts',(-11.3217422525532,-12.4363826689901,
118.621417822938)) ;
#189733=CARTESIAN_POINT('Ctrl Pts',(-11.3320618004314,-12.368073063222,
118.65284950217)) ;
#189734=CARTESIAN_POINT('Ctrl Pts',(-11.4058656648627,-12.3680730960074,
118.628618524481)) ;
#189735=CARTESIAN_POINT('Ctrl Pts',(-11.4796695292939,-12.3680731287928,
118.604387546793)) ;
#189736=CARTESIAN_POINT('Ctrl Pts',(-11.4693499814157,-12.4363827345609,
118.57295586756)) ;
#189737=CARTESIAN_POINT('Ctrl Pts',(-11.372312899221,-12.3469185629382,
118.312891406487)) ;
#189738=CARTESIAN_POINT('Ctrl Pts',(-11.3680187374058,-12.4215734203002,
118.299812080862)) ;
#189739=CARTESIAN_POINT('Ctrl Pts',(-11.2942148686676,-12.4215734050828,
118.324043045432)) ;
#189740=CARTESIAN_POINT('Ctrl Pts',(-11.2204109999293,-12.4215733898654,
118.348274010003)) ;
#189741=CARTESIAN_POINT('Ctrl Pts',(-11.2247051617446,-12.3469185325034,
118.361353335628)) ;
#189742=CARTESIAN_POINT('Ctrl Pts',(-11.2289993235598,-12.2722636751415,
118.374432661253)) ;
#189743=CARTESIAN_POINT('Ctrl Pts',(-11.302803192298,-12.2722636903589,
118.350201696683)) ;
#189744=CARTESIAN_POINT('Ctrl Pts',(-11.3766070610363,-12.2722637055763,
118.325970732112)) ;
#189745=CARTESIAN_POINT('Ctrl Pts',(-11.372312899221,-12.3469185629382,
118.312891406487)) ;
#189746=CARTESIAN_POINT('Ctrl Pts',(-11.270758988364,-12.3346897142696,
118.039141827272)) ;
#189747=CARTESIAN_POINT('Ctrl Pts',(-11.272812768128,-12.410307219777,118.04539730732)) ;
#189748=CARTESIAN_POINT('Ctrl Pts',(-11.1990088967919,-12.4103072275808,
118.069628263978)) ;
#189749=CARTESIAN_POINT('Ctrl Pts',(-11.1252050254558,-12.4103072353845,
118.093859220636)) ;
#189750=CARTESIAN_POINT('Ctrl Pts',(-11.1231512456917,-12.3346897298771,
118.087603740587)) ;
#189751=CARTESIAN_POINT('Ctrl Pts',(-11.1210974659277,-12.2590722243697,
118.081348260539)) ;
#189752=CARTESIAN_POINT('Ctrl Pts',(-11.1949013372638,-12.259072216566,
118.057117303881)) ;
#189753=CARTESIAN_POINT('Ctrl Pts',(-11.2687052085999,-12.2590722087622,
118.032886347224)) ;
#189754=CARTESIAN_POINT('Ctrl Pts',(-11.270758988364,-12.3346897142696,
118.039141827272)) ;
#189755=CARTESIAN_POINT('Ctrl Pts',(-11.1721007998187,-12.3996707792268,
117.77397409113)) ;
#189756=CARTESIAN_POINT('Ctrl Pts',(-11.1803145318333,-12.470861286488,
117.798991791736)) ;
#189757=CARTESIAN_POINT('Ctrl Pts',(-11.1065106607222,-12.4708613194526,
117.823222749078)) ;
#189758=CARTESIAN_POINT('Ctrl Pts',(-11.032706789611,-12.4708613524172,
117.847453706421)) ;
#189759=CARTESIAN_POINT('Ctrl Pts',(-11.0244930575963,-12.3996708451561,
117.822436005816)) ;
#189760=CARTESIAN_POINT('Ctrl Pts',(-11.0162793255817,-12.3284803378949,
117.797418305211)) ;
#189761=CARTESIAN_POINT('Ctrl Pts',(-11.0900831966928,-12.3284803049303,
117.773187347868)) ;
#189762=CARTESIAN_POINT('Ctrl Pts',(-11.163887067804,-12.3284802719657,
117.748956390525)) ;
#189763=CARTESIAN_POINT('Ctrl Pts',(-11.1721007998187,-12.3996707792268,
117.77397409113)) ;
#189764=CARTESIAN_POINT('Ctrl Pts',(-11.0813833295911,-12.5380776390174,
117.5332221053)) ;
#189765=CARTESIAN_POINT('Ctrl Pts',(-11.0952068472566,-12.5997094329327,
117.575326307758)) ;
#189766=CARTESIAN_POINT('Ctrl Pts',(-11.0214029785273,-12.5997094914945,
117.599557272356)) ;
#189767=CARTESIAN_POINT('Ctrl Pts',(-10.9475991097979,-12.5997095500564,
117.623788236953)) ;
#189768=CARTESIAN_POINT('Ctrl Pts',(-10.9337755921324,-12.5380777561411,
117.581684034495)) ;
#189769=CARTESIAN_POINT('Ctrl Pts',(-10.9199520744669,-12.4764459622258,
117.539579832036)) ;
#189770=CARTESIAN_POINT('Ctrl Pts',(-10.9937559431962,-12.476445903664,
117.515348867439)) ;
#189771=CARTESIAN_POINT('Ctrl Pts',(-11.0675598119255,-12.4764458451021,
117.491117902841)) ;
#189772=CARTESIAN_POINT('Ctrl Pts',(-11.0813833295911,-12.5380776390174,
117.5332221053)) ;
#189773=CARTESIAN_POINT('Ctrl Pts',(-11.0052275153054,-12.739380812412,
117.336728726965)) ;
#189774=CARTESIAN_POINT('Ctrl Pts',(-11.0236543762053,-12.7870487344557,
117.392853970097)) ;
#189775=CARTESIAN_POINT('Ctrl Pts',(-10.9498505125397,-12.7870488154654,
117.417084950118)) ;
#189776=CARTESIAN_POINT('Ctrl Pts',(-10.876046648874,-12.7870488964751,
117.441315930138)) ;
#189777=CARTESIAN_POINT('Ctrl Pts',(-10.8576197879741,-12.7393809744314,
117.385190687007)) ;
#189778=CARTESIAN_POINT('Ctrl Pts',(-10.8391929270742,-12.6917130523877,
117.329065443875)) ;
#189779=CARTESIAN_POINT('Ctrl Pts',(-10.9129967907399,-12.691712971378,
117.304834463854)) ;
#189780=CARTESIAN_POINT('Ctrl Pts',(-10.9868006544055,-12.6917128903682,
117.280603483834)) ;
#189781=CARTESIAN_POINT('Ctrl Pts',(-11.0052275153054,-12.739380812412,
117.336728726965)) ;
#189782=CARTESIAN_POINT('Ctrl Pts',(-10.9480638418633,-12.9893867745162,
117.198103000491)) ;
#189783=CARTESIAN_POINT('Ctrl Pts',(-10.9697745011554,-13.0196703754918,
117.264230163634)) ;
#189784=CARTESIAN_POINT('Ctrl Pts',(-10.8959706446165,-13.0196704733174,
117.288461165362)) ;
#189785=CARTESIAN_POINT('Ctrl Pts',(-10.8221667880775,-13.019670571143,
117.312692167089)) ;
#189786=CARTESIAN_POINT('Ctrl Pts',(-10.8004561287854,-12.9893869701674,
117.246565003946)) ;
#189787=CARTESIAN_POINT('Ctrl Pts',(-10.7787454694932,-12.9591033691919,
117.180437840802)) ;
#189788=CARTESIAN_POINT('Ctrl Pts',(-10.8525493260322,-12.9591032713663,
117.156206839075)) ;
#189789=CARTESIAN_POINT('Ctrl Pts',(-10.9263531825711,-12.9591031735407,
117.131975837347)) ;
#189790=CARTESIAN_POINT('Ctrl Pts',(-10.9480638418633,-12.9893867745162,
117.198103000491)) ;
#189791=CARTESIAN_POINT('Ctrl Pts',(-10.91326793993,-13.2694171615401,117.12751697522)) ;
#189792=CARTESIAN_POINT('Ctrl Pts',(-10.9367074543696,-13.2801946819997,
117.198909952163)) ;
#189793=CARTESIAN_POINT('Ctrl Pts',(-10.8629036063477,-13.2801947890163,
117.223140979832)) ;
#189794=CARTESIAN_POINT('Ctrl Pts',(-10.7890997583258,-13.2801948960329,
117.247372007501)) ;
#189795=CARTESIAN_POINT('Ctrl Pts',(-10.7656602438862,-13.2694173755733,
117.175979030557)) ;
#189796=CARTESIAN_POINT('Ctrl Pts',(-10.7422207294466,-13.2586398551137,
117.104586053614)) ;
#189797=CARTESIAN_POINT('Ctrl Pts',(-10.8160245774685,-13.2586397480971,
117.080355025945)) ;
#189798=CARTESIAN_POINT('Ctrl Pts',(-10.8898284254904,-13.2586396410806,
117.056123998276)) ;
#189799=CARTESIAN_POINT('Ctrl Pts',(-10.91326793993,-13.2694171615401,117.12751697522)) ;
#189800=CARTESIAN_POINT('Ctrl Pts',(-10.9025452534367,-13.5619468890867,
117.130491501621)) ;
#189801=CARTESIAN_POINT('Ctrl Pts',(-10.9260309116402,-13.5523172456924,
117.202025025017)) ;
#189802=CARTESIAN_POINT('Ctrl Pts',(-10.8522270727192,-13.5523173531236,
117.226256080406)) ;
#189803=CARTESIAN_POINT('Ctrl Pts',(-10.7784232337981,-13.5523174605549,
117.250487135794)) ;
#189804=CARTESIAN_POINT('Ctrl Pts',(-10.7549375755945,-13.5619471039492,
117.178953612398)) ;
#189805=CARTESIAN_POINT('Ctrl Pts',(-10.7314519173909,-13.5715767473435,
117.107420089002)) ;
#189806=CARTESIAN_POINT('Ctrl Pts',(-10.805255756312,-13.5715766399123,
117.083189033613)) ;
#189807=CARTESIAN_POINT('Ctrl Pts',(-10.8790595952331,-13.5715765324811,
117.058957978225)) ;
#189808=CARTESIAN_POINT('Ctrl Pts',(-10.9025452534367,-13.5619468890867,
117.130491501621)) ;
#189809=CARTESIAN_POINT('Ctrl Pts',(-10.915841183644,-13.8411213292838,
117.206227086059)) ;
#189810=CARTESIAN_POINT('Ctrl Pts',(-10.937704050494,-13.8119862931275,
117.272817848839)) ;
#189811=CARTESIAN_POINT('Ctrl Pts',(-10.8639002202108,-13.8119863923944,
117.297048930537)) ;
#189812=CARTESIAN_POINT('Ctrl Pts',(-10.7900963899276,-13.8119864916613,
117.321280012236)) ;
#189813=CARTESIAN_POINT('Ctrl Pts',(-10.7682335230776,-13.8411215278176,
117.254689249455)) ;
#189814=CARTESIAN_POINT('Ctrl Pts',(-10.7463706562276,-13.870256563974,
117.188098486674)) ;
#189815=CARTESIAN_POINT('Ctrl Pts',(-10.8201744865108,-13.8702564647071,
117.163867404976)) ;
#189816=CARTESIAN_POINT('Ctrl Pts',(-10.893978316794,-13.8702563654402,
117.139636323278)) ;
#189817=CARTESIAN_POINT('Ctrl Pts',(-10.915841183644,-13.8411213292838,
117.206227086059)) ;
#189818=CARTESIAN_POINT('Ctrl Pts',(-10.9516849884551,-14.0928083771544,
117.351013070944)) ;
#189819=CARTESIAN_POINT('Ctrl Pts',(-10.9703412062463,-14.0460580395473,
117.407836898122)) ;
#189820=CARTESIAN_POINT('Ctrl Pts',(-10.8965373833647,-14.0460581223417,
117.432068002364)) ;
#189821=CARTESIAN_POINT('Ctrl Pts',(-10.822733560483,-14.0460582051361,
117.456299106607)) ;
#189822=CARTESIAN_POINT('Ctrl Pts',(-10.8040773426918,-14.0928085427432,
117.399475279428)) ;
#189823=CARTESIAN_POINT('Ctrl Pts',(-10.7854211249006,-14.1395588803503,
117.34265145225)) ;
#189824=CARTESIAN_POINT('Ctrl Pts',(-10.8592249477822,-14.1395587975559,
117.318420348007)) ;
#189825=CARTESIAN_POINT('Ctrl Pts',(-10.9330287706639,-14.1395587147615,
117.294189243765)) ;
#189826=CARTESIAN_POINT('Ctrl Pts',(-10.9516849884551,-14.0928083771544,
117.351013070944)) ;
#189827=CARTESIAN_POINT('Ctrl Pts',(-11.0064738727342,-14.2946225939457,
117.553299701914)) ;
#189828=CARTESIAN_POINT('Ctrl Pts',(-11.0206000342901,-14.2337123839225,
117.596325708778)) ;
#189829=CARTESIAN_POINT('Ctrl Pts',(-10.9467962167889,-14.2337124445756,
117.620556829408)) ;
#189830=CARTESIAN_POINT('Ctrl Pts',(-10.8729923992877,-14.2337125052288,
117.644787950038)) ;
#189831=CARTESIAN_POINT('Ctrl Pts',(-10.8588662377318,-14.2946227152521,
117.601761943175)) ;
#189832=CARTESIAN_POINT('Ctrl Pts',(-10.8447400761759,-14.3555329252753,
117.558735936311)) ;
#189833=CARTESIAN_POINT('Ctrl Pts',(-10.9185438936771,-14.3555328646222,
117.534504815681)) ;
#189834=CARTESIAN_POINT('Ctrl Pts',(-10.9923477111784,-14.355532803969,
117.510273695051)) ;
#189835=CARTESIAN_POINT('Ctrl Pts',(-11.0064738727342,-14.2946225939457,
117.553299701914)) ;
#189836=CARTESIAN_POINT('Ctrl Pts',(-11.0756251998262,-14.4342154714355,
117.79936755511)) ;
#189837=CARTESIAN_POINT('Ctrl Pts',(-11.0842111585001,-14.3634681415102,
117.825518997977)) ;
#189838=CARTESIAN_POINT('Ctrl Pts',(-11.0104073439954,-14.3634681764234,
117.849750127735)) ;
#189839=CARTESIAN_POINT('Ctrl Pts',(-10.9366035294908,-14.3634682113365,
117.873981257492)) ;
#189840=CARTESIAN_POINT('Ctrl Pts',(-10.9280175708169,-14.4342155412618,
117.847829814624)) ;
#189841=CARTESIAN_POINT('Ctrl Pts',(-10.919431612143,-14.5049628711871,
117.821678371757)) ;
#189842=CARTESIAN_POINT('Ctrl Pts',(-10.9932354266477,-14.5049628362739,
117.797447241999)) ;
#189843=CARTESIAN_POINT('Ctrl Pts',(-11.0670392411523,-14.5049628013607,
117.773216112242)) ;
#189844=CARTESIAN_POINT('Ctrl Pts',(-11.0756251998262,-14.4342154714355,
117.79936755511)) ;
#189845=CARTESIAN_POINT('Ctrl Pts',(-11.153880257495,-14.5009486089819,
118.073339050419)) ;
#189846=CARTESIAN_POINT('Ctrl Pts',(-11.156278566929,-14.4254353908754,
118.080643912192)) ;
#189847=CARTESIAN_POINT('Ctrl Pts',(-11.0824747524078,-14.4254353992881,
118.104875041898)) ;
#189848=CARTESIAN_POINT('Ctrl Pts',(-11.0086709378866,-14.4254354077009,
118.129106171605)) ;
#189849=CARTESIAN_POINT('Ctrl Pts',(-11.0062726284526,-14.5009486258073,
118.121801309832)) ;
#189850=CARTESIAN_POINT('Ctrl Pts',(-11.0038743190187,-14.5764618439138,
118.114496448059)) ;
#189851=CARTESIAN_POINT('Ctrl Pts',(-11.0776781335399,-14.5764618355011,
118.090265318352)) ;
#189852=CARTESIAN_POINT('Ctrl Pts',(-11.1514819480611,-14.5764618270883,
118.066034188645)) ;
#189853=CARTESIAN_POINT('Ctrl Pts',(-11.153880257495,-14.5009486089819,
118.073339050419)) ;
#189854=CARTESIAN_POINT('Ctrl Pts',(-11.2337163322941,-14.4900601303297,
118.351780652459)) ;
#189855=CARTESIAN_POINT('Ctrl Pts',(-11.2298142925024,-14.4151940072696,
118.339895667138)) ;
#189856=CARTESIAN_POINT('Ctrl Pts',(-11.1560104761921,-14.4151939916633,
118.364126791396)) ;
#189857=CARTESIAN_POINT('Ctrl Pts',(-11.0822066598818,-14.4151939760569,
118.388357915653)) ;
#189858=CARTESIAN_POINT('Ctrl Pts',(-11.0861086996736,-14.490060099117,
118.400242900973)) ;
#189859=CARTESIAN_POINT('Ctrl Pts',(-11.0900107394653,-14.564926222177,
118.412127886294)) ;
#189860=CARTESIAN_POINT('Ctrl Pts',(-11.1638145557756,-14.5649262377834,
118.387896762036)) ;
#189861=CARTESIAN_POINT('Ctrl Pts',(-11.2376183720859,-14.5649262533898,
118.363665637779)) ;
#189862=CARTESIAN_POINT('Ctrl Pts',(-11.2337163322941,-14.4900601303297,
118.351780652459)) ;
#189863=CARTESIAN_POINT('Ctrl Pts',(-11.3100721441772,-14.4021465802023,
118.619936605905)) ;
#189864=CARTESIAN_POINT('Ctrl Pts',(-11.3000967501311,-14.3333051056759,
118.589553163606)) ;
#189865=CARTESIAN_POINT('Ctrl Pts',(-11.2262929293861,-14.3333050707066,
118.613784274357)) ;
#189866=CARTESIAN_POINT('Ctrl Pts',(-11.1524891086412,-14.3333050357374,
118.638015385107)) ;
#189867=CARTESIAN_POINT('Ctrl Pts',(-11.1624645026873,-14.4021465102638,
118.668398827405)) ;
#189868=CARTESIAN_POINT('Ctrl Pts',(-11.1724398967335,-14.4709879847903,
118.698782269704)) ;
#189869=CARTESIAN_POINT('Ctrl Pts',(-11.2462437174784,-14.4709880197595,
118.674551158953)) ;
#189870=CARTESIAN_POINT('Ctrl Pts',(-11.3200475382233,-14.4709880547288,
118.650320048203)) ;
#189871=CARTESIAN_POINT('Ctrl Pts',(-11.3100721441772,-14.4021465802023,
118.619936605905)) ;
#189872=CARTESIAN_POINT('Ctrl Pts',(-11.37566907483,-14.2443882215466,118.855102173573)) ;
#189873=CARTESIAN_POINT('Ctrl Pts',(-11.3603668518626,-14.1864574930971,
118.80849406999)) ;
#189874=CARTESIAN_POINT('Ctrl Pts',(-11.2865630258025,-14.1864574444021,
118.832725164551)) ;
#189875=CARTESIAN_POINT('Ctrl Pts',(-11.2127591997423,-14.1864573957072,
118.856956259112)) ;
#189876=CARTESIAN_POINT('Ctrl Pts',(-11.2280614227097,-14.2443881241568,
118.903564362695)) ;
#189877=CARTESIAN_POINT('Ctrl Pts',(-11.2433636456771,-14.3023188526063,
118.950172466279)) ;
#189878=CARTESIAN_POINT('Ctrl Pts',(-11.3171674717372,-14.3023189013012,
118.925941371718)) ;
#189879=CARTESIAN_POINT('Ctrl Pts',(-11.3909712977974,-14.3023189499961,
118.901710277157)) ;
#189880=CARTESIAN_POINT('Ctrl Pts',(-11.37566907483,-14.2443882215466,118.855102173573)) ;
#189881=CARTESIAN_POINT('Ctrl Pts',(-11.4258059802253,-14.0257063779415,
119.043473900735)) ;
#189882=CARTESIAN_POINT('Ctrl Pts',(-11.4062419396678,-13.9829558305902,
118.983884988605)) ;
#189883=CARTESIAN_POINT('Ctrl Pts',(-11.3324381072493,-13.9829557770323,
119.008116063799)) ;
#189884=CARTESIAN_POINT('Ctrl Pts',(-11.2586342748308,-13.9829557234744,
119.032347138994)) ;
#189885=CARTESIAN_POINT('Ctrl Pts',(-11.2781983153884,-14.0257062708258,
119.091936051124)) ;
#189886=CARTESIAN_POINT('Ctrl Pts',(-11.2977623559459,-14.0684568181771,
119.151524963255)) ;
#189887=CARTESIAN_POINT('Ctrl Pts',(-11.3715661883644,-14.068456871735,
119.12729388806)) ;
#189888=CARTESIAN_POINT('Ctrl Pts',(-11.4453700207828,-14.0684569252929,
119.103062812865)) ;
#189889=CARTESIAN_POINT('Ctrl Pts',(-11.4258059802253,-14.0257063779415,
119.043473900735)) ;
#189890=CARTESIAN_POINT('Ctrl Pts',(-11.4553454834867,-13.7667943185538,
119.168622081409)) ;
#189891=CARTESIAN_POINT('Ctrl Pts',(-11.4329616627383,-13.7420568683352,
119.100444573897)) ;
#189892=CARTESIAN_POINT('Ctrl Pts',(-11.359157824951,-13.7420568128391,
119.124675632739)) ;
#189893=CARTESIAN_POINT('Ctrl Pts',(-11.2853539871637,-13.7420567573429,
119.148906691581)) ;
#189894=CARTESIAN_POINT('Ctrl Pts',(-11.3077378079121,-13.7667942075616,
119.217084199093)) ;
#189895=CARTESIAN_POINT('Ctrl Pts',(-11.3301216286606,-13.7915316577803,
119.285261706605)) ;
#189896=CARTESIAN_POINT('Ctrl Pts',(-11.4039254664479,-13.7915317132764,
119.261030647763)) ;
#189897=CARTESIAN_POINT('Ctrl Pts',(-11.4777293042352,-13.7915317687725,
119.236799588921)) ;
#189898=CARTESIAN_POINT('Ctrl Pts',(-11.4553454834867,-13.7667943185538,
119.168622081409)) ;
#189899=CARTESIAN_POINT('Ctrl Pts',(-11.4621777273754,-13.4796298971122,
119.225070200418)) ;
#189900=CARTESIAN_POINT('Ctrl Pts',(-11.438545300536,-13.4749049518927,
119.153089640415)) ;
#189901=CARTESIAN_POINT('Ctrl Pts',(-11.3647414577201,-13.4749049038309,
119.177320683941)) ;
#189902=CARTESIAN_POINT('Ctrl Pts',(-11.2909376149041,-13.474904855769,
119.201551727466)) ;
#189903=CARTESIAN_POINT('Ctrl Pts',(-11.3145700417435,-13.4796298009885,
119.27353228747)) ;
#189904=CARTESIAN_POINT('Ctrl Pts',(-11.3382024685828,-13.4843547462079,
119.345512847473)) ;
#189905=CARTESIAN_POINT('Ctrl Pts',(-11.4120063113988,-13.4843547942698,
119.321281803947)) ;
#189906=CARTESIAN_POINT('Ctrl Pts',(-11.4858101542147,-13.4843548423316,
119.297050760422)) ;
#189907=CARTESIAN_POINT('Ctrl Pts',(-11.4621777273754,-13.4796298971122,
119.225070200418)) ;
#189908=CARTESIAN_POINT('Ctrl Pts',(-11.4447439616591,-13.1904267551927,
119.207288539011)) ;
#189909=CARTESIAN_POINT('Ctrl Pts',(-11.4215622116791,-13.2058873743104,
119.136680668146)) ;
#189910=CARTESIAN_POINT('Ctrl Pts',(-11.3477583653682,-13.2058873346672,
119.160911701027)) ;
#189911=CARTESIAN_POINT('Ctrl Pts',(-11.2739545190573,-13.205887295024,
119.185142733907)) ;
#189912=CARTESIAN_POINT('Ctrl Pts',(-11.2971362690373,-13.1904266759062,
119.255750604772)) ;
#189913=CARTESIAN_POINT('Ctrl Pts',(-11.3203180190173,-13.1749660567885,
119.326358475637)) ;
#189914=CARTESIAN_POINT('Ctrl Pts',(-11.3941218653282,-13.1749660964317,
119.302127442757)) ;
#189915=CARTESIAN_POINT('Ctrl Pts',(-11.4679257116391,-13.1749661360749,
119.277896409876)) ;
#189916=CARTESIAN_POINT('Ctrl Pts',(-11.4447439616591,-13.1904267551927,
119.207288539011)) ;
#189917=CARTESIAN_POINT('Ctrl Pts',(-11.4032367595843,-12.9149395489465,
119.11653118219)) ;
#189918=CARTESIAN_POINT('Ctrl Pts',(-11.3821797578339,-12.9496591977343,
119.052394951809)) ;
#189919=CARTESIAN_POINT('Ctrl Pts',(-11.3083759098325,-12.9496591712855,
119.076625979541)) ;
#189920=CARTESIAN_POINT('Ctrl Pts',(-11.2345720618312,-12.9496591448368,
119.100857007273)) ;
#189921=CARTESIAN_POINT('Ctrl Pts',(-11.2556290635817,-12.914939496049,
119.164993237654)) ;
#189922=CARTESIAN_POINT('Ctrl Pts',(-11.2766860653321,-12.8802198472613,
119.229129468036)) ;
#189923=CARTESIAN_POINT('Ctrl Pts',(-11.3504899133335,-12.88021987371,119.204898440304)) ;
#189924=CARTESIAN_POINT('Ctrl Pts',(-11.4242937613348,-12.8802199001588,
119.180667412572)) ;
#189925=CARTESIAN_POINT('Ctrl Pts',(-11.4032367595843,-12.9149395489465,
119.11653118219)) ;
#189926=CARTESIAN_POINT('Ctrl Pts',(-11.34057571108,-12.6780026906519,118.960998194151)) ;
#189927=CARTESIAN_POINT('Ctrl Pts',(-11.3231311967939,-12.7293185102392,
118.907865017845)) ;
#189928=CARTESIAN_POINT('Ctrl Pts',(-11.2493273482835,-12.7293184935026,
118.932096044026)) ;
#189929=CARTESIAN_POINT('Ctrl Pts',(-11.1755234997732,-12.729318476766,
118.956327070207)) ;
#189930=CARTESIAN_POINT('Ctrl Pts',(-11.1929680140592,-12.6780026571787,
119.009460246513)) ;
#189931=CARTESIAN_POINT('Ctrl Pts',(-11.2104125283453,-12.6266868375913,
119.062593422819)) ;
#189932=CARTESIAN_POINT('Ctrl Pts',(-11.2842163768557,-12.6266868543279,
119.038362396638)) ;
#189933=CARTESIAN_POINT('Ctrl Pts',(-11.3580202253661,-12.6266868710645,
119.014131370457)) ;
#189934=CARTESIAN_POINT('Ctrl Pts',(-11.34057571108,-12.6780026906519,118.960998194151)) ;
#189935=CARTESIAN_POINT('Ctrl Pts',(-11.2599568255112,-12.492912372698,
118.750912408693)) ;
#189936=CARTESIAN_POINT('Ctrl Pts',(-11.2473811529661,-12.5572296336134,
118.712608938893)) ;
#189937=CARTESIAN_POINT('Ctrl Pts',(-11.173577305252,-12.5572296258791,
118.736839967499)) ;
#189938=CARTESIAN_POINT('Ctrl Pts',(-11.099773457538,-12.5572296181447,
118.761070996106)) ;
#189939=CARTESIAN_POINT('Ctrl Pts',(-11.1123491300831,-12.4929123572293,
118.799374465907)) ;
#189940=CARTESIAN_POINT('Ctrl Pts',(-11.1249248026282,-12.4285950963139,
118.837677935707)) ;
#189941=CARTESIAN_POINT('Ctrl Pts',(-11.1987286503423,-12.4285951040482,
118.8134469071)) ;
#189942=CARTESIAN_POINT('Ctrl Pts',(-11.2725324980563,-12.4285951117825,
118.789215878493)) ;
#189943=CARTESIAN_POINT('Ctrl Pts',(-11.2599568255112,-12.492912372698,
118.750912408693)) ;
#189944=CARTESIAN_POINT('Ctrl Pts',(-11.1664274260683,-12.3740385950698,
118.501529078933)) ;
#189945=CARTESIAN_POINT('Ctrl Pts',(-11.1596290262187,-12.446753464716,
118.480822249738)) ;
#189946=CARTESIAN_POINT('Ctrl Pts',(-11.0858251801177,-12.4467534627922,
118.505053283258)) ;
#189947=CARTESIAN_POINT('Ctrl Pts',(-11.0120213340167,-12.4467534608683,
118.529284316778)) ;
#189948=CARTESIAN_POINT('Ctrl Pts',(-11.0188197338663,-12.374038591222,
118.549991145973)) ;
#189949=CARTESIAN_POINT('Ctrl Pts',(-11.0256181337159,-12.3013237215758,
118.570697975168)) ;
#189950=CARTESIAN_POINT('Ctrl Pts',(-11.0994219798169,-12.3013237234996,
118.546466941648)) ;
#189951=CARTESIAN_POINT('Ctrl Pts',(-11.1732258259179,-12.3013237254235,
118.522235908128)) ;
#189952=CARTESIAN_POINT('Ctrl Pts',(-11.1664274260683,-12.3740385950698,
118.501529078933)) ;
#189953=CARTESIAN_POINT('Ctrl Pts',(-11.0659273383696,-12.3302346237977,
118.230957628629)) ;
#189954=CARTESIAN_POINT('Ctrl Pts',(-11.0654009453968,-12.406117742521,
118.229354320508)) ;
#189955=CARTESIAN_POINT('Ctrl Pts',(-10.991597101039,-12.4061177428899,
118.253585359338)) ;
#189956=CARTESIAN_POINT('Ctrl Pts',(-10.9177932566812,-12.4061177432587,
118.277816398167)) ;
#189957=CARTESIAN_POINT('Ctrl Pts',(-10.918319649654,-12.3302346245354,
118.279419706287)) ;
#189958=CARTESIAN_POINT('Ctrl Pts',(-10.9188460426267,-12.2543515058121,
118.281023014408)) ;
#189959=CARTESIAN_POINT('Ctrl Pts',(-10.9926498869845,-12.2543515054432,
118.256791975578)) ;
#189960=CARTESIAN_POINT('Ctrl Pts',(-11.0664537313423,-12.2543515050743,
118.232560936749)) ;
#189961=CARTESIAN_POINT('Ctrl Pts',(-11.0659273383696,-12.3302346237977,
118.230957628629)) ;
#189962=CARTESIAN_POINT('Ctrl Pts',(-10.9655287020424,-12.3639942142519,
117.960502448918)) ;
#189963=CARTESIAN_POINT('Ctrl Pts',(-10.9712805841424,-12.4376333996041,
117.978021753744)) ;
#189964=CARTESIAN_POINT('Ctrl Pts',(-10.8974767409502,-12.4376333997196,
118.002252796123)) ;
#189965=CARTESIAN_POINT('Ctrl Pts',(-10.8236728977579,-12.4376333998351,
118.026483838503)) ;
#189966=CARTESIAN_POINT('Ctrl Pts',(-10.8179210156579,-12.3639942144829,
118.008964533677)) ;
#189967=CARTESIAN_POINT('Ctrl Pts',(-10.8121691335578,-12.2903550291307,
117.99144522885)) ;
#189968=CARTESIAN_POINT('Ctrl Pts',(-10.8859729767501,-12.2903550290152,
117.967214186471)) ;
#189969=CARTESIAN_POINT('Ctrl Pts',(-10.9597768199423,-12.2903550288997,
117.942983144091)) ;
#189970=CARTESIAN_POINT('Ctrl Pts',(-10.9655287020424,-12.3639942142519,
117.960502448918)) ;
#189971=CARTESIAN_POINT('Ctrl Pts',(-10.8702494346859,-12.4744699305646,
117.706006023523)) ;
#189972=CARTESIAN_POINT('Ctrl Pts',(-10.8819243834061,-12.5405049323792,
117.741566033642)) ;
#189973=CARTESIAN_POINT('Ctrl Pts',(-10.8081205408963,-12.5405049308727,
117.7657970781)) ;
#189974=CARTESIAN_POINT('Ctrl Pts',(-10.7343166983866,-12.5405049293662,
117.790028122558)) ;
#189975=CARTESIAN_POINT('Ctrl Pts',(-10.7226417496664,-12.4744699275516,
117.75446811244)) ;
#189976=CARTESIAN_POINT('Ctrl Pts',(-10.7109668009462,-12.408434925737,
117.718908102322)) ;
#189977=CARTESIAN_POINT('Ctrl Pts',(-10.784770643456,-12.4084349272435,
117.694677057863)) ;
#189978=CARTESIAN_POINT('Ctrl Pts',(-10.8585744859657,-12.40843492875,117.670446013405)) ;
#189979=CARTESIAN_POINT('Ctrl Pts',(-10.8702494346859,-12.4744699305646,
117.706006023523)) ;
#189980=CARTESIAN_POINT('Ctrl Pts',(-10.7883722736656,-12.6502203530517,
117.491779654815)) ;
#189981=CARTESIAN_POINT('Ctrl Pts',(-10.8050539911803,-12.7040802804882,
117.542589474842)) ;
#189982=CARTESIAN_POINT('Ctrl Pts',(-10.7312501484571,-12.7040802781189,
117.56682051865)) ;
#189983=CARTESIAN_POINT('Ctrl Pts',(-10.6574463057339,-12.7040802757496,
117.591051562459)) ;
#189984=CARTESIAN_POINT('Ctrl Pts',(-10.6407645882193,-12.6502203483131,
117.540241742432)) ;
#189985=CARTESIAN_POINT('Ctrl Pts',(-10.6240828707046,-12.5963604208767,
117.489431922405)) ;
#189986=CARTESIAN_POINT('Ctrl Pts',(-10.6978867134277,-12.596360423246,
117.465200878597)) ;
#189987=CARTESIAN_POINT('Ctrl Pts',(-10.7716905561509,-12.5963604256153,
117.440969834788)) ;
#189988=CARTESIAN_POINT('Ctrl Pts',(-10.7883722736656,-12.6502203530517,
117.491779654815)) ;
#189989=CARTESIAN_POINT('Ctrl Pts',(-10.7226751288005,-12.8831101738135,
117.32729459891)) ;
#189990=CARTESIAN_POINT('Ctrl Pts',(-10.7432320047121,-12.9207872316337,
117.389907526118)) ;
#189991=CARTESIAN_POINT('Ctrl Pts',(-10.669428161409,-12.9207872305233,
117.41413856816)) ;
#189992=CARTESIAN_POINT('Ctrl Pts',(-10.5956243181059,-12.9207872294128,
117.438369610202)) ;
#189993=CARTESIAN_POINT('Ctrl Pts',(-10.5750674421944,-12.8831101715926,
117.375756682994)) ;
#189994=CARTESIAN_POINT('Ctrl Pts',(-10.5545105662828,-12.8454331137723,
117.313143755785)) ;
#189995=CARTESIAN_POINT('Ctrl Pts',(-10.6283144095859,-12.8454331148828,
117.288912713743)) ;
#189996=CARTESIAN_POINT('Ctrl Pts',(-10.702118252889,-12.8454331159932,
117.264681671701)) ;
#189997=CARTESIAN_POINT('Ctrl Pts',(-10.7226751288005,-12.8831101738135,
117.32729459891)) ;
#189998=CARTESIAN_POINT('Ctrl Pts',(-10.6785821123709,-13.1530763913863,
117.228387939344)) ;
#189999=CARTESIAN_POINT('Ctrl Pts',(-10.7015154333077,-13.1719578711027,
117.298239134592)) ;
#190000=CARTESIAN_POINT('Ctrl Pts',(-10.6277115895755,-13.1719578734333,
117.322470175327)) ;
#190001=CARTESIAN_POINT('Ctrl Pts',(-10.5539077458432,-13.1719578757638,
117.346701216061)) ;
#190002=CARTESIAN_POINT('Ctrl Pts',(-10.5309744249064,-13.1530763960474,
117.276850020814)) ;
#190003=CARTESIAN_POINT('Ctrl Pts',(-10.5080411039696,-13.134194916331,
117.206998825567)) ;
#190004=CARTESIAN_POINT('Ctrl Pts',(-10.5818449477019,-13.1341949140004,
117.182767784832)) ;
#190005=CARTESIAN_POINT('Ctrl Pts',(-10.6556487914341,-13.1341949116699,
117.158536744097)) ;
#190006=CARTESIAN_POINT('Ctrl Pts',(-10.6785821123709,-13.1530763913863,
117.228387939344)) ;
#190007=CARTESIAN_POINT('Ctrl Pts',(-10.6579116055234,-13.4431032907692,
117.20097789324)) ;
#190008=CARTESIAN_POINT('Ctrl Pts',(-10.6815861390285,-13.4417610754161,
117.273086702264)) ;
#190009=CARTESIAN_POINT('Ctrl Pts',(-10.6077822955129,-13.4417610837383,
117.297317743659)) ;
#190010=CARTESIAN_POINT('Ctrl Pts',(-10.5339784519973,-13.4417610920606,
117.321548785054)) ;
#190011=CARTESIAN_POINT('Ctrl Pts',(-10.5103039184922,-13.4431033074138,
117.24943997603)) ;
#190012=CARTESIAN_POINT('Ctrl Pts',(-10.486629384987,-13.4444455227669,
117.177331167006)) ;
#190013=CARTESIAN_POINT('Ctrl Pts',(-10.5604332285026,-13.4444455144446,
117.153100125611)) ;
#190014=CARTESIAN_POINT('Ctrl Pts',(-10.6342370720182,-13.4444455061224,
117.128869084216)) ;
#190015=CARTESIAN_POINT('Ctrl Pts',(-10.6579116055234,-13.4431032907692,
117.20097789324)) ;
#190016=CARTESIAN_POINT('Ctrl Pts',(-10.6616166491097,-13.7301505723016,
117.247656025822)) ;
#190017=CARTESIAN_POINT('Ctrl Pts',(-10.684334421916,-13.7087638139034,
117.316850696012)) ;
#190018=CARTESIAN_POINT('Ctrl Pts',(-10.6105305796162,-13.7087638278677,
117.34108174111)) ;
#190019=CARTESIAN_POINT('Ctrl Pts',(-10.5367267373163,-13.7087638418319,
117.365312786208)) ;
#190020=CARTESIAN_POINT('Ctrl Pts',(-10.5140089645101,-13.7301506002301,
117.296118116017)) ;
#190021=CARTESIAN_POINT('Ctrl Pts',(-10.4912911917038,-13.7515373586284,
117.226923445826)) ;
#190022=CARTESIAN_POINT('Ctrl Pts',(-10.5650950340036,-13.7515373446641,
117.202692400729)) ;
#190023=CARTESIAN_POINT('Ctrl Pts',(-10.6388988763035,-13.7515373306999,
117.178461355631)) ;
#190024=CARTESIAN_POINT('Ctrl Pts',(-10.6616166491097,-13.7301505723016,
117.247656025822)) ;
#190025=CARTESIAN_POINT('Ctrl Pts',(-10.6885692655636,-13.9953629945928,
117.365213136604)) ;
#190026=CARTESIAN_POINT('Ctrl Pts',(-10.708704220682,-13.9554274129798,
117.426540960711)) ;
#190027=CARTESIAN_POINT('Ctrl Pts',(-10.6349003807089,-13.9554274317702,
117.450772012895)) ;
#190028=CARTESIAN_POINT('Ctrl Pts',(-10.5610965407357,-13.9554274505607,
117.47500306508)) ;
#190029=CARTESIAN_POINT('Ctrl Pts',(-10.5409615856173,-13.9953630321736,
117.413675240973)) ;
#190030=CARTESIAN_POINT('Ctrl Pts',(-10.5208266304989,-14.0352986137866,
117.352347416867)) ;
#190031=CARTESIAN_POINT('Ctrl Pts',(-10.5946304704721,-14.0352985949962,
117.328116364682)) ;
#190032=CARTESIAN_POINT('Ctrl Pts',(-10.6684343104452,-14.0352985762058,
117.303885312498)) ;
#190033=CARTESIAN_POINT('Ctrl Pts',(-10.6885692655636,-13.9953629945928,
117.365213136604)) ;
#190034=CARTESIAN_POINT('Ctrl Pts',(-10.7360390503692,-14.2191243988368,
117.545218751564)) ;
#190035=CARTESIAN_POINT('Ctrl Pts',(-10.7521557686961,-14.1635077763497,
117.594307674595)) ;
#190036=CARTESIAN_POINT('Ctrl Pts',(-10.6783519318786,-14.1635077969098,
117.618538736391)) ;
#190037=CARTESIAN_POINT('Ctrl Pts',(-10.604548095061,-14.16350781747,117.642769798187)) ;
#190038=CARTESIAN_POINT('Ctrl Pts',(-10.5884313767342,-14.2191244399571,
117.593680875156)) ;
#190039=CARTESIAN_POINT('Ctrl Pts',(-10.5723146584073,-14.2747410624442,
117.544591952124)) ;
#190040=CARTESIAN_POINT('Ctrl Pts',(-10.6461184952249,-14.2747410418841,
117.520360890328)) ;
#190041=CARTESIAN_POINT('Ctrl Pts',(-10.7199223320424,-14.2747410213239,
117.496129828532)) ;
#190042=CARTESIAN_POINT('Ctrl Pts',(-10.7360390503692,-14.2191243988368,
117.545218751564)) ;
#190043=CARTESIAN_POINT('Ctrl Pts',(-10.8004224513246,-14.3863702551061,
117.77697919627)) ;
#190044=CARTESIAN_POINT('Ctrl Pts',(-10.8113293964078,-14.318995498507,
117.810199990393)) ;
#190045=CARTESIAN_POINT('Ctrl Pts',(-10.7375255639529,-14.3189955173641,
117.834431065477)) ;
#190046=CARTESIAN_POINT('Ctrl Pts',(-10.6637217314981,-14.3189955362211,
117.858662140561)) ;
#190047=CARTESIAN_POINT('Ctrl Pts',(-10.6528147864148,-14.3863702928201,
117.825441346437)) ;
#190048=CARTESIAN_POINT('Ctrl Pts',(-10.6419078413316,-14.4537450494192,
117.792220552313)) ;
#190049=CARTESIAN_POINT('Ctrl Pts',(-10.7157116737865,-14.4537450305621,
117.76798947723)) ;
#190050=CARTESIAN_POINT('Ctrl Pts',(-10.7895155062413,-14.4537450117051,
117.743758402146)) ;
#190051=CARTESIAN_POINT('Ctrl Pts',(-10.8004224513246,-14.3863702551061,
117.77697919627)) ;
#190052=CARTESIAN_POINT('Ctrl Pts',(-10.8752502952428,-14.4829184358348,
118.040206328883)) ;
#190053=CARTESIAN_POINT('Ctrl Pts',(-10.8802177774422,-14.408705819493,
118.055336477252)) ;
#190054=CARTESIAN_POINT('Ctrl Pts',(-10.8064139483773,-14.4087058298003,
118.079567562661)) ;
#190055=CARTESIAN_POINT('Ctrl Pts',(-10.7326101193124,-14.4087058401076,
118.10379864807)) ;
#190056=CARTESIAN_POINT('Ctrl Pts',(-10.727642637113,-14.4829184564494,
118.088668499701)) ;
#190057=CARTESIAN_POINT('Ctrl Pts',(-10.7226751549136,-14.5571310727912,
118.073538351333)) ;
#190058=CARTESIAN_POINT('Ctrl Pts',(-10.7964789839785,-14.5571310624839,
118.049307265924)) ;
#190059=CARTESIAN_POINT('Ctrl Pts',(-10.8702828130435,-14.5571310521766,
118.025076180515)) ;
#190060=CARTESIAN_POINT('Ctrl Pts',(-10.8752502952428,-14.4829184358348,
118.040206328883)) ;
#190061=CARTESIAN_POINT('Ctrl Pts',(-10.9554503612226,-14.5038609743369,
118.320003608547)) ;
#190062=CARTESIAN_POINT('Ctrl Pts',(-10.9540905544359,-14.4280787626501,
118.31586185539)) ;
#190063=CARTESIAN_POINT('Ctrl Pts',(-10.8802867285745,-14.4280787598768,
118.340092950556)) ;
#190064=CARTESIAN_POINT('Ctrl Pts',(-10.806482902713,-14.4280787571034,
118.364324045722)) ;
#190065=CARTESIAN_POINT('Ctrl Pts',(-10.8078427094997,-14.5038609687901,
118.36846579888)) ;
#190066=CARTESIAN_POINT('Ctrl Pts',(-10.8092025162864,-14.5796431804768,
118.372607552037)) ;
#190067=CARTESIAN_POINT('Ctrl Pts',(-10.8830063421479,-14.5796431832502,
118.34837645687)) ;
#190068=CARTESIAN_POINT('Ctrl Pts',(-10.9568101680093,-14.5796431860236,
118.324145361704)) ;
#190069=CARTESIAN_POINT('Ctrl Pts',(-10.9554503612226,-14.5038609743369,
118.320003608547)) ;
#190070=CARTESIAN_POINT('Ctrl Pts',(-11.0338946450071,-14.4469649885374,
118.594339392381)) ;
#190071=CARTESIAN_POINT('Ctrl Pts',(-11.0263233894398,-14.3750457551338,
118.571278568299)) ;
#190072=CARTESIAN_POINT('Ctrl Pts',(-10.9525195650589,-14.3750457349022,
118.595509667975)) ;
#190073=CARTESIAN_POINT('Ctrl Pts',(-10.878715740678,-14.3750457146707,
118.619740767651)) ;
#190074=CARTESIAN_POINT('Ctrl Pts',(-10.8862869962453,-14.4469649480743,
118.642801591733)) ;
#190075=CARTESIAN_POINT('Ctrl Pts',(-10.8938582518126,-14.5188841814779,
118.665862415815)) ;
#190076=CARTESIAN_POINT('Ctrl Pts',(-10.9676620761935,-14.5188842017095,
118.641631316139)) ;
#190077=CARTESIAN_POINT('Ctrl Pts',(-11.0414659005744,-14.518884221941,
118.617400216464)) ;
#190078=CARTESIAN_POINT('Ctrl Pts',(-11.0338946450071,-14.4469649885374,
118.594339392381)) ;
#190079=CARTESIAN_POINT('Ctrl Pts',(-11.1046254927112,-14.3162777489947,
118.845269515741)) ;
#190080=CARTESIAN_POINT('Ctrl Pts',(-11.0913705484774,-14.2533785894399,
118.804897092878)) ;
#190081=CARTESIAN_POINT('Ctrl Pts',(-11.0175667238931,-14.2533785490254,
118.829128191934)) ;
#190082=CARTESIAN_POINT('Ctrl Pts',(-10.9437628993088,-14.253378508611,
118.853359290991)) ;
#190083=CARTESIAN_POINT('Ctrl Pts',(-10.9570178435427,-14.3162776681657,
118.893731713853)) ;
#190084=CARTESIAN_POINT('Ctrl Pts',(-10.9702727877766,-14.3791768277205,
118.934104136716)) ;
#190085=CARTESIAN_POINT('Ctrl Pts',(-11.0440766123608,-14.379176868135,
118.90987303766)) ;
#190086=CARTESIAN_POINT('Ctrl Pts',(-11.1178804369451,-14.3791769085495,
118.885641938604)) ;
#190087=CARTESIAN_POINT('Ctrl Pts',(-11.1046254927112,-14.3162777489947,
118.845269515741)) ;
#190088=CARTESIAN_POINT('Ctrl Pts',(-11.1615630301732,-14.1213118802641,
119.054150344886)) ;
#190089=CARTESIAN_POINT('Ctrl Pts',(-11.1435799622605,-14.0719335115926,
118.999376820032)) ;
#190090=CARTESIAN_POINT('Ctrl Pts',(-11.0697761351519,-14.0719334508548,
119.0236079114)) ;
#190091=CARTESIAN_POINT('Ctrl Pts',(-10.9959723080433,-14.0719333901169,
119.047839002768)) ;
#190092=CARTESIAN_POINT('Ctrl Pts',(-11.013955375956,-14.1213117587884,
119.102612527621)) ;
#190093=CARTESIAN_POINT('Ctrl Pts',(-11.0319384438687,-14.1706901274599,
119.157386052474)) ;
#190094=CARTESIAN_POINT('Ctrl Pts',(-11.1057422709773,-14.1706901881977,
119.133154961106)) ;
#190095=CARTESIAN_POINT('Ctrl Pts',(-11.1795460980859,-14.1706902489356,
119.108923869739)) ;
#190096=CARTESIAN_POINT('Ctrl Pts',(-11.1615630301732,-14.1213118802641,
119.054150344886)) ;
#190097=CARTESIAN_POINT('Ctrl Pts',(-11.2000141105456,-13.8756723338256,
119.206771292959)) ;
#190098=CARTESIAN_POINT('Ctrl Pts',(-11.1785857096267,-13.8433718742573,
119.141503839532)) ;
#190099=CARTESIAN_POINT('Ctrl Pts',(-11.1047818778379,-13.8433717952861,
119.165734916645)) ;
#190100=CARTESIAN_POINT('Ctrl Pts',(-11.0309780460491,-13.8433717163149,
119.189965993757)) ;
#190101=CARTESIAN_POINT('Ctrl Pts',(-11.0524064469679,-13.8756721758832,
119.255233447184)) ;
#190102=CARTESIAN_POINT('Ctrl Pts',(-11.0738348478868,-13.9079726354515,
119.32050090061)) ;
#190103=CARTESIAN_POINT('Ctrl Pts',(-11.1476386796756,-13.9079727144228,
119.296269823498)) ;
#190104=CARTESIAN_POINT('Ctrl Pts',(-11.2214425114645,-13.907972793394,
119.272038746385)) ;
#190105=CARTESIAN_POINT('Ctrl Pts',(-11.2000141105456,-13.8756723338256,
119.206771292959)) ;
#190106=CARTESIAN_POINT('Ctrl Pts',(-11.2163100996261,-13.597140902686,
119.291910614714)) ;
#190107=CARTESIAN_POINT('Ctrl Pts',(-11.1929780886912,-13.584239435371,
119.220845072204)) ;
#190108=CARTESIAN_POINT('Ctrl Pts',(-11.1191742502117,-13.5842393431877,
119.245076128938)) ;
#190109=CARTESIAN_POINT('Ctrl Pts',(-11.0453704117322,-13.5842392510044,
119.269307185671)) ;
#190110=CARTESIAN_POINT('Ctrl Pts',(-11.068702422667,-13.5971407183194,
119.340372728181)) ;
#190111=CARTESIAN_POINT('Ctrl Pts',(-11.0920344336019,-13.6100421856345,
119.41143827069)) ;
#190112=CARTESIAN_POINT('Ctrl Pts',(-11.1658382720815,-13.6100422778178,
119.387207213956)) ;
#190113=CARTESIAN_POINT('Ctrl Pts',(-11.239642110561,-13.6100423700011,
119.362976157223)) ;
#190114=CARTESIAN_POINT('Ctrl Pts',(-11.2163100996261,-13.597140902686,
119.291910614714)) ;
#190115=CARTESIAN_POINT('Ctrl Pts',(-11.2087112550923,-13.3072582096283,
119.304089569254)) ;
#190116=CARTESIAN_POINT('Ctrl Pts',(-11.1851449455377,-13.3145766205793,
119.23231039087)) ;
#190117=CARTESIAN_POINT('Ctrl Pts',(-11.1113410991254,-13.3145765231922,
119.256541423441)) ;
#190118=CARTESIAN_POINT('Ctrl Pts',(-11.0375372527131,-13.3145764258051,
119.280772456013)) ;
#190119=CARTESIAN_POINT('Ctrl Pts',(-11.0611035622676,-13.3072580148542,
119.352551634397)) ;
#190120=CARTESIAN_POINT('Ctrl Pts',(-11.0846698718222,-13.2999396039032,
119.424330812782)) ;
#190121=CARTESIAN_POINT('Ctrl Pts',(-11.1584737182345,-13.2999397012903,
119.40009978021)) ;
#190122=CARTESIAN_POINT('Ctrl Pts',(-11.2322775646468,-13.2999397986774,
119.375868747639)) ;
#190123=CARTESIAN_POINT('Ctrl Pts',(-11.2087112550923,-13.3072582096283,
119.304089569254)) ;
#190124=CARTESIAN_POINT('Ctrl Pts',(-11.176929955516,-13.023884652308,119.242788774443)) ;
#190125=CARTESIAN_POINT('Ctrl Pts',(-11.1548134261834,-13.0509977629016,
119.175425392607)) ;
#190126=CARTESIAN_POINT('Ctrl Pts',(-11.0810095713045,-13.0509976674412,
119.199656399391)) ;
#190127=CARTESIAN_POINT('Ctrl Pts',(-11.0072057164255,-13.0509975719808,
119.223887406175)) ;
#190128=CARTESIAN_POINT('Ctrl Pts',(-11.0293222457582,-13.0238844613873,
119.29125078801)) ;
#190129=CARTESIAN_POINT('Ctrl Pts',(-11.0514387750908,-12.9967713507938,
119.358614169846)) ;
#190130=CARTESIAN_POINT('Ctrl Pts',(-11.1252426299697,-12.9967714462542,
119.334383163062)) ;
#190131=CARTESIAN_POINT('Ctrl Pts',(-11.1990464848487,-12.9967715417145,
119.310152156278)) ;
#190132=CARTESIAN_POINT('Ctrl Pts',(-11.176929955516,-13.023884652308,119.242788774443)) ;
#190133=CARTESIAN_POINT('Ctrl Pts',(-11.122465034715,-12.7690113233817,
119.112365611642)) ;
#190134=CARTESIAN_POINT('Ctrl Pts',(-11.1033846730978,-12.8139584952445,
119.054249906723)) ;
#190135=CARTESIAN_POINT('Ctrl Pts',(-11.0295808101122,-12.813958410504,
119.078480888815)) ;
#190136=CARTESIAN_POINT('Ctrl Pts',(-10.9557769471266,-12.8139583257634,
119.102711870907)) ;
#190137=CARTESIAN_POINT('Ctrl Pts',(-10.9748573087438,-12.7690111539007,
119.160827575826)) ;
#190138=CARTESIAN_POINT('Ctrl Pts',(-10.9939376703611,-12.7240639820379,
119.218943280745)) ;
#190139=CARTESIAN_POINT('Ctrl Pts',(-11.0677415333467,-12.7240640667784,
119.194712298653)) ;
#190140=CARTESIAN_POINT('Ctrl Pts',(-11.1415453963323,-12.724064151519,
119.170481316561)) ;
#190141=CARTESIAN_POINT('Ctrl Pts',(-11.122465034715,-12.7690113233817,
119.112365611642)) ;
#190142=CARTESIAN_POINT('Ctrl Pts',(-11.0484836538836,-12.5606194771078,
118.922504182192)) ;
#190143=CARTESIAN_POINT('Ctrl Pts',(-11.0338062707941,-12.6201819472302,
118.877799239411)) ;
#190144=CARTESIAN_POINT('Ctrl Pts',(-10.9600024009755,-12.6201818809856,
118.902030200691)) ;
#190145=CARTESIAN_POINT('Ctrl Pts',(-10.8861985311569,-12.620181814741,
118.92626116197)) ;
#190146=CARTESIAN_POINT('Ctrl Pts',(-10.9008759142464,-12.5606193446187,
118.970966104751)) ;
#190147=CARTESIAN_POINT('Ctrl Pts',(-10.9155532973358,-12.5010568744963,
119.015671047533)) ;
#190148=CARTESIAN_POINT('Ctrl Pts',(-10.9893571671545,-12.5010569407409,
118.991440086253)) ;
#190149=CARTESIAN_POINT('Ctrl Pts',(-11.0631610369731,-12.5010570069855,
118.967209124973)) ;
#190150=CARTESIAN_POINT('Ctrl Pts',(-11.0484836538836,-12.5606194771078,
118.922504182192)) ;
#190151=CARTESIAN_POINT('Ctrl Pts',(-10.9596194230083,-12.413760463827,
118.687278216149)) ;
#190152=CARTESIAN_POINT('Ctrl Pts',(-10.9503912303216,-12.4836640016496,
118.659170628094)) ;
#190153=CARTESIAN_POINT('Ctrl Pts',(-10.8765873557,-12.4836639599655,118.683401574745)) ;
#190154=CARTESIAN_POINT('Ctrl Pts',(-10.8027834810785,-12.4836639182814,
118.707632521395)) ;
#190155=CARTESIAN_POINT('Ctrl Pts',(-10.8120116737651,-12.4137603804588,
118.73574010945)) ;
#190156=CARTESIAN_POINT('Ctrl Pts',(-10.8212398664518,-12.3438568426362,
118.763847697506)) ;
#190157=CARTESIAN_POINT('Ctrl Pts',(-10.8950437410734,-12.3438568843203,
118.739616750855)) ;
#190158=CARTESIAN_POINT('Ctrl Pts',(-10.968847615695,-12.3438569260044,
118.715385804204)) ;
#190159=CARTESIAN_POINT('Ctrl Pts',(-10.9596194230083,-12.413760463827,
118.687278216149)) ;
#190160=CARTESIAN_POINT('Ctrl Pts',(-10.861301775566,-12.3386970972896,
118.42329982477)) ;
#190161=CARTESIAN_POINT('Ctrl Pts',(-10.8581899088794,-12.4139449164538,
118.41382157885)) ;
#190162=CARTESIAN_POINT('Ctrl Pts',(-10.7843860319931,-12.4139449029389,
118.438052518602)) ;
#190163=CARTESIAN_POINT('Ctrl Pts',(-10.7105821551067,-12.4139448894239,
118.462283458355)) ;
#190164=CARTESIAN_POINT('Ctrl Pts',(-10.7136940217933,-12.3386970702597,
118.471761704275)) ;
#190165=CARTESIAN_POINT('Ctrl Pts',(-10.71680588848,-12.2634492510955,118.481239950195)) ;
#190166=CARTESIAN_POINT('Ctrl Pts',(-10.7906097653663,-12.2634492646105,
118.457009010442)) ;
#190167=CARTESIAN_POINT('Ctrl Pts',(-10.8644136422527,-12.2634492781254,
118.43277807069)) ;
#190168=CARTESIAN_POINT('Ctrl Pts',(-10.861301775566,-12.3386970972896,
118.42329982477)) ;
#190169=CARTESIAN_POINT('Ctrl Pts',(-10.7600017865258,-12.3409867725706,
118.150207238855)) ;
#190170=CARTESIAN_POINT('Ctrl Pts',(-10.7632241796794,-12.4161865646984,
118.160022126406)) ;
#190171=CARTESIAN_POINT('Ctrl Pts',(-10.6894203032958,-12.4161865800311,
118.18425306769)) ;
#190172=CARTESIAN_POINT('Ctrl Pts',(-10.6156164269123,-12.4161865953639,
118.208484008974)) ;
#190173=CARTESIAN_POINT('Ctrl Pts',(-10.6123940337586,-12.3409868032361,
118.198669121423)) ;
#190174=CARTESIAN_POINT('Ctrl Pts',(-10.609171640605,-12.2657870111083,
118.188854233873)) ;
#190175=CARTESIAN_POINT('Ctrl Pts',(-10.6829755169886,-12.2657869957756,
118.164623292589)) ;
#190176=CARTESIAN_POINT('Ctrl Pts',(-10.7567793933721,-12.2657869804429,
118.140392351305)) ;
#190177=CARTESIAN_POINT('Ctrl Pts',(-10.7600017865258,-12.3409867725706,
118.150207238855)) ;
#190178=CARTESIAN_POINT('Ctrl Pts',(-10.6620478041179,-12.4204578395528,
117.88734093994)) ;
#190179=CARTESIAN_POINT('Ctrl Pts',(-10.6713795731896,-12.4902214392955,
117.915764000842)) ;
#190180=CARTESIAN_POINT('Ctrl Pts',(-10.5975756999991,-12.4902214812087,
117.939994951852)) ;
#190181=CARTESIAN_POINT('Ctrl Pts',(-10.5237718268086,-12.4902215231219,
117.964225902861)) ;
#190182=CARTESIAN_POINT('Ctrl Pts',(-10.514440057737,-12.4204579233792,
117.93580284196)) ;
#190183=CARTESIAN_POINT('Ctrl Pts',(-10.5051082886654,-12.3506943236366,
117.907379781058)) ;
#190184=CARTESIAN_POINT('Ctrl Pts',(-10.5789121618558,-12.3506942817234,
117.883148830048)) ;
#190185=CARTESIAN_POINT('Ctrl Pts',(-10.6527160350463,-12.3506942398102,
117.858917879039)) ;
#190186=CARTESIAN_POINT('Ctrl Pts',(-10.6620478041179,-12.4204578395528,
117.88734093994)) ;
#190187=CARTESIAN_POINT('Ctrl Pts',(-10.573847688419,-12.5714299256093,
117.654168216919)) ;
#190188=CARTESIAN_POINT('Ctrl Pts',(-10.5886173544689,-12.6307574701192,
117.699154234686)) ;
#190189=CARTESIAN_POINT('Ctrl Pts',(-10.514813486715,-12.6307575336333,
117.723385202254)) ;
#190190=CARTESIAN_POINT('Ctrl Pts',(-10.441009618961,-12.6307575971475,
117.747616169822)) ;
#190191=CARTESIAN_POINT('Ctrl Pts',(-10.4262399529111,-12.5714300526376,
117.702630152056)) ;
#190192=CARTESIAN_POINT('Ctrl Pts',(-10.4114702868613,-12.5121025081277,
117.65764413429)) ;
#190193=CARTESIAN_POINT('Ctrl Pts',(-10.4852741546152,-12.5121024446135,
117.633413166721)) ;
#190194=CARTESIAN_POINT('Ctrl Pts',(-10.5590780223691,-12.5121023810993,
117.609182199153)) ;
#190195=CARTESIAN_POINT('Ctrl Pts',(-10.573847688419,-12.5714299256093,
117.654168216919)) ;
#190196=CARTESIAN_POINT('Ctrl Pts',(-10.5009899435521,-12.7828129113163,
117.467691180829)) ;
#190197=CARTESIAN_POINT('Ctrl Pts',(-10.520135271516,-12.8274711161602,
117.526004758861)) ;
#190198=CARTESIAN_POINT('Ctrl Pts',(-10.446331410711,-12.82747119449,117.550235747595)) ;
#190199=CARTESIAN_POINT('Ctrl Pts',(-10.3725275499061,-12.8274712728199,
117.574466736329)) ;
#190200=CARTESIAN_POINT('Ctrl Pts',(-10.3533822219422,-12.782813067976,
117.516153158297)) ;
#190201=CARTESIAN_POINT('Ctrl Pts',(-10.3342368939783,-12.7381548631321,
117.457839580264)) ;
#190202=CARTESIAN_POINT('Ctrl Pts',(-10.4080407547832,-12.7381547848022,
117.43360859153)) ;
#190203=CARTESIAN_POINT('Ctrl Pts',(-10.4818446155882,-12.7381547064724,
117.409377602796)) ;
#190204=CARTESIAN_POINT('Ctrl Pts',(-10.5009899435521,-12.7828129113163,
117.467691180829)) ;
#190205=CARTESIAN_POINT('Ctrl Pts',(-10.4477866958819,-13.0396896566704,
117.341091891166)) ;
#190206=CARTESIAN_POINT('Ctrl Pts',(-10.4699418299774,-13.0664804040034,
117.40857285315)) ;
#190207=CARTESIAN_POINT('Ctrl Pts',(-10.3961379769048,-13.0664804892966,
117.432803865435)) ;
#190208=CARTESIAN_POINT('Ctrl Pts',(-10.3223341238321,-13.0664805745898,
117.457034877721)) ;
#190209=CARTESIAN_POINT('Ctrl Pts',(-10.3001789897366,-13.0396898272568,
117.389553915737)) ;
#190210=CARTESIAN_POINT('Ctrl Pts',(-10.278023855641,-13.0128990799238,
117.322072953753)) ;
#190211=CARTESIAN_POINT('Ctrl Pts',(-10.3518277087136,-13.0128989946306,
117.297841941468)) ;
#190212=CARTESIAN_POINT('Ctrl Pts',(-10.4256315617863,-13.0128989093375,
117.273610929183)) ;
#190213=CARTESIAN_POINT('Ctrl Pts',(-10.4477866958819,-13.0396896566704,
117.341091891166)) ;
#190214=CARTESIAN_POINT('Ctrl Pts',(-10.4173299629953,-13.3246405733811,
117.283892429125)) ;
#190215=CARTESIAN_POINT('Ctrl Pts',(-10.4409090851197,-13.3315770270648,
117.355710629024)) ;
#190216=CARTESIAN_POINT('Ctrl Pts',(-10.3671052396779,-13.331577110356,
117.379941664552)) ;
#190217=CARTESIAN_POINT('Ctrl Pts',(-10.2933013942362,-13.3315771936471,
117.40417270008)) ;
#190218=CARTESIAN_POINT('Ctrl Pts',(-10.2697222721119,-13.3246407399634,
117.332354500181)) ;
#190219=CARTESIAN_POINT('Ctrl Pts',(-10.2461431499876,-13.3177042862798,
117.260536300282)) ;
#190220=CARTESIAN_POINT('Ctrl Pts',(-10.3199469954293,-13.3177042029886,
117.236305264754)) ;
#190221=CARTESIAN_POINT('Ctrl Pts',(-10.393750840871,-13.3177041196975,
117.212074229227)) ;
#190222=CARTESIAN_POINT('Ctrl Pts',(-10.4173299629953,-13.3246405733811,
117.283892429125)) ;
#190223=CARTESIAN_POINT('Ctrl Pts',(-10.4112128032642,-13.6149949699245,
117.300663470431)) ;
#190224=CARTESIAN_POINT('Ctrl Pts',(-10.4345220214507,-13.6016695488901,
117.371659586614)) ;
#190225=CARTESIAN_POINT('Ctrl Pts',(-10.3607181825812,-13.6016696242958,
117.39589064216)) ;
#190226=CARTESIAN_POINT('Ctrl Pts',(-10.2869143437116,-13.6016696997014,
117.420121697705)) ;
#190227=CARTESIAN_POINT('Ctrl Pts',(-10.2636051255251,-13.6149951207358,
117.349125581522)) ;
#190228=CARTESIAN_POINT('Ctrl Pts',(-10.2402959073386,-13.6283205417703,
117.278129465339)) ;
#190229=CARTESIAN_POINT('Ctrl Pts',(-10.3140997462082,-13.6283204663646,
117.253898409794)) ;
#190230=CARTESIAN_POINT('Ctrl Pts',(-10.3879035850777,-13.6283203909589,
117.229667354248)) ;
#190231=CARTESIAN_POINT('Ctrl Pts',(-10.4112128032642,-13.6149949699245,
117.300663470431)) ;
#190232=CARTESIAN_POINT('Ctrl Pts',(-10.4289381058465,-13.8916396903177,
117.39010694689)) ;
#190233=CARTESIAN_POINT('Ctrl Pts',(-10.4503113588195,-13.8589788645426,
117.455206425549)) ;
#190234=CARTESIAN_POINT('Ctrl Pts',(-10.3765075249951,-13.8589789264578,
117.479437496461)) ;
#190235=CARTESIAN_POINT('Ctrl Pts',(-10.3027036911708,-13.858978988373,
117.503668567374)) ;
#190236=CARTESIAN_POINT('Ctrl Pts',(-10.2813304381978,-13.891639814148,
117.438569088715)) ;
#190237=CARTESIAN_POINT('Ctrl Pts',(-10.2599571852247,-13.9243006399231,
117.373469610057)) ;
#190238=CARTESIAN_POINT('Ctrl Pts',(-10.3337610190491,-13.9243005780079,
117.349238539144)) ;
#190239=CARTESIAN_POINT('Ctrl Pts',(-10.4075648528735,-13.9243005160927,
117.325007468232)) ;
#190240=CARTESIAN_POINT('Ctrl Pts',(-10.4289381058465,-13.8916396903177,
117.39010694689)) ;
#190241=CARTESIAN_POINT('Ctrl Pts',(-10.468506753606,-14.1343825887975,
117.546066895377)) ;
#190242=CARTESIAN_POINT('Ctrl Pts',(-10.4864163346107,-14.0847239411806,
117.600616588237)) ;
#190243=CARTESIAN_POINT('Ctrl Pts',(-10.4126125039408,-14.0847239865753,
117.624847668757)) ;
#190244=CARTESIAN_POINT('Ctrl Pts',(-10.3388086732709,-14.0847240319701,
117.649078749278)) ;
#190245=CARTESIAN_POINT('Ctrl Pts',(-10.3208990922662,-14.134382679587,
117.594529056418)) ;
#190246=CARTESIAN_POINT('Ctrl Pts',(-10.3029895112616,-14.1840413272039,
117.539979363559)) ;
#190247=CARTESIAN_POINT('Ctrl Pts',(-10.3767933419314,-14.1840412818091,
117.515748283038)) ;
#190248=CARTESIAN_POINT('Ctrl Pts',(-10.4505971726013,-14.1840412364144,
117.491517202517)) ;
#190249=CARTESIAN_POINT('Ctrl Pts',(-10.468506753606,-14.1343825887975,
117.546066895377)) ;
#190250=CARTESIAN_POINT('Ctrl Pts',(-10.5266399323651,-14.3263844089833,
117.758714791445)) ;
#190251=CARTESIAN_POINT('Ctrl Pts',(-10.539781502399,-14.2632443878997,
117.798741892392)) ;
#190252=CARTESIAN_POINT('Ctrl Pts',(-10.4659776724899,-14.263244415508,
117.82297297523)) ;
#190253=CARTESIAN_POINT('Ctrl Pts',(-10.3921738425808,-14.2632444431164,
117.847204058068)) ;
#190254=CARTESIAN_POINT('Ctrl Pts',(-10.3790322725469,-14.3263844642,117.807176957121)) ;
#190255=CARTESIAN_POINT('Ctrl Pts',(-10.3658907025129,-14.3895244852836,
117.767149856173)) ;
#190256=CARTESIAN_POINT('Ctrl Pts',(-10.439694532422,-14.3895244576753,
117.742918773336)) ;
#190257=CARTESIAN_POINT('Ctrl Pts',(-10.5134983623311,-14.3895244300669,
117.718687690498)) ;
#190258=CARTESIAN_POINT('Ctrl Pts',(-10.5266399323651,-14.3263844089833,
117.758714791445)) ;
#190259=CARTESIAN_POINT('Ctrl Pts',(-10.5977223470439,-14.4524065463604,
118.010565142517)) ;
#190260=CARTESIAN_POINT('Ctrl Pts',(-10.6051893156736,-14.3803719566858,
118.033308323326)) ;
#190261=CARTESIAN_POINT('Ctrl Pts',(-10.5313854853145,-14.3803719694669,
118.057539404794)) ;
#190262=CARTESIAN_POINT('Ctrl Pts',(-10.4575816549555,-14.3803719822481,
118.081770486261)) ;
#190263=CARTESIAN_POINT('Ctrl Pts',(-10.4501146863257,-14.4524065719227,
118.059027305451)) ;
#190264=CARTESIAN_POINT('Ctrl Pts',(-10.442647717696,-14.5244411615974,
118.036284124642)) ;
#190265=CARTESIAN_POINT('Ctrl Pts',(-10.5164515480551,-14.5244411488162,
118.012053043175)) ;
#190266=CARTESIAN_POINT('Ctrl Pts',(-10.5902553784142,-14.5244411360351,
117.987821961707)) ;
#190267=CARTESIAN_POINT('Ctrl Pts',(-10.5977223470439,-14.4524065463604,
118.010565142517)) ;
#190268=CARTESIAN_POINT('Ctrl Pts',(-10.6769157709103,-14.5048820459499,
118.287401592442)) ;
#190269=CARTESIAN_POINT('Ctrl Pts',(-10.6781273667279,-14.4290737092712,
118.291091917164)) ;
#190270=CARTESIAN_POINT('Ctrl Pts',(-10.6043235337896,-14.4290737099999,
118.315322990775)) ;
#190271=CARTESIAN_POINT('Ctrl Pts',(-10.5305197008513,-14.4290737107285,
118.339554064386)) ;
#190272=CARTESIAN_POINT('Ctrl Pts',(-10.5293081050337,-14.5048820474072,
118.335863739665)) ;
#190273=CARTESIAN_POINT('Ctrl Pts',(-10.5280965092161,-14.5806903840858,
118.332173414943)) ;
#190274=CARTESIAN_POINT('Ctrl Pts',(-10.6019003421544,-14.5806903833572,
118.307942341331)) ;
#190275=CARTESIAN_POINT('Ctrl Pts',(-10.6757041750927,-14.5806903826285,
118.28371126772)) ;
#190276=CARTESIAN_POINT('Ctrl Pts',(-10.6769157709103,-14.5048820459499,
118.287401592442)) ;
#190277=CARTESIAN_POINT('Ctrl Pts',(-10.7565713057278,-14.4792643387988,
118.565341880977)) ;
#190278=CARTESIAN_POINT('Ctrl Pts',(-10.7514919843651,-14.4051302441696,
118.549871087139)) ;
#190279=CARTESIAN_POINT('Ctrl Pts',(-10.6776881489865,-14.4051302376983,
118.574102153317)) ;
#190280=CARTESIAN_POINT('Ctrl Pts',(-10.603884313608,-14.405130231227,118.598333219496)) ;
#190281=CARTESIAN_POINT('Ctrl Pts',(-10.6089636349707,-14.4792643258562,
118.613804013335)) ;
#190282=CARTESIAN_POINT('Ctrl Pts',(-10.6140429563333,-14.5533984204853,
118.629274807173)) ;
#190283=CARTESIAN_POINT('Ctrl Pts',(-10.6878467917119,-14.5533984269566,
118.605043740994)) ;
#190284=CARTESIAN_POINT('Ctrl Pts',(-10.7616506270905,-14.5533984334279,
118.580812674816)) ;
#190285=CARTESIAN_POINT('Ctrl Pts',(-10.7565713057278,-14.4792643387988,
118.565341880977)) ;
#190286=CARTESIAN_POINT('Ctrl Pts',(-10.8312394732339,-14.3777623982077,
118.828257574301)) ;
#190287=CARTESIAN_POINT('Ctrl Pts',(-10.8202044172732,-14.3106033154662,
118.794646573987)) ;
#190288=CARTESIAN_POINT('Ctrl Pts',(-10.7464005788549,-14.3106033061414,
118.818877630907)) ;
#190289=CARTESIAN_POINT('Ctrl Pts',(-10.6725967404366,-14.3106032968165,
118.843108687828)) ;
#190290=CARTESIAN_POINT('Ctrl Pts',(-10.6836317963974,-14.377762379558,
118.876719688142)) ;
#190291=CARTESIAN_POINT('Ctrl Pts',(-10.6946668523581,-14.4449214622994,
118.910330688456)) ;
#190292=CARTESIAN_POINT('Ctrl Pts',(-10.7684706907764,-14.4449214716243,
118.886099631536)) ;
#190293=CARTESIAN_POINT('Ctrl Pts',(-10.8422745291946,-14.4449214809491,
118.861868574615)) ;
#190294=CARTESIAN_POINT('Ctrl Pts',(-10.8312394732339,-14.3777623982077,
118.828257574301)) ;
#190295=CARTESIAN_POINT('Ctrl Pts',(-10.8943486068065,-14.2077004202751,
119.055900281951)) ;
#190296=CARTESIAN_POINT('Ctrl Pts',(-10.8781572711893,-14.1523145589373,
119.006584085897)) ;
#190297=CARTESIAN_POINT('Ctrl Pts',(-10.8043534303052,-14.1523145504394,
119.030815135306)) ;
#190298=CARTESIAN_POINT('Ctrl Pts',(-10.7305495894211,-14.1523145419415,
119.055046184716)) ;
#190299=CARTESIAN_POINT('Ctrl Pts',(-10.7467409250382,-14.2077004032793,
119.10436238077)) ;
#190300=CARTESIAN_POINT('Ctrl Pts',(-10.7629322606553,-14.2630862646171,
119.153678576825)) ;
#190301=CARTESIAN_POINT('Ctrl Pts',(-10.8367361015395,-14.2630862731151,
119.129447527415)) ;
#190302=CARTESIAN_POINT('Ctrl Pts',(-10.9105399424236,-14.263086281613,
119.105216478005)) ;
#190303=CARTESIAN_POINT('Ctrl Pts',(-10.8943486068065,-14.2077004202751,
119.055900281951)) ;
#190304=CARTESIAN_POINT('Ctrl Pts',(-10.9409131008362,-13.980362420234,
119.23327739182)) ;
#190305=CARTESIAN_POINT('Ctrl Pts',(-10.9207102013615,-13.9407671671798,
119.171742619647)) ;
#190306=CARTESIAN_POINT('Ctrl Pts',(-10.8469063586303,-13.9407671625387,
119.195973663431)) ;
#190307=CARTESIAN_POINT('Ctrl Pts',(-10.7731025158991,-13.9407671578977,
119.220204707215)) ;
#190308=CARTESIAN_POINT('Ctrl Pts',(-10.7933054153738,-13.980362410952,
119.281739479387)) ;
#190309=CARTESIAN_POINT('Ctrl Pts',(-10.8135083148485,-14.0199576640062,
119.34327425156)) ;
#190310=CARTESIAN_POINT('Ctrl Pts',(-10.8873121575797,-14.0199576686472,
119.319043207776)) ;
#190311=CARTESIAN_POINT('Ctrl Pts',(-10.9611160003109,-14.0199576732883,
119.294812163993)) ;
#190312=CARTESIAN_POINT('Ctrl Pts',(-10.9409131008362,-13.980362420234,
119.23327739182)) ;
#190313=CARTESIAN_POINT('Ctrl Pts',(-10.9665178595046,-13.7128487430244,
119.346765660867)) ;
#190314=CARTESIAN_POINT('Ctrl Pts',(-10.9437620232542,-13.6918738812675,
119.277455055282)) ;
#190315=CARTESIAN_POINT('Ctrl Pts',(-10.8699581797813,-13.6918738808366,
119.301686096807)) ;
#190316=CARTESIAN_POINT('Ctrl Pts',(-10.7961543363084,-13.6918738804057,
119.325917138332)) ;
#190317=CARTESIAN_POINT('Ctrl Pts',(-10.8189101725589,-13.7128487421626,
119.395227743917)) ;
#190318=CARTESIAN_POINT('Ctrl Pts',(-10.8416660088093,-13.7338236039195,
119.464538349502)) ;
#190319=CARTESIAN_POINT('Ctrl Pts',(-10.9154698522822,-13.7338236043504,
119.440307307977)) ;
#190320=CARTESIAN_POINT('Ctrl Pts',(-10.9892736957551,-13.7338236047813,
119.416076266453)) ;
#190321=CARTESIAN_POINT('Ctrl Pts',(-10.9665178595046,-13.7128487430244,
119.346765660867)) ;
#190322=CARTESIAN_POINT('Ctrl Pts',(-10.9686843945112,-13.4250762896625,
119.388764927315)) ;
#190323=CARTESIAN_POINT('Ctrl Pts',(-10.9450107520713,-13.4241646281582,
119.316658832214)) ;
#190324=CARTESIAN_POINT('Ctrl Pts',(-10.8712069085982,-13.424164630414,
119.340889873738)) ;
#190325=CARTESIAN_POINT('Ctrl Pts',(-10.7974030651251,-13.4241646326699,
119.365120915263)) ;
#190326=CARTESIAN_POINT('Ctrl Pts',(-10.821076707565,-13.4250762941742,
119.437227010363)) ;
#190327=CARTESIAN_POINT('Ctrl Pts',(-10.844750350005,-13.4259879556785,
119.509333105464)) ;
#190328=CARTESIAN_POINT('Ctrl Pts',(-10.9185541934781,-13.4259879534226,
119.48510206394)) ;
#190329=CARTESIAN_POINT('Ctrl Pts',(-10.9923580369512,-13.4259879511667,
119.460871022416)) ;
#190330=CARTESIAN_POINT('Ctrl Pts',(-10.9686843945112,-13.4250762896625,
119.388764927315)) ;
#190331=CARTESIAN_POINT('Ctrl Pts',(-10.9467663089628,-13.1369898154444,
119.357371205815)) ;
#190332=CARTESIAN_POINT('Ctrl Pts',(-10.92385617065,-13.1561933535751,119.28759062112)) ;
#190333=CARTESIAN_POINT('Ctrl Pts',(-10.8500523275358,-13.1561933570076,
119.311821663738)) ;
#190334=CARTESIAN_POINT('Ctrl Pts',(-10.7762484844217,-13.15619336044,119.336052706355)) ;
#190335=CARTESIAN_POINT('Ctrl Pts',(-10.7991586227345,-13.1369898223093,
119.40583329105)) ;
#190336=CARTESIAN_POINT('Ctrl Pts',(-10.8220687610474,-13.1177862841786,
119.475613875745)) ;
#190337=CARTESIAN_POINT('Ctrl Pts',(-10.8958726041615,-13.1177862807461,
119.451382833128)) ;
#190338=CARTESIAN_POINT('Ctrl Pts',(-10.9696764472756,-13.1177862773137,
119.42715179051)) ;
#190339=CARTESIAN_POINT('Ctrl Pts',(-10.9467663089628,-13.1369898154444,
119.357371205815)) ;
#190340=CARTESIAN_POINT('Ctrl Pts',(-10.9008150940902,-12.8663855366991,
119.253146965752)) ;
#190341=CARTESIAN_POINT('Ctrl Pts',(-10.8803401623047,-12.9045144387046,
119.190783627186)) ;
#190342=CARTESIAN_POINT('Ctrl Pts',(-10.8065363192358,-12.9045144401406,
119.215014669941)) ;
#190343=CARTESIAN_POINT('Ctrl Pts',(-10.732732476167,-12.9045144415766,
119.239245712697)) ;
#190344=CARTESIAN_POINT('Ctrl Pts',(-10.7532074079525,-12.8663855395711,
119.301609051263)) ;
#190345=CARTESIAN_POINT('Ctrl Pts',(-10.7736823397381,-12.8282566375656,
119.36397238983)) ;
#190346=CARTESIAN_POINT('Ctrl Pts',(-10.8474861828069,-12.8282566361296,
119.339741347074)) ;
#190347=CARTESIAN_POINT('Ctrl Pts',(-10.9212900258757,-12.8282566346936,
119.315510304319)) ;
#190348=CARTESIAN_POINT('Ctrl Pts',(-10.9008150940902,-12.8663855366991,
119.253146965752)) ;
#190349=CARTESIAN_POINT('Ctrl Pts',(-10.8345412319917,-12.6384940512534,
119.086571197061)) ;
#190350=CARTESIAN_POINT('Ctrl Pts',(-10.817933850772,-12.6925911695923,
119.035987793437)) ;
#190351=CARTESIAN_POINT('Ctrl Pts',(-10.7441300072107,-12.6925911686239,
119.060218834692)) ;
#190352=CARTESIAN_POINT('Ctrl Pts',(-10.6703261636495,-12.6925911676555,
119.084449875948)) ;
#190353=CARTESIAN_POINT('Ctrl Pts',(-10.6869335448692,-12.6384940493165,
119.135033279572)) ;
#190354=CARTESIAN_POINT('Ctrl Pts',(-10.7035409260888,-12.5843969309776,
119.185616683196)) ;
#190355=CARTESIAN_POINT('Ctrl Pts',(-10.7773447696501,-12.584396931946,
119.16138564194)) ;
#190356=CARTESIAN_POINT('Ctrl Pts',(-10.8511486132114,-12.5843969329144,
119.137154600685)) ;
#190357=CARTESIAN_POINT('Ctrl Pts',(-10.8345412319917,-12.6384940512534,
119.086571197061)) ;
#190358=CARTESIAN_POINT('Ctrl Pts',(-10.7508843645138,-12.4647340958094,
118.867309476952)) ;
#190359=CARTESIAN_POINT('Ctrl Pts',(-10.7393585365561,-12.5310434351584,
118.832203664559)) ;
#190360=CARTESIAN_POINT('Ctrl Pts',(-10.6655546915337,-12.5310434317377,
118.856434701364)) ;
#190361=CARTESIAN_POINT('Ctrl Pts',(-10.5917508465113,-12.5310434283171,
118.880665738169)) ;
#190362=CARTESIAN_POINT('Ctrl Pts',(-10.603276674469,-12.4647340889681,
118.915771550563)) ;
#190363=CARTESIAN_POINT('Ctrl Pts',(-10.6148025024268,-12.3984247496191,
118.950877362956)) ;
#190364=CARTESIAN_POINT('Ctrl Pts',(-10.6886063474492,-12.3984247530398,
118.926646326151)) ;
#190365=CARTESIAN_POINT('Ctrl Pts',(-10.7624101924716,-12.3984247564605,
118.902415289346)) ;
#190366=CARTESIAN_POINT('Ctrl Pts',(-10.7508843645138,-12.4647340958094,
118.867309476952)) ;
#190367=CARTESIAN_POINT('Ctrl Pts',(-10.65582614901,-12.3600064377204,118.613172394745)) ;
#190368=CARTESIAN_POINT('Ctrl Pts',(-10.6501884550795,-12.4337245690079,
118.59600088844)) ;
#190369=CARTESIAN_POINT('Ctrl Pts',(-10.5763846080915,-12.4337245657129,
118.620231919259)) ;
#190370=CARTESIAN_POINT('Ctrl Pts',(-10.5025807611034,-12.4337245624179,
118.644462950077)) ;
#190371=CARTESIAN_POINT('Ctrl Pts',(-10.5082184550339,-12.3600064311304,
118.661634456381)) ;
#190372=CARTESIAN_POINT('Ctrl Pts',(-10.5138561489644,-12.286288299843,
118.678805962685)) ;
#190373=CARTESIAN_POINT('Ctrl Pts',(-10.5876599959525,-12.286288303138,
118.654574931867)) ;
#190374=CARTESIAN_POINT('Ctrl Pts',(-10.6614638429405,-12.286288306433,
118.630343901049)) ;
#190375=CARTESIAN_POINT('Ctrl Pts',(-10.65582614901,-12.3600064377204,118.613172394745)) ;
#190376=CARTESIAN_POINT('Ctrl Pts',(-10.5550274625865,-12.3305764766961,
118.341594134656)) ;
#190377=CARTESIAN_POINT('Ctrl Pts',(-10.5556862943649,-12.4064564353267,
118.343600829588)) ;
#190378=CARTESIAN_POINT('Ctrl Pts',(-10.4818824450957,-12.4064564352426,
118.367831853458)) ;
#190379=CARTESIAN_POINT('Ctrl Pts',(-10.4080785958265,-12.4064564351584,
118.392062877328)) ;
#190380=CARTESIAN_POINT('Ctrl Pts',(-10.4074197640481,-12.3305764765278,
118.390056182396)) ;
#190381=CARTESIAN_POINT('Ctrl Pts',(-10.4067609322696,-12.2546965178971,
118.388049487464)) ;
#190382=CARTESIAN_POINT('Ctrl Pts',(-10.4805647815389,-12.2546965179813,
118.363818463594)) ;
#190383=CARTESIAN_POINT('Ctrl Pts',(-10.5543686308081,-12.2546965180655,
118.339587439724)) ;
#190384=CARTESIAN_POINT('Ctrl Pts',(-10.5550274625865,-12.3305764766961,
118.341594134656)) ;
#190385=CARTESIAN_POINT('Ctrl Pts',(-10.4547480010087,-12.3793274592069,
118.071699282546)) ;
#190386=CARTESIAN_POINT('Ctrl Pts',(-10.4616740800548,-12.4519136571081,
118.092795001273)) ;
#190387=CARTESIAN_POINT('Ctrl Pts',(-10.3878702284318,-12.4519136645641,
118.117026017974)) ;
#190388=CARTESIAN_POINT('Ctrl Pts',(-10.3140663768089,-12.4519136720201,
118.141257034675)) ;
#190389=CARTESIAN_POINT('Ctrl Pts',(-10.3071402977628,-12.379327474119,
118.120161315948)) ;
#190390=CARTESIAN_POINT('Ctrl Pts',(-10.3002142187167,-12.3067412762178,
118.099065597221)) ;
#190391=CARTESIAN_POINT('Ctrl Pts',(-10.3740180703397,-12.3067412687618,
118.07483458052)) ;
#190392=CARTESIAN_POINT('Ctrl Pts',(-10.4478219219626,-12.3067412613058,
118.050603563819)) ;
#190393=CARTESIAN_POINT('Ctrl Pts',(-10.4547480010087,-12.3793274592069,
118.071699282546)) ;
#190394=CARTESIAN_POINT('Ctrl Pts',(-10.3621291537513,-12.5020990421703,
117.824980763251)) ;
#190395=CARTESIAN_POINT('Ctrl Pts',(-10.3747997470748,-12.5662179845147,
117.863573345446)) ;
#190396=CARTESIAN_POINT('Ctrl Pts',(-10.3009958943635,-12.5662180028208,
117.887804358831)) ;
#190397=CARTESIAN_POINT('Ctrl Pts',(-10.2271920416521,-12.5662180211268,
117.912035372217)) ;
#190398=CARTESIAN_POINT('Ctrl Pts',(-10.2145214483286,-12.5020990787824,
117.873442790023)) ;
#190399=CARTESIAN_POINT('Ctrl Pts',(-10.2018508550051,-12.4379801364379,
117.834850207828)) ;
#190400=CARTESIAN_POINT('Ctrl Pts',(-10.2756547077164,-12.4379801181319,
117.810619194442)) ;
#190401=CARTESIAN_POINT('Ctrl Pts',(-10.3494585604278,-12.4379800998258,
117.786388181056)) ;
#190402=CARTESIAN_POINT('Ctrl Pts',(-10.3621291537513,-12.5020990421703,
117.824980763251)) ;
#190403=CARTESIAN_POINT('Ctrl Pts',(-10.28233167392,-12.6906392671464,117.617412412838)) ;
#190404=CARTESIAN_POINT('Ctrl Pts',(-10.2998578268941,-12.7416870715668,
117.670794246116)) ;
#190405=CARTESIAN_POINT('Ctrl Pts',(-10.226053974148,-12.7416871035792,
117.695025259396)) ;
#190406=CARTESIAN_POINT('Ctrl Pts',(-10.1522501214019,-12.7416871355915,
117.719256272676)) ;
#190407=CARTESIAN_POINT('Ctrl Pts',(-10.1347239684278,-12.6906393311711,
117.665874439398)) ;
#190408=CARTESIAN_POINT('Ctrl Pts',(-10.1171978154537,-12.6395915267507,
117.61249260612)) ;
#190409=CARTESIAN_POINT('Ctrl Pts',(-10.1910016681997,-12.6395914947383,
117.58826159284)) ;
#190410=CARTESIAN_POINT('Ctrl Pts',(-10.2648055209459,-12.639591462726,
117.564030579559)) ;
#190411=CARTESIAN_POINT('Ctrl Pts',(-10.28233167392,-12.6906392671464,117.617412412838)) ;
#190412=CARTESIAN_POINT('Ctrl Pts',(-10.2205479280091,-12.9321841999642,
117.464807021943)) ;
#190413=CARTESIAN_POINT('Ctrl Pts',(-10.2416769947665,-12.9664415034876,
117.529162749087)) ;
#190414=CARTESIAN_POINT('Ctrl Pts',(-10.1678731436798,-12.9664415511475,
117.553393767422)) ;
#190415=CARTESIAN_POINT('Ctrl Pts',(-10.0940692925932,-12.9664415988073,
117.577624785756)) ;
#190416=CARTESIAN_POINT('Ctrl Pts',(-10.0729402258358,-12.9321842952839,
117.513269058612)) ;
#190417=CARTESIAN_POINT('Ctrl Pts',(-10.0518111590785,-12.8979269917605,
117.448913331469)) ;
#190418=CARTESIAN_POINT('Ctrl Pts',(-10.1256150101652,-12.8979269441006,
117.424682313134)) ;
#190419=CARTESIAN_POINT('Ctrl Pts',(-10.1994188612518,-12.8979268964408,
117.4004512948)) ;
#190420=CARTESIAN_POINT('Ctrl Pts',(-10.2205479280091,-12.9321841999642,
117.464807021943)) ;
#190421=CARTESIAN_POINT('Ctrl Pts',(-10.1807928433781,-13.2070342064579,
117.379088560202)) ;
#190422=CARTESIAN_POINT('Ctrl Pts',(-10.2039961426259,-13.2221513251204,
117.449762064688)) ;
#190423=CARTESIAN_POINT('Ctrl Pts',(-10.1301922952923,-13.2221513851254,
117.473993094454)) ;
#190424=CARTESIAN_POINT('Ctrl Pts',(-10.0563884479586,-13.2221514451304,
117.498224124219)) ;
#190425=CARTESIAN_POINT('Ctrl Pts',(-10.0331851487109,-13.2070343264679,
117.427550619733)) ;
#190426=CARTESIAN_POINT('Ctrl Pts',(-10.0099818494631,-13.1919172078054,
117.356877115248)) ;
#190427=CARTESIAN_POINT('Ctrl Pts',(-10.0837856967967,-13.1919171478004,
117.332646085482)) ;
#190428=CARTESIAN_POINT('Ctrl Pts',(-10.1575895441303,-13.1919170877954,
117.308415055717)) ;
#190429=CARTESIAN_POINT('Ctrl Pts',(-10.1807928433781,-13.2070342064579,
117.379088560202)) ;
#190430=CARTESIAN_POINT('Ctrl Pts',(-10.1647556271092,-13.4981307625057,
117.365766560135)) ;
#190431=CARTESIAN_POINT('Ctrl Pts',(-10.1883771632764,-13.4929460625343,
117.437713946625)) ;
#190432=CARTESIAN_POINT('Ctrl Pts',(-10.1145733212772,-13.492946132437,
117.461944992639)) ;
#190433=CARTESIAN_POINT('Ctrl Pts',(-10.040769479278,-13.4929462023397,
117.486176038652)) ;
#190434=CARTESIAN_POINT('Ctrl Pts',(-10.0171479431107,-13.4981309023111,
117.414228652161)) ;
#190435=CARTESIAN_POINT('Ctrl Pts',(-9.99352640694351,-13.5033156022825,
117.342281265671)) ;
#190436=CARTESIAN_POINT('Ctrl Pts',(-10.0673302489427,-13.5033155323798,
117.318050219658)) ;
#190437=CARTESIAN_POINT('Ctrl Pts',(-10.1411340909419,-13.5033154624771,
117.293819173644)) ;
#190438=CARTESIAN_POINT('Ctrl Pts',(-10.1647556271092,-13.4981307625057,
117.365766560135)) ;
#190439=CARTESIAN_POINT('Ctrl Pts',(-10.1729059089313,-13.7819922849582,
117.425914749233)) ;
#190440=CARTESIAN_POINT('Ctrl Pts',(-10.1952615851707,-13.7569816324817,
117.494006530502)) ;
#190441=CARTESIAN_POINT('Ctrl Pts',(-10.121457749576,-13.7569817049211,
117.518237596022)) ;
#190442=CARTESIAN_POINT('Ctrl Pts',(-10.0476539139814,-13.7569817773604,
117.542468661543)) ;
#190443=CARTESIAN_POINT('Ctrl Pts',(-10.025298237742,-13.7819924298369,
117.474376880274)) ;
#190444=CARTESIAN_POINT('Ctrl Pts',(-10.0029425615027,-13.8070030823134,
117.406285099005)) ;
#190445=CARTESIAN_POINT('Ctrl Pts',(-10.0767463970973,-13.807003009874,
117.382054033484)) ;
#190446=CARTESIAN_POINT('Ctrl Pts',(-10.150550232692,-13.8070029374347,
117.357822967964)) ;
#190447=CARTESIAN_POINT('Ctrl Pts',(-10.1729059089313,-13.7819922849582,
117.425914749233)) ;
#190448=CARTESIAN_POINT('Ctrl Pts',(-10.2041166916304,-14.041794726603,
117.55658075774)) ;
#190449=CARTESIAN_POINT('Ctrl Pts',(-10.2235892247858,-13.9986090894959,
117.61589095021)) ;
#190450=CARTESIAN_POINT('Ctrl Pts',(-10.1497853964037,-13.998609159369,
117.640122037698)) ;
#190451=CARTESIAN_POINT('Ctrl Pts',(-10.0759815680215,-13.998609229242,
117.664353125187)) ;
#190452=CARTESIAN_POINT('Ctrl Pts',(-10.0565090348661,-14.0417948663491,
117.605042932717)) ;
#190453=CARTESIAN_POINT('Ctrl Pts',(-10.0370365017106,-14.0849805034562,
117.545732740248)) ;
#190454=CARTESIAN_POINT('Ctrl Pts',(-10.1108403300928,-14.0849804335832,
117.52150165276)) ;
#190455=CARTESIAN_POINT('Ctrl Pts',(-10.1846441584749,-14.0849803637101,
117.497270565271)) ;
#190456=CARTESIAN_POINT('Ctrl Pts',(-10.2041166916304,-14.041794726603,
117.55658075774)) ;
#190457=CARTESIAN_POINT('Ctrl Pts',(-10.2550233033811,-14.255449164482,
117.747005840351)) ;
#190458=CARTESIAN_POINT('Ctrl Pts',(-10.2702380565919,-14.197284228839,
117.793347521988)) ;
#190459=CARTESIAN_POINT('Ctrl Pts',(-10.1964342348443,-14.197284287096,
117.817578629684)) ;
#190460=CARTESIAN_POINT('Ctrl Pts',(-10.1226304130967,-14.197284345353,
117.84180973738)) ;
#190461=CARTESIAN_POINT('Ctrl Pts',(-10.1074156598859,-14.2554492809961,
117.795468055743)) ;
#190462=CARTESIAN_POINT('Ctrl Pts',(-10.0922009066752,-14.3136142166391,
117.749126374106)) ;
#190463=CARTESIAN_POINT('Ctrl Pts',(-10.1660047284228,-14.3136141583821,
117.72489526641)) ;
#190464=CARTESIAN_POINT('Ctrl Pts',(-10.2398085501704,-14.313614100125,
117.700664158713)) ;
#190465=CARTESIAN_POINT('Ctrl Pts',(-10.2550233033811,-14.255449164482,
117.747005840351)) ;
#190466=CARTESIAN_POINT('Ctrl Pts',(-10.3219217787568,-14.4102492008634,
117.986414030523)) ;
#190467=CARTESIAN_POINT('Ctrl Pts',(-10.3317506903204,-14.3411914994799,
118.016351307379)) ;
#190468=CARTESIAN_POINT('Ctrl Pts',(-10.2579468745014,-14.3411915397154,
118.040582433133)) ;
#190469=CARTESIAN_POINT('Ctrl Pts',(-10.1841430586823,-14.3411915799509,
118.064813558886)) ;
#190470=CARTESIAN_POINT('Ctrl Pts',(-10.1743141471187,-14.4102492813345,
118.034876282031)) ;
#190471=CARTESIAN_POINT('Ctrl Pts',(-10.1644852355551,-14.4793069827181,
118.004939005175)) ;
#190472=CARTESIAN_POINT('Ctrl Pts',(-10.2382890513741,-14.4793069424825,
117.980707879422)) ;
#190473=CARTESIAN_POINT('Ctrl Pts',(-10.3120928671932,-14.479306902247,
117.956476753668)) ;
#190474=CARTESIAN_POINT('Ctrl Pts',(-10.3219217787568,-14.4102492008634,
117.986414030523)) ;
#190475=CARTESIAN_POINT('Ctrl Pts',(-10.3980811903642,-14.4927425304254,
118.253658438679)) ;
#190476=CARTESIAN_POINT('Ctrl Pts',(-10.401877290509,-14.4178249477771,
118.265220745276)) ;
#190477=CARTESIAN_POINT('Ctrl Pts',(-10.3280734781105,-14.4178249636249,
118.289451881448)) ;
#190478=CARTESIAN_POINT('Ctrl Pts',(-10.254269665712,-14.4178249794727,
118.31368301762)) ;
#190479=CARTESIAN_POINT('Ctrl Pts',(-10.2504735655672,-14.4927425621209,
118.302120711023)) ;
#190480=CARTESIAN_POINT('Ctrl Pts',(-10.2466774654224,-14.5676601447692,
118.290558404426)) ;
#190481=CARTESIAN_POINT('Ctrl Pts',(-10.3204812778209,-14.5676601289214,
118.266327268254)) ;
#190482=CARTESIAN_POINT('Ctrl Pts',(-10.3942850902194,-14.5676601130736,
118.242096132082)) ;
#190483=CARTESIAN_POINT('Ctrl Pts',(-10.3980811903642,-14.4927425304254,
118.253658438679)) ;
#190484=CARTESIAN_POINT('Ctrl Pts',(-10.4784322706411,-14.4990616510816,
118.533888978582)) ;
#190485=CARTESIAN_POINT('Ctrl Pts',(-10.4758897404157,-14.4235929848165,
118.526144839733)) ;
#190486=CARTESIAN_POINT('Ctrl Pts',(-10.4020859293724,-14.4235929732871,
118.550375980033)) ;
#190487=CARTESIAN_POINT('Ctrl Pts',(-10.3282821183291,-14.4235929617576,
118.574607120333)) ;
#190488=CARTESIAN_POINT('Ctrl Pts',(-10.3308246485545,-14.4990616280226,
118.582351259182)) ;
#190489=CARTESIAN_POINT('Ctrl Pts',(-10.3333671787799,-14.5745302942877,
118.59009539803)) ;
#190490=CARTESIAN_POINT('Ctrl Pts',(-10.4071709898231,-14.5745303058172,
118.56586425773)) ;
#190491=CARTESIAN_POINT('Ctrl Pts',(-10.4809748008665,-14.5745303173466,
118.541633117431)) ;
#190492=CARTESIAN_POINT('Ctrl Pts',(-10.4784322706411,-14.4990616510816,
118.533888978582)) ;
#190493=CARTESIAN_POINT('Ctrl Pts',(-10.5559396621602,-14.4278621718276,
118.805402129203)) ;
#190494=CARTESIAN_POINT('Ctrl Pts',(-10.5472488614899,-14.3572534635398,
118.778931350552)) ;
#190495=CARTESIAN_POINT('Ctrl Pts',(-10.4734450490211,-14.357253423911,
118.80316248651)) ;
#190496=CARTESIAN_POINT('Ctrl Pts',(-10.3996412365523,-14.3572533842822,
118.827393622468)) ;
#190497=CARTESIAN_POINT('Ctrl Pts',(-10.4083320372227,-14.4278620925699,
118.853864401119)) ;
#190498=CARTESIAN_POINT('Ctrl Pts',(-10.4170228378929,-14.4984708008576,
118.880335179769)) ;
#190499=CARTESIAN_POINT('Ctrl Pts',(-10.4908266503617,-14.4984708404865,
118.856104043811)) ;
#190500=CARTESIAN_POINT('Ctrl Pts',(-10.5646304628305,-14.4984708801153,
118.831872907853)) ;
#190501=CARTESIAN_POINT('Ctrl Pts',(-10.5559396621602,-14.4278621718276,
118.805402129203)) ;
#190502=CARTESIAN_POINT('Ctrl Pts',(-10.6246350611719,-14.2839264835508,
119.050194569323)) ;
#190503=CARTESIAN_POINT('Ctrl Pts',(-10.6103996640293,-14.2232622888904,
119.006835844406)) ;
#190504=CARTESIAN_POINT('Ctrl Pts',(-10.5365958475133,-14.2232622233179,
119.031066968037)) ;
#190505=CARTESIAN_POINT('Ctrl Pts',(-10.4627920309972,-14.2232621577455,
119.055298091668)) ;
#190506=CARTESIAN_POINT('Ctrl Pts',(-10.4770274281398,-14.2839263524059,
119.098656816584)) ;
#190507=CARTESIAN_POINT('Ctrl Pts',(-10.4912628252824,-14.3445905470663,
119.142015541501)) ;
#190508=CARTESIAN_POINT('Ctrl Pts',(-10.5650666417984,-14.3445906126388,
119.11778441787)) ;
#190509=CARTESIAN_POINT('Ctrl Pts',(-10.6388704583145,-14.3445906782112,
119.09355329424)) ;
#190510=CARTESIAN_POINT('Ctrl Pts',(-10.6246350611719,-14.2839264835508,
119.050194569323)) ;
#190511=CARTESIAN_POINT('Ctrl Pts',(-10.6784414228845,-14.0776636855761,
119.249607301814)) ;
#190512=CARTESIAN_POINT('Ctrl Pts',(-10.6596932344536,-14.0313099788708,
119.19250334277)) ;
#190513=CARTESIAN_POINT('Ctrl Pts',(-10.5858894115044,-14.0313098927161,
119.216734446806)) ;
#190514=CARTESIAN_POINT('Ctrl Pts',(-10.5120855885552,-14.0313098065613,
119.240965550842)) ;
#190515=CARTESIAN_POINT('Ctrl Pts',(-10.5308337769861,-14.0776635132666,
119.298069509887)) ;
#190516=CARTESIAN_POINT('Ctrl Pts',(-10.549581965417,-14.1240172199719,
119.355173468931)) ;
#190517=CARTESIAN_POINT('Ctrl Pts',(-10.6233857883662,-14.1240173061266,
119.330942364894)) ;
#190518=CARTESIAN_POINT('Ctrl Pts',(-10.6971896113153,-14.1240173922814,
119.306711260858)) ;
#190519=CARTESIAN_POINT('Ctrl Pts',(-10.6784414228845,-14.0776636855761,
119.249607301814)) ;
#190520=CARTESIAN_POINT('Ctrl Pts',(-10.7127437309599,-13.825817961869,
119.38938959783)) ;
#190521=CARTESIAN_POINT('Ctrl Pts',(-10.6908424609061,-13.7969788395993,
119.322681860926)) ;
#190522=CARTESIAN_POINT('Ctrl Pts',(-10.6170386300113,-13.7969787399069,
119.346912940761)) ;
#190523=CARTESIAN_POINT('Ctrl Pts',(-10.5432347991165,-13.7969786402144,
119.371144020597)) ;
#190524=CARTESIAN_POINT('Ctrl Pts',(-10.5651360691703,-13.8258177624841,
119.437851757501)) ;
#190525=CARTESIAN_POINT('Ctrl Pts',(-10.5870373392241,-13.8546568847537,
119.504559494405)) ;
#190526=CARTESIAN_POINT('Ctrl Pts',(-10.6608411701189,-13.8546569844462,
119.48032841457)) ;
#190527=CARTESIAN_POINT('Ctrl Pts',(-10.7346450010137,-13.8546570841386,
119.456097334734)) ;
#190528=CARTESIAN_POINT('Ctrl Pts',(-10.7127437309599,-13.825817961869,
119.38938959783)) ;
#190529=CARTESIAN_POINT('Ctrl Pts',(-10.7247246250284,-13.5431962708422,
119.461411594824)) ;
#190530=CARTESIAN_POINT('Ctrl Pts',(-10.7012190404884,-13.5340457388908,
119.389817374893)) ;
#190531=CARTESIAN_POINT('Ctrl Pts',(-10.6274152007733,-13.5340456342861,
119.414048427863)) ;
#190532=CARTESIAN_POINT('Ctrl Pts',(-10.5536113610583,-13.5340455296813,
119.438279480834)) ;
#190533=CARTESIAN_POINT('Ctrl Pts',(-10.5771169455982,-13.5431960616327,
119.509873700765)) ;
#190534=CARTESIAN_POINT('Ctrl Pts',(-10.6006225301382,-13.5523465935841,
119.581467920696)) ;
#190535=CARTESIAN_POINT('Ctrl Pts',(-10.6744263698533,-13.5523466981889,
119.557236867726)) ;
#190536=CARTESIAN_POINT('Ctrl Pts',(-10.7482302095684,-13.5523468027936,
119.533005814755)) ;
#190537=CARTESIAN_POINT('Ctrl Pts',(-10.7247246250284,-13.5431962708422,
119.461411594824)) ;
#190538=CARTESIAN_POINT('Ctrl Pts',(-10.712517892844,-13.2523620051609,
119.45965594129)) ;
#190539=CARTESIAN_POINT('Ctrl Pts',(-10.6890964715402,-13.2635030369063,
119.388318069056)) ;
#190540=CARTESIAN_POINT('Ctrl Pts',(-10.6152926231585,-13.2635029359697,
119.412549095629)) ;
#190541=CARTESIAN_POINT('Ctrl Pts',(-10.5414887747767,-13.2635028350331,
119.436780122202)) ;
#190542=CARTESIAN_POINT('Ctrl Pts',(-10.5649101960805,-13.2523618032878,
119.508117994436)) ;
#190543=CARTESIAN_POINT('Ctrl Pts',(-10.5883316173843,-13.2412207715424,
119.57945586667)) ;
#190544=CARTESIAN_POINT('Ctrl Pts',(-10.6621354657661,-13.241220872479,
119.555224840097)) ;
#190545=CARTESIAN_POINT('Ctrl Pts',(-10.7359393141478,-13.2412209734156,
119.530993813524)) ;
#190546=CARTESIAN_POINT('Ctrl Pts',(-10.712517892844,-13.2523620051609,
119.45965594129)) ;
#190547=CARTESIAN_POINT('Ctrl Pts',(-10.6762276498122,-12.972854005055,
119.384625156595)) ;
#190548=CARTESIAN_POINT('Ctrl Pts',(-10.6545701505956,-13.0035262645876,
119.318659906517)) ;
#190549=CARTESIAN_POINT('Ctrl Pts',(-10.5807662945932,-13.0035261755681,
119.342890909878)) ;
#190550=CARTESIAN_POINT('Ctrl Pts',(-10.5069624385908,-13.0035260865486,
119.36712191324)) ;
#190551=CARTESIAN_POINT('Ctrl Pts',(-10.5286199378074,-12.9728538270159,
119.433087163318)) ;
#190552=CARTESIAN_POINT('Ctrl Pts',(-10.5502774370239,-12.9421815674833,
119.499052413396)) ;
#190553=CARTESIAN_POINT('Ctrl Pts',(-10.6240812930263,-12.9421816565028,
119.474821410034)) ;
#190554=CARTESIAN_POINT('Ctrl Pts',(-10.6978851490287,-12.9421817455224,
119.450590406672)) ;
#190555=CARTESIAN_POINT('Ctrl Pts',(-10.6762276498122,-12.972854005055,
119.384625156595)) ;
#190556=CARTESIAN_POINT('Ctrl Pts',(-10.6180038705804,-12.7260422771964,
119.242651094908)) ;
#190557=CARTESIAN_POINT('Ctrl Pts',(-10.5996471848408,-12.7739923813095,
119.186739590185)) ;
#190558=CARTESIAN_POINT('Ctrl Pts',(-10.5258433228096,-12.7739923097986,
119.210970575184)) ;
#190559=CARTESIAN_POINT('Ctrl Pts',(-10.4520394607784,-12.7739922382878,
119.235201560183)) ;
#190560=CARTESIAN_POINT('Ctrl Pts',(-10.470396146518,-12.7260421341746,
119.291113064906)) ;
#190561=CARTESIAN_POINT('Ctrl Pts',(-10.4887528322575,-12.6780920300614,
119.347024569628)) ;
#190562=CARTESIAN_POINT('Ctrl Pts',(-10.5625566942887,-12.6780921015723,
119.32279358463)) ;
#190563=CARTESIAN_POINT('Ctrl Pts',(-10.6363605563199,-12.6780921730832,
119.298562599631)) ;
#190564=CARTESIAN_POINT('Ctrl Pts',(-10.6180038705804,-12.7260422771964,
119.242651094908)) ;
#190565=CARTESIAN_POINT('Ctrl Pts',(-10.5404232380422,-12.5272823112894,
119.04200368921)) ;
#190566=CARTESIAN_POINT('Ctrl Pts',(-10.5267175930382,-12.5891820336003,
119.000258504269)) ;
#190567=CARTESIAN_POINT('Ctrl Pts',(-10.4529137276197,-12.5891819848851,
119.02448947895)) ;
#190568=CARTESIAN_POINT('Ctrl Pts',(-10.3791098622012,-12.58918193617,119.048720453632)) ;
#190569=CARTESIAN_POINT('Ctrl Pts',(-10.3928155072053,-12.5272822138591,
119.090465638574)) ;
#190570=CARTESIAN_POINT('Ctrl Pts',(-10.4065211522092,-12.4653824915483,
119.132210823515)) ;
#190571=CARTESIAN_POINT('Ctrl Pts',(-10.4803250176277,-12.4653825402634,
119.107979848833)) ;
#190572=CARTESIAN_POINT('Ctrl Pts',(-10.5541288830462,-12.4653825889786,
119.083748874151)) ;
#190573=CARTESIAN_POINT('Ctrl Pts',(-10.5404232380422,-12.5272823112894,
119.04200368921)) ;
#190574=CARTESIAN_POINT('Ctrl Pts',(-10.4495581259175,-12.3938739809445,
118.800583074419)) ;
#190575=CARTESIAN_POINT('Ctrl Pts',(-10.44144472112,-12.4651813337181,118.775870950958)) ;
#190576=CARTESIAN_POINT('Ctrl Pts',(-10.3676408542443,-12.4651813074342,
118.800101921202)) ;
#190577=CARTESIAN_POINT('Ctrl Pts',(-10.2938369873686,-12.4651812811503,
118.824332891445)) ;
#190578=CARTESIAN_POINT('Ctrl Pts',(-10.3019503921661,-12.3938739283766,
118.849045014906)) ;
#190579=CARTESIAN_POINT('Ctrl Pts',(-10.3100637969636,-12.322566575603,
118.873757138366)) ;
#190580=CARTESIAN_POINT('Ctrl Pts',(-10.3838676638393,-12.3225666018869,
118.849526168123)) ;
#190581=CARTESIAN_POINT('Ctrl Pts',(-10.4576715307149,-12.3225666281708,
118.825295197879)) ;
#190582=CARTESIAN_POINT('Ctrl Pts',(-10.4495581259175,-12.3938739809445,
118.800583074419)) ;
#190583=CARTESIAN_POINT('Ctrl Pts',(-10.3500894578653,-12.3331330123649,
118.53313055352)) ;
#190584=CARTESIAN_POINT('Ctrl Pts',(-10.348173757062,-12.4087892430706,
118.527295636584)) ;
#190585=CARTESIAN_POINT('Ctrl Pts',(-10.2743698913232,-12.408789238365,
118.551526610291)) ;
#190586=CARTESIAN_POINT('Ctrl Pts',(-10.2005660255843,-12.4087892336594,
118.575757583997)) ;
#190587=CARTESIAN_POINT('Ctrl Pts',(-10.2024817263876,-12.3331330029537,
118.581592500933)) ;
#190588=CARTESIAN_POINT('Ctrl Pts',(-10.2043974271909,-12.257476772248,
118.587427417868)) ;
#190589=CARTESIAN_POINT('Ctrl Pts',(-10.2782012929297,-12.2574767769536,
118.563196444162)) ;
#190590=CARTESIAN_POINT('Ctrl Pts',(-10.3520051586686,-12.2574767816592,
118.538965470456)) ;
#190591=CARTESIAN_POINT('Ctrl Pts',(-10.3500894578653,-12.3331330123649,
118.53313055352)) ;
#190592=CARTESIAN_POINT('Ctrl Pts',(-10.2491542011391,-12.3500900604043,
118.261071608061)) ;
#190593=CARTESIAN_POINT('Ctrl Pts',(-10.2535509429431,-12.4246766699504,
118.274463372938)) ;
#190594=CARTESIAN_POINT('Ctrl Pts',(-10.1797470798509,-12.4246766830339,
118.298694354706)) ;
#190595=CARTESIAN_POINT('Ctrl Pts',(-10.1059432167588,-12.4246766961173,
118.322925336473)) ;
#190596=CARTESIAN_POINT('Ctrl Pts',(-10.1015464749548,-12.3500900865712,
118.309533571596)) ;
#190597=CARTESIAN_POINT('Ctrl Pts',(-10.0971497331507,-12.2755034770251,
118.296141806718)) ;
#190598=CARTESIAN_POINT('Ctrl Pts',(-10.1709535962429,-12.2755034639416,
118.27191082495)) ;
#190599=CARTESIAN_POINT('Ctrl Pts',(-10.2447574593351,-12.2755034508582,
118.247679843183)) ;
#190600=CARTESIAN_POINT('Ctrl Pts',(-10.2491542011391,-12.3500900604043,
118.261071608061)) ;
#190601=CARTESIAN_POINT('Ctrl Pts',(-10.1522204522322,-12.4439523224458,
118.001438639181)) ;
#190602=CARTESIAN_POINT('Ctrl Pts',(-10.1626549630217,-12.5120989674076,
118.033220474389)) ;
#190603=CARTESIAN_POINT('Ctrl Pts',(-10.0888511045098,-12.5120989925412,
118.057451470107)) ;
#190604=CARTESIAN_POINT('Ctrl Pts',(-10.0150472459978,-12.5120990176749,
118.081682465826)) ;
#190605=CARTESIAN_POINT('Ctrl Pts',(-10.0046127352084,-12.4439523727131,
118.049900630617)) ;
#190606=CARTESIAN_POINT('Ctrl Pts',(-9.99417822441887,-12.3758057277512,
118.018118795408)) ;
#190607=CARTESIAN_POINT('Ctrl Pts',(-10.0679820829308,-12.3758057026176,
117.99388779969)) ;
#190608=CARTESIAN_POINT('Ctrl Pts',(-10.1417859414427,-12.3758056774839,
117.969656803972)) ;
#190609=CARTESIAN_POINT('Ctrl Pts',(-10.1522204522322,-12.4439523224458,
118.001438639181)) ;
#190610=CARTESIAN_POINT('Ctrl Pts',(-10.0665263018171,-12.607738556858,
117.775916927757)) ;
#190611=CARTESIAN_POINT('Ctrl Pts',(-10.0822256130435,-12.6645527953263,
117.823734495797)) ;
#190612=CARTESIAN_POINT('Ctrl Pts',(-10.0084217591895,-12.6645528262529,
117.847965505703)) ;
#190613=CARTESIAN_POINT('Ctrl Pts',(-9.93461790533546,-12.6645528571796,
117.872196515608)) ;
#190614=CARTESIAN_POINT('Ctrl Pts',(-9.91891859410901,-12.6077386187113,
117.824378947568)) ;
#190615=CARTESIAN_POINT('Ctrl Pts',(-9.90321928288255,-12.5509243802431,
117.776561379528)) ;
#190616=CARTESIAN_POINT('Ctrl Pts',(-9.97702313673659,-12.5509243493165,
117.752330369622)) ;
#190617=CARTESIAN_POINT('Ctrl Pts',(-10.0508269905906,-12.5509243183898,
117.728099359717)) ;
#190618=CARTESIAN_POINT('Ctrl Pts',(-10.0665263018171,-12.607738556858,
117.775916927757)) ;
#190619=CARTESIAN_POINT('Ctrl Pts',(-9.9973141738669,-12.8282760815645,
117.600428827391)) ;
#190620=CARTESIAN_POINT('Ctrl Pts',(-10.0171388338787,-12.8697778180786,
117.660811542349)) ;
#190621=CARTESIAN_POINT('Ctrl Pts',(-9.94333498419105,-12.8697778506645,
117.685042564945)) ;
#190622=CARTESIAN_POINT('Ctrl Pts',(-9.86953113450339,-12.8697778832504,
117.70927358754)) ;
#190623=CARTESIAN_POINT('Ctrl Pts',(-9.84970647449161,-12.8282761467363,
117.648890872582)) ;
#190624=CARTESIAN_POINT('Ctrl Pts',(-9.8298818144798,-12.7867744102223,
117.588508157623)) ;
#190625=CARTESIAN_POINT('Ctrl Pts',(-9.90368566416747,-12.7867743776364,
117.564277135028)) ;
#190626=CARTESIAN_POINT('Ctrl Pts',(-9.97748951385512,-12.7867743450505,
117.540046112432)) ;
#190627=CARTESIAN_POINT('Ctrl Pts',(-9.9973141738669,-12.8282760815645,
117.600428827391)) ;
#190628=CARTESIAN_POINT('Ctrl Pts',(-9.94813424492341,-13.0924261676405,
117.486171962013)) ;
#190629=CARTESIAN_POINT('Ctrl Pts',(-9.97068753593406,-13.1155471529824,
117.554865646909)) ;
#190630=CARTESIAN_POINT('Ctrl Pts',(-9.8968836900418,-13.1155471809982,
117.579096681065)) ;
#190631=CARTESIAN_POINT('Ctrl Pts',(-9.82307984414954,-13.1155472090139,
117.60332771522)) ;
#190632=CARTESIAN_POINT('Ctrl Pts',(-9.80052655313887,-13.092426223672,
117.534634030324)) ;
#190633=CARTESIAN_POINT('Ctrl Pts',(-9.7779732621282,-13.06930523833,117.465940345428)) ;
#190634=CARTESIAN_POINT('Ctrl Pts',(-9.85177710802046,-13.0693052103143,
117.441709311273)) ;
#190635=CARTESIAN_POINT('Ctrl Pts',(-9.9255809539127,-13.0693051822985,
117.417478277117)) ;
#190636=CARTESIAN_POINT('Ctrl Pts',(-9.94813424492341,-13.0924261676405,
117.486171962013)) ;
#190637=CARTESIAN_POINT('Ctrl Pts',(-9.92229665695523,-13.3792544087802,
117.442915109267)) ;
#190638=CARTESIAN_POINT('Ctrl Pts',(-9.94595477750255,-13.3823829246599,
117.514973926819)) ;
#190639=CARTESIAN_POINT('Ctrl Pts',(-9.87215093408175,-13.3823829459244,
117.539204968502)) ;
#190640=CARTESIAN_POINT('Ctrl Pts',(-9.79834709066094,-13.3823829671888,
117.563436010186)) ;
#190641=CARTESIAN_POINT('Ctrl Pts',(-9.77468897011363,-13.3792544513091,
117.491377192633)) ;
#190642=CARTESIAN_POINT('Ctrl Pts',(-9.75103084956629,-13.3761259354293,
117.419318375081)) ;
#190643=CARTESIAN_POINT('Ctrl Pts',(-9.82483469298709,-13.3761259141649,
117.395087333397)) ;
#190644=CARTESIAN_POINT('Ctrl Pts',(-9.8986385364079,-13.3761258929005,
117.370856291714)) ;
#190645=CARTESIAN_POINT('Ctrl Pts',(-9.92229665695523,-13.3792544087802,
117.442915109267)) ;
#190646=CARTESIAN_POINT('Ctrl Pts',(-9.9207435467235,-13.6698091146606,
117.47374538968)) ;
#190647=CARTESIAN_POINT('Ctrl Pts',(-9.94381007459405,-13.6526542862593,
117.54400231155)) ;
#190648=CARTESIAN_POINT('Ctrl Pts',(-9.87000623233327,-13.6526542988554,
117.568233356767)) ;
#190649=CARTESIAN_POINT('Ctrl Pts',(-9.79620239007249,-13.6526543114514,
117.592464401983)) ;
#190650=CARTESIAN_POINT('Ctrl Pts',(-9.77313586220196,-13.6698091398527,
117.522207480113)) ;
#190651=CARTESIAN_POINT('Ctrl Pts',(-9.75006933433139,-13.686963968254,
117.451950558243)) ;
#190652=CARTESIAN_POINT('Ctrl Pts',(-9.82387317659218,-13.686963955658,
117.427719513027)) ;
#190653=CARTESIAN_POINT('Ctrl Pts',(-9.89767701885295,-13.6869639430619,
117.40348846781)) ;
#190654=CARTESIAN_POINT('Ctrl Pts',(-9.9207435467235,-13.6698091146606,
117.47374538968)) ;
#190655=CARTESIAN_POINT('Ctrl Pts',(-9.94290969392009,-13.9412445098837,
117.576695883073)) ;
#190656=CARTESIAN_POINT('Ctrl Pts',(-9.96372985878011,-13.9051106030385,
117.640110745778)) ;
#190657=CARTESIAN_POINT('Ctrl Pts',(-9.88992601655304,-13.9051106090347,
117.664341791097)) ;
#190658=CARTESIAN_POINT('Ctrl Pts',(-9.81612217432595,-13.905110615031,
117.688572836417)) ;
#190659=CARTESIAN_POINT('Ctrl Pts',(-9.79530200946594,-13.9412445218762,
117.625157973711)) ;
#190660=CARTESIAN_POINT('Ctrl Pts',(-9.7744818446059,-13.9773784287214,
117.561743111006)) ;
#190661=CARTESIAN_POINT('Ctrl Pts',(-9.84828568683299,-13.9773784227252,
117.537512065686)) ;
#190662=CARTESIAN_POINT('Ctrl Pts',(-9.92208952906005,-13.9773784167289,
117.513281020367)) ;
#190663=CARTESIAN_POINT('Ctrl Pts',(-9.94290969392009,-13.9412445098837,
117.576695883073)) ;
#190664=CARTESIAN_POINT('Ctrl Pts',(-9.9861032646117,-14.1747166899893,
117.74357571091)) ;
#190665=CARTESIAN_POINT('Ctrl Pts',(-10.0032076914057,-14.1222263839683,
117.795673035085)) ;
#190666=CARTESIAN_POINT('Ctrl Pts',(-9.92940384865615,-14.1222263855747,
117.819904078812)) ;
#190667=CARTESIAN_POINT('Ctrl Pts',(-9.85560000590656,-14.122226387181,
117.84413512254)) ;
#190668=CARTESIAN_POINT('Ctrl Pts',(-9.8384955791125,-14.1747166932021,
117.792037798365)) ;
#190669=CARTESIAN_POINT('Ctrl Pts',(-9.82139115231847,-14.2272069992232,
117.739940474191)) ;
#190670=CARTESIAN_POINT('Ctrl Pts',(-9.89519499506806,-14.2272069976168,
117.715709430463)) ;
#190671=CARTESIAN_POINT('Ctrl Pts',(-9.96899883781767,-14.2272069960104,
117.691478386735)) ;
#190672=CARTESIAN_POINT('Ctrl Pts',(-9.9861032646117,-14.1747166899893,
117.74357571091)) ;
#190673=CARTESIAN_POINT('Ctrl Pts',(-10.0471796021649,-14.355514528968,
117.96520267545)) ;
#190674=CARTESIAN_POINT('Ctrl Pts',(-10.0593081194111,-14.2903204554486,
118.002144182084)) ;
#190675=CARTESIAN_POINT('Ctrl Pts',(-9.98550427561081,-14.2903204543728,
118.026375222612)) ;
#190676=CARTESIAN_POINT('Ctrl Pts',(-9.91170043181045,-14.290320453297,
118.050606263139)) ;
#190677=CARTESIAN_POINT('Ctrl Pts',(-9.89957191456421,-14.3555145268165,
118.013664756505)) ;
#190678=CARTESIAN_POINT('Ctrl Pts',(-9.88744339731793,-14.4207086003359,
117.97672324987)) ;
#190679=CARTESIAN_POINT('Ctrl Pts',(-9.96124724111826,-14.4207086014117,
117.952492209343)) ;
#190680=CARTESIAN_POINT('Ctrl Pts',(-10.0350510849186,-14.4207086024875,
117.928261168815)) ;
#190681=CARTESIAN_POINT('Ctrl Pts',(-10.0471796021649,-14.355514528968,
117.96520267545)) ;
#190682=CARTESIAN_POINT('Ctrl Pts',(-10.1202605083237,-14.4682461385157,
118.223189643421)) ;
#190683=CARTESIAN_POINT('Ctrl Pts',(-10.1265714543446,-14.3950833007867,
118.242411766797)) ;
#190684=CARTESIAN_POINT('Ctrl Pts',(-10.0527676099358,-14.3950832998909,
118.266642805471)) ;
#190685=CARTESIAN_POINT('Ctrl Pts',(-9.97896376552697,-14.395083298995,
118.290873844145)) ;
#190686=CARTESIAN_POINT('Ctrl Pts',(-9.97265281950605,-14.468246136724,
118.271651720769)) ;
#190687=CARTESIAN_POINT('Ctrl Pts',(-9.96634187348515,-14.5414089744529,
118.252429597393)) ;
#190688=CARTESIAN_POINT('Ctrl Pts',(-10.040145717894,-14.5414089753487,
118.228198558719)) ;
#190689=CARTESIAN_POINT('Ctrl Pts',(-10.1139495623028,-14.5414089762446,
118.203967520045)) ;
#190690=CARTESIAN_POINT('Ctrl Pts',(-10.1202605083237,-14.4682461385157,
118.223189643421)) ;
#190691=CARTESIAN_POINT('Ctrl Pts',(-10.2000975446143,-14.5059599121584,
118.501953451591)) ;
#190692=CARTESIAN_POINT('Ctrl Pts',(-10.2001061244579,-14.4300548891346,
118.501979584462)) ;
#190693=CARTESIAN_POINT('Ctrl Pts',(-10.1263022802071,-14.4300548892677,
118.526210623618)) ;
#190694=CARTESIAN_POINT('Ctrl Pts',(-10.0524984359563,-14.4300548894008,
118.550441662773)) ;
#190695=CARTESIAN_POINT('Ctrl Pts',(-10.0524898561127,-14.5059599124246,
118.550415529902)) ;
#190696=CARTESIAN_POINT('Ctrl Pts',(-10.0524812762691,-14.5818649354484,
118.55038939703)) ;
#190697=CARTESIAN_POINT('Ctrl Pts',(-10.1262851205199,-14.5818649353153,
118.526158357875)) ;
#190698=CARTESIAN_POINT('Ctrl Pts',(-10.2000889647707,-14.5818649351822,
118.50192731872)) ;
#190699=CARTESIAN_POINT('Ctrl Pts',(-10.2000975446143,-14.5059599121584,
118.501953451591)) ;
#190700=CARTESIAN_POINT('Ctrl Pts',(-10.279142301007,-14.4658731530402,
118.777992572)) ;
#190701=CARTESIAN_POINT('Ctrl Pts',(-10.2729014028888,-14.3926562072765,
118.758983803308)) ;
#190702=CARTESIAN_POINT('Ctrl Pts',(-10.1990975593153,-14.3926562077147,
118.783214844527)) ;
#190703=CARTESIAN_POINT('Ctrl Pts',(-10.1252937157419,-14.3926562081529,
118.807445885745)) ;
#190704=CARTESIAN_POINT('Ctrl Pts',(-10.1315346138602,-14.4658731539167,
118.826454654437)) ;
#190705=CARTESIAN_POINT('Ctrl Pts',(-10.1377755119784,-14.5390900996804,
118.845463423128)) ;
#190706=CARTESIAN_POINT('Ctrl Pts',(-10.2115793555519,-14.5390900992422,
118.821232381909)) ;
#190707=CARTESIAN_POINT('Ctrl Pts',(-10.2853831991253,-14.539090098804,
118.797001340691)) ;
#190708=CARTESIAN_POINT('Ctrl Pts',(-10.279142301007,-14.4658731530402,
118.777992572)) ;
#190709=CARTESIAN_POINT('Ctrl Pts',(-10.352240241271,-14.3505784504634,
119.036184934344)) ;
#190710=CARTESIAN_POINT('Ctrl Pts',(-10.3401503369545,-14.2853046871927,
118.999361036421)) ;
#190711=CARTESIAN_POINT('Ctrl Pts',(-10.266346494636,-14.2853046856717,
119.023592081462)) ;
#190712=CARTESIAN_POINT('Ctrl Pts',(-10.1925426523175,-14.2853046841507,
119.047823126503)) ;
#190713=CARTESIAN_POINT('Ctrl Pts',(-10.204632556634,-14.3505784474213,
119.084647024426)) ;
#190714=CARTESIAN_POINT('Ctrl Pts',(-10.2167224609505,-14.4158522106919,
119.121470922348)) ;
#190715=CARTESIAN_POINT('Ctrl Pts',(-10.290526303269,-14.4158522122129,
119.097239877307)) ;
#190716=CARTESIAN_POINT('Ctrl Pts',(-10.3643301455875,-14.415852213734,
119.073008832266)) ;
#190717=CARTESIAN_POINT('Ctrl Pts',(-10.352240241271,-14.3505784504634,
119.036184934344)) ;
#190718=CARTESIAN_POINT('Ctrl Pts',(-10.4126879463665,-14.1680509006919,
119.255822408057)) ;
#190719=CARTESIAN_POINT('Ctrl Pts',(-10.3956244954864,-14.1154268840112,
119.203849889661)) ;
#190720=CARTESIAN_POINT('Ctrl Pts',(-10.3218206543467,-14.1154268771774,
119.228080938293)) ;
#190721=CARTESIAN_POINT('Ctrl Pts',(-10.248016813207,-14.1154268703437,
119.252311986924)) ;
#190722=CARTESIAN_POINT('Ctrl Pts',(-10.2650802640871,-14.1680508870244,
119.30428450532)) ;
#190723=CARTESIAN_POINT('Ctrl Pts',(-10.2821437149672,-14.220674903705,
119.356257023716)) ;
#190724=CARTESIAN_POINT('Ctrl Pts',(-10.3559475561069,-14.2206749105388,
119.332025975084)) ;
#190725=CARTESIAN_POINT('Ctrl Pts',(-10.4297513972466,-14.2206749173726,
119.307794926453)) ;
#190726=CARTESIAN_POINT('Ctrl Pts',(-10.4126879463665,-14.1680509006919,
119.255822408057)) ;
#190727=CARTESIAN_POINT('Ctrl Pts',(-10.4553302025288,-13.9327426687889,
119.421085323347)) ;
#190728=CARTESIAN_POINT('Ctrl Pts',(-10.4345324484994,-13.8964722980425,
119.357738719966)) ;
#190729=CARTESIAN_POINT('Ctrl Pts',(-10.3607286076222,-13.8964722840852,
119.381969769397)) ;
#190730=CARTESIAN_POINT('Ctrl Pts',(-10.286924766745,-13.896472270128,119.406200818828)) ;
#190731=CARTESIAN_POINT('Ctrl Pts',(-10.3077225207744,-13.9327426408744,
119.469547422208)) ;
#190732=CARTESIAN_POINT('Ctrl Pts',(-10.3285202748037,-13.9690130116207,
119.532894025589)) ;
#190733=CARTESIAN_POINT('Ctrl Pts',(-10.4023241156809,-13.969013025578,
119.508662976158)) ;
#190734=CARTESIAN_POINT('Ctrl Pts',(-10.4761279565581,-13.9690130395352,
119.484431926727)) ;
#190735=CARTESIAN_POINT('Ctrl Pts',(-10.4553302025288,-13.9327426687889,
119.421085323347)) ;
#190736=CARTESIAN_POINT('Ctrl Pts',(-10.4767300292865,-13.660519783253,
119.521681152881)) ;
#190737=CARTESIAN_POINT('Ctrl Pts',(-10.4536751293628,-13.6432040400609,
119.451459647159)) ;
#190738=CARTESIAN_POINT('Ctrl Pts',(-10.3798712878056,-13.6432040175434,
119.475690694518)) ;
#190739=CARTESIAN_POINT('Ctrl Pts',(-10.3060674462484,-13.643203995026,
119.499921741878)) ;
#190740=CARTESIAN_POINT('Ctrl Pts',(-10.329122346172,-13.6605197382181,
119.570143247601)) ;
#190741=CARTESIAN_POINT('Ctrl Pts',(-10.3521772460956,-13.6778354814103,
119.640364753323)) ;
#190742=CARTESIAN_POINT('Ctrl Pts',(-10.4259810876529,-13.6778355039277,
119.616133705964)) ;
#190743=CARTESIAN_POINT('Ctrl Pts',(-10.4997849292101,-13.6778355264452,
119.591902658604)) ;
#190744=CARTESIAN_POINT('Ctrl Pts',(-10.4767300292865,-13.660519783253,
119.521681152881)) ;
#190745=CARTESIAN_POINT('Ctrl Pts',(-10.4743674522874,-13.3693405601706,
119.550093043289)) ;
#190746=CARTESIAN_POINT('Ctrl Pts',(-10.4507071759646,-13.3723302960764,
119.478027658547)) ;
#190747=CARTESIAN_POINT('Ctrl Pts',(-10.3769033323417,-13.3723302632285,
119.502258699615)) ;
#190748=CARTESIAN_POINT('Ctrl Pts',(-10.3030994887188,-13.3723302303806,
119.526489740682)) ;
#190749=CARTESIAN_POINT('Ctrl Pts',(-10.3267597650416,-13.3693404944748,
119.598555125425)) ;
#190750=CARTESIAN_POINT('Ctrl Pts',(-10.3504200413644,-13.3663507585691,
119.670620510168)) ;
#190751=CARTESIAN_POINT('Ctrl Pts',(-10.4242238849873,-13.366350791417,
119.6463894691)) ;
#190752=CARTESIAN_POINT('Ctrl Pts',(-10.4980277286102,-13.3663508242649,
119.622158428032)) ;
#190753=CARTESIAN_POINT('Ctrl Pts',(-10.4743674522874,-13.3693405601706,
119.550093043289)) ;
#190754=CARTESIAN_POINT('Ctrl Pts',(-10.4477380288771,-13.0834454323783,
119.504368831108)) ;
#190755=CARTESIAN_POINT('Ctrl Pts',(-10.4251707000769,-13.1064007088209,
119.435632388021)) ;
#190756=CARTESIAN_POINT('Ctrl Pts',(-10.3513668529602,-13.1064006698969,
119.459863418448)) ;
#190757=CARTESIAN_POINT('Ctrl Pts',(-10.2775630058435,-13.1064006309729,
119.484094448874)) ;
#190758=CARTESIAN_POINT('Ctrl Pts',(-10.3001303346437,-13.0834453545303,
119.552830891961)) ;
#190759=CARTESIAN_POINT('Ctrl Pts',(-10.3226976634438,-13.0604900780877,
119.621567335047)) ;
#190760=CARTESIAN_POINT('Ctrl Pts',(-10.3965015105605,-13.0604901170117,
119.597336304621)) ;
#190761=CARTESIAN_POINT('Ctrl Pts',(-10.4703053576772,-13.0604901559357,
119.573105274194)) ;
#190762=CARTESIAN_POINT('Ctrl Pts',(-10.4477380288771,-13.0834454323783,
119.504368831108)) ;
#190763=CARTESIAN_POINT('Ctrl Pts',(-10.3980917229495,-12.8212149019315,
119.388565275558)) ;
#190764=CARTESIAN_POINT('Ctrl Pts',(-10.3782253674531,-12.8625120463937,
119.328055561196)) ;
#190765=CARTESIAN_POINT('Ctrl Pts',(-10.3044215158748,-12.8625120051449,
119.352286578033)) ;
#190766=CARTESIAN_POINT('Ctrl Pts',(-10.2306176642965,-12.8625119638961,
119.37651759487)) ;
#190767=CARTESIAN_POINT('Ctrl Pts',(-10.250484019793,-12.8212148194339,
119.437027309232)) ;
#190768=CARTESIAN_POINT('Ctrl Pts',(-10.2703503752895,-12.7799176749718,
119.497537023594)) ;
#190769=CARTESIAN_POINT('Ctrl Pts',(-10.3441542268677,-12.7799177162206,
119.473306006757)) ;
#190770=CARTESIAN_POINT('Ctrl Pts',(-10.417958078446,-12.7799177574694,
119.44907498992)) ;
#190771=CARTESIAN_POINT('Ctrl Pts',(-10.3980917229495,-12.8212149019315,
119.388565275558)) ;
#190772=CARTESIAN_POINT('Ctrl Pts',(-10.3280493110319,-12.6012650290221,
119.21069278713)) ;
#190773=CARTESIAN_POINT('Ctrl Pts',(-10.3123106560122,-12.6579784616352,
119.16275538225)) ;
#190774=CARTESIAN_POINT('Ctrl Pts',(-10.2385067992872,-12.6579784230308,
119.186986383411)) ;
#190775=CARTESIAN_POINT('Ctrl Pts',(-10.164702942562,-12.6579783844264,
119.211217384571)) ;
#190776=CARTESIAN_POINT('Ctrl Pts',(-10.1804415975817,-12.6012649518134,
119.259154789451)) ;
#190777=CARTESIAN_POINT('Ctrl Pts',(-10.1961802526014,-12.5445515192003,
119.30709219433)) ;
#190778=CARTESIAN_POINT('Ctrl Pts',(-10.2699841093265,-12.5445515578047,
119.28286119317)) ;
#190779=CARTESIAN_POINT('Ctrl Pts',(-10.3437879660516,-12.5445515964091,
119.258630192009)) ;
#190780=CARTESIAN_POINT('Ctrl Pts',(-10.3280493110319,-12.6012650290221,
119.21069278713)) ;
#190781=CARTESIAN_POINT('Ctrl Pts',(-10.2417633229291,-12.4396335453714,
118.983410941354)) ;
#190782=CARTESIAN_POINT('Ctrl Pts',(-10.2312909677737,-12.5077139487023,
118.951513835972)) ;
#190783=CARTESIAN_POINT('Ctrl Pts',(-10.1574871057891,-12.5077139189152,
118.975744821113)) ;
#190784=CARTESIAN_POINT('Ctrl Pts',(-10.0836832438045,-12.5077138891282,
118.999975806254)) ;
#190785=CARTESIAN_POINT('Ctrl Pts',(-10.0941555989599,-12.4396334857973,
119.031872911636)) ;
#190786=CARTESIAN_POINT('Ctrl Pts',(-10.1046279541153,-12.3715530824664,
119.063770017018)) ;
#190787=CARTESIAN_POINT('Ctrl Pts',(-10.1784318160999,-12.3715531122535,
119.039539031877)) ;
#190788=CARTESIAN_POINT('Ctrl Pts',(-10.2522356780844,-12.3715531420405,
119.015308046736)) ;
#190789=CARTESIAN_POINT('Ctrl Pts',(-10.2417633229291,-12.4396335453714,
118.983410941354)) ;
#190790=CARTESIAN_POINT('Ctrl Pts',(-10.1449346240586,-12.3483868402897,
118.723968564828)) ;
#190791=CARTESIAN_POINT('Ctrl Pts',(-10.1404732357698,-12.4229364888091,
118.710379894499)) ;
#190792=CARTESIAN_POINT('Ctrl Pts',(-10.0666693694827,-12.4229364744478,
118.734610866535)) ;
#190793=CARTESIAN_POINT('Ctrl Pts',(-9.99286550319555,-12.4229364600866,
118.758841838571)) ;
#190794=CARTESIAN_POINT('Ctrl Pts',(-9.99732689148439,-12.3483868115671,
118.772430508901)) ;
#190795=CARTESIAN_POINT('Ctrl Pts',(-10.0017882797732,-12.2738371630477,
118.78601917923)) ;
#190796=CARTESIAN_POINT('Ctrl Pts',(-10.0755921460604,-12.2738371774089,
118.761788207194)) ;
#190797=CARTESIAN_POINT('Ctrl Pts',(-10.1493960123475,-12.2738371917702,
118.737557235158)) ;
#190798=CARTESIAN_POINT('Ctrl Pts',(-10.1449346240586,-12.3483868402897,
118.723968564828)) ;
#190799=CARTESIAN_POINT('Ctrl Pts',(-10.0435893086032,-12.3339887574785,
118.450796152108)) ;
#190800=CARTESIAN_POINT('Ctrl Pts',(-10.0454623318421,-12.4096519181944,
118.45650107709)) ;
#190801=CARTESIAN_POINT('Ctrl Pts',(-9.97165846281568,-12.4096519246285,
118.480732040783)) ;
#190802=CARTESIAN_POINT('Ctrl Pts',(-9.89785459378927,-12.4096519310626,
118.504963004476)) ;
#190803=CARTESIAN_POINT('Ctrl Pts',(-9.89598157055043,-12.3339887703467,
118.499258079494)) ;
#190804=CARTESIAN_POINT('Ctrl Pts',(-9.89410854731156,-12.2583256096307,
118.493553154512)) ;
#190805=CARTESIAN_POINT('Ctrl Pts',(-9.96791241633798,-12.2583256031966,
118.469322190819)) ;
#190806=CARTESIAN_POINT('Ctrl Pts',(-10.0417162853644,-12.2583255967626,
118.445091227126)) ;
#190807=CARTESIAN_POINT('Ctrl Pts',(-10.0435893086032,-12.3339887574785,
118.450796152108)) ;
#190808=CARTESIAN_POINT('Ctrl Pts',(-9.94475629597229,-12.3966946761742,
118.185097834847)) ;
#190809=CARTESIAN_POINT('Ctrl Pts',(-9.95280117473567,-12.4680894419109,
118.209601235821)) ;
#190810=CARTESIAN_POINT('Ctrl Pts',(-9.8789973054581,-12.4680894717794,
118.233832198748)) ;
#190811=CARTESIAN_POINT('Ctrl Pts',(-9.80519343618053,-12.4680895016479,
118.258063161676)) ;
#190812=CARTESIAN_POINT('Ctrl Pts',(-9.79714855741716,-12.3966947359113,
118.233559760702)) ;
#190813=CARTESIAN_POINT('Ctrl Pts',(-9.78910367865378,-12.3252999701746,
118.209056359728)) ;
#190814=CARTESIAN_POINT('Ctrl Pts',(-9.86290754793137,-12.3252999403061,
118.184825396801)) ;
#190815=CARTESIAN_POINT('Ctrl Pts',(-9.93671141720893,-12.3252999104375,
118.160594433873)) ;
#190816=CARTESIAN_POINT('Ctrl Pts',(-9.94475629597229,-12.3966946761742,
118.185097834847)) ;
#190817=CARTESIAN_POINT('Ctrl Pts',(-9.85341967036429,-12.5338429010278,
117.942589305257)) ;
#190818=CARTESIAN_POINT('Ctrl Pts',(-9.8671146551736,-12.5957672263305,
117.984302017465)) ;
#190819=CARTESIAN_POINT('Ctrl Pts',(-9.79331078750242,-12.5957672815326,
118.008532985286)) ;
#190820=CARTESIAN_POINT('Ctrl Pts',(-9.71950691983124,-12.5957673367347,
118.032763953106)) ;
#190821=CARTESIAN_POINT('Ctrl Pts',(-9.70581193502193,-12.533843011432,
117.991051240898)) ;
#190822=CARTESIAN_POINT('Ctrl Pts',(-9.69211695021262,-12.4719186861293,
117.94933852869)) ;
#190823=CARTESIAN_POINT('Ctrl Pts',(-9.7659208178838,-12.4719186309272,
117.92510756087)) ;
#190824=CARTESIAN_POINT('Ctrl Pts',(-9.83972468555498,-12.4719185757251,
117.900876593049)) ;
#190825=CARTESIAN_POINT('Ctrl Pts',(-9.85341967036429,-12.5338429010278,
117.942589305257)) ;
#190826=CARTESIAN_POINT('Ctrl Pts',(-9.77721000168019,-12.7326606979156,
117.745753431851)) ;
#190827=CARTESIAN_POINT('Ctrl Pts',(-9.79551548151559,-12.780794213553,
117.801508967934)) ;
#190828=CARTESIAN_POINT('Ctrl Pts',(-9.72171161855032,-12.7807942904156,
117.825739950088)) ;
#190829=CARTESIAN_POINT('Ctrl Pts',(-9.64790775558505,-12.7807943672782,
117.849970932242)) ;
#190830=CARTESIAN_POINT('Ctrl Pts',(-9.62960227574966,-12.7326608516408,
117.794215396159)) ;
#190831=CARTESIAN_POINT('Ctrl Pts',(-9.61129679591425,-12.6845273360034,
117.738459860075)) ;
#190832=CARTESIAN_POINT('Ctrl Pts',(-9.68510065887952,-12.6845272591408,
117.714228877921)) ;
#190833=CARTESIAN_POINT('Ctrl Pts',(-9.75890452184478,-12.6845271822782,
117.689997895767)) ;
#190834=CARTESIAN_POINT('Ctrl Pts',(-9.77721000168019,-12.7326606979156,
117.745753431851)) ;
#190835=CARTESIAN_POINT('Ctrl Pts',(-9.71941528284546,-12.9811862243396,
117.605182017047)) ;
#190836=CARTESIAN_POINT('Ctrl Pts',(-9.74104880236432,-13.0120391573078,
117.671074224952)) ;
#190837=CARTESIAN_POINT('Ctrl Pts',(-9.66724494595711,-13.0120392516688,
117.69530522708)) ;
#190838=CARTESIAN_POINT('Ctrl Pts',(-9.5934410895499,-13.0120393460298,
117.719536229209)) ;
#190839=CARTESIAN_POINT('Ctrl Pts',(-9.57180757003104,-12.9811864130616,
117.653644021304)) ;
#190840=CARTESIAN_POINT('Ctrl Pts',(-9.55017405051217,-12.9503334800935,
117.587751813399)) ;
#190841=CARTESIAN_POINT('Ctrl Pts',(-9.62397790691939,-12.9503333857324,
117.56352081127)) ;
#190842=CARTESIAN_POINT('Ctrl Pts',(-9.6977817633266,-12.9503332913714,
117.539289809141)) ;
#190843=CARTESIAN_POINT('Ctrl Pts',(-9.71941528284546,-12.9811862243396,
117.605182017047)) ;
#190844=CARTESIAN_POINT('Ctrl Pts',(-9.68389597109276,-13.260918115125,
117.532433827482)) ;
#190845=CARTESIAN_POINT('Ctrl Pts',(-9.70730780262489,-13.2722865612631,
117.603742486795)) ;
#190846=CARTESIAN_POINT('Ctrl Pts',(-9.63350395438863,-13.2722866661501,
117.627973513811)) ;
#190847=CARTESIAN_POINT('Ctrl Pts',(-9.55970010615233,-13.2722867710372,
117.652204540827)) ;
#190848=CARTESIAN_POINT('Ctrl Pts',(-9.53628827462019,-13.2609183248991,
117.580895881514)) ;
#190849=CARTESIAN_POINT('Ctrl Pts',(-9.51287644308806,-13.249549878761,
117.509587222201)) ;
#190850=CARTESIAN_POINT('Ctrl Pts',(-9.58668029132435,-13.249549773874,
117.485356195185)) ;
#190851=CARTESIAN_POINT('Ctrl Pts',(-9.66048413956062,-13.249549668987,
117.461125168169)) ;
#190852=CARTESIAN_POINT('Ctrl Pts',(-9.68389597109276,-13.260918115125,
117.532433827482)) ;
#190853=CARTESIAN_POINT('Ctrl Pts',(-9.67242963948662,-13.5531074788782,
117.533099665877)) ;
#190854=CARTESIAN_POINT('Ctrl Pts',(-9.69594021851786,-13.5440933427765,
117.604709094102)) ;
#190855=CARTESIAN_POINT('Ctrl Pts',(-9.62213637927301,-13.5440934499071,
117.628940148505)) ;
#190856=CARTESIAN_POINT('Ctrl Pts',(-9.54833254002818,-13.5440935570377,
117.653171202907)) ;
#190857=CARTESIAN_POINT('Ctrl Pts',(-9.52482196099694,-13.5531076931393,
117.581561774682)) ;
#190858=CARTESIAN_POINT('Ctrl Pts',(-9.5013113819657,-13.5621218292409,
117.509952346458)) ;
#190859=CARTESIAN_POINT('Ctrl Pts',(-9.57511522121055,-13.5621217221104,
117.485721292055)) ;
#190860=CARTESIAN_POINT('Ctrl Pts',(-9.64891906045538,-13.5621216149798,
117.461490237653)) ;
#190861=CARTESIAN_POINT('Ctrl Pts',(-9.67242963948662,-13.5531074788782,
117.533099665877)) ;
#190862=CARTESIAN_POINT('Ctrl Pts',(-9.68511244301849,-13.8336246591284,
117.607072550047)) ;
#190863=CARTESIAN_POINT('Ctrl Pts',(-9.70704089076989,-13.8050124160848,
117.673863061661)) ;
#190864=CARTESIAN_POINT('Ctrl Pts',(-9.63323706028518,-13.805012516226,
117.698094142745)) ;
#190865=CARTESIAN_POINT('Ctrl Pts',(-9.55943322980046,-13.8050126163672,
117.72232522383)) ;
#190866=CARTESIAN_POINT('Ctrl Pts',(-9.53750478204908,-13.8336248594109,
117.655534712216)) ;
#190867=CARTESIAN_POINT('Ctrl Pts',(-9.51557633429766,-13.8622371024545,
117.588744200601)) ;
#190868=CARTESIAN_POINT('Ctrl Pts',(-9.58938016478238,-13.8622370023133,
117.564513119517)) ;
#190869=CARTESIAN_POINT('Ctrl Pts',(-9.66318399526709,-13.8622369021721,
117.540282038433)) ;
#190870=CARTESIAN_POINT('Ctrl Pts',(-9.68511244301849,-13.8336246591284,
117.607072550047)) ;
#190871=CARTESIAN_POINT('Ctrl Pts',(-9.7201246877408,-14.0853767704005,
117.749151870546)) ;
#190872=CARTESIAN_POINT('Ctrl Pts',(-9.73890794499503,-14.0391458019482,
117.806362639386)) ;
#190873=CARTESIAN_POINT('Ctrl Pts',(-9.66510412230631,-14.0391458872152,
117.830593744216)) ;
#190874=CARTESIAN_POINT('Ctrl Pts',(-9.59130029961758,-14.0391459724823,
117.854824849046)) ;
#190875=CARTESIAN_POINT('Ctrl Pts',(-9.57251704236337,-14.0853769409346,
117.797614080206)) ;
#190876=CARTESIAN_POINT('Ctrl Pts',(-9.55373378510916,-14.131607909387,
117.740403311365)) ;
#190877=CARTESIAN_POINT('Ctrl Pts',(-9.62753760779788,-14.1316078241199,
117.716172206536)) ;
#190878=CARTESIAN_POINT('Ctrl Pts',(-9.70134143048658,-14.1316077388528,
117.691941101706)) ;
#190879=CARTESIAN_POINT('Ctrl Pts',(-9.7201246877408,-14.0853767704005,
117.749151870546)) ;
#190880=CARTESIAN_POINT('Ctrl Pts',(-9.77484710365909,-14.2903978532202,
117.951517261547)) ;
#190881=CARTESIAN_POINT('Ctrl Pts',(-9.7890995255308,-14.2297838798409,
117.994927836903)) ;
#190882=CARTESIAN_POINT('Ctrl Pts',(-9.71529570863531,-14.2297839428811,
118.019158959378)) ;
#190883=CARTESIAN_POINT('Ctrl Pts',(-9.6414918917398,-14.2297840059213,
118.043390081853)) ;
#190884=CARTESIAN_POINT('Ctrl Pts',(-9.62723946986811,-14.2903979793006,
117.999979506497)) ;
#190885=CARTESIAN_POINT('Ctrl Pts',(-9.61298704799638,-14.3510119526798,
117.95656893114)) ;
#190886=CARTESIAN_POINT('Ctrl Pts',(-9.68679086489188,-14.3510118896396,
117.932337808665)) ;
#190887=CARTESIAN_POINT('Ctrl Pts',(-9.76059468178738,-14.3510118265994,
117.90810668619)) ;
#190888=CARTESIAN_POINT('Ctrl Pts',(-9.77484710365909,-14.2903978532202,
117.951517261547)) ;
#190889=CARTESIAN_POINT('Ctrl Pts',(-9.84334910457871,-14.430884933304,
118.195415358412)) ;
#190890=CARTESIAN_POINT('Ctrl Pts',(-9.8521105935028,-14.36037249955,118.222101438012)) ;
#190891=CARTESIAN_POINT('Ctrl Pts',(-9.77830678021269,-14.3603725370538,
118.246332571468)) ;
#190892=CARTESIAN_POINT('Ctrl Pts',(-9.70450296692257,-14.3603725745575,
118.270563704924)) ;
#190893=CARTESIAN_POINT('Ctrl Pts',(-9.69574147799849,-14.4308850083114,
118.243877625325)) ;
#190894=CARTESIAN_POINT('Ctrl Pts',(-9.6869799890744,-14.5013974420654,
118.217191545725)) ;
#190895=CARTESIAN_POINT('Ctrl Pts',(-9.76078380236452,-14.5013974045617,
118.192960412269)) ;
#190896=CARTESIAN_POINT('Ctrl Pts',(-9.83458761565463,-14.501397367058,
118.168729278813)) ;
#190897=CARTESIAN_POINT('Ctrl Pts',(-9.84334910457871,-14.430884933304,
118.195415358412)) ;
#190898=CARTESIAN_POINT('Ctrl Pts',(-9.92122616212989,-14.5000545452193,
118.468156118046)) ;
#190899=CARTESIAN_POINT('Ctrl Pts',(-9.92382827917419,-14.4246071586731,
118.47608174479)) ;
#190900=CARTESIAN_POINT('Ctrl Pts',(-9.85002446664451,-14.4246071686467,
118.500312880563)) ;
#190901=CARTESIAN_POINT('Ctrl Pts',(-9.77622065411485,-14.4246071786203,
118.524544016335)) ;
#190902=CARTESIAN_POINT('Ctrl Pts',(-9.77361853707056,-14.5000545651665,
118.516618389591)) ;
#190903=CARTESIAN_POINT('Ctrl Pts',(-9.77101642002627,-14.5755019517128,
118.508692762847)) ;
#190904=CARTESIAN_POINT('Ctrl Pts',(-9.84482023255593,-14.5755019417391,
118.484461627074)) ;
#190905=CARTESIAN_POINT('Ctrl Pts',(-9.9186240450856,-14.5755019317655,
118.460230491302)) ;
#190906=CARTESIAN_POINT('Ctrl Pts',(-9.92122616212989,-14.5000545452193,
118.468156118046)) ;
#190907=CARTESIAN_POINT('Ctrl Pts',(-10.0013588136134,-14.4915166284975,
118.74761997857)) ;
#190908=CARTESIAN_POINT('Ctrl Pts',(-9.99763779706234,-14.4165522893736,
118.736286360703)) ;
#190909=CARTESIAN_POINT('Ctrl Pts',(-9.9238339828673,-14.4165522733908,
118.760517491403)) ;
#190910=CARTESIAN_POINT('Ctrl Pts',(-9.85003016867226,-14.4165522574081,
118.784748622103)) ;
#190911=CARTESIAN_POINT('Ctrl Pts',(-9.85375118522337,-14.491516596532,
118.796082239971)) ;
#190912=CARTESIAN_POINT('Ctrl Pts',(-9.85747220177447,-14.566480935656,
118.807415857838)) ;
#190913=CARTESIAN_POINT('Ctrl Pts',(-9.93127601596952,-14.5664809516387,
118.783184727138)) ;
#190914=CARTESIAN_POINT('Ctrl Pts',(-10.0050798301646,-14.5664809676215,
118.758953596437)) ;
#190915=CARTESIAN_POINT('Ctrl Pts',(-10.0013588136134,-14.4915166284975,
118.74761997857)) ;
#190916=CARTESIAN_POINT('Ctrl Pts',(-10.0779474866917,-14.4057133919849,
119.016492386824)) ;
#190917=CARTESIAN_POINT('Ctrl Pts',(-10.0681370537657,-14.3366264116548,
118.986611389331)) ;
#190918=CARTESIAN_POINT('Ctrl Pts',(-9.99433323529747,-14.3366263740412,
119.010842507016)) ;
#190919=CARTESIAN_POINT('Ctrl Pts',(-9.92052941682924,-14.3366263364276,
119.035073624701)) ;
#190920=CARTESIAN_POINT('Ctrl Pts',(-9.93033984975523,-14.4057133167577,
119.064954622193)) ;
#190921=CARTESIAN_POINT('Ctrl Pts',(-9.94015028268123,-14.4748002970877,
119.094835619686)) ;
#190922=CARTESIAN_POINT('Ctrl Pts',(-10.0139541011495,-14.4748003347014,
119.070604502001)) ;
#190923=CARTESIAN_POINT('Ctrl Pts',(-10.0877579196177,-14.474800372315,
119.046373384316)) ;
#190924=CARTESIAN_POINT('Ctrl Pts',(-10.0779474866917,-14.4057133919849,
119.016492386824)) ;
#190925=CARTESIAN_POINT('Ctrl Pts',(-10.1439356362234,-14.2496052022137,
119.252877640221)) ;
#190926=CARTESIAN_POINT('Ctrl Pts',(-10.1287707813893,-14.1913134689692,
119.206687937649)) ;
#190927=CARTESIAN_POINT('Ctrl Pts',(-10.0549669574364,-14.1913134155293,
119.230919038628)) ;
#190928=CARTESIAN_POINT('Ctrl Pts',(-9.98116313348346,-14.1913133620894,
119.255150139607)) ;
#190929=CARTESIAN_POINT('Ctrl Pts',(-9.9963279883176,-14.2496050953339,
119.30133984218)) ;
#190930=CARTESIAN_POINT('Ctrl Pts',(-10.0114928431517,-14.3078968285784,
119.347529544752)) ;
#190931=CARTESIAN_POINT('Ctrl Pts',(-10.0852966671046,-14.3078968820183,
119.323298443772)) ;
#190932=CARTESIAN_POINT('Ctrl Pts',(-10.1591004910575,-14.3078969354582,
119.299067342793)) ;
#190933=CARTESIAN_POINT('Ctrl Pts',(-10.1439356362234,-14.2496052022137,
119.252877640221)) ;
#190934=CARTESIAN_POINT('Ctrl Pts',(-10.1943912071192,-14.0337448610519,
119.442029357324)) ;
#190935=CARTESIAN_POINT('Ctrl Pts',(-10.1749466541285,-13.9904362158164,
119.382804384838)) ;
#190936=CARTESIAN_POINT('Ctrl Pts',(-10.1011428237473,-13.9904361538178,
119.407035466237)) ;
#190937=CARTESIAN_POINT('Ctrl Pts',(-10.027338993366,-13.9904360918192,
119.431266547637)) ;
#190938=CARTESIAN_POINT('Ctrl Pts',(-10.0467835463566,-14.0337447370547,
119.490491520124)) ;
#190939=CARTESIAN_POINT('Ctrl Pts',(-10.0662280993472,-14.0770533822902,
119.54971649261)) ;
#190940=CARTESIAN_POINT('Ctrl Pts',(-10.1400319297285,-14.0770534442888,
119.525485411211)) ;
#190941=CARTESIAN_POINT('Ctrl Pts',(-10.2138357601098,-14.0770535062874,
119.501254329811)) ;
#190942=CARTESIAN_POINT('Ctrl Pts',(-10.1943912071192,-14.0337448610519,
119.442029357324)) ;
#190943=CARTESIAN_POINT('Ctrl Pts',(-10.2248051700175,-13.774289830103,
119.570067049263)) ;
#190944=CARTESIAN_POINT('Ctrl Pts',(-10.2024751831986,-13.7490307967716,
119.50205351104)) ;
#190945=CARTESIAN_POINT('Ctrl Pts',(-10.1286713464233,-13.7490307328435,
119.526284572964)) ;
#190946=CARTESIAN_POINT('Ctrl Pts',(-10.0548675096479,-13.7490306689154,
119.550515634889)) ;
#190947=CARTESIAN_POINT('Ctrl Pts',(-10.0771974964669,-13.7742897022469,
119.618529173111)) ;
#190948=CARTESIAN_POINT('Ctrl Pts',(-10.0995274832858,-13.7995487355784,
119.686542711334)) ;
#190949=CARTESIAN_POINT('Ctrl Pts',(-10.1733313200612,-13.7995487995064,
119.66231164941)) ;
#190950=CARTESIAN_POINT('Ctrl Pts',(-10.2471351568365,-13.7995488634345,
119.638080587485)) ;
#190951=CARTESIAN_POINT('Ctrl Pts',(-10.2248051700175,-13.774289830103,
119.570067049263)) ;
#190952=CARTESIAN_POINT('Ctrl Pts',(-10.2322343776425,-13.4875484100679,
119.628322764206)) ;
#190953=CARTESIAN_POINT('Ctrl Pts',(-10.2086144448205,-13.4822714043299,
119.556380258782)) ;
#190954=CARTESIAN_POINT('Ctrl Pts',(-10.1348106023241,-13.4822713469427,
119.580611303281)) ;
#190955=CARTESIAN_POINT('Ctrl Pts',(-10.0610067598278,-13.4822712895556,
119.60484234778)) ;
#190956=CARTESIAN_POINT('Ctrl Pts',(-10.0846266926498,-13.4875482952936,
119.676784853204)) ;
#190957=CARTESIAN_POINT('Ctrl Pts',(-10.1082466254719,-13.4928253010316,
119.748727358628)) ;
#190958=CARTESIAN_POINT('Ctrl Pts',(-10.1820504679682,-13.4928253584187,
119.724496314129)) ;
#190959=CARTESIAN_POINT('Ctrl Pts',(-10.2558543104646,-13.4928254158059,
119.70026526963)) ;
#190960=CARTESIAN_POINT('Ctrl Pts',(-10.2322343776425,-13.4875484100679,
119.628322764206)) ;
#190961=CARTESIAN_POINT('Ctrl Pts',(-10.2155030787286,-13.1987144632943,
119.612621471267)) ;
#190962=CARTESIAN_POINT('Ctrl Pts',(-10.1922860890302,-13.2135962190273,
119.541906265711)) ;
#190963=CARTESIAN_POINT('Ctrl Pts',(-10.1184822422072,-13.2135961694435,
119.566137297032)) ;
#190964=CARTESIAN_POINT('Ctrl Pts',(-10.0446783953842,-13.2135961198597,
119.590368328353)) ;
#190965=CARTESIAN_POINT('Ctrl Pts',(-10.0678953850826,-13.1987143641267,
119.661083533908)) ;
#190966=CARTESIAN_POINT('Ctrl Pts',(-10.091112374781,-13.1838326083937,
119.731798739464)) ;
#190967=CARTESIAN_POINT('Ctrl Pts',(-10.164916221604,-13.1838326579775,
119.707567708143)) ;
#190968=CARTESIAN_POINT('Ctrl Pts',(-10.238720068427,-13.1838327075613,
119.683336676822)) ;
#190969=CARTESIAN_POINT('Ctrl Pts',(-10.2155030787286,-13.1987144632943,
119.612621471267)) ;
#190970=CARTESIAN_POINT('Ctrl Pts',(-10.1748040815892,-12.9229602452279,
119.524251932971)) ;
#190971=CARTESIAN_POINT('Ctrl Pts',(-10.1536568930331,-12.9571183444642,
119.459841007927)) ;
#190972=CARTESIAN_POINT('Ctrl Pts',(-10.0798530435771,-12.9571183085152,
119.484072031228)) ;
#190973=CARTESIAN_POINT('Ctrl Pts',(-10.0060491941211,-12.9571182725662,
119.508303054529)) ;
#190974=CARTESIAN_POINT('Ctrl Pts',(-10.0271963826772,-12.9229601733299,
119.572713979573)) ;
#190975=CARTESIAN_POINT('Ctrl Pts',(-10.0483435712333,-12.8888020740936,
119.637124904618)) ;
#190976=CARTESIAN_POINT('Ctrl Pts',(-10.1221474206893,-12.8888021100426,
119.612893881317)) ;
#190977=CARTESIAN_POINT('Ctrl Pts',(-10.1959512701453,-12.8888021459916,
119.588662858015)) ;
#190978=CARTESIAN_POINT('Ctrl Pts',(-10.1748040815892,-12.9229602452279,
119.524251932971)) ;
#190979=CARTESIAN_POINT('Ctrl Pts',(-10.1124465818058,-12.6836290013039,
119.36980293551)) ;
#190980=CARTESIAN_POINT('Ctrl Pts',(-10.0948870427062,-12.7345497889164,
119.316319412014)) ;
#190981=CARTESIAN_POINT('Ctrl Pts',(-10.0210831923806,-12.7345497658022,
119.340550432667)) ;
#190982=CARTESIAN_POINT('Ctrl Pts',(-9.94727934205508,-12.734549742688,
119.36478145332)) ;
#190983=CARTESIAN_POINT('Ctrl Pts',(-9.9648388811547,-12.6836289550754,
119.418264976815)) ;
#190984=CARTESIAN_POINT('Ctrl Pts',(-9.98239842025433,-12.6327081674629,
119.471748500311)) ;
#190985=CARTESIAN_POINT('Ctrl Pts',(-10.0562022705799,-12.6327081905771,
119.447517479658)) ;
#190986=CARTESIAN_POINT('Ctrl Pts',(-10.1300061209054,-12.6327082136913,
119.423286459006)) ;
#190987=CARTESIAN_POINT('Ctrl Pts',(-10.1124465818058,-12.6836290013039,
119.36980293551)) ;
#190988=CARTESIAN_POINT('Ctrl Pts',(-10.032243567432,-12.4971808863818,
119.160966196631)) ;
#190989=CARTESIAN_POINT('Ctrl Pts',(-10.0195239505098,-12.5611972883497,
119.122224295324)) ;
#190990=CARTESIAN_POINT('Ctrl Pts',(-9.94572010065391,-12.5611972760957,
119.146455317408)) ;
#190991=CARTESIAN_POINT('Ctrl Pts',(-9.87191625079806,-12.5611972638417,
119.170686339491)) ;
#190992=CARTESIAN_POINT('Ctrl Pts',(-9.88463586772028,-12.4971808618738,
119.209428240797)) ;
#190993=CARTESIAN_POINT('Ctrl Pts',(-9.89735548464251,-12.4331644599059,
119.248170142104)) ;
#190994=CARTESIAN_POINT('Ctrl Pts',(-9.97115933449836,-12.4331644721599,
119.22393912002)) ;
#190995=CARTESIAN_POINT('Ctrl Pts',(-10.0449631843542,-12.4331644844139,
119.199708097937)) ;
#190996=CARTESIAN_POINT('Ctrl Pts',(-10.032243567432,-12.4971808863818,
119.160966196631)) ;
#190997=CARTESIAN_POINT('Ctrl Pts',(-9.93941244595383,-12.3766482309411,
118.91356140389)) ;
#190998=CARTESIAN_POINT('Ctrl Pts',(-9.93242405862038,-12.4491772372763,
118.89227590331)) ;
#190999=CARTESIAN_POINT('Ctrl Pts',(-9.85862020998783,-12.4491772329469,
118.916506929119)) ;
#191000=CARTESIAN_POINT('Ctrl Pts',(-9.78481636135525,-12.4491772286174,
118.940737954929)) ;
#191001=CARTESIAN_POINT('Ctrl Pts',(-9.7918047486887,-12.3766482222823,
118.962023455509)) ;
#191002=CARTESIAN_POINT('Ctrl Pts',(-9.79879313602213,-12.3041192159472,
118.983308956088)) ;
#191003=CARTESIAN_POINT('Ctrl Pts',(-9.87259698465468,-12.3041192202766,
118.959077930279)) ;
#191004=CARTESIAN_POINT('Ctrl Pts',(-9.94640083328725,-12.304119224606,
118.93484690447)) ;
#191005=CARTESIAN_POINT('Ctrl Pts',(-9.93941244595383,-12.3766482309411,
118.91356140389)) ;
#191006=CARTESIAN_POINT('Ctrl Pts',(-9.83867669766088,-12.3303160635296,
118.642394997812)) ;
#191007=CARTESIAN_POINT('Ctrl Pts',(-9.83797380881755,-12.406190350598,
118.640254111632)) ;
#191008=CARTESIAN_POINT('Ctrl Pts',(-9.76416996259023,-12.4061903509704,
118.664485144767)) ;
#191009=CARTESIAN_POINT('Ctrl Pts',(-9.69036611636291,-12.4061903513427,
118.688716177902)) ;
#191010=CARTESIAN_POINT('Ctrl Pts',(-9.69106900520625,-12.3303160642744,
118.690857064083)) ;
#191011=CARTESIAN_POINT('Ctrl Pts',(-9.69177189404958,-12.254441777206,
118.692997950263)) ;
#191012=CARTESIAN_POINT('Ctrl Pts',(-9.7655757402769,-12.2544417768337,
118.668766917128)) ;
#191013=CARTESIAN_POINT('Ctrl Pts',(-9.8393795865042,-12.2544417764613,
118.644535883993)) ;
#191014=CARTESIAN_POINT('Ctrl Pts',(-9.83867669766088,-12.3303160635296,
118.642394997812)) ;
#191015=CARTESIAN_POINT('Ctrl Pts',(-9.73837574668705,-12.3620878034078,
118.372182541714)) ;
#191016=CARTESIAN_POINT('Ctrl Pts',(-9.74394510030878,-12.4358572257211,
118.389145894146)) ;
#191017=CARTESIAN_POINT('Ctrl Pts',(-9.67014125555776,-12.435857227174,
118.413376931778)) ;
#191018=CARTESIAN_POINT('Ctrl Pts',(-9.59633741080671,-12.4358572286269,
118.43760796941)) ;
#191019=CARTESIAN_POINT('Ctrl Pts',(-9.59076805718501,-12.3620878063136,
118.420644616978)) ;
#191020=CARTESIAN_POINT('Ctrl Pts',(-9.58519870356327,-12.2883183840004,
118.403681264546)) ;
#191021=CARTESIAN_POINT('Ctrl Pts',(-9.65900254831429,-12.2883183825475,
118.379450226914)) ;
#191022=CARTESIAN_POINT('Ctrl Pts',(-9.73280639306531,-12.2883183810946,
118.355219189282)) ;
#191023=CARTESIAN_POINT('Ctrl Pts',(-9.73837574668705,-12.3620878034078,
118.372182541714)) ;
#191024=CARTESIAN_POINT('Ctrl Pts',(-9.64331761099955,-12.4693107333451,
118.118151143645)) ;
#191025=CARTESIAN_POINT('Ctrl Pts',(-9.65479830623516,-12.5357038324563,
118.153119488932)) ;
#191026=CARTESIAN_POINT('Ctrl Pts',(-9.58099446292707,-12.5357038327128,
118.177350530959)) ;
#191027=CARTESIAN_POINT('Ctrl Pts',(-9.50719061961899,-12.5357038329694,
118.201581572986)) ;
#191028=CARTESIAN_POINT('Ctrl Pts',(-9.49570992438338,-12.4693107338582,
118.166613227698)) ;
#191029=CARTESIAN_POINT('Ctrl Pts',(-9.48422922914777,-12.402917634747,
118.131644882411)) ;
#191030=CARTESIAN_POINT('Ctrl Pts',(-9.55803307245587,-12.4029176344904,
118.107413840384)) ;
#191031=CARTESIAN_POINT('Ctrl Pts',(-9.63183691576394,-12.4029176342339,
118.083182798358)) ;
#191032=CARTESIAN_POINT('Ctrl Pts',(-9.64331761099955,-12.4693107333451,
118.118151143645)) ;
#191033=CARTESIAN_POINT('Ctrl Pts',(-9.56006119087889,-12.645191135036,
117.900125999057)) ;
#191034=CARTESIAN_POINT('Ctrl Pts',(-9.57663687909926,-12.6994019736038,
117.950612870956)) ;
#191035=CARTESIAN_POINT('Ctrl Pts',(-9.50283303638179,-12.6994019715653,
117.974843914782)) ;
#191036=CARTESIAN_POINT('Ctrl Pts',(-9.42902919366433,-12.6994019695268,
117.999074958608)) ;
#191037=CARTESIAN_POINT('Ctrl Pts',(-9.41245350544398,-12.6451911309591,
117.948588086708)) ;
#191038=CARTESIAN_POINT('Ctrl Pts',(-9.39587781722363,-12.5909802923914,
117.898101214808)) ;
#191039=CARTESIAN_POINT('Ctrl Pts',(-9.46968165994109,-12.5909802944298,
117.873870170982)) ;
#191040=CARTESIAN_POINT('Ctrl Pts',(-9.54348550265856,-12.5909802964683,
117.849639127157)) ;
#191041=CARTESIAN_POINT('Ctrl Pts',(-9.56006119087889,-12.645191135036,
117.900125999057)) ;
#191042=CARTESIAN_POINT('Ctrl Pts',(-9.49421241414551,-12.8761323945115,
117.735033267654)) ;
#191043=CARTESIAN_POINT('Ctrl Pts',(-9.51467678263965,-12.9142969383445,
117.797364432234)) ;
#191044=CARTESIAN_POINT('Ctrl Pts',(-9.44087293971269,-12.9142969355883,
117.821595475422)) ;
#191045=CARTESIAN_POINT('Ctrl Pts',(-9.3670690967857,-12.9142969328321,
117.84582651861)) ;
#191046=CARTESIAN_POINT('Ctrl Pts',(-9.34660472829156,-12.8761323889991,
117.783495354029)) ;
#191047=CARTESIAN_POINT('Ctrl Pts',(-9.32614035979739,-12.8379678451661,
117.721164189449)) ;
#191048=CARTESIAN_POINT('Ctrl Pts',(-9.39994420272437,-12.8379678479223,
117.696933146261)) ;
#191049=CARTESIAN_POINT('Ctrl Pts',(-9.47374804565133,-12.8379678506785,
117.672702103074)) ;
#191050=CARTESIAN_POINT('Ctrl Pts',(-9.49421241414551,-12.8761323945115,
117.735033267654)) ;
#191051=CARTESIAN_POINT('Ctrl Pts',(-9.44952047826331,-13.1443073603244,
117.634195686389)) ;
#191052=CARTESIAN_POINT('Ctrl Pts',(-9.47240530569183,-13.1638021990363,
117.703899178321)) ;
#191053=CARTESIAN_POINT('Ctrl Pts',(-9.39860146235271,-13.16380219707,117.728130220253)) ;
#191054=CARTESIAN_POINT('Ctrl Pts',(-9.32479761901359,-13.1638021951038,
117.752361262185)) ;
#191055=CARTESIAN_POINT('Ctrl Pts',(-9.30191279158505,-13.1443073563919,
117.682657770253)) ;
#191056=CARTESIAN_POINT('Ctrl Pts',(-9.27902796415653,-13.12481251768,117.612954278321)) ;
#191057=CARTESIAN_POINT('Ctrl Pts',(-9.35283180749566,-13.1248125196462,
117.588723236389)) ;
#191058=CARTESIAN_POINT('Ctrl Pts',(-9.42663565083478,-13.1248125216125,
117.564492194457)) ;
#191059=CARTESIAN_POINT('Ctrl Pts',(-9.44952047826331,-13.1443073603244,
117.634195686389)) ;
#191060=CARTESIAN_POINT('Ctrl Pts',(-9.42806301659363,-13.4354170804365,
117.604552144975)) ;
#191061=CARTESIAN_POINT('Ctrl Pts',(-9.45174090939818,-13.4346128293488,
117.676671185992)) ;
#191062=CARTESIAN_POINT('Ctrl Pts',(-9.37793706587032,-13.4346128319822,
117.70090222735)) ;
#191063=CARTESIAN_POINT('Ctrl Pts',(-9.30413322234245,-13.4346128346157,
117.725133268707)) ;
#191064=CARTESIAN_POINT('Ctrl Pts',(-9.28045532953792,-13.4354170857033,
117.653014227689)) ;
#191065=CARTESIAN_POINT('Ctrl Pts',(-9.25677743673337,-13.436221336791,
117.580895186672)) ;
#191066=CARTESIAN_POINT('Ctrl Pts',(-9.33058128026124,-13.4362213341576,
117.556664145314)) ;
#191067=CARTESIAN_POINT('Ctrl Pts',(-9.40438512378909,-13.4362213315242,
117.532433103957)) ;
#191068=CARTESIAN_POINT('Ctrl Pts',(-9.42806301659363,-13.4354170804365,
117.604552144975)) ;
#191069=CARTESIAN_POINT('Ctrl Pts',(-9.43113345781473,-13.7221366616439,
117.649216366819)) ;
#191070=CARTESIAN_POINT('Ctrl Pts',(-9.45390061019574,-13.7013113003572,
117.718561439368)) ;
#191071=CARTESIAN_POINT('Ctrl Pts',(-9.38009676726755,-13.7013113073341,
117.742792482551)) ;
#191072=CARTESIAN_POINT('Ctrl Pts',(-9.30629292433936,-13.7013113143109,
117.767023525735)) ;
#191073=CARTESIAN_POINT('Ctrl Pts',(-9.28352577195833,-13.7221366755976,
117.697678453187)) ;
#191074=CARTESIAN_POINT('Ctrl Pts',(-9.26075861957731,-13.7429620368844,
117.628333380638)) ;
#191075=CARTESIAN_POINT('Ctrl Pts',(-9.3345624625055,-13.7429620299075,
117.604102337454)) ;
#191076=CARTESIAN_POINT('Ctrl Pts',(-9.4083663054337,-13.7429620229307,
117.57987129427)) ;
#191077=CARTESIAN_POINT('Ctrl Pts',(-9.43113345781473,-13.7221366616439,
117.649216366819)) ;
#191078=CARTESIAN_POINT('Ctrl Pts',(-9.45742319346762,-13.9882040306806,
117.764746473513)) ;
#191079=CARTESIAN_POINT('Ctrl Pts',(-9.47765409992438,-13.948770536174,
117.826366550077)) ;
#191080=CARTESIAN_POINT('Ctrl Pts',(-9.40385025854739,-13.9487705477941,
117.850597597986)) ;
#191081=CARTESIAN_POINT('Ctrl Pts',(-9.33004641717041,-13.9487705594142,
117.874828645894)) ;
#191082=CARTESIAN_POINT('Ctrl Pts',(-9.30981551071365,-13.9882040539209,
117.81320856933)) ;
#191083=CARTESIAN_POINT('Ctrl Pts',(-9.28958460425689,-14.0276375484275,
117.751588492765)) ;
#191084=CARTESIAN_POINT('Ctrl Pts',(-9.36338844563387,-14.0276375368073,
117.727357444856)) ;
#191085=CARTESIAN_POINT('Ctrl Pts',(-9.43719228701085,-14.0276375251872,
117.703126396948)) ;
#191086=CARTESIAN_POINT('Ctrl Pts',(-9.45742319346762,-13.9882040306806,
117.764746473513)) ;
#191087=CARTESIAN_POINT('Ctrl Pts',(-9.50431469901294,-14.2132831582582,
117.942967310221)) ;
#191088=CARTESIAN_POINT('Ctrl Pts',(-9.52056835396493,-14.1580769970448,
117.9924733203)) ;
#191089=CARTESIAN_POINT('Ctrl Pts',(-9.44676451495778,-14.1580770113055,
118.016704375426)) ;
#191090=CARTESIAN_POINT('Ctrl Pts',(-9.37296067595063,-14.1580770255661,
118.040935430553)) ;
#191091=CARTESIAN_POINT('Ctrl Pts',(-9.35670702099861,-14.2132831867795,
117.991429420474)) ;
#191092=CARTESIAN_POINT('Ctrl Pts',(-9.34045336604661,-14.2684893479928,
117.941923410395)) ;
#191093=CARTESIAN_POINT('Ctrl Pts',(-9.41425720505376,-14.2684893337322,
117.917692355268)) ;
#191094=CARTESIAN_POINT('Ctrl Pts',(-9.48806104406092,-14.2684893194715,
117.893461300141)) ;
#191095=CARTESIAN_POINT('Ctrl Pts',(-9.50431469901294,-14.2132831582582,
117.942967310221)) ;
#191096=CARTESIAN_POINT('Ctrl Pts',(-9.56833785438296,-14.3825130038358,
118.17365809311)) ;
#191097=CARTESIAN_POINT('Ctrl Pts',(-9.57940645753599,-14.3154103550948,
118.20737127182)) ;
#191098=CARTESIAN_POINT('Ctrl Pts',(-9.50560262233898,-14.3154103696642,
118.231602338552)) ;
#191099=CARTESIAN_POINT('Ctrl Pts',(-9.43179878714198,-14.3154103842335,
118.255833405283)) ;
#191100=CARTESIAN_POINT('Ctrl Pts',(-9.42073018398896,-14.3825130329745,
118.222120226574)) ;
#191101=CARTESIAN_POINT('Ctrl Pts',(-9.40966158083592,-14.4496156817154,
118.188407047864)) ;
#191102=CARTESIAN_POINT('Ctrl Pts',(-9.48346541603292,-14.4496156671461,
118.164175981132)) ;
#191103=CARTESIAN_POINT('Ctrl Pts',(-9.55726925122993,-14.4496156525767,
118.1399449144)) ;
#191104=CARTESIAN_POINT('Ctrl Pts',(-9.56833785438296,-14.3825130038358,
118.17365809311)) ;
#191105=CARTESIAN_POINT('Ctrl Pts',(-9.64282625620299,-14.4810713491466,
118.435803129355)) ;
#191106=CARTESIAN_POINT('Ctrl Pts',(-9.64798025335909,-14.4069908889082,
118.451501372389)) ;
#191107=CARTESIAN_POINT('Ctrl Pts',(-9.57417642109813,-14.4069908973545,
118.475732448064)) ;
#191108=CARTESIAN_POINT('Ctrl Pts',(-9.50037258883717,-14.4069909058008,
118.499963523738)) ;
#191109=CARTESIAN_POINT('Ctrl Pts',(-9.49521859168107,-14.4810713660392,
118.484265280704)) ;
#191110=CARTESIAN_POINT('Ctrl Pts',(-9.49006459452497,-14.5551518262776,
118.468567037671)) ;
#191111=CARTESIAN_POINT('Ctrl Pts',(-9.56386842678596,-14.5551518178313,
118.444335961996)) ;
#191112=CARTESIAN_POINT('Ctrl Pts',(-9.6376722590469,-14.555151809385,118.420104886322)) ;
#191113=CARTESIAN_POINT('Ctrl Pts',(-9.64282625620299,-14.4810713491466,
118.435803129355)) ;
#191114=CARTESIAN_POINT('Ctrl Pts',(-9.72303088811142,-14.5044054817918,
118.715641377644)) ;
#191115=CARTESIAN_POINT('Ctrl Pts',(-9.72185690535189,-14.4285885279282,
118.712065614687)) ;
#191116=CARTESIAN_POINT('Ctrl Pts',(-9.64805307633812,-14.4285885262166,
118.736296700252)) ;
#191117=CARTESIAN_POINT('Ctrl Pts',(-9.57424924732434,-14.4285885245051,
118.760527785817)) ;
#191118=CARTESIAN_POINT('Ctrl Pts',(-9.57542323008388,-14.5044054783686,
118.764103548774)) ;
#191119=CARTESIAN_POINT('Ctrl Pts',(-9.57659721284341,-14.5802224322322,
118.767679311731)) ;
#191120=CARTESIAN_POINT('Ctrl Pts',(-9.65040104185718,-14.5802224339438,
118.743448226166)) ;
#191121=CARTESIAN_POINT('Ctrl Pts',(-9.72420487087096,-14.5802224356554,
118.719217140601)) ;
#191122=CARTESIAN_POINT('Ctrl Pts',(-9.72303088811142,-14.5044054817918,
118.715641377644)) ;
#191123=CARTESIAN_POINT('Ctrl Pts',(-9.80169380240826,-14.4496129795719,
118.990681507836)) ;
#191124=CARTESIAN_POINT('Ctrl Pts',(-9.79429250812283,-14.377512086332,
118.96813835858)) ;
#191125=CARTESIAN_POINT('Ctrl Pts',(-9.72048868096979,-14.3775120696296,
118.992369449812)) ;
#191126=CARTESIAN_POINT('Ctrl Pts',(-9.64668485381674,-14.3775120529272,
119.016600541045)) ;
#191127=CARTESIAN_POINT('Ctrl Pts',(-9.65408614810217,-14.449612946167,
119.039143690301)) ;
#191128=CARTESIAN_POINT('Ctrl Pts',(-9.66148744238758,-14.5217138394069,
119.061686839557)) ;
#191129=CARTESIAN_POINT('Ctrl Pts',(-9.73529126954064,-14.5217138561093,
119.037455748325)) ;
#191130=CARTESIAN_POINT('Ctrl Pts',(-9.80909509669367,-14.5217138728117,
119.013224657093)) ;
#191131=CARTESIAN_POINT('Ctrl Pts',(-9.80169380240826,-14.4496129795719,
118.990681507836)) ;
#191132=CARTESIAN_POINT('Ctrl Pts',(-9.87269202902114,-14.3209948065222,
119.242404449809)) ;
#191133=CARTESIAN_POINT('Ctrl Pts',(-9.85958903526633,-14.2577695417982,
119.202494843768)) ;
#191134=CARTESIAN_POINT('Ctrl Pts',(-9.78578520837554,-14.257769507085,
119.226725935799)) ;
#191135=CARTESIAN_POINT('Ctrl Pts',(-9.71198138148474,-14.2577694723718,
119.25095702783)) ;
#191136=CARTESIAN_POINT('Ctrl Pts',(-9.72508437523955,-14.3209947370958,
119.290866633871)) ;
#191137=CARTESIAN_POINT('Ctrl Pts',(-9.73818736899434,-14.3842200018198,
119.330776239912)) ;
#191138=CARTESIAN_POINT('Ctrl Pts',(-9.81199119588514,-14.384220036533,
119.306545147881)) ;
#191139=CARTESIAN_POINT('Ctrl Pts',(-9.88579502277594,-14.3842200712462,
119.28231405585)) ;
#191140=CARTESIAN_POINT('Ctrl Pts',(-9.87269202902114,-14.3209948065222,
119.242404449809)) ;
#191141=CARTESIAN_POINT('Ctrl Pts',(-9.93011353231494,-14.1276267553148,
119.452772844541)) ;
#191142=CARTESIAN_POINT('Ctrl Pts',(-9.91224855578811,-14.0778104825488,
119.398359007162)) ;
#191143=CARTESIAN_POINT('Ctrl Pts',(-9.83844472708885,-14.077810428769,
119.422590093684)) ;
#191144=CARTESIAN_POINT('Ctrl Pts',(-9.7646408983896,-14.0778103749893,
119.446821180207)) ;
#191145=CARTESIAN_POINT('Ctrl Pts',(-9.78250587491643,-14.1276266477552,
119.501235017587)) ;
#191146=CARTESIAN_POINT('Ctrl Pts',(-9.80037085144328,-14.1774429205212,
119.555648854967)) ;
#191147=CARTESIAN_POINT('Ctrl Pts',(-9.87417468014253,-14.177442974301,
119.531417768444)) ;
#191148=CARTESIAN_POINT('Ctrl Pts',(-9.94797850884177,-14.1774430280807,
119.507186681921)) ;
#191149=CARTESIAN_POINT('Ctrl Pts',(-9.93011353231494,-14.1276267553148,
119.452772844541)) ;
#191150=CARTESIAN_POINT('Ctrl Pts',(-9.96912456086633,-13.88341485216,119.607067761314)) ;
#191151=CARTESIAN_POINT('Ctrl Pts',(-9.94777603635157,-13.8505765249219,
119.542043598682)) ;
#191152=CARTESIAN_POINT('Ctrl Pts',(-9.8739722037022,-13.8505764535514,
119.566274673173)) ;
#191153=CARTESIAN_POINT('Ctrl Pts',(-9.80016837105283,-13.850576382181,
119.590505747665)) ;
#191154=CARTESIAN_POINT('Ctrl Pts',(-9.82151689556758,-13.8834147094192,
119.655529910297)) ;
#191155=CARTESIAN_POINT('Ctrl Pts',(-9.84286542008233,-13.9162530366573,
119.720554072928)) ;
#191156=CARTESIAN_POINT('Ctrl Pts',(-9.9166692527317,-13.9162531080278,
119.696322998437)) ;
#191157=CARTESIAN_POINT('Ctrl Pts',(-9.99047308538107,-13.9162531793982,
119.672091923946)) ;
#191158=CARTESIAN_POINT('Ctrl Pts',(-9.96912456086633,-13.88341485216,119.607067761314)) ;
#191159=CARTESIAN_POINT('Ctrl Pts',(-9.98608738662717,-13.605636693064,
119.694232674666)) ;
#191160=CARTESIAN_POINT('Ctrl Pts',(-9.96278900243976,-13.5921442428259,
119.623269553942)) ;
#191161=CARTESIAN_POINT('Ctrl Pts',(-9.88898516382017,-13.5921441578331,
119.647500610249)) ;
#191162=CARTESIAN_POINT('Ctrl Pts',(-9.81518132520059,-13.5921440728403,
119.671731666556)) ;
#191163=CARTESIAN_POINT('Ctrl Pts',(-9.83847970938801,-13.6056365230784,
119.74269478728)) ;
#191164=CARTESIAN_POINT('Ctrl Pts',(-9.86177809357544,-13.6191289733166,
119.813657908004)) ;
#191165=CARTESIAN_POINT('Ctrl Pts',(-9.93558193219503,-13.6191290583094,
119.789426851697)) ;
#191166=CARTESIAN_POINT('Ctrl Pts',(-10.0093857708146,-13.6191291433021,
119.76519579539)) ;
#191167=CARTESIAN_POINT('Ctrl Pts',(-9.98608738662717,-13.605636693064,
119.694232674666)) ;
#191168=CARTESIAN_POINT('Ctrl Pts',(-9.97927918663981,-13.3159385103922,
119.708801041575)) ;
#191169=CARTESIAN_POINT('Ctrl Pts',(-9.95569186707513,-13.3226522577716,
119.636957870211)) ;
#191170=CARTESIAN_POINT('Ctrl Pts',(-9.88188802115178,-13.3226521665054,
119.661188904272)) ;
#191171=CARTESIAN_POINT('Ctrl Pts',(-9.80808417522844,-13.3226520752392,
119.685419938333)) ;
#191172=CARTESIAN_POINT('Ctrl Pts',(-9.83167149479313,-13.3159383278597,
119.757263109697)) ;
#191173=CARTESIAN_POINT('Ctrl Pts',(-9.85525881435782,-13.3092245804803,
119.829106281061)) ;
#191174=CARTESIAN_POINT('Ctrl Pts',(-9.92906266028116,-13.3092246717465,
119.804875247)) ;
#191175=CARTESIAN_POINT('Ctrl Pts',(-10.0028665062045,-13.3092247630127,
119.780644212939)) ;
#191176=CARTESIAN_POINT('Ctrl Pts',(-9.97927918663981,-13.3159385103922,
119.708801041575)) ;
#191177=CARTESIAN_POINT('Ctrl Pts',(-9.947822664236,-13.0300093756574,119.6487613202)) ;
#191178=CARTESIAN_POINT('Ctrl Pts',(-9.92565661232397,-13.0566953178852,
119.581247100649)) ;
#191179=CARTESIAN_POINT('Ctrl Pts',(-9.85185275806088,-13.0566952256386,
119.605478109308)) ;
#191180=CARTESIAN_POINT('Ctrl Pts',(-9.7780489037978,-13.0566951333921,
119.629709117968)) ;
#191181=CARTESIAN_POINT('Ctrl Pts',(-9.80021495570981,-13.0300091911643,
119.697223337518)) ;
#191182=CARTESIAN_POINT('Ctrl Pts',(-9.82238100762185,-13.0033232489365,
119.764737557069)) ;
#191183=CARTESIAN_POINT('Ctrl Pts',(-9.89618486188495,-13.003323341183,
119.74050654841)) ;
#191184=CARTESIAN_POINT('Ctrl Pts',(-9.96998871614802,-13.0033234334296,
119.71627553975)) ;
#191185=CARTESIAN_POINT('Ctrl Pts',(-9.947822664236,-13.0300093756574,119.6487613202)) ;
#191186=CARTESIAN_POINT('Ctrl Pts',(-9.8944105320407,-12.7764992730081,
119.521214509144)) ;
#191187=CARTESIAN_POINT('Ctrl Pts',(-9.87521436237714,-12.820923286975,
119.462746071682)) ;
#191188=CARTESIAN_POINT('Ctrl Pts',(-9.80141050039616,-12.8209232050731,
119.486977056834)) ;
#191189=CARTESIAN_POINT('Ctrl Pts',(-9.72760663841516,-12.8209231231712,
119.511208041986)) ;
#191190=CARTESIAN_POINT('Ctrl Pts',(-9.74680280807871,-12.7764991092043,
119.569676479447)) ;
#191191=CARTESIAN_POINT('Ctrl Pts',(-9.76599897774222,-12.7320750952375,
119.628144916909)) ;
#191192=CARTESIAN_POINT('Ctrl Pts',(-9.83980283972324,-12.7320751771394,
119.603913931757)) ;
#191193=CARTESIAN_POINT('Ctrl Pts',(-9.91360670170422,-12.7320752590413,
119.579682946605)) ;
#191194=CARTESIAN_POINT('Ctrl Pts',(-9.8944105320407,-12.7764992730081,
119.521214509144)) ;
#191195=CARTESIAN_POINT('Ctrl Pts',(-9.82070657807217,-12.5655360581605,
119.33234328729)) ;
#191196=CARTESIAN_POINT('Ctrl Pts',(-9.80589079521809,-12.6247539701097,
119.2872168012)) ;
#191197=CARTESIAN_POINT('Ctrl Pts',(-9.73208692613494,-12.6247539044987,
119.31144776472)) ;
#191198=CARTESIAN_POINT('Ctrl Pts',(-9.65828305705181,-12.6247538388877,
119.335678728239)) ;
#191199=CARTESIAN_POINT('Ctrl Pts',(-9.67309883990591,-12.5655359269385,
119.38080521433)) ;
#191200=CARTESIAN_POINT('Ctrl Pts',(-9.68791462276,-12.5063180149893,119.42593170042)) ;
#191201=CARTESIAN_POINT('Ctrl Pts',(-9.76171849184312,-12.5063180806004,
119.4017007369)) ;
#191202=CARTESIAN_POINT('Ctrl Pts',(-9.83552236092627,-12.5063181462114,
119.37746977338)) ;
#191203=CARTESIAN_POINT('Ctrl Pts',(-9.82070657807217,-12.5655360581605,
119.33234328729)) ;
#191204=CARTESIAN_POINT('Ctrl Pts',(-9.73221917304687,-12.4169761529621,
119.098239780795)) ;
#191205=CARTESIAN_POINT('Ctrl Pts',(-9.72282668729767,-12.4866530449287,
119.069631782602)) ;
#191206=CARTESIAN_POINT('Ctrl Pts',(-9.649022813112,-12.4866530028469,119.093862730581)) ;
#191207=CARTESIAN_POINT('Ctrl Pts',(-9.5752189389263,-12.4866529607651,
119.118093678559)) ;
#191208=CARTESIAN_POINT('Ctrl Pts',(-9.58461142467551,-12.4169760687985,
119.146701676752)) ;
#191209=CARTESIAN_POINT('Ctrl Pts',(-9.59400391042471,-12.3472991768318,
119.175309674945)) ;
#191210=CARTESIAN_POINT('Ctrl Pts',(-9.6678077846104,-12.3472992189136,
119.151078726967)) ;
#191211=CARTESIAN_POINT('Ctrl Pts',(-9.74161165879609,-12.3472992609954,
119.126847778988)) ;
#191212=CARTESIAN_POINT('Ctrl Pts',(-9.73221917304687,-12.4169761529621,
119.098239780795)) ;
#191213=CARTESIAN_POINT('Ctrl Pts',(-9.63396562356762,-12.339692635442,
118.834500805048)) ;
#191214=CARTESIAN_POINT('Ctrl Pts',(-9.63068383128753,-12.4148681964576,
118.824504993183)) ;
#191215=CARTESIAN_POINT('Ctrl Pts',(-9.55687995436833,-12.4148681820189,
118.848735932836)) ;
#191216=CARTESIAN_POINT('Ctrl Pts',(-9.48307607744914,-12.4148681675802,
118.872966872488)) ;
#191217=CARTESIAN_POINT('Ctrl Pts',(-9.48635786972923,-12.3396926065646,
118.882962684353)) ;
#191218=CARTESIAN_POINT('Ctrl Pts',(-9.48963966200935,-12.264517045549,
118.892958496218)) ;
#191219=CARTESIAN_POINT('Ctrl Pts',(-9.56344353892853,-12.2645170599877,
118.868727556566)) ;
#191220=CARTESIAN_POINT('Ctrl Pts',(-9.63724741584773,-12.2645170744263,
118.844496616913)) ;
#191221=CARTESIAN_POINT('Ctrl Pts',(-9.63396562356762,-12.339692635442,
118.834500805048)) ;
#191222=CARTESIAN_POINT('Ctrl Pts',(-9.53271625870816,-12.3399218128255,
118.561543074817)) ;
#191223=CARTESIAN_POINT('Ctrl Pts',(-9.53576535287959,-12.4151926619622,
118.570830121603)) ;
#191224=CARTESIAN_POINT('Ctrl Pts',(-9.46196147602193,-12.4151926765907,
118.595061061442)) ;
#191225=CARTESIAN_POINT('Ctrl Pts',(-9.38815759916426,-12.4151926912192,
118.619292001282)) ;
#191226=CARTESIAN_POINT('Ctrl Pts',(-9.38510850499285,-12.3399218420826,
118.610004954497)) ;
#191227=CARTESIAN_POINT('Ctrl Pts',(-9.38205941082139,-12.2646509929459,
118.600717907712)) ;
#191228=CARTESIAN_POINT('Ctrl Pts',(-9.45586328767907,-12.2646509783174,
118.576486967872)) ;
#191229=CARTESIAN_POINT('Ctrl Pts',(-9.52966716453673,-12.2646509636889,
118.552256028032)) ;
#191230=CARTESIAN_POINT('Ctrl Pts',(-9.53271625870816,-12.3399218128255,
118.561543074817)) ;
#191231=CARTESIAN_POINT('Ctrl Pts',(-9.43473348009199,-12.4170982893213,
118.298531776641)) ;
#191232=CARTESIAN_POINT('Ctrl Pts',(-9.44389485074115,-12.4870926783877,
118.326435831388)) ;
#191233=CARTESIAN_POINT('Ctrl Pts',(-9.37009097662917,-12.4870927205449,
118.35066677959)) ;
#191234=CARTESIAN_POINT('Ctrl Pts',(-9.2962871025172,-12.4870927627021,
118.374897727793)) ;
#191235=CARTESIAN_POINT('Ctrl Pts',(-9.28712573186802,-12.4170983736357,
118.346993673047)) ;
#191236=CARTESIAN_POINT('Ctrl Pts',(-9.27796436121887,-12.3471039845693,
118.319089618301)) ;
#191237=CARTESIAN_POINT('Ctrl Pts',(-9.35176823533084,-12.3471039424121,
118.294858670098)) ;
#191238=CARTESIAN_POINT('Ctrl Pts',(-9.42557210944283,-12.3471039002549,
118.270627721895)) ;
#191239=CARTESIAN_POINT('Ctrl Pts',(-9.43473348009199,-12.4170982893213,
118.298531776641)) ;
#191240=CARTESIAN_POINT('Ctrl Pts',(-9.34612142005041,-12.5661915214183,
118.064123452786)) ;
#191241=CARTESIAN_POINT('Ctrl Pts',(-9.36074871887772,-12.6258811352282,
118.108675842885)) ;
#191242=CARTESIAN_POINT('Ctrl Pts',(-9.28694484996586,-12.6258812005672,
118.132906806927)) ;
#191243=CARTESIAN_POINT('Ctrl Pts',(-9.21314098105396,-12.6258812659061,
118.157137770968)) ;
#191244=CARTESIAN_POINT('Ctrl Pts',(-9.19851368222664,-12.5661916520963,
118.112585380869)) ;
#191245=CARTESIAN_POINT('Ctrl Pts',(-9.1838863833993,-12.5065020382865,
118.068032990769)) ;
#191246=CARTESIAN_POINT('Ctrl Pts',(-9.25769025231121,-12.5065019729475,
118.043802026728)) ;
#191247=CARTESIAN_POINT('Ctrl Pts',(-9.33149412122307,-12.5065019076085,
118.019571062686)) ;
#191248=CARTESIAN_POINT('Ctrl Pts',(-9.34612142005041,-12.5661915214183,
118.064123452786)) ;
#191249=CARTESIAN_POINT('Ctrl Pts',(-9.27272433522268,-12.7760910985915,
117.876015426606)) ;
#191250=CARTESIAN_POINT('Ctrl Pts',(-9.29176439552139,-12.8212153371298,
117.934008376216)) ;
#191251=CARTESIAN_POINT('Ctrl Pts',(-9.2179605335698,-12.8212154191497,
117.958239361457)) ;
#191252=CARTESIAN_POINT('Ctrl Pts',(-9.14415667161822,-12.8212155011696,
117.982470346699)) ;
#191253=CARTESIAN_POINT('Ctrl Pts',(-9.12511661131953,-12.7760912626314,
117.924477397089)) ;
#191254=CARTESIAN_POINT('Ctrl Pts',(-9.10607655102083,-12.7309670240931,
117.866484447479)) ;
#191255=CARTESIAN_POINT('Ctrl Pts',(-9.1798804129724,-12.7309669420732,
117.842253462237)) ;
#191256=CARTESIAN_POINT('Ctrl Pts',(-9.25368427492398,-12.7309668600532,
117.818022476996)) ;
#191257=CARTESIAN_POINT('Ctrl Pts',(-9.27272433522268,-12.7760910985915,
117.876015426606)) ;
#191258=CARTESIAN_POINT('Ctrl Pts',(-9.21878702259048,-13.0327329322163,
117.747284173735)) ;
#191259=CARTESIAN_POINT('Ctrl Pts',(-9.24088580050292,-13.0600070239695,
117.81459348377)) ;
#191260=CARTESIAN_POINT('Ctrl Pts',(-9.1670819466148,-13.0600071142797,
117.838824493571)) ;
#191261=CARTESIAN_POINT('Ctrl Pts',(-9.09327809272665,-13.0600072045899,
117.863055503372)) ;
#191262=CARTESIAN_POINT('Ctrl Pts',(-9.07117931481421,-13.0327331128366,
117.795746193338)) ;
#191263=CARTESIAN_POINT('Ctrl Pts',(-9.04908053690176,-13.0054590210833,
117.728436883303)) ;
#191264=CARTESIAN_POINT('Ctrl Pts',(-9.12288439078989,-13.0054589307732,
117.704205873502)) ;
#191265=CARTESIAN_POINT('Ctrl Pts',(-9.19668824467802,-13.005458840463,
117.679974863701)) ;
#191266=CARTESIAN_POINT('Ctrl Pts',(-9.21878702259048,-13.0327329322163,
117.747284173735)) ;
#191267=CARTESIAN_POINT('Ctrl Pts',(-9.18778602878387,-13.3169814944794,
117.688392704249)) ;
#191268=CARTESIAN_POINT('Ctrl Pts',(-9.21134730464771,-13.3244510016564,
117.760156547187)) ;
#191269=CARTESIAN_POINT('Ctrl Pts',(-9.13754345877924,-13.3244510916003,
117.784387581415)) ;
#191270=CARTESIAN_POINT('Ctrl Pts',(-9.06373961291076,-13.3244511815443,
117.808618615643)) ;
#191271=CARTESIAN_POINT('Ctrl Pts',(-9.04017833704691,-13.3169816743673,
117.736854772705)) ;
#191272=CARTESIAN_POINT('Ctrl Pts',(-9.01661706118305,-13.3095121671903,
117.665090929766)) ;
#191273=CARTESIAN_POINT('Ctrl Pts',(-9.09042090705155,-13.3095120772463,
117.640859895538)) ;
#191274=CARTESIAN_POINT('Ctrl Pts',(-9.16422475292001,-13.3095119873024,
117.61662886131)) ;
#191275=CARTESIAN_POINT('Ctrl Pts',(-9.18778602878387,-13.3169814944794,
117.688392704249)) ;
#191276=CARTESIAN_POINT('Ctrl Pts',(-9.18098202319864,-13.6065319682423,
117.70296148096)) ;
#191277=CARTESIAN_POINT('Ctrl Pts',(-9.20432341160334,-13.593796615994,
117.774055582276)) ;
#191278=CARTESIAN_POINT('Ctrl Pts',(-9.13051957298211,-13.5937966997554,
117.798286638578)) ;
#191279=CARTESIAN_POINT('Ctrl Pts',(-9.05671573436087,-13.5937967835168,
117.82251769488)) ;
#191280=CARTESIAN_POINT('Ctrl Pts',(-9.03337434595617,-13.6065321357651,
117.751423593564)) ;
#191281=CARTESIAN_POINT('Ctrl Pts',(-9.01003295755148,-13.6192674880133,
117.680329492249)) ;
#191282=CARTESIAN_POINT('Ctrl Pts',(-9.08383679617271,-13.6192674042519,
117.656098435947)) ;
#191283=CARTESIAN_POINT('Ctrl Pts',(-9.15764063479395,-13.6192673204905,
117.631867379645)) ;
#191284=CARTESIAN_POINT('Ctrl Pts',(-9.18098202319864,-13.6065319682423,
117.70296148096)) ;
#191285=CARTESIAN_POINT('Ctrl Pts',(-9.19808875904426,-13.8845186470045,
117.790606361168)) ;
#191286=CARTESIAN_POINT('Ctrl Pts',(-9.21953568780673,-13.8523553116745,
117.855930244232)) ;
#191287=CARTESIAN_POINT('Ctrl Pts',(-9.14573185495254,-13.852355381399,
117.880161318099)) ;
#191288=CARTESIAN_POINT('Ctrl Pts',(-9.07192802209835,-13.8523554511235,
117.904392391967)) ;
#191289=CARTESIAN_POINT('Ctrl Pts',(-9.0504810933359,-13.8845187864536,
117.839068508903)) ;
#191290=CARTESIAN_POINT('Ctrl Pts',(-9.02903416457341,-13.9166821217837,
117.773744625839)) ;
#191291=CARTESIAN_POINT('Ctrl Pts',(-9.10283799742762,-13.9166820520591,
117.749513551972)) ;
#191292=CARTESIAN_POINT('Ctrl Pts',(-9.17664183028178,-13.9166819823346,
117.725282478104)) ;
#191293=CARTESIAN_POINT('Ctrl Pts',(-9.19808875904426,-13.8845186470045,
117.790606361168)) ;
#191294=CARTESIAN_POINT('Ctrl Pts',(-9.23700591797465,-14.1277890814299,
117.944490651807)) ;
#191295=CARTESIAN_POINT('Ctrl Pts',(-9.25503655471375,-14.0785921493268,
117.999409060714)) ;
#191296=CARTESIAN_POINT('Ctrl Pts',(-9.1812327258708,-14.0785922024829,
118.0236401468)) ;
#191297=CARTESIAN_POINT('Ctrl Pts',(-9.10742889702784,-14.0785922556391,
118.047871232885)) ;
#191298=CARTESIAN_POINT('Ctrl Pts',(-9.08939826028874,-14.1277891877422,
117.992952823977)) ;
#191299=CARTESIAN_POINT('Ctrl Pts',(-9.07136762354965,-14.1769861198453,
117.93803441507)) ;
#191300=CARTESIAN_POINT('Ctrl Pts',(-9.14517145239261,-14.1769860666892,
117.913803328985)) ;
#191301=CARTESIAN_POINT('Ctrl Pts',(-9.21897528123558,-14.1769860135331,
117.8895722429)) ;
#191302=CARTESIAN_POINT('Ctrl Pts',(-9.23700591797465,-14.1277890814299,
117.944490651807)) ;
#191303=CARTESIAN_POINT('Ctrl Pts',(-9.29456875476075,-14.3214999944636,
118.155368644358)) ;
#191304=CARTESIAN_POINT('Ctrl Pts',(-9.30787208960374,-14.2587034430882,
118.195888454611)) ;
#191305=CARTESIAN_POINT('Ctrl Pts',(-9.23406826234362,-14.2587034768352,
118.220119545517)) ;
#191306=CARTESIAN_POINT('Ctrl Pts',(-9.16026443508352,-14.2587035105822,
118.244350636423)) ;
#191307=CARTESIAN_POINT('Ctrl Pts',(-9.14696110024054,-14.3215000619577,
118.203830826171)) ;
#191308=CARTESIAN_POINT('Ctrl Pts',(-9.13365776539753,-14.3842966133332,
118.163311015918)) ;
#191309=CARTESIAN_POINT('Ctrl Pts',(-9.20746159265764,-14.3842965795861,
118.139079925012)) ;
#191310=CARTESIAN_POINT('Ctrl Pts',(-9.28126541991776,-14.3842965458391,
118.114848834105)) ;
#191311=CARTESIAN_POINT('Ctrl Pts',(-9.29456875476075,-14.3214999944636,
118.155368644358)) ;
#191312=CARTESIAN_POINT('Ctrl Pts',(-9.36558798569984,-14.4499114443817,
118.40714452843)) ;
#191313=CARTESIAN_POINT('Ctrl Pts',(-9.37321903855488,-14.3780538242765,
118.430387483132)) ;
#191314=CARTESIAN_POINT('Ctrl Pts',(-9.29941521096486,-14.37805384036,118.454618573033)) ;
#191315=CARTESIAN_POINT('Ctrl Pts',(-9.22561138337483,-14.3780538564435,
118.478849662934)) ;
#191316=CARTESIAN_POINT('Ctrl Pts',(-9.2179803305198,-14.4499114765488,
118.455606708232)) ;
#191317=CARTESIAN_POINT('Ctrl Pts',(-9.21034927766476,-14.521769096654,
118.43236375353)) ;
#191318=CARTESIAN_POINT('Ctrl Pts',(-9.28415310525479,-14.5217690805705,
118.408132663629)) ;
#191319=CARTESIAN_POINT('Ctrl Pts',(-9.3579569328448,-14.521769064487,118.383901573727)) ;
#191320=CARTESIAN_POINT('Ctrl Pts',(-9.36558798569984,-14.4499114443817,
118.40714452843)) ;
#191321=CARTESIAN_POINT('Ctrl Pts',(-9.44439581983412,-14.5043711676863,
118.682688731011)) ;
#191322=CARTESIAN_POINT('Ctrl Pts',(-9.44580117430657,-14.4286019200682,
118.686969213129)) ;
#191323=CARTESIAN_POINT('Ctrl Pts',(-9.37199734464163,-14.4286019216996,
118.71120029671)) ;
#191324=CARTESIAN_POINT('Ctrl Pts',(-9.29819351497668,-14.4286019233309,
118.735431380292)) ;
#191325=CARTESIAN_POINT('Ctrl Pts',(-9.29678816050424,-14.504371170949,
118.731150898174)) ;
#191326=CARTESIAN_POINT('Ctrl Pts',(-9.29538280603177,-14.5801404185671,
118.726870416056)) ;
#191327=CARTESIAN_POINT('Ctrl Pts',(-9.36918663569673,-14.5801404169357,
118.702639332474)) ;
#191328=CARTESIAN_POINT('Ctrl Pts',(-9.44299046536166,-14.5801404153043,
118.678408248893)) ;
#191329=CARTESIAN_POINT('Ctrl Pts',(-9.44439581983412,-14.5043711676863,
118.682688731011)) ;
#191330=CARTESIAN_POINT('Ctrl Pts',(-9.5241527941287,-14.481209763182,118.960955450656)) ;
#191331=CARTESIAN_POINT('Ctrl Pts',(-9.51926017308425,-14.4069431255803,
118.946053315668)) ;
#191332=CARTESIAN_POINT('Ctrl Pts',(-9.44545634078204,-14.4069431170847,
118.970284391217)) ;
#191333=CARTESIAN_POINT('Ctrl Pts',(-9.37165250847984,-14.4069431085892,
118.994515466766)) ;
#191334=CARTESIAN_POINT('Ctrl Pts',(-9.37654512952428,-14.4812097461908,
119.009417601753)) ;
#191335=CARTESIAN_POINT('Ctrl Pts',(-9.38143775056871,-14.5554763837924,
119.024319736741)) ;
#191336=CARTESIAN_POINT('Ctrl Pts',(-9.45524158287093,-14.555476392288,
119.000088661192)) ;
#191337=CARTESIAN_POINT('Ctrl Pts',(-9.52904541517314,-14.5554764007836,
118.975857585643)) ;
#191338=CARTESIAN_POINT('Ctrl Pts',(-9.5241527941287,-14.481209763182,118.960955450656)) ;
#191339=CARTESIAN_POINT('Ctrl Pts',(-9.59915417164219,-14.3816923411007,
119.22493046164)) ;
#191340=CARTESIAN_POINT('Ctrl Pts',(-9.58828196244955,-14.3142615616255,
119.191815466132)) ;
#191341=CARTESIAN_POINT('Ctrl Pts',(-9.51447812654902,-14.3142615481585,
119.216046530721)) ;
#191342=CARTESIAN_POINT('Ctrl Pts',(-9.44067429064847,-14.3142615346915,
119.240277595309)) ;
#191343=CARTESIAN_POINT('Ctrl Pts',(-9.45154649984112,-14.3816923141668,
119.273392590818)) ;
#191344=CARTESIAN_POINT('Ctrl Pts',(-9.46241870903376,-14.449123093642,
119.306507586327)) ;
#191345=CARTESIAN_POINT('Ctrl Pts',(-9.5362225449343,-14.449123107109,119.282276521738)) ;
#191346=CARTESIAN_POINT('Ctrl Pts',(-9.61002638083482,-14.4491231205759,
119.258045457149)) ;
#191347=CARTESIAN_POINT('Ctrl Pts',(-9.59915417164219,-14.3816923411007,
119.22493046164)) ;
#191348=CARTESIAN_POINT('Ctrl Pts',(-9.66271309070694,-14.2134896291755,
119.453949550053)) ;
#191349=CARTESIAN_POINT('Ctrl Pts',(-9.64665334575257,-14.1577013578714,
119.405034157769)) ;
#191350=CARTESIAN_POINT('Ctrl Pts',(-9.57284950669676,-14.1577013437741,
119.429265212747)) ;
#191351=CARTESIAN_POINT('Ctrl Pts',(-9.49904566764095,-14.1577013296769,
119.453496267726)) ;
#191352=CARTESIAN_POINT('Ctrl Pts',(-9.51510541259531,-14.2134896009809,
119.50241166001)) ;
#191353=CARTESIAN_POINT('Ctrl Pts',(-9.53116515754968,-14.269277872285,
119.551327052294)) ;
#191354=CARTESIAN_POINT('Ctrl Pts',(-9.60496899660549,-14.2692778863823,
119.527095997316)) ;
#191355=CARTESIAN_POINT('Ctrl Pts',(-9.6787728356613,-14.2692779004795,
119.502864942338)) ;
#191356=CARTESIAN_POINT('Ctrl Pts',(-9.66271309070694,-14.2134896291755,
119.453949550053)) ;
#191357=CARTESIAN_POINT('Ctrl Pts',(-9.70990503125504,-13.9864989351748,
119.633376033993)) ;
#191358=CARTESIAN_POINT('Ctrl Pts',(-9.68978709639809,-13.9464758835493,
119.572100050222)) ;
#191359=CARTESIAN_POINT('Ctrl Pts',(-9.61598325463275,-13.9464758738248,
119.596331096948)) ;
#191360=CARTESIAN_POINT('Ctrl Pts',(-9.54217941286741,-13.9464758641003,
119.620562143673)) ;
#191361=CARTESIAN_POINT('Ctrl Pts',(-9.56229734772436,-13.9864989157259,
119.681838127444)) ;
#191362=CARTESIAN_POINT('Ctrl Pts',(-9.5824152825813,-14.0265219673515,
119.743114111215)) ;
#191363=CARTESIAN_POINT('Ctrl Pts',(-9.65621912434665,-14.0265219770759,
119.718883064489)) ;
#191364=CARTESIAN_POINT('Ctrl Pts',(-9.73002296611199,-14.0265219868004,
119.694652017763)) ;
#191365=CARTESIAN_POINT('Ctrl Pts',(-9.70990503125504,-13.9864989351748,
119.633376033993)) ;
#191366=CARTESIAN_POINT('Ctrl Pts',(-9.73598202444326,-13.7220237261921,
119.748017635008)) ;
#191367=CARTESIAN_POINT('Ctrl Pts',(-9.71328442430442,-13.7004075787871,
119.678884407102)) ;
#191368=CARTESIAN_POINT('Ctrl Pts',(-9.6394805813284,-13.7004075723778,
119.70311545014)) ;
#191369=CARTESIAN_POINT('Ctrl Pts',(-9.5656767383524,-13.7004075659685,
119.727346493179)) ;
#191370=CARTESIAN_POINT('Ctrl Pts',(-9.58837433849125,-13.7220237133736,
119.796479721084)) ;
#191371=CARTESIAN_POINT('Ctrl Pts',(-9.61107193863009,-13.7436398607786,
119.86561294899)) ;
#191372=CARTESIAN_POINT('Ctrl Pts',(-9.6848757816061,-13.7436398671878,
119.841381905952)) ;
#191373=CARTESIAN_POINT('Ctrl Pts',(-9.75867962458211,-13.7436398735971,
119.817150862914)) ;
#191374=CARTESIAN_POINT('Ctrl Pts',(-9.73598202444326,-13.7220237261921,
119.748017635008)) ;
#191375=CARTESIAN_POINT('Ctrl Pts',(-9.73888236422256,-13.4322464163541,
119.792546805507)) ;
#191376=CARTESIAN_POINT('Ctrl Pts',(-9.71520923913131,-13.4308324436495,
119.720442286112)) ;
#191377=CARTESIAN_POINT('Ctrl Pts',(-9.64140539559821,-13.4308324430486,
119.744673327453)) ;
#191378=CARTESIAN_POINT('Ctrl Pts',(-9.56760155206506,-13.4308324424476,
119.768904368795)) ;
#191379=CARTESIAN_POINT('Ctrl Pts',(-9.59127467715629,-13.4322464151522,
119.841008888189)) ;
#191380=CARTESIAN_POINT('Ctrl Pts',(-9.61494780224751,-13.4336603878567,
119.913113407584)) ;
#191381=CARTESIAN_POINT('Ctrl Pts',(-9.68875164578064,-13.4336603884577,
119.888882366242)) ;
#191382=CARTESIAN_POINT('Ctrl Pts',(-9.76255548931378,-13.4336603890586,
119.864651324901)) ;
#191383=CARTESIAN_POINT('Ctrl Pts',(-9.73888236422256,-13.4322464163541,
119.792546805507)) ;
#191384=CARTESIAN_POINT('Ctrl Pts',(-9.71766042455426,-13.1452897052538,
119.763098775571)) ;
#191385=CARTESIAN_POINT('Ctrl Pts',(-9.69470574929104,-13.1639105046461,
119.693182538477)) ;
#191386=CARTESIAN_POINT('Ctrl Pts',(-9.62090190597256,-13.1639105064164,
119.717413580472)) ;
#191387=CARTESIAN_POINT('Ctrl Pts',(-9.54709806265407,-13.1639105081867,
119.741644622467)) ;
#191388=CARTESIAN_POINT('Ctrl Pts',(-9.57005273791729,-13.1452897087944,
119.811560859561)) ;
#191389=CARTESIAN_POINT('Ctrl Pts',(-9.59300741318051,-13.1266689094021,
119.881477096656)) ;
#191390=CARTESIAN_POINT('Ctrl Pts',(-9.666811256499,-13.1266689076317,119.857246054661)) ;
#191391=CARTESIAN_POINT('Ctrl Pts',(-9.74061509981748,-13.1266689058614,
119.833015012666)) ;
#191392=CARTESIAN_POINT('Ctrl Pts',(-9.71766042455426,-13.1452897052538,
119.763098775571)) ;
#191393=CARTESIAN_POINT('Ctrl Pts',(-9.67235419941848,-12.8735307541799,
119.660876832314)) ;
#191394=CARTESIAN_POINT('Ctrl Pts',(-9.65178857018535,-12.9111570713961,
119.598237243989)) ;
#191395=CARTESIAN_POINT('Ctrl Pts',(-9.57798472730891,-12.9111570744422,
119.622468287331)) ;
#191396=CARTESIAN_POINT('Ctrl Pts',(-9.5041808844325,-12.9111570774884,
119.646699330672)) ;
#191397=CARTESIAN_POINT('Ctrl Pts',(-9.52474651366562,-12.8735307602723,
119.709338918997)) ;
#191398=CARTESIAN_POINT('Ctrl Pts',(-9.54531214289875,-12.8359044430562,
119.771978507321)) ;
#191399=CARTESIAN_POINT('Ctrl Pts',(-9.61911598577518,-12.83590444001,119.74774746398)) ;
#191400=CARTESIAN_POINT('Ctrl Pts',(-9.6929198286516,-12.8359044369638,
119.723516420638)) ;
#191401=CARTESIAN_POINT('Ctrl Pts',(-9.67235419941848,-12.8735307541799,
119.660876832314)) ;
#191402=CARTESIAN_POINT('Ctrl Pts',(-9.60679604063529,-12.6449175335016,
119.496385341549)) ;
#191403=CARTESIAN_POINT('Ctrl Pts',(-9.59004978947933,-12.6985622170396,
119.445378962574)) ;
#191404=CARTESIAN_POINT('Ctrl Pts',(-9.51624594666137,-12.698562218704,
119.469610006093)) ;
#191405=CARTESIAN_POINT('Ctrl Pts',(-9.44244210384339,-12.6985622203683,
119.493841049613)) ;
#191406=CARTESIAN_POINT('Ctrl Pts',(-9.45918835499932,-12.6449175368303,
119.544847428588)) ;
#191407=CARTESIAN_POINT('Ctrl Pts',(-9.47593460615524,-12.5912728532923,
119.595853807563)) ;
#191408=CARTESIAN_POINT('Ctrl Pts',(-9.54973844897323,-12.5912728516279,
119.571622764043)) ;
#191409=CARTESIAN_POINT('Ctrl Pts',(-9.6235422917912,-12.5912728499636,
119.547391720524)) ;
#191410=CARTESIAN_POINT('Ctrl Pts',(-9.60679604063529,-12.6449175335016,
119.496385341549)) ;
#191411=CARTESIAN_POINT('Ctrl Pts',(-9.52374541645956,-12.4692026417619,
119.278925596776)) ;
#191412=CARTESIAN_POINT('Ctrl Pts',(-9.51203907941057,-12.5351960145383,
119.243269982934)) ;
#191413=CARTESIAN_POINT('Ctrl Pts',(-9.43823523604837,-12.5351960141678,
119.267501024796)) ;
#191414=CARTESIAN_POINT('Ctrl Pts',(-9.36443139268619,-12.5351960137972,
119.291732066658)) ;
#191415=CARTESIAN_POINT('Ctrl Pts',(-9.3761377297352,-12.4692026410208,
119.3273876805)) ;
#191416=CARTESIAN_POINT('Ctrl Pts',(-9.38784406678419,-12.4032092682444,
119.363043294341)) ;
#191417=CARTESIAN_POINT('Ctrl Pts',(-9.46164791014638,-12.4032092686149,
119.33881225248)) ;
#191418=CARTESIAN_POINT('Ctrl Pts',(-9.53545175350857,-12.4032092689855,
119.314581210618)) ;
#191419=CARTESIAN_POINT('Ctrl Pts',(-9.52374541645956,-12.4692026417619,
119.278925596776)) ;
#191420=CARTESIAN_POINT('Ctrl Pts',(-9.42830467125578,-12.3617390442732,
119.023858845481)) ;
#191421=CARTESIAN_POINT('Ctrl Pts',(-9.42250815332207,-12.4353332114667,
119.006203587009)) ;
#191422=CARTESIAN_POINT('Ctrl Pts',(-9.34870430822669,-12.4353332096564,
119.030434623592)) ;
#191423=CARTESIAN_POINT('Ctrl Pts',(-9.27490046313128,-12.4353332078462,
119.054665660175)) ;
#191424=CARTESIAN_POINT('Ctrl Pts',(-9.28069698106498,-12.3617390406526,
119.072320918647)) ;
#191425=CARTESIAN_POINT('Ctrl Pts',(-9.28649349899868,-12.2881448734591,
119.089976177118)) ;
#191426=CARTESIAN_POINT('Ctrl Pts',(-9.36029734409406,-12.2881448752694,
119.065745140535)) ;
#191427=CARTESIAN_POINT('Ctrl Pts',(-9.43410118918947,-12.2881448770796,
119.041514103952)) ;
#191428=CARTESIAN_POINT('Ctrl Pts',(-9.42830467125578,-12.3617390442732,
119.023858845481)) ;
#191429=CARTESIAN_POINT('Ctrl Pts',(-9.32805694090023,-12.3304471936261,
118.753786408682)) ;
#191430=CARTESIAN_POINT('Ctrl Pts',(-9.32852185600717,-12.4063328156575,
118.755202464884)) ;
#191431=CARTESIAN_POINT('Ctrl Pts',(-9.25471800936834,-12.4063328154178,
118.779433496766)) ;
#191432=CARTESIAN_POINT('Ctrl Pts',(-9.18091416272954,-12.4063328151781,
118.803664528648)) ;
#191433=CARTESIAN_POINT('Ctrl Pts',(-9.18044924762258,-12.3304471931467,
118.802248472446)) ;
#191434=CARTESIAN_POINT('Ctrl Pts',(-9.17998433251566,-12.2545615711153,
118.800832416244)) ;
#191435=CARTESIAN_POINT('Ctrl Pts',(-9.25378817915447,-12.254561571355,
118.776601384362)) ;
#191436=CARTESIAN_POINT('Ctrl Pts',(-9.32759202579329,-12.2545615715947,
118.75237035248)) ;
#191437=CARTESIAN_POINT('Ctrl Pts',(-9.32805694090023,-12.3304471936261,
118.753786408682)) ;
#191438=CARTESIAN_POINT('Ctrl Pts',(-9.22771837840066,-12.376595059269,
118.483689651131)) ;
#191439=CARTESIAN_POINT('Ctrl Pts',(-9.23445495121477,-12.4493688880087,
118.50420816464)) ;
#191440=CARTESIAN_POINT('Ctrl Pts',(-9.16065110249134,-12.4493688924278,
118.528439190173)) ;
#191441=CARTESIAN_POINT('Ctrl Pts',(-9.08684725376789,-12.4493688968469,
118.552670215705)) ;
#191442=CARTESIAN_POINT('Ctrl Pts',(-9.0801106809538,-12.3765950681072,
118.532151702196)) ;
#191443=CARTESIAN_POINT('Ctrl Pts',(-9.07337410813971,-12.3038212393674,
118.511633188686)) ;
#191444=CARTESIAN_POINT('Ctrl Pts',(-9.14717795686315,-12.3038212349483,
118.487402163154)) ;
#191445=CARTESIAN_POINT('Ctrl Pts',(-9.22098180558658,-12.3038212305292,
118.463171137621)) ;
#191446=CARTESIAN_POINT('Ctrl Pts',(-9.22771837840066,-12.376595059269,
118.483689651131)) ;
#191447=CARTESIAN_POINT('Ctrl Pts',(-9.13441934511046,-12.4977240769561,
118.235035472375)) ;
#191448=CARTESIAN_POINT('Ctrl Pts',(-9.14694502691882,-12.5621460088863,
118.273186677651)) ;
#191449=CARTESIAN_POINT('Ctrl Pts',(-9.07314117653568,-12.5621460220276,
118.297417698128)) ;
#191450=CARTESIAN_POINT('Ctrl Pts',(-8.99933732615257,-12.5621460351689,
118.321648718606)) ;
#191451=CARTESIAN_POINT('Ctrl Pts',(-8.9868116443442,-12.4977241032387,
118.283497513329)) ;
#191452=CARTESIAN_POINT('Ctrl Pts',(-8.97428596253584,-12.4333021713085,
118.245346308053)) ;
#191453=CARTESIAN_POINT('Ctrl Pts',(-9.04808981291898,-12.4333021581672,
118.221115287576)) ;
#191454=CARTESIAN_POINT('Ctrl Pts',(-9.12189366330211,-12.4333021450259,
118.196884267098)) ;
#191455=CARTESIAN_POINT('Ctrl Pts',(-9.13441934511046,-12.4977240769561,
118.235035472375)) ;
#191456=CARTESIAN_POINT('Ctrl Pts',(-9.05412590445871,-12.6852356935121,
118.026023195874)) ;
#191457=CARTESIAN_POINT('Ctrl Pts',(-9.07154033274177,-12.736658719336,
118.079064733939)) ;
#191458=CARTESIAN_POINT('Ctrl Pts',(-8.99773648181564,-12.7366587448055,
118.103295752762)) ;
#191459=CARTESIAN_POINT('Ctrl Pts',(-8.92393263088948,-12.7366587702751,
118.127526771585)) ;
#191460=CARTESIAN_POINT('Ctrl Pts',(-8.90651820260644,-12.6852357444512,
118.074485233521)) ;
#191461=CARTESIAN_POINT('Ctrl Pts',(-8.88910377432337,-12.6338127186274,
118.021443695456)) ;
#191462=CARTESIAN_POINT('Ctrl Pts',(-8.96290762524951,-12.6338126931579,
117.997212676633)) ;
#191463=CARTESIAN_POINT('Ctrl Pts',(-9.03671147617565,-12.6338126676883,
117.972981657809)) ;
#191464=CARTESIAN_POINT('Ctrl Pts',(-9.05412590445871,-12.6852356935121,
118.026023195874)) ;
#191465=CARTESIAN_POINT('Ctrl Pts',(-8.99222443458086,-12.9233901911912,
117.872760424297)) ;
#191466=CARTESIAN_POINT('Ctrl Pts',(-9.01325581855126,-12.9582592987456,
117.93681862566)) ;
#191467=CARTESIAN_POINT('Ctrl Pts',(-8.93945196899214,-12.958259335733,
117.961049648647)) ;
#191468=CARTESIAN_POINT('Ctrl Pts',(-8.86564811943302,-12.9582593727203,
117.985280671634)) ;
#191469=CARTESIAN_POINT('Ctrl Pts',(-8.84461673546261,-12.9233902651659,
117.921222470271)) ;
#191470=CARTESIAN_POINT('Ctrl Pts',(-8.82358535149221,-12.8885211576114,
117.857164268908)) ;
#191471=CARTESIAN_POINT('Ctrl Pts',(-8.89738920105133,-12.8885211206241,
117.832933245921)) ;
#191472=CARTESIAN_POINT('Ctrl Pts',(-8.97119305061046,-12.8885210836367,
117.808702222934)) ;
#191473=CARTESIAN_POINT('Ctrl Pts',(-8.99222443458086,-12.9233901911912,
117.872760424297)) ;
#191474=CARTESIAN_POINT('Ctrl Pts',(-8.95143036020703,-13.1995574427629,
117.78415630209)) ;
#191475=CARTESIAN_POINT('Ctrl Pts',(-8.97460286631076,-13.2151953803477,
117.854736015799)) ;
#191476=CARTESIAN_POINT('Ctrl Pts',(-8.90079901934515,-13.2151954315295,
117.878967046685)) ;
#191477=CARTESIAN_POINT('Ctrl Pts',(-8.82699517237954,-13.2151954827113,
117.903198077571)) ;
#191478=CARTESIAN_POINT('Ctrl Pts',(-8.80382266627582,-13.1995575451265,
117.832618363863)) ;
#191479=CARTESIAN_POINT('Ctrl Pts',(-8.7806501601721,-13.1839196075417,
117.762038650154)) ;
#191480=CARTESIAN_POINT('Ctrl Pts',(-8.8544540071377,-13.1839195563599,
117.737807619268)) ;
#191481=CARTESIAN_POINT('Ctrl Pts',(-8.92825785410331,-13.1839195051781,
117.713576588382)) ;
#191482=CARTESIAN_POINT('Ctrl Pts',(-8.95143036020703,-13.1995574427629,
117.78415630209)) ;
#191483=CARTESIAN_POINT('Ctrl Pts',(-8.93482201587667,-13.4900175633602,
117.769023857071)) ;
#191484=CARTESIAN_POINT('Ctrl Pts',(-8.95845396264376,-13.4853985697917,
117.841002952746)) ;
#191485=CARTESIAN_POINT('Ctrl Pts',(-8.88465012030017,-13.4853986306042,
117.86523399771)) ;
#191486=CARTESIAN_POINT('Ctrl Pts',(-8.81084627795657,-13.4853986914167,
117.889465042674)) ;
#191487=CARTESIAN_POINT('Ctrl Pts',(-8.7872143311895,-13.4900176849852,
117.817485946999)) ;
#191488=CARTESIAN_POINT('Ctrl Pts',(-8.7635823844224,-13.4946366785538,
117.745506851324)) ;
#191489=CARTESIAN_POINT('Ctrl Pts',(-8.837386226766,-13.4946366177413,117.72127580636)) ;
#191490=CARTESIAN_POINT('Ctrl Pts',(-8.91119006910959,-13.4946365569288,
117.697044761396)) ;
#191491=CARTESIAN_POINT('Ctrl Pts',(-8.93482201587667,-13.4900175633602,
117.769023857071)) ;
#191492=CARTESIAN_POINT('Ctrl Pts',(-8.94231588505226,-13.7743854626431,
117.827189380347)) ;
#191493=CARTESIAN_POINT('Ctrl Pts',(-8.96472742648635,-13.7499058485971,
117.895451318152)) ;
#191494=CARTESIAN_POINT('Ctrl Pts',(-8.89092358984129,-13.7499059130724,
117.919682380473)) ;
#191495=CARTESIAN_POINT('Ctrl Pts',(-8.81711975319624,-13.7499059775478,
117.943913442794)) ;
#191496=CARTESIAN_POINT('Ctrl Pts',(-8.79470821176214,-13.7743855915938,
117.875651504989)) ;
#191497=CARTESIAN_POINT('Ctrl Pts',(-8.77229667032804,-13.7988652056398,
117.807389567185)) ;
#191498=CARTESIAN_POINT('Ctrl Pts',(-8.84610050697309,-13.7988651411644,
117.783158504863)) ;
#191499=CARTESIAN_POINT('Ctrl Pts',(-8.91990434361816,-13.7988650766891,
117.758927442542)) ;
#191500=CARTESIAN_POINT('Ctrl Pts',(-8.94231588505226,-13.7743854626431,
117.827189380347)) ;
#191501=CARTESIAN_POINT('Ctrl Pts',(-8.97275889862437,-14.034295085312,
117.955380252604)) ;
#191502=CARTESIAN_POINT('Ctrl Pts',(-8.99234358787894,-13.9916338194208,
118.015032054628)) ;
#191503=CARTESIAN_POINT('Ctrl Pts',(-8.91853975771521,-13.9916338823601,
118.03926313669)) ;
#191504=CARTESIAN_POINT('Ctrl Pts',(-8.84473592755146,-13.9916339452994,
118.063494218752)) ;
#191505=CARTESIAN_POINT('Ctrl Pts',(-8.82515123829691,-14.0342952111906,
118.003842416728)) ;
#191506=CARTESIAN_POINT('Ctrl Pts',(-8.80556654904233,-14.0769564770818,
117.944190614704)) ;
#191507=CARTESIAN_POINT('Ctrl Pts',(-8.87937037920607,-14.0769564141425,
117.919959532642)) ;
#191508=CARTESIAN_POINT('Ctrl Pts',(-8.9531742093698,-14.0769563512032,
117.89572845058)) ;
#191509=CARTESIAN_POINT('Ctrl Pts',(-8.97275889862437,-14.034295085312,
117.955380252604)) ;
#191510=CARTESIAN_POINT('Ctrl Pts',(-9.02327149966453,-14.2500983716934,
118.144707533452)) ;
#191511=CARTESIAN_POINT('Ctrl Pts',(-9.0386239611536,-14.1923084690493,
118.191468652428)) ;
#191512=CARTESIAN_POINT('Ctrl Pts',(-8.96482013749476,-14.1923085231576,
118.215699754303)) ;
#191513=CARTESIAN_POINT('Ctrl Pts',(-8.89101631383591,-14.192308577266,
118.239930856178)) ;
#191514=CARTESIAN_POINT('Ctrl Pts',(-8.87566385234682,-14.2500984799102,
118.193169737202)) ;
#191515=CARTESIAN_POINT('Ctrl Pts',(-8.86031139085772,-14.3078883825543,
118.146408618226)) ;
#191516=CARTESIAN_POINT('Ctrl Pts',(-8.93411521451657,-14.307888328446,
118.122177516351)) ;
#191517=CARTESIAN_POINT('Ctrl Pts',(-9.00791903817544,-14.3078882743376,
118.097946414476)) ;
#191518=CARTESIAN_POINT('Ctrl Pts',(-9.02327149966453,-14.2500983716934,
118.144707533452)) ;
#191519=CARTESIAN_POINT('Ctrl Pts',(-9.08946157962158,-14.4061684747286,
118.381787624125)) ;
#191520=CARTESIAN_POINT('Ctrl Pts',(-9.0994811477014,-14.3373982174877,
118.412305610108)) ;
#191521=CARTESIAN_POINT('Ctrl Pts',(-9.02567732968049,-14.3373982554781,
118.436536729156)) ;
#191522=CARTESIAN_POINT('Ctrl Pts',(-8.95187351165958,-14.3373982934686,
118.460767848203)) ;
#191523=CARTESIAN_POINT('Ctrl Pts',(-8.94185394357977,-14.4061685507095,
118.430249862219)) ;
#191524=CARTESIAN_POINT('Ctrl Pts',(-8.93183437549992,-14.4749388079505,
118.399731876235)) ;
#191525=CARTESIAN_POINT('Ctrl Pts',(-9.00563819352086,-14.47493876996,118.375500757188)) ;
#191526=CARTESIAN_POINT('Ctrl Pts',(-9.07944201154175,-14.4749387319696,
118.351269638141)) ;
#191527=CARTESIAN_POINT('Ctrl Pts',(-9.08946157962158,-14.4061684747286,
118.381787624125)) ;
#191528=CARTESIAN_POINT('Ctrl Pts',(-9.16561443892928,-14.4915146282391,
118.649122210678)) ;
#191529=CARTESIAN_POINT('Ctrl Pts',(-9.1695996827275,-14.4166858315879,
118.661260618433)) ;
#191530=CARTESIAN_POINT('Ctrl Pts',(-9.09579586856763,-14.4166858475525,
118.68549174924)) ;
#191531=CARTESIAN_POINT('Ctrl Pts',(-9.02199205440779,-14.4166858635172,
118.709722880047)) ;
#191532=CARTESIAN_POINT('Ctrl Pts',(-9.01800681060956,-14.4915146601683,
118.697584472293)) ;
#191533=CARTESIAN_POINT('Ctrl Pts',(-9.01402156681139,-14.5663434568195,
118.685446064538)) ;
#191534=CARTESIAN_POINT('Ctrl Pts',(-9.08782538097122,-14.5663434408549,
118.661214933731)) ;
#191535=CARTESIAN_POINT('Ctrl Pts',(-9.16162919513109,-14.5663434248902,
118.636983802923)) ;
#191536=CARTESIAN_POINT('Ctrl Pts',(-9.16561443892928,-14.4915146282391,
118.649122210678)) ;
#191537=CARTESIAN_POINT('Ctrl Pts',(-9.24634855912068,-14.4998611303634,
118.930692891984)) ;
#191538=CARTESIAN_POINT('Ctrl Pts',(-9.2439651474815,-14.4243396117057,
118.923433402744)) ;
#191539=CARTESIAN_POINT('Ctrl Pts',(-9.17016133536057,-14.4243396013487,
118.947664539761)) ;
#191540=CARTESIAN_POINT('Ctrl Pts',(-9.09635752323964,-14.4243395909917,
118.971895676779)) ;
#191541=CARTESIAN_POINT('Ctrl Pts',(-9.09874093487882,-14.4998611096494,
118.979155166019)) ;
#191542=CARTESIAN_POINT('Ctrl Pts',(-9.10112434651799,-14.5753826283071,
118.986414655258)) ;
#191543=CARTESIAN_POINT('Ctrl Pts',(-9.17492815863893,-14.5753826386642,
118.962183518241)) ;
#191544=CARTESIAN_POINT('Ctrl Pts',(-9.24873197075985,-14.5753826490212,
118.937952381223)) ;
#191545=CARTESIAN_POINT('Ctrl Pts',(-9.24634855912068,-14.4998611303634,
118.930692891984)) ;
#191546=CARTESIAN_POINT('Ctrl Pts',(-9.32363756664781,-14.4309678249663,
119.201372357098)) ;
#191547=CARTESIAN_POINT('Ctrl Pts',(-9.31512481565251,-14.3601461164253,
119.17544388909)) ;
#191548=CARTESIAN_POINT('Ctrl Pts',(-9.24132100236167,-14.3601460788116,
119.199675022545)) ;
#191549=CARTESIAN_POINT('Ctrl Pts',(-9.16751718907081,-14.3601460411978,
119.223906155999)) ;
#191550=CARTESIAN_POINT('Ctrl Pts',(-9.1760299400661,-14.4309677497388,
119.249834624006)) ;
#191551=CARTESIAN_POINT('Ctrl Pts',(-9.1845426910614,-14.5017894582798,
119.275763092013)) ;
#191552=CARTESIAN_POINT('Ctrl Pts',(-9.25834650435227,-14.5017894958936,
119.251531958559)) ;
#191553=CARTESIAN_POINT('Ctrl Pts',(-9.33215031764312,-14.5017895335074,
119.227300825105)) ;
#191554=CARTESIAN_POINT('Ctrl Pts',(-9.32363756664781,-14.4309678249663,
119.201372357098)) ;
#191555=CARTESIAN_POINT('Ctrl Pts',(-9.39258979887019,-14.2895356443573,
119.446881447834)) ;
#191556=CARTESIAN_POINT('Ctrl Pts',(-9.37851621544446,-14.2284839799428,
119.404015581425)) ;
#191557=CARTESIAN_POINT('Ctrl Pts',(-9.30471239868478,-14.228483916303,
119.428246704314)) ;
#191558=CARTESIAN_POINT('Ctrl Pts',(-9.23090858192508,-14.2284838526632,
119.452477827202)) ;
#191559=CARTESIAN_POINT('Ctrl Pts',(-9.24498216535079,-14.2895355170776,
119.495343693611)) ;
#191560=CARTESIAN_POINT('Ctrl Pts',(-9.25905574877654,-14.3505871814921,
119.538209560021)) ;
#191561=CARTESIAN_POINT('Ctrl Pts',(-9.33285956553622,-14.3505872451319,
119.513978437132)) ;
#191562=CARTESIAN_POINT('Ctrl Pts',(-9.40666338229591,-14.3505873087717,
119.489747314244)) ;
#191563=CARTESIAN_POINT('Ctrl Pts',(-9.39258979887019,-14.2895356443573,
119.446881447834)) ;
#191564=CARTESIAN_POINT('Ctrl Pts',(-9.4470024036837,-14.0847982621001,
119.648180996783)) ;
#191565=CARTESIAN_POINT('Ctrl Pts',(-9.42837319306047,-14.0379502045981,
119.591439424947)) ;
#191566=CARTESIAN_POINT('Ctrl Pts',(-9.35456937033141,-14.0379501191932,
119.615670529654)) ;
#191567=CARTESIAN_POINT('Ctrl Pts',(-9.28076554760235,-14.0379500337882,
119.639901634361)) ;
#191568=CARTESIAN_POINT('Ctrl Pts',(-9.29939475822559,-14.0847980912902,
119.696643206197)) ;
#191569=CARTESIAN_POINT('Ctrl Pts',(-9.31802396884881,-14.1316461487922,
119.753384778032)) ;
#191570=CARTESIAN_POINT('Ctrl Pts',(-9.39182779157788,-14.1316462341972,
119.729153673326)) ;
#191571=CARTESIAN_POINT('Ctrl Pts',(-9.46563161430695,-14.1316463196022,
119.704922568619)) ;
#191572=CARTESIAN_POINT('Ctrl Pts',(-9.4470024036837,-14.0847982621001,
119.648180996783)) ;
#191573=CARTESIAN_POINT('Ctrl Pts',(-9.48202871648516,-13.8335759567493,
119.790243958502)) ;
#191574=CARTESIAN_POINT('Ctrl Pts',(-9.46019456732522,-13.8041981863265,
119.723740660991)) ;
#191575=CARTESIAN_POINT('Ctrl Pts',(-9.38639073681574,-13.8041980860306,
119.747971742)) ;
#191576=CARTESIAN_POINT('Ctrl Pts',(-9.31258690630627,-13.8041979857347,
119.772202823009)) ;
#191577=CARTESIAN_POINT('Ctrl Pts',(-9.33442105546621,-13.8335757561575,
119.83870612052)) ;
#191578=CARTESIAN_POINT('Ctrl Pts',(-9.35625520462616,-13.8629535265802,
119.905209418031)) ;
#191579=CARTESIAN_POINT('Ctrl Pts',(-9.43005903513562,-13.8629536268761,
119.880978337022)) ;
#191580=CARTESIAN_POINT('Ctrl Pts',(-9.5038628656451,-13.8629537271721,
119.856747256013)) ;
#191581=CARTESIAN_POINT('Ctrl Pts',(-9.48202871648516,-13.8335759567493,
119.790243958502)) ;
#191582=CARTESIAN_POINT('Ctrl Pts',(-9.49463933409684,-13.5504534645936,
119.86430996683)) ;
#191583=CARTESIAN_POINT('Ctrl Pts',(-9.4711543977437,-13.5407982837148,
119.792778637903)) ;
#191584=CARTESIAN_POINT('Ctrl Pts',(-9.39735055836403,-13.540798177125,
119.817009691895)) ;
#191585=CARTESIAN_POINT('Ctrl Pts',(-9.32354671898437,-13.5407980705352,
119.841240745887)) ;
#191586=CARTESIAN_POINT('Ctrl Pts',(-9.34703165533753,-13.5504532514139,
119.912772074813)) ;
#191587=CARTESIAN_POINT('Ctrl Pts',(-9.37051659169066,-13.5601084322927,
119.98430340374)) ;
#191588=CARTESIAN_POINT('Ctrl Pts',(-9.44432043107033,-13.5601085388825,
119.960072349748)) ;
#191589=CARTESIAN_POINT('Ctrl Pts',(-9.51812427045,-13.5601086454724,119.935841295756)) ;
#191590=CARTESIAN_POINT('Ctrl Pts',(-9.49463933409684,-13.5504534645936,
119.86430996683)) ;
#191591=CARTESIAN_POINT('Ctrl Pts',(-9.48316140353234,-13.261274370137,
119.864568700158)) ;
#191592=CARTESIAN_POINT('Ctrl Pts',(-9.45971434880432,-13.2717947138784,
119.793152752578)) ;
#191593=CARTESIAN_POINT('Ctrl Pts',(-9.38591050056251,-13.2717946091373,
119.817383779577)) ;
#191594=CARTESIAN_POINT('Ctrl Pts',(-9.31210665232066,-13.2717945043963,
119.841614806576)) ;
#191595=CARTESIAN_POINT('Ctrl Pts',(-9.33555370704867,-13.2612741606549,
119.913030754156)) ;
#191596=CARTESIAN_POINT('Ctrl Pts',(-9.35900076177666,-13.2507538169135,
119.984446701736)) ;
#191597=CARTESIAN_POINT('Ctrl Pts',(-9.4328046100185,-13.2507539216545,
119.960215674737)) ;
#191598=CARTESIAN_POINT('Ctrl Pts',(-9.50660845826033,-13.2507540263956,
119.935984647738)) ;
#191599=CARTESIAN_POINT('Ctrl Pts',(-9.48316140353234,-13.261274370137,
119.864568700158)) ;
#191600=CARTESIAN_POINT('Ctrl Pts',(-9.44760475251543,-12.9807689853667,
119.791808570075)) ;
#191601=CARTESIAN_POINT('Ctrl Pts',(-9.42586969078854,-13.0108889686765,
119.725607077008)) ;
#191602=CARTESIAN_POINT('Ctrl Pts',(-9.35206583439519,-13.0108888747282,
119.749838079179)) ;
#191603=CARTESIAN_POINT('Ctrl Pts',(-9.27826197800183,-13.0108887807799,
119.77406908135)) ;
#191604=CARTESIAN_POINT('Ctrl Pts',(-9.29999703972874,-12.9807687974702,
119.840270574417)) ;
#191605=CARTESIAN_POINT('Ctrl Pts',(-9.32173210145563,-12.9506488141604,
119.906472067483)) ;
#191606=CARTESIAN_POINT('Ctrl Pts',(-9.39553595784899,-12.9506489081087,
119.882241065313)) ;
#191607=CARTESIAN_POINT('Ctrl Pts',(-9.46933981424234,-12.950649002057,
119.858010063142)) ;
#191608=CARTESIAN_POINT('Ctrl Pts',(-9.44760475251543,-12.9807689853667,
119.791808570075)) ;
#191609=CARTESIAN_POINT('Ctrl Pts',(-9.38982768745498,-12.7323944980461,
119.651262965745)) ;
#191610=CARTESIAN_POINT('Ctrl Pts',(-9.37136074583974,-12.7799004526929,
119.595015639306)) ;
#191611=CARTESIAN_POINT('Ctrl Pts',(-9.29755688290444,-12.7799003762679,
119.619246621551)) ;
#191612=CARTESIAN_POINT('Ctrl Pts',(-9.22375301996916,-12.7799002998429,
119.643477603796)) ;
#191613=CARTESIAN_POINT('Ctrl Pts',(-9.24221996158439,-12.7323943451961,
119.699724930235)) ;
#191614=CARTESIAN_POINT('Ctrl Pts',(-9.26068690319964,-12.6848883905494,
119.755972256675)) ;
#191615=CARTESIAN_POINT('Ctrl Pts',(-9.33449076613494,-12.6848884669744,
119.73174127443)) ;
#191616=CARTESIAN_POINT('Ctrl Pts',(-9.4082946290702,-12.6848885433994,
119.707510292184)) ;
#191617=CARTESIAN_POINT('Ctrl Pts',(-9.38982768745498,-12.7323944980461,
119.651262965745)) ;
#191618=CARTESIAN_POINT('Ctrl Pts',(-9.31302269296055,-12.5325218808407,
119.452855618209)) ;
#191619=CARTESIAN_POINT('Ctrl Pts',(-9.29915514898113,-12.594053905958,
119.410617314963)) ;
#191620=CARTESIAN_POINT('Ctrl Pts',(-9.22535128175568,-12.5940538521665,
119.434848284141)) ;
#191621=CARTESIAN_POINT('Ctrl Pts',(-9.15154741453021,-12.594053798375,
119.459079253319)) ;
#191622=CARTESIAN_POINT('Ctrl Pts',(-9.16541495850962,-12.5325217732577,
119.501317556565)) ;
#191623=CARTESIAN_POINT('Ctrl Pts',(-9.17928250248903,-12.4709897481403,
119.543555859811)) ;
#191624=CARTESIAN_POINT('Ctrl Pts',(-9.2530863697145,-12.4709898019318,
119.519324890633)) ;
#191625=CARTESIAN_POINT('Ctrl Pts',(-9.32689023693996,-12.4709898557234,
119.495093921455)) ;
#191626=CARTESIAN_POINT('Ctrl Pts',(-9.31302269296055,-12.5325218808407,
119.452855618209)) ;
#191627=CARTESIAN_POINT('Ctrl Pts',(-9.2220091378968,-12.3964669498525,
119.211168926867)) ;
#191628=CARTESIAN_POINT('Ctrl Pts',(-9.21373997527486,-12.4675909509527,
119.185982390066)) ;
#191629=CARTESIAN_POINT('Ctrl Pts',(-9.13993610636165,-12.4675909216126,
119.210213354104)) ;
#191630=CARTESIAN_POINT('Ctrl Pts',(-9.06613223744845,-12.4675908922725,
119.234444318141)) ;
#191631=CARTESIAN_POINT('Ctrl Pts',(-9.07440140007039,-12.3964668911723,
119.259630854942)) ;
#191632=CARTESIAN_POINT('Ctrl Pts',(-9.08267056269233,-12.3253428900721,
119.284817391743)) ;
#191633=CARTESIAN_POINT('Ctrl Pts',(-9.15647443160554,-12.3253429194122,
119.260586427706)) ;
#191634=CARTESIAN_POINT('Ctrl Pts',(-9.23027830051874,-12.3253429487523,
119.236355463668)) ;
#191635=CARTESIAN_POINT('Ctrl Pts',(-9.2220091378968,-12.3964669498525,
119.211168926867)) ;
#191636=CARTESIAN_POINT('Ctrl Pts',(-9.12316400642471,-12.3339203423186,
118.945439966049)) ;
#191637=CARTESIAN_POINT('Ctrl Pts',(-9.12105247455863,-12.4095182646376,
118.939008579113)) ;
#191638=CARTESIAN_POINT('Ctrl Pts',(-9.04724860595158,-12.4095182584409,
118.963239544083)) ;
#191639=CARTESIAN_POINT('Ctrl Pts',(-8.97344473734454,-12.4095182522441,
118.987470509053)) ;
#191640=CARTESIAN_POINT('Ctrl Pts',(-8.97555626921059,-12.3339203299251,
118.993901895989)) ;
#191641=CARTESIAN_POINT('Ctrl Pts',(-8.97766780107668,-12.2583224076062,
119.000333282924)) ;
#191642=CARTESIAN_POINT('Ctrl Pts',(-9.05147166968372,-12.2583224138029,
118.976102317954)) ;
#191643=CARTESIAN_POINT('Ctrl Pts',(-9.12527553829077,-12.2583224199996,
118.951871352984)) ;
#191644=CARTESIAN_POINT('Ctrl Pts',(-9.12316400642471,-12.3339203423186,
118.945439966049)) ;
#191645=CARTESIAN_POINT('Ctrl Pts',(-9.02196719116671,-12.3484596551531,
118.672664621969)) ;
#191646=CARTESIAN_POINT('Ctrl Pts',(-9.02618431696446,-12.4231567143316,
118.685509305294)) ;
#191647=CARTESIAN_POINT('Ctrl Pts',(-8.95238045100166,-12.423156728635,
118.709740278318)) ;
#191648=CARTESIAN_POINT('Ctrl Pts',(-8.87857658503889,-12.4231567429385,
118.733971251342)) ;
#191649=CARTESIAN_POINT('Ctrl Pts',(-8.87435945924114,-12.34845968376,118.721126568017)) ;
#191650=CARTESIAN_POINT('Ctrl Pts',(-8.87014233344338,-12.2737626245815,
118.708281884692)) ;
#191651=CARTESIAN_POINT('Ctrl Pts',(-8.94394619940617,-12.2737626102781,
118.684050911668)) ;
#191652=CARTESIAN_POINT('Ctrl Pts',(-9.01775006536895,-12.2737625959746,
118.659819938644)) ;
#191653=CARTESIAN_POINT('Ctrl Pts',(-9.02196719116671,-12.3484596551531,
118.672664621969)) ;
#191654=CARTESIAN_POINT('Ctrl Pts',(-8.9249315758202,-12.44015832593,118.412680001706)) ;
#191655=CARTESIAN_POINT('Ctrl Pts',(-8.93519409242402,-12.5085664478243,
118.443937970181)) ;
#191656=CARTESIAN_POINT('Ctrl Pts',(-8.86139023098923,-12.508566476899,
118.468168956996)) ;
#191657=CARTESIAN_POINT('Ctrl Pts',(-8.78758636955445,-12.5085665059736,
118.492399943812)) ;
#191658=CARTESIAN_POINT('Ctrl Pts',(-8.77732385295063,-12.4401583840793,
118.461141975338)) ;
#191659=CARTESIAN_POINT('Ctrl Pts',(-8.76706133634684,-12.371750262185,
118.429884006863)) ;
#191660=CARTESIAN_POINT('Ctrl Pts',(-8.84086519778162,-12.3717502331104,
118.405653020048)) ;
#191661=CARTESIAN_POINT('Ctrl Pts',(-8.9146690592164,-12.3717502040357,
118.381422033232)) ;
#191662=CARTESIAN_POINT('Ctrl Pts',(-8.9249315758202,-12.44015832593,118.412680001706)) ;
#191663=CARTESIAN_POINT('Ctrl Pts',(-8.83885025035531,-12.6016814204418,
118.185950248879)) ;
#191664=CARTESIAN_POINT('Ctrl Pts',(-8.85440481641178,-12.6589156114348,
118.23332694628)) ;
#191665=CARTESIAN_POINT('Ctrl Pts',(-8.78060096001723,-12.6589156492429,
118.257557948447)) ;
#191666=CARTESIAN_POINT('Ctrl Pts',(-8.70679710362268,-12.6589156870509,
118.281788950615)) ;
#191667=CARTESIAN_POINT('Ctrl Pts',(-8.69124253756622,-12.6016814960579,
118.234412253214)) ;
#191668=CARTESIAN_POINT('Ctrl Pts',(-8.67568797150973,-12.5444473050649,
118.187035555813)) ;
#191669=CARTESIAN_POINT('Ctrl Pts',(-8.7494918279043,-12.5444472672568,
118.162804553645)) ;
#191670=CARTESIAN_POINT('Ctrl Pts',(-8.82329568429883,-12.5444472294488,
118.138573551478)) ;
#191671=CARTESIAN_POINT('Ctrl Pts',(-8.83885025035531,-12.6016814204418,
118.185950248879)) ;
#191672=CARTESIAN_POINT('Ctrl Pts',(-8.76869825092151,-12.8223735055108,
118.007837352754)) ;
#191673=CARTESIAN_POINT('Ctrl Pts',(-8.78843878657979,-12.8642856579198,
118.067963838344)) ;
#191674=CARTESIAN_POINT('Ctrl Pts',(-8.71463493540657,-12.8642856973606,
118.092194856415)) ;
#191675=CARTESIAN_POINT('Ctrl Pts',(-8.64083108423339,-12.8642857368014,
118.116425874486)) ;
#191676=CARTESIAN_POINT('Ctrl Pts',(-8.6210905485751,-12.8223735843924,
118.056299388895)) ;
#191677=CARTESIAN_POINT('Ctrl Pts',(-8.60135001291686,-12.7804614319833,
117.996172903305)) ;
#191678=CARTESIAN_POINT('Ctrl Pts',(-8.67515386409004,-12.7804613925425,
117.971941885234)) ;
#191679=CARTESIAN_POINT('Ctrl Pts',(-8.74895771526325,-12.7804613531017,
117.947710867163)) ;
#191680=CARTESIAN_POINT('Ctrl Pts',(-8.76869825092151,-12.8223735055108,
118.007837352754)) ;
#191681=CARTESIAN_POINT('Ctrl Pts',(-8.71926001658606,-13.0840251447648,
117.892569881876)) ;
#191682=CARTESIAN_POINT('Ctrl Pts',(-8.74175151045566,-13.1077315684995,
117.961075342452)) ;
#191683=CARTESIAN_POINT('Ctrl Pts',(-8.6679476634762,-13.1077316062093,
117.985306373297)) ;
#191684=CARTESIAN_POINT('Ctrl Pts',(-8.59414381649674,-13.1077316439191,
118.009537404141)) ;
#191685=CARTESIAN_POINT('Ctrl Pts',(-8.57165232262716,-13.0840252201844,
117.941031943565)) ;
#191686=CARTESIAN_POINT('Ctrl Pts',(-8.54916082875752,-13.0603187964498,
117.872526482989)) ;
#191687=CARTESIAN_POINT('Ctrl Pts',(-8.62296467573699,-13.06031875874,117.848295452145)) ;
#191688=CARTESIAN_POINT('Ctrl Pts',(-8.69676852271643,-13.0603187210301,
117.8240644213)) ;
#191689=CARTESIAN_POINT('Ctrl Pts',(-8.71926001658606,-13.0840251447648,
117.892569881876)) ;
#191690=CARTESIAN_POINT('Ctrl Pts',(-8.69264272124601,-13.370624374638,
117.846967346644)) ;
#191691=CARTESIAN_POINT('Ctrl Pts',(-8.7162928406045,-13.3743556073404,
117.919001793682)) ;
#191692=CARTESIAN_POINT('Ctrl Pts',(-8.64248899702783,-13.3743556381557,
117.943232834891)) ;
#191693=CARTESIAN_POINT('Ctrl Pts',(-8.56868515345113,-13.3743556689709,
117.967463876099)) ;
#191694=CARTESIAN_POINT('Ctrl Pts',(-8.54503503409265,-13.3706244362685,
117.895429429062)) ;
#191695=CARTESIAN_POINT('Ctrl Pts',(-8.52138491473414,-13.3668932035661,
117.823394982024)) ;
#191696=CARTESIAN_POINT('Ctrl Pts',(-8.59518875831084,-13.3668931727509,
117.799163940815)) ;
#191697=CARTESIAN_POINT('Ctrl Pts',(-8.66899260188751,-13.3668931419356,
117.774932899606)) ;
#191698=CARTESIAN_POINT('Ctrl Pts',(-8.69264272124601,-13.370624374638,
117.846967346644)) ;
#191699=CARTESIAN_POINT('Ctrl Pts',(-8.69038448104888,-13.6607958553262,
117.875577804038)) ;
#191700=CARTESIAN_POINT('Ctrl Pts',(-8.71349373520954,-13.6442717980086,
117.945964863113)) ;
#191701=CARTESIAN_POINT('Ctrl Pts',(-8.63968989357253,-13.6442718197528,
117.970195910229)) ;
#191702=CARTESIAN_POINT('Ctrl Pts',(-8.56588605193551,-13.6442718414971,
117.994426957346)) ;
#191703=CARTESIAN_POINT('Ctrl Pts',(-8.54277679777483,-13.6607958988147,
117.924039898271)) ;
#191704=CARTESIAN_POINT('Ctrl Pts',(-8.51966754361415,-13.6773199561323,
117.853652839196)) ;
#191705=CARTESIAN_POINT('Ctrl Pts',(-8.59347138525118,-13.6773199343881,
117.82942179208)) ;
#191706=CARTESIAN_POINT('Ctrl Pts',(-8.6672752268882,-13.6773199126438,
117.805190744963)) ;
#191707=CARTESIAN_POINT('Ctrl Pts',(-8.69038448104888,-13.6607958553262,
117.875577804038)) ;
#191708=CARTESIAN_POINT('Ctrl Pts',(-8.711753214821,-13.9332273193549,117.976096242106)) ;
#191709=CARTESIAN_POINT('Ctrl Pts',(-8.73267209967682,-13.8976559253995,
118.039811789834)) ;
#191710=CARTESIAN_POINT('Ctrl Pts',(-8.65886825869564,-13.8976559384048,
118.064042838948)) ;
#191711=CARTESIAN_POINT('Ctrl Pts',(-8.58506441771443,-13.8976559514102,
118.088273888062)) ;
#191712=CARTESIAN_POINT('Ctrl Pts',(-8.56414553285862,-13.9332273453655,
118.024558340334)) ;
#191713=CARTESIAN_POINT('Ctrl Pts',(-8.54322664800276,-13.9687987393209,
117.960842792606)) ;
#191714=CARTESIAN_POINT('Ctrl Pts',(-8.61703048898397,-13.9687987263155,
117.936611743492)) ;
#191715=CARTESIAN_POINT('Ctrl Pts',(-8.69083432996515,-13.9687987133102,
117.912380694378)) ;
#191716=CARTESIAN_POINT('Ctrl Pts',(-8.711753214821,-13.9332273193549,117.976096242106)) ;
#191717=CARTESIAN_POINT('Ctrl Pts',(-8.75479531072491,-14.1696161307288,
118.142792114175)) ;
#191718=CARTESIAN_POINT('Ctrl Pts',(-8.77200370839762,-14.117484643747,
118.195206116772)) ;
#191719=CARTESIAN_POINT('Ctrl Pts',(-8.6981998667684,-14.1174846489895,
118.219437163913)) ;
#191720=CARTESIAN_POINT('Ctrl Pts',(-8.62439602513918,-14.117484654232,
118.243668211053)) ;
#191721=CARTESIAN_POINT('Ctrl Pts',(-8.60718762746647,-14.1696161412137,
118.191254208456)) ;
#191722=CARTESIAN_POINT('Ctrl Pts',(-8.58997922979378,-14.2217476281955,
118.138840205859)) ;
#191723=CARTESIAN_POINT('Ctrl Pts',(-8.66378307142299,-14.221747622953,
118.114609158719)) ;
#191724=CARTESIAN_POINT('Ctrl Pts',(-8.73758691305221,-14.2217476177105,
118.090378111578)) ;
#191725=CARTESIAN_POINT('Ctrl Pts',(-8.75479531072491,-14.1696161307288,
118.142792114175)) ;
#191726=CARTESIAN_POINT('Ctrl Pts',(-8.8148406701214,-14.3504842744957,
118.360928178299)) ;
#191727=CARTESIAN_POINT('Ctrl Pts',(-8.82715272549973,-14.285645743084,
118.39842871237)) ;
#191728=CARTESIAN_POINT('Ctrl Pts',(-8.75334888310061,-14.2856457445399,
118.422659757166)) ;
#191729=CARTESIAN_POINT('Ctrl Pts',(-8.67954504070153,-14.2856457459958,
118.446890801961)) ;
#191730=CARTESIAN_POINT('Ctrl Pts',(-8.6672329853232,-14.3504842774075,
118.40939026789)) ;
#191731=CARTESIAN_POINT('Ctrl Pts',(-8.65492092994486,-14.4153228088192,
118.371889733819)) ;
#191732=CARTESIAN_POINT('Ctrl Pts',(-8.72872477234397,-14.4153228073633,
118.347658689024)) ;
#191733=CARTESIAN_POINT('Ctrl Pts',(-8.80252861474306,-14.4153228059074,
118.323427644228)) ;
#191734=CARTESIAN_POINT('Ctrl Pts',(-8.8148406701214,-14.3504842744957,
118.360928178299)) ;
#191735=CARTESIAN_POINT('Ctrl Pts',(-8.88828842378017,-14.4664314373378,
118.620362245209)) ;
#191736=CARTESIAN_POINT('Ctrl Pts',(-8.89475089159606,-14.393398523113,
118.640045879492)) ;
#191737=CARTESIAN_POINT('Ctrl Pts',(-8.82094704774123,-14.3933985223856,
118.664276919853)) ;
#191738=CARTESIAN_POINT('Ctrl Pts',(-8.74714320388638,-14.3933985216583,
118.688507960215)) ;
#191739=CARTESIAN_POINT('Ctrl Pts',(-8.7406807360705,-14.4664314358832,
118.668824325932)) ;
#191740=CARTESIAN_POINT('Ctrl Pts',(-8.73421826825462,-14.539464350108,
118.64914069165)) ;
#191741=CARTESIAN_POINT('Ctrl Pts',(-8.80802211210946,-14.5394643508353,
118.624909651288)) ;
#191742=CARTESIAN_POINT('Ctrl Pts',(-8.88182595596429,-14.5394643515627,
118.600678610927)) ;
#191743=CARTESIAN_POINT('Ctrl Pts',(-8.88828842378017,-14.4664314373378,
118.620362245209)) ;
#191744=CARTESIAN_POINT('Ctrl Pts',(-8.96751292468527,-14.505814940549,
118.8970150562)) ;
#191745=CARTESIAN_POINT('Ctrl Pts',(-8.96772137448786,-14.4299235771365,
118.897649960723)) ;
#191746=CARTESIAN_POINT('Ctrl Pts',(-8.89391753013919,-14.4299235770663,
118.92188099958)) ;
#191747=CARTESIAN_POINT('Ctrl Pts',(-8.82011368579049,-14.429923576996,
118.946112038437)) ;
#191748=CARTESIAN_POINT('Ctrl Pts',(-8.81990523598791,-14.5058149404085,
118.945477133914)) ;
#191749=CARTESIAN_POINT('Ctrl Pts',(-8.81969678618531,-14.5817063038209,
118.944842229391)) ;
#191750=CARTESIAN_POINT('Ctrl Pts',(-8.893500630534,-14.5817063038912,118.920611190534)) ;
#191751=CARTESIAN_POINT('Ctrl Pts',(-8.96730447488267,-14.5817063039614,
118.896380151676)) ;
#191752=CARTESIAN_POINT('Ctrl Pts',(-8.96751292468527,-14.505814940549,
118.8970150562)) ;
#191753=CARTESIAN_POINT('Ctrl Pts',(-9.04680096010112,-14.46830400306,119.173859350138)) ;
#191754=CARTESIAN_POINT('Ctrl Pts',(-9.04074169525011,-14.3949198444241,
119.155403807125)) ;
#191755=CARTESIAN_POINT('Ctrl Pts',(-8.96693785085317,-14.3949198453838,
119.179634845835)) ;
#191756=CARTESIAN_POINT('Ctrl Pts',(-8.89313400645622,-14.3949198463436,
119.203865884545)) ;
#191757=CARTESIAN_POINT('Ctrl Pts',(-8.89919327130725,-14.4683040049795,
119.222321427559)) ;
#191758=CARTESIAN_POINT('Ctrl Pts',(-8.90525253615825,-14.5416881636154,
119.240776970572)) ;
#191759=CARTESIAN_POINT('Ctrl Pts',(-8.9790563805552,-14.5416881626556,
119.216545931862)) ;
#191760=CARTESIAN_POINT('Ctrl Pts',(-9.05286022495216,-14.5416881616959,
119.192314893152)) ;
#191761=CARTESIAN_POINT('Ctrl Pts',(-9.04680096010112,-14.46830400306,119.173859350138)) ;
#191762=CARTESIAN_POINT('Ctrl Pts',(-9.12041342587677,-14.3544455833434,
119.433744666185)) ;
#191763=CARTESIAN_POINT('Ctrl Pts',(-9.10846654169691,-14.28890351008,119.397356384606)) ;
#191764=CARTESIAN_POINT('Ctrl Pts',(-9.03466269818544,-14.2889035106551,
119.421587426014)) ;
#191765=CARTESIAN_POINT('Ctrl Pts',(-8.96085885467401,-14.2889035112301,
119.445818467421)) ;
#191766=CARTESIAN_POINT('Ctrl Pts',(-8.97280573885388,-14.3544455844935,
119.482206748999)) ;
#191767=CARTESIAN_POINT('Ctrl Pts',(-8.98475262303375,-14.4199876577569,
119.518595030578)) ;
#191768=CARTESIAN_POINT('Ctrl Pts',(-9.05855646654521,-14.4199876571819,
119.49436398917)) ;
#191769=CARTESIAN_POINT('Ctrl Pts',(-9.13236031005665,-14.4199876566068,
119.470132947763)) ;
#191770=CARTESIAN_POINT('Ctrl Pts',(-9.12041342587677,-14.3544455833434,
119.433744666185)) ;
#191771=CARTESIAN_POINT('Ctrl Pts',(-9.1810115636041,-14.1743504235921,
119.653691355209)) ;
#191772=CARTESIAN_POINT('Ctrl Pts',(-9.16408389144678,-14.1212879349947,
119.602132397024)) ;
#191773=CARTESIAN_POINT('Ctrl Pts',(-9.09028004882841,-14.121287932882,
119.626363441152)) ;
#191774=CARTESIAN_POINT('Ctrl Pts',(-9.01647620621002,-14.1212879307693,
119.650594485279)) ;
#191775=CARTESIAN_POINT('Ctrl Pts',(-9.03340387836735,-14.1743504193667,
119.702153443464)) ;
#191776=CARTESIAN_POINT('Ctrl Pts',(-9.05033155052467,-14.2274129079642,
119.753712401649)) ;
#191777=CARTESIAN_POINT('Ctrl Pts',(-9.12413539314305,-14.2274129100769,
119.729481357522)) ;
#191778=CARTESIAN_POINT('Ctrl Pts',(-9.19793923576142,-14.2274129121895,
119.705250313394)) ;
#191779=CARTESIAN_POINT('Ctrl Pts',(-9.1810115636041,-14.1743504235921,
119.653691355209)) ;
#191780=CARTESIAN_POINT('Ctrl Pts',(-9.22434028506487,-13.9404023706078,
119.821067847651)) ;
#191781=CARTESIAN_POINT('Ctrl Pts',(-9.20362990504079,-13.9035978670998,
119.757987371546)) ;
#191782=CARTESIAN_POINT('Ctrl Pts',(-9.12982606302781,-13.903597860184,
119.782218417518)) ;
#191783=CARTESIAN_POINT('Ctrl Pts',(-9.05602222101485,-13.9035978532681,
119.806449463489)) ;
#191784=CARTESIAN_POINT('Ctrl Pts',(-9.07673260103893,-13.940402356776,
119.869529939594)) ;
#191785=CARTESIAN_POINT('Ctrl Pts',(-9.09744298106302,-13.977206860284,
119.932610415698)) ;
#191786=CARTESIAN_POINT('Ctrl Pts',(-9.17124682307598,-13.9772068671999,
119.908379369727)) ;
#191787=CARTESIAN_POINT('Ctrl Pts',(-9.24505066508896,-13.9772068741157,
119.884148323755)) ;
#191788=CARTESIAN_POINT('Ctrl Pts',(-9.22434028506487,-13.9404023706078,
119.821067847651)) ;
#191789=CARTESIAN_POINT('Ctrl Pts',(-9.24641752481561,-13.6671888266285,
119.923944245978)) ;
#191790=CARTESIAN_POINT('Ctrl Pts',(-9.22339798409645,-13.6494076085659,
119.853830438823)) ;
#191791=CARTESIAN_POINT('Ctrl Pts',(-9.14959414204322,-13.6494075929638,
119.878061484672)) ;
#191792=CARTESIAN_POINT('Ctrl Pts',(-9.07579029998996,-13.6494075773616,
119.902292530521)) ;
#191793=CARTESIAN_POINT('Ctrl Pts',(-9.09880984070912,-13.6671887954242,
119.972406337675)) ;
#191794=CARTESIAN_POINT('Ctrl Pts',(-9.12182938142827,-13.6849700134867,
120.042520144829)) ;
#191795=CARTESIAN_POINT('Ctrl Pts',(-9.19563322348152,-13.6849700290889,
120.018289098981)) ;
#191796=CARTESIAN_POINT('Ctrl Pts',(-9.26943706553476,-13.684970044691,
119.994058053132)) ;
#191797=CARTESIAN_POINT('Ctrl Pts',(-9.24641752481561,-13.6671888266285,
119.923944245978)) ;
#191798=CARTESIAN_POINT('Ctrl Pts',(-9.24470708760251,-13.3783758394987,
119.954073987494)) ;
#191799=CARTESIAN_POINT('Ctrl Pts',(-9.22104244183216,-13.3807343880949,
119.881995294314)) ;
#191800=CARTESIAN_POINT('Ctrl Pts',(-9.14723859835509,-13.3807343653365,
119.906226335826)) ;
#191801=CARTESIAN_POINT('Ctrl Pts',(-9.07343475487802,-13.3807343425781,
119.930457377338)) ;
#191802=CARTESIAN_POINT('Ctrl Pts',(-9.09709940064837,-13.3783757939819,
120.002536070518)) ;
#191803=CARTESIAN_POINT('Ctrl Pts',(-9.12076404641873,-13.3760172453858,
120.074614763697)) ;
#191804=CARTESIAN_POINT('Ctrl Pts',(-9.19456788989579,-13.3760172681442,
120.050383722185)) ;
#191805=CARTESIAN_POINT('Ctrl Pts',(-9.26837173337287,-13.3760172909026,
120.026152680673)) ;
#191806=CARTESIAN_POINT('Ctrl Pts',(-9.24470708760251,-13.3783758394987,
119.954073987494)) ;
#191807=CARTESIAN_POINT('Ctrl Pts',(-9.21880682278639,-13.0914976589315,
119.910642708643)) ;
#191808=CARTESIAN_POINT('Ctrl Pts',(-9.19618261652847,-13.1138898142191,
119.841733026189)) ;
#191809=CARTESIAN_POINT('Ctrl Pts',(-9.12237877045627,-13.113889784642,
119.865964059796)) ;
#191810=CARTESIAN_POINT('Ctrl Pts',(-9.04857492438406,-13.1138897550648,
119.890195093404)) ;
#191811=CARTESIAN_POINT('Ctrl Pts',(-9.07119913064198,-13.0914975997771,
119.959104775858)) ;
#191812=CARTESIAN_POINT('Ctrl Pts',(-9.09382333689987,-13.0691054444894,
120.028014458313)) ;
#191813=CARTESIAN_POINT('Ctrl Pts',(-9.1676271829721,-13.0691054740666,
120.003783424705)) ;
#191814=CARTESIAN_POINT('Ctrl Pts',(-9.24143102904429,-13.0691055036438,
119.979552391098)) ;
#191815=CARTESIAN_POINT('Ctrl Pts',(-9.21880682278639,-13.0914976589315,
119.910642708643)) ;
#191816=CARTESIAN_POINT('Ctrl Pts',(-9.16970010340457,-12.827936357185,
119.796531141099)) ;
#191817=CARTESIAN_POINT('Ctrl Pts',(-9.14973808973235,-12.8687628272745,
119.735730067553)) ;
#191818=CARTESIAN_POINT('Ctrl Pts',(-9.07593423988325,-12.8687627938338,
119.759961089656)) ;
#191819=CARTESIAN_POINT('Ctrl Pts',(-9.00213039003418,-12.868762760393,
119.78419211176)) ;
#191820=CARTESIAN_POINT('Ctrl Pts',(-9.02209240370642,-12.8279362903035,
119.844993185306)) ;
#191821=CARTESIAN_POINT('Ctrl Pts',(-9.04205441737867,-12.7871098202139,
119.905794258852)) ;
#191822=CARTESIAN_POINT('Ctrl Pts',(-9.11585826722775,-12.7871098536547,
119.881563236748)) ;
#191823=CARTESIAN_POINT('Ctrl Pts',(-9.18966211707683,-12.7871098870954,
119.857332214645)) ;
#191824=CARTESIAN_POINT('Ctrl Pts',(-9.16970010340457,-12.827936357185,
119.796531141099)) ;
#191825=CARTESIAN_POINT('Ctrl Pts',(-9.09997329978592,-12.6061166858968,
119.619706123168)) ;
#191826=CARTESIAN_POINT('Ctrl Pts',(-9.08411501804255,-12.662489659223,
119.571404354757)) ;
#191827=CARTESIAN_POINT('Ctrl Pts',(-9.01031116342983,-12.6624896260607,
119.595635362352)) ;
#191828=CARTESIAN_POINT('Ctrl Pts',(-8.93650730881713,-12.6624895928983,
119.619866369947)) ;
#191829=CARTESIAN_POINT('Ctrl Pts',(-8.95236559056048,-12.6061166195721,
119.668168138357)) ;
#191830=CARTESIAN_POINT('Ctrl Pts',(-8.96822387230382,-12.5497436462459,
119.716469906768)) ;
#191831=CARTESIAN_POINT('Ctrl Pts',(-9.04202772691654,-12.5497436794083,
119.692238899173)) ;
#191832=CARTESIAN_POINT('Ctrl Pts',(-9.11583158152926,-12.5497437125706,
119.668007891578)) ;
#191833=CARTESIAN_POINT('Ctrl Pts',(-9.09997329978592,-12.6061166858968,
119.619706123168)) ;
#191834=CARTESIAN_POINT('Ctrl Pts',(-9.01413184976296,-12.4431271546039,
119.393730189171)) ;
#191835=CARTESIAN_POINT('Ctrl Pts',(-9.0035097601658,-12.5109613838961,
119.361377017011)) ;
#191836=CARTESIAN_POINT('Ctrl Pts',(-8.92970590071719,-12.510961357698,
119.385608009876)) ;
#191837=CARTESIAN_POINT('Ctrl Pts',(-8.85590204126855,-12.5109613315,119.409839002741)) ;
#191838=CARTESIAN_POINT('Ctrl Pts',(-8.86652413086572,-12.4431271022078,
119.442192174902)) ;
#191839=CARTESIAN_POINT('Ctrl Pts',(-8.87714622046288,-12.3752928729157,
119.474545347062)) ;
#191840=CARTESIAN_POINT('Ctrl Pts',(-8.95095007991151,-12.3752928991138,
119.450314354197)) ;
#191841=CARTESIAN_POINT('Ctrl Pts',(-9.02475393936012,-12.3752929253118,
119.426083361332)) ;
#191842=CARTESIAN_POINT('Ctrl Pts',(-9.01413184976296,-12.4431271546039,
119.393730189171)) ;
#191843=CARTESIAN_POINT('Ctrl Pts',(-8.91797994965442,-12.3502094912987,
119.136186372322)) ;
#191844=CARTESIAN_POINT('Ctrl Pts',(-8.91332488011852,-12.4246287371788,
119.122007780357)) ;
#191845=CARTESIAN_POINT('Ctrl Pts',(-8.83952101692612,-12.4246287241844,
119.14623876182)) ;
#191846=CARTESIAN_POINT('Ctrl Pts',(-8.76571715373373,-12.42462871119,119.170469743282)) ;
#191847=CARTESIAN_POINT('Ctrl Pts',(-8.77037222326963,-12.35020946531,119.184648335247)) ;
#191848=CARTESIAN_POINT('Ctrl Pts',(-8.77502729280552,-12.2757902194299,
119.198826927212)) ;
#191849=CARTESIAN_POINT('Ctrl Pts',(-8.84883115599792,-12.2757902324242,
119.174595945749)) ;
#191850=CARTESIAN_POINT('Ctrl Pts',(-8.92263501919031,-12.2757902454186,
119.150364964287)) ;
#191851=CARTESIAN_POINT('Ctrl Pts',(-8.91797994965442,-12.3502094912987,
119.136186372322)) ;
#191852=CARTESIAN_POINT('Ctrl Pts',(-8.81678556357941,-12.3330949628537,
118.863432839579)) ;
#191853=CARTESIAN_POINT('Ctrl Pts',(-8.81845498558905,-12.4088168292008,
118.868517628251)) ;
#191854=CARTESIAN_POINT('Ctrl Pts',(-8.744651119493,-12.4088168339974,118.892748600869)) ;
#191855=CARTESIAN_POINT('Ctrl Pts',(-8.67084725339693,-12.408816838794,
118.916979573487)) ;
#191856=CARTESIAN_POINT('Ctrl Pts',(-8.66917783138726,-12.3330949724469,
118.911894784815)) ;
#191857=CARTESIAN_POINT('Ctrl Pts',(-8.66750840937762,-12.2573731060998,
118.906809996142)) ;
#191858=CARTESIAN_POINT('Ctrl Pts',(-8.74131227547369,-12.2573731013032,
118.882579023524)) ;
#191859=CARTESIAN_POINT('Ctrl Pts',(-8.81511614156976,-12.2573730965066,
118.858348050906)) ;
#191860=CARTESIAN_POINT('Ctrl Pts',(-8.81678556357941,-12.3330949628537,
118.863432839579)) ;
#191861=CARTESIAN_POINT('Ctrl Pts',(-8.71722634028701,-12.3941323979468,
118.595736689137)) ;
#191862=CARTESIAN_POINT('Ctrl Pts',(-8.72511363131764,-12.4657028650143,
118.619760103441)) ;
#191863=CARTESIAN_POINT('Ctrl Pts',(-8.65130976405657,-12.4657028918637,
118.64399107251)) ;
#191864=CARTESIAN_POINT('Ctrl Pts',(-8.57750589679551,-12.4657029187131,
118.66822204158)) ;
#191865=CARTESIAN_POINT('Ctrl Pts',(-8.56961860576491,-12.3941324516456,
118.644198627277)) ;
#191866=CARTESIAN_POINT('Ctrl Pts',(-8.56173131473427,-12.3225619845781,
118.620175212973)) ;
#191867=CARTESIAN_POINT('Ctrl Pts',(-8.63553518199533,-12.3225619577287,
118.595944243904)) ;
#191868=CARTESIAN_POINT('Ctrl Pts',(-8.70933904925639,-12.3225619308793,
118.571713274834)) ;
#191869=CARTESIAN_POINT('Ctrl Pts',(-8.71722634028701,-12.3941323979468,
118.595736689137)) ;
#191870=CARTESIAN_POINT('Ctrl Pts',(-8.62633858589104,-12.5280047279255,
118.354282868859)) ;
#191871=CARTESIAN_POINT('Ctrl Pts',(-8.63985083191165,-12.5903323506603,
118.395438988361)) ;
#191872=CARTESIAN_POINT('Ctrl Pts',(-8.56604696618086,-12.5903324003766,
118.419669962092)) ;
#191873=CARTESIAN_POINT('Ctrl Pts',(-8.49224310045005,-12.5903324500929,
118.443900935822)) ;
#191874=CARTESIAN_POINT('Ctrl Pts',(-8.47873085442944,-12.5280048273581,
118.40274481632)) ;
#191875=CARTESIAN_POINT('Ctrl Pts',(-8.46521860840883,-12.4656772046233,
118.361588696818)) ;
#191876=CARTESIAN_POINT('Ctrl Pts',(-8.53902247413964,-12.465677154907,
118.337357723088)) ;
#191877=CARTESIAN_POINT('Ctrl Pts',(-8.61282633987043,-12.4656771051907,
118.313126749357)) ;
#191878=CARTESIAN_POINT('Ctrl Pts',(-8.62633858589104,-12.5280047279255,
118.354282868859)) ;
#191879=CARTESIAN_POINT('Ctrl Pts',(-8.54913265153816,-12.725823043926,
118.15460227813)) ;
#191880=CARTESIAN_POINT('Ctrl Pts',(-8.56732074945708,-12.7744304923816,
118.210000287949)) ;
#191881=CARTESIAN_POINT('Ctrl Pts',(-8.49351688740926,-12.7744305640523,
118.234231272897)) ;
#191882=CARTESIAN_POINT('Ctrl Pts',(-8.41971302536143,-12.7744306357229,
118.258462257845)) ;
#191883=CARTESIAN_POINT('Ctrl Pts',(-8.40152492744251,-12.7258231872673,
118.203064248026)) ;
#191884=CARTESIAN_POINT('Ctrl Pts',(-8.38333682952358,-12.6772157388117,
118.147666238207)) ;
#191885=CARTESIAN_POINT('Ctrl Pts',(-8.45714069157141,-12.677215667141,
118.123435253259)) ;
#191886=CARTESIAN_POINT('Ctrl Pts',(-8.53094455361923,-12.6772155954704,
118.099204268311)) ;
#191887=CARTESIAN_POINT('Ctrl Pts',(-8.54913265153816,-12.725823043926,
118.15460227813)) ;
#191888=CARTESIAN_POINT('Ctrl Pts',(-8.49060543502265,-12.9740366931117,
118.011903735962)) ;
#191889=CARTESIAN_POINT('Ctrl Pts',(-8.51217039092456,-13.0053860395,118.077587110234)) ;
#191890=CARTESIAN_POINT('Ctrl Pts',(-8.43836653480978,-13.0053861296798,
118.101818113253)) ;
#191891=CARTESIAN_POINT('Ctrl Pts',(-8.36456267869501,-13.0053862198596,
118.126049116273)) ;
#191892=CARTESIAN_POINT('Ctrl Pts',(-8.3429977227931,-12.9740368734713,
118.060365742)) ;
#191893=CARTESIAN_POINT('Ctrl Pts',(-8.3214327668912,-12.942687527083,117.994682367728)) ;
#191894=CARTESIAN_POINT('Ctrl Pts',(-8.39523662300597,-12.9426874369032,
117.970451364709)) ;
#191895=CARTESIAN_POINT('Ctrl Pts',(-8.46904047912075,-12.9426873467234,
117.94622036169)) ;
#191896=CARTESIAN_POINT('Ctrl Pts',(-8.49060543502265,-12.9740366931117,
118.011903735962)) ;
#191897=CARTESIAN_POINT('Ctrl Pts',(-8.45445954867268,-13.2534633118697,
117.93728020588)) ;
#191898=CARTESIAN_POINT('Ctrl Pts',(-8.47784570948945,-13.2653501074278,
118.008510676394)) ;
#191899=CARTESIAN_POINT('Ctrl Pts',(-8.40404186114072,-13.2653502091921,
118.032741703068)) ;
#191900=CARTESIAN_POINT('Ctrl Pts',(-8.33023801279197,-13.2653503109564,
118.056972729741)) ;
#191901=CARTESIAN_POINT('Ctrl Pts',(-8.30685185197521,-13.2534635153983,
117.985742259227)) ;
#191902=CARTESIAN_POINT('Ctrl Pts',(-8.28346569115844,-13.2415767198401,
117.914511788712)) ;
#191903=CARTESIAN_POINT('Ctrl Pts',(-8.35726953950717,-13.2415766180759,
117.890280762039)) ;
#191904=CARTESIAN_POINT('Ctrl Pts',(-8.4310733878559,-13.2415765163116,
117.866049735365)) ;
#191905=CARTESIAN_POINT('Ctrl Pts',(-8.45445954867268,-13.2534633118697,
117.93728020588)) ;
#191906=CARTESIAN_POINT('Ctrl Pts',(-8.44237507272009,-13.5448240416985,
117.935968379582)) ;
#191907=CARTESIAN_POINT('Ctrl Pts',(-8.46590485409652,-13.5363866538712,
118.007636295091)) ;
#191908=CARTESIAN_POINT('Ctrl Pts',(-8.39210101449033,-13.5363867591239,
118.031867348393)) ;
#191909=CARTESIAN_POINT('Ctrl Pts',(-8.31829717488412,-13.5363868643766,
118.056098401694)) ;
#191910=CARTESIAN_POINT('Ctrl Pts',(-8.29476739350768,-13.544824252204,
117.984430486186)) ;
#191911=CARTESIAN_POINT('Ctrl Pts',(-8.27123761213126,-13.5532616400314,
117.912762570677)) ;
#191912=CARTESIAN_POINT('Ctrl Pts',(-8.34504145173747,-13.5532615347787,
117.888531517376)) ;
#191913=CARTESIAN_POINT('Ctrl Pts',(-8.41884529134366,-13.553261429526,
117.864300464074)) ;
#191914=CARTESIAN_POINT('Ctrl Pts',(-8.44237507272009,-13.5448240416985,
117.935968379582)) ;
#191915=CARTESIAN_POINT('Ctrl Pts',(-8.45433167813838,-13.8260554927979,
118.007737132418)) ;
#191916=CARTESIAN_POINT('Ctrl Pts',(-8.47632978159744,-13.7979711605236,
118.074739804093)) ;
#191917=CARTESIAN_POINT('Ctrl Pts',(-8.4025259507639,-13.7979712603347,
118.098970884115)) ;
#191918=CARTESIAN_POINT('Ctrl Pts',(-8.32872211993039,-13.7979713601458,
118.123201964137)) ;
#191919=CARTESIAN_POINT('Ctrl Pts',(-8.30672401647134,-13.8260556924201,
118.056199292462)) ;
#191920=CARTESIAN_POINT('Ctrl Pts',(-8.2847259130123,-13.8541400246944,
117.989196620786)) ;
#191921=CARTESIAN_POINT('Ctrl Pts',(-8.35852974384581,-13.8541399248833,
117.964965540765)) ;
#191922=CARTESIAN_POINT('Ctrl Pts',(-8.43233357467934,-13.8541398250722,
117.940734460743)) ;
#191923=CARTESIAN_POINT('Ctrl Pts',(-8.45433167813838,-13.8260554927979,
118.007737132418)) ;
#191924=CARTESIAN_POINT('Ctrl Pts',(-8.4890114847467,-14.0796928172426,
118.148954260656)) ;
#191925=CARTESIAN_POINT('Ctrl Pts',(-8.50788465162799,-14.0338589352342,
118.206438879706)) ;
#191926=CARTESIAN_POINT('Ctrl Pts',(-8.43408082879524,-14.033859021297,
118.230669984097)) ;
#191927=CARTESIAN_POINT('Ctrl Pts',(-8.36027700596246,-14.0338591073598,
118.254901088488)) ;
#191928=CARTESIAN_POINT('Ctrl Pts',(-8.34140383908118,-14.0796929893683,
118.197416469438)) ;
#191929=CARTESIAN_POINT('Ctrl Pts',(-8.32253067219987,-14.1255268713768,
118.139931850387)) ;
#191930=CARTESIAN_POINT('Ctrl Pts',(-8.39633449503265,-14.1255267853139,
118.115700745996)) ;
#191931=CARTESIAN_POINT('Ctrl Pts',(-8.47013831786541,-14.1255266992511,
118.091469641605)) ;
#191932=CARTESIAN_POINT('Ctrl Pts',(-8.4890114847467,-14.0796928172426,
118.148954260656)) ;
#191933=CARTESIAN_POINT('Ctrl Pts',(-8.54257172063092,-14.2840883967328,
118.347363105514)) ;
#191934=CARTESIAN_POINT('Ctrl Pts',(-8.55700344248699,-14.223916620712,
118.391319799648)) ;
#191935=CARTESIAN_POINT('Ctrl Pts',(-8.48319962595063,-14.2239166860408,
118.415550923217)) ;
#191936=CARTESIAN_POINT('Ctrl Pts',(-8.4093958094143,-14.2239167513696,
118.439782046786)) ;
#191937=CARTESIAN_POINT('Ctrl Pts',(-8.39496408755824,-14.2840885273904,
118.395825352652)) ;
#191938=CARTESIAN_POINT('Ctrl Pts',(-8.38053236570218,-14.3442603034112,
118.351868658518)) ;
#191939=CARTESIAN_POINT('Ctrl Pts',(-8.45433618223852,-14.3442602380824,
118.327637534949)) ;
#191940=CARTESIAN_POINT('Ctrl Pts',(-8.52813999877486,-14.3442601727535,
118.30340641138)) ;
#191941=CARTESIAN_POINT('Ctrl Pts',(-8.54257172063092,-14.2840883967328,
118.347363105514)) ;
#191942=CARTESIAN_POINT('Ctrl Pts',(-8.61125485980821,-14.4281001590278,
118.59212459814)) ;
#191943=CARTESIAN_POINT('Ctrl Pts',(-8.62017704976491,-14.3577843512303,
118.619300147099)) ;
#191944=CARTESIAN_POINT('Ctrl Pts',(-8.54637323724559,-14.3577843906291,
118.643531282903)) ;
#191945=CARTESIAN_POINT('Ctrl Pts',(-8.47256942472626,-14.357784430028,
118.667762418707)) ;
#191946=CARTESIAN_POINT('Ctrl Pts',(-8.46364723476955,-14.4281002378256,
118.640586869749)) ;
#191947=CARTESIAN_POINT('Ctrl Pts',(-8.45472504481283,-14.4984160456232,
118.61341132079)) ;
#191948=CARTESIAN_POINT('Ctrl Pts',(-8.52852885733216,-14.4984160062243,
118.589180184986)) ;
#191949=CARTESIAN_POINT('Ctrl Pts',(-8.6023326698515,-14.4984159668254,
118.564949049182)) ;
#191950=CARTESIAN_POINT('Ctrl Pts',(-8.61125485980821,-14.4281001590278,
118.59212459814)) ;
#191951=CARTESIAN_POINT('Ctrl Pts',(-8.68881511671028,-14.4990916302809,
118.863813337563)) ;
#191952=CARTESIAN_POINT('Ctrl Pts',(-8.69160201611696,-14.4237145145617,
118.872301781483)) ;
#191953=CARTESIAN_POINT('Ctrl Pts',(-8.61779820492839,-14.4237145258999,
118.89653292134)) ;
#191954=CARTESIAN_POINT('Ctrl Pts',(-8.5439943937398,-14.4237145372381,
118.920764061198)) ;
#191955=CARTESIAN_POINT('Ctrl Pts',(-8.54120749433315,-14.4990916529572,
118.912275617278)) ;
#191956=CARTESIAN_POINT('Ctrl Pts',(-8.53842059492649,-14.5744687686764,
118.903787173358)) ;
#191957=CARTESIAN_POINT('Ctrl Pts',(-8.61222440611505,-14.5744687573382,
118.879556033501)) ;
#191958=CARTESIAN_POINT('Ctrl Pts',(-8.68602821730362,-14.574468746,118.855324893643)) ;
#191959=CARTESIAN_POINT('Ctrl Pts',(-8.68881511671028,-14.4990916302809,
118.863813337563)) ;
#191960=CARTESIAN_POINT('Ctrl Pts',(-8.76912430296958,-14.4927693074735,
119.143894083316)) ;
#191961=CARTESIAN_POINT('Ctrl Pts',(-8.76557443984321,-14.4177207882231,
119.133081771065)) ;
#191962=CARTESIAN_POINT('Ctrl Pts',(-8.69177062728724,-14.4177207722467,
119.157312906758)) ;
#191963=CARTESIAN_POINT('Ctrl Pts',(-8.61796681473128,-14.4177207562703,
119.18154404245)) ;
#191964=CARTESIAN_POINT('Ctrl Pts',(-8.62151667785764,-14.4927692755206,
119.192356354701)) ;
#191965=CARTESIAN_POINT('Ctrl Pts',(-8.62506654098401,-14.567817794771,
119.203168666952)) ;
#191966=CARTESIAN_POINT('Ctrl Pts',(-8.69887035353998,-14.5678178107474,
119.17893753126)) ;
#191967=CARTESIAN_POINT('Ctrl Pts',(-8.77267416609596,-14.5678178267238,
119.154706395567)) ;
#191968=CARTESIAN_POINT('Ctrl Pts',(-8.76912430296958,-14.4927693074735,
119.143894083316)) ;
#191969=CARTESIAN_POINT('Ctrl Pts',(-8.84564499663558,-14.4094376546516,
119.412427388764)) ;
#191970=CARTESIAN_POINT('Ctrl Pts',(-8.83601350712255,-14.3400945271198,
119.383091423897)) ;
#191971=CARTESIAN_POINT('Ctrl Pts',(-8.76220969078333,-14.3400944873417,
119.407322548066)) ;
#191972=CARTESIAN_POINT('Ctrl Pts',(-8.68840587444411,-14.3400944475637,
119.431553672236)) ;
#191973=CARTESIAN_POINT('Ctrl Pts',(-8.69803736395715,-14.4094375750955,
119.460889637102)) ;
#191974=CARTESIAN_POINT('Ctrl Pts',(-8.70766885347021,-14.4787807026274,
119.490225601969)) ;
#191975=CARTESIAN_POINT('Ctrl Pts',(-8.78147266980941,-14.4787807424054,
119.4659944778)) ;
#191976=CARTESIAN_POINT('Ctrl Pts',(-8.85527648614863,-14.4787807821835,
119.44176335363)) ;
#191977=CARTESIAN_POINT('Ctrl Pts',(-8.84564499663558,-14.4094376546516,
119.412427388764)) ;
#191978=CARTESIAN_POINT('Ctrl Pts',(-8.91218973923486,-14.2549673486149,
119.650598079917)) ;
#191979=CARTESIAN_POINT('Ctrl Pts',(-8.89716344705603,-14.1963046294673,
119.604830416691)) ;
#191980=CARTESIAN_POINT('Ctrl Pts',(-8.82335962503793,-14.1963045717546,
119.629061523563)) ;
#191981=CARTESIAN_POINT('Ctrl Pts',(-8.74955580301983,-14.1963045140418,
119.653292630436)) ;
#191982=CARTESIAN_POINT('Ctrl Pts',(-8.76458209519867,-14.2549672331893,
119.699060293662)) ;
#191983=CARTESIAN_POINT('Ctrl Pts',(-8.77960838737749,-14.3136299523368,
119.744827956887)) ;
#191984=CARTESIAN_POINT('Ctrl Pts',(-8.85341220939561,-14.3136300100496,
119.720596850015)) ;
#191985=CARTESIAN_POINT('Ctrl Pts',(-8.9272160314137,-14.3136300677624,
119.696365743142)) ;
#191986=CARTESIAN_POINT('Ctrl Pts',(-8.91218973923486,-14.2549673486149,
119.650598079917)) ;
#191987=CARTESIAN_POINT('Ctrl Pts',(-8.96309326723311,-14.0408502140836,
119.841068283191)) ;
#191988=CARTESIAN_POINT('Ctrl Pts',(-8.94375726638346,-13.9970485144641,
119.782173942844)) ;
#191989=CARTESIAN_POINT('Ctrl Pts',(-8.86995343771673,-13.9970484457834,
119.806405029466)) ;
#191990=CARTESIAN_POINT('Ctrl Pts',(-8.79614960904997,-13.9970483771027,
119.830636116088)) ;
#191991=CARTESIAN_POINT('Ctrl Pts',(-8.81548560989961,-14.0408500767222,
119.889530456434)) ;
#191992=CARTESIAN_POINT('Ctrl Pts',(-8.83482161074924,-14.0846517763417,
119.948424796781)) ;
#191993=CARTESIAN_POINT('Ctrl Pts',(-8.908625439416,-14.0846518450224,119.92419371016)) ;
#191994=CARTESIAN_POINT('Ctrl Pts',(-8.98242926808274,-14.0846519137031,
119.899962623538)) ;
#191995=CARTESIAN_POINT('Ctrl Pts',(-8.96309326723311,-14.0408502140836,
119.841068283191)) ;
#191996=CARTESIAN_POINT('Ctrl Pts',(-8.99415259582093,-13.7824650273217,
119.971073817574)) ;
#191997=CARTESIAN_POINT('Ctrl Pts',(-8.97188631073203,-13.7566374523408,
119.903254304363)) ;
#191998=CARTESIAN_POINT('Ctrl Pts',(-8.89808247511074,-13.7566373798381,
119.927485369803)) ;
#191999=CARTESIAN_POINT('Ctrl Pts',(-8.82427863948944,-13.7566373073354,
119.951716435242)) ;
#192000=CARTESIAN_POINT('Ctrl Pts',(-8.84654492457835,-13.7824648823164,
120.019535948453)) ;
#192001=CARTESIAN_POINT('Ctrl Pts',(-8.86881120966723,-13.8082924572973,
120.087355461664)) ;
#192002=CARTESIAN_POINT('Ctrl Pts',(-8.94261504528854,-13.8082925298,120.063124396225)) ;
#192003=CARTESIAN_POINT('Ctrl Pts',(-9.01641888090982,-13.8082926023027,
120.038893330785)) ;
#192004=CARTESIAN_POINT('Ctrl Pts',(-8.99415259582093,-13.7824650273217,
119.971073817574)) ;
#192005=CARTESIAN_POINT('Ctrl Pts',(-9.0023120554926,-13.4963851494492,
120.031528435387)) ;
#192006=CARTESIAN_POINT('Ctrl Pts',(-8.97870554701302,-13.4904923432814,
119.959626818148)) ;
#192007=CARTESIAN_POINT('Ctrl Pts',(-8.90490170488797,-13.4904922758106,
119.983857863778)) ;
#192008=CARTESIAN_POINT('Ctrl Pts',(-8.83109786276295,-13.4904922083398,
120.008088909408)) ;
#192009=CARTESIAN_POINT('Ctrl Pts',(-8.85470437124252,-13.4963850145077,
120.079990526647)) ;
#192010=CARTESIAN_POINT('Ctrl Pts',(-8.87831087972213,-13.5022778206756,
120.151892143886)) ;
#192011=CARTESIAN_POINT('Ctrl Pts',(-8.95211472184715,-13.5022778881464,
120.127661098256)) ;
#192012=CARTESIAN_POINT('Ctrl Pts',(-9.02591856397219,-13.5022779556171,
120.103430052626)) ;
#192013=CARTESIAN_POINT('Ctrl Pts',(-9.0023120554926,-13.4963851494492,
120.031528435387)) ;
#192014=CARTESIAN_POINT('Ctrl Pts',(-8.98624034471568,-13.2068554623175,
120.017906636824)) ;
#192015=CARTESIAN_POINT('Ctrl Pts',(-8.96298924945921,-13.2211688965324,
119.947087551054)) ;
#192016=CARTESIAN_POINT('Ctrl Pts',(-8.88918540217969,-13.2211688373046,
119.971318580984)) ;
#192017=CARTESIAN_POINT('Ctrl Pts',(-8.81538155490015,-13.2211687780768,
119.995549610914)) ;
#192018=CARTESIAN_POINT('Ctrl Pts',(-8.83863265015661,-13.2068553438618,
120.066368696685)) ;
#192019=CARTESIAN_POINT('Ctrl Pts',(-8.86188374541307,-13.1925419096468,
120.137187782455)) ;
#192020=CARTESIAN_POINT('Ctrl Pts',(-8.93568759269262,-13.1925419688746,
120.112956752525)) ;
#192021=CARTESIAN_POINT('Ctrl Pts',(-9.00949143997215,-13.1925420281025,
120.088725722595)) ;
#192022=CARTESIAN_POINT('Ctrl Pts',(-8.98624034471568,-13.2068554623175,
120.017906636824)) ;
#192023=CARTESIAN_POINT('Ctrl Pts',(-8.946364301955,-12.9311896303103,119.931928817403)) ;
#192024=CARTESIAN_POINT('Ctrl Pts',(-8.9251279617825,-12.9647719930566,
119.867246350707)) ;
#192025=CARTESIAN_POINT('Ctrl Pts',(-8.85132411089623,-12.9647719471212,
119.891477369652)) ;
#192026=CARTESIAN_POINT('Ctrl Pts',(-8.77752026000998,-12.9647719011858,
119.915708388597)) ;
#192027=CARTESIAN_POINT('Ctrl Pts',(-8.79875660018247,-12.9311895384395,
119.980390855293)) ;
#192028=CARTESIAN_POINT('Ctrl Pts',(-8.81999294035498,-12.8976071756931,
120.045073321988)) ;
#192029=CARTESIAN_POINT('Ctrl Pts',(-8.89379679124124,-12.8976072216285,
120.020842303044)) ;
#192030=CARTESIAN_POINT('Ctrl Pts',(-8.9676006421275,-12.8976072675639,
119.996611284099)) ;
#192031=CARTESIAN_POINT('Ctrl Pts',(-8.946364301955,-12.9311896303103,119.931928817403)) ;
#192032=CARTESIAN_POINT('Ctrl Pts',(-8.88452827451557,-12.6901579122719,
119.779127065873)) ;
#192033=CARTESIAN_POINT('Ctrl Pts',(-8.86684171688226,-12.7406206917642,
119.72525666422)) ;
#192034=CARTESIAN_POINT('Ctrl Pts',(-8.79303786446268,-12.7406206607923,
119.749487678494)) ;
#192035=CARTESIAN_POINT('Ctrl Pts',(-8.71923401204311,-12.7406206298204,
119.773718692769)) ;
#192036=CARTESIAN_POINT('Ctrl Pts',(-8.73692056967643,-12.6901578503282,
119.827589094422)) ;
#192037=CARTESIAN_POINT('Ctrl Pts',(-8.75460712730975,-12.639695070836,
119.881459496076)) ;
#192038=CARTESIAN_POINT('Ctrl Pts',(-8.82841097972933,-12.6396951018078,
119.857228481802)) ;
#192039=CARTESIAN_POINT('Ctrl Pts',(-8.9022148321489,-12.6396951327797,
119.832997467527)) ;
#192040=CARTESIAN_POINT('Ctrl Pts',(-8.88452827451557,-12.6901579122719,
119.779127065873)) ;
#192041=CARTESIAN_POINT('Ctrl Pts',(-8.80498155763684,-12.5020099307821,
119.572221904851)) ;
#192042=CARTESIAN_POINT('Ctrl Pts',(-8.79209020285993,-12.5656860202673,
119.532956917547)) ;
#192043=CARTESIAN_POINT('Ctrl Pts',(-8.71828635025744,-12.565686002392,
119.557187931264)) ;
#192044=CARTESIAN_POINT('Ctrl Pts',(-8.64448249765493,-12.5656859845167,
119.581418944981)) ;
#192045=CARTESIAN_POINT('Ctrl Pts',(-8.65737385243184,-12.5020098950315,
119.620683932286)) ;
#192046=CARTESIAN_POINT('Ctrl Pts',(-8.67026520720871,-12.4383338055463,
119.65994891959)) ;
#192047=CARTESIAN_POINT('Ctrl Pts',(-8.74406905981123,-12.4383338234216,
119.635717905873)) ;
#192048=CARTESIAN_POINT('Ctrl Pts',(-8.81787291241371,-12.4383338412968,
119.611486892155)) ;
#192049=CARTESIAN_POINT('Ctrl Pts',(-8.80498155763684,-12.5020099307821,
119.572221904851)) ;
#192050=CARTESIAN_POINT('Ctrl Pts',(-8.7115619119402,-12.3786471033838,
119.32335220504)) ;
#192051=CARTESIAN_POINT('Ctrl Pts',(-8.70443569741749,-12.451033969766,
119.301646904946)) ;
#192052=CARTESIAN_POINT('Ctrl Pts',(-8.630631846706,-12.4510339632927,119.325877924423)) ;
#192053=CARTESIAN_POINT('Ctrl Pts',(-8.55682799599452,-12.4510339568193,
119.3501089439)) ;
#192054=CARTESIAN_POINT('Ctrl Pts',(-8.56395421051721,-12.378647090437,
119.371814243995)) ;
#192055=CARTESIAN_POINT('Ctrl Pts',(-8.57108042503996,-12.3062602240548,
119.393519544089)) ;
#192056=CARTESIAN_POINT('Ctrl Pts',(-8.64488427575143,-12.3062602305281,
119.369288524612)) ;
#192057=CARTESIAN_POINT('Ctrl Pts',(-8.71868812646292,-12.3062602370015,
119.345057505135)) ;
#192058=CARTESIAN_POINT('Ctrl Pts',(-8.7115619119402,-12.3786471033838,
119.32335220504)) ;
#192059=CARTESIAN_POINT('Ctrl Pts',(-8.61202742108512,-12.3306796608346,
119.055450282701)) ;
#192060=CARTESIAN_POINT('Ctrl Pts',(-8.61111059814198,-12.4065247391554,
119.052657787592)) ;
#192061=CARTESIAN_POINT('Ctrl Pts',(-8.53730674903535,-12.4065247391449,
119.076888811957)) ;
#192062=CARTESIAN_POINT('Ctrl Pts',(-8.46350289992872,-12.4065247391344,
119.101119836322)) ;
#192063=CARTESIAN_POINT('Ctrl Pts',(-8.46441972287187,-12.3306796608136,
119.103912331432)) ;
#192064=CARTESIAN_POINT('Ctrl Pts',(-8.46533654581499,-12.2548345824928,
119.106704826541)) ;
#192065=CARTESIAN_POINT('Ctrl Pts',(-8.53914039492163,-12.2548345825033,
119.082473802176)) ;
#192066=CARTESIAN_POINT('Ctrl Pts',(-8.61294424402827,-12.2548345825139,
119.05824277781)) ;
#192067=CARTESIAN_POINT('Ctrl Pts',(-8.61202742108512,-12.3306796608346,
119.055450282701)) ;
#192068=CARTESIAN_POINT('Ctrl Pts',(-8.51084890152702,-12.360155377245,
118.782851948086)) ;
#192069=CARTESIAN_POINT('Ctrl Pts',(-8.51625934876444,-12.4340571826112,
118.799331297198)) ;
#192070=CARTESIAN_POINT('Ctrl Pts',(-8.44245550224552,-12.4340571856698,
118.823562329445)) ;
#192071=CARTESIAN_POINT('Ctrl Pts',(-8.36865165572661,-12.4340571887285,
118.847793361692)) ;
#192072=CARTESIAN_POINT('Ctrl Pts',(-8.36324120848917,-12.3601553833623,
118.83131401258)) ;
#192073=CARTESIAN_POINT('Ctrl Pts',(-8.35783076125176,-12.2862535779961,
118.814834663468)) ;
#192074=CARTESIAN_POINT('Ctrl Pts',(-8.43163460777068,-12.2862535749374,
118.790603631221)) ;
#192075=CARTESIAN_POINT('Ctrl Pts',(-8.5054384542896,-12.2862535718788,
118.766372598974)) ;
#192076=CARTESIAN_POINT('Ctrl Pts',(-8.51084890152702,-12.360155377245,
118.782851948086)) ;
#192077=CARTESIAN_POINT('Ctrl Pts',(-8.41582654585043,-12.4653999327267,
118.52883086794)) ;
#192078=CARTESIAN_POINT('Ctrl Pts',(-8.42714754368904,-12.5320640126139,
118.563312800623)) ;
#192079=CARTESIAN_POINT('Ctrl Pts',(-8.35334369898756,-12.5320640153815,
118.587543838406)) ;
#192080=CARTESIAN_POINT('Ctrl Pts',(-8.27953985428609,-12.5320640181491,
118.611774876189)) ;
#192081=CARTESIAN_POINT('Ctrl Pts',(-8.26821885644749,-12.4653999382619,
118.577292943505)) ;
#192082=CARTESIAN_POINT('Ctrl Pts',(-8.25689785860889,-12.3987358583746,
118.542811010821)) ;
#192083=CARTESIAN_POINT('Ctrl Pts',(-8.33070170331036,-12.398735855607,
118.518579973038)) ;
#192084=CARTESIAN_POINT('Ctrl Pts',(-8.40450554801183,-12.3987358528394,
118.494348935256)) ;
#192085=CARTESIAN_POINT('Ctrl Pts',(-8.41582654585043,-12.4653999327267,
118.52883086794)) ;
#192086=CARTESIAN_POINT('Ctrl Pts',(-8.33239181332137,-12.6388027493961,
118.310157345988)) ;
#192087=CARTESIAN_POINT('Ctrl Pts',(-8.34882205720498,-12.6934585985942,
118.360201217838)) ;
#192088=CARTESIAN_POINT('Ctrl Pts',(-8.2750182137703,-12.6934585991624,
118.38443225948)) ;
#192089=CARTESIAN_POINT('Ctrl Pts',(-8.20121437033563,-12.6934585997305,
118.408663301121)) ;
#192090=CARTESIAN_POINT('Ctrl Pts',(-8.18478412645201,-12.6388027505324,
118.35861942927)) ;
#192091=CARTESIAN_POINT('Ctrl Pts',(-8.1683538825684,-12.5841469013344,
118.308575557419)) ;
#192092=CARTESIAN_POINT('Ctrl Pts',(-8.24215772600308,-12.5841469007662,
118.284344515778)) ;
#192093=CARTESIAN_POINT('Ctrl Pts',(-8.31596156943775,-12.584146900198,
118.260113474137)) ;
#192094=CARTESIAN_POINT('Ctrl Pts',(-8.33239181332137,-12.6388027493961,
118.310157345988)) ;
#192095=CARTESIAN_POINT('Ctrl Pts',(-8.26591621181812,-12.8679196576227,
118.143124187206)) ;
#192096=CARTESIAN_POINT('Ctrl Pts',(-8.28627939353487,-12.9066583901742,
118.205147153176)) ;
#192097=CARTESIAN_POINT('Ctrl Pts',(-8.21247555056549,-12.9066583881138,
118.229378196234)) ;
#192098=CARTESIAN_POINT('Ctrl Pts',(-8.13867170759611,-12.9066583860534,
118.253609239292)) ;
#192099=CARTESIAN_POINT('Ctrl Pts',(-8.11830852587934,-12.8679196535019,
118.191586273322)) ;
#192100=CARTESIAN_POINT('Ctrl Pts',(-8.09794534416259,-12.8291809209503,
118.129563307352)) ;
#192101=CARTESIAN_POINT('Ctrl Pts',(-8.17174918713197,-12.8291809230107,
118.105332264294)) ;
#192102=CARTESIAN_POINT('Ctrl Pts',(-8.24555303010134,-12.8291809250711,
118.081101221236)) ;
#192103=CARTESIAN_POINT('Ctrl Pts',(-8.26591621181812,-12.8679196576227,
118.143124187206)) ;
#192104=CARTESIAN_POINT('Ctrl Pts',(-8.22030810185899,-13.1373001966588,
118.039762360663)) ;
#192105=CARTESIAN_POINT('Ctrl Pts',(-8.24315064156721,-13.1572855705815,
118.109337051049)) ;
#192106=CARTESIAN_POINT('Ctrl Pts',(-8.16934679842566,-13.1572855672865,
118.133568093583)) ;
#192107=CARTESIAN_POINT('Ctrl Pts',(-8.0955429552841,-13.1572855639915,
118.157799136117)) ;
#192108=CARTESIAN_POINT('Ctrl Pts',(-8.07270041557589,-13.1373001900688,
118.08822444573)) ;
#192109=CARTESIAN_POINT('Ctrl Pts',(-8.04985787586767,-13.1173148161461,
118.018649755344)) ;
#192110=CARTESIAN_POINT('Ctrl Pts',(-8.12366171900923,-13.1173148194411,
117.99441871281)) ;
#192111=CARTESIAN_POINT('Ctrl Pts',(-8.19746556215078,-13.1173148227361,
117.970187670276)) ;
#192112=CARTESIAN_POINT('Ctrl Pts',(-8.22030810185899,-13.1373001966588,
118.039762360663)) ;
#192113=CARTESIAN_POINT('Ctrl Pts',(-8.19835036718157,-13.4255234275119,
118.008268887877)) ;
#192114=CARTESIAN_POINT('Ctrl Pts',(-8.22202747304424,-13.425412168657,
118.080385532087)) ;
#192115=CARTESIAN_POINT('Ctrl Pts',(-8.14822362956311,-13.4254121666008,
118.104616573587)) ;
#192116=CARTESIAN_POINT('Ctrl Pts',(-8.07441978608198,-13.4254121645446,
118.128847615087)) ;
#192117=CARTESIAN_POINT('Ctrl Pts',(-8.05074268021931,-13.4255234233994,
118.056730970876)) ;
#192118=CARTESIAN_POINT('Ctrl Pts',(-8.02706557435661,-13.4256346822543,
117.984614326666)) ;
#192119=CARTESIAN_POINT('Ctrl Pts',(-8.10086941783775,-13.4256346843105,
117.960383285166)) ;
#192120=CARTESIAN_POINT('Ctrl Pts',(-8.17467326131888,-13.4256346863667,
117.936152243667)) ;
#192121=CARTESIAN_POINT('Ctrl Pts',(-8.19835036718157,-13.4255234275119,
118.008268887877)) ;
#192122=CARTESIAN_POINT('Ctrl Pts',(-8.20061003959541,-13.7140381962048,
118.050644598093)) ;
#192123=CARTESIAN_POINT('Ctrl Pts',(-8.22342961676016,-13.6937806023833,
118.120149348188)) ;
#192124=CARTESIAN_POINT('Ctrl Pts',(-8.14962577334613,-13.6937806037046,
118.144380389892)) ;
#192125=CARTESIAN_POINT('Ctrl Pts',(-8.07582192993207,-13.6937806050258,
118.168611431595)) ;
#192126=CARTESIAN_POINT('Ctrl Pts',(-8.05300235276731,-13.7140381988474,
118.099106681501)) ;
#192127=CARTESIAN_POINT('Ctrl Pts',(-8.03018277560256,-13.7342957926689,
118.029601931407)) ;
#192128=CARTESIAN_POINT('Ctrl Pts',(-8.10398661901661,-13.7342957913476,
118.005370889703)) ;
#192129=CARTESIAN_POINT('Ctrl Pts',(-8.17779046243066,-13.7342957900263,
117.981139847999)) ;
#192130=CARTESIAN_POINT('Ctrl Pts',(-8.20061003959541,-13.7140381962048,
118.050644598093)) ;
#192131=CARTESIAN_POINT('Ctrl Pts',(-8.2262886533452,-13.981013641758,118.164309383492)) ;
#192132=CARTESIAN_POINT('Ctrl Pts',(-8.2466148823236,-13.9420847851826,
118.226219797217)) ;
#192133=CARTESIAN_POINT('Ctrl Pts',(-8.17281103977456,-13.9420847906692,
118.250450841556)) ;
#192134=CARTESIAN_POINT('Ctrl Pts',(-8.09900719722553,-13.9420847961559,
118.274681885894)) ;
#192135=CARTESIAN_POINT('Ctrl Pts',(-8.07868096824714,-13.9810136527313,
118.21277147217)) ;
#192136=CARTESIAN_POINT('Ctrl Pts',(-8.05835473926874,-14.0199425093067,
118.150861058445)) ;
#192137=CARTESIAN_POINT('Ctrl Pts',(-8.13215858181778,-14.01994250382,118.126630014106)) ;
#192138=CARTESIAN_POINT('Ctrl Pts',(-8.2059624243668,-14.0199424983334,
118.102398969767)) ;
#192139=CARTESIAN_POINT('Ctrl Pts',(-8.2262886533452,-13.981013641758,118.164309383492)) ;
#192140=CARTESIAN_POINT('Ctrl Pts',(-8.27273205955447,-14.2077526521797,
118.341223296335)) ;
#192141=CARTESIAN_POINT('Ctrl Pts',(-8.28911130746513,-14.1529353062713,
118.391111842453)) ;
#192142=CARTESIAN_POINT('Ctrl Pts',(-8.21530746668232,-14.1529353151086,
118.415342892171)) ;
#192143=CARTESIAN_POINT('Ctrl Pts',(-8.14150362589951,-14.1529353239459,
118.43957394189)) ;
#192144=CARTESIAN_POINT('Ctrl Pts',(-8.12512437798886,-14.2077526698542,
118.389685395771)) ;
#192145=CARTESIAN_POINT('Ctrl Pts',(-8.10874513007819,-14.2625700157626,
118.339796849653)) ;
#192146=CARTESIAN_POINT('Ctrl Pts',(-8.182548970861,-14.2625700069253,118.315565799935)) ;
#192147=CARTESIAN_POINT('Ctrl Pts',(-8.25635281164381,-14.2625699980881,
118.291334750216)) ;
#192148=CARTESIAN_POINT('Ctrl Pts',(-8.27273205955447,-14.2077526521797,
118.341223296335)) ;
#192149=CARTESIAN_POINT('Ctrl Pts',(-8.33605388433727,-14.3782190485839,
118.569622801418)) ;
#192150=CARTESIAN_POINT('Ctrl Pts',(-8.347300341461,-14.3114194784183,118.603877694822)) ;
#192151=CARTESIAN_POINT('Ctrl Pts',(-8.27349650343915,-14.3114194884178,
118.62810875295)) ;
#192152=CARTESIAN_POINT('Ctrl Pts',(-8.19969266541728,-14.3114194984174,
118.652339811078)) ;
#192153=CARTESIAN_POINT('Ctrl Pts',(-8.18844620829354,-14.378219068583,
118.618084917674)) ;
#192154=CARTESIAN_POINT('Ctrl Pts',(-8.1771997511698,-14.4450186387486,
118.583830024269)) ;
#192155=CARTESIAN_POINT('Ctrl Pts',(-8.25100358919167,-14.445018628749,
118.559598966142)) ;
#192156=CARTESIAN_POINT('Ctrl Pts',(-8.32480742721352,-14.4450186187495,
118.535367908014)) ;
#192157=CARTESIAN_POINT('Ctrl Pts',(-8.33605388433727,-14.3782190485839,
118.569622801418)) ;
#192158=CARTESIAN_POINT('Ctrl Pts',(-8.41067546930047,-14.4794481619843,
118.832358521227)) ;
#192159=CARTESIAN_POINT('Ctrl Pts',(-8.41599441965751,-14.4054839121495,
118.848559185268)) ;
#192160=CARTESIAN_POINT('Ctrl Pts',(-8.34219058465964,-14.4054839189219,
118.872790252606)) ;
#192161=CARTESIAN_POINT('Ctrl Pts',(-8.26838674966178,-14.4054839256943,
118.897021319945)) ;
#192162=CARTESIAN_POINT('Ctrl Pts',(-8.26306779930477,-14.4794481755291,
118.880820655904)) ;
#192163=CARTESIAN_POINT('Ctrl Pts',(-8.25774884894772,-14.5534124253639,
118.864619991863)) ;
#192164=CARTESIAN_POINT('Ctrl Pts',(-8.33155268394558,-14.5534124185915,
118.840388924525)) ;
#192165=CARTESIAN_POINT('Ctrl Pts',(-8.40535651894344,-14.5534124118191,
118.816157857186)) ;
#192166=CARTESIAN_POINT('Ctrl Pts',(-8.41067546930047,-14.4794481619843,
118.832358521227)) ;
#192167=CARTESIAN_POINT('Ctrl Pts',(-8.49060294650496,-14.5047934992133,
119.111248928823)) ;
#192168=CARTESIAN_POINT('Ctrl Pts',(-8.48961555716104,-14.4289527181918,
119.1082414995)) ;
#192169=CARTESIAN_POINT('Ctrl Pts',(-8.41581172498398,-14.4289527172552,
119.13247257543)) ;
#192170=CARTESIAN_POINT('Ctrl Pts',(-8.34200789280688,-14.4289527163185,
119.15670365136)) ;
#192171=CARTESIAN_POINT('Ctrl Pts',(-8.34299528215081,-14.5047934973399,
119.159711080683)) ;
#192172=CARTESIAN_POINT('Ctrl Pts',(-8.34398267149472,-14.5806342783613,
119.162718510006)) ;
#192173=CARTESIAN_POINT('Ctrl Pts',(-8.41778650367179,-14.580634279298,
119.138487434076)) ;
#192174=CARTESIAN_POINT('Ctrl Pts',(-8.49159033584886,-14.5806342802347,
119.114256358146)) ;
#192175=CARTESIAN_POINT('Ctrl Pts',(-8.49060294650496,-14.5047934992133,
119.111248928823)) ;
#192176=CARTESIAN_POINT('Ctrl Pts',(-8.56952664834317,-14.4522183736054,
119.387142880941)) ;
#192177=CARTESIAN_POINT('Ctrl Pts',(-8.56229269511265,-14.3799386549208,
119.365109425723)) ;
#192178=CARTESIAN_POINT('Ctrl Pts',(-8.48848886515389,-14.3799386416776,
119.38934050841)) ;
#192179=CARTESIAN_POINT('Ctrl Pts',(-8.41468503519511,-14.3799386284344,
119.413571591096)) ;
#192180=CARTESIAN_POINT('Ctrl Pts',(-8.42191898842563,-14.452218347119,
119.435605046314)) ;
#192181=CARTESIAN_POINT('Ctrl Pts',(-8.42915294165614,-14.5244980658035,
119.457638501531)) ;
#192182=CARTESIAN_POINT('Ctrl Pts',(-8.50295677161491,-14.5244980790467,
119.433407418845)) ;
#192183=CARTESIAN_POINT('Ctrl Pts',(-8.57676060157369,-14.5244980922899,
119.409176336158)) ;
#192184=CARTESIAN_POINT('Ctrl Pts',(-8.56952664834317,-14.4522183736054,
119.387142880941)) ;
#192185=CARTESIAN_POINT('Ctrl Pts',(-8.64082192792583,-14.3254100791536,
119.639777714158)) ;
#192186=CARTESIAN_POINT('Ctrl Pts',(-8.62786556152258,-14.2618795112896,
119.600314711553)) ;
#192187=CARTESIAN_POINT('Ctrl Pts',(-8.5540617322727,-14.2618794820993,
119.624545796399)) ;
#192188=CARTESIAN_POINT('Ctrl Pts',(-8.48025790302279,-14.261879452909,
119.648776881244)) ;
#192189=CARTESIAN_POINT('Ctrl Pts',(-8.49321426942607,-14.325410020773,
119.68823988385)) ;
#192190=CARTESIAN_POINT('Ctrl Pts',(-8.50617063582931,-14.3889405886369,
119.727702886455)) ;
#192191=CARTESIAN_POINT('Ctrl Pts',(-8.57997446507921,-14.3889406178272,
119.703471801609)) ;
#192192=CARTESIAN_POINT('Ctrl Pts',(-8.6537782943291,-14.3889406470175,
119.679240716764)) ;
#192193=CARTESIAN_POINT('Ctrl Pts',(-8.64082192792583,-14.3254100791536,
119.639777714158)) ;
#192194=CARTESIAN_POINT('Ctrl Pts',(-8.69855299299028,-14.1342773327245,
119.850992494174)) ;
#192195=CARTESIAN_POINT('Ctrl Pts',(-8.68081527062798,-14.0839997344191,
119.796966252638)) ;
#192196=CARTESIAN_POINT('Ctrl Pts',(-8.60701144003505,-14.0839996884698,
119.821197333393)) ;
#192197=CARTESIAN_POINT('Ctrl Pts',(-8.53320760944215,-14.0839996425206,
119.845428414148)) ;
#192198=CARTESIAN_POINT('Ctrl Pts',(-8.55094533180445,-14.134277240826,
119.899454655684)) ;
#192199=CARTESIAN_POINT('Ctrl Pts',(-8.56868305416677,-14.1845548391315,
119.95348089722)) ;
#192200=CARTESIAN_POINT('Ctrl Pts',(-8.64248688475969,-14.1845548850807,
119.929249816465)) ;
#192201=CARTESIAN_POINT('Ctrl Pts',(-8.7162907153526,-14.18455493103,119.90501873571)) ;
#192202=CARTESIAN_POINT('Ctrl Pts',(-8.69855299299028,-14.1342773327245,
119.850992494174)) ;
#192203=CARTESIAN_POINT('Ctrl Pts',(-8.73823026219567,-13.8911855385649,
120.007348076147)) ;
#192204=CARTESIAN_POINT('Ctrl Pts',(-8.71696200923995,-13.8578071985554,
119.942568407905)) ;
#192205=CARTESIAN_POINT('Ctrl Pts',(-8.64315817558926,-13.8578071355948,
119.966799479347)) ;
#192206=CARTESIAN_POINT('Ctrl Pts',(-8.56935434193856,-13.8578070726341,
119.991030550788)) ;
#192207=CARTESIAN_POINT('Ctrl Pts',(-8.59062259489427,-13.8911854126436,
120.05581021903)) ;
#192208=CARTESIAN_POINT('Ctrl Pts',(-8.61189084784997,-13.9245637526531,
120.120589887271)) ;
#192209=CARTESIAN_POINT('Ctrl Pts',(-8.68569468150069,-13.9245638156137,
120.09635881583)) ;
#192210=CARTESIAN_POINT('Ctrl Pts',(-8.75949851515137,-13.9245638785744,
120.072127744389)) ;
#192211=CARTESIAN_POINT('Ctrl Pts',(-8.73823026219567,-13.8911855385649,
120.007348076147)) ;
#192212=CARTESIAN_POINT('Ctrl Pts',(-8.75589442615831,-13.6134122049751,
120.096730914448)) ;
#192213=CARTESIAN_POINT('Ctrl Pts',(-8.73262575513511,-13.5993787020081,
120.025858295372)) ;
#192214=CARTESIAN_POINT('Ctrl Pts',(-8.65882191632523,-13.5993786244693,
120.050089351099)) ;
#192215=CARTESIAN_POINT('Ctrl Pts',(-8.58501807751536,-13.5993785469305,
120.074320406827)) ;
#192216=CARTESIAN_POINT('Ctrl Pts',(-8.60828674853857,-13.6134120498975,
120.145193025903)) ;
#192217=CARTESIAN_POINT('Ctrl Pts',(-8.63155541956179,-13.6274455528644,
120.216065644979)) ;
#192218=CARTESIAN_POINT('Ctrl Pts',(-8.70535925837165,-13.6274456304033,
120.191834589251)) ;
#192219=CARTESIAN_POINT('Ctrl Pts',(-8.77916309718153,-13.6274457079421,
120.167603533524)) ;
#192220=CARTESIAN_POINT('Ctrl Pts',(-8.75589442615831,-13.6134122049751,
120.096730914448)) ;
#192221=CARTESIAN_POINT('Ctrl Pts',(-8.74967783452186,-13.3239481087795,
120.113088049486)) ;
#192222=CARTESIAN_POINT('Ctrl Pts',(-8.72607932381083,-13.3301038926875,
120.041210791831)) ;
#192223=CARTESIAN_POINT('Ctrl Pts',(-8.65227547827315,-13.3301038083537,
120.065441827067)) ;
#192224=CARTESIAN_POINT('Ctrl Pts',(-8.57847163273545,-13.3301037240199,
120.089672862302)) ;
#192225=CARTESIAN_POINT('Ctrl Pts',(-8.60207014344647,-13.3239479401119,
120.161550119957)) ;
#192226=CARTESIAN_POINT('Ctrl Pts',(-8.62566865415748,-13.3177921562039,
120.233427377612)) ;
#192227=CARTESIAN_POINT('Ctrl Pts',(-8.69947249969519,-13.3177922405377,
120.209196342377)) ;
#192228=CARTESIAN_POINT('Ctrl Pts',(-8.77327634523286,-13.3177923248715,
120.184965307141)) ;
#192229=CARTESIAN_POINT('Ctrl Pts',(-8.74967783452186,-13.3239481087795,
120.113088049486)) ;
#192230=CARTESIAN_POINT('Ctrl Pts',(-8.71923606193324,-13.0394391601657,
120.05588628759)) ;
#192231=CARTESIAN_POINT('Ctrl Pts',(-8.69699356662627,-13.0654672913968,
119.988139233932)) ;
#192232=CARTESIAN_POINT('Ctrl Pts',(-8.62318971345324,-13.0654672055952,
120.012370245912)) ;
#192233=CARTESIAN_POINT('Ctrl Pts',(-8.54938586028022,-13.0654671197937,
120.036601257892)) ;
#192234=CARTESIAN_POINT('Ctrl Pts',(-8.57162835558722,-13.0394389885626,
120.104348311549)) ;
#192235=CARTESIAN_POINT('Ctrl Pts',(-8.59387085089422,-13.0134108573315,
120.172095365206)) ;
#192236=CARTESIAN_POINT('Ctrl Pts',(-8.66767470406722,-13.0134109431331,
120.147864353226)) ;
#192237=CARTESIAN_POINT('Ctrl Pts',(-8.74147855724025,-13.0134110289346,
120.123633341247)) ;
#192238=CARTESIAN_POINT('Ctrl Pts',(-8.71923606193324,-13.0394391601657,
120.05588628759)) ;
#192239=CARTESIAN_POINT('Ctrl Pts',(-8.66606319630121,-12.7825526473998,
119.929370423015)) ;
#192240=CARTESIAN_POINT('Ctrl Pts',(-8.64676730794358,-12.8265535642734,
119.870598258589)) ;
#192241=CARTESIAN_POINT('Ctrl Pts',(-8.57296344702554,-12.8265534855134,
119.894829246979)) ;
#192242=CARTESIAN_POINT('Ctrl Pts',(-8.49915958610749,-12.8265534067534,
119.919060235368)) ;
#192243=CARTESIAN_POINT('Ctrl Pts',(-8.5184554744651,-12.7825524898798,
119.977832399794)) ;
#192244=CARTESIAN_POINT('Ctrl Pts',(-8.53775136282272,-12.7385515730062,
120.03660456422)) ;
#192245=CARTESIAN_POINT('Ctrl Pts',(-8.61155522374078,-12.7385516517662,
120.012373575831)) ;
#192246=CARTESIAN_POINT('Ctrl Pts',(-8.68535908465883,-12.7385517305262,
119.988142587441)) ;
#192247=CARTESIAN_POINT('Ctrl Pts',(-8.66606319630121,-12.7825526473998,
119.929370423015)) ;
#192248=CARTESIAN_POINT('Ctrl Pts',(-8.59271043085412,-12.5702685769134,
119.741585147016)) ;
#192249=CARTESIAN_POINT('Ctrl Pts',(-8.57777001188604,-12.6291549421708,
119.696079039497)) ;
#192250=CARTESIAN_POINT('Ctrl Pts',(-8.50396614376988,-12.629154878069,
119.720310005963)) ;
#192251=CARTESIAN_POINT('Ctrl Pts',(-8.43016227565372,-12.6291548139673,
119.744540972428)) ;
#192252=CARTESIAN_POINT('Ctrl Pts',(-8.44510269462181,-12.57026844871,119.790047079946)) ;
#192253=CARTESIAN_POINT('Ctrl Pts',(-8.46004311358988,-12.5113820834526,
119.835553187465)) ;
#192254=CARTESIAN_POINT('Ctrl Pts',(-8.53384698170604,-12.5113821475544,
119.811322221)) ;
#192255=CARTESIAN_POINT('Ctrl Pts',(-8.6076508498222,-12.5113822116561,
119.787091254535)) ;
#192256=CARTESIAN_POINT('Ctrl Pts',(-8.59271043085412,-12.5702685769134,
119.741585147016)) ;
#192257=CARTESIAN_POINT('Ctrl Pts',(-8.50491328859232,-12.4204037087553,
119.509450907549)) ;
#192258=CARTESIAN_POINT('Ctrl Pts',(-8.4953507374057,-12.4898390976006,
119.480324917526)) ;
#192259=CARTESIAN_POINT('Ctrl Pts',(-8.42154686411292,-12.4898390557385,
119.504555868224)) ;
#192260=CARTESIAN_POINT('Ctrl Pts',(-8.34774299082012,-12.4898390138765,
119.528786818922)) ;
#192261=CARTESIAN_POINT('Ctrl Pts',(-8.35730554200674,-12.4204036250312,
119.557912808945)) ;
#192262=CARTESIAN_POINT('Ctrl Pts',(-8.36686809319335,-12.3509682361859,
119.587038798968)) ;
#192263=CARTESIAN_POINT('Ctrl Pts',(-8.44067196648614,-12.3509682780479,
119.56280784827)) ;
#192264=CARTESIAN_POINT('Ctrl Pts',(-8.51447583977895,-12.35096831991,119.538576897572)) ;
#192265=CARTESIAN_POINT('Ctrl Pts',(-8.50491328859232,-12.4204037087553,
119.509450907549)) ;
#192266=CARTESIAN_POINT('Ctrl Pts',(-8.40683399712527,-12.3408608148814,
119.246251031593)) ;
#192267=CARTESIAN_POINT('Ctrl Pts',(-8.4033695857143,-12.4159518832881,
119.235698991346)) ;
#192268=CARTESIAN_POINT('Ctrl Pts',(-8.32956570922843,-12.4159518680668,
119.259929932318)) ;
#192269=CARTESIAN_POINT('Ctrl Pts',(-8.25576183274256,-12.4159518528455,
119.28416087329)) ;
#192270=CARTESIAN_POINT('Ctrl Pts',(-8.25922624415353,-12.3408607844389,
119.294712913538)) ;
#192271=CARTESIAN_POINT('Ctrl Pts',(-8.2626906555645,-12.2657697160322,
119.305264953785)) ;
#192272=CARTESIAN_POINT('Ctrl Pts',(-8.33649453205038,-12.2657697312535,
119.281034012813)) ;
#192273=CARTESIAN_POINT('Ctrl Pts',(-8.41029840853624,-12.2657697464747,
119.256803071841)) ;
#192274=CARTESIAN_POINT('Ctrl Pts',(-8.40683399712527,-12.3408608148814,
119.246251031593)) ;
#192275=CARTESIAN_POINT('Ctrl Pts',(-8.30571590982397,-12.3387915853932,
118.973648699883)) ;
#192276=CARTESIAN_POINT('Ctrl Pts',(-8.30857389731344,-12.414137720195,
118.98235366655)) ;
#192277=CARTESIAN_POINT('Ctrl Pts',(-8.23477002042433,-12.4141377338266,
119.006584606295)) ;
#192278=CARTESIAN_POINT('Ctrl Pts',(-8.16096614353523,-12.4141377474583,
119.030815546039)) ;
#192279=CARTESIAN_POINT('Ctrl Pts',(-8.15810815604576,-12.3387916126566,
119.022110579371)) ;
#192280=CARTESIAN_POINT('Ctrl Pts',(-8.15525016855628,-12.2634454778548,
119.013405612704)) ;
#192281=CARTESIAN_POINT('Ctrl Pts',(-8.22905404544539,-12.2634454642232,
118.98917467296)) ;
#192282=CARTESIAN_POINT('Ctrl Pts',(-8.3028579223345,-12.2634454505915,
118.964943733216)) ;
#192283=CARTESIAN_POINT('Ctrl Pts',(-8.30571590982397,-12.3387915853932,
118.973648699883)) ;
#192284=CARTESIAN_POINT('Ctrl Pts',(-8.20736927607411,-12.4137122483728,
118.709584594176)) ;
#192285=CARTESIAN_POINT('Ctrl Pts',(-8.2163634416192,-12.4839393117036,
118.736979369127)) ;
#192286=CARTESIAN_POINT('Ctrl Pts',(-8.14255956699891,-12.4839393535464,
118.761210315782)) ;
#192287=CARTESIAN_POINT('Ctrl Pts',(-8.06875569237863,-12.4839393953892,
118.785441262436)) ;
#192288=CARTESIAN_POINT('Ctrl Pts',(-8.05976152683357,-12.4137123320584,
118.758046487485)) ;
#192289=CARTESIAN_POINT('Ctrl Pts',(-8.05076736128849,-12.3434852687276,
118.730651712534)) ;
#192290=CARTESIAN_POINT('Ctrl Pts',(-8.12457123590877,-12.3434852268848,
118.706420765879)) ;
#192291=CARTESIAN_POINT('Ctrl Pts',(-8.19837511052905,-12.343485185042,
118.682189819225)) ;
#192292=CARTESIAN_POINT('Ctrl Pts',(-8.20736927607411,-12.4137122483728,
118.709584594176)) ;
#192293=CARTESIAN_POINT('Ctrl Pts',(-8.11806988347709,-12.5618189977429,
118.473239800089)) ;
#192294=CARTESIAN_POINT('Ctrl Pts',(-8.13257443790471,-12.6218107314417,
118.517418330508)) ;
#192295=CARTESIAN_POINT('Ctrl Pts',(-8.05877056827575,-12.6218107975561,
118.541649292365)) ;
#192296=CARTESIAN_POINT('Ctrl Pts',(-7.98496669864682,-12.6218108636706,
118.565880254222)) ;
#192297=CARTESIAN_POINT('Ctrl Pts',(-7.97046214421921,-12.5618191299718,
118.521701723804)) ;
#192298=CARTESIAN_POINT('Ctrl Pts',(-7.95595758979159,-12.501827396273,
118.477523193385)) ;
#192299=CARTESIAN_POINT('Ctrl Pts',(-8.02976145942054,-12.5018273301586,
118.453292231528)) ;
#192300=CARTESIAN_POINT('Ctrl Pts',(-8.10356532904949,-12.5018272640442,
118.42906126967)) ;
#192301=CARTESIAN_POINT('Ctrl Pts',(-8.11806988347709,-12.5618189977429,
118.473239800089)) ;
#192302=CARTESIAN_POINT('Ctrl Pts',(-8.04465640581912,-12.7689119270669,
118.284855280658)) ;
#192303=CARTESIAN_POINT('Ctrl Pts',(-8.06357919075944,-12.814533735282,
118.34249102837)) ;
#192304=CARTESIAN_POINT('Ctrl Pts',(-7.98977532782009,-12.8145338199658,
118.366722010603)) ;
#192305=CARTESIAN_POINT('Ctrl Pts',(-7.91597146488071,-12.8145339046497,
118.390952992836)) ;
#192306=CARTESIAN_POINT('Ctrl Pts',(-7.8970486799404,-12.7689120964346,
118.333317245123)) ;
#192307=CARTESIAN_POINT('Ctrl Pts',(-7.87812589500005,-12.7232902882195,
118.275681497411)) ;
#192308=CARTESIAN_POINT('Ctrl Pts',(-7.95192975793942,-12.7232902035356,
118.251450515178)) ;
#192309=CARTESIAN_POINT('Ctrl Pts',(-8.02573362087878,-12.7232901188518,
118.227219532945)) ;
#192310=CARTESIAN_POINT('Ctrl Pts',(-8.04465640581912,-12.7689119270669,
118.284855280658)) ;
#192311=CARTESIAN_POINT('Ctrl Pts',(-7.98990681541494,-13.0251682484426,
118.1537612682)) ;
#192312=CARTESIAN_POINT('Ctrl Pts',(-8.01194249189055,-13.052967781727,
118.220878381343)) ;
#192313=CARTESIAN_POINT('Ctrl Pts',(-7.93813863719427,-13.0529678764172,
118.245109388683)) ;
#192314=CARTESIAN_POINT('Ctrl Pts',(-7.86433478249799,-13.0529679711075,
118.269340396023)) ;
#192315=CARTESIAN_POINT('Ctrl Pts',(-7.84229910602238,-13.025168437823,
118.20222328288)) ;
#192316=CARTESIAN_POINT('Ctrl Pts',(-7.82026342954678,-12.9973689045386,
118.135106169737)) ;
#192317=CARTESIAN_POINT('Ctrl Pts',(-7.89406728424306,-12.9973688098484,
118.110875162397)) ;
#192318=CARTESIAN_POINT('Ctrl Pts',(-7.96787113893935,-12.9973687151582,
118.086644155057)) ;
#192319=CARTESIAN_POINT('Ctrl Pts',(-7.98990681541494,-13.0251682484426,
118.1537612682)) ;
#192320=CARTESIAN_POINT('Ctrl Pts',(-7.95830518848991,-13.3082750938872,
118.092954291203)) ;
#192321=CARTESIAN_POINT('Ctrl Pts',(-7.98184680689377,-13.3163504016851,
118.164658260563)) ;
#192322=CARTESIAN_POINT('Ctrl Pts',(-7.90804296057227,-13.3163504980826,
118.188889293411)) ;
#192323=CARTESIAN_POINT('Ctrl Pts',(-7.83423911425076,-13.31635059448,118.213120326259)) ;
#192324=CARTESIAN_POINT('Ctrl Pts',(-7.81069749584691,-13.3082752866821,
118.141416356899)) ;
#192325=CARTESIAN_POINT('Ctrl Pts',(-7.78715587744302,-13.3001999788842,
118.069712387539)) ;
#192326=CARTESIAN_POINT('Ctrl Pts',(-7.86095972376454,-13.3001998824867,
118.045481354691)) ;
#192327=CARTESIAN_POINT('Ctrl Pts',(-7.93476357008601,-13.3001997860893,
118.021250321843)) ;
#192328=CARTESIAN_POINT('Ctrl Pts',(-7.95830518848991,-13.3082750938872,
118.092954291203)) ;
#192329=CARTESIAN_POINT('Ctrl Pts',(-7.95079241587088,-13.5983478962611,
118.105425292295)) ;
#192330=CARTESIAN_POINT('Ctrl Pts',(-7.97416229673392,-13.5861829357955,
118.176606176905)) ;
#192331=CARTESIAN_POINT('Ctrl Pts',(-7.90035845823514,-13.5861830266329,
118.20083723358)) ;
#192332=CARTESIAN_POINT('Ctrl Pts',(-7.82655461973636,-13.5861831174704,
118.225068290255)) ;
#192333=CARTESIAN_POINT('Ctrl Pts',(-7.80318473887331,-13.5983480779361,
118.153887405644)) ;
#192334=CARTESIAN_POINT('Ctrl Pts',(-7.77981485801028,-13.6105130384017,
118.082706521034)) ;
#192335=CARTESIAN_POINT('Ctrl Pts',(-7.85361869650906,-13.6105129475642,
118.058475464359)) ;
#192336=CARTESIAN_POINT('Ctrl Pts',(-7.92742253500785,-13.6105128567267,
118.034244407684)) ;
#192337=CARTESIAN_POINT('Ctrl Pts',(-7.95079241587088,-13.5983478962611,
118.105425292295)) ;
#192338=CARTESIAN_POINT('Ctrl Pts',(-7.96711105691976,-13.8761876349326,
118.190549865602)) ;
#192339=CARTESIAN_POINT('Ctrl Pts',(-7.98864383656382,-13.8446061027284,
118.256135236427)) ;
#192340=CARTESIAN_POINT('Ctrl Pts',(-7.91484000469734,-13.8446061808087,
118.280366313303)) ;
#192341=CARTESIAN_POINT('Ctrl Pts',(-7.84103617283086,-13.8446062588889,
118.304597390179)) ;
#192342=CARTESIAN_POINT('Ctrl Pts',(-7.81950339318683,-13.8761877910931,
118.239012019354)) ;
#192343=CARTESIAN_POINT('Ctrl Pts',(-7.79797061354276,-13.9077693232973,
118.173426648529)) ;
#192344=CARTESIAN_POINT('Ctrl Pts',(-7.87177444540925,-13.907769245217,
118.149195571653)) ;
#192345=CARTESIAN_POINT('Ctrl Pts',(-7.94557827727571,-13.9077691671368,
118.124964494777)) ;
#192346=CARTESIAN_POINT('Ctrl Pts',(-7.96711105691976,-13.8761876349326,
118.190549865602)) ;
#192347=CARTESIAN_POINT('Ctrl Pts',(-8.00577117627182,-14.1226645874526,
118.343946067148)) ;
#192348=CARTESIAN_POINT('Ctrl Pts',(-8.0238998963966,-14.0738264529784,
118.399163222083)) ;
#192349=CARTESIAN_POINT('Ctrl Pts',(-7.95009606892581,-14.0738265118824,
118.423394312347)) ;
#192350=CARTESIAN_POINT('Ctrl Pts',(-7.87629224145502,-14.0738265707863,
118.447625402612)) ;
#192351=CARTESIAN_POINT('Ctrl Pts',(-7.85816352133023,-14.1226647052604,
118.392408247677)) ;
#192352=CARTESIAN_POINT('Ctrl Pts',(-7.84003480120545,-14.1715028397345,
118.337191092741)) ;
#192353=CARTESIAN_POINT('Ctrl Pts',(-7.91383862867624,-14.1715027808306,
118.312960002477)) ;
#192354=CARTESIAN_POINT('Ctrl Pts',(-7.98764245614702,-14.1715027219267,
118.288728912213)) ;
#192355=CARTESIAN_POINT('Ctrl Pts',(-8.00577117627182,-14.1226645874526,
118.343946067148)) ;
#192356=CARTESIAN_POINT('Ctrl Pts',(-8.06283714233654,-14.3171342011777,
118.553214565647)) ;
#192357=CARTESIAN_POINT('Ctrl Pts',(-8.07627530082243,-14.2546443269057,
118.594145026798)) ;
#192358=CARTESIAN_POINT('Ctrl Pts',(-8.0024714756415,-14.2546443659289,
118.618376124037)) ;
#192359=CARTESIAN_POINT('Ctrl Pts',(-7.92866765046057,-14.2546444049521,
118.642607221276)) ;
#192360=CARTESIAN_POINT('Ctrl Pts',(-7.9152294919747,-14.3171342792242,
118.601676760125)) ;
#192361=CARTESIAN_POINT('Ctrl Pts',(-7.90179133348882,-14.3796241534962,
118.560746298974)) ;
#192362=CARTESIAN_POINT('Ctrl Pts',(-7.97559515866974,-14.379624114473,
118.536515201735)) ;
#192363=CARTESIAN_POINT('Ctrl Pts',(-8.04939898385068,-14.3796240754498,
118.512284104496)) ;
#192364=CARTESIAN_POINT('Ctrl Pts',(-8.06283714233654,-14.3171342011777,
118.553214565647)) ;
#192365=CARTESIAN_POINT('Ctrl Pts',(-8.13328894628417,-14.4470643657725,
118.803140602869)) ;
#192366=CARTESIAN_POINT('Ctrl Pts',(-8.14109712925884,-14.375408398759,
118.826923067142)) ;
#192367=CARTESIAN_POINT('Ctrl Pts',(-8.06729330458394,-14.3754084186234,
118.851154165922)) ;
#192368=CARTESIAN_POINT('Ctrl Pts',(-7.99348947990904,-14.3754084384878,
118.875385264702)) ;
#192369=CARTESIAN_POINT('Ctrl Pts',(-7.98568129693438,-14.4470644055013,
118.85160280043)) ;
#192370=CARTESIAN_POINT('Ctrl Pts',(-7.97787311395969,-14.5187203725148,
118.827820336157)) ;
#192371=CARTESIAN_POINT('Ctrl Pts',(-8.0516769386346,-14.5187203526504,
118.803589237377)) ;
#192372=CARTESIAN_POINT('Ctrl Pts',(-8.12548076330949,-14.5187203327861,
118.779358138597)) ;
#192373=CARTESIAN_POINT('Ctrl Pts',(-8.13328894628417,-14.4470643657725,
118.803140602869)) ;
#192374=CARTESIAN_POINT('Ctrl Pts',(-8.21185565403187,-14.503923953364,
119.077904388302)) ;
#192375=CARTESIAN_POINT('Ctrl Pts',(-8.21345628147345,-14.4281893560193,
119.082779640171)) ;
#192376=CARTESIAN_POINT('Ctrl Pts',(-8.13965245513209,-14.4281893585944,
119.107010733875)) ;
#192377=CARTESIAN_POINT('Ctrl Pts',(-8.06584862879074,-14.4281893611695,
119.13124182758)) ;
#192378=CARTESIAN_POINT('Ctrl Pts',(-8.06424800134915,-14.5039239585142,
119.126366575712)) ;
#192379=CARTESIAN_POINT('Ctrl Pts',(-8.06264737390758,-14.5796585558589,
119.121491323843)) ;
#192380=CARTESIAN_POINT('Ctrl Pts',(-8.13645120024894,-14.5796585532838,
119.097260230139)) ;
#192381=CARTESIAN_POINT('Ctrl Pts',(-8.21025502659029,-14.5796585507087,
119.073029136434)) ;
#192382=CARTESIAN_POINT('Ctrl Pts',(-8.21185565403187,-14.503923953364,
119.077904388302)) ;
#192383=CARTESIAN_POINT('Ctrl Pts',(-8.2919897821839,-14.4828378904359,
119.357469635026)) ;
#192384=CARTESIAN_POINT('Ctrl Pts',(-8.28726335063194,-14.4084605775559,
119.34307368624)) ;
#192385=CARTESIAN_POINT('Ctrl Pts',(-8.21345952116713,-14.4084605673929,
119.367304770431)) ;
#192386=CARTESIAN_POINT('Ctrl Pts',(-8.13965569170231,-14.40846055723,119.391535854622)) ;
#192387=CARTESIAN_POINT('Ctrl Pts',(-8.14438212325429,-14.48283787011,119.405931803408)) ;
#192388=CARTESIAN_POINT('Ctrl Pts',(-8.14910855480624,-14.5572151829901,
119.420327752194)) ;
#192389=CARTESIAN_POINT('Ctrl Pts',(-8.22291238427106,-14.557215193153,
119.396096668003)) ;
#192390=CARTESIAN_POINT('Ctrl Pts',(-8.29671621373586,-14.557215203316,
119.371865583812)) ;
#192391=CARTESIAN_POINT('Ctrl Pts',(-8.2919897821839,-14.4828378904359,
119.357469635026)) ;
#192392=CARTESIAN_POINT('Ctrl Pts',(-8.3671164306326,-14.385601171439,119.621760366738)) ;
#192393=CARTESIAN_POINT('Ctrl Pts',(-8.35640339197924,-14.3179002562645,
119.589130178826)) ;
#192394=CARTESIAN_POINT('Ctrl Pts',(-8.28259955872094,-14.3179002385077,
119.613361251462)) ;
#192395=CARTESIAN_POINT('Ctrl Pts',(-8.20879572546266,-14.3179002207509,
119.637592324099)) ;
#192396=CARTESIAN_POINT('Ctrl Pts',(-8.21950876411601,-14.3856011359254,
119.670222512011)) ;
#192397=CARTESIAN_POINT('Ctrl Pts',(-8.23022180276934,-14.4533020510999,
119.702852699924)) ;
#192398=CARTESIAN_POINT('Ctrl Pts',(-8.30402563602765,-14.4533020688567,
119.678621627287)) ;
#192399=CARTESIAN_POINT('Ctrl Pts',(-8.37782946928592,-14.4533020866135,
119.65439055465)) ;
#192400=CARTESIAN_POINT('Ctrl Pts',(-8.3671164306326,-14.385601171439,119.621760366738)) ;
#192401=CARTESIAN_POINT('Ctrl Pts',(-8.43129354623971,-14.2179717447503,
119.852851556862)) ;
#192402=CARTESIAN_POINT('Ctrl Pts',(-8.41534602136537,-14.1618723407489,
119.804277968692)) ;
#192403=CARTESIAN_POINT('Ctrl Pts',(-8.34154218406632,-14.161872321804,
119.828509029022)) ;
#192404=CARTESIAN_POINT('Ctrl Pts',(-8.26773834676728,-14.1618723028591,
119.852740089351)) ;
#192405=CARTESIAN_POINT('Ctrl Pts',(-8.28368587164164,-14.2179717068605,
119.901313677521)) ;
#192406=CARTESIAN_POINT('Ctrl Pts',(-8.299633396516,-14.2740711108619,119.94988726569)) ;
#192407=CARTESIAN_POINT('Ctrl Pts',(-8.37343723381503,-14.2740711298068,
119.925656205361)) ;
#192408=CARTESIAN_POINT('Ctrl Pts',(-8.44724107111407,-14.2740711487517,
119.901425145032)) ;
#192409=CARTESIAN_POINT('Ctrl Pts',(-8.43129354623971,-14.2179717447503,
119.852851556862)) ;
#192410=CARTESIAN_POINT('Ctrl Pts',(-8.47844463780643,-13.9957363810985,
120.031646358861)) ;
#192411=CARTESIAN_POINT('Ctrl Pts',(-8.45845292588495,-13.9550697800569,
119.970754829578)) ;
#192412=CARTESIAN_POINT('Ctrl Pts',(-8.38464908591199,-13.95506976129,119.994985881762)) ;
#192413=CARTESIAN_POINT('Ctrl Pts',(-8.31084524593901,-13.9550697425231,
120.019216933947)) ;
#192414=CARTESIAN_POINT('Ctrl Pts',(-8.33083695786049,-13.9957363435648,
120.08010846323)) ;
#192415=CARTESIAN_POINT('Ctrl Pts',(-8.35082866978197,-14.0364029446064,
120.140999992513)) ;
#192416=CARTESIAN_POINT('Ctrl Pts',(-8.42463250975494,-14.0364029633733,
120.116768940328)) ;
#192417=CARTESIAN_POINT('Ctrl Pts',(-8.4984363497279,-14.0364029821402,
120.092537888144)) ;
#192418=CARTESIAN_POINT('Ctrl Pts',(-8.47844463780643,-13.9957363810985,
120.031646358861)) ;
#192419=CARTESIAN_POINT('Ctrl Pts',(-8.50554208777262,-13.7291995183929,
120.149825509069)) ;
#192420=CARTESIAN_POINT('Ctrl Pts',(-8.48289027006436,-13.707082237132,
120.080831726937)) ;
#192421=CARTESIAN_POINT('Ctrl Pts',(-8.40908642760036,-13.7070822245354,
120.105062771535)) ;
#192422=CARTESIAN_POINT('Ctrl Pts',(-8.33528258513637,-13.7070822119389,
120.129293816133)) ;
#192423=CARTESIAN_POINT('Ctrl Pts',(-8.35793440284465,-13.7291994931998,
120.198287598264)) ;
#192424=CARTESIAN_POINT('Ctrl Pts',(-8.38058622055291,-13.7513167744608,
120.267281380396)) ;
#192425=CARTESIAN_POINT('Ctrl Pts',(-8.45439006301691,-13.7513167870574,
120.243050335798)) ;
#192426=CARTESIAN_POINT('Ctrl Pts',(-8.52819390548089,-13.7513167996539,
120.2188192912)) ;
#192427=CARTESIAN_POINT('Ctrl Pts',(-8.50554208777262,-13.7291995183929,
120.149825509069)) ;
#192428=CARTESIAN_POINT('Ctrl Pts',(-8.50912632410288,-13.4423294051305,
120.196103041933)) ;
#192429=CARTESIAN_POINT('Ctrl Pts',(-8.48545842126137,-13.440209694869,
120.124014428538)) ;
#192430=CARTESIAN_POINT('Ctrl Pts',(-8.41165457775546,-13.4402096875426,
120.148245469962)) ;
#192431=CARTESIAN_POINT('Ctrl Pts',(-8.33785073424954,-13.4402096802161,
120.172476511386)) ;
#192432=CARTESIAN_POINT('Ctrl Pts',(-8.36151863709104,-13.4423293904776,
120.244565124781)) ;
#192433=CARTESIAN_POINT('Ctrl Pts',(-8.38518653993252,-13.444449100739,
120.316653738176)) ;
#192434=CARTESIAN_POINT('Ctrl Pts',(-8.45899038343846,-13.4444491080655,
120.292422696752)) ;
#192435=CARTESIAN_POINT('Ctrl Pts',(-8.53279422694436,-13.444449115392,
120.268191655328)) ;
#192436=CARTESIAN_POINT('Ctrl Pts',(-8.50912632410288,-13.4423294051305,
120.196103041933)) ;
#192437=CARTESIAN_POINT('Ctrl Pts',(-8.48842339088641,-13.1524216120436,
120.168582375125)) ;
#192438=CARTESIAN_POINT('Ctrl Pts',(-8.46543005559105,-13.1705421865172,
120.098548385741)) ;
#192439=CARTESIAN_POINT('Ctrl Pts',(-8.39162621191911,-13.1705421848694,
120.12277942666)) ;
#192440=CARTESIAN_POINT('Ctrl Pts',(-8.31782236824715,-13.1705421832215,
120.147010467578)) ;
#192441=CARTESIAN_POINT('Ctrl Pts',(-8.34081570354252,-13.1524216087479,
120.217044456961)) ;
#192442=CARTESIAN_POINT('Ctrl Pts',(-8.36380903883786,-13.1343010342744,
120.287078446345)) ;
#192443=CARTESIAN_POINT('Ctrl Pts',(-8.43761288250982,-13.1343010359222,
120.262847405426)) ;
#192444=CARTESIAN_POINT('Ctrl Pts',(-8.51141672618176,-13.1343010375701,
120.238616364508)) ;
#192445=CARTESIAN_POINT('Ctrl Pts',(-8.48842339088641,-13.1524216120436,
120.168582375125)) ;
#192446=CARTESIAN_POINT('Ctrl Pts',(-8.44428324962565,-12.8827428706973,
120.06951076432)) ;
#192447=CARTESIAN_POINT('Ctrl Pts',(-8.42360575544995,-12.9197213640829,
120.00653045339)) ;
#192448=CARTESIAN_POINT('Ctrl Pts',(-8.3498019121995,-12.9197213654279,
120.030761495592)) ;
#192449=CARTESIAN_POINT('Ctrl Pts',(-8.27599806894903,-12.919721366773,
120.054992537794)) ;
#192450=CARTESIAN_POINT('Ctrl Pts',(-8.29667556312474,-12.8827428733873,
120.117972848725)) ;
#192451=CARTESIAN_POINT('Ctrl Pts',(-8.31735305730044,-12.8457643800017,
120.180953159656)) ;
#192452=CARTESIAN_POINT('Ctrl Pts',(-8.3911569005509,-12.8457643786566,
120.156722117453)) ;
#192453=CARTESIAN_POINT('Ctrl Pts',(-8.46496074380135,-12.8457643773116,
120.132491075251)) ;
#192454=CARTESIAN_POINT('Ctrl Pts',(-8.44428324962565,-12.8827428706973,
120.06951076432)) ;
#192455=CARTESIAN_POINT('Ctrl Pts',(-8.37882269029488,-12.6504179680888,
119.905639294763)) ;
#192456=CARTESIAN_POINT('Ctrl Pts',(-8.36195051844518,-12.7036746706006,
119.854249381688)) ;
#192457=CARTESIAN_POINT('Ctrl Pts',(-8.28814667575038,-12.7036746730312,
119.878480425583)) ;
#192458=CARTESIAN_POINT('Ctrl Pts',(-8.21434283305557,-12.7036746754618,
119.902711469478)) ;
#192459=CARTESIAN_POINT('Ctrl Pts',(-8.23121500490527,-12.65041797295,119.954101382553)) ;
#192460=CARTESIAN_POINT('Ctrl Pts',(-8.24808717675496,-12.5971612704382,
120.005491295628)) ;
#192461=CARTESIAN_POINT('Ctrl Pts',(-8.32189101944977,-12.5971612680076,
119.981260251733)) ;
#192462=CARTESIAN_POINT('Ctrl Pts',(-8.39569486214457,-12.597161265577,
119.957029207838)) ;
#192463=CARTESIAN_POINT('Ctrl Pts',(-8.37882269029488,-12.6504179680888,
119.905639294763)) ;
#192464=CARTESIAN_POINT('Ctrl Pts',(-8.29622142005809,-12.4733695384466,
119.689502394773)) ;
#192465=CARTESIAN_POINT('Ctrl Pts',(-8.28435858733497,-12.5390682481556,
119.653370120416)) ;
#192466=CARTESIAN_POINT('Ctrl Pts',(-8.21055474474865,-12.5390682494468,
119.677601164641)) ;
#192467=CARTESIAN_POINT('Ctrl Pts',(-8.13675090216231,-12.5390682507379,
119.701832208866)) ;
#192468=CARTESIAN_POINT('Ctrl Pts',(-8.14861373488543,-12.4733695410289,
119.737964483223)) ;
#192469=CARTESIAN_POINT('Ctrl Pts',(-8.16047656760854,-12.4076708313198,
119.77409675758)) ;
#192470=CARTESIAN_POINT('Ctrl Pts',(-8.23428041019488,-12.4076708300287,
119.749865713355)) ;
#192471=CARTESIAN_POINT('Ctrl Pts',(-8.30808425278119,-12.4076708287375,
119.72563466913)) ;
#192472=CARTESIAN_POINT('Ctrl Pts',(-8.29622142005809,-12.4733695384466,
119.689502394773)) ;
#192473=CARTESIAN_POINT('Ctrl Pts',(-8.20108241127664,-12.3637277646619,
119.435348643595)) ;
#192474=CARTESIAN_POINT('Ctrl Pts',(-8.19510827341861,-12.4371796156444,
119.417152383597)) ;
#192475=CARTESIAN_POINT('Ctrl Pts',(-8.12130442993599,-12.4371796152465,
119.441383425092)) ;
#192476=CARTESIAN_POINT('Ctrl Pts',(-8.04750058645336,-12.4371796148486,
119.465614466587)) ;
#192477=CARTESIAN_POINT('Ctrl Pts',(-8.0534747243114,-12.3637277638662,
119.483810726586)) ;
#192478=CARTESIAN_POINT('Ctrl Pts',(-8.05944886216942,-12.2902759128838,
119.502006986584)) ;
#192479=CARTESIAN_POINT('Ctrl Pts',(-8.13325270565205,-12.2902759132816,
119.477775945089)) ;
#192480=CARTESIAN_POINT('Ctrl Pts',(-8.20705654913468,-12.2902759136795,
119.453544903594)) ;
#192481=CARTESIAN_POINT('Ctrl Pts',(-8.20108241127664,-12.3637277646619,
119.435348643595)) ;
#192482=CARTESIAN_POINT('Ctrl Pts',(-8.10069311267931,-12.3302633026411,
119.164918199571)) ;
#192483=CARTESIAN_POINT('Ctrl Pts',(-8.10098863908321,-12.4061588446246,
119.165818325233)) ;
#192484=CARTESIAN_POINT('Ctrl Pts',(-8.02718479434802,-12.406158844275,
119.190049362913)) ;
#192485=CARTESIAN_POINT('Ctrl Pts',(-7.95338094961285,-12.4061588439253,
119.214280400593)) ;
#192486=CARTESIAN_POINT('Ctrl Pts',(-7.95308542320895,-12.3302633019418,
119.213380274931)) ;
#192487=CARTESIAN_POINT('Ctrl Pts',(-7.95278989680505,-12.2543677599582,
119.21248014927)) ;
#192488=CARTESIAN_POINT('Ctrl Pts',(-8.02659374154021,-12.2543677603079,
119.18824911159)) ;
#192489=CARTESIAN_POINT('Ctrl Pts',(-8.10039758627541,-12.2543677606575,
119.16401807391)) ;
#192490=CARTESIAN_POINT('Ctrl Pts',(-8.10069311267931,-12.3302633026411,
119.164918199571)) ;
#192491=CARTESIAN_POINT('Ctrl Pts',(-8.00044993799628,-12.3743151570883,
118.895045920248)) ;
#192492=CARTESIAN_POINT('Ctrl Pts',(-8.00701167902443,-12.4472453738058,
118.915031924497)) ;
#192493=CARTESIAN_POINT('Ctrl Pts',(-7.93320783263552,-12.4472453760978,
118.93926295714)) ;
#192494=CARTESIAN_POINT('Ctrl Pts',(-7.85940398624658,-12.4472453783898,
118.963493989783)) ;
#192495=CARTESIAN_POINT('Ctrl Pts',(-7.85284224521843,-12.3743151616723,
118.943507985534)) ;
#192496=CARTESIAN_POINT('Ctrl Pts',(-7.84628050419029,-12.3013849449547,
118.923521981286)) ;
#192497=CARTESIAN_POINT('Ctrl Pts',(-7.92008435057921,-12.3013849426627,
118.899290948643)) ;
#192498=CARTESIAN_POINT('Ctrl Pts',(-7.99388819696813,-12.3013849403707,
118.875059916)) ;
#192499=CARTESIAN_POINT('Ctrl Pts',(-8.00044993799628,-12.3743151570883,
118.895045920248)) ;
#192500=CARTESIAN_POINT('Ctrl Pts',(-7.90710319884704,-12.4928395526405,
118.64614258601)) ;
#192501=CARTESIAN_POINT('Ctrl Pts',(-7.91945933895386,-12.5575998714036,
118.683777394806)) ;
#192502=CARTESIAN_POINT('Ctrl Pts',(-7.84565549110987,-12.5575998792926,
118.708008423017)) ;
#192503=CARTESIAN_POINT('Ctrl Pts',(-7.7718516432659,-12.5575998871817,
118.732239451228)) ;
#192504=CARTESIAN_POINT('Ctrl Pts',(-7.7594955031591,-12.4928395684187,
118.694604642432)) ;
#192505=CARTESIAN_POINT('Ctrl Pts',(-7.74713936305227,-12.4280792496557,
118.656969833636)) ;
#192506=CARTESIAN_POINT('Ctrl Pts',(-7.82094321089625,-12.4280792417666,
118.632738805425)) ;
#192507=CARTESIAN_POINT('Ctrl Pts',(-7.89474705874023,-12.4280792338775,
118.608507777214)) ;
#192508=CARTESIAN_POINT('Ctrl Pts',(-7.90710319884704,-12.4928395526405,
118.64614258601)) ;
#192509=CARTESIAN_POINT('Ctrl Pts',(-7.82605565543513,-12.6792484033362,
118.434964572872)) ;
#192510=CARTESIAN_POINT('Ctrl Pts',(-7.84335047013331,-12.7310874670911,
118.487641787435)) ;
#192511=CARTESIAN_POINT('Ctrl Pts',(-7.76954662110735,-12.7310874856029,
118.511872812046)) ;
#192512=CARTESIAN_POINT('Ctrl Pts',(-7.69574277208138,-12.7310875041147,
118.536103836657)) ;
#192513=CARTESIAN_POINT('Ctrl Pts',(-7.67844795738318,-12.6792484403597,
118.483426622094)) ;
#192514=CARTESIAN_POINT('Ctrl Pts',(-7.66115314268502,-12.6274093766048,
118.430749407531)) ;
#192515=CARTESIAN_POINT('Ctrl Pts',(-7.73495699171098,-12.627409358093,
118.40651838292)) ;
#192516=CARTESIAN_POINT('Ctrl Pts',(-7.80876084073694,-12.6274093395813,
118.382287358309)) ;
#192517=CARTESIAN_POINT('Ctrl Pts',(-7.82605565543513,-12.6792484033362,
118.434964572872)) ;
#192518=CARTESIAN_POINT('Ctrl Pts',(-7.76370923303463,-12.9157037711306,
118.280276167893)) ;
#192519=CARTESIAN_POINT('Ctrl Pts',(-7.78465336230621,-12.9511079256509,
118.344068605718)) ;
#192520=CARTESIAN_POINT('Ctrl Pts',(-7.71084951411926,-12.9511079534963,
118.368299632885)) ;
#192521=CARTESIAN_POINT('Ctrl Pts',(-7.63704566593232,-12.9511079813417,
118.392530660051)) ;
#192522=CARTESIAN_POINT('Ctrl Pts',(-7.61610153666074,-12.9157038268213,
118.328738222226)) ;
#192523=CARTESIAN_POINT('Ctrl Pts',(-7.59515740738914,-12.880299672301,
118.264945784401)) ;
#192524=CARTESIAN_POINT('Ctrl Pts',(-7.6689612555761,-12.8802996444556,
118.240714757234)) ;
#192525=CARTESIAN_POINT('Ctrl Pts',(-7.74276510376304,-12.8802996166102,
118.216483730068)) ;
#192526=CARTESIAN_POINT('Ctrl Pts',(-7.76370923303463,-12.9157037711306,
118.280276167893)) ;
#192527=CARTESIAN_POINT('Ctrl Pts',(-7.7222130498299,-13.1914441677562,
118.189580023527)) ;
#192528=CARTESIAN_POINT('Ctrl Pts',(-7.74534632640251,-13.2076474543041,
118.260040250604)) ;
#192529=CARTESIAN_POINT('Ctrl Pts',(-7.67154247998087,-13.2076474957357,
118.284271283147)) ;
#192530=CARTESIAN_POINT('Ctrl Pts',(-7.59773863355922,-13.2076475371673,
118.30850231569)) ;
#192531=CARTESIAN_POINT('Ctrl Pts',(-7.57460535698663,-13.1914442506193,
118.238042088613)) ;
#192532=CARTESIAN_POINT('Ctrl Pts',(-7.55147208041403,-13.1752409640713,
118.167581861536)) ;
#192533=CARTESIAN_POINT('Ctrl Pts',(-7.62527592683567,-13.1752409226398,
118.143350828993)) ;
#192534=CARTESIAN_POINT('Ctrl Pts',(-7.69907977325731,-13.1752408812082,
118.119119796449)) ;
#192535=CARTESIAN_POINT('Ctrl Pts',(-7.7222130498299,-13.1914441677562,
118.189580023527)) ;
#192536=CARTESIAN_POINT('Ctrl Pts',(-7.70493031502856,-13.4802992555045,
118.172216171245)) ;
#192537=CARTESIAN_POINT('Ctrl Pts',(-7.72857354727237,-13.4763581958197,
118.244229640883)) ;
#192538=CARTESIAN_POINT('Ctrl Pts',(-7.65476970455688,-13.4763582452253,
118.268460684714)) ;
#192539=CARTESIAN_POINT('Ctrl Pts',(-7.58096586184136,-13.4763582946309,
118.292691728546)) ;
#192540=CARTESIAN_POINT('Ctrl Pts',(-7.55732262959753,-13.4802993543157,
118.220678258908)) ;
#192541=CARTESIAN_POINT('Ctrl Pts',(-7.53367939735367,-13.4842404140005,
118.14866478927)) ;
#192542=CARTESIAN_POINT('Ctrl Pts',(-7.60748324006919,-13.4842403645949,
118.124433745439)) ;
#192543=CARTESIAN_POINT('Ctrl Pts',(-7.6812870827847,-13.4842403151893,
118.100202701607)) ;
#192544=CARTESIAN_POINT('Ctrl Pts',(-7.70493031502856,-13.4802992555045,
118.172216171245)) ;
#192545=CARTESIAN_POINT('Ctrl Pts',(-7.71165791300415,-13.7664087624137,
118.228202531316)) ;
#192546=CARTESIAN_POINT('Ctrl Pts',(-7.73413116046454,-13.7424862734231,
118.296652415907)) ;
#192547=CARTESIAN_POINT('Ctrl Pts',(-7.66032732263785,-13.7424863290053,
118.320883474629)) ;
#192548=CARTESIAN_POINT('Ctrl Pts',(-7.58652348481117,-13.7424863845875,
118.345114533351)) ;
#192549=CARTESIAN_POINT('Ctrl Pts',(-7.5640502373508,-13.766408873578,118.276664648761)) ;
#192550=CARTESIAN_POINT('Ctrl Pts',(-7.54157698989042,-13.7903313625685,
118.20821476417)) ;
#192551=CARTESIAN_POINT('Ctrl Pts',(-7.61538082771709,-13.7903313069864,
118.183983705448)) ;
#192552=CARTESIAN_POINT('Ctrl Pts',(-7.68918466554377,-13.7903312514042,
118.159752646726)) ;
#192553=CARTESIAN_POINT('Ctrl Pts',(-7.71165791300415,-13.7664087624137,
118.228202531316)) ;
#192554=CARTESIAN_POINT('Ctrl Pts',(-7.74161114589191,-14.0278445854345,
118.354981969349)) ;
#192555=CARTESIAN_POINT('Ctrl Pts',(-7.76129016724846,-13.98563446645,118.414921091898)) ;
#192556=CARTESIAN_POINT('Ctrl Pts',(-7.68748633547243,-13.9856345227655,
118.439152169049)) ;
#192557=CARTESIAN_POINT('Ctrl Pts',(-7.61368250369641,-13.985634579081,
118.463383246201)) ;
#192558=CARTESIAN_POINT('Ctrl Pts',(-7.59400348233985,-14.0278446980655,
118.403444123652)) ;
#192559=CARTESIAN_POINT('Ctrl Pts',(-7.57432446098331,-14.07005481705,118.343505001104)) ;
#192560=CARTESIAN_POINT('Ctrl Pts',(-7.64812829275933,-14.0700547607345,
118.319273923952)) ;
#192561=CARTESIAN_POINT('Ctrl Pts',(-7.72193212453537,-14.070054704419,
118.295042846801)) ;
#192562=CARTESIAN_POINT('Ctrl Pts',(-7.74161114589191,-14.0278445854345,
118.354981969349)) ;
#192563=CARTESIAN_POINT('Ctrl Pts',(-7.79147735941891,-14.2444016591037,
118.542237068999)) ;
#192564=CARTESIAN_POINT('Ctrl Pts',(-7.80697137655135,-14.1870110797581,
118.589429343793)) ;
#192565=CARTESIAN_POINT('Ctrl Pts',(-7.73316755069903,-14.1870111286872,
118.613660438987)) ;
#192566=CARTESIAN_POINT('Ctrl Pts',(-7.6593637248467,-14.1870111776162,
118.637891534181)) ;
#192567=CARTESIAN_POINT('Ctrl Pts',(-7.64386970771426,-14.2444017569618,
118.590699259387)) ;
#192568=CARTESIAN_POINT('Ctrl Pts',(-7.6283756905818,-14.3017923363074,
118.543506984594)) ;
#192569=CARTESIAN_POINT('Ctrl Pts',(-7.70217951643413,-14.3017922873783,
118.5192758894)) ;
#192570=CARTESIAN_POINT('Ctrl Pts',(-7.77598334228645,-14.3017922384493,
118.495044794206)) ;
#192571=CARTESIAN_POINT('Ctrl Pts',(-7.79147735941891,-14.2444016591037,
118.542237068999)) ;
#192572=CARTESIAN_POINT('Ctrl Pts',(-7.85719638681783,-14.4026063876543,
118.777859695063)) ;
#192573=CARTESIAN_POINT('Ctrl Pts',(-7.86739098952979,-14.3340872602138,
118.808910808447)) ;
#192574=CARTESIAN_POINT('Ctrl Pts',(-7.79358716916343,-14.3340872957345,
118.83314192035)) ;
#192575=CARTESIAN_POINT('Ctrl Pts',(-7.71978334879709,-14.3340873312552,
118.857373032254)) ;
#192576=CARTESIAN_POINT('Ctrl Pts',(-7.70958874608515,-14.4026064586957,
118.82632191887)) ;
#192577=CARTESIAN_POINT('Ctrl Pts',(-7.69939414337321,-14.4711255861363,
118.795270805486)) ;
#192578=CARTESIAN_POINT('Ctrl Pts',(-7.77319796373955,-14.4711255506156,
118.771039693583)) ;
#192579=CARTESIAN_POINT('Ctrl Pts',(-7.84700178410591,-14.4711255150949,
118.74680858168)) ;
#192580=CARTESIAN_POINT('Ctrl Pts',(-7.85719638681783,-14.4026063876543,
118.777859695063)) ;
#192581=CARTESIAN_POINT('Ctrl Pts',(-7.93377264099751,-14.4903817315252,
119.046765235563)) ;
#192582=CARTESIAN_POINT('Ctrl Pts',(-7.93789788343907,-14.4156342594261,
119.059330056695)) ;
#192583=CARTESIAN_POINT('Ctrl Pts',(-7.86409406767712,-14.4156342751567,
119.083561182623)) ;
#192584=CARTESIAN_POINT('Ctrl Pts',(-7.79029025191515,-14.4156342908872,
119.10779230855)) ;
#192585=CARTESIAN_POINT('Ctrl Pts',(-7.7861650094736,-14.4903817629863,
119.095227487418)) ;
#192586=CARTESIAN_POINT('Ctrl Pts',(-7.78203976703203,-14.5651292350854,
119.082662666287)) ;
#192587=CARTESIAN_POINT('Ctrl Pts',(-7.85584358279399,-14.5651292193548,
119.058431540359)) ;
#192588=CARTESIAN_POINT('Ctrl Pts',(-7.92964739855593,-14.5651292036242,
119.034200414431)) ;
#192589=CARTESIAN_POINT('Ctrl Pts',(-7.93377264099751,-14.4903817315252,
119.046765235563)) ;
#192590=CARTESIAN_POINT('Ctrl Pts',(-8.01373210317338,-14.5006966747965,
119.325637975014)) ;
#192591=CARTESIAN_POINT('Ctrl Pts',(-8.0115497988902,-14.4251205193326,
119.318991026449)) ;
#192592=CARTESIAN_POINT('Ctrl Pts',(-7.93774598491779,-14.425120510433,
119.343222157827)) ;
#192593=CARTESIAN_POINT('Ctrl Pts',(-7.86394217094539,-14.4251205015334,
119.367453289206)) ;
#192594=CARTESIAN_POINT('Ctrl Pts',(-7.86612447522857,-14.5006966569974,
119.374100237771)) ;
#192595=CARTESIAN_POINT('Ctrl Pts',(-7.86830677951178,-14.5762728124613,
119.380747186336)) ;
#192596=CARTESIAN_POINT('Ctrl Pts',(-7.94211059348418,-14.5762728213609,
119.356516054957)) ;
#192597=CARTESIAN_POINT('Ctrl Pts',(-8.01591440745658,-14.5762728302605,
119.332284923579)) ;
#192598=CARTESIAN_POINT('Ctrl Pts',(-8.01373210317338,-14.5006966747965,
119.325637975014)) ;
#192599=CARTESIAN_POINT('Ctrl Pts',(-8.09161196909389,-14.4339382681578,
119.598307168471)) ;
#192600=CARTESIAN_POINT('Ctrl Pts',(-8.08325550424145,-14.3629125582236,
119.572854722915)) ;
#192601=CARTESIAN_POINT('Ctrl Pts',(-8.00945168990967,-14.3629125229021,
119.597085853198)) ;
#192602=CARTESIAN_POINT('Ctrl Pts',(-7.93564787557786,-14.3629124875806,
119.621316983482)) ;
#192603=CARTESIAN_POINT('Ctrl Pts',(-7.94400434043028,-14.4339381975148,
119.646769429038)) ;
#192604=CARTESIAN_POINT('Ctrl Pts',(-7.9523608052827,-14.504963907449,119.672221874595)) ;
#192605=CARTESIAN_POINT('Ctrl Pts',(-8.02616461961452,-14.5049639427705,
119.647990744311)) ;
#192606=CARTESIAN_POINT('Ctrl Pts',(-8.0999684339463,-14.504963978092,119.623759614027)) ;
#192607=CARTESIAN_POINT('Ctrl Pts',(-8.09161196909389,-14.4339382681578,
119.598307168471)) ;
#192608=CARTESIAN_POINT('Ctrl Pts',(-8.16098641912054,-14.293783753758,
119.845172580273)) ;
#192609=CARTESIAN_POINT('Ctrl Pts',(-8.14703842436003,-14.2324386627931,
119.802689236725)) ;
#192610=CARTESIAN_POINT('Ctrl Pts',(-8.07323460709228,-14.2324386013355,
119.826920358066)) ;
#192611=CARTESIAN_POINT('Ctrl Pts',(-7.99943078982447,-14.2324385398779,
119.851151479407)) ;
#192612=CARTESIAN_POINT('Ctrl Pts',(-8.01337878458499,-14.2937836308428,
119.893634822955)) ;
#192613=CARTESIAN_POINT('Ctrl Pts',(-8.0273267793455,-14.3551287218076,
119.936118166504)) ;
#192614=CARTESIAN_POINT('Ctrl Pts',(-8.10113059661327,-14.3551287832652,
119.911887045163)) ;
#192615=CARTESIAN_POINT('Ctrl Pts',(-8.17493441388104,-14.3551288447229,
119.887655923821)) ;
#192616=CARTESIAN_POINT('Ctrl Pts',(-8.16098641912054,-14.293783753758,
119.845172580273)) ;
#192617=CARTESIAN_POINT('Ctrl Pts',(-8.21570971002611,-14.0908689343358,
120.047346649353)) ;
#192618=CARTESIAN_POINT('Ctrl Pts',(-8.19718615656026,-14.0436003014087,
119.990926892202)) ;
#192619=CARTESIAN_POINT('Ctrl Pts',(-8.12338233373114,-14.0436002177779,
120.015157996604)) ;
#192620=CARTESIAN_POINT('Ctrl Pts',(-8.04957851090201,-14.0436001341472,
120.039389101006)) ;
#192621=CARTESIAN_POINT('Ctrl Pts',(-8.06810206436785,-14.0908687670742,
120.095808858157)) ;
#192622=CARTESIAN_POINT('Ctrl Pts',(-8.08662561783368,-14.1381374000013,
120.152228615309)) ;
#192623=CARTESIAN_POINT('Ctrl Pts',(-8.16042944066284,-14.1381374836321,
120.127997510907)) ;
#192624=CARTESIAN_POINT('Ctrl Pts',(-8.23423326349196,-14.1381375672628,
120.103766406505)) ;
#192625=CARTESIAN_POINT('Ctrl Pts',(-8.21570971002611,-14.0908689343358,
120.047346649353)) ;
#192626=CARTESIAN_POINT('Ctrl Pts',(-8.25119308463164,-13.8416080598376,
120.190682254416)) ;
#192627=CARTESIAN_POINT('Ctrl Pts',(-8.22943548398096,-13.8116727384737,
120.124412111326)) ;
#192628=CARTESIAN_POINT('Ctrl Pts',(-8.15563165367641,-13.8116726391883,
120.148643192959)) ;
#192629=CARTESIAN_POINT('Ctrl Pts',(-8.08182782337186,-13.8116725399028,
120.172874274592)) ;
#192630=CARTESIAN_POINT('Ctrl Pts',(-8.10358542402254,-13.8416078612666,
120.239144417682)) ;
#192631=CARTESIAN_POINT('Ctrl Pts',(-8.12534302467321,-13.8715431826305,
120.305414560772)) ;
#192632=CARTESIAN_POINT('Ctrl Pts',(-8.19914685497777,-13.871543281916,
120.281183479139)) ;
#192633=CARTESIAN_POINT('Ctrl Pts',(-8.27295068528229,-13.8715433812015,
120.256952397506)) ;
#192634=CARTESIAN_POINT('Ctrl Pts',(-8.25119308463164,-13.8416080598376,
120.190682254416)) ;
#192635=CARTESIAN_POINT('Ctrl Pts',(-8.26455274508899,-13.5600342116363,
120.266919542768)) ;
#192636=CARTESIAN_POINT('Ctrl Pts',(-8.24109469557833,-13.5497128461305,
120.195470106805)) ;
#192637=CARTESIAN_POINT('Ctrl Pts',(-8.16729085657722,-13.5497127385965,
120.21970116195)) ;
#192638=CARTESIAN_POINT('Ctrl Pts',(-8.09348701757607,-13.5497126310626,
120.243932217095)) ;
#192639=CARTESIAN_POINT('Ctrl Pts',(-8.11694506708672,-13.5600339965684,
120.315381653058)) ;
#192640=CARTESIAN_POINT('Ctrl Pts',(-8.14040311659736,-13.5703553620741,
120.386831089021)) ;
#192641=CARTESIAN_POINT('Ctrl Pts',(-8.2142069555985,-13.5703554696081,
120.362600033876)) ;
#192642=CARTESIAN_POINT('Ctrl Pts',(-8.28801079459963,-13.570355577142,
120.338368978732)) ;
#192643=CARTESIAN_POINT('Ctrl Pts',(-8.26455274508899,-13.5600342116363,
120.266919542768)) ;
#192644=CARTESIAN_POINT('Ctrl Pts',(-8.25379252720853,-13.2694053226454,
120.269537469826)) ;
#192645=CARTESIAN_POINT('Ctrl Pts',(-8.23031867646663,-13.2793593921655,
120.198039905872)) ;
#192646=CARTESIAN_POINT('Ctrl Pts',(-8.15651482840728,-13.2793592852709,
120.222270933427)) ;
#192647=CARTESIAN_POINT('Ctrl Pts',(-8.08271098034794,-13.2793591783763,
120.246501960982)) ;
#192648=CARTESIAN_POINT('Ctrl Pts',(-8.10618483108986,-13.2694051088563,
120.317999524935)) ;
#192649=CARTESIAN_POINT('Ctrl Pts',(-8.12965868183175,-13.2594510393362,
120.389497088889)) ;
#192650=CARTESIAN_POINT('Ctrl Pts',(-8.2034625298911,-13.2594511462308,
120.365266061334)) ;
#192651=CARTESIAN_POINT('Ctrl Pts',(-8.27726637795044,-13.2594512531254,
120.341035033779)) ;
#192652=CARTESIAN_POINT('Ctrl Pts',(-8.25379252720853,-13.2694053226454,
120.269537469826)) ;
#192653=CARTESIAN_POINT('Ctrl Pts',(-8.21877794635093,-12.9879324368107,
120.198480845472)) ;
#192654=CARTESIAN_POINT('Ctrl Pts',(-8.19697716664803,-13.0175527392448,
120.132079185993)) ;
#192655=CARTESIAN_POINT('Ctrl Pts',(-8.12317331011067,-13.0175526420622,
120.156310187725)) ;
#192656=CARTESIAN_POINT('Ctrl Pts',(-8.04936945357328,-13.0175525448795,
120.180541189457)) ;
#192657=CARTESIAN_POINT('Ctrl Pts',(-8.07117023327617,-12.9879322424453,
120.246942848936)) ;
#192658=CARTESIAN_POINT('Ctrl Pts',(-8.09297101297905,-12.9583119400111,
120.313344508415)) ;
#192659=CARTESIAN_POINT('Ctrl Pts',(-8.16677486951643,-12.9583120371938,
120.289113506683)) ;
#192660=CARTESIAN_POINT('Ctrl Pts',(-8.24057872605381,-12.9583121343765,
120.264882504951)) ;
#192661=CARTESIAN_POINT('Ctrl Pts',(-8.21877794635093,-12.9879324368107,
120.198480845472)) ;
#192662=CARTESIAN_POINT('Ctrl Pts',(-8.1617475280646,-12.7391527795793,
120.060108032395)) ;
#192663=CARTESIAN_POINT('Ctrl Pts',(-8.14316493865999,-12.786186317019,
120.003508461359)) ;
#192664=CARTESIAN_POINT('Ctrl Pts',(-8.06936107504735,-12.7861862364123,
120.027739441541)) ;
#192665=CARTESIAN_POINT('Ctrl Pts',(-7.99555721143471,-12.7861861558057,
120.051970421724)) ;
#192666=CARTESIAN_POINT('Ctrl Pts',(-8.01413980083932,-12.739152618366,
120.108569992759)) ;
#192667=CARTESIAN_POINT('Ctrl Pts',(-8.03272239024394,-12.6921190809264,
120.165169563794)) ;
#192668=CARTESIAN_POINT('Ctrl Pts',(-8.10652625385659,-12.692119161533,
120.140938583612)) ;
#192669=CARTESIAN_POINT('Ctrl Pts',(-8.18033011746921,-12.6921192421396,
120.11670760343)) ;
#192670=CARTESIAN_POINT('Ctrl Pts',(-8.1617475280646,-12.7391527795793,
120.060108032395)) ;
#192671=CARTESIAN_POINT('Ctrl Pts',(-8.08553845111122,-12.5377712145214,
119.86347894876)) ;
#192672=CARTESIAN_POINT('Ctrl Pts',(-8.07151433693855,-12.5989350569668,
119.82076375785)) ;
#192673=CARTESIAN_POINT('Ctrl Pts',(-7.9977104683385,-12.5989349988532,
119.844994722841)) ;
#192674=CARTESIAN_POINT('Ctrl Pts',(-7.92390659973845,-12.5989349407397,
119.869225687832)) ;
#192675=CARTESIAN_POINT('Ctrl Pts',(-7.93793071391114,-12.5377710982944,
119.911940878743)) ;
#192676=CARTESIAN_POINT('Ctrl Pts',(-7.9519548280838,-12.476607255849,119.954656069653)) ;
#192677=CARTESIAN_POINT('Ctrl Pts',(-8.02575869668384,-12.4766073139625,
119.930425104662)) ;
#192678=CARTESIAN_POINT('Ctrl Pts',(-8.09956256528389,-12.476607372076,
119.90619413967)) ;
#192679=CARTESIAN_POINT('Ctrl Pts',(-8.08553845111122,-12.5377712145214,
119.86347894876)) ;
#192680=CARTESIAN_POINT('Ctrl Pts',(-7.99493866021685,-12.3995925801182,
119.623032110138)) ;
#192681=CARTESIAN_POINT('Ctrl Pts',(-7.98648424887465,-12.4704956782947,
119.597281335481)) ;
#192682=CARTESIAN_POINT('Ctrl Pts',(-7.91268037787084,-12.4704956456056,
119.621512293151)) ;
#192683=CARTESIAN_POINT('Ctrl Pts',(-7.83887650686702,-12.4704956129164,
119.64574325082)) ;
#192684=CARTESIAN_POINT('Ctrl Pts',(-7.84733091820922,-12.39959251474,119.671494025477)) ;
#192685=CARTESIAN_POINT('Ctrl Pts',(-7.85578532955141,-12.3286894165636,
119.697244800134)) ;
#192686=CARTESIAN_POINT('Ctrl Pts',(-7.92958920055522,-12.3286894492527,
119.673013842464)) ;
#192687=CARTESIAN_POINT('Ctrl Pts',(-8.00339307155904,-12.3286894819418,
119.648782884794)) ;
#192688=CARTESIAN_POINT('Ctrl Pts',(-7.99493866021685,-12.3995925801182,
119.623032110138)) ;
#192689=CARTESIAN_POINT('Ctrl Pts',(-7.89593436549806,-12.33457880474,119.356931430303)) ;
#192690=CARTESIAN_POINT('Ctrl Pts',(-7.89364599672396,-12.4101277476762,
119.349961426533)) ;
#192691=CARTESIAN_POINT('Ctrl Pts',(-7.8198421257994,-12.4101277401761,
119.374192384444)) ;
#192692=CARTESIAN_POINT('Ctrl Pts',(-7.74603825487482,-12.410127732676,
119.398423342356)) ;
#192693=CARTESIAN_POINT('Ctrl Pts',(-7.74832662364891,-12.3345787897397,
119.405393346125)) ;
#192694=CARTESIAN_POINT('Ctrl Pts',(-7.750614992423,-12.2590298468035,119.412363349895)) ;
#192695=CARTESIAN_POINT('Ctrl Pts',(-7.82441886334756,-12.2590298543036,
119.388132391984)) ;
#192696=CARTESIAN_POINT('Ctrl Pts',(-7.89822273427213,-12.2590298618037,
119.363901434073)) ;
#192697=CARTESIAN_POINT('Ctrl Pts',(-7.89593436549806,-12.33457880474,119.356931430303)) ;
#192698=CARTESIAN_POINT('Ctrl Pts',(-7.79477633291221,-12.3470312097476,
119.084250661337)) ;
#192699=CARTESIAN_POINT('Ctrl Pts',(-7.7988141092919,-12.4218246112721,
119.096549075109)) ;
#192700=CARTESIAN_POINT('Ctrl Pts',(-7.72501024069841,-12.4218246263605,
119.120780040121)) ;
#192701=CARTESIAN_POINT('Ctrl Pts',(-7.65120637210492,-12.4218246414487,
119.145011005132)) ;
#192702=CARTESIAN_POINT('Ctrl Pts',(-7.64716859572525,-12.3470312399242,
119.13271259136)) ;
#192703=CARTESIAN_POINT('Ctrl Pts',(-7.64313081934554,-12.2722378383997,
119.120414177587)) ;
#192704=CARTESIAN_POINT('Ctrl Pts',(-7.71693468793903,-12.2722378233114,
119.096183212576)) ;
#192705=CARTESIAN_POINT('Ctrl Pts',(-7.79073855653252,-12.2722378082231,
119.071952247565)) ;
#192706=CARTESIAN_POINT('Ctrl Pts',(-7.79477633291221,-12.3470312097476,
119.084250661337)) ;
#192707=CARTESIAN_POINT('Ctrl Pts',(-7.6977506200353,-12.4361986060041,
118.824206306285)) ;
#192708=CARTESIAN_POINT('Ctrl Pts',(-7.7078345844544,-12.5048795255924,
118.854920433421)) ;
#192709=CARTESIAN_POINT('Ctrl Pts',(-7.63403072013485,-12.5048795584336,
118.87915141145)) ;
#192710=CARTESIAN_POINT('Ctrl Pts',(-7.56022685581533,-12.5048795912748,
118.903382389479)) ;
#192711=CARTESIAN_POINT('Ctrl Pts',(-7.55014289139622,-12.4361986716865,
118.872668262343)) ;
#192712=CARTESIAN_POINT('Ctrl Pts',(-7.54005892697714,-12.3675177520983,
118.841954135207)) ;
#192713=CARTESIAN_POINT('Ctrl Pts',(-7.61386279129669,-12.367517719257,
118.817723157178)) ;
#192714=CARTESIAN_POINT('Ctrl Pts',(-7.68766665561624,-12.3675176864158,
118.793492179149)) ;
#192715=CARTESIAN_POINT('Ctrl Pts',(-7.6977506200353,-12.4361986060041,
118.824206306285)) ;
#192716=CARTESIAN_POINT('Ctrl Pts',(-7.61114947056002,-12.5959885808789,
118.595944474179)) ;
#192717=CARTESIAN_POINT('Ctrl Pts',(-7.62656038830856,-12.6536171134987,
118.642883641819)) ;
#192718=CARTESIAN_POINT('Ctrl Pts',(-7.55275652944442,-12.6536171574683,
118.667114636464)) ;
#192719=CARTESIAN_POINT('Ctrl Pts',(-7.47895267058027,-12.653617201438,
118.69134563111)) ;
#192720=CARTESIAN_POINT('Ctrl Pts',(-7.46354175283175,-12.5959886688182,
118.64440646347)) ;
#192721=CARTESIAN_POINT('Ctrl Pts',(-7.44813083508317,-12.5383601361984,
118.597467295831)) ;
#192722=CARTESIAN_POINT('Ctrl Pts',(-7.52193469394733,-12.5383600922288,
118.573236301185)) ;
#192723=CARTESIAN_POINT('Ctrl Pts',(-7.59573855281146,-12.5383600482591,
118.54900530654)) ;
#192724=CARTESIAN_POINT('Ctrl Pts',(-7.61114947056002,-12.5959885808789,
118.595944474179)) ;
#192725=CARTESIAN_POINT('Ctrl Pts',(-7.54064541308495,-12.8143066918053,
118.416638915935)) ;
#192726=CARTESIAN_POINT('Ctrl Pts',(-7.56026899454005,-12.8567794160869,
118.476409177672)) ;
#192727=CARTESIAN_POINT('Ctrl Pts',(-7.48646514127264,-12.8567794648258,
118.500640189364)) ;
#192728=CARTESIAN_POINT('Ctrl Pts',(-7.41266128800525,-12.8567795135646,
118.524871201056)) ;
#192729=CARTESIAN_POINT('Ctrl Pts',(-7.39303770655016,-12.814306789283,
118.46510093932)) ;
#192730=CARTESIAN_POINT('Ctrl Pts',(-7.37341412509507,-12.7718340650015,
118.405330677583)) ;
#192731=CARTESIAN_POINT('Ctrl Pts',(-7.44721797836247,-12.7718340162626,
118.381099665891)) ;
#192732=CARTESIAN_POINT('Ctrl Pts',(-7.52102183162987,-12.7718339675238,
118.356868654199)) ;
#192733=CARTESIAN_POINT('Ctrl Pts',(-7.54064541308495,-12.8143066918053,
118.416638915935)) ;
#192734=CARTESIAN_POINT('Ctrl Pts',(-7.49026997235467,-13.0760276863323,
118.29867594851)) ;
#192735=CARTESIAN_POINT('Ctrl Pts',(-7.51270657196419,-13.1002911910354,
118.367014209835)) ;
#192736=CARTESIAN_POINT('Ctrl Pts',(-7.4389027239676,-13.1002912381593,
118.391245237581)) ;
#192737=CARTESIAN_POINT('Ctrl Pts',(-7.36509887597101,-13.1002912852831,
118.415476265327)) ;
#192738=CARTESIAN_POINT('Ctrl Pts',(-7.34266227636148,-13.07602778058,118.347138004003)) ;
#192739=CARTESIAN_POINT('Ctrl Pts',(-7.32022567675194,-13.0517642758768,
118.278799742678)) ;
#192740=CARTESIAN_POINT('Ctrl Pts',(-7.39402952474855,-13.051764228753,
118.254568714932)) ;
#192741=CARTESIAN_POINT('Ctrl Pts',(-7.46783337274512,-13.0517641816292,
118.230337687185)) ;
#192742=CARTESIAN_POINT('Ctrl Pts',(-7.49026997235467,-13.0760276863323,
118.29867594851)) ;
#192743=CARTESIAN_POINT('Ctrl Pts',(-7.46298666678461,-13.3628060373472,
118.251109449983)) ;
#192744=CARTESIAN_POINT('Ctrl Pts',(-7.48662704438139,-13.3670829170375,
118.32311422501)) ;
#192745=CARTESIAN_POINT('Ctrl Pts',(-7.41282320058781,-13.3670829569658,
118.347345265558)) ;
#192746=CARTESIAN_POINT('Ctrl Pts',(-7.33901935679421,-13.3670829968941,
118.371576306106)) ;
#192747=CARTESIAN_POINT('Ctrl Pts',(-7.31537897919742,-13.3628061172038,
118.299571531079)) ;
#192748=CARTESIAN_POINT('Ctrl Pts',(-7.2917386016006,-13.3585292375136,
118.227566756052)) ;
#192749=CARTESIAN_POINT('Ctrl Pts',(-7.36554244539421,-13.3585291975852,
118.203335715504)) ;
#192750=CARTESIAN_POINT('Ctrl Pts',(-7.4393462891878,-13.3585291576569,
118.179104674956)) ;
#192751=CARTESIAN_POINT('Ctrl Pts',(-7.46298666678461,-13.3628060373472,
118.251109449983)) ;
#192752=CARTESIAN_POINT('Ctrl Pts',(-7.46006094552524,-13.6523296523906,
118.277586231545)) ;
#192753=CARTESIAN_POINT('Ctrl Pts',(-7.48320907995678,-13.6363976370677,
118.348091713465)) ;
#192754=CARTESIAN_POINT('Ctrl Pts',(-7.40940523890514,-13.636397668316,
118.372322762364)) ;
#192755=CARTESIAN_POINT('Ctrl Pts',(-7.33560139785351,-13.6363976995644,
118.396553811264)) ;
#192756=CARTESIAN_POINT('Ctrl Pts',(-7.31245326342196,-13.6523297148873,
118.326048329344)) ;
#192757=CARTESIAN_POINT('Ctrl Pts',(-7.2893051289904,-13.6682617302103,
118.255542847425)) ;
#192758=CARTESIAN_POINT('Ctrl Pts',(-7.36310897004204,-13.6682616989619,
118.231311798525)) ;
#192759=CARTESIAN_POINT('Ctrl Pts',(-7.43691281109367,-13.6682616677135,
118.207080749626)) ;
#192760=CARTESIAN_POINT('Ctrl Pts',(-7.46006094552524,-13.6523296523906,
118.277586231545)) ;
#192761=CARTESIAN_POINT('Ctrl Pts',(-7.48069545348148,-13.9253061411165,
118.375831770847)) ;
#192762=CARTESIAN_POINT('Ctrl Pts',(-7.50170537191064,-13.8902899618178,
118.439824591971)) ;
#192763=CARTESIAN_POINT('Ctrl Pts',(-7.42790153228325,-13.8902899830873,
118.464055645208)) ;
#192764=CARTESIAN_POINT('Ctrl Pts',(-7.35409769265585,-13.8902900043567,
118.488286698446)) ;
#192765=CARTESIAN_POINT('Ctrl Pts',(-7.3330877742267,-13.9253061836553,
118.424293877322)) ;
#192766=CARTESIAN_POINT('Ctrl Pts',(-7.31207785579753,-13.960322362954,
118.360301056197)) ;
#192767=CARTESIAN_POINT('Ctrl Pts',(-7.38588169542493,-13.9603223416845,
118.33607000296)) ;
#192768=CARTESIAN_POINT('Ctrl Pts',(-7.45968553505234,-13.9603223204151,
118.311838949722)) ;
#192769=CARTESIAN_POINT('Ctrl Pts',(-7.48069545348148,-13.9253061411165,
118.375831770847)) ;
#192770=CARTESIAN_POINT('Ctrl Pts',(-7.52318773450401,-14.1634851116196,
118.540904235974)) ;
#192771=CARTESIAN_POINT('Ctrl Pts',(-7.54052484427258,-14.1117847123966,
118.593710274701)) ;
#192772=CARTESIAN_POINT('Ctrl Pts',(-7.46672100428935,-14.1117847230889,
118.617941326854)) ;
#192773=CARTESIAN_POINT('Ctrl Pts',(-7.39291716430611,-14.1117847337813,
118.642172379008)) ;
#192774=CARTESIAN_POINT('Ctrl Pts',(-7.37558005453754,-14.1634851330044,
118.589366340281)) ;
#192775=CARTESIAN_POINT('Ctrl Pts',(-7.35824294476899,-14.2151855322274,
118.536560301554)) ;
#192776=CARTESIAN_POINT('Ctrl Pts',(-7.43204678475222,-14.215185521535,
118.512329249401)) ;
#192777=CARTESIAN_POINT('Ctrl Pts',(-7.50585062473544,-14.2151855108427,
118.488098197247)) ;
#192778=CARTESIAN_POINT('Ctrl Pts',(-7.52318773450401,-14.1634851116196,
118.540904235974)) ;
#192779=CARTESIAN_POINT('Ctrl Pts',(-7.58295692722175,-14.3462889334782,
118.758272828896)) ;
#192780=CARTESIAN_POINT('Ctrl Pts',(-7.59541578115089,-14.2817465742021,
118.796220487547)) ;
#192781=CARTESIAN_POINT('Ctrl Pts',(-7.52161194040355,-14.2817465788419,
118.820451537374)) ;
#192782=CARTESIAN_POINT('Ctrl Pts',(-7.44780809965619,-14.2817465834817,
118.8446825872)) ;
#192783=CARTESIAN_POINT('Ctrl Pts',(-7.43534924572705,-14.3462889427578,
118.806734928548)) ;
#192784=CARTESIAN_POINT('Ctrl Pts',(-7.42289039179789,-14.4108313020339,
118.768787269897)) ;
#192785=CARTESIAN_POINT('Ctrl Pts',(-7.49669423254526,-14.4108312973941,
118.74455622007)) ;
#192786=CARTESIAN_POINT('Ctrl Pts',(-7.5704980732926,-14.4108312927542,
118.720325170244)) ;
#192787=CARTESIAN_POINT('Ctrl Pts',(-7.58295692722175,-14.3462889334782,
118.758272828896)) ;
#192788=CARTESIAN_POINT('Ctrl Pts',(-7.65565943967387,-14.463737953108,
119.015219281916)) ;
#192789=CARTESIAN_POINT('Ctrl Pts',(-7.66232572208676,-14.3908972873577,
119.035523702473)) ;
#192790=CARTESIAN_POINT('Ctrl Pts',(-7.58852187983193,-14.3908972879061,
119.059754747708)) ;
#192791=CARTESIAN_POINT('Ctrl Pts',(-7.51471803757708,-14.3908972884545,
119.083985792943)) ;
#192792=CARTESIAN_POINT('Ctrl Pts',(-7.50805175516422,-14.4637379542048,
119.063681372385)) ;
#192793=CARTESIAN_POINT('Ctrl Pts',(-7.50138547275135,-14.5365786199551,
119.043376951828)) ;
#192794=CARTESIAN_POINT('Ctrl Pts',(-7.57518931500617,-14.5365786194067,
119.019145906593)) ;
#192795=CARTESIAN_POINT('Ctrl Pts',(-7.64899315726101,-14.5365786188583,
118.994914861359)) ;
#192796=CARTESIAN_POINT('Ctrl Pts',(-7.65565943967387,-14.463737953108,
119.015219281916)) ;
#192797=CARTESIAN_POINT('Ctrl Pts',(-7.7350979162589,-14.5058926586063,
119.292671656904)) ;
#192798=CARTESIAN_POINT('Ctrl Pts',(-7.73549259249236,-14.4299991748241,
119.293873777041)) ;
#192799=CARTESIAN_POINT('Ctrl Pts',(-7.66168874891406,-14.4299991745337,
119.318104818244)) ;
#192800=CARTESIAN_POINT('Ctrl Pts',(-7.58788490533576,-14.4299991742434,
119.342335859448)) ;
#192801=CARTESIAN_POINT('Ctrl Pts',(-7.5874902291023,-14.5058926580256,
119.341133739311)) ;
#192802=CARTESIAN_POINT('Ctrl Pts',(-7.58709555286883,-14.5817861418077,
119.339931619175)) ;
#192803=CARTESIAN_POINT('Ctrl Pts',(-7.66089939644714,-14.5817861420981,
119.315700577971)) ;
#192804=CARTESIAN_POINT('Ctrl Pts',(-7.73470324002543,-14.5817861423884,
119.291469536767)) ;
#192805=CARTESIAN_POINT('Ctrl Pts',(-7.7350979162589,-14.5058926586063,
119.292671656904)) ;
#192806=CARTESIAN_POINT('Ctrl Pts',(-7.81459046386314,-14.4703114180475,
119.570193330485)) ;
#192807=CARTESIAN_POINT('Ctrl Pts',(-7.80870234557667,-14.3967894542526,
119.552259072284)) ;
#192808=CARTESIAN_POINT('Ctrl Pts',(-7.73489850128906,-14.3967894548516,
119.576490111328)) ;
#192809=CARTESIAN_POINT('Ctrl Pts',(-7.66109465700145,-14.3967894554506,
119.600721150371)) ;
#192810=CARTESIAN_POINT('Ctrl Pts',(-7.6669827752879,-14.4703114192455,
119.618655408572)) ;
#192811=CARTESIAN_POINT('Ctrl Pts',(-7.67287089357435,-14.5438333830403,
119.636589666772)) ;
#192812=CARTESIAN_POINT('Ctrl Pts',(-7.74667473786198,-14.5438333824413,
119.612358627729)) ;
#192813=CARTESIAN_POINT('Ctrl Pts',(-7.82047858214959,-14.5438333818423,
119.588127588686)) ;
#192814=CARTESIAN_POINT('Ctrl Pts',(-7.81459046386314,-14.4703114180475,
119.570193330485)) ;
#192815=CARTESIAN_POINT('Ctrl Pts',(-7.88822750778698,-14.359046732277,
119.83002759752)) ;
#192816=CARTESIAN_POINT('Ctrl Pts',(-7.87645281961665,-14.2931851690986,
119.794163797256)) ;
#192817=CARTESIAN_POINT('Ctrl Pts',(-7.80264897532485,-14.2931851708445,
119.818394836286)) ;
#192818=CARTESIAN_POINT('Ctrl Pts',(-7.72884513103306,-14.2931851725905,
119.842625875317)) ;
#192819=CARTESIAN_POINT('Ctrl Pts',(-7.74061981920339,-14.3590467357689,
119.878489675581)) ;
#192820=CARTESIAN_POINT('Ctrl Pts',(-7.75239450737372,-14.4249082989473,
119.914353475844)) ;
#192821=CARTESIAN_POINT('Ctrl Pts',(-7.82619835166552,-14.4249082972013,
119.890122436814)) ;
#192822=CARTESIAN_POINT('Ctrl Pts',(-7.90000219595731,-14.4249082954554,
119.865891397783)) ;
#192823=CARTESIAN_POINT('Ctrl Pts',(-7.88822750778698,-14.359046732277,
119.83002759752)) ;
#192824=CARTESIAN_POINT('Ctrl Pts',(-7.94951260678091,-14.1801475215603,
120.05219962572)) ;
#192825=CARTESIAN_POINT('Ctrl Pts',(-7.93270627576756,-14.1266811735188,
120.001010253166)) ;
#192826=CARTESIAN_POINT('Ctrl Pts',(-7.8589024321799,-14.1266811744766,
120.025241294341)) ;
#192827=CARTESIAN_POINT('Ctrl Pts',(-7.78509858859223,-14.1266811754344,
120.049472335516)) ;
#192828=CARTESIAN_POINT('Ctrl Pts',(-7.80190491960559,-14.1801475234759,
120.100661708071)) ;
#192829=CARTESIAN_POINT('Ctrl Pts',(-7.81871125061892,-14.2336138715174,
120.151851080625)) ;
#192830=CARTESIAN_POINT('Ctrl Pts',(-7.89251509420659,-14.2336138705596,
120.12762003945)) ;
#192831=CARTESIAN_POINT('Ctrl Pts',(-7.96631893779426,-14.2336138696018,
120.103388998275)) ;
#192832=CARTESIAN_POINT('Ctrl Pts',(-7.94951260678091,-14.1801475215603,
120.05219962572)) ;
#192833=CARTESIAN_POINT('Ctrl Pts',(-7.99329952727136,-13.9475293921824,
120.220946453046)) ;
#192834=CARTESIAN_POINT('Ctrl Pts',(-7.97267903201572,-13.9102276293421,
120.158139751557)) ;
#192835=CARTESIAN_POINT('Ctrl Pts',(-7.89887518906826,-13.9102276274691,
120.182370794682)) ;
#192836=CARTESIAN_POINT('Ctrl Pts',(-7.82507134612079,-13.910227625596,
120.206601837807)) ;
#192837=CARTESIAN_POINT('Ctrl Pts',(-7.84569184137644,-13.9475293884362,
120.269408539297)) ;
#192838=CARTESIAN_POINT('Ctrl Pts',(-7.86631233663205,-13.9848311512765,
120.332215240786)) ;
#192839=CARTESIAN_POINT('Ctrl Pts',(-7.94011617957952,-13.9848311531496,
120.307984197661)) ;
#192840=CARTESIAN_POINT('Ctrl Pts',(-8.01392002252699,-13.9848311550226,
120.283753154536)) ;
#192841=CARTESIAN_POINT('Ctrl Pts',(-7.99329952727136,-13.9475293921824,
120.220946453046)) ;
#192842=CARTESIAN_POINT('Ctrl Pts',(-8.01597054361897,-13.6767289638667,
120.325436166346)) ;
#192843=CARTESIAN_POINT('Ctrl Pts',(-7.99300362757276,-13.6582814319255,
120.255482645625)) ;
#192844=CARTESIAN_POINT('Ctrl Pts',(-7.91919978485194,-13.6582814248753,
120.279713689441)) ;
#192845=CARTESIAN_POINT('Ctrl Pts',(-7.84539594213114,-13.658281417825,
120.303944733256)) ;
#192846=CARTESIAN_POINT('Ctrl Pts',(-7.86836285817735,-13.6767289497662,
120.373898253977)) ;
#192847=CARTESIAN_POINT('Ctrl Pts',(-7.89132977422359,-13.6951764817073,
120.443851774699)) ;
#192848=CARTESIAN_POINT('Ctrl Pts',(-7.96513361694439,-13.6951764887576,
120.419620730883)) ;
#192849=CARTESIAN_POINT('Ctrl Pts',(-8.0389374596652,-13.6951764958078,
120.395389687068)) ;
#192850=CARTESIAN_POINT('Ctrl Pts',(-8.01597054361897,-13.6767289638667,
120.325436166346)) ;
#192851=CARTESIAN_POINT('Ctrl Pts',(-8.01511316564377,-13.3875048973073,
120.358247068628)) ;
#192852=CARTESIAN_POINT('Ctrl Pts',(-7.99143972407433,-13.3892252145517,
120.286141585044)) ;
#192853=CARTESIAN_POINT('Ctrl Pts',(-7.91763588076485,-13.3892252011116,
120.310372627067)) ;
#192854=CARTESIAN_POINT('Ctrl Pts',(-7.84383203745539,-13.3892251876716,
120.334603669089)) ;
#192855=CARTESIAN_POINT('Ctrl Pts',(-7.86750547902483,-13.3875048704272,
120.406709152673)) ;
#192856=CARTESIAN_POINT('Ctrl Pts',(-7.89117892059427,-13.3857845531828,
120.478814636257)) ;
#192857=CARTESIAN_POINT('Ctrl Pts',(-7.96498276390374,-13.3857845666228,
120.454583594235)) ;
#192858=CARTESIAN_POINT('Ctrl Pts',(-8.03878660721323,-13.3857845800629,
120.430352552212)) ;
#192859=CARTESIAN_POINT('Ctrl Pts',(-8.01511316564377,-13.3875048973073,
120.358247068628)) ;
#192860=CARTESIAN_POINT('Ctrl Pts',(-7.98972953882453,-13.0987597443669,
120.316574379657)) ;
#192861=CARTESIAN_POINT('Ctrl Pts',(-7.96705640494142,-13.1206437742592,
120.247515671714)) ;
#192862=CARTESIAN_POINT('Ctrl Pts',(-7.89325255970313,-13.1206437527101,
120.271746707862)) ;
#192863=CARTESIAN_POINT('Ctrl Pts',(-7.81944871446484,-13.120643731161,
120.29597774401)) ;
#192864=CARTESIAN_POINT('Ctrl Pts',(-7.84212184834797,-13.0987597012687,
120.365036451953)) ;
#192865=CARTESIAN_POINT('Ctrl Pts',(-7.86479498223106,-13.0768756713763,
120.434095159895)) ;
#192866=CARTESIAN_POINT('Ctrl Pts',(-7.93859882746936,-13.0768756929254,
120.409864123748)) ;
#192867=CARTESIAN_POINT('Ctrl Pts',(-8.01240267270764,-13.0768757144745,
120.3856330876)) ;
#192868=CARTESIAN_POINT('Ctrl Pts',(-7.98972953882453,-13.0987597443669,
120.316574379657)) ;
#192869=CARTESIAN_POINT('Ctrl Pts',(-7.94136503643611,-12.8352678817982,
120.204599796384)) ;
#192870=CARTESIAN_POINT('Ctrl Pts',(-7.92130486660037,-12.8755807524781,
120.143499755195)) ;
#192871=CARTESIAN_POINT('Ctrl Pts',(-7.84750101846071,-12.8755807274115,
120.167730782505)) ;
#192872=CARTESIAN_POINT('Ctrl Pts',(-7.77369717032104,-12.8755807023449,
120.191961809816)) ;
#192873=CARTESIAN_POINT('Ctrl Pts',(-7.79375734015679,-12.8352678316651,
120.253061851005)) ;
#192874=CARTESIAN_POINT('Ctrl Pts',(-7.81381750999251,-12.7949549609852,
120.314161892194)) ;
#192875=CARTESIAN_POINT('Ctrl Pts',(-7.88762135813219,-12.7949549860518,
120.289930864884)) ;
#192876=CARTESIAN_POINT('Ctrl Pts',(-7.96142520627183,-12.7949550111184,
120.265699837573)) ;
#192877=CARTESIAN_POINT('Ctrl Pts',(-7.94136503643611,-12.8352678817982,
120.204599796384)) ;
#192878=CARTESIAN_POINT('Ctrl Pts',(-7.87242988112024,-12.6124277096966,
120.030091934832)) ;
#192879=CARTESIAN_POINT('Ctrl Pts',(-7.85642008035131,-12.6683576543549,
119.981328664133)) ;
#192880=CARTESIAN_POINT('Ctrl Pts',(-7.78261622841542,-12.6683576284383,
120.005559679881)) ;
#192881=CARTESIAN_POINT('Ctrl Pts',(-7.7088123764795,-12.6683576025217,
120.029790695629)) ;
#192882=CARTESIAN_POINT('Ctrl Pts',(-7.72482217724844,-12.6124276578634,
120.078553966327)) ;
#192883=CARTESIAN_POINT('Ctrl Pts',(-7.74083197801737,-12.5564977132051,
120.127317237025)) ;
#192884=CARTESIAN_POINT('Ctrl Pts',(-7.81463582995329,-12.5564977391217,
120.103086221278)) ;
#192885=CARTESIAN_POINT('Ctrl Pts',(-7.88843968188919,-12.5564977650383,
120.07885520553)) ;
#192886=CARTESIAN_POINT('Ctrl Pts',(-7.87242988112024,-12.6124277096966,
120.030091934832)) ;
#192887=CARTESIAN_POINT('Ctrl Pts',(-7.78683899646572,-12.4469021309738,
119.804959929397)) ;
#192888=CARTESIAN_POINT('Ctrl Pts',(-7.77604602433129,-12.5144700927407,
119.772086276799)) ;
#192889=CARTESIAN_POINT('Ctrl Pts',(-7.70224216784834,-12.5144700706049,
119.796317278697)) ;
#192890=CARTESIAN_POINT('Ctrl Pts',(-7.62843831136542,-12.514470048469,
119.820548280595)) ;
#192891=CARTESIAN_POINT('Ctrl Pts',(-7.63923128349984,-12.4469020867021,
119.853421933193)) ;
#192892=CARTESIAN_POINT('Ctrl Pts',(-7.65002425563427,-12.3793341249352,
119.88629558579)) ;
#192893=CARTESIAN_POINT('Ctrl Pts',(-7.72382811211722,-12.3793341470711,
119.862064583892)) ;
#192894=CARTESIAN_POINT('Ctrl Pts',(-7.79763196860014,-12.3793341692069,
119.837833581994)) ;
#192895=CARTESIAN_POINT('Ctrl Pts',(-7.78683899646572,-12.4469021309738,
119.804959929397)) ;
#192896=CARTESIAN_POINT('Ctrl Pts',(-7.69042550523445,-12.3516623128813,
119.546789981741)) ;
#192897=CARTESIAN_POINT('Ctrl Pts',(-7.68561405170315,-12.425977537866,
119.532135069522)) ;
#192898=CARTESIAN_POINT('Ctrl Pts',(-7.61181019112561,-12.4259775261186,
119.556366058948)) ;
#192899=CARTESIAN_POINT('Ctrl Pts',(-7.53800633054808,-12.4259775143711,
119.580597048375)) ;
#192900=CARTESIAN_POINT('Ctrl Pts',(-7.5428177840794,-12.3516622893864,
119.595251960594)) ;
#192901=CARTESIAN_POINT('Ctrl Pts',(-7.54762923761071,-12.2773470644017,
119.609906872813)) ;
#192902=CARTESIAN_POINT('Ctrl Pts',(-7.62143309818823,-12.2773470761492,
119.585675883387)) ;
#192903=CARTESIAN_POINT('Ctrl Pts',(-7.69523695876578,-12.2773470878966,
119.56144489396)) ;
#192904=CARTESIAN_POINT('Ctrl Pts',(-7.69042550523445,-12.3516623128813,
119.546789981741)) ;
#192905=CARTESIAN_POINT('Ctrl Pts',(-7.58980441319952,-12.3325403630455,
119.275594411463)) ;
#192906=CARTESIAN_POINT('Ctrl Pts',(-7.59128119877771,-12.4082975181779,
119.280092460837)) ;
#192907=CARTESIAN_POINT('Ctrl Pts',(-7.51747733573818,-12.4082975217576,
119.304323442765)) ;
#192908=CARTESIAN_POINT('Ctrl Pts',(-7.44367347269863,-12.4082975253373,
119.328554424693)) ;
#192909=CARTESIAN_POINT('Ctrl Pts',(-7.44219668712044,-12.3325403702048,
119.324056375318)) ;
#192910=CARTESIAN_POINT('Ctrl Pts',(-7.44071990154224,-12.2567832150723,
119.319558325943)) ;
#192911=CARTESIAN_POINT('Ctrl Pts',(-7.51452376458177,-12.2567832114927,
119.295327344016)) ;
#192912=CARTESIAN_POINT('Ctrl Pts',(-7.58832762762131,-12.256783207913,
119.271096362088)) ;
#192913=CARTESIAN_POINT('Ctrl Pts',(-7.58980441319952,-12.3325403630455,
119.275594411463)) ;
#192914=CARTESIAN_POINT('Ctrl Pts',(-7.48997422897821,-12.3912337324793,
119.007116896225)) ;
#192915=CARTESIAN_POINT('Ctrl Pts',(-7.49768665308937,-12.4630030921761,
119.030607694275)) ;
#192916=CARTESIAN_POINT('Ctrl Pts',(-7.42388278832447,-12.4630031154162,
119.054838670948)) ;
#192917=CARTESIAN_POINT('Ctrl Pts',(-7.35007892355954,-12.4630031386562,
119.07906964762)) ;
#192918=CARTESIAN_POINT('Ctrl Pts',(-7.34236649944839,-12.3912337789595,
119.05557884957)) ;
#192919=CARTESIAN_POINT('Ctrl Pts',(-7.33465407533718,-12.3194644192627,
119.03208805152)) ;
#192920=CARTESIAN_POINT('Ctrl Pts',(-7.40845794010213,-12.3194643960226,
119.007857074848)) ;
#192921=CARTESIAN_POINT('Ctrl Pts',(-7.48226180486705,-12.3194643727826,
118.983626098175)) ;
#192922=CARTESIAN_POINT('Ctrl Pts',(-7.48997422897821,-12.3912337324793,
119.007116896225)) ;
#192923=CARTESIAN_POINT('Ctrl Pts',(-7.39875944406223,-12.5231371749147,
118.764667007709)) ;
#192924=CARTESIAN_POINT('Ctrl Pts',(-7.41211941150982,-12.5858011581757,
118.805359311403)) ;
#192925=CARTESIAN_POINT('Ctrl Pts',(-7.33831554770245,-12.5858012027222,
118.829590290992)) ;
#192926=CARTESIAN_POINT('Ctrl Pts',(-7.26451168389508,-12.5858012472688,
118.853821270581)) ;
#192927=CARTESIAN_POINT('Ctrl Pts',(-7.25115171644747,-12.5231372640078,
118.813128966887)) ;
#192928=CARTESIAN_POINT('Ctrl Pts',(-7.23779174899989,-12.4604732807469,
118.772436663194)) ;
#192929=CARTESIAN_POINT('Ctrl Pts',(-7.31159561280726,-12.4604732362004,
118.748205683605)) ;
#192930=CARTESIAN_POINT('Ctrl Pts',(-7.38539947661462,-12.4604731916538,
118.723974704016)) ;
#192931=CARTESIAN_POINT('Ctrl Pts',(-7.39875944406223,-12.5231371749147,
118.764667007709)) ;
#192932=CARTESIAN_POINT('Ctrl Pts',(-7.32109196511771,-12.7192715563506,
118.563578484396)) ;
#192933=CARTESIAN_POINT('Ctrl Pts',(-7.33915980720696,-12.7683330936011,
118.618610214499)) ;
#192934=CARTESIAN_POINT('Ctrl Pts',(-7.26535594639935,-12.7683331592754,
118.642841203224)) ;
#192935=CARTESIAN_POINT('Ctrl Pts',(-7.19155208559172,-12.7683332249497,
118.66707219195)) ;
#192936=CARTESIAN_POINT('Ctrl Pts',(-7.17348424350248,-12.7192716876992,
118.612040461847)) ;
#192937=CARTESIAN_POINT('Ctrl Pts',(-7.15541640141324,-12.6702101504487,
118.557008731744)) ;
#192938=CARTESIAN_POINT('Ctrl Pts',(-7.22922026222085,-12.6702100847745,
118.532777743019)) ;
#192939=CARTESIAN_POINT('Ctrl Pts',(-7.30302412302846,-12.6702100191002,
118.508546754293)) ;
#192940=CARTESIAN_POINT('Ctrl Pts',(-7.32109196511771,-12.7192715563506,
118.563578484396)) ;
#192941=CARTESIAN_POINT('Ctrl Pts',(-7.2620202481857,-12.9657766439547,
118.419157789103)) ;
#192942=CARTESIAN_POINT('Ctrl Pts',(-7.28350399172834,-12.9976995891968,
118.484593803754)) ;
#192943=CARTESIAN_POINT('Ctrl Pts',(-7.20970013616424,-12.9976996732378,
118.508824808451)) ;
#192944=CARTESIAN_POINT('Ctrl Pts',(-7.13589628060013,-12.9976997572788,
118.533055813148)) ;
#192945=CARTESIAN_POINT('Ctrl Pts',(-7.11441253705749,-12.9657768120367,
118.467619798496)) ;
#192946=CARTESIAN_POINT('Ctrl Pts',(-7.09292879351483,-12.9338538667946,
118.402183783844)) ;
#192947=CARTESIAN_POINT('Ctrl Pts',(-7.16673264907895,-12.9338537827536,
118.377952779148)) ;
#192948=CARTESIAN_POINT('Ctrl Pts',(-7.24053650464305,-12.9338536987126,
118.353721774451)) ;
#192949=CARTESIAN_POINT('Ctrl Pts',(-7.2620202481857,-12.9657766439547,
118.419157789103)) ;
#192950=CARTESIAN_POINT('Ctrl Pts',(-7.22513421757712,-13.2450968718509,
118.342353707646)) ;
#192951=CARTESIAN_POINT('Ctrl Pts',(-7.24848915948865,-13.2575654456473,
118.413489090504)) ;
#192952=CARTESIAN_POINT('Ctrl Pts',(-7.17468531110378,-13.2575655425572,
118.437720117068)) ;
#192953=CARTESIAN_POINT('Ctrl Pts',(-7.10088146271888,-13.2575656394672,
118.461951143631)) ;
#192954=CARTESIAN_POINT('Ctrl Pts',(-7.07752652080735,-13.2450970656709,
118.390815760773)) ;
#192955=CARTESIAN_POINT('Ctrl Pts',(-7.05417157889581,-13.2326284918745,
118.319680377915)) ;
#192956=CARTESIAN_POINT('Ctrl Pts',(-7.12797542728071,-13.2326283949646,
118.295449351351)) ;
#192957=CARTESIAN_POINT('Ctrl Pts',(-7.20177927566557,-13.2326282980546,
118.271218324788)) ;
#192958=CARTESIAN_POINT('Ctrl Pts',(-7.22513421757712,-13.2450968718509,
118.342353707646)) ;
#192959=CARTESIAN_POINT('Ctrl Pts',(-7.21230856442975,-13.5349426349563,
118.338600442269)) ;
#192960=CARTESIAN_POINT('Ctrl Pts',(-7.23586232244513,-13.527193346992,
118.410341386832)) ;
#192961=CARTESIAN_POINT('Ctrl Pts',(-7.16205848236148,-13.5271934482019,
118.43457243868)) ;
#192962=CARTESIAN_POINT('Ctrl Pts',(-7.08825464227779,-13.5271935494119,
118.458803490528)) ;
#192963=CARTESIAN_POINT('Ctrl Pts',(-7.06470088426242,-13.5349428373762,
118.387062545964)) ;
#192964=CARTESIAN_POINT('Ctrl Pts',(-7.04114712624704,-13.5426921253405,
118.315321601401)) ;
#192965=CARTESIAN_POINT('Ctrl Pts',(-7.11495096633071,-13.5426920241306,
118.291090549553)) ;
#192966=CARTESIAN_POINT('Ctrl Pts',(-7.18875480641438,-13.5426919229206,
118.266859497706)) ;
#192967=CARTESIAN_POINT('Ctrl Pts',(-7.21230856442975,-13.5349426349563,
118.338600442269)) ;
#192968=CARTESIAN_POINT('Ctrl Pts',(-7.22361844319658,-13.8188180807124,
118.408663003465)) ;
#192969=CARTESIAN_POINT('Ctrl Pts',(-7.24568040056356,-13.791238496166,
118.475860163881)) ;
#192970=CARTESIAN_POINT('Ctrl Pts',(-7.17187656922055,-13.7912385944122,
118.500091242351)) ;
#192971=CARTESIAN_POINT('Ctrl Pts',(-7.09807273787748,-13.7912386926585,
118.524322320821)) ;
#192972=CARTESIAN_POINT('Ctrl Pts',(-7.07601078051048,-13.8188182772049,
118.457125160405)) ;
#192973=CARTESIAN_POINT('Ctrl Pts',(-7.05394882314345,-13.8463978617513,
118.389927999989)) ;
#192974=CARTESIAN_POINT('Ctrl Pts',(-7.12775265448651,-13.846397763505,
118.365696921519)) ;
#192975=CARTESIAN_POINT('Ctrl Pts',(-7.20155648582953,-13.8463976652588,
118.341465843049)) ;
#192976=CARTESIAN_POINT('Ctrl Pts',(-7.22361844319658,-13.8188180807124,
118.408663003465)) ;
#192977=CARTESIAN_POINT('Ctrl Pts',(-7.25761606914801,-14.0726519250138,
118.547677268349)) ;
#192978=CARTESIAN_POINT('Ctrl Pts',(-7.27660315486712,-14.027309972795,
118.605508865817)) ;
#192979=CARTESIAN_POINT('Ctrl Pts',(-7.20279933161886,-14.027310058674,
118.629739968943)) ;
#192980=CARTESIAN_POINT('Ctrl Pts',(-7.12899550837061,-14.027310144553,
118.653971072068)) ;
#192981=CARTESIAN_POINT('Ctrl Pts',(-7.11000842265151,-14.0726520967719,
118.5961394746)) ;
#192982=CARTESIAN_POINT('Ctrl Pts',(-7.09102133693241,-14.1179940489907,
118.538307877132)) ;
#192983=CARTESIAN_POINT('Ctrl Pts',(-7.16482516018067,-14.1179939631117,
118.514076774006)) ;
#192984=CARTESIAN_POINT('Ctrl Pts',(-7.23862898342892,-14.1179938772327,
118.489845670881)) ;
#192985=CARTESIAN_POINT('Ctrl Pts',(-7.25761606914801,-14.0726519250138,
118.547677268349)) ;
#192986=CARTESIAN_POINT('Ctrl Pts',(-7.31074749652634,-14.2790221021537,
118.744844621079)) ;
#192987=CARTESIAN_POINT('Ctrl Pts',(-7.32532187540961,-14.2192053591173,
118.789235825497)) ;
#192988=CARTESIAN_POINT('Ctrl Pts',(-7.25151805873997,-14.2192054253214,
118.81346694866)) ;
#192989=CARTESIAN_POINT('Ctrl Pts',(-7.17771424207032,-14.2192054915256,
118.837698071823)) ;
#192990=CARTESIAN_POINT('Ctrl Pts',(-7.16313986318704,-14.279022234562,
118.793306867405)) ;
#192991=CARTESIAN_POINT('Ctrl Pts',(-7.14856548430374,-14.3388389775984,
118.748915662987)) ;
#192992=CARTESIAN_POINT('Ctrl Pts',(-7.22236930097341,-14.3388389113943,
118.724684539824)) ;
#192993=CARTESIAN_POINT('Ctrl Pts',(-7.29617311764304,-14.3388388451902,
118.700453416661)) ;
#192994=CARTESIAN_POINT('Ctrl Pts',(-7.31074749652634,-14.2790221021537,
118.744844621079)) ;
#192995=CARTESIAN_POINT('Ctrl Pts',(-7.3788953125628,-14.4246999098251,
118.987880383812)) ;
#192996=CARTESIAN_POINT('Ctrl Pts',(-7.38799957408608,-14.3546239086375,
119.015610493352)) ;
#192997=CARTESIAN_POINT('Ctrl Pts',(-7.31419576194719,-14.3546239496232,
119.039841630315)) ;
#192998=CARTESIAN_POINT('Ctrl Pts',(-7.24039194980831,-14.3546239906089,
119.064072767278)) ;
#192999=CARTESIAN_POINT('Ctrl Pts',(-7.23128768828504,-14.4246999917965,
119.036342657738)) ;
#193000=CARTESIAN_POINT('Ctrl Pts',(-7.22218342676176,-14.4947759929842,
119.008612548198)) ;
#193001=CARTESIAN_POINT('Ctrl Pts',(-7.29598723890066,-14.4947759519985,
118.984381411236)) ;
#193002=CARTESIAN_POINT('Ctrl Pts',(-7.36979105103954,-14.4947759110128,
118.960150274273)) ;
#193003=CARTESIAN_POINT('Ctrl Pts',(-7.3788953125628,-14.4246999098251,
118.987880383812)) ;
#193004=CARTESIAN_POINT('Ctrl Pts',(-7.45654115033611,-14.4982101688668,
119.259955705994)) ;
#193005=CARTESIAN_POINT('Ctrl Pts',(-7.45950188374549,-14.4228974545996,
119.268973620183)) ;
#193006=CARTESIAN_POINT('Ctrl Pts',(-7.38569807341447,-14.4228974671485,
119.293204762652)) ;
#193007=CARTESIAN_POINT('Ctrl Pts',(-7.31189426308347,-14.4228974796974,
119.317435905121)) ;
#193008=CARTESIAN_POINT('Ctrl Pts',(-7.30893352967411,-14.4982101939646,
119.308417990932)) ;
#193009=CARTESIAN_POINT('Ctrl Pts',(-7.30597279626475,-14.5735229082318,
119.299400076744)) ;
#193010=CARTESIAN_POINT('Ctrl Pts',(-7.37977660659575,-14.5735228956829,
119.275168934274)) ;
#193011=CARTESIAN_POINT('Ctrl Pts',(-7.45358041692675,-14.573522883134,
119.250937791805)) ;
#193012=CARTESIAN_POINT('Ctrl Pts',(-7.45654115033611,-14.4982101688668,
119.259955705994)) ;
#193013=CARTESIAN_POINT('Ctrl Pts',(-7.53681769059801,-14.4940193671701,
119.539912255601)) ;
#193014=CARTESIAN_POINT('Ctrl Pts',(-7.53344471814759,-14.4188869609571,
119.529638723729)) ;
#193015=CARTESIAN_POINT('Ctrl Pts',(-7.45964090689752,-14.4188869452096,
119.553869863399)) ;
#193016=CARTESIAN_POINT('Ctrl Pts',(-7.38583709564743,-14.4188869294622,
119.578101003069)) ;
#193017=CARTESIAN_POINT('Ctrl Pts',(-7.38921006809786,-14.4940193356751,
119.588374534941)) ;
#193018=CARTESIAN_POINT('Ctrl Pts',(-7.39258304054826,-14.5691517418881,
119.598648066814)) ;
#193019=CARTESIAN_POINT('Ctrl Pts',(-7.46638685179835,-14.5691517576355,
119.574416927144)) ;
#193020=CARTESIAN_POINT('Ctrl Pts',(-7.54019066304844,-14.569151773383,
119.550185787474)) ;
#193021=CARTESIAN_POINT('Ctrl Pts',(-7.53681769059801,-14.4940193671701,
119.539912255601)) ;
#193022=CARTESIAN_POINT('Ctrl Pts',(-7.61359015495078,-14.4126640845972,
119.809245865358)) ;
#193023=CARTESIAN_POINT('Ctrl Pts',(-7.6041176047322,-14.3430991702555,
119.780394003839)) ;
#193024=CARTESIAN_POINT('Ctrl Pts',(-7.53031378994821,-14.3430991291711,
119.804625132746)) ;
#193025=CARTESIAN_POINT('Ctrl Pts',(-7.45650997516426,-14.3430990880866,
119.828856261652)) ;
#193026=CARTESIAN_POINT('Ctrl Pts',(-7.46598252538283,-14.4126640024283,
119.857708123171)) ;
#193027=CARTESIAN_POINT('Ctrl Pts',(-7.47545507560144,-14.48222891677,119.886559984689)) ;
#193028=CARTESIAN_POINT('Ctrl Pts',(-7.54925889038541,-14.4822289578544,
119.862328855783)) ;
#193029=CARTESIAN_POINT('Ctrl Pts',(-7.62306270516939,-14.4822289989389,
119.838097726877)) ;
#193030=CARTESIAN_POINT('Ctrl Pts',(-7.61359015495078,-14.4126640845972,
119.809245865358)) ;
#193031=CARTESIAN_POINT('Ctrl Pts',(-7.68028577616197,-14.2606219622614,
120.047758542915)) ;
#193032=CARTESIAN_POINT('Ctrl Pts',(-7.66541066509042,-14.2015682240357,
120.002451352817)) ;
#193033=CARTESIAN_POINT('Ctrl Pts',(-7.59160684489074,-14.2015681626728,
120.026682465228)) ;
#193034=CARTESIAN_POINT('Ctrl Pts',(-7.51780302469103,-14.2015681013099,
120.050913577639)) ;
#193035=CARTESIAN_POINT('Ctrl Pts',(-7.53267813576259,-14.2606218395355,
120.096220767737)) ;
#193036=CARTESIAN_POINT('Ctrl Pts',(-7.54755324683412,-14.3196755777612,
120.141527957835)) ;
#193037=CARTESIAN_POINT('Ctrl Pts',(-7.62135706703383,-14.3196756391241,
120.117296845424)) ;
#193038=CARTESIAN_POINT('Ctrl Pts',(-7.6951608872335,-14.319675700487,120.093065733013)) ;
#193039=CARTESIAN_POINT('Ctrl Pts',(-7.68028577616197,-14.2606219622614,
120.047758542915)) ;
#193040=CARTESIAN_POINT('Ctrl Pts',(-7.7318882296266,-14.047641669402,120.240446930669)) ;
#193041=CARTESIAN_POINT('Ctrl Pts',(-7.71265306933839,-14.003368790847,
120.181859734261)) ;
#193042=CARTESIAN_POINT('Ctrl Pts',(-7.63884924213539,-14.0033687165429,
120.206090825341)) ;
#193043=CARTESIAN_POINT('Ctrl Pts',(-7.56504541493244,-14.0033686422388,
120.230321916421)) ;
#193044=CARTESIAN_POINT('Ctrl Pts',(-7.58428057522066,-14.0476415207938,
120.28890911283)) ;
#193045=CARTESIAN_POINT('Ctrl Pts',(-7.60351573550891,-14.0919143993488,
120.347496309238)) ;
#193046=CARTESIAN_POINT('Ctrl Pts',(-7.67731956271188,-14.0919144736529,
120.323265218158)) ;
#193047=CARTESIAN_POINT('Ctrl Pts',(-7.75112338991485,-14.0919145479569,
120.299034127078)) ;
#193048=CARTESIAN_POINT('Ctrl Pts',(-7.7318882296266,-14.047641669402,120.240446930669)) ;
#193049=CARTESIAN_POINT('Ctrl Pts',(-7.76358715017083,-13.7890886844739,
120.37254159039)) ;
#193050=CARTESIAN_POINT('Ctrl Pts',(-7.74137425025259,-13.7628006589206,
120.304884679662)) ;
#193051=CARTESIAN_POINT('Ctrl Pts',(-7.6675704155426,-13.7628005801191,
120.329115747877)) ;
#193052=CARTESIAN_POINT('Ctrl Pts',(-7.59376658083258,-13.7628005013175,
120.353346816092)) ;
#193053=CARTESIAN_POINT('Ctrl Pts',(-7.61597948075081,-13.7890885268708,
120.42100372682)) ;
#193054=CARTESIAN_POINT('Ctrl Pts',(-7.63819238066901,-13.8153765524241,
120.488660637548)) ;
#193055=CARTESIAN_POINT('Ctrl Pts',(-7.71199621537903,-13.8153766312257,
120.464429569334)) ;
#193056=CARTESIAN_POINT('Ctrl Pts',(-7.78580005008903,-13.8153767100272,
120.440198501119)) ;
#193057=CARTESIAN_POINT('Ctrl Pts',(-7.76358715017083,-13.7890886844739,
120.37254159039)) ;
#193058=CARTESIAN_POINT('Ctrl Pts',(-7.77233151699431,-13.5048564724281,
120.434599900892)) ;
#193059=CARTESIAN_POINT('Ctrl Pts',(-7.7487415484172,-13.4983736613525,
120.362748661352)) ;
#193060=CARTESIAN_POINT('Ctrl Pts',(-7.67493770671943,-13.4983735848724,
120.386979708283)) ;
#193061=CARTESIAN_POINT('Ctrl Pts',(-7.60113386502165,-13.4983735083923,
120.411210755214)) ;
#193062=CARTESIAN_POINT('Ctrl Pts',(-7.62472383359876,-13.5048563194679,
120.483061994755)) ;
#193063=CARTESIAN_POINT('Ctrl Pts',(-7.64831380217588,-13.5113391305435,
120.554913234296)) ;
#193064=CARTESIAN_POINT('Ctrl Pts',(-7.72211764387365,-13.5113392070236,
120.530682187364)) ;
#193065=CARTESIAN_POINT('Ctrl Pts',(-7.79592148557143,-13.5113392835037,
120.506451140433)) ;
#193066=CARTESIAN_POINT('Ctrl Pts',(-7.77233151699431,-13.5048564724281,
120.434599900892)) ;
#193067=CARTESIAN_POINT('Ctrl Pts',(-7.75695691433069,-13.2147190164361,
120.42316254752)) ;
#193068=CARTESIAN_POINT('Ctrl Pts',(-7.73367243907768,-13.2284837281292,
120.352241791491)) ;
#193069=CARTESIAN_POINT('Ctrl Pts',(-7.65986859140231,-13.2284836599234,
120.376472820216)) ;
#193070=CARTESIAN_POINT('Ctrl Pts',(-7.58606474372696,-13.2284835917175,
120.40070384894)) ;
#193071=CARTESIAN_POINT('Ctrl Pts',(-7.60934921897998,-13.2147188800244,
120.471624604969)) ;
#193072=CARTESIAN_POINT('Ctrl Pts',(-7.63263369423298,-13.2009541683313,
120.542545360997)) ;
#193073=CARTESIAN_POINT('Ctrl Pts',(-7.70643754190834,-13.2009542365372,
120.518314332273)) ;
#193074=CARTESIAN_POINT('Ctrl Pts',(-7.7802413895837,-13.200954304743,120.494083303548)) ;
#193075=CARTESIAN_POINT('Ctrl Pts',(-7.75695691433069,-13.2147190164361,
120.42316254752)) ;
#193076=CARTESIAN_POINT('Ctrl Pts',(-7.71767702013797,-12.9381997507725,
120.339020142556)) ;
#193077=CARTESIAN_POINT('Ctrl Pts',(-7.69636520807471,-12.9712919342548,
120.27410780048)) ;
#193078=CARTESIAN_POINT('Ctrl Pts',(-7.62256135601241,-12.9712918799021,
120.298338815843)) ;
#193079=CARTESIAN_POINT('Ctrl Pts',(-7.5487575039501,-12.9712918255494,
120.322569831205)) ;
#193080=CARTESIAN_POINT('Ctrl Pts',(-7.5700693160134,-12.9381996420671,
120.387482173282)) ;
#193081=CARTESIAN_POINT('Ctrl Pts',(-7.59138112807666,-12.9051074585849,
120.452394515358)) ;
#193082=CARTESIAN_POINT('Ctrl Pts',(-7.66518498013894,-12.9051075129375,
120.428163499995)) ;
#193083=CARTESIAN_POINT('Ctrl Pts',(-7.73898883220124,-12.9051075672902,
120.403932484633)) ;
#193084=CARTESIAN_POINT('Ctrl Pts',(-7.71767702013797,-12.9381997507725,
120.339020142556)) ;
#193085=CARTESIAN_POINT('Ctrl Pts',(-7.65626840330517,-12.695688487741,
120.187572939771)) ;
#193086=CARTESIAN_POINT('Ctrl Pts',(-7.63847525050966,-12.745763523541,
120.133377866284)) ;
#193087=CARTESIAN_POINT('Ctrl Pts',(-7.56467139637205,-12.7457634857973,
120.157608875326)) ;
#193088=CARTESIAN_POINT('Ctrl Pts',(-7.49086754223442,-12.7457634480537,
120.181839884368)) ;
#193089=CARTESIAN_POINT('Ctrl Pts',(-7.50866069502992,-12.6956884122536,
120.236034957854)) ;
#193090=CARTESIAN_POINT('Ctrl Pts',(-7.5264538478254,-12.6456133764535,
120.29023003134)) ;
#193091=CARTESIAN_POINT('Ctrl Pts',(-7.60025770196303,-12.6456134141972,
120.265999022298)) ;
#193092=CARTESIAN_POINT('Ctrl Pts',(-7.67406155610066,-12.6456134519409,
120.241768013257)) ;
#193093=CARTESIAN_POINT('Ctrl Pts',(-7.65626840330517,-12.695688487741,
120.187572939771)) ;
#193094=CARTESIAN_POINT('Ctrl Pts',(-7.57742636721781,-12.5067830863174,
119.982680330359)) ;
#193095=CARTESIAN_POINT('Ctrl Pts',(-7.56438187186315,-12.5701233290617,
119.942948901362)) ;
#193096=CARTESIAN_POINT('Ctrl Pts',(-7.49057801659502,-12.5701233053132,
119.96717990696)) ;
#193097=CARTESIAN_POINT('Ctrl Pts',(-7.41677416132687,-12.5701232815646,
119.991410912558)) ;
#193098=CARTESIAN_POINT('Ctrl Pts',(-7.42981865668153,-12.5067830388203,
120.031142341556)) ;
#193099=CARTESIAN_POINT('Ctrl Pts',(-7.4428631520362,-12.443442796076,120.070873770554)) ;
#193100=CARTESIAN_POINT('Ctrl Pts',(-7.51666700730434,-12.4434428198246,
120.046642764955)) ;
#193101=CARTESIAN_POINT('Ctrl Pts',(-7.59047086257249,-12.4434428435731,
120.022411759357)) ;
#193102=CARTESIAN_POINT('Ctrl Pts',(-7.57742636721781,-12.5067830863174,
119.982680330359)) ;
#193103=CARTESIAN_POINT('Ctrl Pts',(-7.48481654092851,-12.3815987000844,
119.736103835712)) ;
#193104=CARTESIAN_POINT('Ctrl Pts',(-7.47748391483476,-12.4537757553205,
119.713769839082)) ;
#193105=CARTESIAN_POINT('Ctrl Pts',(-7.40368006110229,-12.4537757450517,
119.738000849357)) ;
#193106=CARTESIAN_POINT('Ctrl Pts',(-7.32987620736981,-12.453775734783,
119.762231859633)) ;
#193107=CARTESIAN_POINT('Ctrl Pts',(-7.33720883346358,-12.3815986795469,
119.784565856264)) ;
#193108=CARTESIAN_POINT('Ctrl Pts',(-7.34454145955733,-12.3094216243108,
119.806899852894)) ;
#193109=CARTESIAN_POINT('Ctrl Pts',(-7.41834531328979,-12.3094216345796,
119.782668842618)) ;
#193110=CARTESIAN_POINT('Ctrl Pts',(-7.49214916702227,-12.3094216448483,
119.758437832343)) ;
#193111=CARTESIAN_POINT('Ctrl Pts',(-7.48481654092851,-12.3815987000844,
119.736103835712)) ;
#193112=CARTESIAN_POINT('Ctrl Pts',(-7.38482566750453,-12.3308693682488,
119.467020622765)) ;
#193113=CARTESIAN_POINT('Ctrl Pts',(-7.3837295176536,-12.4066980840519,
119.463681926591)) ;
#193114=CARTESIAN_POINT('Ctrl Pts',(-7.30992566488976,-12.4066980849149,
119.487912939817)) ;
#193115=CARTESIAN_POINT('Ctrl Pts',(-7.2361218121259,-12.4066980857778,
119.512143953043)) ;
#193116=CARTESIAN_POINT('Ctrl Pts',(-7.23721796197683,-12.3308693699746,
119.515482649216)) ;
#193117=CARTESIAN_POINT('Ctrl Pts',(-7.23831411182774,-12.2550406541715,
119.51882134539)) ;
#193118=CARTESIAN_POINT('Ctrl Pts',(-7.3121179645916,-12.2550406533085,
119.494590332164)) ;
#193119=CARTESIAN_POINT('Ctrl Pts',(-7.38592181735545,-12.2550406524456,
119.470359318938)) ;
#193120=CARTESIAN_POINT('Ctrl Pts',(-7.38482566750453,-12.3308693682488,
119.467020622765)) ;
#193121=CARTESIAN_POINT('Ctrl Pts',(-7.28361307124184,-12.3583046491224,
119.194307222016)) ;
#193122=CARTESIAN_POINT('Ctrl Pts',(-7.28884656543599,-12.4323324318187,
119.210247600737)) ;
#193123=CARTESIAN_POINT('Ctrl Pts',(-7.21504271877939,-12.4323324320423,
119.234478632564)) ;
#193124=CARTESIAN_POINT('Ctrl Pts',(-7.14123887212279,-12.4323324322659,
119.258709664392)) ;
#193125=CARTESIAN_POINT('Ctrl Pts',(-7.13600537792864,-12.3583046495696,
119.242769285671)) ;
#193126=CARTESIAN_POINT('Ctrl Pts',(-7.13077188373449,-12.2842768668734,
119.226828906951)) ;
#193127=CARTESIAN_POINT('Ctrl Pts',(-7.20457573039108,-12.2842768666498,
119.202597875123)) ;
#193128=CARTESIAN_POINT('Ctrl Pts',(-7.27837957704766,-12.2842768664262,
119.178366843295)) ;
#193129=CARTESIAN_POINT('Ctrl Pts',(-7.28361307124184,-12.3583046491224,
119.194307222016)) ;
#193130=CARTESIAN_POINT('Ctrl Pts',(-7.18835949562826,-12.4612718878677,
118.939567373986)) ;
#193131=CARTESIAN_POINT('Ctrl Pts',(-7.19951931791275,-12.5282228863583,
118.973558391361)) ;
#193132=CARTESIAN_POINT('Ctrl Pts',(-7.12571546644994,-12.5282229072686,
118.99778940855)) ;
#193133=CARTESIAN_POINT('Ctrl Pts',(-7.05191161498712,-12.5282229281789,
119.022020425739)) ;
#193134=CARTESIAN_POINT('Ctrl Pts',(-7.04075179270263,-12.4612719296883,
118.988029408363)) ;
#193135=CARTESIAN_POINT('Ctrl Pts',(-7.02959197041813,-12.3943209311977,
118.954038390988)) ;
#193136=CARTESIAN_POINT('Ctrl Pts',(-7.10339582188094,-12.3943209102874,
118.929807373799)) ;
#193137=CARTESIAN_POINT('Ctrl Pts',(-7.17719967334377,-12.3943208893771,
118.90557635661)) ;
#193138=CARTESIAN_POINT('Ctrl Pts',(-7.18835949562826,-12.4612718878677,
118.939567373986)) ;
#193139=CARTESIAN_POINT('Ctrl Pts',(-7.10418260554018,-12.6338543702633,
118.718793259027)) ;
#193140=CARTESIAN_POINT('Ctrl Pts',(-7.12050081610633,-12.6888516916321,
118.768495896363)) ;
#193141=CARTESIAN_POINT('Ctrl Pts',(-7.04669698043341,-12.6888516559685,
118.792726961645)) ;
#193142=CARTESIAN_POINT('Ctrl Pts',(-6.97289314476051,-12.6888516203049,
118.816958026928)) ;
#193143=CARTESIAN_POINT('Ctrl Pts',(-6.95657493419437,-12.6338542989361,
118.767255389592)) ;
#193144=CARTESIAN_POINT('Ctrl Pts',(-6.94025672362824,-12.5788569775673,
118.717552752256)) ;
#193145=CARTESIAN_POINT('Ctrl Pts',(-7.01406055930115,-12.5788570132309,
118.693321686974)) ;
#193146=CARTESIAN_POINT('Ctrl Pts',(-7.08786439497406,-12.5788570488945,
118.669090621691)) ;
#193147=CARTESIAN_POINT('Ctrl Pts',(-7.10418260554018,-12.6338543702633,
118.718793259027)) ;
#193148=CARTESIAN_POINT('Ctrl Pts',(-7.0375316550567,-12.8606317098419,
118.5510569042)) ;
#193149=CARTESIAN_POINT('Ctrl Pts',(-7.0577969319441,-12.8998873118664,
118.612781665881)) ;
#193150=CARTESIAN_POINT('Ctrl Pts',(-6.98399307643361,-12.8998874003437,
118.637012670741)) ;
#193151=CARTESIAN_POINT('Ctrl Pts',(-6.9101892209231,-12.8998874888211,
118.661243675601)) ;
#193152=CARTESIAN_POINT('Ctrl Pts',(-6.88992394403571,-12.8606318867965,
118.599518913921)) ;
#193153=CARTESIAN_POINT('Ctrl Pts',(-6.86965866714829,-12.821376284772,
118.53779415224)) ;
#193154=CARTESIAN_POINT('Ctrl Pts',(-6.94346252265879,-12.8213761962946,
118.51356314738)) ;
#193155=CARTESIAN_POINT('Ctrl Pts',(-7.0172663781693,-12.8213761078173,
118.48933214252)) ;
#193156=CARTESIAN_POINT('Ctrl Pts',(-7.0375316550567,-12.8606317098419,
118.5510569042)) ;
#193157=CARTESIAN_POINT('Ctrl Pts',(-6.99116353791501,-13.129518595729,
118.445436488303)) ;
#193158=CARTESIAN_POINT('Ctrl Pts',(-7.01396188878876,-13.1500300138352,
118.514876590014)) ;
#193159=CARTESIAN_POINT('Ctrl Pts',(-6.94015805847674,-13.1500298440004,
118.539107671625)) ;
#193160=CARTESIAN_POINT('Ctrl Pts',(-6.86635422816467,-13.1500296741656,
118.563338753236)) ;
#193161=CARTESIAN_POINT('Ctrl Pts',(-6.84355587729091,-13.1295182560594,
118.493898651524)) ;
#193162=CARTESIAN_POINT('Ctrl Pts',(-6.82075752641711,-13.1090068379532,
118.424458549812)) ;
#193163=CARTESIAN_POINT('Ctrl Pts',(-6.89456135672918,-13.109007007788,
118.400227468202)) ;
#193164=CARTESIAN_POINT('Ctrl Pts',(-6.96836518704121,-13.1090071776228,
118.375996386591)) ;
#193165=CARTESIAN_POINT('Ctrl Pts',(-6.99116353791501,-13.129518595729,
118.445436488303)) ;
#193166=CARTESIAN_POINT('Ctrl Pts',(-6.97612463268656,-13.3215354698077,
118.423228166981)) ;
#193167=CARTESIAN_POINT('Ctrl Pts',(-6.99950616509918,-13.3286998701254,
118.494444538894)) ;
#193168=CARTESIAN_POINT('Ctrl Pts',(-6.92570231417953,-13.3287000326328,
118.518675557737)) ;
#193169=CARTESIAN_POINT('Ctrl Pts',(-6.85189846325988,-13.3287001951402,
118.54290657658)) ;
#193170=CARTESIAN_POINT('Ctrl Pts',(-6.82851693084728,-13.3215357948224,
118.471690204667)) ;
#193171=CARTESIAN_POINT('Ctrl Pts',(-6.80513539843466,-13.3143713945047,
118.400473832754)) ;
#193172=CARTESIAN_POINT('Ctrl Pts',(-6.87893924935431,-13.3143712319973,
118.376242813911)) ;
#193173=CARTESIAN_POINT('Ctrl Pts',(-6.95274310027397,-13.31437106949,118.352011795068)) ;
#193174=CARTESIAN_POINT('Ctrl Pts',(-6.97612463268656,-13.3215354698077,
118.423228166981)) ;
#193175=CARTESIAN_POINT('Ctrl Pts',(-6.97260578432847,-13.4175644257172,
118.424310057455)) ;
#193176=CARTESIAN_POINT('Ctrl Pts',(-6.9960004985664,-13.4180062659798,
118.495566580825)) ;
#193177=CARTESIAN_POINT('Ctrl Pts',(-6.92219665515706,-13.4180063413679,
118.519797622544)) ;
#193178=CARTESIAN_POINT('Ctrl Pts',(-6.8483928117477,-13.4180064167561,
118.544028664262)) ;
#193179=CARTESIAN_POINT('Ctrl Pts',(-6.82499809750977,-13.4175645764935,
118.472772140891)) ;
#193180=CARTESIAN_POINT('Ctrl Pts',(-6.80160338327183,-13.4171227362309,
118.40151561752)) ;
#193181=CARTESIAN_POINT('Ctrl Pts',(-6.87540722668119,-13.4171226608428,
118.377284575802)) ;
#193182=CARTESIAN_POINT('Ctrl Pts',(-6.94921107009053,-13.4171225854547,
118.353053534084)) ;
#193183=CARTESIAN_POINT('Ctrl Pts',(-6.97260578432847,-13.4175644257172,
118.424310057455)) ;
#193184=CARTESIAN_POINT('',(-18.0519478151656,-12.9727494438644,116.948041367699)) ;
#193185=CARTESIAN_POINT('Ctrl Pts',(-18.0519478151656,-12.9727494438644,
116.948041367699)) ;
#193186=CARTESIAN_POINT('Ctrl Pts',(-18.0518351564328,-12.972911356665,
116.947698227376)) ;
#193187=CARTESIAN_POINT('Ctrl Pts',(-18.0517398746792,-12.9731380019778,
116.947408014528)) ;
#193188=CARTESIAN_POINT('Ctrl Pts',(-18.051557848478,-12.9737505696884,
116.946853592089)) ;
#193189=CARTESIAN_POINT('Ctrl Pts',(-18.0514805222992,-12.9741371839328,
116.946618069025)) ;
#193190=CARTESIAN_POINT('Ctrl Pts',(-18.0512622202171,-12.9755496760429,
116.945953156106)) ;
#193191=CARTESIAN_POINT('Ctrl Pts',(-18.0511751709774,-12.97682332725,116.945688018167)) ;
#193192=CARTESIAN_POINT('Ctrl Pts',(-18.0510064245869,-12.9812525255352,
116.945174043889)) ;
#193193=CARTESIAN_POINT('Ctrl Pts',(-18.0510736978366,-12.985581022285,
116.945378947353)) ;
#193194=CARTESIAN_POINT('Ctrl Pts',(-18.0517201914724,-13.002503579703,
116.947348062656)) ;
#193195=CARTESIAN_POINT('Ctrl Pts',(-18.0528587996904,-13.0192459488949,
116.950816079578)) ;
#193196=CARTESIAN_POINT('Ctrl Pts',(-18.0577446071666,-13.0885454351125,
116.965697460829)) ;
#193197=CARTESIAN_POINT('Ctrl Pts',(-18.0628205806372,-13.1573238043938,
116.981158057011)) ;
#193198=CARTESIAN_POINT('Ctrl Pts',(-18.070265376874,-13.3846429728194,
117.003833705135)) ;
#193199=CARTESIAN_POINT('Ctrl Pts',(-18.0664059866463,-13.5028371896565,
116.992078625212)) ;
#193200=CARTESIAN_POINT('Ctrl Pts',(-18.0512043586578,-13.7248060299085,
116.945776919132)) ;
#193201=CARTESIAN_POINT('Ctrl Pts',(-18.0359840744941,-13.842674137476,
116.899418389356)) ;
#193202=CARTESIAN_POINT('Ctrl Pts',(-17.9911943603994,-14.0637456275394,
116.762996147017)) ;
#193203=CARTESIAN_POINT('Ctrl Pts',(-17.9610731268689,-14.1629071646497,
116.671251729724)) ;
#193204=CARTESIAN_POINT('Ctrl Pts',(-17.8991243194425,-14.2984535233359,
116.482565657706)) ;
#193205=CARTESIAN_POINT('Ctrl Pts',(-17.869856325191,-14.3434390384379,
116.393420069521)) ;
#193206=CARTESIAN_POINT('Ctrl Pts',(-17.8089893867879,-14.4029494275453,
116.208029195989)) ;
#193207=CARTESIAN_POINT('Ctrl Pts',(-17.7780240150196,-14.4178650105577,
116.113713669896)) ;
#193208=CARTESIAN_POINT('Ctrl Pts',(-17.7467422306778,-14.4181080983633,
116.018434402088)) ;
#193209=CARTESIAN_POINT('Ctrl Pts',(-17.7467422306778,-14.4181080983633,
116.018434402088)) ;
#193210=CARTESIAN_POINT('Ctrl Pts',(-17.7140007578702,-14.4183625292707,
115.918709158733)) ;
#193211=CARTESIAN_POINT('Ctrl Pts',(-17.68151856153,-14.4025181298829,115.819773629628)) ;
#193212=CARTESIAN_POINT('Ctrl Pts',(-17.6187304295439,-14.3392564455755,
115.628531110426)) ;
#193213=CARTESIAN_POINT('Ctrl Pts',(-17.5887791967788,-14.2916003512295,
115.53730448808)) ;
#193214=CARTESIAN_POINT('Ctrl Pts',(-17.5267705078295,-14.151880704718,
115.348436026605)) ;
#193215=CARTESIAN_POINT('Ctrl Pts',(-17.4969972022272,-14.0512183347572,
115.257751341639)) ;
#193216=CARTESIAN_POINT('Ctrl Pts',(-17.4510294071444,-13.8180971458324,
115.117740854693)) ;
#193217=CARTESIAN_POINT('Ctrl Pts',(-17.4355506602779,-13.6895955424913,
115.070595089804)) ;
#193218=CARTESIAN_POINT('Ctrl Pts',(-17.4187282219778,-13.4061630903328,
115.019356657033)) ;
#193219=CARTESIAN_POINT('Ctrl Pts',(-17.4210961950408,-13.2885837862808,
115.026569120331)) ;
#193220=CARTESIAN_POINT('Ctrl Pts',(-17.4202558521708,-13.2246311944419,
115.024009571538)) ;
#193221=CARTESIAN_POINT('Ctrl Pts',(-17.4200515924295,-13.2164449755186,
115.023387429323)) ;
#193222=CARTESIAN_POINT('Ctrl Pts',(-17.419495435267,-13.2089958125066,
115.021693464342)) ;
#193223=CARTESIAN_POINT('Ctrl Pts',(-17.4193193828814,-13.207197753218,
115.021157237182)) ;
#193224=CARTESIAN_POINT('Ctrl Pts',(-17.4189816481387,-13.205177369771,
115.020128551648)) ;
#193225=CARTESIAN_POINT('Ctrl Pts',(-17.4188544998161,-13.2045590817019,
115.019741278373)) ;
#193226=CARTESIAN_POINT('Ctrl Pts',(-17.4186056718147,-13.203773671671,
115.018983388429)) ;
#193227=CARTESIAN_POINT('Ctrl Pts',(-17.4184997792349,-13.2035184810664,
115.018660856717)) ;
#193228=CARTESIAN_POINT('Ctrl Pts',(-17.4182739978371,-13.2031822301827,
115.017973163009)) ;
#193229=CARTESIAN_POINT('Ctrl Pts',(-17.4181622393295,-13.2030933380482,
115.017632764627)) ;
#193230=CARTESIAN_POINT('Ctrl Pts',(-17.4179050608403,-13.203058589859,
115.016849440444)) ;
#193231=CARTESIAN_POINT('Ctrl Pts',(-17.4177674591844,-13.2031450748712,
115.016430328002)) ;
#193232=CARTESIAN_POINT('Ctrl Pts',(-17.41741777442,-13.2035491479371,115.015365244631)) ;
#193233=CARTESIAN_POINT('Ctrl Pts',(-17.4172111107158,-13.2039870459215,
115.014735780413)) ;
#193234=CARTESIAN_POINT('Ctrl Pts',(-17.4163518420265,-13.2062236928396,
115.012118586628)) ;
#193235=CARTESIAN_POINT('Ctrl Pts',(-17.4156755712042,-13.2094171488092,
115.010058774739)) ;
#193236=CARTESIAN_POINT('Ctrl Pts',(-17.412733790245,-13.2255158773085,
115.001098584593)) ;
#193237=CARTESIAN_POINT('Ctrl Pts',(-17.4096601818318,-13.2522859045867,
114.991736869173)) ;
#193238=CARTESIAN_POINT('Ctrl Pts',(-17.4014133873562,-13.36215960263,114.966618463816)) ;
#193239=CARTESIAN_POINT('Ctrl Pts',(-17.3966396346497,-13.4847220177897,
114.952078383432)) ;
#193240=CARTESIAN_POINT('Ctrl Pts',(-17.4101561115219,-13.7731365150372,
114.993247391109)) ;
#193241=CARTESIAN_POINT('Ctrl Pts',(-17.4252785357613,-13.9063209144051,
115.039307855321)) ;
#193242=CARTESIAN_POINT('Ctrl Pts',(-17.471242209048,-14.1522077768049,
115.179305787941)) ;
#193243=CARTESIAN_POINT('Ctrl Pts',(-17.5023193439156,-14.261499390111,
115.273961726498)) ;
#193244=CARTESIAN_POINT('Ctrl Pts',(-17.5689134939929,-14.4189847550274,
115.476796762707)) ;
#193245=CARTESIAN_POINT('Ctrl Pts',(-17.6022386411003,-14.4742659640219,
115.578299783772)) ;
#193246=CARTESIAN_POINT('Ctrl Pts',(-17.6729310682834,-14.5486809816127,
115.79361751079)) ;
#193247=CARTESIAN_POINT('Ctrl Pts',(-17.7096845119904,-14.5675899683415,
115.905562570207)) ;
#193248=CARTESIAN_POINT('Ctrl Pts',(-17.746742230677,-14.5678329226988,
116.018434402086)) ;
#193249=CARTESIAN_POINT('Ctrl Pts',(-17.746742167295,-14.5678329187858,
116.01843442664)) ;
#193250=CARTESIAN_POINT('Ctrl Pts',(-17.7601895243844,-14.567921082103,
116.05939291695)) ;
#193251=CARTESIAN_POINT('Ctrl Pts',(-17.773650564873,-14.5655508478998,
116.100392846403)) ;
#193252=CARTESIAN_POINT('Ctrl Pts',(-17.787031093405,-14.5607116311535,
116.141147777371)) ;
#193253=CARTESIAN_POINT('Ctrl Pts',(-17.79258814348,-14.5587018622779,116.158073655273)) ;
#193254=CARTESIAN_POINT('Ctrl Pts',(-17.7981318063432,-14.556266107077,
116.174958757887)) ;
#193255=CARTESIAN_POINT('Ctrl Pts',(-17.8036553329622,-14.5534035696439,
116.191782528751)) ;
#193256=CARTESIAN_POINT('Ctrl Pts',(-17.8294913073762,-14.5400142173367,
116.270474738197)) ;
#193257=CARTESIAN_POINT('Ctrl Pts',(-17.8548772100185,-14.5172883204691,
116.347795870618)) ;
#193258=CARTESIAN_POINT('Ctrl Pts',(-17.8791197239657,-14.4859963413062,
116.421634818916)) ;
#193259=CARTESIAN_POINT('Ctrl Pts',(-17.8846519651774,-14.4788553831903,
116.438485170067)) ;
#193260=CARTESIAN_POINT('Ctrl Pts',(-17.890124692269,-14.4712685294595,
116.45515424542)) ;
#193261=CARTESIAN_POINT('Ctrl Pts',(-17.895529724337,-14.463245285136,116.471617101)) ;
#193262=CARTESIAN_POINT('Ctrl Pts',(-17.9197140688182,-14.4273459783168,
116.545278712161)) ;
#193263=CARTESIAN_POINT('Ctrl Pts',(-17.9425421210597,-14.3827067354943,
116.614809758227)) ;
#193264=CARTESIAN_POINT('Ctrl Pts',(-17.9635089553104,-14.3303836683813,
116.678671009225)) ;
#193265=CARTESIAN_POINT('Ctrl Pts',(-17.9677674696046,-14.3197564784796,
116.691641686961)) ;
#193266=CARTESIAN_POINT('Ctrl Pts',(-17.9719492216382,-14.3088124559315,
116.70437855954)) ;
#193267=CARTESIAN_POINT('Ctrl Pts',(-17.9760500025897,-14.2975606758145,
116.716868876659)) ;
#193268=CARTESIAN_POINT('Ctrl Pts',(-17.9948816875145,-14.2458900353894,
116.774227150459)) ;
#193269=CARTESIAN_POINT('Ctrl Pts',(-18.0120038023616,-14.1877300152514,
116.826380183859)) ;
#193270=CARTESIAN_POINT('Ctrl Pts',(-18.0269924392848,-14.1246319652718,
116.872032027455)) ;
#193271=CARTESIAN_POINT('Ctrl Pts',(-18.0313506096886,-14.1062852633422,
116.885305983896)) ;
#193272=CARTESIAN_POINT('Ctrl Pts',(-18.0355284323829,-14.0875212502638,
116.898030577)) ;
#193273=CARTESIAN_POINT('Ctrl Pts',(-18.0395155550469,-14.0683784694332,
116.910174709315)) ;
#193274=CARTESIAN_POINT('Ctrl Pts',(-18.052265981228,-14.0071617388601,
116.949010450189)) ;
#193275=CARTESIAN_POINT('Ctrl Pts',(-18.0630631813206,-13.9420796939719,
116.981902915811)) ;
#193276=CARTESIAN_POINT('Ctrl Pts',(-18.0717325065314,-13.8743660366255,
117.008305304809)) ;
#193277=CARTESIAN_POINT('Ctrl Pts',(-18.0751147082918,-13.8479486113349,
117.018605784301)) ;
#193278=CARTESIAN_POINT('Ctrl Pts',(-18.0781729329666,-13.8211309228485,
117.027918845113)) ;
#193279=CARTESIAN_POINT('Ctrl Pts',(-18.0808963466438,-13.7939873904681,
117.036213923753)) ;
#193280=CARTESIAN_POINT('Ctrl Pts',(-18.0833540191079,-13.7694924293578,
117.043699597535)) ;
#193281=CARTESIAN_POINT('Ctrl Pts',(-18.0855717988214,-13.7443945944633,
117.050454735962)) ;
#193282=CARTESIAN_POINT('Ctrl Pts',(-18.0875136590947,-13.7189305603966,
117.056369343325)) ;
#193283=CARTESIAN_POINT('Ctrl Pts',(-18.0894566273483,-13.6934519971449,
117.062287325424)) ;
#193284=CARTESIAN_POINT('Ctrl Pts',(-18.0911232849302,-13.667607492928,
117.067363606227)) ;
#193285=CARTESIAN_POINT('Ctrl Pts',(-18.0924927843825,-13.641651804631,
117.071534784123)) ;
#193286=CARTESIAN_POINT('Ctrl Pts',(-18.0938629088252,-13.6156842710903,
117.075707865594)) ;
#193287=CARTESIAN_POINT('Ctrl Pts',(-18.0949355652063,-13.5896061785709,
117.078974927764)) ;
#193288=CARTESIAN_POINT('Ctrl Pts',(-18.0957059946265,-13.5636797249849,
117.081321564011)) ;
#193289=CARTESIAN_POINT('Ctrl Pts',(-18.0963885652904,-13.5407098900162,
117.083400592951)) ;
#193290=CARTESIAN_POINT('Ctrl Pts',(-18.0968341419202,-13.5178594986715,
117.084757876611)) ;
#193291=CARTESIAN_POINT('Ctrl Pts',(-18.0970501559553,-13.4953086850252,
117.085415820508)) ;
#193292=CARTESIAN_POINT('Ctrl Pts',(-18.0972343972258,-13.4760747933397,
117.085976989691)) ;
#193293=CARTESIAN_POINT('Ctrl Pts',(-18.0972584721256,-13.4562541583979,
117.086051100861)) ;
#193294=CARTESIAN_POINT('Ctrl Pts',(-18.0970972387754,-13.4361251533928,
117.085560320937)) ;
#193295=CARTESIAN_POINT('Ctrl Pts',(-18.096936270928,-13.4160292948047,
117.08507034918)) ;
#193296=CARTESIAN_POINT('Ctrl Pts',(-18.0965905110925,-13.3956265064346,
117.084017108433)) ;
#193297=CARTESIAN_POINT('Ctrl Pts',(-18.0960511480064,-13.3751969407049,
117.082373828394)) ;
#193298=CARTESIAN_POINT('Ctrl Pts',(-18.0955200215003,-13.3550793535937,
117.080755642782)) ;
#193299=CARTESIAN_POINT('Ctrl Pts',(-18.0948011763854,-13.3349362383173,
117.078565410166)) ;
#193300=CARTESIAN_POINT('Ctrl Pts',(-18.0939024233134,-13.315031695618,
117.075827468671)) ;
#193301=CARTESIAN_POINT('Ctrl Pts',(-18.0929827637773,-13.2946641407518,
117.073025838185)) ;
#193302=CARTESIAN_POINT('Ctrl Pts',(-18.0918747072663,-13.2745468745331,
117.069650725061)) ;
#193303=CARTESIAN_POINT('Ctrl Pts',(-18.0906039399014,-13.2549521381173,
117.065780494704)) ;
#193304=CARTESIAN_POINT('Ctrl Pts',(-18.0893331725365,-13.2353574017014,
117.061910264347)) ;
#193305=CARTESIAN_POINT('Ctrl Pts',(-18.0878998109875,-13.2162855561395,
117.057545346139)) ;
#193306=CARTESIAN_POINT('Ctrl Pts',(-18.0863458477046,-13.1979917937502,
117.05281222471)) ;
#193307=CARTESIAN_POINT('Ctrl Pts',(-18.0852303988916,-13.1848603666647,
117.049414747603)) ;
#193308=CARTESIAN_POINT('Ctrl Pts',(-18.0839869321607,-13.1713626479556,
117.045627555924)) ;
#193309=CARTESIAN_POINT('Ctrl Pts',(-18.0826311641542,-13.1578519278585,
117.041498054669)) ;
#193310=CARTESIAN_POINT('Ctrl Pts',(-18.0812653772353,-13.1442413656633,
117.037338037049)) ;
#193311=CARTESIAN_POINT('Ctrl Pts',(-18.0797855761015,-13.1306181206681,
117.032830587708)) ;
#193312=CARTESIAN_POINT('Ctrl Pts',(-18.0782238294761,-13.1173287413436,
117.028073704578)) ;
#193313=CARTESIAN_POINT('Ctrl Pts',(-18.0766620828508,-13.1040393620192,
117.023316821449)) ;
#193314=CARTESIAN_POINT('Ctrl Pts',(-18.0750184927648,-13.0910842149795,
117.018310929226)) ;
#193315=CARTESIAN_POINT('Ctrl Pts',(-18.0733406173676,-13.078788559479,
117.01320039149)) ;
#193316=CARTESIAN_POINT('Ctrl Pts',(-18.0721098671841,-13.0697694867344,
117.009451725012)) ;
#193317=CARTESIAN_POINT('Ctrl Pts',(-18.0707717001157,-13.0604578336815,
117.005375967919)) ;
#193318=CARTESIAN_POINT('Ctrl Pts',(-18.0693721051686,-13.0513039505984,
117.001112954701)) ;
#193319=CARTESIAN_POINT('Ctrl Pts',(-18.067964052392,-13.0420947500949,
116.99682417986)) ;
#193320=CARTESIAN_POINT('Ctrl Pts',(-18.0664938193825,-13.033045638422,
116.99234609624)) ;
#193321=CARTESIAN_POINT('Ctrl Pts',(-18.0650230520561,-13.0245905007115,
116.987866421264)) ;
#193322=CARTESIAN_POINT('Ctrl Pts',(-18.0648621543254,-13.0236655328759,
116.987376357659)) ;
#193323=CARTESIAN_POINT('Ctrl Pts',(-18.0647012643362,-13.0227476464585,
116.986886316111)) ;
#193324=CARTESIAN_POINT('Ctrl Pts',(-18.0645404729608,-13.0218373893616,
116.986396571525)) ;
#193325=CARTESIAN_POINT('Ctrl Pts',(-18.0634316111312,-13.0155600044732,
116.983019157306)) ;
#193326=CARTESIAN_POINT('Ctrl Pts',(-18.0622287233154,-13.0090948676773,
116.979355343084)) ;
#193327=CARTESIAN_POINT('Ctrl Pts',(-18.0610103124457,-13.0030224151989,
116.975644247746)) ;
#193328=CARTESIAN_POINT('Ctrl Pts',(-18.0604262701594,-13.0001115998758,
116.973865343224)) ;
#193329=CARTESIAN_POINT('Ctrl Pts',(-18.0598388640937,-12.9972905938871,
116.972076229518)) ;
#193330=CARTESIAN_POINT('Ctrl Pts',(-18.059257840653,-12.9946208870877,
116.970306525865)) ;
#193331=CARTESIAN_POINT('Ctrl Pts',(-18.0582667075183,-12.9900667939414,
116.967287694256)) ;
#193332=CARTESIAN_POINT('Ctrl Pts',(-18.0571961007361,-12.9855090222264,
116.964026798739)) ;
#193333=CARTESIAN_POINT('Ctrl Pts',(-18.0561685336678,-12.9817420257543,
116.960896995246)) ;
#193334=CARTESIAN_POINT('Ctrl Pts',(-18.0555646065479,-12.9795280667821,
116.959057530682)) ;
#193335=CARTESIAN_POINT('Ctrl Pts',(-18.0549412511537,-12.977460262646,
116.957158890829)) ;
#193336=CARTESIAN_POINT('Ctrl Pts',(-18.0543480872734,-12.9758473023832,
116.955352209356)) ;
#193337=CARTESIAN_POINT('Ctrl Pts',(-18.0534287572029,-12.9733474150479,
116.952552078295)) ;
#193338=CARTESIAN_POINT('Ctrl Pts',(-18.0525577104548,-12.9718729041419,
116.949899010344)) ;
#193339=CARTESIAN_POINT('Ctrl Pts',(-18.0519478151656,-12.9727494438644,
116.948041367699)) ;
#193340=CARTESIAN_POINT('',(-29.1489187358159,-13.1500241806476,113.370642219953)) ;
#193341=CARTESIAN_POINT('Ctrl Pts',(-29.1489187358159,-13.1500241806476,
113.370642219953)) ;
#193342=CARTESIAN_POINT('Ctrl Pts',(-29.1481908350552,-13.1438552129684,
113.369207785981)) ;
#193343=CARTESIAN_POINT('Ctrl Pts',(-29.1363218176444,-13.045472096163,
113.345565010115)) ;
#193344=CARTESIAN_POINT('Ctrl Pts',(-29.1042713188461,-12.8597742993635,
113.272543581875)) ;
#193345=CARTESIAN_POINT('Ctrl Pts',(-29.0373324850924,-12.6327839415056,
113.104016096402)) ;
#193346=CARTESIAN_POINT('Ctrl Pts',(-28.9535211541043,-12.4610780963096,
112.884187309328)) ;
#193347=CARTESIAN_POINT('Ctrl Pts',(-28.8575946335874,-12.3578311300529,
112.627637093626)) ;
#193348=CARTESIAN_POINT('Ctrl Pts',(-28.7572250300145,-12.3309709098726,
112.357185420699)) ;
#193349=CARTESIAN_POINT('Ctrl Pts',(-28.6569634591251,-12.3817310335918,
112.087380599263)) ;
#193350=CARTESIAN_POINT('Ctrl Pts',(-28.564509082064,-12.5067458714326,
111.841211648264)) ;
#193351=CARTESIAN_POINT('Ctrl Pts',(-28.4851946394043,-12.6971218835384,
111.635119922408)) ;
#193352=CARTESIAN_POINT('Ctrl Pts',(-28.4241475022264,-12.9391053860727,
111.48464558118)) ;
#193353=CARTESIAN_POINT('Ctrl Pts',(-28.3849524033199,-13.2152764852227,
111.400718831589)) ;
#193354=CARTESIAN_POINT('Ctrl Pts',(-28.3695728344553,-13.505784356226,
111.389304759768)) ;
#193355=CARTESIAN_POINT('Ctrl Pts',(-28.3785666018913,-13.7916119971123,
111.452340850324)) ;
#193356=CARTESIAN_POINT('Ctrl Pts',(-28.4102051428863,-14.0480477215918,
111.583997783673)) ;
#193357=CARTESIAN_POINT('Ctrl Pts',(-28.4617096973959,-14.2608003622883,
111.776342484654)) ;
#193358=CARTESIAN_POINT('Ctrl Pts',(-28.5285966908039,-14.4130997833176,
112.015523906653)) ;
#193359=CARTESIAN_POINT('Ctrl Pts',(-28.6055369658778,-14.494276858583,
112.285430331193)) ;
#193360=CARTESIAN_POINT('Ctrl Pts',(-28.6858402113565,-14.4979516536895,
112.565480733191)) ;
#193361=CARTESIAN_POINT('Ctrl Pts',(-28.7630866534358,-14.4245500702158,
112.836167498554)) ;
#193362=CARTESIAN_POINT('Ctrl Pts',(-28.8312032669878,-14.27912481409,113.079082108179)) ;
#193363=CARTESIAN_POINT('Ctrl Pts',(-28.8845697171654,-14.0717728276009,
113.277121444909)) ;
#193364=CARTESIAN_POINT('Ctrl Pts',(-28.9184685925918,-13.8168218187551,
113.415944332688)) ;
#193365=CARTESIAN_POINT('Ctrl Pts',(-28.9296288975394,-13.535324035321,
113.485246560678)) ;
#193366=CARTESIAN_POINT('Ctrl Pts',(-28.9167824586136,-13.2440746292406,
113.481603030049)) ;
#193367=CARTESIAN_POINT('Ctrl Pts',(-28.879724619622,-12.9648031401168,
113.404286512872)) ;
#193368=CARTESIAN_POINT('Ctrl Pts',(-28.8209010350444,-12.7194345507308,
113.260464724787)) ;
#193369=CARTESIAN_POINT('Ctrl Pts',(-28.7430943016509,-12.5228537207888,
113.059023280909)) ;
#193370=CARTESIAN_POINT('Ctrl Pts',(-28.6517657151193,-12.3910219564108,
112.816257416584)) ;
#193371=CARTESIAN_POINT('Ctrl Pts',(-28.5519605561705,-12.3324946198483,
112.547844627311)) ;
#193372=CARTESIAN_POINT('Ctrl Pts',(-28.4511785871551,-12.3517941049946,
112.2762149844)) ;
#193373=CARTESIAN_POINT('Ctrl Pts',(-28.3546167960162,-12.4476532719571,
112.01766426386)) ;
#193374=CARTESIAN_POINT('Ctrl Pts',(-28.2694260224947,-12.6128436094032,
111.793615869469)) ;
#193375=CARTESIAN_POINT('Ctrl Pts',(-28.2004725461681,-12.8354722898284,
111.619033756946)) ;
#193376=CARTESIAN_POINT('Ctrl Pts',(-28.1518872197862,-13.101408894203,
111.506681708968)) ;
#193377=CARTESIAN_POINT('Ctrl Pts',(-28.1269130732857,-13.3874022195482,
111.465903939157)) ;
#193378=CARTESIAN_POINT('Ctrl Pts',(-28.1259581954368,-13.6768759171903,
111.498450514514)) ;
#193379=CARTESIAN_POINT('Ctrl Pts',(-28.1487784107379,-13.948608493865,
111.603521104352)) ;
#193380=CARTESIAN_POINT('Ctrl Pts',(-28.1927422454497,-14.181257681225,
111.772854625694)) ;
#193381=CARTESIAN_POINT('Ctrl Pts',(-28.25389994631,-14.3592650506284,111.994525378914)) ;
#193382=CARTESIAN_POINT('Ctrl Pts',(-28.3273391635443,-14.4703402370834,
112.253666401676)) ;
#193383=CARTESIAN_POINT('Ctrl Pts',(-28.4071790901361,-14.5059089260168,
112.532398419472)) ;
#193384=CARTESIAN_POINT('Ctrl Pts',(-28.4863373455099,-14.4635906108697,
112.808879001028)) ;
#193385=CARTESIAN_POINT('Ctrl Pts',(-28.5590864820887,-14.3462861335646,
113.06597539471)) ;
#193386=CARTESIAN_POINT('Ctrl Pts',(-28.6190888482877,-14.1620807273187,
113.284252795165)) ;
#193387=CARTESIAN_POINT('Ctrl Pts',(-28.6611716634273,-13.9257450561724,
113.447780698845)) ;
#193388=CARTESIAN_POINT('Ctrl Pts',(-28.6819629618819,-13.6518932520307,
113.54663327576)) ;
#193389=CARTESIAN_POINT('Ctrl Pts',(-28.6788957975661,-13.361350209501,
113.572794442411)) ;
#193390=CARTESIAN_POINT('Ctrl Pts',(-28.6515753370969,-13.0754523993138,
113.525017916636)) ;
#193391=CARTESIAN_POINT('Ctrl Pts',(-28.6012644802897,-12.8139381990977,
113.407216883436)) ;
#193392=CARTESIAN_POINT('Ctrl Pts',(-28.530312795938,-12.5948180944483,
113.22672545771)) ;
#193393=CARTESIAN_POINT('Ctrl Pts',(-28.4441820785393,-12.4362800048722,
112.999678378)) ;
#193394=CARTESIAN_POINT('Ctrl Pts',(-28.3470854955192,-12.346922078608,
112.739452029468)) ;
#193395=CARTESIAN_POINT('Ctrl Pts',(-28.2458303935604,-12.3346186385411,
112.466505819017)) ;
#193396=CARTESIAN_POINT('Ctrl Pts',(-28.1468306373285,-12.3998225687949,
112.200422951598)) ;
#193397=CARTESIAN_POINT('Ctrl Pts',(-28.056410402061,-12.5378477500096,
111.960460656517)) ;
#193398=CARTESIAN_POINT('Ctrl Pts',(-27.9801392408926,-12.7392396507352,
111.763656314593)) ;
#193399=CARTESIAN_POINT('Ctrl Pts',(-27.9229728782281,-12.989236405783,
111.625017894805)) ;
#193400=CARTESIAN_POINT('Ctrl Pts',(-27.8882165238537,-13.269049028932,
111.554529970124)) ;
#193401=CARTESIAN_POINT('Ctrl Pts',(-27.8773822820719,-13.560604521515,
111.557039247534)) ;
#193402=CARTESIAN_POINT('Ctrl Pts',(-27.8908274487406,-13.8423158077137,
111.633558215579)) ;
#193403=CARTESIAN_POINT('Ctrl Pts',(-27.9264541508921,-14.0920492190499,
111.777413603601)) ;
#193404=CARTESIAN_POINT('Ctrl Pts',(-27.9814414275838,-14.2950965364046,
111.980481540082)) ;
#193405=CARTESIAN_POINT('Ctrl Pts',(-28.0507461501417,-14.434335219557,
112.227053017501)) ;
#193406=CARTESIAN_POINT('Ctrl Pts',(-28.1282740613558,-14.5007530721094,
112.498487082343)) ;
#193407=CARTESIAN_POINT('Ctrl Pts',(-28.2086863670135,-14.4901437351793,
112.778942561062)) ;
#193408=CARTESIAN_POINT('Ctrl Pts',(-28.2850462508329,-14.402041943339,
113.047107750682)) ;
#193409=CARTESIAN_POINT('Ctrl Pts',(-28.3507008692899,-14.243691286176,
113.282525581938)) ;
#193410=CARTESIAN_POINT('Ctrl Pts',(-28.4004336980104,-14.0272168477211,
113.469327044574)) ;
#193411=CARTESIAN_POINT('Ctrl Pts',(-28.4302808069805,-13.7664028194368,
113.595698173527)) ;
#193412=CARTESIAN_POINT('Ctrl Pts',(-28.4370991249928,-13.4798811075686,
113.652008520853)) ;
#193413=CARTESIAN_POINT('Ctrl Pts',(-28.4194035357479,-13.1885796838075,
113.633702115265)) ;
#193414=CARTESIAN_POINT('Ctrl Pts',(-28.378412477973,-12.9166253502417,
113.544054690634)) ;
#193415=CARTESIAN_POINT('Ctrl Pts',(-28.3154270405176,-12.6775835687805,
113.387804302381)) ;
#193416=CARTESIAN_POINT('Ctrl Pts',(-28.2345655221718,-12.4925681740676,
113.177035535843)) ;
#193417=CARTESIAN_POINT('Ctrl Pts',(-28.1415965309447,-12.3743553948694,
112.929153696932)) ;
#193418=CARTESIAN_POINT('Ctrl Pts',(-28.0408341461004,-12.3300586716913,
112.657878333238)) ;
#193419=CARTESIAN_POINT('Ctrl Pts',(-27.9401092157344,-12.3643855283945,
112.386554127362)) ;
#193420=CARTESIAN_POINT('Ctrl Pts',(-27.8457507930179,-12.4735026256636,
112.134502190906)) ;
#193421=CARTESIAN_POINT('Ctrl Pts',(-27.7630645931825,-12.6505044221707,
111.918129912256)) ;
#193422=CARTESIAN_POINT('Ctrl Pts',(-27.6975343400792,-12.883421947767,
111.754113424243)) ;
#193423=CARTESIAN_POINT('Ctrl Pts',(-27.6534936872668,-13.1527514798463,
111.655293821054)) ;
#193424=CARTESIAN_POINT('Ctrl Pts',(-27.6327547212792,-13.4437023579035,
111.627785242889)) ;
#193425=CARTESIAN_POINT('Ctrl Pts',(-27.6365620199519,-13.7306193771303,
111.674768692016)) ;
#193426=CARTESIAN_POINT('Ctrl Pts',(-27.6633603539813,-13.9949086675026,
111.791717285722)) ;
#193427=CARTESIAN_POINT('Ctrl Pts',(-27.7111136241826,-14.2196906214034,
111.972774236008)) ;
#193428=CARTESIAN_POINT('Ctrl Pts',(-27.7749357041157,-14.3856064052365,
112.20251553552)) ;
#193429=CARTESIAN_POINT('Ctrl Pts',(-27.850139433854,-14.4829720573525,
112.467091440401)) ;
#193430=CARTESIAN_POINT('Ctrl Pts',(-27.9301015626753,-14.5039687036518,
112.746047500903)) ;
#193431=CARTESIAN_POINT('Ctrl Pts',(-28.0091089868232,-14.4466173797893,
113.02236063873)) ;
#193432=CARTESIAN_POINT('Ctrl Pts',(-28.0794461167512,-14.3162716014842,
113.27191318261)) ;
#193433=CARTESIAN_POINT('Ctrl Pts',(-28.1364440614567,-14.1214968775469,
113.480983026046)) ;
#193434=CARTESIAN_POINT('Ctrl Pts',(-28.1749613485906,-13.8749956323593,
113.633913814206)) ;
#193435=CARTESIAN_POINT('Ctrl Pts',(-28.1911734256759,-13.5974682752699,
113.718666176969)) ;
#193436=CARTESIAN_POINT('Ctrl Pts',(-28.1836078259768,-13.3070931499256,
113.731008103206)) ;
#193437=CARTESIAN_POINT('Ctrl Pts',(-28.1517250328214,-13.0233508116479,
113.669448037719)) ;
#193438=CARTESIAN_POINT('Ctrl Pts',(-28.0972991812598,-12.7688607554056,
113.539098836946)) ;
#193439=CARTESIAN_POINT('Ctrl Pts',(-28.0232821783549,-12.5604071436069,
113.349142464811)) ;
#193440=CARTESIAN_POINT('Ctrl Pts',(-27.9344209561679,-12.4137261008746,
113.113916473714)) ;
#193441=CARTESIAN_POINT('Ctrl Pts',(-27.8363120109697,-12.3387040702925,
112.850499990527)) ;
#193442=CARTESIAN_POINT('Ctrl Pts',(-27.7346441044334,-12.3410592400664,
112.576417227786)) ;
#193443=CARTESIAN_POINT('Ctrl Pts',(-27.6369370950116,-12.4205041979803,
112.314216816515)) ;
#193444=CARTESIAN_POINT('Ctrl Pts',(-27.5486712808213,-12.5715202421064,
112.080868685751)) ;
#193445=CARTESIAN_POINT('Ctrl Pts',(-27.4757703775428,-12.7831706996134,
111.894290358998)) ;
#193446=CARTESIAN_POINT('Ctrl Pts',(-27.4226294303003,-13.0400861903177,
111.76787608117)) ;
#193447=CARTESIAN_POINT('Ctrl Pts',(-27.3922395133834,-13.3242719779506,
111.710785133111)) ;
#193448=CARTESIAN_POINT('Ctrl Pts',(-27.3860860135596,-13.6152878377403,
111.727526925979)) ;
#193449=CARTESIAN_POINT('Ctrl Pts',(-27.4038644204004,-13.8920338673762,
111.817147898947)) ;
#193450=CARTESIAN_POINT('Ctrl Pts',(-27.4434672264958,-14.1346381572922,
111.973208058208)) ;
#193451=CARTESIAN_POINT('Ctrl Pts',(-27.5014596989945,-14.3262307223465,
112.185343141529)) ;
#193452=CARTESIAN_POINT('Ctrl Pts',(-27.572610257217,-14.4523301137118,
112.437438559264)) ;
#193453=CARTESIAN_POINT('Ctrl Pts',(-27.6514424913783,-14.5048566464616,
112.713014331691)) ;
#193454=CARTESIAN_POINT('Ctrl Pts',(-27.7316184422369,-14.4792282215674,
112.992772623)) ;
#193455=CARTESIAN_POINT('Ctrl Pts',(-27.8061587870981,-14.3776591931245,
113.255243325012)) ;
#193456=CARTESIAN_POINT('Ctrl Pts',(-27.8693284879629,-14.2073582471136,
113.483114722588)) ;
#193457=CARTESIAN_POINT('Ctrl Pts',(-27.9157562377959,-13.980463190757,
113.659992780597)) ;
#193458=CARTESIAN_POINT('Ctrl Pts',(-27.9413702245525,-13.7134648384933,
113.773453223393)) ;
#193459=CARTESIAN_POINT('Ctrl Pts',(-27.9436004920684,-13.4252028157263,
113.815706568897)) ;
#193460=CARTESIAN_POINT('Ctrl Pts',(-27.9215804554763,-13.136660084581,
113.78406473884)) ;
#193461=CARTESIAN_POINT('Ctrl Pts',(-27.8759261543426,-12.8674128564449,
113.680553643697)) ;
#193462=CARTESIAN_POINT('Ctrl Pts',(-27.8094158631442,-12.6383938778605,
113.513414911382)) ;
#193463=CARTESIAN_POINT('Ctrl Pts',(-27.7259260844217,-12.465038874388,
113.294584641188)) ;
#193464=CARTESIAN_POINT('Ctrl Pts',(-27.630761291581,-12.3599344396702,
113.040172878809)) ;
#193465=CARTESIAN_POINT('Ctrl Pts',(-27.5296719419162,-12.3306429195518,
112.767809456319)) ;
#193466=CARTESIAN_POINT('Ctrl Pts',(-27.4298006531373,-12.3792038030185,
112.499012174243)) ;
#193467=CARTESIAN_POINT('Ctrl Pts',(-27.3368869719151,-12.502250920438,
112.251503904024)) ;
#193468=CARTESIAN_POINT('Ctrl Pts',(-27.2572469138254,-12.690704289041,
112.044366413114)) ;
#193469=CARTESIAN_POINT('Ctrl Pts',(-27.1956046752294,-12.9312491813812,
111.892066772438)) ;
#193470=CARTESIAN_POINT('Ctrl Pts',(-27.1556968251946,-13.2069304836541,
111.805999837402)) ;
#193471=CARTESIAN_POINT('Ctrl Pts',(-27.1396183503164,-13.4971323588194,
111.792434998313)) ;
#193472=CARTESIAN_POINT('Ctrl Pts',(-27.1478926952953,-13.7832858649534,
111.853261517309)) ;
#193473=CARTESIAN_POINT('Ctrl Pts',(-27.1788426100833,-14.0408293277911,
111.98281261947)) ;
#193474=CARTESIAN_POINT('Ctrl Pts',(-27.2300778195774,-14.255952322556,
112.174490901595)) ;
#193475=CARTESIAN_POINT('Ctrl Pts',(-27.2963594840731,-14.4094466686143,
112.411688111103)) ;
#193476=CARTESIAN_POINT('Ctrl Pts',(-27.3730829374615,-14.4929694646286,
112.680938243989)) ;
#193477=CARTESIAN_POINT('Ctrl Pts',(-27.4533942328739,-14.4990155260453,
112.961017342185)) ;
#193478=CARTESIAN_POINT('Ctrl Pts',(-27.5309746225123,-14.4275804860338,
113.232800584045)) ;
#193479=CARTESIAN_POINT('Ctrl Pts',(-27.5993744489561,-14.284309082368,
113.476532018314)) ;
#193480=CARTESIAN_POINT('Ctrl Pts',(-27.6533609863589,-14.0775350374868,
113.67660042095)) ;
#193481=CARTESIAN_POINT('Ctrl Pts',(-27.6875986228682,-13.8261134335288,
113.816121058213)) ;
#193482=CARTESIAN_POINT('Ctrl Pts',(-27.6996267717849,-13.5428648342343,
113.888368399397)) ;
#193483=CARTESIAN_POINT('Ctrl Pts',(-27.6873576347831,-13.252182353688,
113.886407116913)) ;
#193484=CARTESIAN_POINT('Ctrl Pts',(-27.651195526548,-12.9730234465435,
113.811707238471)) ;
#193485=CARTESIAN_POINT('Ctrl Pts',(-27.5924502457676,-12.724731390434,
113.668397807756)) ;
#193486=CARTESIAN_POINT('Ctrl Pts',(-27.5156633000477,-12.5280561031159,
113.469790960335)) ;
#193487=CARTESIAN_POINT('Ctrl Pts',(-27.4242158235811,-12.3935893009494,
113.226845172422)) ;
#193488=CARTESIAN_POINT('Ctrl Pts',(-27.3251142958241,-12.333081965445,
112.960365809793)) ;
#193489=CARTESIAN_POINT('Ctrl Pts',(-27.2233916702717,-12.3505128306963,
112.686197908057)) ;
#193490=CARTESIAN_POINT('Ctrl Pts',(-27.12763956026,-12.4433828921911,112.429728050708)) ;
#193491=CARTESIAN_POINT('Ctrl Pts',(-27.0415094033996,-12.607349424796,
112.20302769542)) ;
#193492=CARTESIAN_POINT('Ctrl Pts',(-26.9722746864344,-12.8279036385121,
112.027468698458)) ;
#193493=CARTESIAN_POINT('Ctrl Pts',(-26.9229312024064,-13.0930059035689,
111.912843276643)) ;
#193494=CARTESIAN_POINT('Ctrl Pts',(-26.8972324155193,-13.3789266137586,
111.86989142793)) ;
#193495=CARTESIAN_POINT('Ctrl Pts',(-26.89559593885,-13.6686885717782,111.900373113643)) ;
#193496=CARTESIAN_POINT('Ctrl Pts',(-26.9176753989106,-13.9407698971193,
112.00311647252)) ;
#193497=CARTESIAN_POINT('Ctrl Pts',(-26.9611957529866,-14.1754452261927,
112.171205228785)) ;
#193498=CARTESIAN_POINT('Ctrl Pts',(-27.0218558744677,-14.3550939223612,
112.391319568465)) ;
#193499=CARTESIAN_POINT('Ctrl Pts',(-27.0954919754477,-14.468598908444,
112.65127280273)) ;
#193500=CARTESIAN_POINT('Ctrl Pts',(-27.1747095469528,-14.5058659881171,
112.927861658512)) ;
#193501=CARTESIAN_POINT('Ctrl Pts',(-27.2540706728051,-14.465907705861,
113.205009023131)) ;
#193502=CARTESIAN_POINT('Ctrl Pts',(-27.3270117595021,-14.3507454275659,
113.462647263951)) ;
#193503=CARTESIAN_POINT('Ctrl Pts',(-27.3874657468428,-14.1684902162708,
113.682288696207)) ;
#193504=CARTESIAN_POINT('Ctrl Pts',(-27.4302106667087,-13.9330107336615,
113.847901657391)) ;
#193505=CARTESIAN_POINT('Ctrl Pts',(-27.4515998140738,-13.6600763512271,
113.948553659072)) ;
#193506=CARTESIAN_POINT('Ctrl Pts',(-27.4493246185078,-13.3704757504778,
113.977035138527)) ;
#193507=CARTESIAN_POINT('Ctrl Pts',(-27.4224958680665,-13.0823700026988,
113.93098284499)) ;
#193508=CARTESIAN_POINT('Ctrl Pts',(-27.3729809937545,-12.8213180178566,
113.815427357995)) ;
#193509=CARTESIAN_POINT('Ctrl Pts',(-27.3028037991072,-12.6009816910039,
113.637217641596)) ;
#193510=CARTESIAN_POINT('Ctrl Pts',(-27.2168540748088,-12.4399155910324,
113.410819058086)) ;
#193511=CARTESIAN_POINT('Ctrl Pts',(-27.1197079246416,-12.3483508718252,
113.15053363995)) ;
#193512=CARTESIAN_POINT('Ctrl Pts',(-27.0187802117475,-12.3338872424077,
112.878480782108)) ;
#193513=CARTESIAN_POINT('Ctrl Pts',(-26.9193985159767,-12.396923495094,
112.611312558498)) ;
#193514=CARTESIAN_POINT('Ctrl Pts',(-26.8285566748927,-12.5334553693914,
112.370120041222)) ;
#193515=CARTESIAN_POINT('Ctrl Pts',(-26.7522001619182,-12.7322215761211,
112.172876186384)) ;
#193516=CARTESIAN_POINT('Ctrl Pts',(-26.6943187231654,-12.9810049412899,
112.032078055127)) ;
#193517=CARTESIAN_POINT('Ctrl Pts',(-26.6587912592978,-13.2609753303157,
111.959335470938)) ;
#193518=CARTESIAN_POINT('Ctrl Pts',(-26.647319062969,-13.5522070361543,
111.959866894059)) ;
#193519=CARTESIAN_POINT('Ctrl Pts',(-26.6599556627793,-13.8335794690488,
112.033796091262)) ;
#193520=CARTESIAN_POINT('Ctrl Pts',(-26.6950792057711,-14.0854850074698,
112.176258032588)) ;
#193521=CARTESIAN_POINT('Ctrl Pts',(-26.7493678080384,-14.2893882283517,
112.377063192394)) ;
#193522=CARTESIAN_POINT('Ctrl Pts',(-26.8182694831193,-14.4310416708449,
112.622412303935)) ;
#193523=CARTESIAN_POINT('Ctrl Pts',(-26.8960209759952,-14.4999960091202,
112.894701404491)) ;
#193524=CARTESIAN_POINT('Ctrl Pts',(-26.9762322526902,-14.4914668725251,
113.174447910469)) ;
#193525=CARTESIAN_POINT('Ctrl Pts',(-27.0525399232105,-14.4062237339893,
113.44231798111)) ;
#193526=CARTESIAN_POINT('Ctrl Pts',(-27.1188648773087,-14.2495321967945,
113.679899921954)) ;
#193527=CARTESIAN_POINT('Ctrl Pts',(-27.1692281183874,-14.0340281298451,
113.868701151054)) ;
#193528=CARTESIAN_POINT('Ctrl Pts',(-27.1996623984703,-13.7742259092907,
113.99685412237)) ;
#193529=CARTESIAN_POINT('Ctrl Pts',(-27.2071696580136,-13.488993839479,
114.055160255525)) ;
#193530=CARTESIAN_POINT('Ctrl Pts',(-27.1902825049831,-13.1975717487405,
114.039308325117)) ;
#193531=CARTESIAN_POINT('Ctrl Pts',(-27.1498141482332,-12.9237175982201,
113.951393026303)) ;
#193532=CARTESIAN_POINT('Ctrl Pts',(-27.0872605509044,-12.6833926232874,
113.796490915852)) ;
#193533=CARTESIAN_POINT('Ctrl Pts',(-27.0073325603644,-12.4975233316372,
113.588365552072)) ;
#193534=CARTESIAN_POINT('Ctrl Pts',(-26.9141377906141,-12.3765652756753,
113.339997758843)) ;
#193535=CARTESIAN_POINT('Ctrl Pts',(-26.8140599847601,-12.3303669115662,
113.070599618917)) ;
#193536=CARTESIAN_POINT('Ctrl Pts',(-26.7130188584353,-12.3620831181533,
112.798392930309)) ;
#193537=CARTESIAN_POINT('Ctrl Pts',(-26.6179903821788,-12.4697592102098,
112.544455169899)) ;
#193538=CARTESIAN_POINT('Ctrl Pts',(-26.5351639179177,-12.6447797711106,
112.32756700901)) ;
#193539=CARTESIAN_POINT('Ctrl Pts',(-26.4692769172657,-12.8750273852739,
112.162297586987)) ;
#193540=CARTESIAN_POINT('Ctrl Pts',(-26.4243077785298,-13.1453257818208,
112.060890975421)) ;
#193541=CARTESIAN_POINT('Ctrl Pts',(-26.403013785645,-13.4336234546741,
112.031393920208)) ;
#193542=CARTESIAN_POINT('Ctrl Pts',(-26.4060165852795,-13.7229316022969,
112.076174503052)) ;
#193543=CARTESIAN_POINT('Ctrl Pts',(-26.4323125416507,-13.9881204584926,
112.191610815065)) ;
#193544=CARTESIAN_POINT('Ctrl Pts',(-26.4792881537362,-14.2135626266573,
112.370156392619)) ;
#193545=CARTESIAN_POINT('Ctrl Pts',(-26.5430286631922,-14.3820856851378,
112.599827193971)) ;
#193546=CARTESIAN_POINT('Ctrl Pts',(-26.6176671822151,-14.4811007735871,
112.862516248575)) ;
#193547=CARTESIAN_POINT('Ctrl Pts',(-26.6978612990312,-14.5043853087956,
113.142314338476)) ;
#193548=CARTESIAN_POINT('Ctrl Pts',(-26.7765022627845,-14.4497319209782,
113.417276345146)) ;
#193549=CARTESIAN_POINT('Ctrl Pts',(-26.8476800485963,-14.3208489038209,
113.669628788919)) ;
#193550=CARTESIAN_POINT('Ctrl Pts',(-26.9051290746846,-14.1269083086763,
113.880141966721)) ;
#193551=CARTESIAN_POINT('Ctrl Pts',(-26.9439250946234,-13.8839530008224,
114.033597139485)) ;
#193552=CARTESIAN_POINT('Ctrl Pts',(-26.9610011688202,-13.6058131007772,
114.121164169516)) ;
#193553=CARTESIAN_POINT('Ctrl Pts',(-26.9541142012214,-13.3154623494247,
114.135571911121)) ;
#193554=CARTESIAN_POINT('Ctrl Pts',(-26.9227927789619,-13.0305252756843,
114.075814770893)) ;
#193555=CARTESIAN_POINT('Ctrl Pts',(-26.8691774398986,-12.7760411077928,
113.947787130553)) ;
#193556=CARTESIAN_POINT('Ctrl Pts',(-26.7957043233195,-12.5658693797106,
113.759493744326)) ;
#193557=CARTESIAN_POINT('Ctrl Pts',(-26.7071990036801,-12.4170609140262,
113.52535902764)) ;
#193558=CARTESIAN_POINT('Ctrl Pts',(-26.6088521342578,-12.3396249333132,
113.261367652909)) ;
#193559=CARTESIAN_POINT('Ctrl Pts',(-26.5073352253782,-12.340046412335,
112.987690769148)) ;
#193560=CARTESIAN_POINT('Ctrl Pts',(-26.4097025231263,-12.4170460254182,
112.725620310096)) ;
#193561=CARTESIAN_POINT('Ctrl Pts',(-26.3209819060534,-12.5662136094611,
112.490921752616)) ;
#193562=CARTESIAN_POINT('Ctrl Pts',(-26.2476333327786,-12.7760199991739,
112.30293791623)) ;
#193563=CARTESIAN_POINT('Ctrl Pts',(-26.1937928662736,-13.0322696653641,
112.174451982578)) ;
#193564=CARTESIAN_POINT('Ctrl Pts',(-26.1627547455184,-13.3151090323585,
112.115281050215)) ;
#193565=CARTESIAN_POINT('Ctrl Pts',(-26.1558631196965,-13.6075492018493,
112.129940953347)) ;
#193566=CARTESIAN_POINT('Ctrl Pts',(-26.1729300005076,-13.8839937911961,
112.217263774275)) ;
#193567=CARTESIAN_POINT('Ctrl Pts',(-26.2120071941306,-14.1283418739825,
112.371799593747)) ;
#193568=CARTESIAN_POINT('Ctrl Pts',(-26.2693072989749,-14.321085337762,
112.58170002845)) ;
#193569=CARTESIAN_POINT('Ctrl Pts',(-26.3405926471782,-14.4501544762085,
112.834435287317)) ;
#193570=CARTESIAN_POINT('Ctrl Pts',(-26.4193828840965,-14.504350239421,
113.109906480253)) ;
#193571=CARTESIAN_POINT('Ctrl Pts',(-26.4990873137165,-14.4811635345991,
113.387994186648)) ;
#193572=CARTESIAN_POINT('Ctrl Pts',(-26.5741035318335,-14.3816036851556,
113.652018746242)) ;
#193573=CARTESIAN_POINT('Ctrl Pts',(-26.6376352371572,-14.2132115910195,
113.88096634118)) ;
#193574=CARTESIAN_POINT('Ctrl Pts',(-26.6847308687247,-13.9871283531687,
114.059972839669)) ;
#193575=CARTESIAN_POINT('Ctrl Pts',(-26.7108828323385,-13.7209751384546,
114.175063486759)) ;
#193576=CARTESIAN_POINT('Ctrl Pts',(-26.7138425852466,-13.4341833204507,
114.21939759733)) ;
#193577=CARTESIAN_POINT('Ctrl Pts',(-26.692396148443,-13.1440226446982,
114.18967350618)) ;
#193578=CARTESIAN_POINT('Ctrl Pts',(-26.6475602009265,-12.8750223963181,
114.08850476367)) ;
#193579=CARTESIAN_POINT('Ctrl Pts',(-26.5813161216274,-12.6437154561283,
113.922329063855)) ;
#193580=CARTESIAN_POINT('Ctrl Pts',(-26.4986543480993,-12.4695015573388,
113.705836185377)) ;
#193581=CARTESIAN_POINT('Ctrl Pts',(-26.40350334832,-12.3618253102505,113.451569423215)) ;
#193582=CARTESIAN_POINT('Ctrl Pts',(-26.3025135279916,-12.3304086987919,
113.179494242336)) ;
#193583=CARTESIAN_POINT('Ctrl Pts',(-26.2025781370336,-12.3767667157857,
112.910488649315)) ;
#193584=CARTESIAN_POINT('Ctrl Pts',(-26.1095364919782,-12.4973266925111,
112.662514220771)) ;
#193585=CARTESIAN_POINT('Ctrl Pts',(-26.0290482236216,-12.6849702880242,
112.452967860837)) ;
#193586=CARTESIAN_POINT('Ctrl Pts',(-25.967020193737,-12.9239536141708,
112.299425204879)) ;
#193587=CARTESIAN_POINT('Ctrl Pts',(-25.9264894675845,-13.198264514804,
112.211386234531)) ;
#193588=CARTESIAN_POINT('Ctrl Pts',(-25.9096865137876,-13.4887696764051,
112.195672545383)) ;
#193589=CARTESIAN_POINT('Ctrl Pts',(-25.9171975165263,-13.7747050880232,
112.254081199622)) ;
#193590=CARTESIAN_POINT('Ctrl Pts',(-25.9477017056163,-14.0346989777519,
112.382474254739)) ;
#193591=CARTESIAN_POINT('Ctrl Pts',(-25.9983172672415,-14.2504823475427,
112.572150154809)) ;
#193592=CARTESIAN_POINT('Ctrl Pts',(-26.0642269575703,-14.4061007577842,
112.808231529626)) ;
#193593=CARTESIAN_POINT('Ctrl Pts',(-26.141044455505,-14.4917978275685,
113.07789332878)) ;
#193594=CARTESIAN_POINT('Ctrl Pts',(-26.2209372515167,-14.4998539330622,
113.356520375798)) ;
#193595=CARTESIAN_POINT('Ctrl Pts',(-26.2986502411454,-14.4309092256038,
113.628683576885)) ;
#193596=CARTESIAN_POINT('Ctrl Pts',(-26.3674757304941,-14.2894596882656,
113.873752815504)) ;
#193597=CARTESIAN_POINT('Ctrl Pts',(-26.4219359703617,-14.0846391379262,
114.075220353395)) ;
#193598=CARTESIAN_POINT('Ctrl Pts',(-26.4568504724485,-13.833584389583,
114.216907404291)) ;
#193599=CARTESIAN_POINT('Ctrl Pts',(-26.469569796329,-13.5522887119168,
114.291086084856)) ;
#193600=CARTESIAN_POINT('Ctrl Pts',(-26.4579117148728,-13.2592972529684,
114.291267191308)) ;
#193601=CARTESIAN_POINT('Ctrl Pts',(-26.4225035557811,-12.9811038250668,
114.218671706621)) ;
#193602=CARTESIAN_POINT('Ctrl Pts',(-26.3646027960108,-12.7319954339599,
114.077855142364)) ;
#193603=CARTESIAN_POINT('Ctrl Pts',(-26.2880633731457,-12.5329045763516,
113.880121143368)) ;
#193604=CARTESIAN_POINT('Ctrl Pts',(-26.1969121836829,-12.3964115152595,
113.638084995048)) ;
#193605=CARTESIAN_POINT('Ctrl Pts',(-26.097882878132,-12.3338312624075,
113.371853705732)) ;
#193606=CARTESIAN_POINT('Ctrl Pts',(-25.9966525666846,-12.3486707517994,
113.098994699644)) ;
#193607=CARTESIAN_POINT('Ctrl Pts',(-25.9000472227805,-12.4397941697449,
112.840152077552)) ;
#193608=CARTESIAN_POINT('Ctrl Pts',(-25.8135929246481,-12.6021170084136,
112.612453782006)) ;
#193609=CARTESIAN_POINT('Ctrl Pts',(-25.7439720862117,-12.8208593941247,
112.435659485376)) ;
#193610=CARTESIAN_POINT('Ctrl Pts',(-25.6940349138125,-13.084370773037,
112.319151955814)) ;
#193611=CARTESIAN_POINT('Ctrl Pts',(-25.6675129647773,-13.3711928765175,
112.273852263887)) ;
#193612=CARTESIAN_POINT('Ctrl Pts',(-25.6652923171855,-13.6609866789311,
112.302537231817)) ;
#193613=CARTESIAN_POINT('Ctrl Pts',(-25.6865853284364,-13.9327616913683,
112.402736133509)) ;
#193614=CARTESIAN_POINT('Ctrl Pts',(-25.7296598130416,-14.1696775509721,
112.569592493143)) ;
#193615=CARTESIAN_POINT('Ctrl Pts',(-25.789817147401,-14.3505522399701,
112.788110084322)) ;
#193616=CARTESIAN_POINT('Ctrl Pts',(-25.8627735208457,-14.4659895814683,
113.045823772028)) ;
#193617=CARTESIAN_POINT('Ctrl Pts',(-25.9424652085819,-14.5060552317741,
113.324112272392)) ;
#193618=CARTESIAN_POINT('Ctrl Pts',(-26.0220030697392,-14.4677867862301,
113.601843781957)) ;
#193619=CARTESIAN_POINT('Ctrl Pts',(-26.094854630819,-14.3553856703914,
113.859024726864)) ;
#193620=CARTESIAN_POINT('Ctrl Pts',(-26.1560900365016,-14.1738642018268,
114.081250316961)) ;
#193621=CARTESIAN_POINT('Ctrl Pts',(-26.1991928753205,-13.9401973275635,
114.247846762684)) ;
#193622=CARTESIAN_POINT('Ctrl Pts',(-26.2212325199795,-13.6684975496401,
114.35043177796)) ;
#193623=CARTESIAN_POINT('Ctrl Pts',(-26.2196857700443,-13.3792258998284,
114.381117503958)) ;
#193624=CARTESIAN_POINT('Ctrl Pts',(-26.1935600200775,-13.0905267308239,
114.337229266664)) ;
#193625=CARTESIAN_POINT('Ctrl Pts',(-26.1446708799254,-12.8284630006125,
114.223586216955)) ;
#193626=CARTESIAN_POINT('Ctrl Pts',(-26.0750221134765,-12.6065365051644,
114.046995192604)) ;
#193627=CARTESIAN_POINT('Ctrl Pts',(-25.9893085808254,-12.4434900571409,
113.821371187434)) ;
#193628=CARTESIAN_POINT('Ctrl Pts',(-25.8927472268414,-12.3500508502058,
113.562734682547)) ;
#193629=CARTESIAN_POINT('Ctrl Pts',(-25.7915387238206,-12.3331953888952,
113.289941672903)) ;
#193630=CARTESIAN_POINT('Ctrl Pts',(-25.6921668349445,-12.3940161187778,
113.022744551192)) ;
#193631=CARTESIAN_POINT('Ctrl Pts',(-25.6010011665108,-12.5284976067023,
112.780567517695)) ;
#193632=CARTESIAN_POINT('Ctrl Pts',(-25.5241403849889,-12.7253590046235,
112.581767024192)) ;
#193633=CARTESIAN_POINT('Ctrl Pts',(-25.4653269966594,-12.9750336085797,
112.438402703222)) ;
#193634=CARTESIAN_POINT('Ctrl Pts',(-25.4295219032565,-13.2518773391213,
112.364484091442)) ;
#193635=CARTESIAN_POINT('Ctrl Pts',(-25.4172132742783,-13.5442043587849,
112.36261312341)) ;
#193636=CARTESIAN_POINT('Ctrl Pts',(-25.4292212348024,-13.8259451748865,
112.434602285511)) ;
#193637=CARTESIAN_POINT('Ctrl Pts',(-25.4637880029618,-14.0792480619856,
112.575412566812)) ;
#193638=CARTESIAN_POINT('Ctrl Pts',(-25.5175967023213,-14.2845087011992,
112.774736681666)) ;
#193639=CARTESIAN_POINT('Ctrl Pts',(-25.58604236121,-14.4278905637469,113.018639551001)) ;
#193640=CARTESIAN_POINT('Ctrl Pts',(-25.6636620375048,-14.49909499359,113.290546274635)) ;
#193641=CARTESIAN_POINT('Ctrl Pts',(-25.7439225347513,-14.492829252027,
113.570454450893)) ;
#193642=CARTESIAN_POINT('Ctrl Pts',(-25.8206456678488,-14.4093444300335,
113.83969383373)) ;
#193643=CARTESIAN_POINT('Ctrl Pts',(-25.8872186639727,-14.2544052422715,
114.077996994067)) ;
#193644=CARTESIAN_POINT('Ctrl Pts',(-25.9379469965569,-14.0410991720381,
114.267799990034)) ;
#193645=CARTESIAN_POINT('Ctrl Pts',(-25.9690716034183,-13.7816895970119,
114.398141043581)) ;
#193646=CARTESIAN_POINT('Ctrl Pts',(-25.977202611184,-13.4976199910735,
114.4582556851)) ;
#193647=CARTESIAN_POINT('Ctrl Pts',(-25.9611123344456,-13.2063007087737,
114.444798177741)) ;
#193648=CARTESIAN_POINT('Ctrl Pts',(-25.9211552662506,-12.9308185504047,
114.358558160609)) ;
#193649=CARTESIAN_POINT('Ctrl Pts',(-25.8593713827175,-12.690040453889,
114.205882675566)) ;
#193650=CARTESIAN_POINT('Ctrl Pts',(-25.7799037685495,-12.5021903792694,
113.999176989546)) ;
#193651=CARTESIAN_POINT('Ctrl Pts',(-25.6868876116915,-12.3790435207342,
113.751397700364)) ;
#193652=CARTESIAN_POINT('Ctrl Pts',(-25.5868978508818,-12.3305042760163,
113.482273898361)) ;
#193653=CARTESIAN_POINT('Ctrl Pts',(-25.4854179660145,-12.3604684800267,
113.208869990196)) ;
#193654=CARTESIAN_POINT('Ctrl Pts',(-25.3908722354269,-12.4650891112354,
112.956114236995)) ;
#193655=CARTESIAN_POINT('Ctrl Pts',(-25.3069218934639,-12.6397680496829,
112.736110244212)) ;
#193656=CARTESIAN_POINT('Ctrl Pts',(-25.2409292762661,-12.8673926753431,
112.570297954244)) ;
#193657=CARTESIAN_POINT('Ctrl Pts',(-25.1950431269417,-13.138383085188,
112.466309655478)) ;
#193658=CARTESIAN_POINT('Ctrl Pts',(-25.1732970592646,-13.4250580301084,
112.435262725168)) ;
#193659=CARTESIAN_POINT('Ctrl Pts',(-25.175431424128,-13.713663843469,112.477262712461)) ;
#193660=CARTESIAN_POINT('Ctrl Pts',(-25.2013058612131,-13.9818996954329,
112.591702432285)) ;
#193661=CARTESIAN_POINT('Ctrl Pts',(-25.2475462461254,-14.2073240866329,
112.767809158823)) ;
#193662=CARTESIAN_POINT('Ctrl Pts',(-25.3107801482558,-14.3779496982449,
112.995927736214)) ;
#193663=CARTESIAN_POINT('Ctrl Pts',(-25.3855441089235,-14.4795452062324,
113.25916632019)) ;
#193664=CARTESIAN_POINT('Ctrl Pts',(-25.4657056298432,-14.504675613756,
113.538873967324)) ;
#193665=CARTESIAN_POINT('Ctrl Pts',(-25.5441348471131,-14.4524935600785,
113.813035826526)) ;
#193666=CARTESIAN_POINT('Ctrl Pts',(-25.6158038670484,-14.3253673837965,
114.066976143731)) ;
#193667=CARTESIAN_POINT('Ctrl Pts',(-25.6735934060056,-14.1335026343525,
114.278447647152)) ;
#193668=CARTESIAN_POINT('Ctrl Pts',(-25.713031726844,-13.8914689377216,
114.433910815975)) ;
#193669=CARTESIAN_POINT('Ctrl Pts',(-25.7307687812816,-13.6147208150664,
114.523401386807)) ;
#193670=CARTESIAN_POINT('Ctrl Pts',(-25.7245757601632,-13.3237687258409,
114.540012491979)) ;
#193671=CARTESIAN_POINT('Ctrl Pts',(-25.6941237439954,-13.0396242352637,
114.482736350999)) ;
#193672=CARTESIAN_POINT('Ctrl Pts',(-25.6410851839242,-12.7830678889279,
114.356574719083)) ;
#193673=CARTESIAN_POINT('Ctrl Pts',(-25.5676997033759,-12.5704752635878,
114.168721963641)) ;
#193674=CARTESIAN_POINT('Ctrl Pts',(-25.4799422590946,-12.4206416986158,
113.936696566694)) ;
#193675=CARTESIAN_POINT('Ctrl Pts',(-25.381998179666,-12.3408954926335,
113.673866420762)) ;
#193676=CARTESIAN_POINT('Ctrl Pts',(-25.2803675767541,-12.3388375024718,
113.399883536457)) ;
#193677=CARTESIAN_POINT('Ctrl Pts',(-25.1823213194761,-12.413706142133,
113.136628920894)) ;
#193678=CARTESIAN_POINT('Ctrl Pts',(-25.092980715359,-12.5617183582742,
112.900167957605)) ;
#193679=CARTESIAN_POINT('Ctrl Pts',(-25.0195846393668,-12.7688407831079,
112.711834010416)) ;
#193680=CARTESIAN_POINT('Ctrl Pts',(-24.9649866794184,-13.0241117816514,
112.581077125632)) ;
#193681=CARTESIAN_POINT('Ctrl Pts',(-24.9332536836434,-13.3070010234793,
112.51985755415)) ;
#193682=CARTESIAN_POINT('Ctrl Pts',(-24.925629722327,-13.5985554109386,
112.532164471356)) ;
#193683=CARTESIAN_POINT('Ctrl Pts',(-24.9421245854702,-13.8770852609277,
112.617931075453)) ;
#193684=CARTESIAN_POINT('Ctrl Pts',(-24.9804514510273,-14.1214182763711,
112.770005884966)) ;
#193685=CARTESIAN_POINT('Ctrl Pts',(-25.0373635997591,-14.3164119676812,
112.978804934412)) ;
#193686=CARTESIAN_POINT('Ctrl Pts',(-25.1082654742619,-14.4472714989735,
113.230330811616)) ;
#193687=CARTESIAN_POINT('Ctrl Pts',(-25.1868459524037,-14.5039655219921,
113.505134344491)) ;
#193688=CARTESIAN_POINT('Ctrl Pts',(-25.267129516287,-14.4826373105238,
113.785223901541)) ;
#193689=CARTESIAN_POINT('Ctrl Pts',(-25.3418916496393,-14.3855815012644,
114.048250710986)) ;
#193690=CARTESIAN_POINT('Ctrl Pts',(-25.4059102519348,-14.2190969785884,
114.278710495903)) ;
#193691=CARTESIAN_POINT('Ctrl Pts',(-25.4534572816173,-13.9949296481822,
114.4590197693)) ;
#193692=CARTESIAN_POINT('Ctrl Pts',(-25.4803949407615,-13.7298783707897,
114.576500255508)) ;
#193693=CARTESIAN_POINT('Ctrl Pts',(-25.4839639384194,-13.4411780607526,
114.622967439281)) ;
#193694=CARTESIAN_POINT('Ctrl Pts',(-25.4634405619125,-13.1535366585443,
114.595704133561)) ;
#193695=CARTESIAN_POINT('Ctrl Pts',(-25.4188861853407,-12.8812078446008,
114.495722751362)) ;
#193696=CARTESIAN_POINT('Ctrl Pts',(-25.3535678038264,-12.6502697095916,
114.332121264411)) ;
#193697=CARTESIAN_POINT('Ctrl Pts',(-25.271268624716,-12.4736381112203,
114.116796974903)) ;
#193698=CARTESIAN_POINT('Ctrl Pts',(-25.1760059663422,-12.3636957343507,
113.862315910691)) ;
#193699=CARTESIAN_POINT('Ctrl Pts',(-25.0755208022999,-12.3303161657527,
113.59162885322)) ;
#193700=CARTESIAN_POINT('Ctrl Pts',(-24.975387420301,-12.3741418831008,
113.322042926048)) ;
#193701=CARTESIAN_POINT('Ctrl Pts',(-24.8815379026335,-12.4937241519796,
113.071825125992)) ;
#193702=CARTESIAN_POINT('Ctrl Pts',(-24.8012449463837,-12.6783961032596,
112.862605193765)) ;
#193703=CARTESIAN_POINT('Ctrl Pts',(-24.738447605087,-12.9163766433386,
112.706791373276)) ;
#193704=CARTESIAN_POINT('Ctrl Pts',(-24.697217131185,-13.1903758945546,
112.616669578636)) ;
#193705=CARTESIAN_POINT('Ctrl Pts',(-24.679735225327,-13.481432819081,112.598974089601)) ;
#193706=CARTESIAN_POINT('Ctrl Pts',(-24.6866566649467,-13.7673558416161,
112.655538950219)) ;
#193707=CARTESIAN_POINT('Ctrl Pts',(-24.7163960105244,-14.0271101613543,
112.781439555252)) ;
#193708=CARTESIAN_POINT('Ctrl Pts',(-24.7663270399,-14.2445027860115,112.968989653976)) ;
#193709=CARTESIAN_POINT('Ctrl Pts',(-24.8322750811479,-14.4028029107363,
113.205401926826)) ;
#193710=CARTESIAN_POINT('Ctrl Pts',(-24.9082113685337,-14.4900131921161,
113.472067220855)) ;
#193711=CARTESIAN_POINT('Ctrl Pts',(-24.9884934184206,-14.5009049303826,
113.752069619527)) ;
#193712=CARTESIAN_POINT('Ctrl Pts',(-25.0666037768646,-14.4337694493022,
114.025547084295)) ;
#193713=CARTESIAN_POINT('Ctrl Pts',(-25.1357889459536,-14.2939322119372,
114.271744953977)) ;
#193714=CARTESIAN_POINT('Ctrl Pts',(-25.1905524181362,-14.0911613446941,
114.474041191823)) ;
#193715=CARTESIAN_POINT('Ctrl Pts',(-25.2261345436437,-13.8412394795533,
114.617769466887)) ;
#193716=CARTESIAN_POINT('Ctrl Pts',(-25.2394283887284,-13.5592605313859,
114.693848406936)) ;
#193717=CARTESIAN_POINT('Ctrl Pts',(-25.2286664367361,-13.2696223387077,
114.696342245869)) ;
#193718=CARTESIAN_POINT('Ctrl Pts',(-25.1937485823441,-12.9883139496615,
114.625551828042)) ;
#193719=CARTESIAN_POINT('Ctrl Pts',(-25.1365175245661,-12.7386910562247,
114.486687971447)) ;
#193720=CARTESIAN_POINT('Ctrl Pts',(-25.0603010182413,-12.5375785963018,
114.290016712916)) ;
#193721=CARTESIAN_POINT('Ctrl Pts',(-24.9698092052317,-12.3995778757378,
114.049856870399)) ;
#193722=CARTESIAN_POINT('Ctrl Pts',(-24.8707009033833,-12.3345174279643,
113.783475116184)) ;
#193723=CARTESIAN_POINT('Ctrl Pts',(-24.7695605990675,-12.3471393395654,
113.510844338411)) ;
#193724=CARTESIAN_POINT('Ctrl Pts',(-24.6727328214046,-12.4360428670471,
113.251326381663)) ;
#193725=CARTESIAN_POINT('Ctrl Pts',(-24.5859199646112,-12.5962612233629,
113.022510647249)) ;
#193726=CARTESIAN_POINT('Ctrl Pts',(-24.5156431401964,-12.8139558923281,
112.843788818509)) ;
#193727=CARTESIAN_POINT('Ctrl Pts',(-24.4652008507486,-13.0756188660845,
112.725627916536)) ;
#193728=CARTESIAN_POINT('Ctrl Pts',(-24.4379052691479,-13.3624251132735,
112.678030789951)) ;
#193729=CARTESIAN_POINT('Ctrl Pts',(-24.4348796019806,-13.651982180129,
112.704196399724)) ;
#193730=CARTESIAN_POINT('Ctrl Pts',(-24.4558001085789,-13.9268736432231,
112.803588355088)) ;
#193731=CARTESIAN_POINT('Ctrl Pts',(-24.4978634283469,-14.1624927779437,
112.966970517185)) ;
#193732=CARTESIAN_POINT('Ctrl Pts',(-24.5579911299017,-14.3467872124729,
113.185684905417)) ;
#193733=CARTESIAN_POINT('Ctrl Pts',(-24.6305363548121,-14.4636106389172,
113.442047638809)) ;
#193734=CARTESIAN_POINT('Ctrl Pts',(-24.7098618797107,-14.505904926533,
113.719115599711)) ;
#193735=CARTESIAN_POINT('Ctrl Pts',(-24.789457567232,-14.4703681622542,
113.996992018783)) ;
#193736=CARTESIAN_POINT('Ctrl Pts',(-24.8630886166822,-14.359008640194,
114.256813432633)) ;
#193737=CARTESIAN_POINT('Ctrl Pts',(-24.9242076077781,-14.1808823670753,
114.478358262173)) ;
#193738=CARTESIAN_POINT('Ctrl Pts',(-24.9681883548515,-13.9476582149858,
114.647809634132)) ;
#193739=CARTESIAN_POINT('Ctrl Pts',(-24.9908627448388,-13.6767014389998,
114.75232403868)) ;
#193740=CARTESIAN_POINT('Ctrl Pts',(-24.9899695835005,-13.3872299120028,
114.785058404499)) ;
#193741=CARTESIAN_POINT('Ctrl Pts',(-24.9646913454561,-13.0993467868879,
114.743596413779)) ;
#193742=CARTESIAN_POINT('Ctrl Pts',(-24.9162024965776,-12.8349662721153,
114.631357615901)) ;
#193743=CARTESIAN_POINT('Ctrl Pts',(-24.847245455251,-12.6123125745559,
114.45676980248)) ;
#193744=CARTESIAN_POINT('Ctrl Pts',(-24.7618055368288,-12.447065748415,
114.232038687256)) ;
#193745=CARTESIAN_POINT('Ctrl Pts',(-24.6654288827052,-12.3516677675638,
113.973971864171)) ;
#193746=CARTESIAN_POINT('Ctrl Pts',(-24.5645423752006,-12.3325934792249,
113.702063110992)) ;
#193747=CARTESIAN_POINT('Ctrl Pts',(-24.4649295396859,-12.3910918553195,
113.434163508363)) ;
#193748=CARTESIAN_POINT('Ctrl Pts',(-24.37322692579,-12.5239274893633,113.190432787571)) ;
#193749=CARTESIAN_POINT('Ctrl Pts',(-24.2960054560042,-12.7192927751428,
112.990520520361)) ;
#193750=CARTESIAN_POINT('Ctrl Pts',(-24.2369143117434,-12.9658343070978,
112.84605739491)) ;
#193751=CARTESIAN_POINT('Ctrl Pts',(-24.2000431301647,-13.2443245338218,
112.769193829695)) ;
#193752=CARTESIAN_POINT('Ctrl Pts',(-24.187186648989,-13.5367809605308,
112.765670474547)) ;
#193753=CARTESIAN_POINT('Ctrl Pts',(-24.198485812454,-13.8179726435299,
112.835367593194)) ;
#193754=CARTESIAN_POINT('Ctrl Pts',(-24.2324273152291,-14.0724753431544,
112.974281755024)) ;
#193755=CARTESIAN_POINT('Ctrl Pts',(-24.2856593105687,-14.279096140685,
113.171804870744)) ;
#193756=CARTESIAN_POINT('Ctrl Pts',(-24.3538376843237,-14.4248617955916,
113.414949069186)) ;
#193757=CARTESIAN_POINT('Ctrl Pts',(-24.4316472822689,-14.4982152843021,
113.687591297354)) ;
#193758=CARTESIAN_POINT('Ctrl Pts',(-24.511415885813,-14.4941260357652,
113.965774681427)) ;
#193759=CARTESIAN_POINT('Ctrl Pts',(-24.588572932717,-14.4126782343137,
114.236447003153)) ;
#193760=CARTESIAN_POINT('Ctrl Pts',(-24.6553633361676,-14.2599648668114,
114.475326275185)) ;
#193761=CARTESIAN_POINT('Ctrl Pts',(-24.7066777082595,-14.0478524029628,
114.666975267341)) ;
#193762=CARTESIAN_POINT('Ctrl Pts',(-24.7383886959719,-13.7904112840523,
114.79898244504)) ;
#193763=CARTESIAN_POINT('Ctrl Pts',(-24.7472587412919,-13.5044552055669,
114.861642887694)) ;
#193764=CARTESIAN_POINT('Ctrl Pts',(-24.7317360628477,-13.2137879040768,
114.849818087154)) ;
#193765=CARTESIAN_POINT('Ctrl Pts',(-24.6925768386914,-12.9385963486889,
114.765886618446)) ;
#193766=CARTESIAN_POINT('Ctrl Pts',(-24.6315155721698,-12.6966955833364,
114.615366123145)) ;
#193767=CARTESIAN_POINT('Ctrl Pts',(-24.5521621899109,-12.5064217313258,
114.409158146371)) ;
#193768=CARTESIAN_POINT('Ctrl Pts',(-24.4595930056771,-12.3814205030376,
114.162674429355)) ;
#193769=CARTESIAN_POINT('Ctrl Pts',(-24.3591960058421,-12.3309490204366,
113.892499417778)) ;
#193770=CARTESIAN_POINT('Ctrl Pts',(-24.2590492512348,-12.3579787522632,
113.62264874675)) ;
#193771=CARTESIAN_POINT('Ctrl Pts',(-24.1631094563438,-12.461461206882,
113.36607630111)) ;
#193772=CARTESIAN_POINT('Ctrl Pts',(-24.0794846118896,-12.6327579824641,
113.146729045038)) ;
#193773=CARTESIAN_POINT('Ctrl Pts',(-24.0122990421959,-12.8610649262646,
112.977629767465)) ;
#193774=CARTESIAN_POINT('Ctrl Pts',(-23.9662485633249,-13.1282120035714,
112.872739576532)) ;
#193775=CARTESIAN_POINT('Ctrl Pts',(-23.9434524616525,-13.4170777357306,
112.838817161117)) ;
#193776=CARTESIAN_POINT('Ctrl Pts',(-23.9449981053748,-13.7056413839055,
112.878978183992)) ;
#193777=CARTESIAN_POINT('Ctrl Pts',(-23.9701821735012,-13.9747406301587,
112.991309111019)) ;
#193778=CARTESIAN_POINT('Ctrl Pts',(-24.0160072122531,-14.201974810105,
113.166223946965)) ;
#193779=CARTESIAN_POINT('Ctrl Pts',(-24.0787453413408,-14.3739130003505,
113.392766421991)) ;
#193780=CARTESIAN_POINT('Ctrl Pts',(-24.153021958778,-14.4775305035498,
113.654416785986)) ;
#193781=CARTESIAN_POINT('Ctrl Pts',(-24.2334081776458,-14.5050608269986,
113.934939965511)) ;
#193782=CARTESIAN_POINT('Ctrl Pts',(-24.3118138425738,-14.4551363613954,
114.208959708269)) ;
#193783=CARTESIAN_POINT('Ctrl Pts',(-24.3838624730078,-14.3298705824412,
114.464102745858)) ;
#193784=CARTESIAN_POINT('Ctrl Pts',(-24.4418657884039,-14.1407879039854,
114.676048055119)) ;
#193785=CARTESIAN_POINT('Ctrl Pts',(-24.4821519623665,-13.8991517087972,
114.83424842299)) ;
#193786=CARTESIAN_POINT('Ctrl Pts',(-24.5005313129686,-13.622377664187,
114.925775683021)) ;
#193787=CARTESIAN_POINT('Ctrl Pts',(-24.49501436777,-13.3324243748073,114.944342617232)) ;
#193788=CARTESIAN_POINT('Ctrl Pts',(-24.4653775774576,-13.0478498918573,
114.889526808152)) ;
#193789=CARTESIAN_POINT('Ctrl Pts',(-24.4124318331185,-12.7884262570381,
114.76392923946)) ;
#193790=CARTESIAN_POINT('Ctrl Pts',(-24.3401997969462,-12.5764203972658,
114.57925123095)) ;
#193791=CARTESIAN_POINT('Ctrl Pts',(-24.2523979814976,-12.4236100991773,
114.347280755597)) ;
#193792=CARTESIAN_POINT('Ctrl Pts',(-24.1544007543503,-12.3419562515338,
114.084359044048)) ;
#193793=CARTESIAN_POINT('Ctrl Pts',(-24.0529879307825,-12.3379525743983,
113.810967700911)) ;
#193794=CARTESIAN_POINT('Ctrl Pts',(-23.9551105454002,-12.4104778611719,
113.54810794873)) ;
#193795=CARTESIAN_POINT('Ctrl Pts',(-23.8656364276719,-12.5557718304403,
113.311130140898)) ;
#193796=CARTESIAN_POINT('Ctrl Pts',(-23.7913251487216,-12.7621800376528,
113.120181789862)) ;
#193797=CARTESIAN_POINT('Ctrl Pts',(-23.7361036954528,-13.0168738808962,
112.987578292511)) ;
#193798=CARTESIAN_POINT('Ctrl Pts',(-23.703804074422,-13.2984278863564,
112.924531497575)) ;
#193799=CARTESIAN_POINT('Ctrl Pts',(-23.6954444130968,-13.5897265030932,
112.93456078648)) ;
#193800=CARTESIAN_POINT('Ctrl Pts',(-23.7111888510481,-13.8688372211758,
113.018021310344)) ;
#193801=CARTESIAN_POINT('Ctrl Pts',(-23.7490277618584,-14.1152016754008,
113.168722954981)) ;
#193802=CARTESIAN_POINT('Ctrl Pts',(-23.8054647064364,-14.3116011164225,
113.376051058603)) ;
#193803=CARTESIAN_POINT('Ctrl Pts',(-23.8758475364015,-14.4442909382302,
113.625906113769)) ;
#193804=CARTESIAN_POINT('Ctrl Pts',(-23.9543884340958,-14.5033545209173,
113.900640311808)) ;
#193805=CARTESIAN_POINT('Ctrl Pts',(-24.034459322074,-14.4845849990311,
114.179961742102)) ;
#193806=CARTESIAN_POINT('Ctrl Pts',(-24.1098198340275,-14.3894948595566,
114.444970199635)) ;
#193807=CARTESIAN_POINT('Ctrl Pts',(-24.1743167962616,-14.2243477865837,
114.676951586264)) ;
#193808=CARTESIAN_POINT('Ctrl Pts',(-24.222244696456,-14.0022176408066,
114.858320300605)) ;
#193809=CARTESIAN_POINT('Ctrl Pts',(-24.249840889695,-13.738467096939,114.977769983769)) ;
#193810=CARTESIAN_POINT('Ctrl Pts',(-24.2541673118349,-13.4497089979361,
115.026595498721)) ;
#193811=CARTESIAN_POINT('Ctrl Pts',(-24.2342295189752,-13.1612741016994,
115.001189108722)) ;
#193812=CARTESIAN_POINT('Ctrl Pts',(-24.190640216784,-12.8897094409154,
114.903930822118)) ;
#193813=CARTESIAN_POINT('Ctrl Pts',(-24.12571950388,-12.6562456914582,114.741683307062)) ;
#193814=CARTESIAN_POINT('Ctrl Pts',(-24.0436220945344,-12.4776727385034,
114.527047044572)) ;
#193815=CARTESIAN_POINT('Ctrl Pts',(-23.949166950014,-12.3662041520314,
114.27482871689)) ;
#193816=CARTESIAN_POINT('Ctrl Pts',(-23.8486819494618,-12.3300379060018,
114.004176603024)) ;
#193817=CARTESIAN_POINT('Ctrl Pts',(-23.7479716280047,-12.3719948524369,
113.733003975022)) ;
#193818=CARTESIAN_POINT('Ctrl Pts',(-23.6544815761993,-12.4886302946211,
113.483633344995)) ;
#193819=CARTESIAN_POINT('Ctrl Pts',(-23.5734119895845,-12.6716133926028,
113.272144861852)) ;
#193820=CARTESIAN_POINT('Ctrl Pts',(-23.5097546848615,-12.9096205473869,
113.113892958082)) ;
#193821=CARTESIAN_POINT('Ctrl Pts',(-23.4680736791357,-13.1819739695916,
113.02227623672)) ;
#193822=CARTESIAN_POINT('Ctrl Pts',(-23.4498548257593,-13.4720244815185,
113.002241777348)) ;
#193823=CARTESIAN_POINT('Ctrl Pts',(-23.4559991647249,-13.7591219512168,
113.056520534112)) ;
#193824=CARTESIAN_POINT('Ctrl Pts',(-23.4853259386765,-14.0209982570872,
113.181335126666)) ;
#193825=CARTESIAN_POINT('Ctrl Pts',(-23.5345041189141,-14.2386408615737,
113.36640397491)) ;
#193826=CARTESIAN_POINT('Ctrl Pts',(-23.6001054827243,-14.3991847031552,
113.601804261301)) ;
#193827=CARTESIAN_POINT('Ctrl Pts',(-23.6758396635348,-14.4885294284138,
113.867853985645)) ;
#193828=CARTESIAN_POINT('Ctrl Pts',(-23.7560787132041,-14.5016597743674,
114.147723270265)) ;
#193829=CARTESIAN_POINT('Ctrl Pts',(-23.8342305464961,-14.437009415365,
114.421263368043)) ;
#193830=CARTESIAN_POINT('Ctrl Pts',(-23.9038790142128,-14.2988734246617,
114.668946179201)) ;
#193831=CARTESIAN_POINT('Ctrl Pts',(-23.9589267388881,-14.0989764690058,
114.871924271344)) ;
#193832=CARTESIAN_POINT('Ctrl Pts',(-23.9954157212117,-13.8484694868484,
115.01867831934)) ;
#193833=CARTESIAN_POINT('Ctrl Pts',(-24.0092992091124,-13.5679794956402,
115.096428165126)) ;
#193834=CARTESIAN_POINT('Ctrl Pts',(-23.9992431261541,-13.2778704302602,
115.101136556638)) ;
#193835=CARTESIAN_POINT('Ctrl Pts',(-23.9651195032617,-12.9966579805532,
115.03267001783)) ;
#193836=CARTESIAN_POINT('Ctrl Pts',(-23.9083188929157,-12.7449733317735,
114.895243151894)) ;
#193837=CARTESIAN_POINT('Ctrl Pts',(-23.8326075291051,-12.5424420519023,
114.700085714252)) ;
#193838=CARTESIAN_POINT('Ctrl Pts',(-23.7423558200825,-12.4024494998622,
114.460690641158)) ;
#193839=CARTESIAN_POINT('Ctrl Pts',(-23.6437350301605,-12.33540698977,114.195676204108)) ;
#193840=CARTESIAN_POINT('Ctrl Pts',(-23.54230497616,-12.3455818235887,113.922252265825)) ;
#193841=CARTESIAN_POINT('Ctrl Pts',(-23.4449159493085,-12.433061741337,
113.661165866049)) ;
#193842=CARTESIAN_POINT('Ctrl Pts',(-23.3581859160956,-12.5907670484714,
113.432424558756)) ;
#193843=CARTESIAN_POINT('Ctrl Pts',(-23.2872506370322,-12.8072730343164,
113.25175834982)) ;
#193844=CARTESIAN_POINT('Ctrl Pts',(-23.2361882931638,-13.0681776762317,
113.131728504028)) ;
#193845=CARTESIAN_POINT('Ctrl Pts',(-23.2082374843446,-13.3550287065478,
113.082188386664)) ;
#193846=CARTESIAN_POINT('Ctrl Pts',(-23.2046137347424,-13.6436167217993,
113.106398539743)) ;
#193847=CARTESIAN_POINT('Ctrl Pts',(-23.2246473462219,-13.9180811572707,
113.202915786182)) ;
#193848=CARTESIAN_POINT('Ctrl Pts',(-23.2663198478807,-14.156549136634,
113.365316344901)) ;
#193849=CARTESIAN_POINT('Ctrl Pts',(-23.3260277991125,-14.3423727651068,
113.58274099428)) ;
#193850=CARTESIAN_POINT('Ctrl Pts',(-23.3982430302962,-14.4613427108393,
113.838084052962)) ;
#193851=CARTESIAN_POINT('Ctrl Pts',(-23.4778308247352,-14.5057889124528,
114.116110858595)) ;
#193852=CARTESIAN_POINT('Ctrl Pts',(-23.5571252249388,-14.4724226584541,
114.392900262027)) ;
#193853=CARTESIAN_POINT('Ctrl Pts',(-23.6311473330998,-14.3630839653471,
114.653969620511)) ;
#193854=CARTESIAN_POINT('Ctrl Pts',(-23.6926670750486,-14.1865023299291,
114.87674421223)) ;
#193855=CARTESIAN_POINT('Ctrl Pts',(-23.737109657086,-13.9552367476643,
115.047514669265)) ;
#193856=CARTESIAN_POINT('Ctrl Pts',(-23.7605010634612,-13.6844063432408,
115.1543055001)) ;
#193857=CARTESIAN_POINT('Ctrl Pts',(-23.760236922336,-13.395616216205,115.188901213406)) ;
#193858=CARTESIAN_POINT('Ctrl Pts',(-23.7358042656124,-13.1080920804484,
115.149918807693)) ;
#193859=CARTESIAN_POINT('Ctrl Pts',(-23.6876957397051,-12.8414911099526,
115.039017564153)) ;
#193860=CARTESIAN_POINT('Ctrl Pts',(-23.6196197911873,-12.6185827250958,
114.866926329754)) ;
#193861=CARTESIAN_POINT('Ctrl Pts',(-23.5344644232555,-12.4509854490646,
114.643132785995)) ;
#193862=CARTESIAN_POINT('Ctrl Pts',(-23.4384531446303,-12.3534810644787,
114.386130027561)) ;
#193863=CARTESIAN_POINT('Ctrl Pts',(-23.3373005505562,-12.3320089256095,
114.113522831925)) ;
#193864=CARTESIAN_POINT('Ctrl Pts',(-23.2376722572993,-12.3884256006082,
113.845536510079)) ;
#193865=CARTESIAN_POINT('Ctrl Pts',(-23.1459449956219,-12.5185566369419,
113.601605269859)) ;
#193866=CARTESIAN_POINT('Ctrl Pts',(-23.0678884204578,-12.7128146761132,
113.399287149443)) ;
#193867=CARTESIAN_POINT('Ctrl Pts',(-23.0080726213499,-12.9591843124397,
113.25274040277)) ;
#193868=CARTESIAN_POINT('Ctrl Pts',(-22.9707781839292,-13.2359003760254,
113.174438606138)) ;
#193869=CARTESIAN_POINT('Ctrl Pts',(-22.9571487392571,-13.5269168879405,
113.168395654949)) ;
#193870=CARTESIAN_POINT('Ctrl Pts',(-22.9677330810903,-13.8100818853549,
113.236088284649)) ;
#193871=CARTESIAN_POINT('Ctrl Pts',(-23.0011086677166,-14.0658493622321,
113.373303697314)) ;
#193872=CARTESIAN_POINT('Ctrl Pts',(-23.0539725203832,-14.2744004374724,
113.569778136137)) ;
#193873=CARTESIAN_POINT('Ctrl Pts',(-23.1216893204055,-14.4215076088756,
113.811439149396)) ;
#193874=CARTESIAN_POINT('Ctrl Pts',(-23.1988440710271,-14.4970287487176,
114.081882466236)) ;
#193875=CARTESIAN_POINT('Ctrl Pts',(-23.2792349709217,-14.495364180026,
114.362233916425)) ;
#193876=CARTESIAN_POINT('Ctrl Pts',(-23.3563637359517,-14.4159600881982,
114.632728072821)) ;
#193877=CARTESIAN_POINT('Ctrl Pts',(-23.4233024681412,-14.2660479877099,
114.871922390373)) ;
#193878=CARTESIAN_POINT('Ctrl Pts',(-23.4754105644669,-14.0549162780305,
115.066119893745)) ;
#193879=CARTESIAN_POINT('Ctrl Pts',(-23.5077572471595,-13.7973888984154,
115.200198351239)) ;
#193880=CARTESIAN_POINT('Ctrl Pts',(-23.5172572061641,-13.5143192821472,
115.264479052943)) ;
#193881=CARTESIAN_POINT('Ctrl Pts',(-23.5025567461663,-13.2228141005811,
115.255249135668)) ;
#193882=CARTESIAN_POINT('Ctrl Pts',(-23.4640229788602,-12.9463122499942,
115.173287772294)) ;
#193883=CARTESIAN_POINT('Ctrl Pts',(-23.4033068584606,-12.7025112775513,
115.023933887441)) ;
#193884=CARTESIAN_POINT('Ctrl Pts',(-23.3247469439269,-12.5113386435153,
114.819989036996)) ;
#193885=CARTESIAN_POINT('Ctrl Pts',(-23.2322554152184,-12.3839986409936,
114.573835678973)) ;
#193886=CARTESIAN_POINT('Ctrl Pts',(-23.1325124738357,-12.3313598679509,
114.305463729675)) ;
#193887=CARTESIAN_POINT('Ctrl Pts',(-23.0315695868954,-12.3561484752169,
114.033447032347)) ;
#193888=CARTESIAN_POINT('Ctrl Pts',(-22.9354487583315,-12.4578681360596,
113.776309520322)) ;
#193889=CARTESIAN_POINT('Ctrl Pts',(-22.8516194022014,-12.6270814220524,
113.556268256684)) ;
#193890=CARTESIAN_POINT('Ctrl Pts',(-22.7839838450555,-12.8533401319523,
113.385716322209)) ;
#193891=CARTESIAN_POINT('Ctrl Pts',(-22.737057523416,-13.1210491167834,
113.278349913962)) ;
#193892=CARTESIAN_POINT('Ctrl Pts',(-22.7137114782824,-13.40900770729,113.242669521787)) ;
#193893=CARTESIAN_POINT('Ctrl Pts',(-22.7145790475153,-13.6972694862933,
113.280702081642)) ;
#193894=CARTESIAN_POINT('Ctrl Pts',(-22.73888971428,-13.9663054532962,113.390221067271)) ;
#193895=CARTESIAN_POINT('Ctrl Pts',(-22.7845308373615,-14.1969043333081,
113.564878486232)) ;
#193896=CARTESIAN_POINT('Ctrl Pts',(-22.8467313080852,-14.3698914257013,
113.789672047739)) ;
#193897=CARTESIAN_POINT('Ctrl Pts',(-22.9207425971933,-14.4755193866787,
114.050515802976)) ;
#193898=CARTESIAN_POINT('Ctrl Pts',(-23.0006816978968,-14.5054697818126,
114.329505017033)) ;
#193899=CARTESIAN_POINT('Ctrl Pts',(-23.0797492263395,-14.4574393177702,
114.6057916227)) ;
#193900=CARTESIAN_POINT('Ctrl Pts',(-23.1516520346911,-14.3349211938034,
114.860267274073)) ;
#193901=CARTESIAN_POINT('Ctrl Pts',(-23.2103873638468,-14.1470800055845,
115.074578542204)) ;
#193902=CARTESIAN_POINT('Ctrl Pts',(-23.2512289756988,-13.9065331674936,
115.234478316148)) ;
#193903=CARTESIAN_POINT('Ctrl Pts',(-23.2702582801817,-13.630738678715,
115.327956236279)) ;
#193904=CARTESIAN_POINT('Ctrl Pts',(-23.2654718156878,-13.3408270196336,
115.34875619149)) ;
#193905=CARTESIAN_POINT('Ctrl Pts',(-23.2364052797184,-13.0553492265632,
115.295741122605)) ;
#193906=CARTESIAN_POINT('Ctrl Pts',(-23.184450119502,-12.7963986353394,
115.172941175961)) ;
#193907=CARTESIAN_POINT('Ctrl Pts',(-23.112508885965,-12.581755675213,114.98929825524)) ;
#193908=CARTESIAN_POINT('Ctrl Pts',(-23.0250710503237,-12.4271874700909,
114.758426315697)) ;
#193909=CARTESIAN_POINT('Ctrl Pts',(-22.9276247608224,-12.3434882644401,
114.49706508371)) ;
#193910=CARTESIAN_POINT('Ctrl Pts',(-22.826190770514,-12.3367187774922,
114.223618478407)) ;
#193911=CARTESIAN_POINT('Ctrl Pts',(-22.7275355764204,-12.4076100218016,
113.958611864948)) ;
#193912=CARTESIAN_POINT('Ctrl Pts',(-22.6381489586998,-12.5503272886106,
113.721728947846)) ;
#193913=CARTESIAN_POINT('Ctrl Pts',(-22.5630668542689,-12.7556871760659,
113.528549608634)) ;
#193914=CARTESIAN_POINT('Ctrl Pts',(-22.5073121196337,-13.0091921750313,
113.394296840887)) ;
#193915=CARTESIAN_POINT('Ctrl Pts',(-22.4743110003687,-13.2902503547293,
113.32912295841)) ;
#193916=CARTESIAN_POINT('Ctrl Pts',(-22.4652747457874,-13.5823834440121,
113.337185548665)) ;
#193917=CARTESIAN_POINT('Ctrl Pts',(-22.4804477896373,-13.8618181146796,
113.418880666887)) ;
#193918=CARTESIAN_POINT('Ctrl Pts',(-22.517518476082,-14.1083106024044,
113.567088552821)) ;
#193919=CARTESIAN_POINT('Ctrl Pts',(-22.5736052210533,-14.3070623418306,
113.773452298608)) ;
#193920=CARTESIAN_POINT('Ctrl Pts',(-22.6439238545744,-14.4418892785907,
114.023216814566)) ;
#193921=CARTESIAN_POINT('Ctrl Pts',(-22.7221906575843,-14.502692884587,
114.29704932502)) ;
#193922=CARTESIAN_POINT('Ctrl Pts',(-22.8020413108005,-14.4862255258319,
114.575584821507)) ;
#193923=CARTESIAN_POINT('Ctrl Pts',(-22.877609829832,-14.3934141564473,
114.841215988645)) ;
#193924=CARTESIAN_POINT('Ctrl Pts',(-22.9425681516689,-14.2302607448999,
115.074611405796)) ;
#193925=CARTESIAN_POINT('Ctrl Pts',(-22.9912511714667,-14.0081666908763,
115.258483536822)) ;
#193926=CARTESIAN_POINT('Ctrl Pts',(-23.0192337790016,-13.7466548362381,
115.378918754356)) ;
#193927=CARTESIAN_POINT('Ctrl Pts',(-23.0243744063994,-13.4587847124533,
115.430169417964)) ;
#193928=CARTESIAN_POINT('Ctrl Pts',(-23.0049652251957,-13.1685102080527,
115.4065743669)) ;
#193929=CARTESIAN_POINT('Ctrl Pts',(-22.9622751071858,-12.8978336872395,
115.311834565575)) ;
#193930=CARTESIAN_POINT('Ctrl Pts',(-22.8977448880343,-12.6619537350285,
115.150913911777)) ;
#193931=CARTESIAN_POINT('Ctrl Pts',(-22.8158701194052,-12.4816257056073,
114.937014037923)) ;
#193932=CARTESIAN_POINT('Ctrl Pts',(-22.7221314995921,-12.3684889471066,
114.686813418536)) ;
#193933=CARTESIAN_POINT('Ctrl Pts',(-22.6211642213523,-12.3299903879882,
114.414896154153)) ;
#193934=CARTESIAN_POINT('Ctrl Pts',(-22.5210459323926,-12.3696139932957,
114.145284395622)) ;
#193935=CARTESIAN_POINT('Ctrl Pts',(-22.4270329126327,-12.4839372794238,
113.894388923213)) ;
#193936=CARTESIAN_POINT('Ctrl Pts',(-22.3450439580957,-12.6667316342934,
113.680343028654)) ;
#193937=CARTESIAN_POINT('Ctrl Pts',(-22.2812994602008,-12.9020313562946,
113.521591306162)) ;
#193938=CARTESIAN_POINT('Ctrl Pts',(-22.2388473261469,-13.1740426154344,
113.427694180976)) ;
#193939=CARTESIAN_POINT('Ctrl Pts',(-22.2199943655419,-13.4634545824485,
113.40566955685)) ;
#193940=CARTESIAN_POINT('Ctrl Pts',(-22.2254048356507,-13.7505708131454,
113.45766775839)) ;
#193941=CARTESIAN_POINT('Ctrl Pts',(-22.253988225315,-14.0133363300327,
113.580184190739)) ;
#193942=CARTESIAN_POINT('Ctrl Pts',(-22.302884463881,-14.2335678065818,
113.764575325811)) ;
#193943=CARTESIAN_POINT('Ctrl Pts',(-22.3681132301931,-14.3958087768564,
113.998825699408)) ;
#193944=CARTESIAN_POINT('Ctrl Pts',(-22.443875331704,-14.4872051600084,
114.265066140511)) ;
#193945=CARTESIAN_POINT('Ctrl Pts',(-22.5236867142171,-14.5023836342265,
114.543451391417)) ;
#193946=CARTESIAN_POINT('Ctrl Pts',(-22.6023114828813,-14.4395233841403,
114.8185888207)) ;
#193947=CARTESIAN_POINT('Ctrl Pts',(-22.6719122092473,-14.3038981389521,
115.065942143316)) ;
#193948=CARTESIAN_POINT('Ctrl Pts',(-22.7275755368524,-14.1052991872385,
115.270872462987)) ;
#193949=CARTESIAN_POINT('Ctrl Pts',(-22.7645650054977,-13.8563431079666,
115.419085314818)) ;
#193950=CARTESIAN_POINT('Ctrl Pts',(-22.7791798044281,-13.5768529523028,
115.499023031472)) ;
#193951=CARTESIAN_POINT('Ctrl Pts',(-22.7697827423378,-13.2855121533732,
115.505888509514)) ;
#193952=CARTESIAN_POINT('Ctrl Pts',(-22.736267599059,-13.0041275578471,
115.439237761638)) ;
#193953=CARTESIAN_POINT('Ctrl Pts',(-22.6804050530378,-12.7524010633512,
115.304496989377)) ;
#193954=CARTESIAN_POINT('Ctrl Pts',(-22.6049368462365,-12.5474082659178,
115.110214285938)) ;
#193955=CARTESIAN_POINT('Ctrl Pts',(-22.5152721436028,-12.4057612857423,
114.872509443197)) ;
#193956=CARTESIAN_POINT('Ctrl Pts',(-22.416477982246,-12.3361751661113,
114.607093665793)) ;
#193957=CARTESIAN_POINT('Ctrl Pts',(-22.3151654199719,-12.3442704255669,
114.333978009921)) ;
#193958=CARTESIAN_POINT('Ctrl Pts',(-22.2178317346334,-12.4291570429794,
114.072959782331)) ;
#193959=CARTESIAN_POINT('Ctrl Pts',(-22.1305576720065,-12.5849331529663,
113.842608904662)) ;
#193960=CARTESIAN_POINT('Ctrl Pts',(-22.0589049961337,-12.8005108515807,
113.659850775532)) ;
#193961=CARTESIAN_POINT('Ctrl Pts',(-22.0073169664416,-13.060269126664,
113.538192775077)) ;
#193962=CARTESIAN_POINT('Ctrl Pts',(-21.978691089474,-13.3453693583979,
113.486439374298)) ;
#193963=CARTESIAN_POINT('Ctrl Pts',(-21.9743140972656,-13.6361640667827,
113.508607131723)) ;
#193964=CARTESIAN_POINT('Ctrl Pts',(-21.9936997725589,-13.9104324089111,
113.603035067072)) ;
#193965=CARTESIAN_POINT('Ctrl Pts',(-22.0347431039267,-14.1501784561149,
113.763511943349)) ;
#193966=CARTESIAN_POINT('Ctrl Pts',(-22.0939751521265,-14.3377944456025,
113.979478469494)) ;
#193967=CARTESIAN_POINT('Ctrl Pts',(-22.1659929301065,-14.4588735568458,
114.234265903067)) ;
#193968=CARTESIAN_POINT('Ctrl Pts',(-22.2451385688619,-14.5056122473976,
114.510797193633)) ;
#193969=CARTESIAN_POINT('Ctrl Pts',(-22.324940686415,-14.4743736272664,
114.789329071983)) ;
#193970=CARTESIAN_POINT('Ctrl Pts',(-22.3988824387203,-14.3676054099568,
115.049984802301)) ;
#193971=CARTESIAN_POINT('Ctrl Pts',(-22.4609934584054,-14.1926642104704,
115.274637530722)) ;
#193972=CARTESIAN_POINT('Ctrl Pts',(-22.5060098471497,-13.9629645552833,
115.447132030502)) ;
#193973=CARTESIAN_POINT('Ctrl Pts',(-22.5301282053753,-13.6916669453695,
115.556308146258)) ;
#193974=CARTESIAN_POINT('Ctrl Pts',(-22.5305152960144,-13.4042886281479,
115.592739547311)) ;
#193975=CARTESIAN_POINT('Ctrl Pts',(-22.5067605017534,-13.1160881842174,
115.55586845108)) ;
#193976=CARTESIAN_POINT('Ctrl Pts',(-22.4595154178549,-12.8495738757798,
115.447455103037)) ;
#193977=CARTESIAN_POINT('Ctrl Pts',(-22.3918481625051,-12.6242652876755,
115.276723191289)) ;
#193978=CARTESIAN_POINT('Ctrl Pts',(-22.3066463098264,-12.4543477917217,
115.052950743928)) ;
#193979=CARTESIAN_POINT('Ctrl Pts',(-22.2113534668614,-12.3553371823295,
114.797951573092)) ;
#193980=CARTESIAN_POINT('Ctrl Pts',(-22.1099317335009,-12.3315537600446,
114.524642057895)) ;
#193981=CARTESIAN_POINT('Ctrl Pts',(-22.010593220664,-12.3856473127391,
114.257389293014)) ;
#193982=CARTESIAN_POINT('Ctrl Pts',(-21.9183564548921,-12.513656004823,
114.011961870334)) ;
#193983=CARTESIAN_POINT('Ctrl Pts',(-21.839571054505,-12.707439556573,113.807586885716)) ;
#193984=CARTESIAN_POINT('Ctrl Pts',(-21.7797609837458,-12.9500051005904,
113.660688819678)) ;
#193985=CARTESIAN_POINT('Ctrl Pts',(-21.741415490494,-13.2274462581565,
113.579389468672)) ;
#193986=CARTESIAN_POINT('Ctrl Pts',(-21.7271451352815,-13.5192262317475,
113.571491516801)) ;
#193987=CARTESIAN_POINT('Ctrl Pts',(-21.7370271436767,-13.8018769048648,
113.636919707644)) ;
#193988=CARTESIAN_POINT('Ctrl Pts',(-21.7697376558309,-14.058784271986,
113.772109441117)) ;
#193989=CARTESIAN_POINT('Ctrl Pts',(-21.8220819037483,-14.2690401451517,
113.967006518844)) ;
#193990=CARTESIAN_POINT('Ctrl Pts',(-21.8895943124559,-14.418345814643,
114.208124022186)) ;
#193991=CARTESIAN_POINT('Ctrl Pts',(-21.966477791396,-14.4960013207205,
114.477695371654)) ;
#193992=CARTESIAN_POINT('Ctrl Pts',(-22.0471672488081,-14.4962457299704,
114.759096539096)) ;
#193993=CARTESIAN_POINT('Ctrl Pts',(-22.1237856140213,-14.4198799151553,
115.027702043525)) ;
#193994=CARTESIAN_POINT('Ctrl Pts',(-22.1916978524243,-14.2709014086462,
115.270163302908)) ;
#193995=CARTESIAN_POINT('Ctrl Pts',(-22.244095479827,-14.0614284920593,
115.465166551261)) ;
#193996=CARTESIAN_POINT('Ctrl Pts',(-22.2770600984898,-13.8059370930909,
115.601015529285)) ;
#193997=CARTESIAN_POINT('Ctrl Pts',(-22.2872367367097,-13.5211628984478,
115.667631143365)) ;
#193998=CARTESIAN_POINT('Ctrl Pts',(-22.2733014770103,-13.2317212421624,
115.660460390471)) ;
#193999=CARTESIAN_POINT('Ctrl Pts',(-22.2352493339622,-12.953209842425,
115.580148172852)) ;
#194000=CARTESIAN_POINT('Ctrl Pts',(-22.1754856836276,-12.7094642616823,
115.433485637688)) ;
#194001=CARTESIAN_POINT('Ctrl Pts',(-22.0966448910796,-12.5150572905195,
115.22901210739)) ;
#194002=CARTESIAN_POINT('Ctrl Pts',(-22.0054187277231,-12.3871819681861,
114.986327553014)) ;
#194003=CARTESIAN_POINT('Ctrl Pts',(-21.905263733452,-12.3316884564228,
114.716909806915)) ;
#194004=CARTESIAN_POINT('Ctrl Pts',(-21.8045903005962,-12.3542922095437,
114.445593550072)) ;
#194005=CARTESIAN_POINT('Ctrl Pts',(-21.7081146500002,-12.4537268763868,
114.187411168182)) ;
#194006=CARTESIAN_POINT('Ctrl Pts',(-21.6237862011861,-12.6212675456056,
113.965882774821)) ;
#194007=CARTESIAN_POINT('Ctrl Pts',(-21.5556046478956,-12.846192059173,
113.793679096726)) ;
#194008=CARTESIAN_POINT('Ctrl Pts',(-21.5080827888729,-13.1124184461725,
113.684427311798)) ;
#194009=CARTESIAN_POINT('Ctrl Pts',(-21.483971454148,-13.400879749144,113.646523677771)) ;
#194010=CARTESIAN_POINT('Ctrl Pts',(-21.4841119720974,-13.6891262166377,
113.682294540054)) ;
#194011=CARTESIAN_POINT('Ctrl Pts',(-21.5080695511385,-13.9605413879786,
113.790974309993)) ;
#194012=CARTESIAN_POINT('Ctrl Pts',(-21.5525393505442,-14.1894540736428,
113.961580396736)) ;
#194013=CARTESIAN_POINT('Ctrl Pts',(-21.6146814088062,-14.3660067048925,
114.186472926776)) ;
#194014=CARTESIAN_POINT('Ctrl Pts',(-21.6884351663154,-14.4734792612079,
114.446508526122)) ;
#194015=CARTESIAN_POINT('Ctrl Pts',(-21.7683784809354,-14.5056975632985,
114.725551946228)) ;
#194016=CARTESIAN_POINT('Ctrl Pts',(-21.8474157178673,-14.4599236721213,
115.001679784935)) ;
#194017=CARTESIAN_POINT('Ctrl Pts',(-21.9195991566158,-14.3395761921465,
115.257002682461)) ;
#194018=CARTESIAN_POINT('Ctrl Pts',(-21.9788462429372,-14.1535350418836,
115.472880057577)) ;
#194019=CARTESIAN_POINT('Ctrl Pts',(-22.0203775008148,-13.9130985111844,
115.635036561647)) ;
#194020=CARTESIAN_POINT('Ctrl Pts',(-22.0399483640035,-13.6395736822347,
115.72995984664)) ;
#194021=CARTESIAN_POINT('Ctrl Pts',(-22.0358686869632,-13.3487006076146,
115.75305462755)) ;
#194022=CARTESIAN_POINT('Ctrl Pts',(-22.0075438310689,-13.0636371844073,
115.70218883906)) ;
#194023=CARTESIAN_POINT('Ctrl Pts',(-21.9561819767785,-12.803286823163,
115.581244291729)) ;
#194024=CARTESIAN_POINT('Ctrl Pts',(-21.8847933182746,-12.5872505028287,
115.399264233317)) ;
#194025=CARTESIAN_POINT('Ctrl Pts',(-21.7976012004924,-12.4304809457012,
115.169196272267)) ;
#194026=CARTESIAN_POINT('Ctrl Pts',(-21.700169966331,-12.3447676693836,
114.907940821846)) ;
#194027=CARTESIAN_POINT('Ctrl Pts',(-21.5992738440407,-12.3358385329225,
114.635951321801)) ;
#194028=CARTESIAN_POINT('Ctrl Pts',(-21.5003785782672,-12.4042599768703,
114.370232214751)) ;
#194029=CARTESIAN_POINT('Ctrl Pts',(-21.4104042015346,-12.5454038835963,
114.131652978612)) ;
#194030=CARTESIAN_POINT('Ctrl Pts',(-21.3349456169578,-12.7490645526663,
113.9372922249)) ;
#194031=CARTESIAN_POINT('Ctrl Pts',(-21.278705237238,-13.0004109945635,
113.801433245637)) ;
#194032=CARTESIAN_POINT('Ctrl Pts',(-21.2448570719353,-13.281956740539,
113.733818494743)) ;
#194033=CARTESIAN_POINT('Ctrl Pts',(-21.2351498447256,-13.573019683806,
113.739702682927)) ;
#194034=CARTESIAN_POINT('Ctrl Pts',(-21.2495046916565,-13.8532505028034,
113.818910957215)) ;
#194035=CARTESIAN_POINT('Ctrl Pts',(-21.2861585371864,-14.1021597581384,
113.966023254985)) ;
#194036=CARTESIAN_POINT('Ctrl Pts',(-21.3416525533176,-14.3018608409922,
114.170484973414)) ;
#194037=CARTESIAN_POINT('Ctrl Pts',(-21.411315277641,-14.4384983198451,
114.418115610093)) ;
#194038=CARTESIAN_POINT('Ctrl Pts',(-21.4896790967479,-14.5020770602936,
114.692365991293)) ;
#194039=CARTESIAN_POINT('Ctrl Pts',(-21.5697542529171,-14.48777877411,114.971664919752)) ;
#194040=CARTESIAN_POINT('Ctrl Pts',(-21.6455150626232,-14.3970097456745,
115.237875186916)) ;
#194041=CARTESIAN_POINT('Ctrl Pts',(-21.7106846353234,-14.2362612997962,
115.471811422078)) ;
#194042=CARTESIAN_POINT('Ctrl Pts',(-21.7599663610644,-14.0159101115065,
115.65749922043)) ;
#194043=CARTESIAN_POINT('Ctrl Pts',(-21.7887254354454,-13.7543350935969,
115.7804395058)) ;
#194044=CARTESIAN_POINT('Ctrl Pts',(-21.7944517107035,-13.4665595551094,
115.833506874945)) ;
#194045=CARTESIAN_POINT('Ctrl Pts',(-21.7759076496093,-13.1776643244991,
115.812347038779)) ;
#194046=CARTESIAN_POINT('Ctrl Pts',(-21.7336480522878,-12.90467088677,115.719119626664)) ;
#194047=CARTESIAN_POINT('Ctrl Pts',(-21.670032619818,-12.6688603640825,
115.560779753081)) ;
#194048=CARTESIAN_POINT('Ctrl Pts',(-21.5885287279957,-12.48602188738,115.348081223403)) ;
#194049=CARTESIAN_POINT('Ctrl Pts',(-21.4945267923872,-12.3704601308902,
115.097266800152)) ;
#194050=CARTESIAN_POINT('Ctrl Pts',(-21.3942570657881,-12.3301504850153,
114.827261741778)) ;
#194051=CARTESIAN_POINT('Ctrl Pts',(-21.2939223840727,-12.3670848663884,
114.557023720825)) ;
#194052=CARTESIAN_POINT('Ctrl Pts',(-21.1989536269659,-12.4806961242678,
114.303499956068)) ;
#194053=CARTESIAN_POINT('Ctrl Pts',(-21.1174616220678,-12.659847054779,
114.090572179847)) ;
#194054=CARTESIAN_POINT('Ctrl Pts',(-21.0527943299023,-12.8944266812495,
113.929149642183)) ;
#194055=CARTESIAN_POINT('Ctrl Pts',(-21.009715412858,-13.1656332510844,
113.833333116255)) ;
#194056=CARTESIAN_POINT('Ctrl Pts',(-20.9901169836703,-13.455130793988,
113.809077738093)) ;
#194057=CARTESIAN_POINT('Ctrl Pts',(-20.9948751859287,-13.7427936624919,
113.859110662264)) ;
#194058=CARTESIAN_POINT('Ctrl Pts',(-21.0227622802631,-14.0059776158613,
113.979433797495)) ;
#194059=CARTESIAN_POINT('Ctrl Pts',(-21.0711237055155,-14.2279037819529,
114.162216793604)) ;
#194060=CARTESIAN_POINT('Ctrl Pts',(-21.1359737665809,-14.3919406672911,
114.39531754647)) ;
#194061=CARTESIAN_POINT('Ctrl Pts',(-21.211254131552,-14.4855253459423,
114.659978503316)) ;
#194062=CARTESIAN_POINT('Ctrl Pts',(-21.2915339470349,-14.5029122651219,
114.940022641269)) ;
#194063=CARTESIAN_POINT('Ctrl Pts',(-21.3695938610987,-14.4429567945224,
115.213104290298)) ;
#194064=CARTESIAN_POINT('Ctrl Pts',(-21.4400444498509,-14.3088313127917,
115.463288416723)) ;
#194065=CARTESIAN_POINT('Ctrl Pts',(-21.4961500025639,-14.1118280044828,
115.669548634659)) ;
#194066=CARTESIAN_POINT('Ctrl Pts',(-21.5338004050003,-13.8633524569287,
115.819871913818)) ;
#194067=CARTESIAN_POINT('Ctrl Pts',(-21.5489972331909,-13.5856086171591,
115.901434129162)) ;
#194068=CARTESIAN_POINT('Ctrl Pts',(-21.540363783719,-13.29429050433,115.910632149051)) ;
#194069=CARTESIAN_POINT('Ctrl Pts',(-21.5075688559681,-13.0122145331766,
115.846182232389)) ;
#194070=CARTESIAN_POINT('Ctrl Pts',(-21.4520578760768,-12.7583429519339,
115.712662082996)) ;
#194071=CARTESIAN_POINT('Ctrl Pts',(-21.377127791228,-12.5522896132778,
115.51996437081)) ;
#194072=CARTESIAN_POINT('Ctrl Pts',(-21.2880636112646,-12.4090180636989,
115.283992249369)) ;
#194073=CARTESIAN_POINT('Ctrl Pts',(-21.1893528871873,-12.3371174607651,
115.018865437518)) ;
#194074=CARTESIAN_POINT('Ctrl Pts',(-21.0881345102603,-12.3428658905722,
114.745994676073)) ;
#194075=CARTESIAN_POINT('Ctrl Pts',(-20.9904482281693,-12.4257351119528,
114.483961462618)) ;
#194076=CARTESIAN_POINT('Ctrl Pts',(-20.9030223342738,-12.5790185234623,
114.253042471409)) ;
#194077=CARTESIAN_POINT('Ctrl Pts',(-20.8305192061514,-12.7940406828703,
114.067860324909)) ;
#194078=CARTESIAN_POINT('Ctrl Pts',(-20.7785061884323,-13.0518842131347,
113.944776920917)) ;
#194079=CARTESIAN_POINT('Ctrl Pts',(-20.74911735469,-13.3370763555055,113.890776267983)) ;
#194080=CARTESIAN_POINT('Ctrl Pts',(-20.7440079729999,-13.6270297095458,
113.910587476447)) ;
#194081=CARTESIAN_POINT('Ctrl Pts',(-20.7628136407268,-13.9038567932623,
114.003478096107)) ;
#194082=CARTESIAN_POINT('Ctrl Pts',(-20.8034569028155,-14.1447030861545,
114.162759758855)) ;
#194083=CARTESIAN_POINT('Ctrl Pts',(-20.8618372427062,-14.332817774621,
114.375897727997)) ;
#194084=CARTESIAN_POINT('Ctrl Pts',(-20.9337388829321,-14.45646682902,114.630435787986)) ;
#194085=CARTESIAN_POINT('Ctrl Pts',(-21.0127215247643,-14.5053560860543,
114.906444434635)) ;
#194086=CARTESIAN_POINT('Ctrl Pts',(-21.0928080257603,-14.4762759602464,
115.185935827809)) ;
#194087=CARTESIAN_POINT('Ctrl Pts',(-21.166945453464,-14.3712943997113,
115.44718234613)) ;
#194088=CARTESIAN_POINT('Ctrl Pts',(-21.22925533612,-14.1990455522355,115.672287786187)) ;
#194089=CARTESIAN_POINT('Ctrl Pts',(-21.275036309889,-13.969268231171,115.847326008971)) ;
#194090=CARTESIAN_POINT('Ctrl Pts',(-21.2996282826531,-13.7012052922517,
115.957629225369)) ;
#194091=CARTESIAN_POINT('Ctrl Pts',(-21.300776790549,-13.4115854195081,
115.996699140416)) ;
#194092=CARTESIAN_POINT('Ctrl Pts',(-21.2776657782434,-13.1240520278943,
115.961667884177)) ;
#194093=CARTESIAN_POINT('Ctrl Pts',(-21.2310997495999,-12.8565945311091,
115.85532524094)) ;
#194094=CARTESIAN_POINT('Ctrl Pts',(-21.1639038965067,-12.6299321000607,
115.686042104693)) ;
#194095=CARTESIAN_POINT('Ctrl Pts',(-21.0795308737286,-12.458754218581,
115.464633703423)) ;
#194096=CARTESIAN_POINT('Ctrl Pts',(-20.9840008114821,-12.3569969390507,
115.209096703892)) ;
#194097=CARTESIAN_POINT('Ctrl Pts',(-20.8827940549326,-12.3311725454961,
114.936383442419)) ;
#194098=CARTESIAN_POINT('Ctrl Pts',(-20.7831194155453,-12.3830921654557,
114.668177530527)) ;
#194099=CARTESIAN_POINT('Ctrl Pts',(-20.6905057252182,-12.5097082549453,
114.421659452315)) ;
#194100=CARTESIAN_POINT('Ctrl Pts',(-20.611889484645,-12.6999655173835,
114.217488910924)) ;
#194101=CARTESIAN_POINT('Ctrl Pts',(-20.5509672408573,-12.9431519741363,
114.067493771152)) ;
#194102=CARTESIAN_POINT('Ctrl Pts',(-20.5121852559406,-13.2187420743147,
113.984700488241)) ;
#194103=CARTESIAN_POINT('Ctrl Pts',(-20.4971344280026,-13.5111774969548,
113.974526122815)) ;
#194104=CARTESIAN_POINT('Ctrl Pts',(-20.5063387268511,-13.7940494918521,
114.037849430853)) ;
#194105=CARTESIAN_POINT('Ctrl Pts',(-20.5386101711866,-14.0529110285333,
114.171842551174)) ;
#194106=CARTESIAN_POINT('Ctrl Pts',(-20.5902344604345,-14.2634870650102,
114.364365229605)) ;
#194107=CARTESIAN_POINT('Ctrl Pts',(-20.6572920468694,-14.4148461022599,
114.60407461122)) ;
#194108=CARTESIAN_POINT('Ctrl Pts',(-20.7340710302273,-14.494780073978,
114.873368689738)) ;
#194109=CARTESIAN_POINT('Ctrl Pts',(-20.814667921946,-14.4974507314962,
115.154444310866)) ;
#194110=CARTESIAN_POINT('Ctrl Pts',(-20.8916746371351,-14.4229495346006,
115.424337435555)) ;
#194111=CARTESIAN_POINT('Ctrl Pts',(-20.9596595247132,-14.2768020033666,
115.6668461103)) ;
#194112=CARTESIAN_POINT('Ctrl Pts',(-21.012974127338,-14.0672719747909,
115.864923528027)) ;
#194113=CARTESIAN_POINT('Ctrl Pts',(-21.0462752479574,-13.8140437794069,
116.001605423442)) ;
#194114=CARTESIAN_POINT('Ctrl Pts',(-21.057235818105,-13.5305545368903,
116.070529359299)) ;
#194115=CARTESIAN_POINT('Ctrl Pts',(-21.0439982208835,-13.2400469135056,
116.065602507524)) ;
#194116=CARTESIAN_POINT('Ctrl Pts',(-21.0066020047252,-12.9607801917685,
115.987295334548)) ;
#194117=CARTESIAN_POINT('Ctrl Pts',(-20.9473443980316,-12.7157522020321,
115.842202222821)) ;
#194118=CARTESIAN_POINT('Ctrl Pts',(-20.8694399766873,-12.5205021117526,
115.640390114338)) ;
#194119=CARTESIAN_POINT('Ctrl Pts',(-20.7779765651367,-12.3896091910669,
115.397208988666)) ;
#194120=CARTESIAN_POINT('Ctrl Pts',(-20.6779561212234,-12.3322116649338,
115.128190401515)) ;
#194121=CARTESIAN_POINT('Ctrl Pts',(-20.5774147689211,-12.3526193896652,
114.857217210318)) ;
#194122=CARTESIAN_POINT('Ctrl Pts',(-20.480876963674,-12.4495335034968,
114.598771665885)) ;
#194123=CARTESIAN_POINT('Ctrl Pts',(-20.3957540886572,-12.6159519111974,
114.374983031782)) ;
#194124=CARTESIAN_POINT('Ctrl Pts',(-20.3271536623197,-12.8395609374739,
114.201485817632)) ;
#194125=CARTESIAN_POINT('Ctrl Pts',(-20.2791583118047,-13.1036924153161,
114.090643871318)) ;
#194126=CARTESIAN_POINT('Ctrl Pts',(-20.2542197759365,-13.3927905140901,
114.05034234162)) ;
#194127=CARTESIAN_POINT('Ctrl Pts',(-20.2537651631048,-13.6807940128297,
114.084250210379)) ;
#194128=CARTESIAN_POINT('Ctrl Pts',(-20.2767369580529,-13.9516407801447,
114.189702183706)) ;
#194129=CARTESIAN_POINT('Ctrl Pts',(-20.3212515827195,-14.1848191645832,
114.360909549778)) ;
#194130=CARTESIAN_POINT('Ctrl Pts',(-20.3823727653949,-14.3611535147467,
114.582313485388)) ;
#194131=CARTESIAN_POINT('Ctrl Pts',(-20.4563210601665,-14.4717132500286,
114.843190270097)) ;
#194132=CARTESIAN_POINT('Ctrl Pts',(-20.5359913410577,-14.5058049610956,
115.121300978399)) ;
#194133=CARTESIAN_POINT('Ctrl Pts',(-20.6152285993297,-14.4622432474708,
115.398086166475)) ;
#194134=CARTESIAN_POINT('Ctrl Pts',(-20.6876764922037,-14.343914063795,
115.654200032397)) ;
#194135=CARTESIAN_POINT('Ctrl Pts',(-20.7473748229597,-14.1592285094383,
115.871492526232)) ;
#194136=CARTESIAN_POINT('Ctrl Pts',(-20.7892502687807,-13.9218383285055,
116.034450676081)) ;
#194137=CARTESIAN_POINT('Ctrl Pts',(-20.8096697160064,-13.6477929587425,
116.132141353103)) ;
#194138=CARTESIAN_POINT('Ctrl Pts',(-20.8062757150026,-13.3573882946602,
116.157281504951)) ;
#194139=CARTESIAN_POINT('Ctrl Pts',(-20.7786075112858,-13.0713760146383,
116.108481462324)) ;
#194140=CARTESIAN_POINT('Ctrl Pts',(-20.727862298227,-12.8101300373193,
115.989403245096)) ;
#194141=CARTESIAN_POINT('Ctrl Pts',(-20.6569850715304,-12.5926203368979,
115.808983189136)) ;
#194142=CARTESIAN_POINT('Ctrl Pts',(-20.5702654370651,-12.4341144288436,
115.580315447972)) ;
#194143=CARTESIAN_POINT('Ctrl Pts',(-20.4730652679923,-12.346259851331,
115.319760267267)) ;
#194144=CARTESIAN_POINT('Ctrl Pts',(-20.372232841033,-12.3348158852733,
115.047945482228)) ;
#194145=CARTESIAN_POINT('Ctrl Pts',(-20.272459099619,-12.4019396871859,
114.779822675992)) ;
#194146=CARTESIAN_POINT('Ctrl Pts',(-20.1830070427554,-12.5400212389952,
114.542504031555)) ;
#194147=CARTESIAN_POINT('Ctrl Pts',(-20.1067029971044,-12.7426569389483,
114.345713360105)) ;
#194148=CARTESIAN_POINT('Ctrl Pts',(-20.0499392060894,-12.9928209893326,
114.208234860581)) ;
#194149=CARTESIAN_POINT('Ctrl Pts',(-20.0153853295519,-13.274121349933,
114.138514811439)) ;
#194150=CARTESIAN_POINT('Ctrl Pts',(-20.0050410507883,-13.5650423075934,
114.142439305779)) ;
#194151=CARTESIAN_POINT('Ctrl Pts',(-20.0186971571549,-13.8454220244642,
114.219462038445)) ;
#194152=CARTESIAN_POINT('Ctrl Pts',(-20.0547596385372,-14.095635489283,
114.36479225159)) ;
#194153=CARTESIAN_POINT('Ctrl Pts',(-20.1097879472539,-14.2970558104585,
114.56784725279)) ;
#194154=CARTESIAN_POINT('Ctrl Pts',(-20.1793472667708,-14.4359480747077,
114.815266815336)) ;
#194155=CARTESIAN_POINT('Ctrl Pts',(-20.2575026754292,-14.501304829004,
115.088848135438)) ;
#194156=CARTESIAN_POINT('Ctrl Pts',(-20.3373604074522,-14.4893139259723,
115.367374582084)) ;
#194157=CARTESIAN_POINT('Ctrl Pts',(-20.4135150495728,-14.4004454436412,
115.63486985746)) ;
#194158=CARTESIAN_POINT('Ctrl Pts',(-20.4788768821726,-14.2418718140722,
115.86930035727)) ;
#194159=CARTESIAN_POINT('Ctrl Pts',(-20.5287019786929,-14.0233785235775,
116.056610441429)) ;
#194160=CARTESIAN_POINT('Ctrl Pts',(-20.5581714230433,-13.7618917263419,
116.181832379666)) ;
#194161=CARTESIAN_POINT('Ctrl Pts',(-20.5645519553757,-13.4754623735639,
116.236774706755)) ;
#194162=CARTESIAN_POINT('Ctrl Pts',(-20.5467688213249,-13.1862230579374,
116.217949995558)) ;
#194163=CARTESIAN_POINT('Ctrl Pts',(-20.5051147908571,-12.9121173454345,
116.12661145186)) ;
#194164=CARTESIAN_POINT('Ctrl Pts',(-20.4420769531017,-12.6748571224349,
115.970037261179)) ;
#194165=CARTESIAN_POINT('Ctrl Pts',(-20.3606399883835,-12.4898752939566,
115.757680794649)) ;
#194166=CARTESIAN_POINT('Ctrl Pts',(-20.267669228754,-12.3730682967797,
115.5097223699)) ;
#194167=CARTESIAN_POINT('Ctrl Pts',(-20.166688706548,-12.330125354393,115.237846370994)) ;
#194168=CARTESIAN_POINT('Ctrl Pts',(-20.0667473533349,-12.3650026478225,
114.968634787347)) ;
#194169=CARTESIAN_POINT('Ctrl Pts',(-19.9714448335891,-12.4764750890778,
114.714120708034)) ;
#194170=CARTESIAN_POINT('Ctrl Pts',(-19.8896127307638,-12.6535586984017,
114.500104289073)) ;
#194171=CARTESIAN_POINT('Ctrl Pts',(-19.8242138693162,-12.8875907025722,
114.33656955619)) ;
#194172=CARTESIAN_POINT('Ctrl Pts',(-19.7806786916706,-13.1564738506933,
114.239166113218)) ;
#194173=CARTESIAN_POINT('Ctrl Pts',(-19.7602296026469,-13.4476180482474,
114.212556713675)) ;
#194174=CARTESIAN_POINT('Ctrl Pts',(-19.7643490688689,-13.7346448783816,
114.260518004658)) ;
#194175=CARTESIAN_POINT('Ctrl Pts',(-19.7916546783398,-13.9993799399049,
114.37915348673)) ;
#194176=CARTESIAN_POINT('Ctrl Pts',(-19.8393939276307,-14.2219559568416,
114.559939768172)) ;
#194177=CARTESIAN_POINT('Ctrl Pts',(-19.9035549276073,-14.3877271051732,
114.790823935463)) ;
#194178=CARTESIAN_POINT('Ctrl Pts',(-19.9791956729631,-14.4840522417127,
115.05686055136)) ;
#194179=CARTESIAN_POINT('Ctrl Pts',(-20.0588167420593,-14.5035551456864,
115.334617178698)) ;
#194180=CARTESIAN_POINT('Ctrl Pts',(-20.1375552337769,-14.4455933724693,
115.610012047624)) ;
#194181=CARTESIAN_POINT('Ctrl Pts',(-20.2080701569904,-14.3137077173971,
115.860269168483)) ;
#194182=CARTESIAN_POINT('Ctrl Pts',(-20.2646911851614,-14.118290994482,
116.068126903514)) ;
#194183=CARTESIAN_POINT('Ctrl Pts',(-20.3028224443455,-13.8721339097932,
116.21976440383)) ;
#194184=CARTESIAN_POINT('Ctrl Pts',(-20.3188675383437,-13.5943341067766,
116.304015063102)) ;
#194185=CARTESIAN_POINT('Ctrl Pts',(-20.310817084727,-13.3016132059809,
116.315163697483)) ;
#194186=CARTESIAN_POINT('Ctrl Pts',(-20.2787910861107,-13.0203974601351,
116.252886906067)) ;
#194187=CARTESIAN_POINT('Ctrl Pts',(-20.2240804356435,-12.7657619407627,
116.121738912419)) ;
#194188=CARTESIAN_POINT('Ctrl Pts',(-20.149613612166,-12.5577255499837,
115.930492489718)) ;
#194189=CARTESIAN_POINT('Ctrl Pts',(-20.0607208453583,-12.4120606642955,
115.695117936638)) ;
#194190=CARTESIAN_POINT('Ctrl Pts',(-19.9618159399851,-12.3380220880362,
115.429525652929)) ;
#194191=CARTESIAN_POINT('Ctrl Pts',(-19.8611741252131,-12.3416277493325,
115.158205582033)) ;
#194192=CARTESIAN_POINT('Ctrl Pts',(-19.7631652821149,-12.4221117178776,
114.895226151352)) ;
#194193=CARTESIAN_POINT('Ctrl Pts',(-19.6752313663645,-12.5739000669618,
114.662827645649)) ;
#194194=CARTESIAN_POINT('Ctrl Pts',(-19.6024167491396,-12.7865530350162,
114.47657434342)) ;
#194195=CARTESIAN_POINT('Ctrl Pts',(-19.5495231103684,-13.044698151263,
114.350994766483)) ;
#194196=CARTESIAN_POINT('Ctrl Pts',(-19.5196225512715,-13.328059924083,
114.29525984895)) ;
#194197=CARTESIAN_POINT('Ctrl Pts',(-19.5137354281578,-13.6187777866059,
114.312782448992)) ;
#194198=CARTESIAN_POINT('Ctrl Pts',(-19.5318785681101,-13.8959727795492,
114.403613733301)) ;
#194199=CARTESIAN_POINT('Ctrl Pts',(-19.5718247752165,-14.1380897314584,
114.560743510385)) ;
#194200=CARTESIAN_POINT('Ctrl Pts',(-19.6301836363791,-14.3289912800735,
114.774053959867)) ;
#194201=CARTESIAN_POINT('Ctrl Pts',(-19.7013725695596,-14.4536834307714,
115.026197380429)) ;
#194202=CARTESIAN_POINT('Ctrl Pts',(-19.7802758537962,-14.5050447602448,
115.301993496295)) ;
#194203=CARTESIAN_POINT('Ctrl Pts',(-19.8602648502565,-14.4782940097224,
115.581115798134)) ;
#194204=CARTESIAN_POINT('Ctrl Pts',(-19.9347147614836,-14.3758709565101,
115.843310818207)) ;
#194205=CARTESIAN_POINT('Ctrl Pts',(-19.9978520690189,-14.2038414128419,
116.071213910054)) ;
#194206=CARTESIAN_POINT('Ctrl Pts',(-20.0437608055394,-13.9777022974474,
116.246290431743)) ;
#194207=CARTESIAN_POINT('Ctrl Pts',(-20.0692545667737,-13.7081471730545,
116.359670607939)) ;
#194208=CARTESIAN_POINT('Ctrl Pts',(-20.0710088126816,-13.4207218926891,
116.400338260626)) ;
#194209=CARTESIAN_POINT('Ctrl Pts',(-20.0486389329938,-13.1323473586493,
116.367635760185)) ;
#194210=CARTESIAN_POINT('Ctrl Pts',(-20.0027585392029,-12.8640039527127,
116.26336619867)) ;
#194211=CARTESIAN_POINT('Ctrl Pts',(-19.935788026807,-12.6351955964259,
116.094916391057)) ;
#194212=CARTESIAN_POINT('Ctrl Pts',(-19.8524350019228,-12.4633049543151,
115.876360547653)) ;
#194213=CARTESIAN_POINT('Ctrl Pts',(-19.7565552164464,-12.3586842738095,
115.619991906947)) ;
#194214=CARTESIAN_POINT('Ctrl Pts',(-19.6559368636795,-12.3308701665295,
115.348879090383)) ;
#194215=CARTESIAN_POINT('Ctrl Pts',(-19.5559630364021,-12.3804185210795,
115.079826490949)) ;
#194216=CARTESIAN_POINT('Ctrl Pts',(-19.4632285523152,-12.5045865657479,
114.832858816864)) ;
#194217=CARTESIAN_POINT('Ctrl Pts',(-19.3838405577288,-12.6936012415773,
114.626458033077)) ;
#194218=CARTESIAN_POINT('Ctrl Pts',(-19.3222105618298,-12.9362801376937,
114.474398641739)) ;
#194219=CARTESIAN_POINT('Ctrl Pts',(-19.2828604657008,-13.2112926431605,
114.389881775346)) ;
#194220=CARTESIAN_POINT('Ctrl Pts',(-19.2671542279157,-13.5026318637497,
114.377588421652)) ;
#194221=CARTESIAN_POINT('Ctrl Pts',(-19.2757419733594,-13.7865927515763,
114.439120363259)) ;
#194222=CARTESIAN_POINT('Ctrl Pts',(-19.3070927419327,-14.0445932154009,
114.570030945766)) ;
#194223=CARTESIAN_POINT('Ctrl Pts',(-19.358347515694,-14.2581092551482,
114.761608730446)) ;
#194224=CARTESIAN_POINT('Ctrl Pts',(-19.4252783091883,-14.4117380229187,
115.001038317045)) ;
#194225=CARTESIAN_POINT('Ctrl Pts',(-19.5019526631148,-14.4936441507055,
115.270046158408)) ;
#194226=CARTESIAN_POINT('Ctrl Pts',(-19.5823198515389,-14.4983888239063,
115.550327419762)) ;
#194227=CARTESIAN_POINT('Ctrl Pts',(-19.6595477418913,-14.426207251784,
115.82090191206)) ;
#194228=CARTESIAN_POINT('Ctrl Pts',(-19.7280764038109,-14.2809809264381,
116.065217208955)) ;
#194229=CARTESIAN_POINT('Ctrl Pts',(-19.7813206021368,-14.0755731076895,
116.262663449883)) ;
#194230=CARTESIAN_POINT('Ctrl Pts',(-19.8156285654698,-13.8214647968314,
116.402723704513)) ;
#194231=CARTESIAN_POINT('Ctrl Pts',(-19.8271835709341,-13.5390721929965,
116.473371097639)) ;
#194232=CARTESIAN_POINT('Ctrl Pts',(-19.8146134378266,-13.2479213210197,
116.470556422711)) ;
#194233=CARTESIAN_POINT('Ctrl Pts',(-19.7780274303114,-12.9689956696526,
116.394584966036)) ;
#194234=CARTESIAN_POINT('Ctrl Pts',(-19.7192534733058,-12.7220961737177,
116.251055118297)) ;
#194235=CARTESIAN_POINT('Ctrl Pts',(-19.6419060205883,-12.5254520180373,
116.050893527524)) ;
#194236=CARTESIAN_POINT('Ctrl Pts',(-19.5507750838464,-12.3924871288094,
115.808727229059)) ;
#194237=CARTESIAN_POINT('Ctrl Pts',(-19.4509678272437,-12.3327720085306,
115.540332649395)) ;
#194238=CARTESIAN_POINT('Ctrl Pts',(-19.3501879158993,-12.3509988977752,
115.268703339782)) ;
#194239=CARTESIAN_POINT('Ctrl Pts',(-19.2537109950385,-12.4453838611795,
115.010328377215)) ;
#194240=CARTESIAN_POINT('Ctrl Pts',(-19.1680396764701,-12.6100760699984,
114.78492817834)) ;
#194241=CARTESIAN_POINT('Ctrl Pts',(-19.0989285208918,-12.8316470477012,
114.609808039742)) ;
#194242=CARTESIAN_POINT('Ctrl Pts',(-19.0499531759888,-13.0973555362981,
114.496308559562)) ;
#194243=CARTESIAN_POINT('Ctrl Pts',(-19.0246223482772,-13.3829827267331,
114.454418834067)) ;
#194244=CARTESIAN_POINT('Ctrl Pts',(-19.0233599186535,-13.6735145155205,
114.486149491012)) ;
#194245=CARTESIAN_POINT('Ctrl Pts',(-19.0457709783456,-13.9443960540442,
114.589809022558)) ;
#194246=CARTESIAN_POINT('Ctrl Pts',(-19.0894428117511,-14.1780473237906,
114.75829138369)) ;
#194247=CARTESIAN_POINT('Ctrl Pts',(-19.1503829732197,-14.3571729772058,
114.97930953691)) ;
#194248=CARTESIAN_POINT('Ctrl Pts',(-19.2242001392869,-14.4697035049953,
115.239834214336)) ;
#194249=CARTESIAN_POINT('Ctrl Pts',(-19.3035102564175,-14.5058316151569,
115.516726782394)) ;
#194250=CARTESIAN_POINT('Ctrl Pts',(-19.3827642308923,-14.4647781183691,
115.793520482864)) ;
#194251=CARTESIAN_POINT('Ctrl Pts',(-19.4555982839664,-14.3484987257117,
116.050853216229)) ;
#194252=CARTESIAN_POINT('Ctrl Pts',(-19.5158156777424,-14.1655053892491,
116.26975198964)) ;
#194253=CARTESIAN_POINT('Ctrl Pts',(-19.5583308176863,-13.9286208259661,
116.434763630565)) ;
#194254=CARTESIAN_POINT('Ctrl Pts',(-19.5793222342617,-13.6565946963034,
116.5340328038)) ;
#194255=CARTESIAN_POINT('Ctrl Pts',(-19.5766443908906,-13.3650274692435,
116.561521687916)) ;
#194256=CARTESIAN_POINT('Ctrl Pts',(-19.5495669925005,-13.0788343995772,
116.514498473725)) ;
#194257=CARTESIAN_POINT('Ctrl Pts',(-19.4996422792964,-12.8175211583994,
116.397794021949)) ;
#194258=CARTESIAN_POINT('Ctrl Pts',(-19.4293404722098,-12.5984995679009,
116.219119607498)) ;
#194259=CARTESIAN_POINT('Ctrl Pts',(-19.3431976343271,-12.4381081950322,
115.992149215875)) ;
#194260=CARTESIAN_POINT('Ctrl Pts',(-19.2456411710222,-12.3474840033873,
115.730719198245)) ;
#194261=CARTESIAN_POINT('Ctrl Pts',(-19.1449743145035,-12.3342746176406,
115.45936107608)) ;
#194262=CARTESIAN_POINT('Ctrl Pts',(-19.0456937210243,-12.3983523506611,
115.192496748361)) ;
#194263=CARTESIAN_POINT('Ctrl Pts',(-18.9551049831602,-12.5353914606374,
114.952015661837)) ;
#194264=CARTESIAN_POINT('Ctrl Pts',(-18.8783820413473,-12.7368848040207,
114.753966045534)) ;
#194265=CARTESIAN_POINT('Ctrl Pts',(-18.8212505018881,-12.9849643669818,
114.615234103962)) ;
#194266=CARTESIAN_POINT('Ctrl Pts',(-18.785989087223,-13.2657001242146,
114.543367393447)) ;
#194267=CARTESIAN_POINT('Ctrl Pts',(-18.7749409518522,-13.5562446654925,
114.545103589634)) ;
#194268=CARTESIAN_POINT('Ctrl Pts',(-18.7878772786409,-13.837740260252,
114.619989429758)) ;
#194269=CARTESIAN_POINT('Ctrl Pts',(-18.823586104698,-14.0900089023239,
114.76439949876)) ;
#194270=CARTESIAN_POINT('Ctrl Pts',(-18.8778061466655,-14.2916996646196,
114.964766086765)) ;
#194271=CARTESIAN_POINT('Ctrl Pts',(-18.9472129540579,-14.4330905333239,
115.211832429368)) ;
#194272=CARTESIAN_POINT('Ctrl Pts',(-19.0250383188823,-14.5004556458798,
115.484322413278)) ;
#194273=CARTESIAN_POINT('Ctrl Pts',(-19.1050415480743,-14.4906784452632,
115.763353035226)) ;
#194274=CARTESIAN_POINT('Ctrl Pts',(-19.1811866606781,-14.4044504861589,
116.030699387926)) ;
#194275=CARTESIAN_POINT('Ctrl Pts',(-19.2474615033651,-14.2464177648016,
116.26820558113)) ;
#194276=CARTESIAN_POINT('Ctrl Pts',(-19.2975522404832,-14.0296079395376,
116.456228657709)) ;
#194277=CARTESIAN_POINT('Ctrl Pts',(-19.3275320163761,-13.7700542634679,
116.582883427607)) ;
#194278=CARTESIAN_POINT('Ctrl Pts',(-19.3346750163065,-13.4844393542531,
116.640102123225)) ;
#194279=CARTESIAN_POINT('Ctrl Pts',(-19.3174944725961,-13.1938467066394,
116.623262581033)) ;
#194280=CARTESIAN_POINT('Ctrl Pts',(-19.2765712704978,-12.9193998282655,
116.534084192877)) ;
#194281=CARTESIAN_POINT('Ctrl Pts',(-19.2136556163805,-12.679977460876,
116.378071311553)) ;
#194282=CARTESIAN_POINT('Ctrl Pts',(-19.1338523199838,-12.4956043021029,
116.170183536347)) ;
#194283=CARTESIAN_POINT('Ctrl Pts',(-19.0401108727425,-12.3751190535725,
115.920306886088)) ;
#194284=CARTESIAN_POINT('Ctrl Pts',(-18.9401330390511,-12.3303020351126,
115.651151126256)) ;
#194285=CARTESIAN_POINT('Ctrl Pts',(-18.839178326217,-12.3631774170788,
115.379196252521)) ;
#194286=CARTESIAN_POINT('Ctrl Pts',(-18.7446035699514,-12.4713342743348,
115.126509818248)) ;
#194287=CARTESIAN_POINT('Ctrl Pts',(-18.6616637495359,-12.6476404276989,
114.909396069518)) ;
#194288=CARTESIAN_POINT('Ctrl Pts',(-18.5959843317389,-12.8790215196565,
114.744812606196)) ;
#194289=CARTESIAN_POINT('Ctrl Pts',(-18.5513499003185,-13.1499133657009,
114.644442101082)) ;
#194290=CARTESIAN_POINT('Ctrl Pts',(-18.5304611078023,-13.4386144880716,
114.616209853643)) ;
#194291=CARTESIAN_POINT('Ctrl Pts',(-18.5338401235194,-13.7268235527867,
114.662025079469)) ;
#194292=CARTESIAN_POINT('Ctrl Pts',(-18.5603928248668,-13.9914324144424,
114.778219545102)) ;
#194293=CARTESIAN_POINT('Ctrl Pts',(-18.6076829202727,-14.2164140691066,
114.957760632545)) ;
#194294=CARTESIAN_POINT('Ctrl Pts',(-18.6716131600408,-14.384032579335,
115.188003285153)) ;
#194295=CARTESIAN_POINT('Ctrl Pts',(-18.7465062676533,-14.4820529544929,
115.451530561366)) ;
#194296=CARTESIAN_POINT('Ctrl Pts',(-18.8266090365466,-14.5042250600488,
115.730991693486)) ;
#194297=CARTESIAN_POINT('Ctrl Pts',(-18.9055245763069,-14.4479097103847,
116.006958567327)) ;
#194298=CARTESIAN_POINT('Ctrl Pts',(-18.9759850270256,-14.3189148106109,
116.25684843315)) ;
#194299=CARTESIAN_POINT('Ctrl Pts',(-19.0333811299086,-14.1239822238445,
116.467278862587)) ;
#194300=CARTESIAN_POINT('Ctrl Pts',(-19.0719097483262,-13.8804446676162,
116.619916310961)) ;
#194301=CARTESIAN_POINT('Ctrl Pts',(-19.088702598421,-13.6007259227713,
116.70677615132)) ;
#194302=CARTESIAN_POINT('Ctrl Pts',(-19.0813475062609,-13.310886389785,
116.719690814776)) ;
#194303=CARTESIAN_POINT('Ctrl Pts',(-19.0499358228212,-13.0275729196668,
116.659478806876)) ;
#194304=CARTESIAN_POINT('Ctrl Pts',(-18.9956010454947,-12.7715214711428,
116.529545008738)) ;
#194305=CARTESIAN_POINT('Ctrl Pts',(-18.9217241255641,-12.5625540682405,
116.340023816642)) ;
#194306=CARTESIAN_POINT('Ctrl Pts',(-18.8334781141802,-12.4155360311479,
116.106499613622)) ;
#194307=CARTESIAN_POINT('Ctrl Pts',(-18.7350882955953,-12.339199302571,
115.842366036142)) ;
#194308=CARTESIAN_POINT('Ctrl Pts',(-18.6339421925997,-12.3403409953756,
115.569683136395)) ;
#194309=CARTESIAN_POINT('Ctrl Pts',(-18.5356154875398,-12.4190382667156,
115.305787998287)) ;
#194310=CARTESIAN_POINT('Ctrl Pts',(-18.4475845571782,-12.5685297170459,
115.072992627023)) ;
#194311=CARTESIAN_POINT('Ctrl Pts',(-18.3743096061269,-12.7793086778933,
114.885300417553)) ;
#194312=CARTESIAN_POINT('Ctrl Pts',(-18.3207591758651,-13.0361487300971,
114.757699953502)) ;
#194313=CARTESIAN_POINT('Ctrl Pts',(-18.2900556295031,-13.3199156358865,
114.699632332883)) ;
#194314=CARTESIAN_POINT('Ctrl Pts',(-18.2835244771423,-13.61053350134,114.715169773089)) ;
#194315=CARTESIAN_POINT('Ctrl Pts',(-18.300904682681,-13.8877845324202,
114.80358738621)) ;
#194316=CARTESIAN_POINT('Ctrl Pts',(-18.3402955625269,-14.1315208949384,
114.95907694666)) ;
#194317=CARTESIAN_POINT('Ctrl Pts',(-18.3979499293583,-14.3236676354294,
115.170121270634)) ;
#194318=CARTESIAN_POINT('Ctrl Pts',(-18.4691141873596,-14.451213086268,
115.422348614941)) ;
#194319=CARTESIAN_POINT('Ctrl Pts',(-18.5480547946809,-14.5046478984509,
115.698323016836)) ;
#194320=CARTESIAN_POINT('Ctrl Pts',(-18.6278722273307,-14.4801334339684,
115.976822091214)) ;
#194321=CARTESIAN_POINT('Ctrl Pts',(-18.7025035045635,-14.3800974324411,
116.239533090197)) ;
#194322=CARTESIAN_POINT('Ctrl Pts',(-18.7661852178501,-14.2097836883392,
116.469145099282)) ;
#194323=CARTESIAN_POINT('Ctrl Pts',(-18.8126736298305,-13.9844447661634,
116.646062755378)) ;
#194324=CARTESIAN_POINT('Ctrl Pts',(-18.8387106000838,-13.7175338810347,
116.760872830317)) ;
#194325=CARTESIAN_POINT('Ctrl Pts',(-18.8412499966495,-13.4290941380284,
116.804105500737)) ;
#194326=CARTESIAN_POINT('Ctrl Pts',(-18.8195971871137,-13.1407025280343,
116.773545460015)) ;
#194327=CARTESIAN_POINT('Ctrl Pts',(-18.7741929648226,-12.8707969653127,
116.670833856634)) ;
#194328=CARTESIAN_POINT('Ctrl Pts',(-18.7081893525992,-12.6417711077458,
116.505122794438)) ;
#194329=CARTESIAN_POINT('Ctrl Pts',(-18.624745958435,-12.4670674817275,
116.286513958254)) ;
#194330=CARTESIAN_POINT('Ctrl Pts',(-18.5299237726579,-12.3610581795072,
116.033065517688)) ;
#194331=CARTESIAN_POINT('Ctrl Pts',(-18.4285423943449,-12.3304705905987,
115.759931665259)) ;
#194332=CARTESIAN_POINT('Ctrl Pts',(-18.3286734717406,-12.3780041179342,
115.491117750201)) ;
#194333=CARTESIAN_POINT('Ctrl Pts',(-18.2355472337233,-12.5002675543906,
115.242998586149)) ;
#194334=CARTESIAN_POINT('Ctrl Pts',(-18.1559065411703,-12.6872113223539,
115.03574587489)) ;
#194335=CARTESIAN_POINT('Ctrl Pts',(-18.0936528156396,-12.928470822573,
114.881781285062)) ;
#194336=CARTESIAN_POINT('Ctrl Pts',(-18.053566961881,-13.2034657060163,
114.795110966265)) ;
#194337=CARTESIAN_POINT('Ctrl Pts',(-18.0372153758526,-13.4939400108665,
114.780761585915)) ;
#194338=CARTESIAN_POINT('Ctrl Pts',(-18.045087176113,-13.7785749983251,
114.84013824791)) ;
#194339=CARTESIAN_POINT('Ctrl Pts',(-18.0758126785522,-14.0376123935157,
114.969142216543)) ;
#194340=CARTESIAN_POINT('Ctrl Pts',(-18.126546298458,-14.2526152270872,
115.159131089373)) ;
#194341=CARTESIAN_POINT('Ctrl Pts',(-18.1929627182085,-14.4080507138092,
115.39693012817)) ;
#194342=CARTESIAN_POINT('Ctrl Pts',(-18.2695829032393,-14.4922598223547,
115.665846830142)) ;
#194343=CARTESIAN_POINT('Ctrl Pts',(-18.3495327203372,-14.4995566650645,
115.94467290167)) ;
#194344=CARTESIAN_POINT('Ctrl Pts',(-18.4275077803074,-14.4291954268347,
116.217786788456)) ;
#194345=CARTESIAN_POINT('Ctrl Pts',(-18.4961354751818,-14.2862746553945,
116.462278671806)) ;
#194346=CARTESIAN_POINT('Ctrl Pts',(-18.5499768620455,-14.0821782924177,
116.661608442272)) ;
#194347=CARTESIAN_POINT('Ctrl Pts',(-18.5848332719322,-13.8298750263426,
116.803243954575)) ;
#194348=CARTESIAN_POINT('Ctrl Pts',(-18.597136541653,-13.5470860719876,
116.876296357144)) ;
#194349=CARTESIAN_POINT('Ctrl Pts',(-18.5852386802465,-13.2560613841224,
116.875504551637)) ;
#194350=CARTESIAN_POINT('Ctrl Pts',(-18.549259012026,-12.9762949722028,
116.801413358043)) ;
#194351=CARTESIAN_POINT('Ctrl Pts',(-18.4912772241492,-12.729021213087,
116.66017876415)) ;
#194352=CARTESIAN_POINT('Ctrl Pts',(-18.4142572250889,-12.5300504685621,
116.461103914665)) ;
#194353=CARTESIAN_POINT('Ctrl Pts',(-18.3230315098279,-12.3949013412461,
116.218789967548)) ;
#194354=CARTESIAN_POINT('Ctrl Pts',(-18.223852812221,-12.3334783627152,
115.952132037095)) ;
#194355=CARTESIAN_POINT('Ctrl Pts',(-18.1228645176016,-12.3494129205617,
115.679929191813)) ;
#194356=CARTESIAN_POINT('Ctrl Pts',(-18.0261149973896,-12.4418688951199,
115.420743578469)) ;
#194357=CARTESIAN_POINT('Ctrl Pts',(-17.9399661082425,-12.6051421932678,
115.193941498684)) ;
#194358=CARTESIAN_POINT('Ctrl Pts',(-17.8706577437902,-12.824581983231,
115.018086912983)) ;
#194359=CARTESIAN_POINT('Ctrl Pts',(-17.8211647568461,-13.0878606072953,
114.902837359147)) ;
#194360=CARTESIAN_POINT('Ctrl Pts',(-17.7949112979524,-13.3747557627756,
114.858346400162)) ;
#194361=CARTESIAN_POINT('Ctrl Pts',(-17.7930142307547,-13.6654070056361,
114.888132109586)) ;
#194362=CARTESIAN_POINT('Ctrl Pts',(-17.8147252087611,-13.9370542943595,
114.989647338605)) ;
#194363=CARTESIAN_POINT('Ctrl Pts',(-17.8580728556449,-14.1729033532404,
115.157292589129)) ;
#194364=CARTESIAN_POINT('Ctrl Pts',(-17.9184133421674,-14.3528610645483,
115.376351104933)) ;
#194365=CARTESIAN_POINT('Ctrl Pts',(-17.991766676009,-14.4673900074207,
115.635384696762)) ;
#194366=CARTESIAN_POINT('Ctrl Pts',(-18.0711284340199,-14.5059091307987,
115.912498667304)) ;
#194367=CARTESIAN_POINT('Ctrl Pts',(-18.1505342643703,-14.467003448986,
116.1897784186)) ;
#194368=CARTESIAN_POINT('Ctrl Pts',(-18.2236575677772,-14.3526296857438,
116.448006484568)) ;
#194369=CARTESIAN_POINT('Ctrl Pts',(-18.2841253649015,-14.1719531187117,
116.667560097024)) ;
#194370=CARTESIAN_POINT('Ctrl Pts',(-18.3272925522858,-13.936583984801,
116.834555335885)) ;
#194371=CARTESIAN_POINT('Ctrl Pts',(-18.3489789369998,-13.6642946874373,
116.936073490923)) ;
#194372=CARTESIAN_POINT('Ctrl Pts',(-18.3470303613831,-13.3747428455626,
116.965562261399)) ;
#194373=CARTESIAN_POINT('Ctrl Pts',(-18.3207665837922,-13.0876482903165,
116.921069134503)) ;
#194374=CARTESIAN_POINT('Ctrl Pts',(-18.2712815660308,-12.8243385253649,
116.805840132971)) ;
#194375=CARTESIAN_POINT('Ctrl Pts',(-18.2015034322164,-12.6038922563675,
116.628754857575)) ;
#194376=CARTESIAN_POINT('Ctrl Pts',(-18.1155659825145,-12.4415502102937,
116.402472433253)) ;
#194377=CARTESIAN_POINT('Ctrl Pts',(-18.0188186140626,-12.3493107874977,
116.143292052209)) ;
#194378=CARTESIAN_POINT('Ctrl Pts',(-17.917965944462,-12.3333698024851,
115.871447888668)) ;
#194379=CARTESIAN_POINT('Ctrl Pts',(-17.8179951285442,-12.3958418590805,
115.602676622725)) ;
#194380=CARTESIAN_POINT('Ctrl Pts',(-17.7275667072708,-12.5305465195612,
115.362515531508)) ;
#194381=CARTESIAN_POINT('Ctrl Pts',(-17.6506148333136,-12.7291635452138,
115.163608506426)) ;
#194382=CARTESIAN_POINT('Ctrl Pts',(-17.5925315518145,-12.9771312925897,
115.022149073148)) ;
#194383=CARTESIAN_POINT('Ctrl Pts',(-17.5565878319294,-13.2574946761857,
114.948229481288)) ;
#194384=CARTESIAN_POINT('Ctrl Pts',(-17.5448475110634,-13.5486172877669,
114.947929919244)) ;
#194385=CARTESIAN_POINT('Ctrl Pts',(-17.5571682124288,-13.8299622964239,
115.020863384168)) ;
#194386=CARTESIAN_POINT('Ctrl Pts',(-17.5919536420937,-14.082140489746,
115.162256577588)) ;
#194387=CARTESIAN_POINT('Ctrl Pts',(-17.6460547424978,-14.2871395255682,
115.362533542529)) ;
#194388=CARTESIAN_POINT('Ctrl Pts',(-17.7149985645736,-14.4298488440199,
115.608097682744)) ;
#194389=CARTESIAN_POINT('Ctrl Pts',(-17.7923224785126,-14.4994383097765,
115.878923588417)) ;
#194390=CARTESIAN_POINT('Ctrl Pts',(-17.8726588843966,-14.4922423916848,
116.159099968041)) ;
#194391=CARTESIAN_POINT('Ctrl Pts',(-17.9492605892441,-14.4074859363464,
116.427972082509)) ;
#194392=CARTESIAN_POINT('Ctrl Pts',(-18.0153695983152,-14.2527213410347,
116.664674816876)) ;
#194393=CARTESIAN_POINT('Ctrl Pts',(-18.0662184898938,-14.0372448891262,
116.855097648155)) ;
#194394=CARTESIAN_POINT('Ctrl Pts',(-18.0969238178348,-13.7782273369584,
116.984027397216)) ;
#194395=CARTESIAN_POINT('Ctrl Pts',(-18.1047200617367,-13.4921296981973,
117.043351119596)) ;
#194396=CARTESIAN_POINT('Ctrl Pts',(-18.0891514169294,-13.217409939261,
117.029459791734)) ;
#194397=CARTESIAN_POINT('Ctrl Pts',(-18.0654405919642,-13.0469696088692,
116.979117868373)) ;
#194398=CARTESIAN_POINT('Ctrl Pts',(-18.0519478151656,-12.9727494438644,
116.948041367699)) ;
#194399=CARTESIAN_POINT('',(-29.0978033499347,-13.1317299129408,113.463978642533)) ;
#194400=CARTESIAN_POINT('Origin',(-29.0751148924065,-13.1500241806476,113.394873261672)) ;
#194401=CARTESIAN_POINT('',(-29.0524264348783,-13.1683184483544,113.32576788081)) ;
#194402=CARTESIAN_POINT('Origin',(-29.0751148924065,-13.1500241806476,113.394873261672)) ;
#194403=CARTESIAN_POINT('Origin',(-29.0751148924065,-13.1500241806476,113.394873261672)) ;
#194404=CARTESIAN_POINT('Ctrl Pts',(-29.1489187358159,-13.1500241806476,
113.370642219953)) ;
#194405=CARTESIAN_POINT('Ctrl Pts',(-29.1501712550706,-13.1861488576831,
113.380503101533)) ;
#194406=CARTESIAN_POINT('Ctrl Pts',(-29.1532918849611,-13.2629207728781,
113.383238925643)) ;
#194407=CARTESIAN_POINT('Ctrl Pts',(-29.158850654713,-13.3681754735787,
113.336140363464)) ;
#194408=CARTESIAN_POINT('Ctrl Pts',(-29.1641549311487,-13.4419954208924,
113.247282880188)) ;
#194409=CARTESIAN_POINT('Ctrl Pts',(-29.1668024185619,-13.4603090867706,
113.172355715138)) ;
#194410=CARTESIAN_POINT('Ctrl Pts',(-29.1677657801251,-13.4607127643287,
113.134762231593)) ;
#194411=CARTESIAN_POINT('Ctrl Pts',(-29.1262302782877,-13.1683184483544,
113.301536839092)) ;
#194412=CARTESIAN_POINT('Ctrl Pts',(-29.12711604839,-13.1940059114669,113.308742056967)) ;
#194413=CARTESIAN_POINT('Ctrl Pts',(-29.1293290715985,-13.2486867737934,
113.311073820728)) ;
#194414=CARTESIAN_POINT('Ctrl Pts',(-29.1332857460124,-13.3239058135206,
113.278044278162)) ;
#194415=CARTESIAN_POINT('Ctrl Pts',(-29.1370736300659,-13.3769362528745,
113.215107919416)) ;
#194416=CARTESIAN_POINT('Ctrl Pts',(-29.1389728533701,-13.3903536795156,
113.161819186649)) ;
#194417=CARTESIAN_POINT('Ctrl Pts',(-29.1396668443893,-13.3908270508895,
113.135038642707)) ;
#194418=CARTESIAN_POINT('Ctrl Pts',(-29.0524264348783,-13.1683184483544,
113.32576788081)) ;
#194419=CARTESIAN_POINT('Ctrl Pts',(-29.0534550311952,-13.1977103078297,
113.333412909135)) ;
#194420=CARTESIAN_POINT('Ctrl Pts',(-29.0560057529408,-13.2599976587319,
113.334883492462)) ;
#194421=CARTESIAN_POINT('Ctrl Pts',(-29.0605207617359,-13.3449026924378,
113.295661398383)) ;
#194422=CARTESIAN_POINT('Ctrl Pts',(-29.0648049091706,-13.4039111623081,
113.222879629767)) ;
#194423=CARTESIAN_POINT('Ctrl Pts',(-29.0669264092244,-13.4180394153483,
113.161936094993)) ;
#194424=CARTESIAN_POINT('Ctrl Pts',(-29.0676926945815,-13.4180036036418,
113.131444278443)) ;
#194425=CARTESIAN_POINT('Ctrl Pts',(-28.9786225914689,-13.1683184483544,
113.349998922528)) ;
#194426=CARTESIAN_POINT('Ctrl Pts',(-28.9797940140003,-13.2014147041926,
113.358083761303)) ;
#194427=CARTESIAN_POINT('Ctrl Pts',(-28.9826824342832,-13.2713085436704,
113.358693164196)) ;
#194428=CARTESIAN_POINT('Ctrl Pts',(-28.9877557774593,-13.365899571355,
113.313278518605)) ;
#194429=CARTESIAN_POINT('Ctrl Pts',(-28.9925361882752,-13.4308860717416,
113.230651340118)) ;
#194430=CARTESIAN_POINT('Ctrl Pts',(-28.9948799650788,-13.4457251511809,
113.162053003337)) ;
#194431=CARTESIAN_POINT('Ctrl Pts',(-28.9957185447737,-13.445180156394,
113.12784991418)) ;
#194432=CARTESIAN_POINT('Ctrl Pts',(-29.0013110489971,-13.1500241806476,
113.41910430339)) ;
#194433=CARTESIAN_POINT('Ctrl Pts',(-29.002849220681,-13.1935576504088,
113.429844805869)) ;
#194434=CARTESIAN_POINT('Ctrl Pts',(-29.0066452476457,-13.2855425427551,
113.430858269111)) ;
#194435=CARTESIAN_POINT('Ctrl Pts',(-29.0133206861599,-13.4101692314131,
113.371374603907)) ;
#194436=CARTESIAN_POINT('Ctrl Pts',(-29.019617489358,-13.4959452397595,
113.26282630089)) ;
#194437=CARTESIAN_POINT('Ctrl Pts',(-29.0227095302706,-13.515680558436,
113.172589531826)) ;
#194438=CARTESIAN_POINT('Ctrl Pts',(-29.0238174805094,-13.5150658698332,
113.127573503066)) ;
#194439=CARTESIAN_POINT('Ctrl Pts',(-29.0239995065253,-13.1317299129408,
113.488209684252)) ;
#194440=CARTESIAN_POINT('Ctrl Pts',(-29.0259044273616,-13.185700596625,
113.501605850436)) ;
#194441=CARTESIAN_POINT('Ctrl Pts',(-29.0306080610083,-13.2997765418398,
113.503023374026)) ;
#194442=CARTESIAN_POINT('Ctrl Pts',(-29.0388855948605,-13.4544388914713,
113.429470689208)) ;
#194443=CARTESIAN_POINT('Ctrl Pts',(-29.0466987904407,-13.5610044077774,
113.295001261662)) ;
#194444=CARTESIAN_POINT('Ctrl Pts',(-29.0505390954623,-13.585635965691,
113.183126060316)) ;
#194445=CARTESIAN_POINT('Ctrl Pts',(-29.0519164162452,-13.5849515832724,
113.127297091952)) ;
#194446=CARTESIAN_POINT('Ctrl Pts',(-29.0978033499347,-13.1317299129408,
113.463978642533)) ;
#194447=CARTESIAN_POINT('Ctrl Pts',(-29.0995654445564,-13.1819962002622,
113.476934998268)) ;
#194448=CARTESIAN_POINT('Ctrl Pts',(-29.103931379666,-13.2884656569013,
113.479213702292)) ;
#194449=CARTESIAN_POINT('Ctrl Pts',(-29.111650579137,-13.433442012554,113.411853568987)) ;
#194450=CARTESIAN_POINT('Ctrl Pts',(-29.1189675113361,-13.5340294983438,
113.287229551311)) ;
#194451=CARTESIAN_POINT('Ctrl Pts',(-29.122585539608,-13.5579502298583,
113.183009151971)) ;
#194452=CARTESIAN_POINT('Ctrl Pts',(-29.1238905660531,-13.5577750305201,
113.130891456215)) ;
#194453=CARTESIAN_POINT('Ctrl Pts',(-29.1716071933441,-13.1317299129408,
113.439747600815)) ;
#194454=CARTESIAN_POINT('Ctrl Pts',(-29.1732264617512,-13.1782918038993,
113.4522641461)) ;
#194455=CARTESIAN_POINT('Ctrl Pts',(-29.1772546983237,-13.2771547719628,
113.455404030558)) ;
#194456=CARTESIAN_POINT('Ctrl Pts',(-29.1844155634136,-13.4124451336368,
113.394236448766)) ;
#194457=CARTESIAN_POINT('Ctrl Pts',(-29.1912362322315,-13.5070545889103,
113.27945784096)) ;
#194458=CARTESIAN_POINT('Ctrl Pts',(-29.1946319837536,-13.5302644940257,
113.182892243627)) ;
#194459=CARTESIAN_POINT('Ctrl Pts',(-29.1958647158609,-13.5305984777679,
113.134485820479)) ;
#194460=CARTESIAN_POINT('Ctrl Pts',(-29.1489187358159,-13.1500241806476,
113.370642219953)) ;
#194461=CARTESIAN_POINT('Ctrl Pts',(-29.1501712550706,-13.1861488576831,
113.380503101533)) ;
#194462=CARTESIAN_POINT('Ctrl Pts',(-29.1532918849611,-13.2629207728781,
113.383238925643)) ;
#194463=CARTESIAN_POINT('Ctrl Pts',(-29.158850654713,-13.3681754735787,
113.336140363464)) ;
#194464=CARTESIAN_POINT('Ctrl Pts',(-29.1641549311487,-13.4419954208924,
113.247282880188)) ;
#194465=CARTESIAN_POINT('Ctrl Pts',(-29.1668024185619,-13.4603090867706,
113.172355715138)) ;
#194466=CARTESIAN_POINT('Ctrl Pts',(-29.1677657801251,-13.4607127643287,
113.134762231593)) ;
#194467=CARTESIAN_POINT('',(-29.1677657801251,-13.4607127643287,113.134762231593)) ;
#194468=CARTESIAN_POINT('Ctrl Pts',(-29.1489187358159,-13.1500241806476,
113.370642219953)) ;
#194469=CARTESIAN_POINT('Ctrl Pts',(-29.1501712550706,-13.1861488576831,
113.380503101533)) ;
#194470=CARTESIAN_POINT('Ctrl Pts',(-29.1532918849611,-13.2629207728781,
113.383238925643)) ;
#194471=CARTESIAN_POINT('Ctrl Pts',(-29.158850654713,-13.3681754735787,
113.336140363464)) ;
#194472=CARTESIAN_POINT('Ctrl Pts',(-29.1641549311487,-13.4419954208924,
113.247282880188)) ;
#194473=CARTESIAN_POINT('Ctrl Pts',(-29.1668024185619,-13.4603090867706,
113.172355715138)) ;
#194474=CARTESIAN_POINT('Ctrl Pts',(-29.1677657801251,-13.4607127643287,
113.134762231593)) ;
#194475=CARTESIAN_POINT('Origin',(-29.0957916303173,-13.4878893170809,113.131167867329)) ;
#194476=CARTESIAN_POINT('Ctrl Pts',(-29.1677657801251,-13.4607127643287,
113.134762231593)) ;
#194477=CARTESIAN_POINT('Ctrl Pts',(-29.1774333842888,-13.4607136600768,
112.751611216526)) ;
#194478=CARTESIAN_POINT('Ctrl Pts',(-29.1871009884525,-13.460714555825,
112.368460201459)) ;
#194479=CARTESIAN_POINT('Ctrl Pts',(-29.1967685926162,-13.4607154515732,
111.985309186393)) ;
#194480=CARTESIAN_POINT('Ctrl Pts',(-29.1396668443893,-13.3908270508895,
113.135038642707)) ;
#194481=CARTESIAN_POINT('Ctrl Pts',(-29.149334448553,-13.3908279466377,
112.75188762764)) ;
#194482=CARTESIAN_POINT('Ctrl Pts',(-29.1590020527167,-13.3908288423858,
112.368736612573)) ;
#194483=CARTESIAN_POINT('Ctrl Pts',(-29.1686696568804,-13.390829738134,
111.985585597507)) ;
#194484=CARTESIAN_POINT('Ctrl Pts',(-29.0676926945815,-13.4180036036418,
113.131444278443)) ;
#194485=CARTESIAN_POINT('Ctrl Pts',(-29.0773602987452,-13.4180044993899,
112.748293263377)) ;
#194486=CARTESIAN_POINT('Ctrl Pts',(-29.0870279029089,-13.4180053951381,
112.36514224831)) ;
#194487=CARTESIAN_POINT('Ctrl Pts',(-29.0966955070725,-13.4180062908863,
111.981991233243)) ;
#194488=CARTESIAN_POINT('Ctrl Pts',(-28.9957185447737,-13.445180156394,
113.12784991418)) ;
#194489=CARTESIAN_POINT('Ctrl Pts',(-29.0053861489373,-13.4451810521422,
112.744698899113)) ;
#194490=CARTESIAN_POINT('Ctrl Pts',(-29.015053753101,-13.4451819478904,
112.361547884046)) ;
#194491=CARTESIAN_POINT('Ctrl Pts',(-29.0247213572647,-13.4451828436386,
111.97839686898)) ;
#194492=CARTESIAN_POINT('Ctrl Pts',(-29.0238174805094,-13.5150658698332,
113.127573503066)) ;
#194493=CARTESIAN_POINT('Ctrl Pts',(-29.0334850846731,-13.5150667655814,
112.744422487999)) ;
#194494=CARTESIAN_POINT('Ctrl Pts',(-29.0431526888368,-13.5150676613296,
112.361271472932)) ;
#194495=CARTESIAN_POINT('Ctrl Pts',(-29.0528202930005,-13.5150685570778,
111.978120457866)) ;
#194496=CARTESIAN_POINT('Ctrl Pts',(-29.0519164162452,-13.5849515832724,
113.127297091952)) ;
#194497=CARTESIAN_POINT('Ctrl Pts',(-29.0615840204089,-13.5849524790206,
112.744146076885)) ;
#194498=CARTESIAN_POINT('Ctrl Pts',(-29.0712516245726,-13.5849533747688,
112.360995061818)) ;
#194499=CARTESIAN_POINT('Ctrl Pts',(-29.0809192287363,-13.5849542705169,
111.977844046752)) ;
#194500=CARTESIAN_POINT('Ctrl Pts',(-29.1238905660531,-13.5577750305201,
113.130891456215)) ;
#194501=CARTESIAN_POINT('Ctrl Pts',(-29.1335581702167,-13.5577759262683,
112.747740441148)) ;
#194502=CARTESIAN_POINT('Ctrl Pts',(-29.1432257743804,-13.5577768220165,
112.364589426082)) ;
#194503=CARTESIAN_POINT('Ctrl Pts',(-29.1528933785441,-13.5577777177647,
111.981438411015)) ;
#194504=CARTESIAN_POINT('Ctrl Pts',(-29.1958647158609,-13.5305984777679,
113.134485820479)) ;
#194505=CARTESIAN_POINT('Ctrl Pts',(-29.2055323200246,-13.530599373516,
112.751334805412)) ;
#194506=CARTESIAN_POINT('Ctrl Pts',(-29.2151999241883,-13.5306002692642,
112.368183790345)) ;
#194507=CARTESIAN_POINT('Ctrl Pts',(-29.2248675283519,-13.5306011650124,
111.985032775279)) ;
#194508=CARTESIAN_POINT('Ctrl Pts',(-29.1677657801251,-13.4607127643287,
113.134762231593)) ;
#194509=CARTESIAN_POINT('Ctrl Pts',(-29.1774333842888,-13.4607136600768,
112.751611216526)) ;
#194510=CARTESIAN_POINT('Ctrl Pts',(-29.1871009884525,-13.460714555825,
112.368460201459)) ;
#194511=CARTESIAN_POINT('Ctrl Pts',(-29.1967685926162,-13.4607154515732,
111.985309186393)) ;
#194512=CARTESIAN_POINT('',(-29.1967685926162,-13.4607154515732,111.985309186393)) ;
#194513=CARTESIAN_POINT('',(-29.1677657801251,-13.4607127643287,113.134762231593)) ;
#194514=CARTESIAN_POINT('',(-29.1248995454595,-13.562875855635,111.980154590046)) ;
#194515=CARTESIAN_POINT('Origin',(-29.1247944428083,-13.4878920043255,111.981714822129)) ;
#194516=CARTESIAN_POINT('',(-29.1246892014358,-13.4129081530202,111.983275048377)) ;
#194517=CARTESIAN_POINT('Origin',(-29.1247944428083,-13.4878920043255,111.981714822129)) ;
#194518=CARTESIAN_POINT('Origin',(-29.1247944428083,-13.4878920043255,111.981714822129)) ;
#194519=CARTESIAN_POINT('Ctrl Pts',(-29.1967685926162,-13.4607154515732,
111.985309186393)) ;
#194520=CARTESIAN_POINT('Ctrl Pts',(-29.20372433272,-13.4607154515732,111.919496169812)) ;
#194521=CARTESIAN_POINT('Ctrl Pts',(-29.2391616569514,-13.4607154515732,
111.786249874406)) ;
#194522=CARTESIAN_POINT('Ctrl Pts',(-29.3531737828725,-13.4607154515732,
111.608725138771)) ;
#194523=CARTESIAN_POINT('Ctrl Pts',(-29.5178000156693,-13.4607154515732,
111.473552139375)) ;
#194524=CARTESIAN_POINT('Ctrl Pts',(-29.7125058569765,-13.4607154515732,
111.39418874148)) ;
#194525=CARTESIAN_POINT('Ctrl Pts',(-29.9214770342181,-13.4607154515732,
111.374286592167)) ;
#194526=CARTESIAN_POINT('Ctrl Pts',(-30.129031067933,-13.4607154515732,
111.417939881308)) ;
#194527=CARTESIAN_POINT('Ctrl Pts',(-30.3108273632114,-13.4607154515732,
111.522718871897)) ;
#194528=CARTESIAN_POINT('Ctrl Pts',(-30.4475054824147,-13.4607154515732,
111.674400413727)) ;
#194529=CARTESIAN_POINT('Ctrl Pts',(-30.5306819470581,-13.4607154515732,
111.859696163125)) ;
#194530=CARTESIAN_POINT('Ctrl Pts',(-30.5515845507338,-13.4607154515732,
112.065598309889)) ;
#194531=CARTESIAN_POINT('Ctrl Pts',(-30.505144819815,-13.4607154515732,
112.268886698136)) ;
#194532=CARTESIAN_POINT('Ctrl Pts',(-30.3992903014189,-13.4607154515732,
112.446856086907)) ;
#194533=CARTESIAN_POINT('Ctrl Pts',(-30.2443913742949,-13.4607154515732,
112.587215246961)) ;
#194534=CARTESIAN_POINT('Ctrl Pts',(-30.0504246992742,-13.4607154515732,
112.677419162906)) ;
#194535=CARTESIAN_POINT('Ctrl Pts',(-29.8384424605617,-13.4607154515732,
112.704782293005)) ;
#194536=CARTESIAN_POINT('Ctrl Pts',(-29.7003053480643,-13.4607154515732,
112.680623972109)) ;
#194537=CARTESIAN_POINT('Ctrl Pts',(-29.6364905070076,-13.4607154515732,
112.659288401873)) ;
#194538=CARTESIAN_POINT('Ctrl Pts',(-29.1686696568804,-13.390829738134,
111.985585597507)) ;
#194539=CARTESIAN_POINT('Ctrl Pts',(-29.1756547434426,-13.390829738134,
111.917020083641)) ;
#194540=CARTESIAN_POINT('Ctrl Pts',(-29.212039584699,-13.390829738134,111.778121325125)) ;
#194541=CARTESIAN_POINT('Ctrl Pts',(-29.3300921411966,-13.390829738134,
111.59281646223)) ;
#194542=CARTESIAN_POINT('Ctrl Pts',(-29.5010310293307,-13.390829738134,
111.451428992033)) ;
#194543=CARTESIAN_POINT('Ctrl Pts',(-29.7035209080743,-13.390829738134,
111.368050962531)) ;
#194544=CARTESIAN_POINT('Ctrl Pts',(-29.9211042383572,-13.390829738134,
111.346544328624)) ;
#194545=CARTESIAN_POINT('Ctrl Pts',(-30.1374625031161,-13.390829738134,
111.391231429979)) ;
#194546=CARTESIAN_POINT('Ctrl Pts',(-30.3272332269861,-13.390829738134,
111.499672718509)) ;
#194547=CARTESIAN_POINT('Ctrl Pts',(-30.4701946296492,-13.390829738134,
111.657128061289)) ;
#194548=CARTESIAN_POINT('Ctrl Pts',(-30.557562095135,-13.390829738134,111.84978988896)) ;
#194549=CARTESIAN_POINT('Ctrl Pts',(-30.5801472209913,-13.390829738134,
112.064144238615)) ;
#194550=CARTESIAN_POINT('Ctrl Pts',(-30.5325790354759,-13.390829738134,
112.276027895464)) ;
#194551=CARTESIAN_POINT('Ctrl Pts',(-30.4230251037581,-13.390829738134,
112.4617653852)) ;
#194552=CARTESIAN_POINT('Ctrl Pts',(-30.262238546402,-13.390829738134,112.608517564604)) ;
#194553=CARTESIAN_POINT('Ctrl Pts',(-30.0605613896538,-13.390829738134,
112.703182459841)) ;
#194554=CARTESIAN_POINT('Ctrl Pts',(-29.8398712403783,-13.390829738134,
112.732470410434)) ;
#194555=CARTESIAN_POINT('Ctrl Pts',(-29.6958938251326,-13.390829738134,
112.707826831835)) ;
#194556=CARTESIAN_POINT('Ctrl Pts',(-29.629340767279,-13.390829738134,112.685845544367)) ;
#194557=CARTESIAN_POINT('Ctrl Pts',(-29.0966955070725,-13.4180062908863,
111.981991233243)) ;
#194558=CARTESIAN_POINT('Ctrl Pts',(-29.1042018243928,-13.4180062908863,
111.906366156869)) ;
#194559=CARTESIAN_POINT('Ctrl Pts',(-29.1439282935352,-13.4180062908863,
111.753105943509)) ;
#194560=CARTESIAN_POINT('Ctrl Pts',(-29.2735847434014,-13.4180062908863,
111.548452874742)) ;
#194561=CARTESIAN_POINT('Ctrl Pts',(-29.4616903508979,-13.4180062908863,
111.392083350338)) ;
#194562=CARTESIAN_POINT('Ctrl Pts',(-29.6847569451829,-13.4180062908863,
111.299594335584)) ;
#194563=CARTESIAN_POINT('Ctrl Pts',(-29.9246462294043,-13.4180062908863,
111.275288997659)) ;
#194564=CARTESIAN_POINT('Ctrl Pts',(-30.163374541951,-13.4180062908863,
111.323977785698)) ;
#194565=CARTESIAN_POINT('Ctrl Pts',(-30.3729651263444,-13.4180062908863,
111.443039456787)) ;
#194566=CARTESIAN_POINT('Ctrl Pts',(-30.531075074711,-13.4180062908863,
111.616275157639)) ;
#194567=CARTESIAN_POINT('Ctrl Pts',(-30.6279770680687,-13.4180062908863,
111.828483329082)) ;
#194568=CARTESIAN_POINT('Ctrl Pts',(-30.6534993343581,-13.4180062908863,
112.064787262698)) ;
#194569=CARTESIAN_POINT('Ctrl Pts',(-30.601649394132,-13.4180062908863,
112.298557128891)) ;
#194570=CARTESIAN_POINT('Ctrl Pts',(-30.4813664747353,-13.4180062908863,
112.503664191636)) ;
#194571=CARTESIAN_POINT('Ctrl Pts',(-30.3044722648641,-13.4180062908863,
112.665921754)) ;
#194572=CARTESIAN_POINT('Ctrl Pts',(-30.0823343436128,-13.4180062908863,
112.770854415123)) ;
#194573=CARTESIAN_POINT('Ctrl Pts',(-29.839041196435,-13.4180062908863,
112.803748518785)) ;
#194574=CARTESIAN_POINT('Ctrl Pts',(-29.6801920694942,-13.4180062908863,
112.77696504109)) ;
#194575=CARTESIAN_POINT('Ctrl Pts',(-29.6067342129979,-13.4180062908863,
112.752907176841)) ;
#194576=CARTESIAN_POINT('Ctrl Pts',(-29.0247213572647,-13.4451828436386,
111.97839686898)) ;
#194577=CARTESIAN_POINT('Ctrl Pts',(-29.0327489053431,-13.4451828436386,
111.895712230097)) ;
#194578=CARTESIAN_POINT('Ctrl Pts',(-29.0758170023715,-13.4451828436386,
111.728090561893)) ;
#194579=CARTESIAN_POINT('Ctrl Pts',(-29.2170773456061,-13.4451828436386,
111.504089287253)) ;
#194580=CARTESIAN_POINT('Ctrl Pts',(-29.4223496724652,-13.4451828436386,
111.332737708643)) ;
#194581=CARTESIAN_POINT('Ctrl Pts',(-29.6659929822914,-13.4451828436386,
111.231137708637)) ;
#194582=CARTESIAN_POINT('Ctrl Pts',(-29.9281882204513,-13.4451828436386,
111.204033666694)) ;
#194583=CARTESIAN_POINT('Ctrl Pts',(-30.189286580786,-13.4451828436386,
111.256724141416)) ;
#194584=CARTESIAN_POINT('Ctrl Pts',(-30.4186970257026,-13.4451828436386,
111.386406195065)) ;
#194585=CARTESIAN_POINT('Ctrl Pts',(-30.5919555197728,-13.4451828436386,
111.575422253988)) ;
#194586=CARTESIAN_POINT('Ctrl Pts',(-30.6983920410023,-13.4451828436386,
111.807176769205)) ;
#194587=CARTESIAN_POINT('Ctrl Pts',(-30.7268514477248,-13.4451828436386,
112.065430286781)) ;
#194588=CARTESIAN_POINT('Ctrl Pts',(-30.6707197527881,-13.4451828436386,
112.321086362319)) ;
#194589=CARTESIAN_POINT('Ctrl Pts',(-30.5397078457124,-13.4451828436386,
112.545562998072)) ;
#194590=CARTESIAN_POINT('Ctrl Pts',(-30.3467059833262,-13.4451828436386,
112.723325943396)) ;
#194591=CARTESIAN_POINT('Ctrl Pts',(-30.1041072975719,-13.4451828436386,
112.838526370406)) ;
#194592=CARTESIAN_POINT('Ctrl Pts',(-29.8382111524917,-13.4451828436386,
112.875026627135)) ;
#194593=CARTESIAN_POINT('Ctrl Pts',(-29.6644903138558,-13.4451828436386,
112.846103250345)) ;
#194594=CARTESIAN_POINT('Ctrl Pts',(-29.5841276587169,-13.4451828436386,
112.819968809314)) ;
#194595=CARTESIAN_POINT('Ctrl Pts',(-29.0528202930005,-13.5150685570778,
111.978120457866)) ;
#194596=CARTESIAN_POINT('Ctrl Pts',(-29.0608184946204,-13.5150685570778,
111.898188316268)) ;
#194597=CARTESIAN_POINT('Ctrl Pts',(-29.1029390746239,-13.5150685570778,
111.736219111174)) ;
#194598=CARTESIAN_POINT('Ctrl Pts',(-29.2401589872819,-13.5150685570778,
111.519997963795)) ;
#194599=CARTESIAN_POINT('Ctrl Pts',(-29.4391186588037,-13.5150685570778,
111.354860855985)) ;
#194600=CARTESIAN_POINT('Ctrl Pts',(-29.6749779311936,-13.5150685570778,
111.257275487585)) ;
#194601=CARTESIAN_POINT('Ctrl Pts',(-29.9285610163122,-13.5150685570778,
111.231775930237)) ;
#194602=CARTESIAN_POINT('Ctrl Pts',(-30.1808551456028,-13.5150685570778,
111.283432592745)) ;
#194603=CARTESIAN_POINT('Ctrl Pts',(-30.4022911619279,-13.5150685570778,
111.409452348454)) ;
#194604=CARTESIAN_POINT('Ctrl Pts',(-30.5692663725382,-13.5150685570778,
111.592694606426)) ;
#194605=CARTESIAN_POINT('Ctrl Pts',(-30.6715118929254,-13.5150685570778,
111.817083043369)) ;
#194606=CARTESIAN_POINT('Ctrl Pts',(-30.6982887774674,-13.5150685570778,
112.066884358055)) ;
#194607=CARTESIAN_POINT('Ctrl Pts',(-30.6432855371273,-13.5150685570778,
112.313945164991)) ;
#194608=CARTESIAN_POINT('Ctrl Pts',(-30.5159730433732,-13.5150685570778,
112.530653699779)) ;
#194609=CARTESIAN_POINT('Ctrl Pts',(-30.3288588112191,-13.5150685570778,
112.702023625753)) ;
#194610=CARTESIAN_POINT('Ctrl Pts',(-30.0939706071923,-13.5150685570778,
112.812763073471)) ;
#194611=CARTESIAN_POINT('Ctrl Pts',(-29.8367823726751,-13.5150685570778,
112.847338509706)) ;
#194612=CARTESIAN_POINT('Ctrl Pts',(-29.6689018367874,-13.5150685570778,
112.818900390618)) ;
#194613=CARTESIAN_POINT('Ctrl Pts',(-29.5912773984455,-13.5150685570778,
112.79341166682)) ;
#194614=CARTESIAN_POINT('Ctrl Pts',(-29.0809192287363,-13.5849542705169,
111.977844046752)) ;
#194615=CARTESIAN_POINT('Ctrl Pts',(-29.0888880838978,-13.5849542705169,
111.90066440244)) ;
#194616=CARTESIAN_POINT('Ctrl Pts',(-29.1300611468763,-13.5849542705169,
111.744347660455)) ;
#194617=CARTESIAN_POINT('Ctrl Pts',(-29.2632406289578,-13.5849542705169,
111.535906640336)) ;
#194618=CARTESIAN_POINT('Ctrl Pts',(-29.4558876451423,-13.5849542705169,
111.376984003328)) ;
#194619=CARTESIAN_POINT('Ctrl Pts',(-29.6839628800958,-13.5849542705169,
111.283413266534)) ;
#194620=CARTESIAN_POINT('Ctrl Pts',(-29.9289338121731,-13.5849542705169,
111.259518193781)) ;
#194621=CARTESIAN_POINT('Ctrl Pts',(-30.1724237104197,-13.5849542705169,
111.310141044074)) ;
#194622=CARTESIAN_POINT('Ctrl Pts',(-30.3858852981532,-13.5849542705169,
111.432498501842)) ;
#194623=CARTESIAN_POINT('Ctrl Pts',(-30.5465772253037,-13.5849542705169,
111.609966958864)) ;
#194624=CARTESIAN_POINT('Ctrl Pts',(-30.6446317448485,-13.5849542705169,
111.826989317534)) ;
#194625=CARTESIAN_POINT('Ctrl Pts',(-30.6697261072099,-13.5849542705169,
112.068338429329)) ;
#194626=CARTESIAN_POINT('Ctrl Pts',(-30.6158513214665,-13.5849542705169,
112.306803967663)) ;
#194627=CARTESIAN_POINT('Ctrl Pts',(-30.492238241034,-13.5849542705169,
112.515744401486)) ;
#194628=CARTESIAN_POINT('Ctrl Pts',(-30.311011639112,-13.5849542705169,
112.680721308109)) ;
#194629=CARTESIAN_POINT('Ctrl Pts',(-30.0838339168126,-13.5849542705169,
112.786999776536)) ;
#194630=CARTESIAN_POINT('Ctrl Pts',(-29.8353535928585,-13.5849542705169,
112.819650392276)) ;
#194631=CARTESIAN_POINT('Ctrl Pts',(-29.6733133597191,-13.5849542705169,
112.791697530891)) ;
#194632=CARTESIAN_POINT('Ctrl Pts',(-29.5984271381742,-13.5849542705169,
112.766854524325)) ;
#194633=CARTESIAN_POINT('Ctrl Pts',(-29.1528933785441,-13.5577777177647,
111.981438411015)) ;
#194634=CARTESIAN_POINT('Ctrl Pts',(-29.1603410029476,-13.5577777177647,
111.911318329212)) ;
#194635=CARTESIAN_POINT('Ctrl Pts',(-29.19817243804,-13.5577777177647,111.769363042071)) ;
#194636=CARTESIAN_POINT('Ctrl Pts',(-29.319748026753,-13.5577777177647,
111.580270227824)) ;
#194637=CARTESIAN_POINT('Ctrl Pts',(-29.4952283235751,-13.5577777177647,
111.436329645022)) ;
#194638=CARTESIAN_POINT('Ctrl Pts',(-29.7027268429873,-13.5577777177647,
111.351869893481)) ;
#194639=CARTESIAN_POINT('Ctrl Pts',(-29.925391821126,-13.5577777177647,
111.330773524746)) ;
#194640=CARTESIAN_POINT('Ctrl Pts',(-30.1465116715848,-13.5577777177647,
111.377394688355)) ;
#194641=CARTESIAN_POINT('Ctrl Pts',(-30.340153398795,-13.5577777177647,
111.489131763564)) ;
#194642=CARTESIAN_POINT('Ctrl Pts',(-30.4856967802419,-13.5577777177647,
111.650819862515)) ;
#194643=CARTESIAN_POINT('Ctrl Pts',(-30.5742167719148,-13.5577777177647,
111.848295877412)) ;
#194644=CARTESIAN_POINT('Ctrl Pts',(-30.5963739938431,-13.5577777177647,
112.067695405246)) ;
#194645=CARTESIAN_POINT('Ctrl Pts',(-30.5467809628103,-13.5577777177647,
112.284274734236)) ;
#194646=CARTESIAN_POINT('Ctrl Pts',(-30.4338968700568,-13.5577777177647,
112.473845595049)) ;
#194647=CARTESIAN_POINT('Ctrl Pts',(-30.2687779206499,-13.5577777177647,
112.623317118714)) ;
#194648=CARTESIAN_POINT('Ctrl Pts',(-30.0620609628536,-13.5577777177647,
112.719327821253)) ;
#194649=CARTESIAN_POINT('Ctrl Pts',(-29.8361836368019,-13.5577777177647,
112.748372283926)) ;
#194650=CARTESIAN_POINT('Ctrl Pts',(-29.6890151153575,-13.5577777177647,
112.722559321637)) ;
#194651=CARTESIAN_POINT('Ctrl Pts',(-29.6210336924552,-13.5577777177647,
112.699792891852)) ;
#194652=CARTESIAN_POINT('Ctrl Pts',(-29.2248675283519,-13.5306011650124,
111.985032775279)) ;
#194653=CARTESIAN_POINT('Ctrl Pts',(-29.2317939219973,-13.5306011650124,
111.921972255984)) ;
#194654=CARTESIAN_POINT('Ctrl Pts',(-29.2662837292037,-13.5306011650124,
111.794378423687)) ;
#194655=CARTESIAN_POINT('Ctrl Pts',(-29.3762554245483,-13.5306011650124,
111.624633815312)) ;
#194656=CARTESIAN_POINT('Ctrl Pts',(-29.5345690020079,-13.5306011650124,
111.495675286717)) ;
#194657=CARTESIAN_POINT('Ctrl Pts',(-29.7214908058787,-13.5306011650124,
111.420326520428)) ;
#194658=CARTESIAN_POINT('Ctrl Pts',(-29.921849830079,-13.5306011650124,
111.402028855711)) ;
#194659=CARTESIAN_POINT('Ctrl Pts',(-30.1205996327499,-13.5306011650124,
111.444648332636)) ;
#194660=CARTESIAN_POINT('Ctrl Pts',(-30.2944214994368,-13.5306011650124,
111.545765025285)) ;
#194661=CARTESIAN_POINT('Ctrl Pts',(-30.4248163351801,-13.5306011650124,
111.691672766166)) ;
#194662=CARTESIAN_POINT('Ctrl Pts',(-30.5038017989812,-13.5306011650124,
111.86960243729)) ;
#194663=CARTESIAN_POINT('Ctrl Pts',(-30.5230218804764,-13.5306011650124,
112.067052381163)) ;
#194664=CARTESIAN_POINT('Ctrl Pts',(-30.4777106041542,-13.5306011650124,
112.261745500808)) ;
#194665=CARTESIAN_POINT('Ctrl Pts',(-30.3755554990797,-13.5306011650124,
112.431946788613)) ;
#194666=CARTESIAN_POINT('Ctrl Pts',(-30.2265442021878,-13.5306011650124,
112.565912929318)) ;
#194667=CARTESIAN_POINT('Ctrl Pts',(-30.0402880088946,-13.5306011650124,
112.65165586597)) ;
#194668=CARTESIAN_POINT('Ctrl Pts',(-29.8370136807451,-13.5306011650124,
112.677094175575)) ;
#194669=CARTESIAN_POINT('Ctrl Pts',(-29.7047168709959,-13.5306011650124,
112.653421112382)) ;
#194670=CARTESIAN_POINT('Ctrl Pts',(-29.6436402467363,-13.5306011650124,
112.632731259378)) ;
#194671=CARTESIAN_POINT('Ctrl Pts',(-29.1967685926162,-13.4607154515732,
111.985309186393)) ;
#194672=CARTESIAN_POINT('Ctrl Pts',(-29.20372433272,-13.4607154515732,111.919496169812)) ;
#194673=CARTESIAN_POINT('Ctrl Pts',(-29.2391616569514,-13.4607154515732,
111.786249874406)) ;
#194674=CARTESIAN_POINT('Ctrl Pts',(-29.3531737828725,-13.4607154515732,
111.608725138771)) ;
#194675=CARTESIAN_POINT('Ctrl Pts',(-29.5178000156693,-13.4607154515732,
111.473552139375)) ;
#194676=CARTESIAN_POINT('Ctrl Pts',(-29.7125058569765,-13.4607154515732,
111.39418874148)) ;
#194677=CARTESIAN_POINT('Ctrl Pts',(-29.9214770342181,-13.4607154515732,
111.374286592167)) ;
#194678=CARTESIAN_POINT('Ctrl Pts',(-30.129031067933,-13.4607154515732,
111.417939881308)) ;
#194679=CARTESIAN_POINT('Ctrl Pts',(-30.3108273632114,-13.4607154515732,
111.522718871897)) ;
#194680=CARTESIAN_POINT('Ctrl Pts',(-30.4475054824147,-13.4607154515732,
111.674400413727)) ;
#194681=CARTESIAN_POINT('Ctrl Pts',(-30.5306819470581,-13.4607154515732,
111.859696163125)) ;
#194682=CARTESIAN_POINT('Ctrl Pts',(-30.5515845507338,-13.4607154515732,
112.065598309889)) ;
#194683=CARTESIAN_POINT('Ctrl Pts',(-30.505144819815,-13.4607154515732,
112.268886698136)) ;
#194684=CARTESIAN_POINT('Ctrl Pts',(-30.3992903014189,-13.4607154515732,
112.446856086907)) ;
#194685=CARTESIAN_POINT('Ctrl Pts',(-30.2443913742949,-13.4607154515732,
112.587215246961)) ;
#194686=CARTESIAN_POINT('Ctrl Pts',(-30.0504246992742,-13.4607154515732,
112.677419162906)) ;
#194687=CARTESIAN_POINT('Ctrl Pts',(-29.8384424605617,-13.4607154515732,
112.704782293005)) ;
#194688=CARTESIAN_POINT('Ctrl Pts',(-29.7003053480643,-13.4607154515732,
112.680623972109)) ;
#194689=CARTESIAN_POINT('Ctrl Pts',(-29.6364905070076,-13.4607154515732,
112.659288401873)) ;
#194690=CARTESIAN_POINT('Ctrl Pts',(-29.1967685926162,-13.4607154515732,
111.985309186393)) ;
#194691=CARTESIAN_POINT('Ctrl Pts',(-29.20372433272,-13.4607154515732,111.919496169812)) ;
#194692=CARTESIAN_POINT('Ctrl Pts',(-29.2391616569514,-13.4607154515732,
111.786249874406)) ;
#194693=CARTESIAN_POINT('Ctrl Pts',(-29.3531737828725,-13.4607154515732,
111.608725138771)) ;
#194694=CARTESIAN_POINT('Ctrl Pts',(-29.5178000156693,-13.4607154515732,
111.473552139375)) ;
#194695=CARTESIAN_POINT('Ctrl Pts',(-29.7125058569765,-13.4607154515732,
111.39418874148)) ;
#194696=CARTESIAN_POINT('Ctrl Pts',(-29.9214770342181,-13.4607154515732,
111.374286592167)) ;
#194697=CARTESIAN_POINT('Ctrl Pts',(-30.129031067933,-13.4607154515732,
111.417939881308)) ;
#194698=CARTESIAN_POINT('Ctrl Pts',(-30.3108273632114,-13.4607154515732,
111.522718871897)) ;
#194699=CARTESIAN_POINT('Ctrl Pts',(-30.4475054824147,-13.4607154515732,
111.674400413727)) ;
#194700=CARTESIAN_POINT('Ctrl Pts',(-30.5306819470581,-13.4607154515732,
111.859696163125)) ;
#194701=CARTESIAN_POINT('Ctrl Pts',(-30.5515845507338,-13.4607154515732,
112.065598309889)) ;
#194702=CARTESIAN_POINT('Ctrl Pts',(-30.505144819815,-13.4607154515732,
112.268886698136)) ;
#194703=CARTESIAN_POINT('Ctrl Pts',(-30.3992903014189,-13.4607154515732,
112.446856086907)) ;
#194704=CARTESIAN_POINT('Ctrl Pts',(-30.2443913742949,-13.4607154515732,
112.587215246961)) ;
#194705=CARTESIAN_POINT('Ctrl Pts',(-30.0504246992742,-13.4607154515732,
112.677419162906)) ;
#194706=CARTESIAN_POINT('Ctrl Pts',(-29.8384424605617,-13.4607154515732,
112.704782293005)) ;
#194707=CARTESIAN_POINT('Ctrl Pts',(-29.7003053480643,-13.4607154515732,
112.680623972109)) ;
#194708=CARTESIAN_POINT('Ctrl Pts',(-29.6364905070076,-13.4607154515732,
112.659288401873)) ;
#194709=CARTESIAN_POINT('Origin',(-17.8642992765666,-11.5234495205728,116.376494196106)) ;
#194710=CARTESIAN_POINT('Origin',(-17.6291851847899,-11.5234495205728,115.660374608073)) ;
#196737=UNCERTAINTY_MEASURE_WITH_UNIT(LENGTH_MEASURE(0.01),#196742,
'DISTANCE_ACCURACY_VALUE',
'Maximum model space distance between geometric entities at asserted c
onnectivities') ;
#196738=UNCERTAINTY_MEASURE_WITH_UNIT(LENGTH_MEASURE(0.01),#196742,
'DISTANCE_ACCURACY_VALUE',
'Maximum model space distance between geometric entities at asserted c
onnectivities') ;
#196740=(
GEOMETRIC_REPRESENTATION_CONTEXT(3)
GLOBAL_UNCERTAINTY_ASSIGNED_CONTEXT((#196737))
GLOBAL_UNIT_ASSIGNED_CONTEXT((#196742,#196744,#196745))
REPRESENTATION_CONTEXT('','3D')
) ;
#196741=(
GEOMETRIC_REPRESENTATION_CONTEXT(3)
GLOBAL_UNCERTAINTY_ASSIGNED_CONTEXT((#196738))
GLOBAL_UNIT_ASSIGNED_CONTEXT((#196742,#196744,#196745))
REPRESENTATION_CONTEXT('','3D')
) ;
#196742=(
LENGTH_UNIT()
NAMED_UNIT(*)
SI_UNIT(.MILLI.,.METRE.)
) ;
#196744=(
NAMED_UNIT(*)
PLANE_ANGLE_UNIT()
SI_UNIT($,.RADIAN.)
) ;
#196745=(
NAMED_UNIT(*)
SI_UNIT($,.STERADIAN.)
SOLID_ANGLE_UNIT()
) ;
#196753=PRODUCT_DEFINITION_CONTEXT('part definition',#196761,'design') ;
#196761=APPLICATION_CONTEXT(
'Core Data for Automotive Mechanical Design Process') ;
#196762=PRODUCT_CONTEXT('part definition',#196761,'mechanical') ;
#196765=PRESENTATION_STYLE_ASSIGNMENT((#196767)) ;
#196767=SURFACE_STYLE_USAGE(.BOTH.,#196769) ;
#196769=SURFACE_SIDE_STYLE('',(#196771)) ;
#196771=SURFACE_STYLE_FILL_AREA(#196773) ;
#196773=FILL_AREA_STYLE('Steel - Satin',(#196775)) ;
#196775=FILL_AREA_STYLE_COLOUR('Steel - Satin',#196777) ;
#196777=COLOUR_RGB('Steel - Satin', 0.09019608, 0.27058824, 0.51372549) ;
#197139=CARTESIAN_POINT ( '', ( 0.0, 0.0, 0.0 ) ) ;
#197140=DIRECTION ( '', ( 0.0, 0.0, 1.0 ) ) ;
#197141=DIRECTION ( '', ( 1.0, 0.0, 0.0 ) ) ;
#197142=AXIS2_PLACEMENT_3D ( '', #197139, #197140, #197141 ) ;
#197143=ADVANCED_BREP_SHAPE_REPRESENTATION ( 'Exit Return Spring', ( #353, #197142, #197153, #197433 ), #196740 ) ;
#197144=PRODUCT( 'Exit Return Spring', 'Exit Return Spring', '', ( #196762 ) ) ;
#197145=PRODUCT_DEFINITION_FORMATION ( '', '', #197144 ) ;
#197146=PRODUCT_DEFINITION( 'Exit Return Spring', 'Exit Return Spring', #197145, #196753 ) ;
#197147=PRODUCT_DEFINITION_SHAPE ( '', '', #197146 ) ;
#197148=SHAPE_DEFINITION_REPRESENTATION ( #197147, #197143 ) ;
#197150=CARTESIAN_POINT ( '', ( 0.0, 0.0, 0.0 ) ) ;
#197151=DIRECTION ( '', ( 0.0, 0.0, 1.0 ) ) ;
#197152=DIRECTION ( '', ( 1.0, 0.0, 0.0 ) ) ;
#197153=AXIS2_PLACEMENT_3D ( '', #197150, #197151, #197152 ) ;
#197430=CARTESIAN_POINT ( '', ( 0.0, 0.0, 0.0 ) ) ;
#197431=DIRECTION ( '', ( 0.0, 0.0, 1.0 ) ) ;
#197432=DIRECTION ( '', ( 1.0, 0.0, 0.0 ) ) ;
#197433=AXIS2_PLACEMENT_3D ( '', #197430, #197431, #197432 ) ;
ENDSEC;
END-ISO-10303-21;
